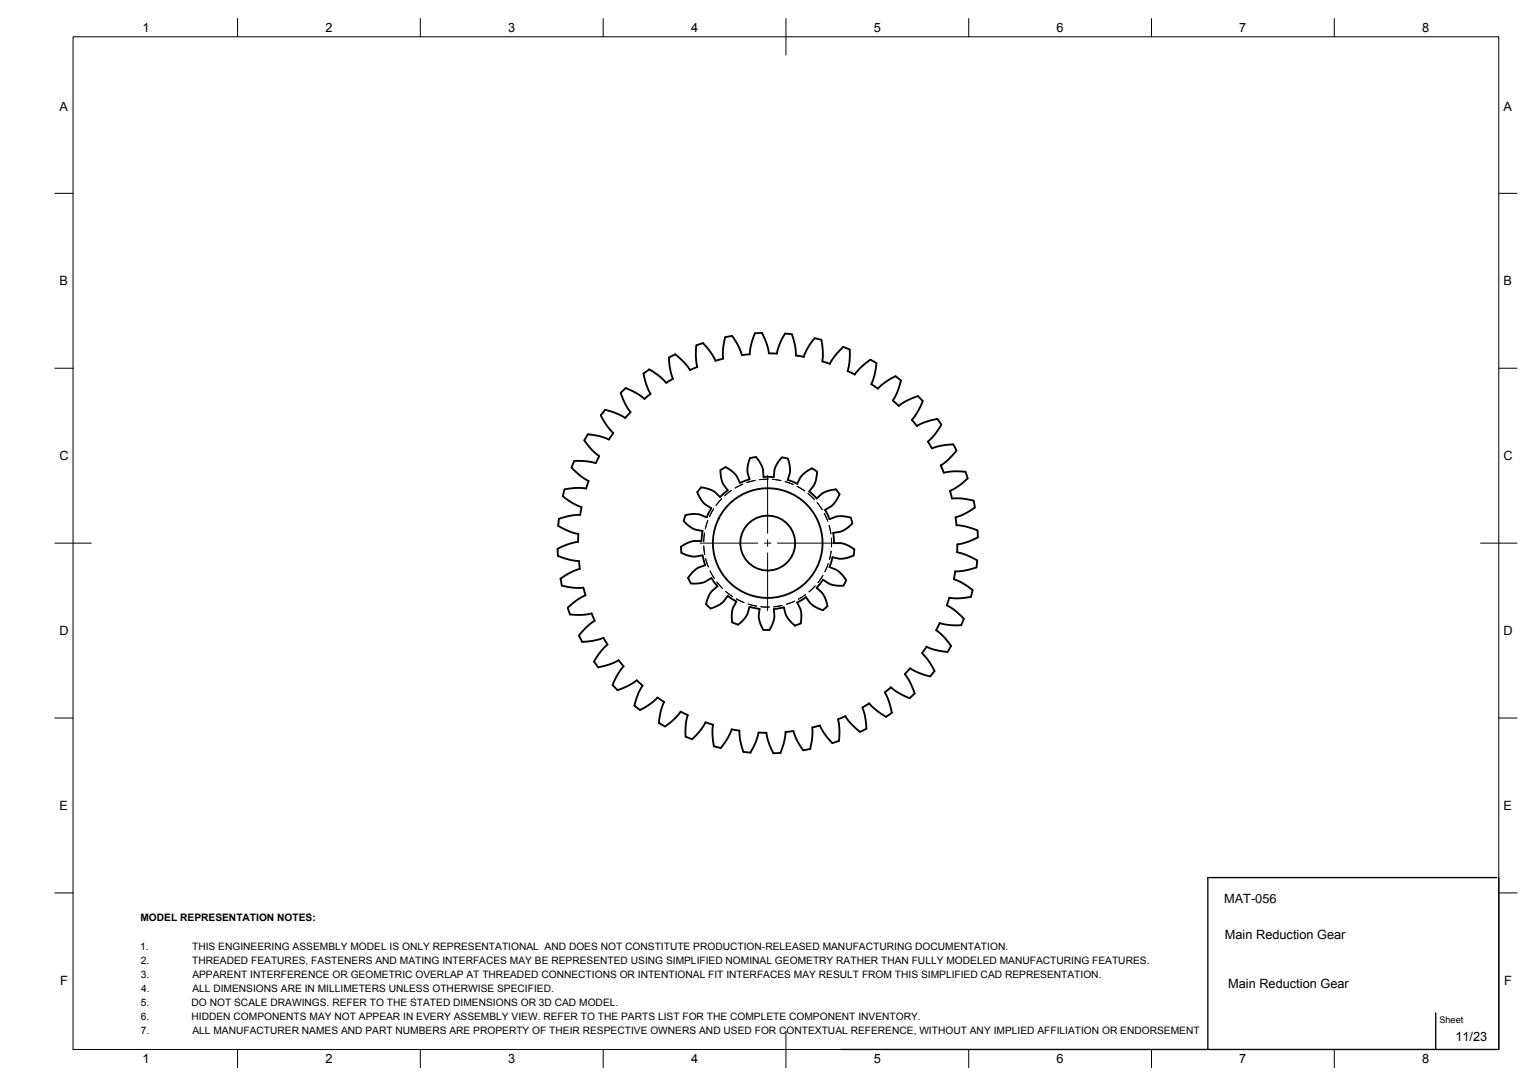
ISO-10303-21;
HEADER;
/* Generated by software containing ST-Developer
 * from STEP Tools, Inc. (www.steptools.com) 
 */

FILE_DESCRIPTION(
/* description */ (''),
/* implementation_level */ '2;1');

FILE_NAME(
/* name */ 'Main Reduction Gear.step',
/* time_stamp */ '2026-10-28T16:47:13+01:00',
/* author */ (''),
/* organization */ (''),
/* preprocessor_version */ 'ST-DEVELOPER v20.2',
/* originating_system */ 'Autodesk Translation Framework v15.17.0.0',
/* authorisation */ '');

FILE_SCHEMA (('AUTOMOTIVE_DESIGN { 1 0 10303 214 3 1 1 }'));
ENDSEC;

DATA;
#10=MECHANICAL_DESIGN_GEOMETRIC_PRESENTATION_REPRESENTATION('',(#4576,#4577),#459242);
#4412=SHAPE_REPRESENTATION_RELATIONSHIP('SRR','None',#459337,#4433);
#4433=ADVANCED_BREP_SHAPE_REPRESENTATION('',(#4456,#4457),#459226);
#4456=MANIFOLD_SOLID_BREP('Gear44',#94634);
#4457=MANIFOLD_SOLID_BREP('Gear17',#94635);
#4576=STYLED_ITEM('',(#459519),#4456);
#4577=STYLED_ITEM('',(#459519),#4457);
#5187=FACE_BOUND('',#13996,.T.);
#5188=FACE_BOUND('',#14004,.T.);
#5189=FACE_BOUND('',#14010,.T.);
#5190=FACE_BOUND('',#14013,.T.);
#5191=FACE_BOUND('',#14066,.T.);
#5192=FACE_BOUND('',#14120,.T.);
#5608=PLANE('',#98688);
#5609=PLANE('',#98701);
#5610=PLANE('',#98708);
#5611=PLANE('',#98709);
#5612=PLANE('',#98710);
#5613=PLANE('',#98749);
#5614=PLANE('',#98752);
#5615=PLANE('',#98755);
#5616=PLANE('',#98758);
#5617=PLANE('',#98761);
#5618=PLANE('',#98764);
#5619=PLANE('',#98767);
#5620=PLANE('',#98770);
#5621=PLANE('',#98773);
#5622=PLANE('',#98776);
#5623=PLANE('',#98779);
#5624=PLANE('',#98782);
#5625=PLANE('',#98785);
#5626=PLANE('',#98788);
#5627=PLANE('',#98791);
#5628=PLANE('',#98794);
#5629=PLANE('',#98797);
#5630=PLANE('',#98800);
#5631=PLANE('',#98801);
#5632=PLANE('',#98819);
#5633=PLANE('',#98821);
#5634=PLANE('',#98823);
#5635=PLANE('',#98825);
#5636=PLANE('',#98826);
#5637=PLANE('',#98828);
#5638=PLANE('',#98829);
#5639=PLANE('',#98832);
#5640=PLANE('',#98834);
#5641=PLANE('',#98837);
#5642=PLANE('',#98838);
#5643=PLANE('',#98840);
#5644=PLANE('',#98841);
#5645=PLANE('',#98844);
#5646=PLANE('',#98846);
#5647=PLANE('',#98849);
#5648=PLANE('',#98850);
#5649=PLANE('',#98855);
#6215=B_SPLINE_SURFACE_WITH_KNOTS('',5,1,((#153547,#153548),(#153549,#153550),
(#153551,#153552),(#153553,#153554),(#153555,#153556),(#153557,#153558),
(#153559,#153560),(#153561,#153562),(#153563,#153564),(#153565,#153566),
(#153567,#153568),(#153569,#153570),(#153571,#153572),(#153573,#153574),
(#153575,#153576),(#153577,#153578),(#153579,#153580),(#153581,#153582),
(#153583,#153584),(#153585,#153586),(#153587,#153588),(#153589,#153590),
(#153591,#153592),(#153593,#153594),(#153595,#153596),(#153597,#153598),
(#153599,#153600),(#153601,#153602),(#153603,#153604),(#153605,#153606),
(#153607,#153608),(#153609,#153610),(#153611,#153612),(#153613,#153614),
(#153615,#153616),(#153617,#153618),(#153619,#153620),(#153621,#153622),
(#153623,#153624),(#153625,#153626),(#153627,#153628),(#153629,#153630),
(#153631,#153632),(#153633,#153634),(#153635,#153636),(#153637,#153638),
(#153639,#153640),(#153641,#153642),(#153643,#153644),(#153645,#153646),
(#153647,#153648),(#153649,#153650),(#153651,#153652),(#153653,#153654),
(#153655,#153656),(#153657,#153658),(#153659,#153660),(#153661,#153662),
(#153663,#153664),(#153665,#153666),(#153667,#153668),(#153669,#153670),
(#153671,#153672),(#153673,#153674),(#153675,#153676),(#153677,#153678),
(#153679,#153680),(#153681,#153682),(#153683,#153684),(#153685,#153686),
(#153687,#153688),(#153689,#153690),(#153691,#153692),(#153693,#153694),
(#153695,#153696),(#153697,#153698),(#153699,#153700),(#153701,#153702),
(#153703,#153704),(#153705,#153706),(#153707,#153708),(#153709,#153710),
(#153711,#153712),(#153713,#153714),(#153715,#153716),(#153717,#153718),
(#153719,#153720),(#153721,#153722),(#153723,#153724),(#153725,#153726),
(#153727,#153728),(#153729,#153730),(#153731,#153732),(#153733,#153734),
(#153735,#153736),(#153737,#153738),(#153739,#153740),(#153741,#153742),
(#153743,#153744),(#153745,#153746),(#153747,#153748),(#153749,#153750),
(#153751,#153752),(#153753,#153754),(#153755,#153756),(#153757,#153758),
(#153759,#153760),(#153761,#153762),(#153763,#153764),(#153765,#153766),
(#153767,#153768),(#153769,#153770),(#153771,#153772),(#153773,#153774),
(#153775,#153776),(#153777,#153778),(#153779,#153780),(#153781,#153782),
(#153783,#153784),(#153785,#153786),(#153787,#153788),(#153789,#153790),
(#153791,#153792),(#153793,#153794),(#153795,#153796),(#153797,#153798),
(#153799,#153800),(#153801,#153802),(#153803,#153804),(#153805,#153806),
(#153807,#153808),(#153809,#153810),(#153811,#153812),(#153813,#153814),
(#153815,#153816),(#153817,#153818),(#153819,#153820),(#153821,#153822),
(#153823,#153824),(#153825,#153826),(#153827,#153828),(#153829,#153830),
(#153831,#153832),(#153833,#153834),(#153835,#153836),(#153837,#153838),
(#153839,#153840),(#153841,#153842),(#153843,#153844),(#153845,#153846),
(#153847,#153848),(#153849,#153850),(#153851,#153852),(#153853,#153854),
(#153855,#153856),(#153857,#153858),(#153859,#153860),(#153861,#153862),
(#153863,#153864),(#153865,#153866),(#153867,#153868),(#153869,#153870),
(#153871,#153872),(#153873,#153874),(#153875,#153876),(#153877,#153878),
(#153879,#153880),(#153881,#153882),(#153883,#153884),(#153885,#153886),
(#153887,#153888),(#153889,#153890),(#153891,#153892),(#153893,#153894),
(#153895,#153896),(#153897,#153898),(#153899,#153900),(#153901,#153902),
(#153903,#153904),(#153905,#153906),(#153907,#153908),(#153909,#153910),
(#153911,#153912),(#153913,#153914),(#153915,#153916),(#153917,#153918),
(#153919,#153920),(#153921,#153922),(#153923,#153924),(#153925,#153926),
(#153927,#153928),(#153929,#153930),(#153931,#153932),(#153933,#153934),
(#153935,#153936),(#153937,#153938),(#153939,#153940),(#153941,#153942),
(#153943,#153944),(#153945,#153946),(#153947,#153948),(#153949,#153950),
(#153951,#153952),(#153953,#153954),(#153955,#153956),(#153957,#153958),
(#153959,#153960),(#153961,#153962),(#153963,#153964),(#153965,#153966),
(#153967,#153968),(#153969,#153970),(#153971,#153972),(#153973,#153974),
(#153975,#153976),(#153977,#153978),(#153979,#153980),(#153981,#153982),
(#153983,#153984),(#153985,#153986),(#153987,#153988),(#153989,#153990),
(#153991,#153992),(#153993,#153994),(#153995,#153996),(#153997,#153998),
(#153999,#154000),(#154001,#154002),(#154003,#154004),(#154005,#154006),
(#154007,#154008),(#154009,#154010),(#154011,#154012),(#154013,#154014),
(#154015,#154016),(#154017,#154018),(#154019,#154020),(#154021,#154022),
(#154023,#154024),(#154025,#154026),(#154027,#154028),(#154029,#154030),
(#154031,#154032),(#154033,#154034),(#154035,#154036),(#154037,#154038),
(#154039,#154040),(#154041,#154042),(#154043,#154044),(#154045,#154046),
(#154047,#154048),(#154049,#154050),(#154051,#154052),(#154053,#154054),
(#154055,#154056),(#154057,#154058),(#154059,#154060),(#154061,#154062),
(#154063,#154064),(#154065,#154066),(#154067,#154068),(#154069,#154070),
(#154071,#154072),(#154073,#154074),(#154075,#154076),(#154077,#154078),
(#154079,#154080),(#154081,#154082),(#154083,#154084),(#154085,#154086),
(#154087,#154088),(#154089,#154090),(#154091,#154092),(#154093,#154094),
(#154095,#154096),(#154097,#154098),(#154099,#154100),(#154101,#154102),
(#154103,#154104),(#154105,#154106),(#154107,#154108),(#154109,#154110),
(#154111,#154112),(#154113,#154114),(#154115,#154116),(#154117,#154118),
(#154119,#154120),(#154121,#154122),(#154123,#154124),(#154125,#154126),
(#154127,#154128),(#154129,#154130),(#154131,#154132),(#154133,#154134),
(#154135,#154136),(#154137,#154138),(#154139,#154140),(#154141,#154142),
(#154143,#154144),(#154145,#154146),(#154147,#154148),(#154149,#154150),
(#154151,#154152),(#154153,#154154),(#154155,#154156),(#154157,#154158),
(#154159,#154160),(#154161,#154162),(#154163,#154164),(#154165,#154166),
(#154167,#154168),(#154169,#154170),(#154171,#154172),(#154173,#154174),
(#154175,#154176),(#154177,#154178),(#154179,#154180),(#154181,#154182),
(#154183,#154184),(#154185,#154186),(#154187,#154188),(#154189,#154190),
(#154191,#154192),(#154193,#154194),(#154195,#154196),(#154197,#154198),
(#154199,#154200),(#154201,#154202),(#154203,#154204),(#154205,#154206),
(#154207,#154208),(#154209,#154210),(#154211,#154212),(#154213,#154214),
(#154215,#154216),(#154217,#154218),(#154219,#154220),(#154221,#154222),
(#154223,#154224),(#154225,#154226),(#154227,#154228),(#154229,#154230),
(#154231,#154232),(#154233,#154234),(#154235,#154236),(#154237,#154238),
(#154239,#154240),(#154241,#154242),(#154243,#154244),(#154245,#154246),
(#154247,#154248),(#154249,#154250),(#154251,#154252),(#154253,#154254),
(#154255,#154256),(#154257,#154258),(#154259,#154260),(#154261,#154262),
(#154263,#154264),(#154265,#154266),(#154267,#154268),(#154269,#154270),
(#154271,#154272),(#154273,#154274),(#154275,#154276),(#154277,#154278),
(#154279,#154280),(#154281,#154282),(#154283,#154284),(#154285,#154286),
(#154287,#154288),(#154289,#154290),(#154291,#154292),(#154293,#154294),
(#154295,#154296),(#154297,#154298),(#154299,#154300),(#154301,#154302),
(#154303,#154304),(#154305,#154306),(#154307,#154308),(#154309,#154310),
(#154311,#154312),(#154313,#154314),(#154315,#154316),(#154317,#154318),
(#154319,#154320),(#154321,#154322),(#154323,#154324),(#154325,#154326),
(#154327,#154328),(#154329,#154330),(#154331,#154332),(#154333,#154334),
(#154335,#154336),(#154337,#154338),(#154339,#154340),(#154341,#154342),
(#154343,#154344),(#154345,#154346),(#154347,#154348),(#154349,#154350),
(#154351,#154352),(#154353,#154354),(#154355,#154356),(#154357,#154358),
(#154359,#154360),(#154361,#154362),(#154363,#154364),(#154365,#154366),
(#154367,#154368),(#154369,#154370),(#154371,#154372),(#154373,#154374),
(#154375,#154376),(#154377,#154378),(#154379,#154380),(#154381,#154382),
(#154383,#154384),(#154385,#154386),(#154387,#154388),(#154389,#154390),
(#154391,#154392),(#154393,#154394),(#154395,#154396),(#154397,#154398),
(#154399,#154400),(#154401,#154402),(#154403,#154404),(#154405,#154406),
(#154407,#154408),(#154409,#154410),(#154411,#154412),(#154413,#154414),
(#154415,#154416),(#154417,#154418),(#154419,#154420),(#154421,#154422),
(#154423,#154424),(#154425,#154426),(#154427,#154428),(#154429,#154430),
(#154431,#154432),(#154433,#154434),(#154435,#154436),(#154437,#154438),
(#154439,#154440),(#154441,#154442),(#154443,#154444),(#154445,#154446),
(#154447,#154448),(#154449,#154450),(#154451,#154452),(#154453,#154454),
(#154455,#154456),(#154457,#154458),(#154459,#154460),(#154461,#154462),
(#154463,#154464),(#154465,#154466),(#154467,#154468),(#154469,#154470),
(#154471,#154472),(#154473,#154474),(#154475,#154476),(#154477,#154478),
(#154479,#154480),(#154481,#154482),(#154483,#154484),(#154485,#154486),
(#154487,#154488),(#154489,#154490)),.UNSPECIFIED.,.F.,.F.,.F.,(6,1,1,1,
1,1,1,1,1,1,1,1,1,1,1,1,1,1,1,1,1,1,1,1,1,1,1,1,1,1,1,1,1,1,1,1,1,1,1,1,
1,1,1,1,1,1,1,1,1,1,1,1,1,1,1,1,1,1,1,1,1,1,1,1,1,1,1,1,1,1,1,1,1,1,1,1,
1,1,1,1,1,1,1,1,1,1,1,1,1,1,1,1,1,1,1,1,1,1,1,1,1,1,1,1,1,1,1,1,1,1,1,1,
1,1,1,1,1,1,1,1,1,1,1,1,1,1,1,1,1,1,1,1,1,1,1,1,1,1,1,1,1,1,1,1,1,1,1,1,
1,1,1,1,1,1,1,1,1,1,1,1,1,1,1,1,1,1,1,1,1,1,1,1,1,1,1,1,1,1,1,1,1,1,1,1,
1,1,1,1,1,1,1,1,1,1,1,1,1,1,1,1,1,1,1,1,1,1,1,1,1,1,1,1,1,1,1,1,1,1,1,1,
1,1,1,1,1,1,1,1,1,1,1,1,1,1,1,1,1,1,1,1,1,1,1,1,1,1,1,1,1,1,1,1,1,1,1,1,
1,1,1,1,1,1,1,1,1,1,1,1,1,1,1,1,1,1,1,1,1,1,1,1,1,1,1,1,1,1,1,1,1,1,1,1,
1,1,1,1,1,1,1,1,1,1,1,1,1,1,1,1,1,1,1,1,1,1,1,1,1,1,1,1,1,1,1,1,1,1,1,1,
1,1,1,1,1,1,1,1,1,1,1,1,1,1,1,1,1,1,1,1,1,1,1,1,1,1,1,1,1,1,1,1,1,1,1,1,
1,1,1,1,1,1,1,1,1,1,1,1,1,1,1,1,1,1,1,1,1,1,1,1,1,1,1,1,1,1,1,1,1,1,1,1,
1,1,1,1,1,1,1,1,1,1,1,1,1,1,1,1,1,1,1,1,1,1,1,1,1,1,1,1,1,1,1,1,1,1,1,1,
1,1,1,1,1,1,1,1,1,1,1,1,1,1,1,1,1,1,1,1,1,1,1,1,1,1,1,1,1,1,1,6),(2,2),
(0.143172103,0.144954128,0.146788991,0.148623853,0.150458716,0.152293578,
0.15412844,0.155963303,0.157798165,0.159633028,0.16146789,0.163302752,0.165137615,
0.166972477,0.168807339,0.170642202,0.172477064,0.174311927,0.176146789,
0.177981651,0.179816514,0.181651376,0.183486239,0.185321101,0.187155963,
0.188990826,0.190825688,0.19266055,0.194495413,0.196330275,0.198165138,
0.2,0.201834862,0.203669725,0.205504587,0.20733945,0.209174312,0.211009174,
0.212844037,0.214678899,0.216513761,0.218348624,0.220183486,0.222018349,
0.223853211,0.225688073,0.227522936,0.229357798,0.231192661,0.233027523,
0.234862385,0.236697248,0.23853211,0.240366972,0.242201835,0.244036697,
0.24587156,0.247706422,0.249541284,0.251376147,0.253211009,0.255045872,
0.256880734,0.258715596,0.260550459,0.262385321,0.264220183,0.266055046,
0.267889908,0.269724771,0.271559633,0.273394495,0.275229358,0.27706422,
0.278899083,0.280733945,0.282568807,0.28440367,0.286238532,0.288073394,
0.289908257,0.291743119,0.293577982,0.295412844,0.297247706,0.299082569,
0.300917431,0.302752294,0.304587156,0.306422018,0.308256881,0.310091743,
0.311926606,0.313761468,0.31559633,0.317431193,0.319266055,0.321100917,
0.32293578,0.324770642,0.326605505,0.328440367,0.330275229,0.332110092,
0.333944954,0.335779817,0.337614679,0.339449541,0.341284404,0.343119266,
0.344954128,0.346788991,0.348623853,0.350458716,0.352293578,0.35412844,
0.355963303,0.357798165,0.359633028,0.36146789,0.363302752,0.365137615,
0.366972477,0.368807339,0.370642202,0.372477064,0.374311927,0.376146789,
0.377981651,0.379816514,0.381651376,0.383486239,0.385321101,0.387155963,
0.388990826,0.390825688,0.39266055,0.394495413,0.396330275,0.398165138,
0.4,0.401834862,0.403669725,0.405504587,0.40733945,0.409174312,0.411009174,
0.412844037,0.414678899,0.416513761,0.418348624,0.420183486,0.422018349,
0.423853211,0.425688073,0.427522936,0.429357798,0.431192661,0.433027523,
0.434862385,0.436697248,0.43853211,0.440366972,0.442201835,0.444036697,
0.44587156,0.447706422,0.449541284,0.451376147,0.453211009,0.455045872,
0.456880734,0.458715596,0.460550459,0.462385321,0.464220183,0.466055046,
0.467889908,0.469724771,0.471559633,0.473394495,0.475229358,0.47706422,
0.478899083,0.480733945,0.482568807,0.48440367,0.486238532,0.488073394,
0.489908257,0.491743119,0.493577982,0.495412844,0.497247706,0.499082569,
0.500917431,0.502752294,0.504587156,0.506422018,0.508256881,0.510091743,
0.511926606,0.513761468,0.51559633,0.517431193,0.519266055,0.521100917,
0.52293578,0.524770642,0.526605505,0.528440367,0.530275229,0.532110092,
0.533944954,0.535779817,0.537614679,0.539449541,0.541284404,0.543119266,
0.544954128,0.546788991,0.548623853,0.550458716,0.552293578,0.55412844,
0.555963303,0.557798165,0.559633028,0.56146789,0.563302752,0.565137615,
0.566972477,0.568807339,0.570642202,0.572477064,0.574311927,0.576146789,
0.577981651,0.579816514,0.581651376,0.583486239,0.585321101,0.587155963,
0.588990826,0.590825688,0.59266055,0.594495413,0.596330275,0.598165138,
0.6,0.601834862,0.603669725,0.605504587,0.60733945,0.609174312,0.611009174,
0.612844037,0.614678899,0.616513761,0.618348624,0.620183486,0.622018349,
0.623853211,0.625688073,0.627522936,0.629357798,0.631192661,0.633027523,
0.634862385,0.636697248,0.63853211,0.640366972,0.642201835,0.644036697,
0.64587156,0.647706422,0.649541284,0.651376147,0.653211009,0.655045872,
0.656880734,0.658715596,0.660550459,0.662385321,0.664220183,0.666055046,
0.667889908,0.669724771,0.671559633,0.673394495,0.675229358,0.67706422,
0.678899083,0.680733945,0.682568807,0.68440367,0.686238532,0.688073394,
0.689908257,0.691743119,0.693577982,0.695412844,0.697247706,0.699082569,
0.700917431,0.702752294,0.704587156,0.706422018,0.708256881,0.710091743,
0.711926606,0.713761468,0.71559633,0.717431193,0.719266055,0.721100917,
0.72293578,0.724770642,0.726605505,0.728440367,0.730275229,0.732110092,
0.733944954,0.735779817,0.737614679,0.739449541,0.741284404,0.743119266,
0.744954128,0.746788991,0.748623853,0.750458716,0.752293578,0.75412844,
0.755963303,0.757798165,0.759633028,0.76146789,0.763302752,0.765137615,
0.766972477,0.768807339,0.770642202,0.772477064,0.774311927,0.776146789,
0.777981651,0.779816514,0.781651376,0.783486239,0.785321101,0.787155963,
0.788990826,0.790825688,0.79266055,0.794495413,0.796330275,0.798165138,
0.8,0.801834862,0.803669725,0.805504587,0.80733945,0.809174312,0.811009174,
0.812844037,0.814678899,0.816513761,0.818348624,0.820183486,0.822018349,
0.823853211,0.825688073,0.827522936,0.829357798,0.831192661,0.833027523,
0.834862385,0.836697248,0.83853211,0.840366972,0.842201835,0.844036697,
0.84587156,0.847706422,0.849541284,0.851376147,0.853211009,0.855045872,
0.856880734,0.858715596,0.860550459,0.862385321,0.864220183,0.866055046,
0.867889908,0.869724771,0.871559633,0.873394495,0.875229358,0.87706422,
0.878899083,0.880733945,0.882568807,0.88440367,0.886238532,0.888073394,
0.889908257,0.891743119,0.893577982,0.895412844,0.897247706,0.899082569,
0.900917431,0.902752294,0.904587156,0.906422018,0.908256881,0.910091743,
0.911926606,0.913761468,0.91559633,0.917431193,0.919266055,0.921100917,
0.92293578,0.924770642,0.926605505,0.928440367,0.930275229,0.932110092,
0.933944954,0.935779817,0.937614679,0.939449541,0.941284404,0.943119266,
0.944954128,0.946788991,0.948623853,0.950458716,0.952293578,0.95412844,
0.955963303,0.957798165,0.959633028,0.96146789,0.963302752,0.965137615,
0.966972477,0.968807339,0.970642202,0.972477064,0.974311927,0.976146789,
0.977981651,0.979816514,0.981651376,0.983486239,0.985321101,0.987155963,
0.988990826,0.990825688,0.99266055,0.994495413,0.996330275,0.998165138,
1.),(0.,0.36),.UNSPECIFIED.);
#6216=B_SPLINE_SURFACE_WITH_KNOTS('',5,1,((#155436,#155437),(#155438,#155439),
(#155440,#155441),(#155442,#155443),(#155444,#155445),(#155446,#155447),
(#155448,#155449),(#155450,#155451),(#155452,#155453),(#155454,#155455),
(#155456,#155457),(#155458,#155459),(#155460,#155461),(#155462,#155463),
(#155464,#155465),(#155466,#155467),(#155468,#155469),(#155470,#155471),
(#155472,#155473),(#155474,#155475),(#155476,#155477),(#155478,#155479),
(#155480,#155481),(#155482,#155483),(#155484,#155485),(#155486,#155487),
(#155488,#155489),(#155490,#155491),(#155492,#155493),(#155494,#155495),
(#155496,#155497),(#155498,#155499),(#155500,#155501),(#155502,#155503),
(#155504,#155505),(#155506,#155507),(#155508,#155509),(#155510,#155511),
(#155512,#155513),(#155514,#155515),(#155516,#155517),(#155518,#155519),
(#155520,#155521),(#155522,#155523),(#155524,#155525),(#155526,#155527),
(#155528,#155529),(#155530,#155531),(#155532,#155533),(#155534,#155535),
(#155536,#155537),(#155538,#155539),(#155540,#155541),(#155542,#155543),
(#155544,#155545),(#155546,#155547),(#155548,#155549),(#155550,#155551),
(#155552,#155553),(#155554,#155555),(#155556,#155557),(#155558,#155559),
(#155560,#155561),(#155562,#155563),(#155564,#155565),(#155566,#155567),
(#155568,#155569),(#155570,#155571),(#155572,#155573),(#155574,#155575),
(#155576,#155577),(#155578,#155579),(#155580,#155581),(#155582,#155583),
(#155584,#155585),(#155586,#155587),(#155588,#155589),(#155590,#155591),
(#155592,#155593),(#155594,#155595),(#155596,#155597),(#155598,#155599),
(#155600,#155601),(#155602,#155603),(#155604,#155605),(#155606,#155607),
(#155608,#155609),(#155610,#155611),(#155612,#155613),(#155614,#155615),
(#155616,#155617),(#155618,#155619),(#155620,#155621),(#155622,#155623),
(#155624,#155625),(#155626,#155627),(#155628,#155629),(#155630,#155631),
(#155632,#155633),(#155634,#155635),(#155636,#155637),(#155638,#155639),
(#155640,#155641),(#155642,#155643),(#155644,#155645),(#155646,#155647),
(#155648,#155649),(#155650,#155651),(#155652,#155653),(#155654,#155655),
(#155656,#155657),(#155658,#155659),(#155660,#155661),(#155662,#155663),
(#155664,#155665),(#155666,#155667),(#155668,#155669),(#155670,#155671),
(#155672,#155673),(#155674,#155675),(#155676,#155677),(#155678,#155679),
(#155680,#155681),(#155682,#155683),(#155684,#155685),(#155686,#155687),
(#155688,#155689),(#155690,#155691),(#155692,#155693),(#155694,#155695),
(#155696,#155697),(#155698,#155699),(#155700,#155701),(#155702,#155703),
(#155704,#155705),(#155706,#155707),(#155708,#155709),(#155710,#155711),
(#155712,#155713),(#155714,#155715),(#155716,#155717),(#155718,#155719),
(#155720,#155721),(#155722,#155723),(#155724,#155725),(#155726,#155727),
(#155728,#155729),(#155730,#155731),(#155732,#155733),(#155734,#155735),
(#155736,#155737),(#155738,#155739),(#155740,#155741),(#155742,#155743),
(#155744,#155745),(#155746,#155747),(#155748,#155749),(#155750,#155751),
(#155752,#155753),(#155754,#155755),(#155756,#155757),(#155758,#155759),
(#155760,#155761),(#155762,#155763),(#155764,#155765),(#155766,#155767),
(#155768,#155769),(#155770,#155771),(#155772,#155773),(#155774,#155775),
(#155776,#155777),(#155778,#155779),(#155780,#155781),(#155782,#155783),
(#155784,#155785),(#155786,#155787),(#155788,#155789),(#155790,#155791),
(#155792,#155793),(#155794,#155795),(#155796,#155797),(#155798,#155799),
(#155800,#155801),(#155802,#155803),(#155804,#155805),(#155806,#155807),
(#155808,#155809),(#155810,#155811),(#155812,#155813),(#155814,#155815),
(#155816,#155817),(#155818,#155819),(#155820,#155821),(#155822,#155823),
(#155824,#155825),(#155826,#155827),(#155828,#155829),(#155830,#155831),
(#155832,#155833),(#155834,#155835),(#155836,#155837),(#155838,#155839),
(#155840,#155841),(#155842,#155843),(#155844,#155845),(#155846,#155847),
(#155848,#155849),(#155850,#155851),(#155852,#155853),(#155854,#155855),
(#155856,#155857),(#155858,#155859),(#155860,#155861),(#155862,#155863),
(#155864,#155865),(#155866,#155867),(#155868,#155869),(#155870,#155871),
(#155872,#155873),(#155874,#155875),(#155876,#155877),(#155878,#155879),
(#155880,#155881),(#155882,#155883),(#155884,#155885),(#155886,#155887),
(#155888,#155889),(#155890,#155891),(#155892,#155893),(#155894,#155895),
(#155896,#155897),(#155898,#155899),(#155900,#155901),(#155902,#155903),
(#155904,#155905),(#155906,#155907),(#155908,#155909),(#155910,#155911),
(#155912,#155913),(#155914,#155915),(#155916,#155917),(#155918,#155919),
(#155920,#155921),(#155922,#155923),(#155924,#155925),(#155926,#155927),
(#155928,#155929),(#155930,#155931),(#155932,#155933),(#155934,#155935),
(#155936,#155937),(#155938,#155939),(#155940,#155941),(#155942,#155943),
(#155944,#155945),(#155946,#155947),(#155948,#155949),(#155950,#155951),
(#155952,#155953),(#155954,#155955),(#155956,#155957),(#155958,#155959),
(#155960,#155961),(#155962,#155963),(#155964,#155965),(#155966,#155967),
(#155968,#155969),(#155970,#155971),(#155972,#155973),(#155974,#155975),
(#155976,#155977),(#155978,#155979),(#155980,#155981),(#155982,#155983),
(#155984,#155985),(#155986,#155987),(#155988,#155989),(#155990,#155991),
(#155992,#155993),(#155994,#155995),(#155996,#155997),(#155998,#155999),
(#156000,#156001),(#156002,#156003),(#156004,#156005),(#156006,#156007),
(#156008,#156009),(#156010,#156011),(#156012,#156013),(#156014,#156015),
(#156016,#156017),(#156018,#156019),(#156020,#156021),(#156022,#156023),
(#156024,#156025),(#156026,#156027),(#156028,#156029),(#156030,#156031),
(#156032,#156033),(#156034,#156035),(#156036,#156037),(#156038,#156039),
(#156040,#156041),(#156042,#156043),(#156044,#156045),(#156046,#156047),
(#156048,#156049),(#156050,#156051),(#156052,#156053),(#156054,#156055),
(#156056,#156057),(#156058,#156059),(#156060,#156061),(#156062,#156063),
(#156064,#156065),(#156066,#156067),(#156068,#156069),(#156070,#156071),
(#156072,#156073),(#156074,#156075),(#156076,#156077),(#156078,#156079),
(#156080,#156081),(#156082,#156083),(#156084,#156085),(#156086,#156087),
(#156088,#156089),(#156090,#156091),(#156092,#156093),(#156094,#156095),
(#156096,#156097),(#156098,#156099),(#156100,#156101),(#156102,#156103),
(#156104,#156105),(#156106,#156107),(#156108,#156109),(#156110,#156111),
(#156112,#156113),(#156114,#156115),(#156116,#156117),(#156118,#156119),
(#156120,#156121),(#156122,#156123),(#156124,#156125),(#156126,#156127),
(#156128,#156129),(#156130,#156131),(#156132,#156133),(#156134,#156135),
(#156136,#156137),(#156138,#156139),(#156140,#156141),(#156142,#156143),
(#156144,#156145),(#156146,#156147),(#156148,#156149),(#156150,#156151),
(#156152,#156153),(#156154,#156155),(#156156,#156157),(#156158,#156159),
(#156160,#156161),(#156162,#156163),(#156164,#156165),(#156166,#156167),
(#156168,#156169),(#156170,#156171),(#156172,#156173),(#156174,#156175),
(#156176,#156177),(#156178,#156179),(#156180,#156181),(#156182,#156183),
(#156184,#156185),(#156186,#156187),(#156188,#156189),(#156190,#156191),
(#156192,#156193),(#156194,#156195),(#156196,#156197),(#156198,#156199),
(#156200,#156201),(#156202,#156203),(#156204,#156205),(#156206,#156207),
(#156208,#156209),(#156210,#156211),(#156212,#156213),(#156214,#156215),
(#156216,#156217),(#156218,#156219),(#156220,#156221),(#156222,#156223),
(#156224,#156225),(#156226,#156227),(#156228,#156229),(#156230,#156231),
(#156232,#156233),(#156234,#156235),(#156236,#156237),(#156238,#156239),
(#156240,#156241),(#156242,#156243),(#156244,#156245),(#156246,#156247),
(#156248,#156249),(#156250,#156251),(#156252,#156253),(#156254,#156255),
(#156256,#156257),(#156258,#156259),(#156260,#156261),(#156262,#156263),
(#156264,#156265),(#156266,#156267),(#156268,#156269),(#156270,#156271),
(#156272,#156273),(#156274,#156275),(#156276,#156277),(#156278,#156279),
(#156280,#156281),(#156282,#156283),(#156284,#156285),(#156286,#156287),
(#156288,#156289),(#156290,#156291),(#156292,#156293),(#156294,#156295),
(#156296,#156297),(#156298,#156299),(#156300,#156301),(#156302,#156303),
(#156304,#156305),(#156306,#156307),(#156308,#156309),(#156310,#156311),
(#156312,#156313),(#156314,#156315),(#156316,#156317),(#156318,#156319),
(#156320,#156321),(#156322,#156323),(#156324,#156325),(#156326,#156327),
(#156328,#156329),(#156330,#156331),(#156332,#156333),(#156334,#156335),
(#156336,#156337),(#156338,#156339),(#156340,#156341),(#156342,#156343),
(#156344,#156345),(#156346,#156347),(#156348,#156349),(#156350,#156351),
(#156352,#156353),(#156354,#156355),(#156356,#156357),(#156358,#156359),
(#156360,#156361),(#156362,#156363),(#156364,#156365),(#156366,#156367),
(#156368,#156369),(#156370,#156371),(#156372,#156373),(#156374,#156375),
(#156376,#156377),(#156378,#156379)),.UNSPECIFIED.,.F.,.F.,.F.,(6,1,1,1,
1,1,1,1,1,1,1,1,1,1,1,1,1,1,1,1,1,1,1,1,1,1,1,1,1,1,1,1,1,1,1,1,1,1,1,1,
1,1,1,1,1,1,1,1,1,1,1,1,1,1,1,1,1,1,1,1,1,1,1,1,1,1,1,1,1,1,1,1,1,1,1,1,
1,1,1,1,1,1,1,1,1,1,1,1,1,1,1,1,1,1,1,1,1,1,1,1,1,1,1,1,1,1,1,1,1,1,1,1,
1,1,1,1,1,1,1,1,1,1,1,1,1,1,1,1,1,1,1,1,1,1,1,1,1,1,1,1,1,1,1,1,1,1,1,1,
1,1,1,1,1,1,1,1,1,1,1,1,1,1,1,1,1,1,1,1,1,1,1,1,1,1,1,1,1,1,1,1,1,1,1,1,
1,1,1,1,1,1,1,1,1,1,1,1,1,1,1,1,1,1,1,1,1,1,1,1,1,1,1,1,1,1,1,1,1,1,1,1,
1,1,1,1,1,1,1,1,1,1,1,1,1,1,1,1,1,1,1,1,1,1,1,1,1,1,1,1,1,1,1,1,1,1,1,1,
1,1,1,1,1,1,1,1,1,1,1,1,1,1,1,1,1,1,1,1,1,1,1,1,1,1,1,1,1,1,1,1,1,1,1,1,
1,1,1,1,1,1,1,1,1,1,1,1,1,1,1,1,1,1,1,1,1,1,1,1,1,1,1,1,1,1,1,1,1,1,1,1,
1,1,1,1,1,1,1,1,1,1,1,1,1,1,1,1,1,1,1,1,1,1,1,1,1,1,1,1,1,1,1,1,1,1,1,1,
1,1,1,1,1,1,1,1,1,1,1,1,1,1,1,1,1,1,1,1,1,1,1,1,1,1,1,1,1,1,1,1,1,1,1,1,
1,1,1,1,1,1,1,1,1,1,1,1,1,1,1,1,1,1,1,1,1,1,1,1,1,1,1,1,1,1,1,1,1,1,1,1,
1,1,1,1,1,1,1,1,1,1,1,1,1,1,1,1,1,1,1,1,1,1,1,1,1,1,1,1,1,1,1,6),(2,2),
(-1.,-0.998165138,-0.996330275,-0.994495413,-0.99266055,-0.990825688,-0.988990826,
-0.987155963,-0.985321101,-0.983486239,-0.981651376,-0.979816514,-0.977981651,
-0.976146789,-0.974311927,-0.972477064,-0.970642202,-0.968807339,-0.966972477,
-0.965137615,-0.963302752,-0.96146789,-0.959633028,-0.957798165,-0.955963303,
-0.95412844,-0.952293578,-0.950458716,-0.948623853,-0.946788991,-0.944954128,
-0.943119266,-0.941284404,-0.939449541,-0.937614679,-0.935779817,-0.933944954,
-0.932110092,-0.930275229,-0.928440367,-0.926605505,-0.924770642,-0.92293578,
-0.921100917,-0.919266055,-0.917431193,-0.91559633,-0.913761468,-0.911926606,
-0.910091743,-0.908256881,-0.906422018,-0.904587156,-0.902752294,-0.900917431,
-0.899082569,-0.897247706,-0.895412844,-0.893577982,-0.891743119,-0.889908257,
-0.888073394,-0.886238532,-0.88440367,-0.882568807,-0.880733945,-0.878899083,
-0.87706422,-0.875229358,-0.873394495,-0.871559633,-0.869724771,-0.867889908,
-0.866055046,-0.864220183,-0.862385321,-0.860550459,-0.858715596,-0.856880734,
-0.855045872,-0.853211009,-0.851376147,-0.849541284,-0.847706422,-0.84587156,
-0.844036697,-0.842201835,-0.840366972,-0.83853211,-0.836697248,-0.834862385,
-0.833027523,-0.831192661,-0.829357798,-0.827522936,-0.825688073,-0.823853211,
-0.822018349,-0.820183486,-0.818348624,-0.816513761,-0.814678899,-0.812844037,
-0.811009174,-0.809174312,-0.80733945,-0.805504587,-0.803669725,-0.801834862,
-0.8,-0.798165138,-0.796330275,-0.794495413,-0.79266055,-0.790825688,-0.788990826,
-0.787155963,-0.785321101,-0.783486239,-0.781651376,-0.779816514,-0.777981651,
-0.776146789,-0.774311927,-0.772477064,-0.770642202,-0.768807339,-0.766972477,
-0.765137615,-0.763302752,-0.76146789,-0.759633028,-0.757798165,-0.755963303,
-0.75412844,-0.752293578,-0.750458716,-0.748623853,-0.746788991,-0.744954128,
-0.743119266,-0.741284404,-0.739449541,-0.737614679,-0.735779817,-0.733944954,
-0.732110092,-0.730275229,-0.728440367,-0.726605505,-0.724770642,-0.72293578,
-0.721100917,-0.719266055,-0.717431193,-0.71559633,-0.713761468,-0.711926606,
-0.710091743,-0.708256881,-0.706422018,-0.704587156,-0.702752294,-0.700917431,
-0.699082569,-0.697247706,-0.695412844,-0.693577982,-0.691743119,-0.689908257,
-0.688073394,-0.686238532,-0.68440367,-0.682568807,-0.680733945,-0.678899083,
-0.67706422,-0.675229358,-0.673394495,-0.671559633,-0.669724771,-0.667889908,
-0.666055046,-0.664220183,-0.662385321,-0.660550459,-0.658715596,-0.656880734,
-0.655045872,-0.653211009,-0.651376147,-0.649541284,-0.647706422,-0.64587156,
-0.644036697,-0.642201835,-0.640366972,-0.63853211,-0.636697248,-0.634862385,
-0.633027523,-0.631192661,-0.629357798,-0.627522936,-0.625688073,-0.623853211,
-0.622018349,-0.620183486,-0.618348624,-0.616513761,-0.614678899,-0.612844037,
-0.611009174,-0.609174312,-0.60733945,-0.605504587,-0.603669725,-0.601834862,
-0.6,-0.598165138,-0.596330275,-0.594495413,-0.59266055,-0.590825688,-0.588990826,
-0.587155963,-0.585321101,-0.583486239,-0.581651376,-0.579816514,-0.577981651,
-0.576146789,-0.574311927,-0.572477064,-0.570642202,-0.568807339,-0.566972477,
-0.565137615,-0.563302752,-0.56146789,-0.559633028,-0.557798165,-0.555963303,
-0.55412844,-0.552293578,-0.550458716,-0.548623853,-0.546788991,-0.544954128,
-0.543119266,-0.541284404,-0.539449541,-0.537614679,-0.535779817,-0.533944954,
-0.532110092,-0.530275229,-0.528440367,-0.526605505,-0.524770642,-0.52293578,
-0.521100917,-0.519266055,-0.517431193,-0.51559633,-0.513761468,-0.511926606,
-0.510091743,-0.508256881,-0.506422018,-0.504587156,-0.502752294,-0.500917431,
-0.499082569,-0.497247706,-0.495412844,-0.493577982,-0.491743119,-0.489908257,
-0.488073394,-0.486238532,-0.48440367,-0.482568807,-0.480733945,-0.478899083,
-0.47706422,-0.475229358,-0.473394495,-0.471559633,-0.469724771,-0.467889908,
-0.466055046,-0.464220183,-0.462385321,-0.460550459,-0.458715596,-0.456880734,
-0.455045872,-0.453211009,-0.451376147,-0.449541284,-0.447706422,-0.44587156,
-0.444036697,-0.442201835,-0.440366972,-0.43853211,-0.436697248,-0.434862385,
-0.433027523,-0.431192661,-0.429357798,-0.427522936,-0.425688073,-0.423853211,
-0.422018349,-0.420183486,-0.418348624,-0.416513761,-0.414678899,-0.412844037,
-0.411009174,-0.409174312,-0.40733945,-0.405504587,-0.403669725,-0.401834862,
-0.4,-0.398165138,-0.396330275,-0.394495413,-0.39266055,-0.390825688,-0.388990826,
-0.387155963,-0.385321101,-0.383486239,-0.381651376,-0.379816514,-0.377981651,
-0.376146789,-0.374311927,-0.372477064,-0.370642202,-0.368807339,-0.366972477,
-0.365137615,-0.363302752,-0.36146789,-0.359633028,-0.357798165,-0.355963303,
-0.35412844,-0.352293578,-0.350458716,-0.348623853,-0.346788991,-0.344954128,
-0.343119266,-0.341284404,-0.339449541,-0.337614679,-0.335779817,-0.333944954,
-0.332110092,-0.330275229,-0.328440367,-0.326605505,-0.324770642,-0.32293578,
-0.321100917,-0.319266055,-0.317431193,-0.31559633,-0.313761468,-0.311926606,
-0.310091743,-0.308256881,-0.306422018,-0.304587156,-0.302752294,-0.300917431,
-0.299082569,-0.297247706,-0.295412844,-0.293577982,-0.291743119,-0.289908257,
-0.288073394,-0.286238532,-0.28440367,-0.282568807,-0.280733945,-0.278899083,
-0.27706422,-0.275229358,-0.273394495,-0.271559633,-0.269724771,-0.267889908,
-0.266055046,-0.264220183,-0.262385321,-0.260550459,-0.258715596,-0.256880734,
-0.255045872,-0.253211009,-0.251376147,-0.249541284,-0.247706422,-0.24587156,
-0.244036697,-0.242201835,-0.240366972,-0.23853211,-0.236697248,-0.234862385,
-0.233027523,-0.231192661,-0.229357798,-0.227522936,-0.225688073,-0.223853211,
-0.222018349,-0.220183486,-0.218348624,-0.216513761,-0.214678899,-0.212844037,
-0.211009174,-0.209174312,-0.20733945,-0.205504587,-0.203669725,-0.201834862,
-0.2,-0.198165138,-0.196330275,-0.194495413,-0.19266055,-0.190825688,-0.188990826,
-0.187155963,-0.185321101,-0.183486239,-0.181651376,-0.179816514,-0.177981651,
-0.176146789,-0.174311927,-0.172477064,-0.170642202,-0.168807339,-0.166972477,
-0.165137615,-0.163302752,-0.16146789,-0.159633028,-0.157798165,-0.155963303,
-0.15412844,-0.152293578,-0.150458716,-0.148623853,-0.146788991,-0.144954128,
-0.143172103),(0.,0.36),.UNSPECIFIED.);
#6217=B_SPLINE_SURFACE_WITH_KNOTS('',5,1,((#157342,#157343),(#157344,#157345),
(#157346,#157347),(#157348,#157349),(#157350,#157351),(#157352,#157353),
(#157354,#157355),(#157356,#157357),(#157358,#157359),(#157360,#157361),
(#157362,#157363),(#157364,#157365),(#157366,#157367),(#157368,#157369),
(#157370,#157371),(#157372,#157373),(#157374,#157375),(#157376,#157377),
(#157378,#157379),(#157380,#157381),(#157382,#157383),(#157384,#157385),
(#157386,#157387),(#157388,#157389),(#157390,#157391),(#157392,#157393),
(#157394,#157395),(#157396,#157397),(#157398,#157399),(#157400,#157401),
(#157402,#157403),(#157404,#157405),(#157406,#157407),(#157408,#157409),
(#157410,#157411),(#157412,#157413),(#157414,#157415),(#157416,#157417),
(#157418,#157419),(#157420,#157421),(#157422,#157423),(#157424,#157425),
(#157426,#157427),(#157428,#157429),(#157430,#157431),(#157432,#157433),
(#157434,#157435),(#157436,#157437),(#157438,#157439),(#157440,#157441),
(#157442,#157443),(#157444,#157445),(#157446,#157447),(#157448,#157449),
(#157450,#157451),(#157452,#157453),(#157454,#157455),(#157456,#157457),
(#157458,#157459),(#157460,#157461),(#157462,#157463),(#157464,#157465),
(#157466,#157467),(#157468,#157469),(#157470,#157471),(#157472,#157473),
(#157474,#157475),(#157476,#157477),(#157478,#157479),(#157480,#157481),
(#157482,#157483),(#157484,#157485),(#157486,#157487),(#157488,#157489),
(#157490,#157491),(#157492,#157493),(#157494,#157495),(#157496,#157497),
(#157498,#157499),(#157500,#157501),(#157502,#157503),(#157504,#157505),
(#157506,#157507),(#157508,#157509),(#157510,#157511),(#157512,#157513),
(#157514,#157515),(#157516,#157517),(#157518,#157519),(#157520,#157521),
(#157522,#157523),(#157524,#157525),(#157526,#157527),(#157528,#157529),
(#157530,#157531),(#157532,#157533),(#157534,#157535),(#157536,#157537),
(#157538,#157539),(#157540,#157541),(#157542,#157543),(#157544,#157545),
(#157546,#157547),(#157548,#157549),(#157550,#157551),(#157552,#157553),
(#157554,#157555),(#157556,#157557),(#157558,#157559),(#157560,#157561),
(#157562,#157563),(#157564,#157565),(#157566,#157567),(#157568,#157569),
(#157570,#157571),(#157572,#157573),(#157574,#157575),(#157576,#157577),
(#157578,#157579),(#157580,#157581),(#157582,#157583),(#157584,#157585),
(#157586,#157587),(#157588,#157589),(#157590,#157591),(#157592,#157593),
(#157594,#157595),(#157596,#157597),(#157598,#157599),(#157600,#157601),
(#157602,#157603),(#157604,#157605),(#157606,#157607),(#157608,#157609),
(#157610,#157611),(#157612,#157613),(#157614,#157615),(#157616,#157617),
(#157618,#157619),(#157620,#157621),(#157622,#157623),(#157624,#157625),
(#157626,#157627),(#157628,#157629),(#157630,#157631),(#157632,#157633),
(#157634,#157635),(#157636,#157637),(#157638,#157639),(#157640,#157641),
(#157642,#157643),(#157644,#157645),(#157646,#157647),(#157648,#157649),
(#157650,#157651),(#157652,#157653),(#157654,#157655),(#157656,#157657),
(#157658,#157659),(#157660,#157661),(#157662,#157663),(#157664,#157665),
(#157666,#157667),(#157668,#157669),(#157670,#157671),(#157672,#157673),
(#157674,#157675),(#157676,#157677),(#157678,#157679),(#157680,#157681),
(#157682,#157683),(#157684,#157685),(#157686,#157687),(#157688,#157689),
(#157690,#157691),(#157692,#157693),(#157694,#157695),(#157696,#157697),
(#157698,#157699),(#157700,#157701),(#157702,#157703),(#157704,#157705),
(#157706,#157707),(#157708,#157709),(#157710,#157711),(#157712,#157713),
(#157714,#157715),(#157716,#157717),(#157718,#157719),(#157720,#157721),
(#157722,#157723),(#157724,#157725),(#157726,#157727),(#157728,#157729),
(#157730,#157731),(#157732,#157733),(#157734,#157735),(#157736,#157737),
(#157738,#157739),(#157740,#157741),(#157742,#157743),(#157744,#157745),
(#157746,#157747),(#157748,#157749),(#157750,#157751),(#157752,#157753),
(#157754,#157755),(#157756,#157757),(#157758,#157759),(#157760,#157761),
(#157762,#157763),(#157764,#157765),(#157766,#157767),(#157768,#157769),
(#157770,#157771),(#157772,#157773),(#157774,#157775),(#157776,#157777),
(#157778,#157779),(#157780,#157781),(#157782,#157783),(#157784,#157785),
(#157786,#157787),(#157788,#157789),(#157790,#157791),(#157792,#157793),
(#157794,#157795),(#157796,#157797),(#157798,#157799),(#157800,#157801),
(#157802,#157803),(#157804,#157805),(#157806,#157807),(#157808,#157809),
(#157810,#157811),(#157812,#157813),(#157814,#157815),(#157816,#157817),
(#157818,#157819),(#157820,#157821),(#157822,#157823),(#157824,#157825),
(#157826,#157827),(#157828,#157829),(#157830,#157831),(#157832,#157833),
(#157834,#157835),(#157836,#157837),(#157838,#157839),(#157840,#157841),
(#157842,#157843),(#157844,#157845),(#157846,#157847),(#157848,#157849),
(#157850,#157851),(#157852,#157853),(#157854,#157855),(#157856,#157857),
(#157858,#157859),(#157860,#157861),(#157862,#157863),(#157864,#157865),
(#157866,#157867),(#157868,#157869),(#157870,#157871),(#157872,#157873),
(#157874,#157875),(#157876,#157877),(#157878,#157879),(#157880,#157881),
(#157882,#157883),(#157884,#157885),(#157886,#157887),(#157888,#157889),
(#157890,#157891),(#157892,#157893),(#157894,#157895),(#157896,#157897),
(#157898,#157899),(#157900,#157901),(#157902,#157903),(#157904,#157905),
(#157906,#157907),(#157908,#157909),(#157910,#157911),(#157912,#157913),
(#157914,#157915),(#157916,#157917),(#157918,#157919),(#157920,#157921),
(#157922,#157923),(#157924,#157925),(#157926,#157927),(#157928,#157929),
(#157930,#157931),(#157932,#157933),(#157934,#157935),(#157936,#157937),
(#157938,#157939),(#157940,#157941),(#157942,#157943),(#157944,#157945),
(#157946,#157947),(#157948,#157949),(#157950,#157951),(#157952,#157953),
(#157954,#157955),(#157956,#157957),(#157958,#157959),(#157960,#157961),
(#157962,#157963),(#157964,#157965),(#157966,#157967),(#157968,#157969),
(#157970,#157971),(#157972,#157973),(#157974,#157975),(#157976,#157977),
(#157978,#157979),(#157980,#157981),(#157982,#157983),(#157984,#157985),
(#157986,#157987),(#157988,#157989),(#157990,#157991),(#157992,#157993),
(#157994,#157995),(#157996,#157997),(#157998,#157999),(#158000,#158001),
(#158002,#158003),(#158004,#158005),(#158006,#158007),(#158008,#158009),
(#158010,#158011),(#158012,#158013),(#158014,#158015),(#158016,#158017),
(#158018,#158019),(#158020,#158021),(#158022,#158023),(#158024,#158025),
(#158026,#158027),(#158028,#158029),(#158030,#158031),(#158032,#158033),
(#158034,#158035),(#158036,#158037),(#158038,#158039),(#158040,#158041),
(#158042,#158043),(#158044,#158045),(#158046,#158047),(#158048,#158049),
(#158050,#158051),(#158052,#158053),(#158054,#158055),(#158056,#158057),
(#158058,#158059),(#158060,#158061),(#158062,#158063),(#158064,#158065),
(#158066,#158067),(#158068,#158069),(#158070,#158071),(#158072,#158073),
(#158074,#158075),(#158076,#158077),(#158078,#158079),(#158080,#158081),
(#158082,#158083),(#158084,#158085),(#158086,#158087),(#158088,#158089),
(#158090,#158091),(#158092,#158093),(#158094,#158095),(#158096,#158097),
(#158098,#158099),(#158100,#158101),(#158102,#158103),(#158104,#158105),
(#158106,#158107),(#158108,#158109),(#158110,#158111),(#158112,#158113),
(#158114,#158115),(#158116,#158117),(#158118,#158119),(#158120,#158121),
(#158122,#158123),(#158124,#158125),(#158126,#158127),(#158128,#158129),
(#158130,#158131),(#158132,#158133),(#158134,#158135),(#158136,#158137),
(#158138,#158139),(#158140,#158141),(#158142,#158143),(#158144,#158145),
(#158146,#158147),(#158148,#158149),(#158150,#158151),(#158152,#158153),
(#158154,#158155),(#158156,#158157),(#158158,#158159),(#158160,#158161),
(#158162,#158163),(#158164,#158165),(#158166,#158167),(#158168,#158169),
(#158170,#158171),(#158172,#158173),(#158174,#158175),(#158176,#158177),
(#158178,#158179),(#158180,#158181),(#158182,#158183),(#158184,#158185),
(#158186,#158187),(#158188,#158189),(#158190,#158191),(#158192,#158193),
(#158194,#158195),(#158196,#158197),(#158198,#158199),(#158200,#158201),
(#158202,#158203),(#158204,#158205),(#158206,#158207),(#158208,#158209),
(#158210,#158211),(#158212,#158213),(#158214,#158215),(#158216,#158217),
(#158218,#158219),(#158220,#158221),(#158222,#158223),(#158224,#158225),
(#158226,#158227),(#158228,#158229),(#158230,#158231),(#158232,#158233),
(#158234,#158235),(#158236,#158237),(#158238,#158239),(#158240,#158241),
(#158242,#158243),(#158244,#158245),(#158246,#158247),(#158248,#158249),
(#158250,#158251),(#158252,#158253),(#158254,#158255),(#158256,#158257),
(#158258,#158259),(#158260,#158261),(#158262,#158263),(#158264,#158265),
(#158266,#158267),(#158268,#158269),(#158270,#158271),(#158272,#158273),
(#158274,#158275),(#158276,#158277),(#158278,#158279),(#158280,#158281),
(#158282,#158283),(#158284,#158285)),.UNSPECIFIED.,.F.,.F.,.F.,(6,1,1,1,
1,1,1,1,1,1,1,1,1,1,1,1,1,1,1,1,1,1,1,1,1,1,1,1,1,1,1,1,1,1,1,1,1,1,1,1,
1,1,1,1,1,1,1,1,1,1,1,1,1,1,1,1,1,1,1,1,1,1,1,1,1,1,1,1,1,1,1,1,1,1,1,1,
1,1,1,1,1,1,1,1,1,1,1,1,1,1,1,1,1,1,1,1,1,1,1,1,1,1,1,1,1,1,1,1,1,1,1,1,
1,1,1,1,1,1,1,1,1,1,1,1,1,1,1,1,1,1,1,1,1,1,1,1,1,1,1,1,1,1,1,1,1,1,1,1,
1,1,1,1,1,1,1,1,1,1,1,1,1,1,1,1,1,1,1,1,1,1,1,1,1,1,1,1,1,1,1,1,1,1,1,1,
1,1,1,1,1,1,1,1,1,1,1,1,1,1,1,1,1,1,1,1,1,1,1,1,1,1,1,1,1,1,1,1,1,1,1,1,
1,1,1,1,1,1,1,1,1,1,1,1,1,1,1,1,1,1,1,1,1,1,1,1,1,1,1,1,1,1,1,1,1,1,1,1,
1,1,1,1,1,1,1,1,1,1,1,1,1,1,1,1,1,1,1,1,1,1,1,1,1,1,1,1,1,1,1,1,1,1,1,1,
1,1,1,1,1,1,1,1,1,1,1,1,1,1,1,1,1,1,1,1,1,1,1,1,1,1,1,1,1,1,1,1,1,1,1,1,
1,1,1,1,1,1,1,1,1,1,1,1,1,1,1,1,1,1,1,1,1,1,1,1,1,1,1,1,1,1,1,1,1,1,1,1,
1,1,1,1,1,1,1,1,1,1,1,1,1,1,1,1,1,1,1,1,1,1,1,1,1,1,1,1,1,1,1,1,1,1,1,1,
1,1,1,1,1,1,1,1,1,1,1,1,1,1,1,1,1,1,1,1,1,1,1,1,1,1,1,1,1,1,1,1,1,1,1,1,
1,1,1,1,1,1,1,1,1,1,1,1,1,1,1,1,1,1,1,1,1,1,1,1,1,1,1,1,1,1,1,6),(2,2),
(-1.,-0.998165138,-0.996330275,-0.994495413,-0.99266055,-0.990825688,-0.988990826,
-0.987155963,-0.985321101,-0.983486239,-0.981651376,-0.979816514,-0.977981651,
-0.976146789,-0.974311927,-0.972477064,-0.970642202,-0.968807339,-0.966972477,
-0.965137615,-0.963302752,-0.96146789,-0.959633028,-0.957798165,-0.955963303,
-0.95412844,-0.952293578,-0.950458716,-0.948623853,-0.946788991,-0.944954128,
-0.943119266,-0.941284404,-0.939449541,-0.937614679,-0.935779817,-0.933944954,
-0.932110092,-0.930275229,-0.928440367,-0.926605505,-0.924770642,-0.92293578,
-0.921100917,-0.919266055,-0.917431193,-0.91559633,-0.913761468,-0.911926606,
-0.910091743,-0.908256881,-0.906422018,-0.904587156,-0.902752294,-0.900917431,
-0.899082569,-0.897247706,-0.895412844,-0.893577982,-0.891743119,-0.889908257,
-0.888073394,-0.886238532,-0.88440367,-0.882568807,-0.880733945,-0.878899083,
-0.87706422,-0.875229358,-0.873394495,-0.871559633,-0.869724771,-0.867889908,
-0.866055046,-0.864220183,-0.862385321,-0.860550459,-0.858715596,-0.856880734,
-0.855045872,-0.853211009,-0.851376147,-0.849541284,-0.847706422,-0.84587156,
-0.844036697,-0.842201835,-0.840366972,-0.83853211,-0.836697248,-0.834862385,
-0.833027523,-0.831192661,-0.829357798,-0.827522936,-0.825688073,-0.823853211,
-0.822018349,-0.820183486,-0.818348624,-0.816513761,-0.814678899,-0.812844037,
-0.811009174,-0.809174312,-0.80733945,-0.805504587,-0.803669725,-0.801834862,
-0.8,-0.798165138,-0.796330275,-0.794495413,-0.79266055,-0.790825688,-0.788990826,
-0.787155963,-0.785321101,-0.783486239,-0.781651376,-0.779816514,-0.777981651,
-0.776146789,-0.774311927,-0.772477064,-0.770642202,-0.768807339,-0.766972477,
-0.765137615,-0.763302752,-0.76146789,-0.759633028,-0.757798165,-0.755963303,
-0.75412844,-0.752293578,-0.750458716,-0.748623853,-0.746788991,-0.744954128,
-0.743119266,-0.741284404,-0.739449541,-0.737614679,-0.735779817,-0.733944954,
-0.732110092,-0.730275229,-0.728440367,-0.726605505,-0.724770642,-0.72293578,
-0.721100917,-0.719266055,-0.717431193,-0.71559633,-0.713761468,-0.711926606,
-0.710091743,-0.708256881,-0.706422018,-0.704587156,-0.702752294,-0.700917431,
-0.699082569,-0.697247706,-0.695412844,-0.693577982,-0.691743119,-0.689908257,
-0.688073394,-0.686238532,-0.68440367,-0.682568807,-0.680733945,-0.678899083,
-0.67706422,-0.675229358,-0.673394495,-0.671559633,-0.669724771,-0.667889908,
-0.666055046,-0.664220183,-0.662385321,-0.660550459,-0.658715596,-0.656880734,
-0.655045872,-0.653211009,-0.651376147,-0.649541284,-0.647706422,-0.64587156,
-0.644036697,-0.642201835,-0.640366972,-0.63853211,-0.636697248,-0.634862385,
-0.633027523,-0.631192661,-0.629357798,-0.627522936,-0.625688073,-0.623853211,
-0.622018349,-0.620183486,-0.618348624,-0.616513761,-0.614678899,-0.612844037,
-0.611009174,-0.609174312,-0.60733945,-0.605504587,-0.603669725,-0.601834862,
-0.6,-0.598165138,-0.596330275,-0.594495413,-0.59266055,-0.590825688,-0.588990826,
-0.587155963,-0.585321101,-0.583486239,-0.581651376,-0.579816514,-0.577981651,
-0.576146789,-0.574311927,-0.572477064,-0.570642202,-0.568807339,-0.566972477,
-0.565137615,-0.563302752,-0.56146789,-0.559633028,-0.557798165,-0.555963303,
-0.55412844,-0.552293578,-0.550458716,-0.548623853,-0.546788991,-0.544954128,
-0.543119266,-0.541284404,-0.539449541,-0.537614679,-0.535779817,-0.533944954,
-0.532110092,-0.530275229,-0.528440367,-0.526605505,-0.524770642,-0.52293578,
-0.521100917,-0.519266055,-0.517431193,-0.51559633,-0.513761468,-0.511926606,
-0.510091743,-0.508256881,-0.506422018,-0.504587156,-0.502752294,-0.500917431,
-0.499082569,-0.497247706,-0.495412844,-0.493577982,-0.491743119,-0.489908257,
-0.488073394,-0.486238532,-0.48440367,-0.482568807,-0.480733945,-0.478899083,
-0.47706422,-0.475229358,-0.473394495,-0.471559633,-0.469724771,-0.467889908,
-0.466055046,-0.464220183,-0.462385321,-0.460550459,-0.458715596,-0.456880734,
-0.455045872,-0.453211009,-0.451376147,-0.449541284,-0.447706422,-0.44587156,
-0.444036697,-0.442201835,-0.440366972,-0.43853211,-0.436697248,-0.434862385,
-0.433027523,-0.431192661,-0.429357798,-0.427522936,-0.425688073,-0.423853211,
-0.422018349,-0.420183486,-0.418348624,-0.416513761,-0.414678899,-0.412844037,
-0.411009174,-0.409174312,-0.40733945,-0.405504587,-0.403669725,-0.401834862,
-0.4,-0.398165138,-0.396330275,-0.394495413,-0.39266055,-0.390825688,-0.388990826,
-0.387155963,-0.385321101,-0.383486239,-0.381651376,-0.379816514,-0.377981651,
-0.376146789,-0.374311927,-0.372477064,-0.370642202,-0.368807339,-0.366972477,
-0.365137615,-0.363302752,-0.36146789,-0.359633028,-0.357798165,-0.355963303,
-0.35412844,-0.352293578,-0.350458716,-0.348623853,-0.346788991,-0.344954128,
-0.343119266,-0.341284404,-0.339449541,-0.337614679,-0.335779817,-0.333944954,
-0.332110092,-0.330275229,-0.328440367,-0.326605505,-0.324770642,-0.32293578,
-0.321100917,-0.319266055,-0.317431193,-0.31559633,-0.313761468,-0.311926606,
-0.310091743,-0.308256881,-0.306422018,-0.304587156,-0.302752294,-0.300917431,
-0.299082569,-0.297247706,-0.295412844,-0.293577982,-0.291743119,-0.289908257,
-0.288073394,-0.286238532,-0.28440367,-0.282568807,-0.280733945,-0.278899083,
-0.27706422,-0.275229358,-0.273394495,-0.271559633,-0.269724771,-0.267889908,
-0.266055046,-0.264220183,-0.262385321,-0.260550459,-0.258715596,-0.256880734,
-0.255045872,-0.253211009,-0.251376147,-0.249541284,-0.247706422,-0.24587156,
-0.244036697,-0.242201835,-0.240366972,-0.23853211,-0.236697248,-0.234862385,
-0.233027523,-0.231192661,-0.229357798,-0.227522936,-0.225688073,-0.223853211,
-0.222018349,-0.220183486,-0.218348624,-0.216513761,-0.214678899,-0.212844037,
-0.211009174,-0.209174312,-0.20733945,-0.205504587,-0.203669725,-0.201834862,
-0.2,-0.198165138,-0.196330275,-0.194495413,-0.19266055,-0.190825688,-0.188990826,
-0.187155963,-0.185321101,-0.183486239,-0.181651376,-0.179816514,-0.177981651,
-0.176146789,-0.174311927,-0.172477064,-0.170642202,-0.168807339,-0.166972477,
-0.165137615,-0.163302752,-0.16146789,-0.159633028,-0.157798165,-0.155963303,
-0.15412844,-0.152293578,-0.150458716,-0.148623853,-0.146788991,-0.144954128,
-0.143172103),(0.,0.36),.UNSPECIFIED.);
#6218=B_SPLINE_SURFACE_WITH_KNOTS('',5,1,((#158927,#158928),(#158929,#158930),
(#158931,#158932),(#158933,#158934),(#158935,#158936),(#158937,#158938),
(#158939,#158940),(#158941,#158942),(#158943,#158944),(#158945,#158946),
(#158947,#158948),(#158949,#158950),(#158951,#158952),(#158953,#158954),
(#158955,#158956),(#158957,#158958),(#158959,#158960),(#158961,#158962),
(#158963,#158964),(#158965,#158966),(#158967,#158968),(#158969,#158970),
(#158971,#158972),(#158973,#158974),(#158975,#158976),(#158977,#158978),
(#158979,#158980),(#158981,#158982),(#158983,#158984),(#158985,#158986),
(#158987,#158988),(#158989,#158990),(#158991,#158992),(#158993,#158994),
(#158995,#158996),(#158997,#158998),(#158999,#159000),(#159001,#159002),
(#159003,#159004),(#159005,#159006),(#159007,#159008),(#159009,#159010),
(#159011,#159012),(#159013,#159014),(#159015,#159016),(#159017,#159018),
(#159019,#159020),(#159021,#159022),(#159023,#159024),(#159025,#159026),
(#159027,#159028),(#159029,#159030),(#159031,#159032),(#159033,#159034),
(#159035,#159036),(#159037,#159038),(#159039,#159040),(#159041,#159042),
(#159043,#159044),(#159045,#159046),(#159047,#159048),(#159049,#159050),
(#159051,#159052),(#159053,#159054),(#159055,#159056),(#159057,#159058),
(#159059,#159060),(#159061,#159062),(#159063,#159064),(#159065,#159066),
(#159067,#159068),(#159069,#159070),(#159071,#159072),(#159073,#159074),
(#159075,#159076),(#159077,#159078),(#159079,#159080),(#159081,#159082),
(#159083,#159084),(#159085,#159086),(#159087,#159088),(#159089,#159090),
(#159091,#159092),(#159093,#159094),(#159095,#159096),(#159097,#159098),
(#159099,#159100),(#159101,#159102),(#159103,#159104),(#159105,#159106),
(#159107,#159108),(#159109,#159110),(#159111,#159112),(#159113,#159114),
(#159115,#159116),(#159117,#159118),(#159119,#159120),(#159121,#159122),
(#159123,#159124),(#159125,#159126),(#159127,#159128),(#159129,#159130),
(#159131,#159132),(#159133,#159134),(#159135,#159136),(#159137,#159138),
(#159139,#159140),(#159141,#159142),(#159143,#159144),(#159145,#159146),
(#159147,#159148),(#159149,#159150),(#159151,#159152),(#159153,#159154),
(#159155,#159156),(#159157,#159158),(#159159,#159160),(#159161,#159162),
(#159163,#159164),(#159165,#159166),(#159167,#159168),(#159169,#159170),
(#159171,#159172),(#159173,#159174),(#159175,#159176),(#159177,#159178),
(#159179,#159180),(#159181,#159182),(#159183,#159184),(#159185,#159186),
(#159187,#159188),(#159189,#159190),(#159191,#159192),(#159193,#159194),
(#159195,#159196),(#159197,#159198),(#159199,#159200),(#159201,#159202),
(#159203,#159204),(#159205,#159206),(#159207,#159208),(#159209,#159210),
(#159211,#159212),(#159213,#159214),(#159215,#159216),(#159217,#159218),
(#159219,#159220),(#159221,#159222),(#159223,#159224),(#159225,#159226),
(#159227,#159228),(#159229,#159230),(#159231,#159232),(#159233,#159234),
(#159235,#159236),(#159237,#159238),(#159239,#159240),(#159241,#159242),
(#159243,#159244),(#159245,#159246),(#159247,#159248),(#159249,#159250),
(#159251,#159252),(#159253,#159254),(#159255,#159256),(#159257,#159258),
(#159259,#159260),(#159261,#159262),(#159263,#159264),(#159265,#159266),
(#159267,#159268),(#159269,#159270),(#159271,#159272),(#159273,#159274),
(#159275,#159276),(#159277,#159278),(#159279,#159280),(#159281,#159282),
(#159283,#159284),(#159285,#159286),(#159287,#159288),(#159289,#159290),
(#159291,#159292),(#159293,#159294),(#159295,#159296),(#159297,#159298),
(#159299,#159300),(#159301,#159302),(#159303,#159304),(#159305,#159306),
(#159307,#159308),(#159309,#159310),(#159311,#159312),(#159313,#159314),
(#159315,#159316),(#159317,#159318),(#159319,#159320),(#159321,#159322),
(#159323,#159324),(#159325,#159326),(#159327,#159328),(#159329,#159330),
(#159331,#159332),(#159333,#159334),(#159335,#159336),(#159337,#159338),
(#159339,#159340),(#159341,#159342),(#159343,#159344),(#159345,#159346),
(#159347,#159348),(#159349,#159350),(#159351,#159352),(#159353,#159354),
(#159355,#159356),(#159357,#159358),(#159359,#159360),(#159361,#159362),
(#159363,#159364),(#159365,#159366),(#159367,#159368),(#159369,#159370),
(#159371,#159372),(#159373,#159374),(#159375,#159376),(#159377,#159378),
(#159379,#159380),(#159381,#159382),(#159383,#159384),(#159385,#159386),
(#159387,#159388),(#159389,#159390),(#159391,#159392),(#159393,#159394),
(#159395,#159396),(#159397,#159398),(#159399,#159400),(#159401,#159402),
(#159403,#159404),(#159405,#159406),(#159407,#159408),(#159409,#159410),
(#159411,#159412),(#159413,#159414),(#159415,#159416),(#159417,#159418),
(#159419,#159420),(#159421,#159422),(#159423,#159424),(#159425,#159426),
(#159427,#159428),(#159429,#159430),(#159431,#159432),(#159433,#159434),
(#159435,#159436),(#159437,#159438),(#159439,#159440),(#159441,#159442),
(#159443,#159444),(#159445,#159446),(#159447,#159448),(#159449,#159450),
(#159451,#159452),(#159453,#159454),(#159455,#159456),(#159457,#159458),
(#159459,#159460),(#159461,#159462),(#159463,#159464),(#159465,#159466),
(#159467,#159468),(#159469,#159470),(#159471,#159472),(#159473,#159474),
(#159475,#159476),(#159477,#159478),(#159479,#159480),(#159481,#159482),
(#159483,#159484),(#159485,#159486),(#159487,#159488),(#159489,#159490),
(#159491,#159492),(#159493,#159494),(#159495,#159496),(#159497,#159498),
(#159499,#159500),(#159501,#159502),(#159503,#159504),(#159505,#159506),
(#159507,#159508),(#159509,#159510),(#159511,#159512),(#159513,#159514),
(#159515,#159516),(#159517,#159518),(#159519,#159520),(#159521,#159522),
(#159523,#159524),(#159525,#159526),(#159527,#159528),(#159529,#159530),
(#159531,#159532),(#159533,#159534),(#159535,#159536),(#159537,#159538),
(#159539,#159540),(#159541,#159542),(#159543,#159544),(#159545,#159546),
(#159547,#159548),(#159549,#159550),(#159551,#159552),(#159553,#159554),
(#159555,#159556),(#159557,#159558),(#159559,#159560),(#159561,#159562),
(#159563,#159564),(#159565,#159566),(#159567,#159568),(#159569,#159570),
(#159571,#159572),(#159573,#159574),(#159575,#159576),(#159577,#159578),
(#159579,#159580),(#159581,#159582),(#159583,#159584),(#159585,#159586),
(#159587,#159588),(#159589,#159590),(#159591,#159592),(#159593,#159594),
(#159595,#159596),(#159597,#159598),(#159599,#159600),(#159601,#159602),
(#159603,#159604),(#159605,#159606),(#159607,#159608),(#159609,#159610),
(#159611,#159612),(#159613,#159614),(#159615,#159616),(#159617,#159618),
(#159619,#159620),(#159621,#159622),(#159623,#159624),(#159625,#159626),
(#159627,#159628),(#159629,#159630),(#159631,#159632),(#159633,#159634),
(#159635,#159636),(#159637,#159638),(#159639,#159640),(#159641,#159642),
(#159643,#159644),(#159645,#159646),(#159647,#159648),(#159649,#159650),
(#159651,#159652),(#159653,#159654),(#159655,#159656),(#159657,#159658),
(#159659,#159660),(#159661,#159662),(#159663,#159664),(#159665,#159666),
(#159667,#159668),(#159669,#159670),(#159671,#159672),(#159673,#159674),
(#159675,#159676),(#159677,#159678),(#159679,#159680),(#159681,#159682),
(#159683,#159684),(#159685,#159686),(#159687,#159688),(#159689,#159690),
(#159691,#159692),(#159693,#159694),(#159695,#159696),(#159697,#159698),
(#159699,#159700),(#159701,#159702),(#159703,#159704),(#159705,#159706),
(#159707,#159708),(#159709,#159710),(#159711,#159712),(#159713,#159714),
(#159715,#159716),(#159717,#159718),(#159719,#159720),(#159721,#159722),
(#159723,#159724),(#159725,#159726),(#159727,#159728),(#159729,#159730),
(#159731,#159732),(#159733,#159734),(#159735,#159736),(#159737,#159738),
(#159739,#159740),(#159741,#159742),(#159743,#159744),(#159745,#159746),
(#159747,#159748),(#159749,#159750),(#159751,#159752),(#159753,#159754),
(#159755,#159756),(#159757,#159758),(#159759,#159760),(#159761,#159762),
(#159763,#159764),(#159765,#159766),(#159767,#159768),(#159769,#159770),
(#159771,#159772),(#159773,#159774),(#159775,#159776),(#159777,#159778),
(#159779,#159780),(#159781,#159782),(#159783,#159784),(#159785,#159786),
(#159787,#159788),(#159789,#159790),(#159791,#159792),(#159793,#159794),
(#159795,#159796),(#159797,#159798),(#159799,#159800),(#159801,#159802),
(#159803,#159804),(#159805,#159806),(#159807,#159808),(#159809,#159810),
(#159811,#159812),(#159813,#159814),(#159815,#159816),(#159817,#159818),
(#159819,#159820),(#159821,#159822),(#159823,#159824),(#159825,#159826),
(#159827,#159828),(#159829,#159830),(#159831,#159832),(#159833,#159834),
(#159835,#159836),(#159837,#159838),(#159839,#159840),(#159841,#159842),
(#159843,#159844),(#159845,#159846),(#159847,#159848),(#159849,#159850),
(#159851,#159852),(#159853,#159854),(#159855,#159856),(#159857,#159858),
(#159859,#159860),(#159861,#159862),(#159863,#159864),(#159865,#159866),
(#159867,#159868),(#159869,#159870)),.UNSPECIFIED.,.F.,.F.,.F.,(6,1,1,1,
1,1,1,1,1,1,1,1,1,1,1,1,1,1,1,1,1,1,1,1,1,1,1,1,1,1,1,1,1,1,1,1,1,1,1,1,
1,1,1,1,1,1,1,1,1,1,1,1,1,1,1,1,1,1,1,1,1,1,1,1,1,1,1,1,1,1,1,1,1,1,1,1,
1,1,1,1,1,1,1,1,1,1,1,1,1,1,1,1,1,1,1,1,1,1,1,1,1,1,1,1,1,1,1,1,1,1,1,1,
1,1,1,1,1,1,1,1,1,1,1,1,1,1,1,1,1,1,1,1,1,1,1,1,1,1,1,1,1,1,1,1,1,1,1,1,
1,1,1,1,1,1,1,1,1,1,1,1,1,1,1,1,1,1,1,1,1,1,1,1,1,1,1,1,1,1,1,1,1,1,1,1,
1,1,1,1,1,1,1,1,1,1,1,1,1,1,1,1,1,1,1,1,1,1,1,1,1,1,1,1,1,1,1,1,1,1,1,1,
1,1,1,1,1,1,1,1,1,1,1,1,1,1,1,1,1,1,1,1,1,1,1,1,1,1,1,1,1,1,1,1,1,1,1,1,
1,1,1,1,1,1,1,1,1,1,1,1,1,1,1,1,1,1,1,1,1,1,1,1,1,1,1,1,1,1,1,1,1,1,1,1,
1,1,1,1,1,1,1,1,1,1,1,1,1,1,1,1,1,1,1,1,1,1,1,1,1,1,1,1,1,1,1,1,1,1,1,1,
1,1,1,1,1,1,1,1,1,1,1,1,1,1,1,1,1,1,1,1,1,1,1,1,1,1,1,1,1,1,1,1,1,1,1,1,
1,1,1,1,1,1,1,1,1,1,1,1,1,1,1,1,1,1,1,1,1,1,1,1,1,1,1,1,1,1,1,1,1,1,1,1,
1,1,1,1,1,1,1,1,1,1,1,1,1,1,1,1,1,1,1,1,1,1,1,1,1,1,1,1,1,1,1,1,1,1,1,1,
1,1,1,1,1,1,1,1,1,1,1,1,1,1,1,1,1,1,1,1,1,1,1,1,1,1,1,1,1,1,1,6),(2,2),
(0.143172103,0.144954128,0.146788991,0.148623853,0.150458716,0.152293578,
0.15412844,0.155963303,0.157798165,0.159633028,0.16146789,0.163302752,0.165137615,
0.166972477,0.168807339,0.170642202,0.172477064,0.174311927,0.176146789,
0.177981651,0.179816514,0.181651376,0.183486239,0.185321101,0.187155963,
0.188990826,0.190825688,0.19266055,0.194495413,0.196330275,0.198165138,
0.2,0.201834862,0.203669725,0.205504587,0.20733945,0.209174312,0.211009174,
0.212844037,0.214678899,0.216513761,0.218348624,0.220183486,0.222018349,
0.223853211,0.225688073,0.227522936,0.229357798,0.231192661,0.233027523,
0.234862385,0.236697248,0.23853211,0.240366972,0.242201835,0.244036697,
0.24587156,0.247706422,0.249541284,0.251376147,0.253211009,0.255045872,
0.256880734,0.258715596,0.260550459,0.262385321,0.264220183,0.266055046,
0.267889908,0.269724771,0.271559633,0.273394495,0.275229358,0.27706422,
0.278899083,0.280733945,0.282568807,0.28440367,0.286238532,0.288073394,
0.289908257,0.291743119,0.293577982,0.295412844,0.297247706,0.299082569,
0.300917431,0.302752294,0.304587156,0.306422018,0.308256881,0.310091743,
0.311926606,0.313761468,0.31559633,0.317431193,0.319266055,0.321100917,
0.32293578,0.324770642,0.326605505,0.328440367,0.330275229,0.332110092,
0.333944954,0.335779817,0.337614679,0.339449541,0.341284404,0.343119266,
0.344954128,0.346788991,0.348623853,0.350458716,0.352293578,0.35412844,
0.355963303,0.357798165,0.359633028,0.36146789,0.363302752,0.365137615,
0.366972477,0.368807339,0.370642202,0.372477064,0.374311927,0.376146789,
0.377981651,0.379816514,0.381651376,0.383486239,0.385321101,0.387155963,
0.388990826,0.390825688,0.39266055,0.394495413,0.396330275,0.398165138,
0.4,0.401834862,0.403669725,0.405504587,0.40733945,0.409174312,0.411009174,
0.412844037,0.414678899,0.416513761,0.418348624,0.420183486,0.422018349,
0.423853211,0.425688073,0.427522936,0.429357798,0.431192661,0.433027523,
0.434862385,0.436697248,0.43853211,0.440366972,0.442201835,0.444036697,
0.44587156,0.447706422,0.449541284,0.451376147,0.453211009,0.455045872,
0.456880734,0.458715596,0.460550459,0.462385321,0.464220183,0.466055046,
0.467889908,0.469724771,0.471559633,0.473394495,0.475229358,0.47706422,
0.478899083,0.480733945,0.482568807,0.48440367,0.486238532,0.488073394,
0.489908257,0.491743119,0.493577982,0.495412844,0.497247706,0.499082569,
0.500917431,0.502752294,0.504587156,0.506422018,0.508256881,0.510091743,
0.511926606,0.513761468,0.51559633,0.517431193,0.519266055,0.521100917,
0.52293578,0.524770642,0.526605505,0.528440367,0.530275229,0.532110092,
0.533944954,0.535779817,0.537614679,0.539449541,0.541284404,0.543119266,
0.544954128,0.546788991,0.548623853,0.550458716,0.552293578,0.55412844,
0.555963303,0.557798165,0.559633028,0.56146789,0.563302752,0.565137615,
0.566972477,0.568807339,0.570642202,0.572477064,0.574311927,0.576146789,
0.577981651,0.579816514,0.581651376,0.583486239,0.585321101,0.587155963,
0.588990826,0.590825688,0.59266055,0.594495413,0.596330275,0.598165138,
0.6,0.601834862,0.603669725,0.605504587,0.60733945,0.609174312,0.611009174,
0.612844037,0.614678899,0.616513761,0.618348624,0.620183486,0.622018349,
0.623853211,0.625688073,0.627522936,0.629357798,0.631192661,0.633027523,
0.634862385,0.636697248,0.63853211,0.640366972,0.642201835,0.644036697,
0.64587156,0.647706422,0.649541284,0.651376147,0.653211009,0.655045872,
0.656880734,0.658715596,0.660550459,0.662385321,0.664220183,0.666055046,
0.667889908,0.669724771,0.671559633,0.673394495,0.675229358,0.67706422,
0.678899083,0.680733945,0.682568807,0.68440367,0.686238532,0.688073394,
0.689908257,0.691743119,0.693577982,0.695412844,0.697247706,0.699082569,
0.700917431,0.702752294,0.704587156,0.706422018,0.708256881,0.710091743,
0.711926606,0.713761468,0.71559633,0.717431193,0.719266055,0.721100917,
0.72293578,0.724770642,0.726605505,0.728440367,0.730275229,0.732110092,
0.733944954,0.735779817,0.737614679,0.739449541,0.741284404,0.743119266,
0.744954128,0.746788991,0.748623853,0.750458716,0.752293578,0.75412844,
0.755963303,0.757798165,0.759633028,0.76146789,0.763302752,0.765137615,
0.766972477,0.768807339,0.770642202,0.772477064,0.774311927,0.776146789,
0.777981651,0.779816514,0.781651376,0.783486239,0.785321101,0.787155963,
0.788990826,0.790825688,0.79266055,0.794495413,0.796330275,0.798165138,
0.8,0.801834862,0.803669725,0.805504587,0.80733945,0.809174312,0.811009174,
0.812844037,0.814678899,0.816513761,0.818348624,0.820183486,0.822018349,
0.823853211,0.825688073,0.827522936,0.829357798,0.831192661,0.833027523,
0.834862385,0.836697248,0.83853211,0.840366972,0.842201835,0.844036697,
0.84587156,0.847706422,0.849541284,0.851376147,0.853211009,0.855045872,
0.856880734,0.858715596,0.860550459,0.862385321,0.864220183,0.866055046,
0.867889908,0.869724771,0.871559633,0.873394495,0.875229358,0.87706422,
0.878899083,0.880733945,0.882568807,0.88440367,0.886238532,0.888073394,
0.889908257,0.891743119,0.893577982,0.895412844,0.897247706,0.899082569,
0.900917431,0.902752294,0.904587156,0.906422018,0.908256881,0.910091743,
0.911926606,0.913761468,0.91559633,0.917431193,0.919266055,0.921100917,
0.92293578,0.924770642,0.926605505,0.928440367,0.930275229,0.932110092,
0.933944954,0.935779817,0.937614679,0.939449541,0.941284404,0.943119266,
0.944954128,0.946788991,0.948623853,0.950458716,0.952293578,0.95412844,
0.955963303,0.957798165,0.959633028,0.96146789,0.963302752,0.965137615,
0.966972477,0.968807339,0.970642202,0.972477064,0.974311927,0.976146789,
0.977981651,0.979816514,0.981651376,0.983486239,0.985321101,0.987155963,
0.988990826,0.990825688,0.99266055,0.994495413,0.996330275,0.998165138,
1.),(0.,0.36),.UNSPECIFIED.);
#6219=B_SPLINE_SURFACE_WITH_KNOTS('',5,1,((#160830,#160831),(#160832,#160833),
(#160834,#160835),(#160836,#160837),(#160838,#160839),(#160840,#160841),
(#160842,#160843),(#160844,#160845),(#160846,#160847),(#160848,#160849),
(#160850,#160851),(#160852,#160853),(#160854,#160855),(#160856,#160857),
(#160858,#160859),(#160860,#160861),(#160862,#160863),(#160864,#160865),
(#160866,#160867),(#160868,#160869),(#160870,#160871),(#160872,#160873),
(#160874,#160875),(#160876,#160877),(#160878,#160879),(#160880,#160881),
(#160882,#160883),(#160884,#160885),(#160886,#160887),(#160888,#160889),
(#160890,#160891),(#160892,#160893),(#160894,#160895),(#160896,#160897),
(#160898,#160899),(#160900,#160901),(#160902,#160903),(#160904,#160905),
(#160906,#160907),(#160908,#160909),(#160910,#160911),(#160912,#160913),
(#160914,#160915),(#160916,#160917),(#160918,#160919),(#160920,#160921),
(#160922,#160923),(#160924,#160925),(#160926,#160927),(#160928,#160929),
(#160930,#160931),(#160932,#160933),(#160934,#160935),(#160936,#160937),
(#160938,#160939),(#160940,#160941),(#160942,#160943),(#160944,#160945),
(#160946,#160947),(#160948,#160949),(#160950,#160951),(#160952,#160953),
(#160954,#160955),(#160956,#160957),(#160958,#160959),(#160960,#160961),
(#160962,#160963),(#160964,#160965),(#160966,#160967),(#160968,#160969),
(#160970,#160971),(#160972,#160973),(#160974,#160975),(#160976,#160977),
(#160978,#160979),(#160980,#160981),(#160982,#160983),(#160984,#160985),
(#160986,#160987),(#160988,#160989),(#160990,#160991),(#160992,#160993),
(#160994,#160995),(#160996,#160997),(#160998,#160999),(#161000,#161001),
(#161002,#161003),(#161004,#161005),(#161006,#161007),(#161008,#161009),
(#161010,#161011),(#161012,#161013),(#161014,#161015),(#161016,#161017),
(#161018,#161019),(#161020,#161021),(#161022,#161023),(#161024,#161025),
(#161026,#161027),(#161028,#161029),(#161030,#161031),(#161032,#161033),
(#161034,#161035),(#161036,#161037),(#161038,#161039),(#161040,#161041),
(#161042,#161043),(#161044,#161045),(#161046,#161047),(#161048,#161049),
(#161050,#161051),(#161052,#161053),(#161054,#161055),(#161056,#161057),
(#161058,#161059),(#161060,#161061),(#161062,#161063),(#161064,#161065),
(#161066,#161067),(#161068,#161069),(#161070,#161071),(#161072,#161073),
(#161074,#161075),(#161076,#161077),(#161078,#161079),(#161080,#161081),
(#161082,#161083),(#161084,#161085),(#161086,#161087),(#161088,#161089),
(#161090,#161091),(#161092,#161093),(#161094,#161095),(#161096,#161097),
(#161098,#161099),(#161100,#161101),(#161102,#161103),(#161104,#161105),
(#161106,#161107),(#161108,#161109),(#161110,#161111),(#161112,#161113),
(#161114,#161115),(#161116,#161117),(#161118,#161119),(#161120,#161121),
(#161122,#161123),(#161124,#161125),(#161126,#161127),(#161128,#161129),
(#161130,#161131),(#161132,#161133),(#161134,#161135),(#161136,#161137),
(#161138,#161139),(#161140,#161141),(#161142,#161143),(#161144,#161145),
(#161146,#161147),(#161148,#161149),(#161150,#161151),(#161152,#161153),
(#161154,#161155),(#161156,#161157),(#161158,#161159),(#161160,#161161),
(#161162,#161163),(#161164,#161165),(#161166,#161167),(#161168,#161169),
(#161170,#161171),(#161172,#161173),(#161174,#161175),(#161176,#161177),
(#161178,#161179),(#161180,#161181),(#161182,#161183),(#161184,#161185),
(#161186,#161187),(#161188,#161189),(#161190,#161191),(#161192,#161193),
(#161194,#161195),(#161196,#161197),(#161198,#161199),(#161200,#161201),
(#161202,#161203),(#161204,#161205),(#161206,#161207),(#161208,#161209),
(#161210,#161211),(#161212,#161213),(#161214,#161215),(#161216,#161217),
(#161218,#161219),(#161220,#161221),(#161222,#161223),(#161224,#161225),
(#161226,#161227),(#161228,#161229),(#161230,#161231),(#161232,#161233),
(#161234,#161235),(#161236,#161237),(#161238,#161239),(#161240,#161241),
(#161242,#161243),(#161244,#161245),(#161246,#161247),(#161248,#161249),
(#161250,#161251),(#161252,#161253),(#161254,#161255),(#161256,#161257),
(#161258,#161259),(#161260,#161261),(#161262,#161263),(#161264,#161265),
(#161266,#161267),(#161268,#161269),(#161270,#161271),(#161272,#161273),
(#161274,#161275),(#161276,#161277),(#161278,#161279),(#161280,#161281),
(#161282,#161283),(#161284,#161285),(#161286,#161287),(#161288,#161289),
(#161290,#161291),(#161292,#161293),(#161294,#161295),(#161296,#161297),
(#161298,#161299),(#161300,#161301),(#161302,#161303),(#161304,#161305),
(#161306,#161307),(#161308,#161309),(#161310,#161311),(#161312,#161313),
(#161314,#161315),(#161316,#161317),(#161318,#161319),(#161320,#161321),
(#161322,#161323),(#161324,#161325),(#161326,#161327),(#161328,#161329),
(#161330,#161331),(#161332,#161333),(#161334,#161335),(#161336,#161337),
(#161338,#161339),(#161340,#161341),(#161342,#161343),(#161344,#161345),
(#161346,#161347),(#161348,#161349),(#161350,#161351),(#161352,#161353),
(#161354,#161355),(#161356,#161357),(#161358,#161359),(#161360,#161361),
(#161362,#161363),(#161364,#161365),(#161366,#161367),(#161368,#161369),
(#161370,#161371),(#161372,#161373),(#161374,#161375),(#161376,#161377),
(#161378,#161379),(#161380,#161381),(#161382,#161383),(#161384,#161385),
(#161386,#161387),(#161388,#161389),(#161390,#161391),(#161392,#161393),
(#161394,#161395),(#161396,#161397),(#161398,#161399),(#161400,#161401),
(#161402,#161403),(#161404,#161405),(#161406,#161407),(#161408,#161409),
(#161410,#161411),(#161412,#161413),(#161414,#161415),(#161416,#161417),
(#161418,#161419),(#161420,#161421),(#161422,#161423),(#161424,#161425),
(#161426,#161427),(#161428,#161429),(#161430,#161431),(#161432,#161433),
(#161434,#161435),(#161436,#161437),(#161438,#161439),(#161440,#161441),
(#161442,#161443),(#161444,#161445),(#161446,#161447),(#161448,#161449),
(#161450,#161451),(#161452,#161453),(#161454,#161455),(#161456,#161457),
(#161458,#161459),(#161460,#161461),(#161462,#161463),(#161464,#161465),
(#161466,#161467),(#161468,#161469),(#161470,#161471),(#161472,#161473),
(#161474,#161475),(#161476,#161477),(#161478,#161479),(#161480,#161481),
(#161482,#161483),(#161484,#161485),(#161486,#161487),(#161488,#161489),
(#161490,#161491),(#161492,#161493),(#161494,#161495),(#161496,#161497),
(#161498,#161499),(#161500,#161501),(#161502,#161503),(#161504,#161505),
(#161506,#161507),(#161508,#161509),(#161510,#161511),(#161512,#161513),
(#161514,#161515),(#161516,#161517),(#161518,#161519),(#161520,#161521),
(#161522,#161523),(#161524,#161525),(#161526,#161527),(#161528,#161529),
(#161530,#161531),(#161532,#161533),(#161534,#161535),(#161536,#161537),
(#161538,#161539),(#161540,#161541),(#161542,#161543),(#161544,#161545),
(#161546,#161547),(#161548,#161549),(#161550,#161551),(#161552,#161553),
(#161554,#161555),(#161556,#161557),(#161558,#161559),(#161560,#161561),
(#161562,#161563),(#161564,#161565),(#161566,#161567),(#161568,#161569),
(#161570,#161571),(#161572,#161573),(#161574,#161575),(#161576,#161577),
(#161578,#161579),(#161580,#161581),(#161582,#161583),(#161584,#161585),
(#161586,#161587),(#161588,#161589),(#161590,#161591),(#161592,#161593),
(#161594,#161595),(#161596,#161597),(#161598,#161599),(#161600,#161601),
(#161602,#161603),(#161604,#161605),(#161606,#161607),(#161608,#161609),
(#161610,#161611),(#161612,#161613),(#161614,#161615),(#161616,#161617),
(#161618,#161619),(#161620,#161621),(#161622,#161623),(#161624,#161625),
(#161626,#161627),(#161628,#161629),(#161630,#161631),(#161632,#161633),
(#161634,#161635),(#161636,#161637),(#161638,#161639),(#161640,#161641),
(#161642,#161643),(#161644,#161645),(#161646,#161647),(#161648,#161649),
(#161650,#161651),(#161652,#161653),(#161654,#161655),(#161656,#161657),
(#161658,#161659),(#161660,#161661),(#161662,#161663),(#161664,#161665),
(#161666,#161667),(#161668,#161669),(#161670,#161671),(#161672,#161673),
(#161674,#161675),(#161676,#161677),(#161678,#161679),(#161680,#161681),
(#161682,#161683),(#161684,#161685),(#161686,#161687),(#161688,#161689),
(#161690,#161691),(#161692,#161693),(#161694,#161695),(#161696,#161697),
(#161698,#161699),(#161700,#161701),(#161702,#161703),(#161704,#161705),
(#161706,#161707),(#161708,#161709),(#161710,#161711),(#161712,#161713),
(#161714,#161715),(#161716,#161717),(#161718,#161719),(#161720,#161721),
(#161722,#161723),(#161724,#161725),(#161726,#161727),(#161728,#161729),
(#161730,#161731),(#161732,#161733),(#161734,#161735),(#161736,#161737),
(#161738,#161739),(#161740,#161741),(#161742,#161743),(#161744,#161745),
(#161746,#161747),(#161748,#161749),(#161750,#161751),(#161752,#161753),
(#161754,#161755),(#161756,#161757),(#161758,#161759),(#161760,#161761),
(#161762,#161763),(#161764,#161765),(#161766,#161767),(#161768,#161769),
(#161770,#161771),(#161772,#161773)),.UNSPECIFIED.,.F.,.F.,.F.,(6,1,1,1,
1,1,1,1,1,1,1,1,1,1,1,1,1,1,1,1,1,1,1,1,1,1,1,1,1,1,1,1,1,1,1,1,1,1,1,1,
1,1,1,1,1,1,1,1,1,1,1,1,1,1,1,1,1,1,1,1,1,1,1,1,1,1,1,1,1,1,1,1,1,1,1,1,
1,1,1,1,1,1,1,1,1,1,1,1,1,1,1,1,1,1,1,1,1,1,1,1,1,1,1,1,1,1,1,1,1,1,1,1,
1,1,1,1,1,1,1,1,1,1,1,1,1,1,1,1,1,1,1,1,1,1,1,1,1,1,1,1,1,1,1,1,1,1,1,1,
1,1,1,1,1,1,1,1,1,1,1,1,1,1,1,1,1,1,1,1,1,1,1,1,1,1,1,1,1,1,1,1,1,1,1,1,
1,1,1,1,1,1,1,1,1,1,1,1,1,1,1,1,1,1,1,1,1,1,1,1,1,1,1,1,1,1,1,1,1,1,1,1,
1,1,1,1,1,1,1,1,1,1,1,1,1,1,1,1,1,1,1,1,1,1,1,1,1,1,1,1,1,1,1,1,1,1,1,1,
1,1,1,1,1,1,1,1,1,1,1,1,1,1,1,1,1,1,1,1,1,1,1,1,1,1,1,1,1,1,1,1,1,1,1,1,
1,1,1,1,1,1,1,1,1,1,1,1,1,1,1,1,1,1,1,1,1,1,1,1,1,1,1,1,1,1,1,1,1,1,1,1,
1,1,1,1,1,1,1,1,1,1,1,1,1,1,1,1,1,1,1,1,1,1,1,1,1,1,1,1,1,1,1,1,1,1,1,1,
1,1,1,1,1,1,1,1,1,1,1,1,1,1,1,1,1,1,1,1,1,1,1,1,1,1,1,1,1,1,1,1,1,1,1,1,
1,1,1,1,1,1,1,1,1,1,1,1,1,1,1,1,1,1,1,1,1,1,1,1,1,1,1,1,1,1,1,1,1,1,1,1,
1,1,1,1,1,1,1,1,1,1,1,1,1,1,1,1,1,1,1,1,1,1,1,1,1,1,1,1,1,1,1,6),(2,2),
(0.143172103,0.144954128,0.146788991,0.148623853,0.150458716,0.152293578,
0.15412844,0.155963303,0.157798165,0.159633028,0.16146789,0.163302752,0.165137615,
0.166972477,0.168807339,0.170642202,0.172477064,0.174311927,0.176146789,
0.177981651,0.179816514,0.181651376,0.183486239,0.185321101,0.187155963,
0.188990826,0.190825688,0.19266055,0.194495413,0.196330275,0.198165138,
0.2,0.201834862,0.203669725,0.205504587,0.20733945,0.209174312,0.211009174,
0.212844037,0.214678899,0.216513761,0.218348624,0.220183486,0.222018349,
0.223853211,0.225688073,0.227522936,0.229357798,0.231192661,0.233027523,
0.234862385,0.236697248,0.23853211,0.240366972,0.242201835,0.244036697,
0.24587156,0.247706422,0.249541284,0.251376147,0.253211009,0.255045872,
0.256880734,0.258715596,0.260550459,0.262385321,0.264220183,0.266055046,
0.267889908,0.269724771,0.271559633,0.273394495,0.275229358,0.27706422,
0.278899083,0.280733945,0.282568807,0.28440367,0.286238532,0.288073394,
0.289908257,0.291743119,0.293577982,0.295412844,0.297247706,0.299082569,
0.300917431,0.302752294,0.304587156,0.306422018,0.308256881,0.310091743,
0.311926606,0.313761468,0.31559633,0.317431193,0.319266055,0.321100917,
0.32293578,0.324770642,0.326605505,0.328440367,0.330275229,0.332110092,
0.333944954,0.335779817,0.337614679,0.339449541,0.341284404,0.343119266,
0.344954128,0.346788991,0.348623853,0.350458716,0.352293578,0.35412844,
0.355963303,0.357798165,0.359633028,0.36146789,0.363302752,0.365137615,
0.366972477,0.368807339,0.370642202,0.372477064,0.374311927,0.376146789,
0.377981651,0.379816514,0.381651376,0.383486239,0.385321101,0.387155963,
0.388990826,0.390825688,0.39266055,0.394495413,0.396330275,0.398165138,
0.4,0.401834862,0.403669725,0.405504587,0.40733945,0.409174312,0.411009174,
0.412844037,0.414678899,0.416513761,0.418348624,0.420183486,0.422018349,
0.423853211,0.425688073,0.427522936,0.429357798,0.431192661,0.433027523,
0.434862385,0.436697248,0.43853211,0.440366972,0.442201835,0.444036697,
0.44587156,0.447706422,0.449541284,0.451376147,0.453211009,0.455045872,
0.456880734,0.458715596,0.460550459,0.462385321,0.464220183,0.466055046,
0.467889908,0.469724771,0.471559633,0.473394495,0.475229358,0.47706422,
0.478899083,0.480733945,0.482568807,0.48440367,0.486238532,0.488073394,
0.489908257,0.491743119,0.493577982,0.495412844,0.497247706,0.499082569,
0.500917431,0.502752294,0.504587156,0.506422018,0.508256881,0.510091743,
0.511926606,0.513761468,0.51559633,0.517431193,0.519266055,0.521100917,
0.52293578,0.524770642,0.526605505,0.528440367,0.530275229,0.532110092,
0.533944954,0.535779817,0.537614679,0.539449541,0.541284404,0.543119266,
0.544954128,0.546788991,0.548623853,0.550458716,0.552293578,0.55412844,
0.555963303,0.557798165,0.559633028,0.56146789,0.563302752,0.565137615,
0.566972477,0.568807339,0.570642202,0.572477064,0.574311927,0.576146789,
0.577981651,0.579816514,0.581651376,0.583486239,0.585321101,0.587155963,
0.588990826,0.590825688,0.59266055,0.594495413,0.596330275,0.598165138,
0.6,0.601834862,0.603669725,0.605504587,0.60733945,0.609174312,0.611009174,
0.612844037,0.614678899,0.616513761,0.618348624,0.620183486,0.622018349,
0.623853211,0.625688073,0.627522936,0.629357798,0.631192661,0.633027523,
0.634862385,0.636697248,0.63853211,0.640366972,0.642201835,0.644036697,
0.64587156,0.647706422,0.649541284,0.651376147,0.653211009,0.655045872,
0.656880734,0.658715596,0.660550459,0.662385321,0.664220183,0.666055046,
0.667889908,0.669724771,0.671559633,0.673394495,0.675229358,0.67706422,
0.678899083,0.680733945,0.682568807,0.68440367,0.686238532,0.688073394,
0.689908257,0.691743119,0.693577982,0.695412844,0.697247706,0.699082569,
0.700917431,0.702752294,0.704587156,0.706422018,0.708256881,0.710091743,
0.711926606,0.713761468,0.71559633,0.717431193,0.719266055,0.721100917,
0.72293578,0.724770642,0.726605505,0.728440367,0.730275229,0.732110092,
0.733944954,0.735779817,0.737614679,0.739449541,0.741284404,0.743119266,
0.744954128,0.746788991,0.748623853,0.750458716,0.752293578,0.75412844,
0.755963303,0.757798165,0.759633028,0.76146789,0.763302752,0.765137615,
0.766972477,0.768807339,0.770642202,0.772477064,0.774311927,0.776146789,
0.777981651,0.779816514,0.781651376,0.783486239,0.785321101,0.787155963,
0.788990826,0.790825688,0.79266055,0.794495413,0.796330275,0.798165138,
0.8,0.801834862,0.803669725,0.805504587,0.80733945,0.809174312,0.811009174,
0.812844037,0.814678899,0.816513761,0.818348624,0.820183486,0.822018349,
0.823853211,0.825688073,0.827522936,0.829357798,0.831192661,0.833027523,
0.834862385,0.836697248,0.83853211,0.840366972,0.842201835,0.844036697,
0.84587156,0.847706422,0.849541284,0.851376147,0.853211009,0.855045872,
0.856880734,0.858715596,0.860550459,0.862385321,0.864220183,0.866055046,
0.867889908,0.869724771,0.871559633,0.873394495,0.875229358,0.87706422,
0.878899083,0.880733945,0.882568807,0.88440367,0.886238532,0.888073394,
0.889908257,0.891743119,0.893577982,0.895412844,0.897247706,0.899082569,
0.900917431,0.902752294,0.904587156,0.906422018,0.908256881,0.910091743,
0.911926606,0.913761468,0.91559633,0.917431193,0.919266055,0.921100917,
0.92293578,0.924770642,0.926605505,0.928440367,0.930275229,0.932110092,
0.933944954,0.935779817,0.937614679,0.939449541,0.941284404,0.943119266,
0.944954128,0.946788991,0.948623853,0.950458716,0.952293578,0.95412844,
0.955963303,0.957798165,0.959633028,0.96146789,0.963302752,0.965137615,
0.966972477,0.968807339,0.970642202,0.972477064,0.974311927,0.976146789,
0.977981651,0.979816514,0.981651376,0.983486239,0.985321101,0.987155963,
0.988990826,0.990825688,0.99266055,0.994495413,0.996330275,0.998165138,
1.),(0.,0.36),.UNSPECIFIED.);
#6220=B_SPLINE_SURFACE_WITH_KNOTS('',5,1,((#162430,#162431),(#162432,#162433),
(#162434,#162435),(#162436,#162437),(#162438,#162439),(#162440,#162441),
(#162442,#162443),(#162444,#162445),(#162446,#162447),(#162448,#162449),
(#162450,#162451),(#162452,#162453),(#162454,#162455),(#162456,#162457),
(#162458,#162459),(#162460,#162461),(#162462,#162463),(#162464,#162465),
(#162466,#162467),(#162468,#162469),(#162470,#162471),(#162472,#162473),
(#162474,#162475),(#162476,#162477),(#162478,#162479),(#162480,#162481),
(#162482,#162483),(#162484,#162485),(#162486,#162487),(#162488,#162489),
(#162490,#162491),(#162492,#162493),(#162494,#162495),(#162496,#162497),
(#162498,#162499),(#162500,#162501),(#162502,#162503),(#162504,#162505),
(#162506,#162507),(#162508,#162509),(#162510,#162511),(#162512,#162513),
(#162514,#162515),(#162516,#162517),(#162518,#162519),(#162520,#162521),
(#162522,#162523),(#162524,#162525),(#162526,#162527),(#162528,#162529),
(#162530,#162531),(#162532,#162533),(#162534,#162535),(#162536,#162537),
(#162538,#162539),(#162540,#162541),(#162542,#162543),(#162544,#162545),
(#162546,#162547),(#162548,#162549),(#162550,#162551),(#162552,#162553),
(#162554,#162555),(#162556,#162557),(#162558,#162559),(#162560,#162561),
(#162562,#162563),(#162564,#162565),(#162566,#162567),(#162568,#162569),
(#162570,#162571),(#162572,#162573),(#162574,#162575),(#162576,#162577),
(#162578,#162579),(#162580,#162581),(#162582,#162583),(#162584,#162585),
(#162586,#162587),(#162588,#162589),(#162590,#162591),(#162592,#162593),
(#162594,#162595),(#162596,#162597),(#162598,#162599),(#162600,#162601),
(#162602,#162603),(#162604,#162605),(#162606,#162607),(#162608,#162609),
(#162610,#162611),(#162612,#162613),(#162614,#162615),(#162616,#162617),
(#162618,#162619),(#162620,#162621),(#162622,#162623),(#162624,#162625),
(#162626,#162627),(#162628,#162629),(#162630,#162631),(#162632,#162633),
(#162634,#162635),(#162636,#162637),(#162638,#162639),(#162640,#162641),
(#162642,#162643),(#162644,#162645),(#162646,#162647),(#162648,#162649),
(#162650,#162651),(#162652,#162653),(#162654,#162655),(#162656,#162657),
(#162658,#162659),(#162660,#162661),(#162662,#162663),(#162664,#162665),
(#162666,#162667),(#162668,#162669),(#162670,#162671),(#162672,#162673),
(#162674,#162675),(#162676,#162677),(#162678,#162679),(#162680,#162681),
(#162682,#162683),(#162684,#162685),(#162686,#162687),(#162688,#162689),
(#162690,#162691),(#162692,#162693),(#162694,#162695),(#162696,#162697),
(#162698,#162699),(#162700,#162701),(#162702,#162703),(#162704,#162705),
(#162706,#162707),(#162708,#162709),(#162710,#162711),(#162712,#162713),
(#162714,#162715),(#162716,#162717),(#162718,#162719),(#162720,#162721),
(#162722,#162723),(#162724,#162725),(#162726,#162727),(#162728,#162729),
(#162730,#162731),(#162732,#162733),(#162734,#162735),(#162736,#162737),
(#162738,#162739),(#162740,#162741),(#162742,#162743),(#162744,#162745),
(#162746,#162747),(#162748,#162749),(#162750,#162751),(#162752,#162753),
(#162754,#162755),(#162756,#162757),(#162758,#162759),(#162760,#162761),
(#162762,#162763),(#162764,#162765),(#162766,#162767),(#162768,#162769),
(#162770,#162771),(#162772,#162773),(#162774,#162775),(#162776,#162777),
(#162778,#162779),(#162780,#162781),(#162782,#162783),(#162784,#162785),
(#162786,#162787),(#162788,#162789),(#162790,#162791),(#162792,#162793),
(#162794,#162795),(#162796,#162797),(#162798,#162799),(#162800,#162801),
(#162802,#162803),(#162804,#162805),(#162806,#162807),(#162808,#162809),
(#162810,#162811),(#162812,#162813),(#162814,#162815),(#162816,#162817),
(#162818,#162819),(#162820,#162821),(#162822,#162823),(#162824,#162825),
(#162826,#162827),(#162828,#162829),(#162830,#162831),(#162832,#162833),
(#162834,#162835),(#162836,#162837),(#162838,#162839),(#162840,#162841),
(#162842,#162843),(#162844,#162845),(#162846,#162847),(#162848,#162849),
(#162850,#162851),(#162852,#162853),(#162854,#162855),(#162856,#162857),
(#162858,#162859),(#162860,#162861),(#162862,#162863),(#162864,#162865),
(#162866,#162867),(#162868,#162869),(#162870,#162871),(#162872,#162873),
(#162874,#162875),(#162876,#162877),(#162878,#162879),(#162880,#162881),
(#162882,#162883),(#162884,#162885),(#162886,#162887),(#162888,#162889),
(#162890,#162891),(#162892,#162893),(#162894,#162895),(#162896,#162897),
(#162898,#162899),(#162900,#162901),(#162902,#162903),(#162904,#162905),
(#162906,#162907),(#162908,#162909),(#162910,#162911),(#162912,#162913),
(#162914,#162915),(#162916,#162917),(#162918,#162919),(#162920,#162921),
(#162922,#162923),(#162924,#162925),(#162926,#162927),(#162928,#162929),
(#162930,#162931),(#162932,#162933),(#162934,#162935),(#162936,#162937),
(#162938,#162939),(#162940,#162941),(#162942,#162943),(#162944,#162945),
(#162946,#162947),(#162948,#162949),(#162950,#162951),(#162952,#162953),
(#162954,#162955),(#162956,#162957),(#162958,#162959),(#162960,#162961),
(#162962,#162963),(#162964,#162965),(#162966,#162967),(#162968,#162969),
(#162970,#162971),(#162972,#162973),(#162974,#162975),(#162976,#162977),
(#162978,#162979),(#162980,#162981),(#162982,#162983),(#162984,#162985),
(#162986,#162987),(#162988,#162989),(#162990,#162991),(#162992,#162993),
(#162994,#162995),(#162996,#162997),(#162998,#162999),(#163000,#163001),
(#163002,#163003),(#163004,#163005),(#163006,#163007),(#163008,#163009),
(#163010,#163011),(#163012,#163013),(#163014,#163015),(#163016,#163017),
(#163018,#163019),(#163020,#163021),(#163022,#163023),(#163024,#163025),
(#163026,#163027),(#163028,#163029),(#163030,#163031),(#163032,#163033),
(#163034,#163035),(#163036,#163037),(#163038,#163039),(#163040,#163041),
(#163042,#163043),(#163044,#163045),(#163046,#163047),(#163048,#163049),
(#163050,#163051),(#163052,#163053),(#163054,#163055),(#163056,#163057),
(#163058,#163059),(#163060,#163061),(#163062,#163063),(#163064,#163065),
(#163066,#163067),(#163068,#163069),(#163070,#163071),(#163072,#163073),
(#163074,#163075),(#163076,#163077),(#163078,#163079),(#163080,#163081),
(#163082,#163083),(#163084,#163085),(#163086,#163087),(#163088,#163089),
(#163090,#163091),(#163092,#163093),(#163094,#163095),(#163096,#163097),
(#163098,#163099),(#163100,#163101),(#163102,#163103),(#163104,#163105),
(#163106,#163107),(#163108,#163109),(#163110,#163111),(#163112,#163113),
(#163114,#163115),(#163116,#163117),(#163118,#163119),(#163120,#163121),
(#163122,#163123),(#163124,#163125),(#163126,#163127),(#163128,#163129),
(#163130,#163131),(#163132,#163133),(#163134,#163135),(#163136,#163137),
(#163138,#163139),(#163140,#163141),(#163142,#163143),(#163144,#163145),
(#163146,#163147),(#163148,#163149),(#163150,#163151),(#163152,#163153),
(#163154,#163155),(#163156,#163157),(#163158,#163159),(#163160,#163161),
(#163162,#163163),(#163164,#163165),(#163166,#163167),(#163168,#163169),
(#163170,#163171),(#163172,#163173),(#163174,#163175),(#163176,#163177),
(#163178,#163179),(#163180,#163181),(#163182,#163183),(#163184,#163185),
(#163186,#163187),(#163188,#163189),(#163190,#163191),(#163192,#163193),
(#163194,#163195),(#163196,#163197),(#163198,#163199),(#163200,#163201),
(#163202,#163203),(#163204,#163205),(#163206,#163207),(#163208,#163209),
(#163210,#163211),(#163212,#163213),(#163214,#163215),(#163216,#163217),
(#163218,#163219),(#163220,#163221),(#163222,#163223),(#163224,#163225),
(#163226,#163227),(#163228,#163229),(#163230,#163231),(#163232,#163233),
(#163234,#163235),(#163236,#163237),(#163238,#163239),(#163240,#163241),
(#163242,#163243),(#163244,#163245),(#163246,#163247),(#163248,#163249),
(#163250,#163251),(#163252,#163253),(#163254,#163255),(#163256,#163257),
(#163258,#163259),(#163260,#163261),(#163262,#163263),(#163264,#163265),
(#163266,#163267),(#163268,#163269),(#163270,#163271),(#163272,#163273),
(#163274,#163275),(#163276,#163277),(#163278,#163279),(#163280,#163281),
(#163282,#163283),(#163284,#163285),(#163286,#163287),(#163288,#163289),
(#163290,#163291),(#163292,#163293),(#163294,#163295),(#163296,#163297),
(#163298,#163299),(#163300,#163301),(#163302,#163303),(#163304,#163305),
(#163306,#163307),(#163308,#163309),(#163310,#163311),(#163312,#163313),
(#163314,#163315),(#163316,#163317),(#163318,#163319),(#163320,#163321),
(#163322,#163323),(#163324,#163325),(#163326,#163327),(#163328,#163329),
(#163330,#163331),(#163332,#163333),(#163334,#163335),(#163336,#163337),
(#163338,#163339),(#163340,#163341),(#163342,#163343),(#163344,#163345),
(#163346,#163347),(#163348,#163349),(#163350,#163351),(#163352,#163353),
(#163354,#163355),(#163356,#163357),(#163358,#163359),(#163360,#163361),
(#163362,#163363),(#163364,#163365),(#163366,#163367),(#163368,#163369),
(#163370,#163371),(#163372,#163373)),.UNSPECIFIED.,.F.,.F.,.F.,(6,1,1,1,
1,1,1,1,1,1,1,1,1,1,1,1,1,1,1,1,1,1,1,1,1,1,1,1,1,1,1,1,1,1,1,1,1,1,1,1,
1,1,1,1,1,1,1,1,1,1,1,1,1,1,1,1,1,1,1,1,1,1,1,1,1,1,1,1,1,1,1,1,1,1,1,1,
1,1,1,1,1,1,1,1,1,1,1,1,1,1,1,1,1,1,1,1,1,1,1,1,1,1,1,1,1,1,1,1,1,1,1,1,
1,1,1,1,1,1,1,1,1,1,1,1,1,1,1,1,1,1,1,1,1,1,1,1,1,1,1,1,1,1,1,1,1,1,1,1,
1,1,1,1,1,1,1,1,1,1,1,1,1,1,1,1,1,1,1,1,1,1,1,1,1,1,1,1,1,1,1,1,1,1,1,1,
1,1,1,1,1,1,1,1,1,1,1,1,1,1,1,1,1,1,1,1,1,1,1,1,1,1,1,1,1,1,1,1,1,1,1,1,
1,1,1,1,1,1,1,1,1,1,1,1,1,1,1,1,1,1,1,1,1,1,1,1,1,1,1,1,1,1,1,1,1,1,1,1,
1,1,1,1,1,1,1,1,1,1,1,1,1,1,1,1,1,1,1,1,1,1,1,1,1,1,1,1,1,1,1,1,1,1,1,1,
1,1,1,1,1,1,1,1,1,1,1,1,1,1,1,1,1,1,1,1,1,1,1,1,1,1,1,1,1,1,1,1,1,1,1,1,
1,1,1,1,1,1,1,1,1,1,1,1,1,1,1,1,1,1,1,1,1,1,1,1,1,1,1,1,1,1,1,1,1,1,1,1,
1,1,1,1,1,1,1,1,1,1,1,1,1,1,1,1,1,1,1,1,1,1,1,1,1,1,1,1,1,1,1,1,1,1,1,1,
1,1,1,1,1,1,1,1,1,1,1,1,1,1,1,1,1,1,1,1,1,1,1,1,1,1,1,1,1,1,1,1,1,1,1,1,
1,1,1,1,1,1,1,1,1,1,1,1,1,1,1,1,1,1,1,1,1,1,1,1,1,1,1,1,1,1,1,6),(2,2),
(-1.,-0.998165138,-0.996330275,-0.994495413,-0.99266055,-0.990825688,-0.988990826,
-0.987155963,-0.985321101,-0.983486239,-0.981651376,-0.979816514,-0.977981651,
-0.976146789,-0.974311927,-0.972477064,-0.970642202,-0.968807339,-0.966972477,
-0.965137615,-0.963302752,-0.96146789,-0.959633028,-0.957798165,-0.955963303,
-0.95412844,-0.952293578,-0.950458716,-0.948623853,-0.946788991,-0.944954128,
-0.943119266,-0.941284404,-0.939449541,-0.937614679,-0.935779817,-0.933944954,
-0.932110092,-0.930275229,-0.928440367,-0.926605505,-0.924770642,-0.92293578,
-0.921100917,-0.919266055,-0.917431193,-0.91559633,-0.913761468,-0.911926606,
-0.910091743,-0.908256881,-0.906422018,-0.904587156,-0.902752294,-0.900917431,
-0.899082569,-0.897247706,-0.895412844,-0.893577982,-0.891743119,-0.889908257,
-0.888073394,-0.886238532,-0.88440367,-0.882568807,-0.880733945,-0.878899083,
-0.87706422,-0.875229358,-0.873394495,-0.871559633,-0.869724771,-0.867889908,
-0.866055046,-0.864220183,-0.862385321,-0.860550459,-0.858715596,-0.856880734,
-0.855045872,-0.853211009,-0.851376147,-0.849541284,-0.847706422,-0.84587156,
-0.844036697,-0.842201835,-0.840366972,-0.83853211,-0.836697248,-0.834862385,
-0.833027523,-0.831192661,-0.829357798,-0.827522936,-0.825688073,-0.823853211,
-0.822018349,-0.820183486,-0.818348624,-0.816513761,-0.814678899,-0.812844037,
-0.811009174,-0.809174312,-0.80733945,-0.805504587,-0.803669725,-0.801834862,
-0.8,-0.798165138,-0.796330275,-0.794495413,-0.79266055,-0.790825688,-0.788990826,
-0.787155963,-0.785321101,-0.783486239,-0.781651376,-0.779816514,-0.777981651,
-0.776146789,-0.774311927,-0.772477064,-0.770642202,-0.768807339,-0.766972477,
-0.765137615,-0.763302752,-0.76146789,-0.759633028,-0.757798165,-0.755963303,
-0.75412844,-0.752293578,-0.750458716,-0.748623853,-0.746788991,-0.744954128,
-0.743119266,-0.741284404,-0.739449541,-0.737614679,-0.735779817,-0.733944954,
-0.732110092,-0.730275229,-0.728440367,-0.726605505,-0.724770642,-0.72293578,
-0.721100917,-0.719266055,-0.717431193,-0.71559633,-0.713761468,-0.711926606,
-0.710091743,-0.708256881,-0.706422018,-0.704587156,-0.702752294,-0.700917431,
-0.699082569,-0.697247706,-0.695412844,-0.693577982,-0.691743119,-0.689908257,
-0.688073394,-0.686238532,-0.68440367,-0.682568807,-0.680733945,-0.678899083,
-0.67706422,-0.675229358,-0.673394495,-0.671559633,-0.669724771,-0.667889908,
-0.666055046,-0.664220183,-0.662385321,-0.660550459,-0.658715596,-0.656880734,
-0.655045872,-0.653211009,-0.651376147,-0.649541284,-0.647706422,-0.64587156,
-0.644036697,-0.642201835,-0.640366972,-0.63853211,-0.636697248,-0.634862385,
-0.633027523,-0.631192661,-0.629357798,-0.627522936,-0.625688073,-0.623853211,
-0.622018349,-0.620183486,-0.618348624,-0.616513761,-0.614678899,-0.612844037,
-0.611009174,-0.609174312,-0.60733945,-0.605504587,-0.603669725,-0.601834862,
-0.6,-0.598165138,-0.596330275,-0.594495413,-0.59266055,-0.590825688,-0.588990826,
-0.587155963,-0.585321101,-0.583486239,-0.581651376,-0.579816514,-0.577981651,
-0.576146789,-0.574311927,-0.572477064,-0.570642202,-0.568807339,-0.566972477,
-0.565137615,-0.563302752,-0.56146789,-0.559633028,-0.557798165,-0.555963303,
-0.55412844,-0.552293578,-0.550458716,-0.548623853,-0.546788991,-0.544954128,
-0.543119266,-0.541284404,-0.539449541,-0.537614679,-0.535779817,-0.533944954,
-0.532110092,-0.530275229,-0.528440367,-0.526605505,-0.524770642,-0.52293578,
-0.521100917,-0.519266055,-0.517431193,-0.51559633,-0.513761468,-0.511926606,
-0.510091743,-0.508256881,-0.506422018,-0.504587156,-0.502752294,-0.500917431,
-0.499082569,-0.497247706,-0.495412844,-0.493577982,-0.491743119,-0.489908257,
-0.488073394,-0.486238532,-0.48440367,-0.482568807,-0.480733945,-0.478899083,
-0.47706422,-0.475229358,-0.473394495,-0.471559633,-0.469724771,-0.467889908,
-0.466055046,-0.464220183,-0.462385321,-0.460550459,-0.458715596,-0.456880734,
-0.455045872,-0.453211009,-0.451376147,-0.449541284,-0.447706422,-0.44587156,
-0.444036697,-0.442201835,-0.440366972,-0.43853211,-0.436697248,-0.434862385,
-0.433027523,-0.431192661,-0.429357798,-0.427522936,-0.425688073,-0.423853211,
-0.422018349,-0.420183486,-0.418348624,-0.416513761,-0.414678899,-0.412844037,
-0.411009174,-0.409174312,-0.40733945,-0.405504587,-0.403669725,-0.401834862,
-0.4,-0.398165138,-0.396330275,-0.394495413,-0.39266055,-0.390825688,-0.388990826,
-0.387155963,-0.385321101,-0.383486239,-0.381651376,-0.379816514,-0.377981651,
-0.376146789,-0.374311927,-0.372477064,-0.370642202,-0.368807339,-0.366972477,
-0.365137615,-0.363302752,-0.36146789,-0.359633028,-0.357798165,-0.355963303,
-0.35412844,-0.352293578,-0.350458716,-0.348623853,-0.346788991,-0.344954128,
-0.343119266,-0.341284404,-0.339449541,-0.337614679,-0.335779817,-0.333944954,
-0.332110092,-0.330275229,-0.328440367,-0.326605505,-0.324770642,-0.32293578,
-0.321100917,-0.319266055,-0.317431193,-0.31559633,-0.313761468,-0.311926606,
-0.310091743,-0.308256881,-0.306422018,-0.304587156,-0.302752294,-0.300917431,
-0.299082569,-0.297247706,-0.295412844,-0.293577982,-0.291743119,-0.289908257,
-0.288073394,-0.286238532,-0.28440367,-0.282568807,-0.280733945,-0.278899083,
-0.27706422,-0.275229358,-0.273394495,-0.271559633,-0.269724771,-0.267889908,
-0.266055046,-0.264220183,-0.262385321,-0.260550459,-0.258715596,-0.256880734,
-0.255045872,-0.253211009,-0.251376147,-0.249541284,-0.247706422,-0.24587156,
-0.244036697,-0.242201835,-0.240366972,-0.23853211,-0.236697248,-0.234862385,
-0.233027523,-0.231192661,-0.229357798,-0.227522936,-0.225688073,-0.223853211,
-0.222018349,-0.220183486,-0.218348624,-0.216513761,-0.214678899,-0.212844037,
-0.211009174,-0.209174312,-0.20733945,-0.205504587,-0.203669725,-0.201834862,
-0.2,-0.198165138,-0.196330275,-0.194495413,-0.19266055,-0.190825688,-0.188990826,
-0.187155963,-0.185321101,-0.183486239,-0.181651376,-0.179816514,-0.177981651,
-0.176146789,-0.174311927,-0.172477064,-0.170642202,-0.168807339,-0.166972477,
-0.165137615,-0.163302752,-0.16146789,-0.159633028,-0.157798165,-0.155963303,
-0.15412844,-0.152293578,-0.150458716,-0.148623853,-0.146788991,-0.144954128,
-0.143172103),(0.,0.36),.UNSPECIFIED.);
#6221=B_SPLINE_SURFACE_WITH_KNOTS('',5,1,((#164030,#164031),(#164032,#164033),
(#164034,#164035),(#164036,#164037),(#164038,#164039),(#164040,#164041),
(#164042,#164043),(#164044,#164045),(#164046,#164047),(#164048,#164049),
(#164050,#164051),(#164052,#164053),(#164054,#164055),(#164056,#164057),
(#164058,#164059),(#164060,#164061),(#164062,#164063),(#164064,#164065),
(#164066,#164067),(#164068,#164069),(#164070,#164071),(#164072,#164073),
(#164074,#164075),(#164076,#164077),(#164078,#164079),(#164080,#164081),
(#164082,#164083),(#164084,#164085),(#164086,#164087),(#164088,#164089),
(#164090,#164091),(#164092,#164093),(#164094,#164095),(#164096,#164097),
(#164098,#164099),(#164100,#164101),(#164102,#164103),(#164104,#164105),
(#164106,#164107),(#164108,#164109),(#164110,#164111),(#164112,#164113),
(#164114,#164115),(#164116,#164117),(#164118,#164119),(#164120,#164121),
(#164122,#164123),(#164124,#164125),(#164126,#164127),(#164128,#164129),
(#164130,#164131),(#164132,#164133),(#164134,#164135),(#164136,#164137),
(#164138,#164139),(#164140,#164141),(#164142,#164143),(#164144,#164145),
(#164146,#164147),(#164148,#164149),(#164150,#164151),(#164152,#164153),
(#164154,#164155),(#164156,#164157),(#164158,#164159),(#164160,#164161),
(#164162,#164163),(#164164,#164165),(#164166,#164167),(#164168,#164169),
(#164170,#164171),(#164172,#164173),(#164174,#164175),(#164176,#164177),
(#164178,#164179),(#164180,#164181),(#164182,#164183),(#164184,#164185),
(#164186,#164187),(#164188,#164189),(#164190,#164191),(#164192,#164193),
(#164194,#164195),(#164196,#164197),(#164198,#164199),(#164200,#164201),
(#164202,#164203),(#164204,#164205),(#164206,#164207),(#164208,#164209),
(#164210,#164211),(#164212,#164213),(#164214,#164215),(#164216,#164217),
(#164218,#164219),(#164220,#164221),(#164222,#164223),(#164224,#164225),
(#164226,#164227),(#164228,#164229),(#164230,#164231),(#164232,#164233),
(#164234,#164235),(#164236,#164237),(#164238,#164239),(#164240,#164241),
(#164242,#164243),(#164244,#164245),(#164246,#164247),(#164248,#164249),
(#164250,#164251),(#164252,#164253),(#164254,#164255),(#164256,#164257),
(#164258,#164259),(#164260,#164261),(#164262,#164263),(#164264,#164265),
(#164266,#164267),(#164268,#164269),(#164270,#164271),(#164272,#164273),
(#164274,#164275),(#164276,#164277),(#164278,#164279),(#164280,#164281),
(#164282,#164283),(#164284,#164285),(#164286,#164287),(#164288,#164289),
(#164290,#164291),(#164292,#164293),(#164294,#164295),(#164296,#164297),
(#164298,#164299),(#164300,#164301),(#164302,#164303),(#164304,#164305),
(#164306,#164307),(#164308,#164309),(#164310,#164311),(#164312,#164313),
(#164314,#164315),(#164316,#164317),(#164318,#164319),(#164320,#164321),
(#164322,#164323),(#164324,#164325),(#164326,#164327),(#164328,#164329),
(#164330,#164331),(#164332,#164333),(#164334,#164335),(#164336,#164337),
(#164338,#164339),(#164340,#164341),(#164342,#164343),(#164344,#164345),
(#164346,#164347),(#164348,#164349),(#164350,#164351),(#164352,#164353),
(#164354,#164355),(#164356,#164357),(#164358,#164359),(#164360,#164361),
(#164362,#164363),(#164364,#164365),(#164366,#164367),(#164368,#164369),
(#164370,#164371),(#164372,#164373),(#164374,#164375),(#164376,#164377),
(#164378,#164379),(#164380,#164381),(#164382,#164383),(#164384,#164385),
(#164386,#164387),(#164388,#164389),(#164390,#164391),(#164392,#164393),
(#164394,#164395),(#164396,#164397),(#164398,#164399),(#164400,#164401),
(#164402,#164403),(#164404,#164405),(#164406,#164407),(#164408,#164409),
(#164410,#164411),(#164412,#164413),(#164414,#164415),(#164416,#164417),
(#164418,#164419),(#164420,#164421),(#164422,#164423),(#164424,#164425),
(#164426,#164427),(#164428,#164429),(#164430,#164431),(#164432,#164433),
(#164434,#164435),(#164436,#164437),(#164438,#164439),(#164440,#164441),
(#164442,#164443),(#164444,#164445),(#164446,#164447),(#164448,#164449),
(#164450,#164451),(#164452,#164453),(#164454,#164455),(#164456,#164457),
(#164458,#164459),(#164460,#164461),(#164462,#164463),(#164464,#164465),
(#164466,#164467),(#164468,#164469),(#164470,#164471),(#164472,#164473),
(#164474,#164475),(#164476,#164477),(#164478,#164479),(#164480,#164481),
(#164482,#164483),(#164484,#164485),(#164486,#164487),(#164488,#164489),
(#164490,#164491),(#164492,#164493),(#164494,#164495),(#164496,#164497),
(#164498,#164499),(#164500,#164501),(#164502,#164503),(#164504,#164505),
(#164506,#164507),(#164508,#164509),(#164510,#164511),(#164512,#164513),
(#164514,#164515),(#164516,#164517),(#164518,#164519),(#164520,#164521),
(#164522,#164523),(#164524,#164525),(#164526,#164527),(#164528,#164529),
(#164530,#164531),(#164532,#164533),(#164534,#164535),(#164536,#164537),
(#164538,#164539),(#164540,#164541),(#164542,#164543),(#164544,#164545),
(#164546,#164547),(#164548,#164549),(#164550,#164551),(#164552,#164553),
(#164554,#164555),(#164556,#164557),(#164558,#164559),(#164560,#164561),
(#164562,#164563),(#164564,#164565),(#164566,#164567),(#164568,#164569),
(#164570,#164571),(#164572,#164573),(#164574,#164575),(#164576,#164577),
(#164578,#164579),(#164580,#164581),(#164582,#164583),(#164584,#164585),
(#164586,#164587),(#164588,#164589),(#164590,#164591),(#164592,#164593),
(#164594,#164595),(#164596,#164597),(#164598,#164599),(#164600,#164601),
(#164602,#164603),(#164604,#164605),(#164606,#164607),(#164608,#164609),
(#164610,#164611),(#164612,#164613),(#164614,#164615),(#164616,#164617),
(#164618,#164619),(#164620,#164621),(#164622,#164623),(#164624,#164625),
(#164626,#164627),(#164628,#164629),(#164630,#164631),(#164632,#164633),
(#164634,#164635),(#164636,#164637),(#164638,#164639),(#164640,#164641),
(#164642,#164643),(#164644,#164645),(#164646,#164647),(#164648,#164649),
(#164650,#164651),(#164652,#164653),(#164654,#164655),(#164656,#164657),
(#164658,#164659),(#164660,#164661),(#164662,#164663),(#164664,#164665),
(#164666,#164667),(#164668,#164669),(#164670,#164671),(#164672,#164673),
(#164674,#164675),(#164676,#164677),(#164678,#164679),(#164680,#164681),
(#164682,#164683),(#164684,#164685),(#164686,#164687),(#164688,#164689),
(#164690,#164691),(#164692,#164693),(#164694,#164695),(#164696,#164697),
(#164698,#164699),(#164700,#164701),(#164702,#164703),(#164704,#164705),
(#164706,#164707),(#164708,#164709),(#164710,#164711),(#164712,#164713),
(#164714,#164715),(#164716,#164717),(#164718,#164719),(#164720,#164721),
(#164722,#164723),(#164724,#164725),(#164726,#164727),(#164728,#164729),
(#164730,#164731),(#164732,#164733),(#164734,#164735),(#164736,#164737),
(#164738,#164739),(#164740,#164741),(#164742,#164743),(#164744,#164745),
(#164746,#164747),(#164748,#164749),(#164750,#164751),(#164752,#164753),
(#164754,#164755),(#164756,#164757),(#164758,#164759),(#164760,#164761),
(#164762,#164763),(#164764,#164765),(#164766,#164767),(#164768,#164769),
(#164770,#164771),(#164772,#164773),(#164774,#164775),(#164776,#164777),
(#164778,#164779),(#164780,#164781),(#164782,#164783),(#164784,#164785),
(#164786,#164787),(#164788,#164789),(#164790,#164791),(#164792,#164793),
(#164794,#164795),(#164796,#164797),(#164798,#164799),(#164800,#164801),
(#164802,#164803),(#164804,#164805),(#164806,#164807),(#164808,#164809),
(#164810,#164811),(#164812,#164813),(#164814,#164815),(#164816,#164817),
(#164818,#164819),(#164820,#164821),(#164822,#164823),(#164824,#164825),
(#164826,#164827),(#164828,#164829),(#164830,#164831),(#164832,#164833),
(#164834,#164835),(#164836,#164837),(#164838,#164839),(#164840,#164841),
(#164842,#164843),(#164844,#164845),(#164846,#164847),(#164848,#164849),
(#164850,#164851),(#164852,#164853),(#164854,#164855),(#164856,#164857),
(#164858,#164859),(#164860,#164861),(#164862,#164863),(#164864,#164865),
(#164866,#164867),(#164868,#164869),(#164870,#164871),(#164872,#164873),
(#164874,#164875),(#164876,#164877),(#164878,#164879),(#164880,#164881),
(#164882,#164883),(#164884,#164885),(#164886,#164887),(#164888,#164889),
(#164890,#164891),(#164892,#164893),(#164894,#164895),(#164896,#164897),
(#164898,#164899),(#164900,#164901),(#164902,#164903),(#164904,#164905),
(#164906,#164907),(#164908,#164909),(#164910,#164911),(#164912,#164913),
(#164914,#164915),(#164916,#164917),(#164918,#164919),(#164920,#164921),
(#164922,#164923),(#164924,#164925),(#164926,#164927),(#164928,#164929),
(#164930,#164931),(#164932,#164933),(#164934,#164935),(#164936,#164937),
(#164938,#164939),(#164940,#164941),(#164942,#164943),(#164944,#164945),
(#164946,#164947),(#164948,#164949),(#164950,#164951),(#164952,#164953),
(#164954,#164955),(#164956,#164957),(#164958,#164959),(#164960,#164961),
(#164962,#164963),(#164964,#164965),(#164966,#164967),(#164968,#164969),
(#164970,#164971),(#164972,#164973)),.UNSPECIFIED.,.F.,.F.,.F.,(6,1,1,1,
1,1,1,1,1,1,1,1,1,1,1,1,1,1,1,1,1,1,1,1,1,1,1,1,1,1,1,1,1,1,1,1,1,1,1,1,
1,1,1,1,1,1,1,1,1,1,1,1,1,1,1,1,1,1,1,1,1,1,1,1,1,1,1,1,1,1,1,1,1,1,1,1,
1,1,1,1,1,1,1,1,1,1,1,1,1,1,1,1,1,1,1,1,1,1,1,1,1,1,1,1,1,1,1,1,1,1,1,1,
1,1,1,1,1,1,1,1,1,1,1,1,1,1,1,1,1,1,1,1,1,1,1,1,1,1,1,1,1,1,1,1,1,1,1,1,
1,1,1,1,1,1,1,1,1,1,1,1,1,1,1,1,1,1,1,1,1,1,1,1,1,1,1,1,1,1,1,1,1,1,1,1,
1,1,1,1,1,1,1,1,1,1,1,1,1,1,1,1,1,1,1,1,1,1,1,1,1,1,1,1,1,1,1,1,1,1,1,1,
1,1,1,1,1,1,1,1,1,1,1,1,1,1,1,1,1,1,1,1,1,1,1,1,1,1,1,1,1,1,1,1,1,1,1,1,
1,1,1,1,1,1,1,1,1,1,1,1,1,1,1,1,1,1,1,1,1,1,1,1,1,1,1,1,1,1,1,1,1,1,1,1,
1,1,1,1,1,1,1,1,1,1,1,1,1,1,1,1,1,1,1,1,1,1,1,1,1,1,1,1,1,1,1,1,1,1,1,1,
1,1,1,1,1,1,1,1,1,1,1,1,1,1,1,1,1,1,1,1,1,1,1,1,1,1,1,1,1,1,1,1,1,1,1,1,
1,1,1,1,1,1,1,1,1,1,1,1,1,1,1,1,1,1,1,1,1,1,1,1,1,1,1,1,1,1,1,1,1,1,1,1,
1,1,1,1,1,1,1,1,1,1,1,1,1,1,1,1,1,1,1,1,1,1,1,1,1,1,1,1,1,1,1,1,1,1,1,1,
1,1,1,1,1,1,1,1,1,1,1,1,1,1,1,1,1,1,1,1,1,1,1,1,1,1,1,1,1,1,1,6),(2,2),
(-1.,-0.998165138,-0.996330275,-0.994495413,-0.99266055,-0.990825688,-0.988990826,
-0.987155963,-0.985321101,-0.983486239,-0.981651376,-0.979816514,-0.977981651,
-0.976146789,-0.974311927,-0.972477064,-0.970642202,-0.968807339,-0.966972477,
-0.965137615,-0.963302752,-0.96146789,-0.959633028,-0.957798165,-0.955963303,
-0.95412844,-0.952293578,-0.950458716,-0.948623853,-0.946788991,-0.944954128,
-0.943119266,-0.941284404,-0.939449541,-0.937614679,-0.935779817,-0.933944954,
-0.932110092,-0.930275229,-0.928440367,-0.926605505,-0.924770642,-0.92293578,
-0.921100917,-0.919266055,-0.917431193,-0.91559633,-0.913761468,-0.911926606,
-0.910091743,-0.908256881,-0.906422018,-0.904587156,-0.902752294,-0.900917431,
-0.899082569,-0.897247706,-0.895412844,-0.893577982,-0.891743119,-0.889908257,
-0.888073394,-0.886238532,-0.88440367,-0.882568807,-0.880733945,-0.878899083,
-0.87706422,-0.875229358,-0.873394495,-0.871559633,-0.869724771,-0.867889908,
-0.866055046,-0.864220183,-0.862385321,-0.860550459,-0.858715596,-0.856880734,
-0.855045872,-0.853211009,-0.851376147,-0.849541284,-0.847706422,-0.84587156,
-0.844036697,-0.842201835,-0.840366972,-0.83853211,-0.836697248,-0.834862385,
-0.833027523,-0.831192661,-0.829357798,-0.827522936,-0.825688073,-0.823853211,
-0.822018349,-0.820183486,-0.818348624,-0.816513761,-0.814678899,-0.812844037,
-0.811009174,-0.809174312,-0.80733945,-0.805504587,-0.803669725,-0.801834862,
-0.8,-0.798165138,-0.796330275,-0.794495413,-0.79266055,-0.790825688,-0.788990826,
-0.787155963,-0.785321101,-0.783486239,-0.781651376,-0.779816514,-0.777981651,
-0.776146789,-0.774311927,-0.772477064,-0.770642202,-0.768807339,-0.766972477,
-0.765137615,-0.763302752,-0.76146789,-0.759633028,-0.757798165,-0.755963303,
-0.75412844,-0.752293578,-0.750458716,-0.748623853,-0.746788991,-0.744954128,
-0.743119266,-0.741284404,-0.739449541,-0.737614679,-0.735779817,-0.733944954,
-0.732110092,-0.730275229,-0.728440367,-0.726605505,-0.724770642,-0.72293578,
-0.721100917,-0.719266055,-0.717431193,-0.71559633,-0.713761468,-0.711926606,
-0.710091743,-0.708256881,-0.706422018,-0.704587156,-0.702752294,-0.700917431,
-0.699082569,-0.697247706,-0.695412844,-0.693577982,-0.691743119,-0.689908257,
-0.688073394,-0.686238532,-0.68440367,-0.682568807,-0.680733945,-0.678899083,
-0.67706422,-0.675229358,-0.673394495,-0.671559633,-0.669724771,-0.667889908,
-0.666055046,-0.664220183,-0.662385321,-0.660550459,-0.658715596,-0.656880734,
-0.655045872,-0.653211009,-0.651376147,-0.649541284,-0.647706422,-0.64587156,
-0.644036697,-0.642201835,-0.640366972,-0.63853211,-0.636697248,-0.634862385,
-0.633027523,-0.631192661,-0.629357798,-0.627522936,-0.625688073,-0.623853211,
-0.622018349,-0.620183486,-0.618348624,-0.616513761,-0.614678899,-0.612844037,
-0.611009174,-0.609174312,-0.60733945,-0.605504587,-0.603669725,-0.601834862,
-0.6,-0.598165138,-0.596330275,-0.594495413,-0.59266055,-0.590825688,-0.588990826,
-0.587155963,-0.585321101,-0.583486239,-0.581651376,-0.579816514,-0.577981651,
-0.576146789,-0.574311927,-0.572477064,-0.570642202,-0.568807339,-0.566972477,
-0.565137615,-0.563302752,-0.56146789,-0.559633028,-0.557798165,-0.555963303,
-0.55412844,-0.552293578,-0.550458716,-0.548623853,-0.546788991,-0.544954128,
-0.543119266,-0.541284404,-0.539449541,-0.537614679,-0.535779817,-0.533944954,
-0.532110092,-0.530275229,-0.528440367,-0.526605505,-0.524770642,-0.52293578,
-0.521100917,-0.519266055,-0.517431193,-0.51559633,-0.513761468,-0.511926606,
-0.510091743,-0.508256881,-0.506422018,-0.504587156,-0.502752294,-0.500917431,
-0.499082569,-0.497247706,-0.495412844,-0.493577982,-0.491743119,-0.489908257,
-0.488073394,-0.486238532,-0.48440367,-0.482568807,-0.480733945,-0.478899083,
-0.47706422,-0.475229358,-0.473394495,-0.471559633,-0.469724771,-0.467889908,
-0.466055046,-0.464220183,-0.462385321,-0.460550459,-0.458715596,-0.456880734,
-0.455045872,-0.453211009,-0.451376147,-0.449541284,-0.447706422,-0.44587156,
-0.444036697,-0.442201835,-0.440366972,-0.43853211,-0.436697248,-0.434862385,
-0.433027523,-0.431192661,-0.429357798,-0.427522936,-0.425688073,-0.423853211,
-0.422018349,-0.420183486,-0.418348624,-0.416513761,-0.414678899,-0.412844037,
-0.411009174,-0.409174312,-0.40733945,-0.405504587,-0.403669725,-0.401834862,
-0.4,-0.398165138,-0.396330275,-0.394495413,-0.39266055,-0.390825688,-0.388990826,
-0.387155963,-0.385321101,-0.383486239,-0.381651376,-0.379816514,-0.377981651,
-0.376146789,-0.374311927,-0.372477064,-0.370642202,-0.368807339,-0.366972477,
-0.365137615,-0.363302752,-0.36146789,-0.359633028,-0.357798165,-0.355963303,
-0.35412844,-0.352293578,-0.350458716,-0.348623853,-0.346788991,-0.344954128,
-0.343119266,-0.341284404,-0.339449541,-0.337614679,-0.335779817,-0.333944954,
-0.332110092,-0.330275229,-0.328440367,-0.326605505,-0.324770642,-0.32293578,
-0.321100917,-0.319266055,-0.317431193,-0.31559633,-0.313761468,-0.311926606,
-0.310091743,-0.308256881,-0.306422018,-0.304587156,-0.302752294,-0.300917431,
-0.299082569,-0.297247706,-0.295412844,-0.293577982,-0.291743119,-0.289908257,
-0.288073394,-0.286238532,-0.28440367,-0.282568807,-0.280733945,-0.278899083,
-0.27706422,-0.275229358,-0.273394495,-0.271559633,-0.269724771,-0.267889908,
-0.266055046,-0.264220183,-0.262385321,-0.260550459,-0.258715596,-0.256880734,
-0.255045872,-0.253211009,-0.251376147,-0.249541284,-0.247706422,-0.24587156,
-0.244036697,-0.242201835,-0.240366972,-0.23853211,-0.236697248,-0.234862385,
-0.233027523,-0.231192661,-0.229357798,-0.227522936,-0.225688073,-0.223853211,
-0.222018349,-0.220183486,-0.218348624,-0.216513761,-0.214678899,-0.212844037,
-0.211009174,-0.209174312,-0.20733945,-0.205504587,-0.203669725,-0.201834862,
-0.2,-0.198165138,-0.196330275,-0.194495413,-0.19266055,-0.190825688,-0.188990826,
-0.187155963,-0.185321101,-0.183486239,-0.181651376,-0.179816514,-0.177981651,
-0.176146789,-0.174311927,-0.172477064,-0.170642202,-0.168807339,-0.166972477,
-0.165137615,-0.163302752,-0.16146789,-0.159633028,-0.157798165,-0.155963303,
-0.15412844,-0.152293578,-0.150458716,-0.148623853,-0.146788991,-0.144954128,
-0.143172103),(0.,0.36),.UNSPECIFIED.);
#6222=B_SPLINE_SURFACE_WITH_KNOTS('',5,1,((#165627,#165628),(#165629,#165630),
(#165631,#165632),(#165633,#165634),(#165635,#165636),(#165637,#165638),
(#165639,#165640),(#165641,#165642),(#165643,#165644),(#165645,#165646),
(#165647,#165648),(#165649,#165650),(#165651,#165652),(#165653,#165654),
(#165655,#165656),(#165657,#165658),(#165659,#165660),(#165661,#165662),
(#165663,#165664),(#165665,#165666),(#165667,#165668),(#165669,#165670),
(#165671,#165672),(#165673,#165674),(#165675,#165676),(#165677,#165678),
(#165679,#165680),(#165681,#165682),(#165683,#165684),(#165685,#165686),
(#165687,#165688),(#165689,#165690),(#165691,#165692),(#165693,#165694),
(#165695,#165696),(#165697,#165698),(#165699,#165700),(#165701,#165702),
(#165703,#165704),(#165705,#165706),(#165707,#165708),(#165709,#165710),
(#165711,#165712),(#165713,#165714),(#165715,#165716),(#165717,#165718),
(#165719,#165720),(#165721,#165722),(#165723,#165724),(#165725,#165726),
(#165727,#165728),(#165729,#165730),(#165731,#165732),(#165733,#165734),
(#165735,#165736),(#165737,#165738),(#165739,#165740),(#165741,#165742),
(#165743,#165744),(#165745,#165746),(#165747,#165748),(#165749,#165750),
(#165751,#165752),(#165753,#165754),(#165755,#165756),(#165757,#165758),
(#165759,#165760),(#165761,#165762),(#165763,#165764),(#165765,#165766),
(#165767,#165768),(#165769,#165770),(#165771,#165772),(#165773,#165774),
(#165775,#165776),(#165777,#165778),(#165779,#165780),(#165781,#165782),
(#165783,#165784),(#165785,#165786),(#165787,#165788),(#165789,#165790),
(#165791,#165792),(#165793,#165794),(#165795,#165796),(#165797,#165798),
(#165799,#165800),(#165801,#165802),(#165803,#165804),(#165805,#165806),
(#165807,#165808),(#165809,#165810),(#165811,#165812),(#165813,#165814),
(#165815,#165816),(#165817,#165818),(#165819,#165820),(#165821,#165822),
(#165823,#165824),(#165825,#165826),(#165827,#165828),(#165829,#165830),
(#165831,#165832),(#165833,#165834),(#165835,#165836),(#165837,#165838),
(#165839,#165840),(#165841,#165842),(#165843,#165844),(#165845,#165846),
(#165847,#165848),(#165849,#165850),(#165851,#165852),(#165853,#165854),
(#165855,#165856),(#165857,#165858),(#165859,#165860),(#165861,#165862),
(#165863,#165864),(#165865,#165866),(#165867,#165868),(#165869,#165870),
(#165871,#165872),(#165873,#165874),(#165875,#165876),(#165877,#165878),
(#165879,#165880),(#165881,#165882),(#165883,#165884),(#165885,#165886),
(#165887,#165888),(#165889,#165890),(#165891,#165892),(#165893,#165894),
(#165895,#165896),(#165897,#165898),(#165899,#165900),(#165901,#165902),
(#165903,#165904),(#165905,#165906),(#165907,#165908),(#165909,#165910),
(#165911,#165912),(#165913,#165914),(#165915,#165916),(#165917,#165918),
(#165919,#165920),(#165921,#165922),(#165923,#165924),(#165925,#165926),
(#165927,#165928),(#165929,#165930),(#165931,#165932),(#165933,#165934),
(#165935,#165936),(#165937,#165938),(#165939,#165940),(#165941,#165942),
(#165943,#165944),(#165945,#165946),(#165947,#165948),(#165949,#165950),
(#165951,#165952),(#165953,#165954),(#165955,#165956),(#165957,#165958),
(#165959,#165960),(#165961,#165962),(#165963,#165964),(#165965,#165966),
(#165967,#165968),(#165969,#165970),(#165971,#165972),(#165973,#165974),
(#165975,#165976),(#165977,#165978),(#165979,#165980),(#165981,#165982),
(#165983,#165984),(#165985,#165986),(#165987,#165988),(#165989,#165990),
(#165991,#165992),(#165993,#165994),(#165995,#165996),(#165997,#165998),
(#165999,#166000),(#166001,#166002),(#166003,#166004),(#166005,#166006),
(#166007,#166008),(#166009,#166010),(#166011,#166012),(#166013,#166014),
(#166015,#166016),(#166017,#166018),(#166019,#166020),(#166021,#166022),
(#166023,#166024),(#166025,#166026),(#166027,#166028),(#166029,#166030),
(#166031,#166032),(#166033,#166034),(#166035,#166036),(#166037,#166038),
(#166039,#166040),(#166041,#166042),(#166043,#166044),(#166045,#166046),
(#166047,#166048),(#166049,#166050),(#166051,#166052),(#166053,#166054),
(#166055,#166056),(#166057,#166058),(#166059,#166060),(#166061,#166062),
(#166063,#166064),(#166065,#166066),(#166067,#166068),(#166069,#166070),
(#166071,#166072),(#166073,#166074),(#166075,#166076),(#166077,#166078),
(#166079,#166080),(#166081,#166082),(#166083,#166084),(#166085,#166086),
(#166087,#166088),(#166089,#166090),(#166091,#166092),(#166093,#166094),
(#166095,#166096),(#166097,#166098),(#166099,#166100),(#166101,#166102),
(#166103,#166104),(#166105,#166106),(#166107,#166108),(#166109,#166110),
(#166111,#166112),(#166113,#166114),(#166115,#166116),(#166117,#166118),
(#166119,#166120),(#166121,#166122),(#166123,#166124),(#166125,#166126),
(#166127,#166128),(#166129,#166130),(#166131,#166132),(#166133,#166134),
(#166135,#166136),(#166137,#166138),(#166139,#166140),(#166141,#166142),
(#166143,#166144),(#166145,#166146),(#166147,#166148),(#166149,#166150),
(#166151,#166152),(#166153,#166154),(#166155,#166156),(#166157,#166158),
(#166159,#166160),(#166161,#166162),(#166163,#166164),(#166165,#166166),
(#166167,#166168),(#166169,#166170),(#166171,#166172),(#166173,#166174),
(#166175,#166176),(#166177,#166178),(#166179,#166180),(#166181,#166182),
(#166183,#166184),(#166185,#166186),(#166187,#166188),(#166189,#166190),
(#166191,#166192),(#166193,#166194),(#166195,#166196),(#166197,#166198),
(#166199,#166200),(#166201,#166202),(#166203,#166204),(#166205,#166206),
(#166207,#166208),(#166209,#166210),(#166211,#166212),(#166213,#166214),
(#166215,#166216),(#166217,#166218),(#166219,#166220),(#166221,#166222),
(#166223,#166224),(#166225,#166226),(#166227,#166228),(#166229,#166230),
(#166231,#166232),(#166233,#166234),(#166235,#166236),(#166237,#166238),
(#166239,#166240),(#166241,#166242),(#166243,#166244),(#166245,#166246),
(#166247,#166248),(#166249,#166250),(#166251,#166252),(#166253,#166254),
(#166255,#166256),(#166257,#166258),(#166259,#166260),(#166261,#166262),
(#166263,#166264),(#166265,#166266),(#166267,#166268),(#166269,#166270),
(#166271,#166272),(#166273,#166274),(#166275,#166276),(#166277,#166278),
(#166279,#166280),(#166281,#166282),(#166283,#166284),(#166285,#166286),
(#166287,#166288),(#166289,#166290),(#166291,#166292),(#166293,#166294),
(#166295,#166296),(#166297,#166298),(#166299,#166300),(#166301,#166302),
(#166303,#166304),(#166305,#166306),(#166307,#166308),(#166309,#166310),
(#166311,#166312),(#166313,#166314),(#166315,#166316),(#166317,#166318),
(#166319,#166320),(#166321,#166322),(#166323,#166324),(#166325,#166326),
(#166327,#166328),(#166329,#166330),(#166331,#166332),(#166333,#166334),
(#166335,#166336),(#166337,#166338),(#166339,#166340),(#166341,#166342),
(#166343,#166344),(#166345,#166346),(#166347,#166348),(#166349,#166350),
(#166351,#166352),(#166353,#166354),(#166355,#166356),(#166357,#166358),
(#166359,#166360),(#166361,#166362),(#166363,#166364),(#166365,#166366),
(#166367,#166368),(#166369,#166370),(#166371,#166372),(#166373,#166374),
(#166375,#166376),(#166377,#166378),(#166379,#166380),(#166381,#166382),
(#166383,#166384),(#166385,#166386),(#166387,#166388),(#166389,#166390),
(#166391,#166392),(#166393,#166394),(#166395,#166396),(#166397,#166398),
(#166399,#166400),(#166401,#166402),(#166403,#166404),(#166405,#166406),
(#166407,#166408),(#166409,#166410),(#166411,#166412),(#166413,#166414),
(#166415,#166416),(#166417,#166418),(#166419,#166420),(#166421,#166422),
(#166423,#166424),(#166425,#166426),(#166427,#166428),(#166429,#166430),
(#166431,#166432),(#166433,#166434),(#166435,#166436),(#166437,#166438),
(#166439,#166440),(#166441,#166442),(#166443,#166444),(#166445,#166446),
(#166447,#166448),(#166449,#166450),(#166451,#166452),(#166453,#166454),
(#166455,#166456),(#166457,#166458),(#166459,#166460),(#166461,#166462),
(#166463,#166464),(#166465,#166466),(#166467,#166468),(#166469,#166470),
(#166471,#166472),(#166473,#166474),(#166475,#166476),(#166477,#166478),
(#166479,#166480),(#166481,#166482),(#166483,#166484),(#166485,#166486),
(#166487,#166488),(#166489,#166490),(#166491,#166492),(#166493,#166494),
(#166495,#166496),(#166497,#166498),(#166499,#166500),(#166501,#166502),
(#166503,#166504),(#166505,#166506),(#166507,#166508),(#166509,#166510),
(#166511,#166512),(#166513,#166514),(#166515,#166516),(#166517,#166518),
(#166519,#166520),(#166521,#166522),(#166523,#166524),(#166525,#166526),
(#166527,#166528),(#166529,#166530),(#166531,#166532),(#166533,#166534),
(#166535,#166536),(#166537,#166538),(#166539,#166540),(#166541,#166542),
(#166543,#166544),(#166545,#166546),(#166547,#166548),(#166549,#166550),
(#166551,#166552),(#166553,#166554),(#166555,#166556),(#166557,#166558),
(#166559,#166560),(#166561,#166562),(#166563,#166564),(#166565,#166566),
(#166567,#166568),(#166569,#166570)),.UNSPECIFIED.,.F.,.F.,.F.,(6,1,1,1,
1,1,1,1,1,1,1,1,1,1,1,1,1,1,1,1,1,1,1,1,1,1,1,1,1,1,1,1,1,1,1,1,1,1,1,1,
1,1,1,1,1,1,1,1,1,1,1,1,1,1,1,1,1,1,1,1,1,1,1,1,1,1,1,1,1,1,1,1,1,1,1,1,
1,1,1,1,1,1,1,1,1,1,1,1,1,1,1,1,1,1,1,1,1,1,1,1,1,1,1,1,1,1,1,1,1,1,1,1,
1,1,1,1,1,1,1,1,1,1,1,1,1,1,1,1,1,1,1,1,1,1,1,1,1,1,1,1,1,1,1,1,1,1,1,1,
1,1,1,1,1,1,1,1,1,1,1,1,1,1,1,1,1,1,1,1,1,1,1,1,1,1,1,1,1,1,1,1,1,1,1,1,
1,1,1,1,1,1,1,1,1,1,1,1,1,1,1,1,1,1,1,1,1,1,1,1,1,1,1,1,1,1,1,1,1,1,1,1,
1,1,1,1,1,1,1,1,1,1,1,1,1,1,1,1,1,1,1,1,1,1,1,1,1,1,1,1,1,1,1,1,1,1,1,1,
1,1,1,1,1,1,1,1,1,1,1,1,1,1,1,1,1,1,1,1,1,1,1,1,1,1,1,1,1,1,1,1,1,1,1,1,
1,1,1,1,1,1,1,1,1,1,1,1,1,1,1,1,1,1,1,1,1,1,1,1,1,1,1,1,1,1,1,1,1,1,1,1,
1,1,1,1,1,1,1,1,1,1,1,1,1,1,1,1,1,1,1,1,1,1,1,1,1,1,1,1,1,1,1,1,1,1,1,1,
1,1,1,1,1,1,1,1,1,1,1,1,1,1,1,1,1,1,1,1,1,1,1,1,1,1,1,1,1,1,1,1,1,1,1,1,
1,1,1,1,1,1,1,1,1,1,1,1,1,1,1,1,1,1,1,1,1,1,1,1,1,1,1,1,1,1,1,1,1,1,1,1,
1,1,1,1,1,1,1,1,1,1,1,1,1,1,1,1,1,1,1,1,1,1,1,1,1,1,1,1,1,1,1,6),(2,2),
(0.143172103,0.144954128,0.146788991,0.148623853,0.150458716,0.152293578,
0.15412844,0.155963303,0.157798165,0.159633028,0.16146789,0.163302752,0.165137615,
0.166972477,0.168807339,0.170642202,0.172477064,0.174311927,0.176146789,
0.177981651,0.179816514,0.181651376,0.183486239,0.185321101,0.187155963,
0.188990826,0.190825688,0.19266055,0.194495413,0.196330275,0.198165138,
0.2,0.201834862,0.203669725,0.205504587,0.20733945,0.209174312,0.211009174,
0.212844037,0.214678899,0.216513761,0.218348624,0.220183486,0.222018349,
0.223853211,0.225688073,0.227522936,0.229357798,0.231192661,0.233027523,
0.234862385,0.236697248,0.23853211,0.240366972,0.242201835,0.244036697,
0.24587156,0.247706422,0.249541284,0.251376147,0.253211009,0.255045872,
0.256880734,0.258715596,0.260550459,0.262385321,0.264220183,0.266055046,
0.267889908,0.269724771,0.271559633,0.273394495,0.275229358,0.27706422,
0.278899083,0.280733945,0.282568807,0.28440367,0.286238532,0.288073394,
0.289908257,0.291743119,0.293577982,0.295412844,0.297247706,0.299082569,
0.300917431,0.302752294,0.304587156,0.306422018,0.308256881,0.310091743,
0.311926606,0.313761468,0.31559633,0.317431193,0.319266055,0.321100917,
0.32293578,0.324770642,0.326605505,0.328440367,0.330275229,0.332110092,
0.333944954,0.335779817,0.337614679,0.339449541,0.341284404,0.343119266,
0.344954128,0.346788991,0.348623853,0.350458716,0.352293578,0.35412844,
0.355963303,0.357798165,0.359633028,0.36146789,0.363302752,0.365137615,
0.366972477,0.368807339,0.370642202,0.372477064,0.374311927,0.376146789,
0.377981651,0.379816514,0.381651376,0.383486239,0.385321101,0.387155963,
0.388990826,0.390825688,0.39266055,0.394495413,0.396330275,0.398165138,
0.4,0.401834862,0.403669725,0.405504587,0.40733945,0.409174312,0.411009174,
0.412844037,0.414678899,0.416513761,0.418348624,0.420183486,0.422018349,
0.423853211,0.425688073,0.427522936,0.429357798,0.431192661,0.433027523,
0.434862385,0.436697248,0.43853211,0.440366972,0.442201835,0.444036697,
0.44587156,0.447706422,0.449541284,0.451376147,0.453211009,0.455045872,
0.456880734,0.458715596,0.460550459,0.462385321,0.464220183,0.466055046,
0.467889908,0.469724771,0.471559633,0.473394495,0.475229358,0.47706422,
0.478899083,0.480733945,0.482568807,0.48440367,0.486238532,0.488073394,
0.489908257,0.491743119,0.493577982,0.495412844,0.497247706,0.499082569,
0.500917431,0.502752294,0.504587156,0.506422018,0.508256881,0.510091743,
0.511926606,0.513761468,0.51559633,0.517431193,0.519266055,0.521100917,
0.52293578,0.524770642,0.526605505,0.528440367,0.530275229,0.532110092,
0.533944954,0.535779817,0.537614679,0.539449541,0.541284404,0.543119266,
0.544954128,0.546788991,0.548623853,0.550458716,0.552293578,0.55412844,
0.555963303,0.557798165,0.559633028,0.56146789,0.563302752,0.565137615,
0.566972477,0.568807339,0.570642202,0.572477064,0.574311927,0.576146789,
0.577981651,0.579816514,0.581651376,0.583486239,0.585321101,0.587155963,
0.588990826,0.590825688,0.59266055,0.594495413,0.596330275,0.598165138,
0.6,0.601834862,0.603669725,0.605504587,0.60733945,0.609174312,0.611009174,
0.612844037,0.614678899,0.616513761,0.618348624,0.620183486,0.622018349,
0.623853211,0.625688073,0.627522936,0.629357798,0.631192661,0.633027523,
0.634862385,0.636697248,0.63853211,0.640366972,0.642201835,0.644036697,
0.64587156,0.647706422,0.649541284,0.651376147,0.653211009,0.655045872,
0.656880734,0.658715596,0.660550459,0.662385321,0.664220183,0.666055046,
0.667889908,0.669724771,0.671559633,0.673394495,0.675229358,0.67706422,
0.678899083,0.680733945,0.682568807,0.68440367,0.686238532,0.688073394,
0.689908257,0.691743119,0.693577982,0.695412844,0.697247706,0.699082569,
0.700917431,0.702752294,0.704587156,0.706422018,0.708256881,0.710091743,
0.711926606,0.713761468,0.71559633,0.717431193,0.719266055,0.721100917,
0.72293578,0.724770642,0.726605505,0.728440367,0.730275229,0.732110092,
0.733944954,0.735779817,0.737614679,0.739449541,0.741284404,0.743119266,
0.744954128,0.746788991,0.748623853,0.750458716,0.752293578,0.75412844,
0.755963303,0.757798165,0.759633028,0.76146789,0.763302752,0.765137615,
0.766972477,0.768807339,0.770642202,0.772477064,0.774311927,0.776146789,
0.777981651,0.779816514,0.781651376,0.783486239,0.785321101,0.787155963,
0.788990826,0.790825688,0.79266055,0.794495413,0.796330275,0.798165138,
0.8,0.801834862,0.803669725,0.805504587,0.80733945,0.809174312,0.811009174,
0.812844037,0.814678899,0.816513761,0.818348624,0.820183486,0.822018349,
0.823853211,0.825688073,0.827522936,0.829357798,0.831192661,0.833027523,
0.834862385,0.836697248,0.83853211,0.840366972,0.842201835,0.844036697,
0.84587156,0.847706422,0.849541284,0.851376147,0.853211009,0.855045872,
0.856880734,0.858715596,0.860550459,0.862385321,0.864220183,0.866055046,
0.867889908,0.869724771,0.871559633,0.873394495,0.875229358,0.87706422,
0.878899083,0.880733945,0.882568807,0.88440367,0.886238532,0.888073394,
0.889908257,0.891743119,0.893577982,0.895412844,0.897247706,0.899082569,
0.900917431,0.902752294,0.904587156,0.906422018,0.908256881,0.910091743,
0.911926606,0.913761468,0.91559633,0.917431193,0.919266055,0.921100917,
0.92293578,0.924770642,0.926605505,0.928440367,0.930275229,0.932110092,
0.933944954,0.935779817,0.937614679,0.939449541,0.941284404,0.943119266,
0.944954128,0.946788991,0.948623853,0.950458716,0.952293578,0.95412844,
0.955963303,0.957798165,0.959633028,0.96146789,0.963302752,0.965137615,
0.966972477,0.968807339,0.970642202,0.972477064,0.974311927,0.976146789,
0.977981651,0.979816514,0.981651376,0.983486239,0.985321101,0.987155963,
0.988990826,0.990825688,0.99266055,0.994495413,0.996330275,0.998165138,
1.),(0.,0.36),.UNSPECIFIED.);
#6223=B_SPLINE_SURFACE_WITH_KNOTS('',5,1,((#167230,#167231),(#167232,#167233),
(#167234,#167235),(#167236,#167237),(#167238,#167239),(#167240,#167241),
(#167242,#167243),(#167244,#167245),(#167246,#167247),(#167248,#167249),
(#167250,#167251),(#167252,#167253),(#167254,#167255),(#167256,#167257),
(#167258,#167259),(#167260,#167261),(#167262,#167263),(#167264,#167265),
(#167266,#167267),(#167268,#167269),(#167270,#167271),(#167272,#167273),
(#167274,#167275),(#167276,#167277),(#167278,#167279),(#167280,#167281),
(#167282,#167283),(#167284,#167285),(#167286,#167287),(#167288,#167289),
(#167290,#167291),(#167292,#167293),(#167294,#167295),(#167296,#167297),
(#167298,#167299),(#167300,#167301),(#167302,#167303),(#167304,#167305),
(#167306,#167307),(#167308,#167309),(#167310,#167311),(#167312,#167313),
(#167314,#167315),(#167316,#167317),(#167318,#167319),(#167320,#167321),
(#167322,#167323),(#167324,#167325),(#167326,#167327),(#167328,#167329),
(#167330,#167331),(#167332,#167333),(#167334,#167335),(#167336,#167337),
(#167338,#167339),(#167340,#167341),(#167342,#167343),(#167344,#167345),
(#167346,#167347),(#167348,#167349),(#167350,#167351),(#167352,#167353),
(#167354,#167355),(#167356,#167357),(#167358,#167359),(#167360,#167361),
(#167362,#167363),(#167364,#167365),(#167366,#167367),(#167368,#167369),
(#167370,#167371),(#167372,#167373),(#167374,#167375),(#167376,#167377),
(#167378,#167379),(#167380,#167381),(#167382,#167383),(#167384,#167385),
(#167386,#167387),(#167388,#167389),(#167390,#167391),(#167392,#167393),
(#167394,#167395),(#167396,#167397),(#167398,#167399),(#167400,#167401),
(#167402,#167403),(#167404,#167405),(#167406,#167407),(#167408,#167409),
(#167410,#167411),(#167412,#167413),(#167414,#167415),(#167416,#167417),
(#167418,#167419),(#167420,#167421),(#167422,#167423),(#167424,#167425),
(#167426,#167427),(#167428,#167429),(#167430,#167431),(#167432,#167433),
(#167434,#167435),(#167436,#167437),(#167438,#167439),(#167440,#167441),
(#167442,#167443),(#167444,#167445),(#167446,#167447),(#167448,#167449),
(#167450,#167451),(#167452,#167453),(#167454,#167455),(#167456,#167457),
(#167458,#167459),(#167460,#167461),(#167462,#167463),(#167464,#167465),
(#167466,#167467),(#167468,#167469),(#167470,#167471),(#167472,#167473),
(#167474,#167475),(#167476,#167477),(#167478,#167479),(#167480,#167481),
(#167482,#167483),(#167484,#167485),(#167486,#167487),(#167488,#167489),
(#167490,#167491),(#167492,#167493),(#167494,#167495),(#167496,#167497),
(#167498,#167499),(#167500,#167501),(#167502,#167503),(#167504,#167505),
(#167506,#167507),(#167508,#167509),(#167510,#167511),(#167512,#167513),
(#167514,#167515),(#167516,#167517),(#167518,#167519),(#167520,#167521),
(#167522,#167523),(#167524,#167525),(#167526,#167527),(#167528,#167529),
(#167530,#167531),(#167532,#167533),(#167534,#167535),(#167536,#167537),
(#167538,#167539),(#167540,#167541),(#167542,#167543),(#167544,#167545),
(#167546,#167547),(#167548,#167549),(#167550,#167551),(#167552,#167553),
(#167554,#167555),(#167556,#167557),(#167558,#167559),(#167560,#167561),
(#167562,#167563),(#167564,#167565),(#167566,#167567),(#167568,#167569),
(#167570,#167571),(#167572,#167573),(#167574,#167575),(#167576,#167577),
(#167578,#167579),(#167580,#167581),(#167582,#167583),(#167584,#167585),
(#167586,#167587),(#167588,#167589),(#167590,#167591),(#167592,#167593),
(#167594,#167595),(#167596,#167597),(#167598,#167599),(#167600,#167601),
(#167602,#167603),(#167604,#167605),(#167606,#167607),(#167608,#167609),
(#167610,#167611),(#167612,#167613),(#167614,#167615),(#167616,#167617),
(#167618,#167619),(#167620,#167621),(#167622,#167623),(#167624,#167625),
(#167626,#167627),(#167628,#167629),(#167630,#167631),(#167632,#167633),
(#167634,#167635),(#167636,#167637),(#167638,#167639),(#167640,#167641),
(#167642,#167643),(#167644,#167645),(#167646,#167647),(#167648,#167649),
(#167650,#167651),(#167652,#167653),(#167654,#167655),(#167656,#167657),
(#167658,#167659),(#167660,#167661),(#167662,#167663),(#167664,#167665),
(#167666,#167667),(#167668,#167669),(#167670,#167671),(#167672,#167673),
(#167674,#167675),(#167676,#167677),(#167678,#167679),(#167680,#167681),
(#167682,#167683),(#167684,#167685),(#167686,#167687),(#167688,#167689),
(#167690,#167691),(#167692,#167693),(#167694,#167695),(#167696,#167697),
(#167698,#167699),(#167700,#167701),(#167702,#167703),(#167704,#167705),
(#167706,#167707),(#167708,#167709),(#167710,#167711),(#167712,#167713),
(#167714,#167715),(#167716,#167717),(#167718,#167719),(#167720,#167721),
(#167722,#167723),(#167724,#167725),(#167726,#167727),(#167728,#167729),
(#167730,#167731),(#167732,#167733),(#167734,#167735),(#167736,#167737),
(#167738,#167739),(#167740,#167741),(#167742,#167743),(#167744,#167745),
(#167746,#167747),(#167748,#167749),(#167750,#167751),(#167752,#167753),
(#167754,#167755),(#167756,#167757),(#167758,#167759),(#167760,#167761),
(#167762,#167763),(#167764,#167765),(#167766,#167767),(#167768,#167769),
(#167770,#167771),(#167772,#167773),(#167774,#167775),(#167776,#167777),
(#167778,#167779),(#167780,#167781),(#167782,#167783),(#167784,#167785),
(#167786,#167787),(#167788,#167789),(#167790,#167791),(#167792,#167793),
(#167794,#167795),(#167796,#167797),(#167798,#167799),(#167800,#167801),
(#167802,#167803),(#167804,#167805),(#167806,#167807),(#167808,#167809),
(#167810,#167811),(#167812,#167813),(#167814,#167815),(#167816,#167817),
(#167818,#167819),(#167820,#167821),(#167822,#167823),(#167824,#167825),
(#167826,#167827),(#167828,#167829),(#167830,#167831),(#167832,#167833),
(#167834,#167835),(#167836,#167837),(#167838,#167839),(#167840,#167841),
(#167842,#167843),(#167844,#167845),(#167846,#167847),(#167848,#167849),
(#167850,#167851),(#167852,#167853),(#167854,#167855),(#167856,#167857),
(#167858,#167859),(#167860,#167861),(#167862,#167863),(#167864,#167865),
(#167866,#167867),(#167868,#167869),(#167870,#167871),(#167872,#167873),
(#167874,#167875),(#167876,#167877),(#167878,#167879),(#167880,#167881),
(#167882,#167883),(#167884,#167885),(#167886,#167887),(#167888,#167889),
(#167890,#167891),(#167892,#167893),(#167894,#167895),(#167896,#167897),
(#167898,#167899),(#167900,#167901),(#167902,#167903),(#167904,#167905),
(#167906,#167907),(#167908,#167909),(#167910,#167911),(#167912,#167913),
(#167914,#167915),(#167916,#167917),(#167918,#167919),(#167920,#167921),
(#167922,#167923),(#167924,#167925),(#167926,#167927),(#167928,#167929),
(#167930,#167931),(#167932,#167933),(#167934,#167935),(#167936,#167937),
(#167938,#167939),(#167940,#167941),(#167942,#167943),(#167944,#167945),
(#167946,#167947),(#167948,#167949),(#167950,#167951),(#167952,#167953),
(#167954,#167955),(#167956,#167957),(#167958,#167959),(#167960,#167961),
(#167962,#167963),(#167964,#167965),(#167966,#167967),(#167968,#167969),
(#167970,#167971),(#167972,#167973),(#167974,#167975),(#167976,#167977),
(#167978,#167979),(#167980,#167981),(#167982,#167983),(#167984,#167985),
(#167986,#167987),(#167988,#167989),(#167990,#167991),(#167992,#167993),
(#167994,#167995),(#167996,#167997),(#167998,#167999),(#168000,#168001),
(#168002,#168003),(#168004,#168005),(#168006,#168007),(#168008,#168009),
(#168010,#168011),(#168012,#168013),(#168014,#168015),(#168016,#168017),
(#168018,#168019),(#168020,#168021),(#168022,#168023),(#168024,#168025),
(#168026,#168027),(#168028,#168029),(#168030,#168031),(#168032,#168033),
(#168034,#168035),(#168036,#168037),(#168038,#168039),(#168040,#168041),
(#168042,#168043),(#168044,#168045),(#168046,#168047),(#168048,#168049),
(#168050,#168051),(#168052,#168053),(#168054,#168055),(#168056,#168057),
(#168058,#168059),(#168060,#168061),(#168062,#168063),(#168064,#168065),
(#168066,#168067),(#168068,#168069),(#168070,#168071),(#168072,#168073),
(#168074,#168075),(#168076,#168077),(#168078,#168079),(#168080,#168081),
(#168082,#168083),(#168084,#168085),(#168086,#168087),(#168088,#168089),
(#168090,#168091),(#168092,#168093),(#168094,#168095),(#168096,#168097),
(#168098,#168099),(#168100,#168101),(#168102,#168103),(#168104,#168105),
(#168106,#168107),(#168108,#168109),(#168110,#168111),(#168112,#168113),
(#168114,#168115),(#168116,#168117),(#168118,#168119),(#168120,#168121),
(#168122,#168123),(#168124,#168125),(#168126,#168127),(#168128,#168129),
(#168130,#168131),(#168132,#168133),(#168134,#168135),(#168136,#168137),
(#168138,#168139),(#168140,#168141),(#168142,#168143),(#168144,#168145),
(#168146,#168147),(#168148,#168149),(#168150,#168151),(#168152,#168153),
(#168154,#168155),(#168156,#168157),(#168158,#168159),(#168160,#168161),
(#168162,#168163),(#168164,#168165),(#168166,#168167),(#168168,#168169),
(#168170,#168171),(#168172,#168173)),.UNSPECIFIED.,.F.,.F.,.F.,(6,1,1,1,
1,1,1,1,1,1,1,1,1,1,1,1,1,1,1,1,1,1,1,1,1,1,1,1,1,1,1,1,1,1,1,1,1,1,1,1,
1,1,1,1,1,1,1,1,1,1,1,1,1,1,1,1,1,1,1,1,1,1,1,1,1,1,1,1,1,1,1,1,1,1,1,1,
1,1,1,1,1,1,1,1,1,1,1,1,1,1,1,1,1,1,1,1,1,1,1,1,1,1,1,1,1,1,1,1,1,1,1,1,
1,1,1,1,1,1,1,1,1,1,1,1,1,1,1,1,1,1,1,1,1,1,1,1,1,1,1,1,1,1,1,1,1,1,1,1,
1,1,1,1,1,1,1,1,1,1,1,1,1,1,1,1,1,1,1,1,1,1,1,1,1,1,1,1,1,1,1,1,1,1,1,1,
1,1,1,1,1,1,1,1,1,1,1,1,1,1,1,1,1,1,1,1,1,1,1,1,1,1,1,1,1,1,1,1,1,1,1,1,
1,1,1,1,1,1,1,1,1,1,1,1,1,1,1,1,1,1,1,1,1,1,1,1,1,1,1,1,1,1,1,1,1,1,1,1,
1,1,1,1,1,1,1,1,1,1,1,1,1,1,1,1,1,1,1,1,1,1,1,1,1,1,1,1,1,1,1,1,1,1,1,1,
1,1,1,1,1,1,1,1,1,1,1,1,1,1,1,1,1,1,1,1,1,1,1,1,1,1,1,1,1,1,1,1,1,1,1,1,
1,1,1,1,1,1,1,1,1,1,1,1,1,1,1,1,1,1,1,1,1,1,1,1,1,1,1,1,1,1,1,1,1,1,1,1,
1,1,1,1,1,1,1,1,1,1,1,1,1,1,1,1,1,1,1,1,1,1,1,1,1,1,1,1,1,1,1,1,1,1,1,1,
1,1,1,1,1,1,1,1,1,1,1,1,1,1,1,1,1,1,1,1,1,1,1,1,1,1,1,1,1,1,1,1,1,1,1,1,
1,1,1,1,1,1,1,1,1,1,1,1,1,1,1,1,1,1,1,1,1,1,1,1,1,1,1,1,1,1,1,6),(2,2),
(0.143172103,0.144954128,0.146788991,0.148623853,0.150458716,0.152293578,
0.15412844,0.155963303,0.157798165,0.159633028,0.16146789,0.163302752,0.165137615,
0.166972477,0.168807339,0.170642202,0.172477064,0.174311927,0.176146789,
0.177981651,0.179816514,0.181651376,0.183486239,0.185321101,0.187155963,
0.188990826,0.190825688,0.19266055,0.194495413,0.196330275,0.198165138,
0.2,0.201834862,0.203669725,0.205504587,0.20733945,0.209174312,0.211009174,
0.212844037,0.214678899,0.216513761,0.218348624,0.220183486,0.222018349,
0.223853211,0.225688073,0.227522936,0.229357798,0.231192661,0.233027523,
0.234862385,0.236697248,0.23853211,0.240366972,0.242201835,0.244036697,
0.24587156,0.247706422,0.249541284,0.251376147,0.253211009,0.255045872,
0.256880734,0.258715596,0.260550459,0.262385321,0.264220183,0.266055046,
0.267889908,0.269724771,0.271559633,0.273394495,0.275229358,0.27706422,
0.278899083,0.280733945,0.282568807,0.28440367,0.286238532,0.288073394,
0.289908257,0.291743119,0.293577982,0.295412844,0.297247706,0.299082569,
0.300917431,0.302752294,0.304587156,0.306422018,0.308256881,0.310091743,
0.311926606,0.313761468,0.31559633,0.317431193,0.319266055,0.321100917,
0.32293578,0.324770642,0.326605505,0.328440367,0.330275229,0.332110092,
0.333944954,0.335779817,0.337614679,0.339449541,0.341284404,0.343119266,
0.344954128,0.346788991,0.348623853,0.350458716,0.352293578,0.35412844,
0.355963303,0.357798165,0.359633028,0.36146789,0.363302752,0.365137615,
0.366972477,0.368807339,0.370642202,0.372477064,0.374311927,0.376146789,
0.377981651,0.379816514,0.381651376,0.383486239,0.385321101,0.387155963,
0.388990826,0.390825688,0.39266055,0.394495413,0.396330275,0.398165138,
0.4,0.401834862,0.403669725,0.405504587,0.40733945,0.409174312,0.411009174,
0.412844037,0.414678899,0.416513761,0.418348624,0.420183486,0.422018349,
0.423853211,0.425688073,0.427522936,0.429357798,0.431192661,0.433027523,
0.434862385,0.436697248,0.43853211,0.440366972,0.442201835,0.444036697,
0.44587156,0.447706422,0.449541284,0.451376147,0.453211009,0.455045872,
0.456880734,0.458715596,0.460550459,0.462385321,0.464220183,0.466055046,
0.467889908,0.469724771,0.471559633,0.473394495,0.475229358,0.47706422,
0.478899083,0.480733945,0.482568807,0.48440367,0.486238532,0.488073394,
0.489908257,0.491743119,0.493577982,0.495412844,0.497247706,0.499082569,
0.500917431,0.502752294,0.504587156,0.506422018,0.508256881,0.510091743,
0.511926606,0.513761468,0.51559633,0.517431193,0.519266055,0.521100917,
0.52293578,0.524770642,0.526605505,0.528440367,0.530275229,0.532110092,
0.533944954,0.535779817,0.537614679,0.539449541,0.541284404,0.543119266,
0.544954128,0.546788991,0.548623853,0.550458716,0.552293578,0.55412844,
0.555963303,0.557798165,0.559633028,0.56146789,0.563302752,0.565137615,
0.566972477,0.568807339,0.570642202,0.572477064,0.574311927,0.576146789,
0.577981651,0.579816514,0.581651376,0.583486239,0.585321101,0.587155963,
0.588990826,0.590825688,0.59266055,0.594495413,0.596330275,0.598165138,
0.6,0.601834862,0.603669725,0.605504587,0.60733945,0.609174312,0.611009174,
0.612844037,0.614678899,0.616513761,0.618348624,0.620183486,0.622018349,
0.623853211,0.625688073,0.627522936,0.629357798,0.631192661,0.633027523,
0.634862385,0.636697248,0.63853211,0.640366972,0.642201835,0.644036697,
0.64587156,0.647706422,0.649541284,0.651376147,0.653211009,0.655045872,
0.656880734,0.658715596,0.660550459,0.662385321,0.664220183,0.666055046,
0.667889908,0.669724771,0.671559633,0.673394495,0.675229358,0.67706422,
0.678899083,0.680733945,0.682568807,0.68440367,0.686238532,0.688073394,
0.689908257,0.691743119,0.693577982,0.695412844,0.697247706,0.699082569,
0.700917431,0.702752294,0.704587156,0.706422018,0.708256881,0.710091743,
0.711926606,0.713761468,0.71559633,0.717431193,0.719266055,0.721100917,
0.72293578,0.724770642,0.726605505,0.728440367,0.730275229,0.732110092,
0.733944954,0.735779817,0.737614679,0.739449541,0.741284404,0.743119266,
0.744954128,0.746788991,0.748623853,0.750458716,0.752293578,0.75412844,
0.755963303,0.757798165,0.759633028,0.76146789,0.763302752,0.765137615,
0.766972477,0.768807339,0.770642202,0.772477064,0.774311927,0.776146789,
0.777981651,0.779816514,0.781651376,0.783486239,0.785321101,0.787155963,
0.788990826,0.790825688,0.79266055,0.794495413,0.796330275,0.798165138,
0.8,0.801834862,0.803669725,0.805504587,0.80733945,0.809174312,0.811009174,
0.812844037,0.814678899,0.816513761,0.818348624,0.820183486,0.822018349,
0.823853211,0.825688073,0.827522936,0.829357798,0.831192661,0.833027523,
0.834862385,0.836697248,0.83853211,0.840366972,0.842201835,0.844036697,
0.84587156,0.847706422,0.849541284,0.851376147,0.853211009,0.855045872,
0.856880734,0.858715596,0.860550459,0.862385321,0.864220183,0.866055046,
0.867889908,0.869724771,0.871559633,0.873394495,0.875229358,0.87706422,
0.878899083,0.880733945,0.882568807,0.88440367,0.886238532,0.888073394,
0.889908257,0.891743119,0.893577982,0.895412844,0.897247706,0.899082569,
0.900917431,0.902752294,0.904587156,0.906422018,0.908256881,0.910091743,
0.911926606,0.913761468,0.91559633,0.917431193,0.919266055,0.921100917,
0.92293578,0.924770642,0.926605505,0.928440367,0.930275229,0.932110092,
0.933944954,0.935779817,0.937614679,0.939449541,0.941284404,0.943119266,
0.944954128,0.946788991,0.948623853,0.950458716,0.952293578,0.95412844,
0.955963303,0.957798165,0.959633028,0.96146789,0.963302752,0.965137615,
0.966972477,0.968807339,0.970642202,0.972477064,0.974311927,0.976146789,
0.977981651,0.979816514,0.981651376,0.983486239,0.985321101,0.987155963,
0.988990826,0.990825688,0.99266055,0.994495413,0.996330275,0.998165138,
1.),(0.,0.36),.UNSPECIFIED.);
#6224=B_SPLINE_SURFACE_WITH_KNOTS('',5,1,((#169118,#169119),(#169120,#169121),
(#169122,#169123),(#169124,#169125),(#169126,#169127),(#169128,#169129),
(#169130,#169131),(#169132,#169133),(#169134,#169135),(#169136,#169137),
(#169138,#169139),(#169140,#169141),(#169142,#169143),(#169144,#169145),
(#169146,#169147),(#169148,#169149),(#169150,#169151),(#169152,#169153),
(#169154,#169155),(#169156,#169157),(#169158,#169159),(#169160,#169161),
(#169162,#169163),(#169164,#169165),(#169166,#169167),(#169168,#169169),
(#169170,#169171),(#169172,#169173),(#169174,#169175),(#169176,#169177),
(#169178,#169179),(#169180,#169181),(#169182,#169183),(#169184,#169185),
(#169186,#169187),(#169188,#169189),(#169190,#169191),(#169192,#169193),
(#169194,#169195),(#169196,#169197),(#169198,#169199),(#169200,#169201),
(#169202,#169203),(#169204,#169205),(#169206,#169207),(#169208,#169209),
(#169210,#169211),(#169212,#169213),(#169214,#169215),(#169216,#169217),
(#169218,#169219),(#169220,#169221),(#169222,#169223),(#169224,#169225),
(#169226,#169227),(#169228,#169229),(#169230,#169231),(#169232,#169233),
(#169234,#169235),(#169236,#169237),(#169238,#169239),(#169240,#169241),
(#169242,#169243),(#169244,#169245),(#169246,#169247),(#169248,#169249),
(#169250,#169251),(#169252,#169253),(#169254,#169255),(#169256,#169257),
(#169258,#169259),(#169260,#169261),(#169262,#169263),(#169264,#169265),
(#169266,#169267),(#169268,#169269),(#169270,#169271),(#169272,#169273),
(#169274,#169275),(#169276,#169277),(#169278,#169279),(#169280,#169281),
(#169282,#169283),(#169284,#169285),(#169286,#169287),(#169288,#169289),
(#169290,#169291),(#169292,#169293),(#169294,#169295),(#169296,#169297),
(#169298,#169299),(#169300,#169301),(#169302,#169303),(#169304,#169305),
(#169306,#169307),(#169308,#169309),(#169310,#169311),(#169312,#169313),
(#169314,#169315),(#169316,#169317),(#169318,#169319),(#169320,#169321),
(#169322,#169323),(#169324,#169325),(#169326,#169327),(#169328,#169329),
(#169330,#169331),(#169332,#169333),(#169334,#169335),(#169336,#169337),
(#169338,#169339),(#169340,#169341),(#169342,#169343),(#169344,#169345),
(#169346,#169347),(#169348,#169349),(#169350,#169351),(#169352,#169353),
(#169354,#169355),(#169356,#169357),(#169358,#169359),(#169360,#169361),
(#169362,#169363),(#169364,#169365),(#169366,#169367),(#169368,#169369),
(#169370,#169371),(#169372,#169373),(#169374,#169375),(#169376,#169377),
(#169378,#169379),(#169380,#169381),(#169382,#169383),(#169384,#169385),
(#169386,#169387),(#169388,#169389),(#169390,#169391),(#169392,#169393),
(#169394,#169395),(#169396,#169397),(#169398,#169399),(#169400,#169401),
(#169402,#169403),(#169404,#169405),(#169406,#169407),(#169408,#169409),
(#169410,#169411),(#169412,#169413),(#169414,#169415),(#169416,#169417),
(#169418,#169419),(#169420,#169421),(#169422,#169423),(#169424,#169425),
(#169426,#169427),(#169428,#169429),(#169430,#169431),(#169432,#169433),
(#169434,#169435),(#169436,#169437),(#169438,#169439),(#169440,#169441),
(#169442,#169443),(#169444,#169445),(#169446,#169447),(#169448,#169449),
(#169450,#169451),(#169452,#169453),(#169454,#169455),(#169456,#169457),
(#169458,#169459),(#169460,#169461),(#169462,#169463),(#169464,#169465),
(#169466,#169467),(#169468,#169469),(#169470,#169471),(#169472,#169473),
(#169474,#169475),(#169476,#169477),(#169478,#169479),(#169480,#169481),
(#169482,#169483),(#169484,#169485),(#169486,#169487),(#169488,#169489),
(#169490,#169491),(#169492,#169493),(#169494,#169495),(#169496,#169497),
(#169498,#169499),(#169500,#169501),(#169502,#169503),(#169504,#169505),
(#169506,#169507),(#169508,#169509),(#169510,#169511),(#169512,#169513),
(#169514,#169515),(#169516,#169517),(#169518,#169519),(#169520,#169521),
(#169522,#169523),(#169524,#169525),(#169526,#169527),(#169528,#169529),
(#169530,#169531),(#169532,#169533),(#169534,#169535),(#169536,#169537),
(#169538,#169539),(#169540,#169541),(#169542,#169543),(#169544,#169545),
(#169546,#169547),(#169548,#169549),(#169550,#169551),(#169552,#169553),
(#169554,#169555),(#169556,#169557),(#169558,#169559),(#169560,#169561),
(#169562,#169563),(#169564,#169565),(#169566,#169567),(#169568,#169569),
(#169570,#169571),(#169572,#169573),(#169574,#169575),(#169576,#169577),
(#169578,#169579),(#169580,#169581),(#169582,#169583),(#169584,#169585),
(#169586,#169587),(#169588,#169589),(#169590,#169591),(#169592,#169593),
(#169594,#169595),(#169596,#169597),(#169598,#169599),(#169600,#169601),
(#169602,#169603),(#169604,#169605),(#169606,#169607),(#169608,#169609),
(#169610,#169611),(#169612,#169613),(#169614,#169615),(#169616,#169617),
(#169618,#169619),(#169620,#169621),(#169622,#169623),(#169624,#169625),
(#169626,#169627),(#169628,#169629),(#169630,#169631),(#169632,#169633),
(#169634,#169635),(#169636,#169637),(#169638,#169639),(#169640,#169641),
(#169642,#169643),(#169644,#169645),(#169646,#169647),(#169648,#169649),
(#169650,#169651),(#169652,#169653),(#169654,#169655),(#169656,#169657),
(#169658,#169659),(#169660,#169661),(#169662,#169663),(#169664,#169665),
(#169666,#169667),(#169668,#169669),(#169670,#169671),(#169672,#169673),
(#169674,#169675),(#169676,#169677),(#169678,#169679),(#169680,#169681),
(#169682,#169683),(#169684,#169685),(#169686,#169687),(#169688,#169689),
(#169690,#169691),(#169692,#169693),(#169694,#169695),(#169696,#169697),
(#169698,#169699),(#169700,#169701),(#169702,#169703),(#169704,#169705),
(#169706,#169707),(#169708,#169709),(#169710,#169711),(#169712,#169713),
(#169714,#169715),(#169716,#169717),(#169718,#169719),(#169720,#169721),
(#169722,#169723),(#169724,#169725),(#169726,#169727),(#169728,#169729),
(#169730,#169731),(#169732,#169733),(#169734,#169735),(#169736,#169737),
(#169738,#169739),(#169740,#169741),(#169742,#169743),(#169744,#169745),
(#169746,#169747),(#169748,#169749),(#169750,#169751),(#169752,#169753),
(#169754,#169755),(#169756,#169757),(#169758,#169759),(#169760,#169761),
(#169762,#169763),(#169764,#169765),(#169766,#169767),(#169768,#169769),
(#169770,#169771),(#169772,#169773),(#169774,#169775),(#169776,#169777),
(#169778,#169779),(#169780,#169781),(#169782,#169783),(#169784,#169785),
(#169786,#169787),(#169788,#169789),(#169790,#169791),(#169792,#169793),
(#169794,#169795),(#169796,#169797),(#169798,#169799),(#169800,#169801),
(#169802,#169803),(#169804,#169805),(#169806,#169807),(#169808,#169809),
(#169810,#169811),(#169812,#169813),(#169814,#169815),(#169816,#169817),
(#169818,#169819),(#169820,#169821),(#169822,#169823),(#169824,#169825),
(#169826,#169827),(#169828,#169829),(#169830,#169831),(#169832,#169833),
(#169834,#169835),(#169836,#169837),(#169838,#169839),(#169840,#169841),
(#169842,#169843),(#169844,#169845),(#169846,#169847),(#169848,#169849),
(#169850,#169851),(#169852,#169853),(#169854,#169855),(#169856,#169857),
(#169858,#169859),(#169860,#169861),(#169862,#169863),(#169864,#169865),
(#169866,#169867),(#169868,#169869),(#169870,#169871),(#169872,#169873),
(#169874,#169875),(#169876,#169877),(#169878,#169879),(#169880,#169881),
(#169882,#169883),(#169884,#169885),(#169886,#169887),(#169888,#169889),
(#169890,#169891),(#169892,#169893),(#169894,#169895),(#169896,#169897),
(#169898,#169899),(#169900,#169901),(#169902,#169903),(#169904,#169905),
(#169906,#169907),(#169908,#169909),(#169910,#169911),(#169912,#169913),
(#169914,#169915),(#169916,#169917),(#169918,#169919),(#169920,#169921),
(#169922,#169923),(#169924,#169925),(#169926,#169927),(#169928,#169929),
(#169930,#169931),(#169932,#169933),(#169934,#169935),(#169936,#169937),
(#169938,#169939),(#169940,#169941),(#169942,#169943),(#169944,#169945),
(#169946,#169947),(#169948,#169949),(#169950,#169951),(#169952,#169953),
(#169954,#169955),(#169956,#169957),(#169958,#169959),(#169960,#169961),
(#169962,#169963),(#169964,#169965),(#169966,#169967),(#169968,#169969),
(#169970,#169971),(#169972,#169973),(#169974,#169975),(#169976,#169977),
(#169978,#169979),(#169980,#169981),(#169982,#169983),(#169984,#169985),
(#169986,#169987),(#169988,#169989),(#169990,#169991),(#169992,#169993),
(#169994,#169995),(#169996,#169997),(#169998,#169999),(#170000,#170001),
(#170002,#170003),(#170004,#170005),(#170006,#170007),(#170008,#170009),
(#170010,#170011),(#170012,#170013),(#170014,#170015),(#170016,#170017),
(#170018,#170019),(#170020,#170021),(#170022,#170023),(#170024,#170025),
(#170026,#170027),(#170028,#170029),(#170030,#170031),(#170032,#170033),
(#170034,#170035),(#170036,#170037),(#170038,#170039),(#170040,#170041),
(#170042,#170043),(#170044,#170045),(#170046,#170047),(#170048,#170049),
(#170050,#170051),(#170052,#170053),(#170054,#170055),(#170056,#170057),
(#170058,#170059),(#170060,#170061)),.UNSPECIFIED.,.F.,.F.,.F.,(6,1,1,1,
1,1,1,1,1,1,1,1,1,1,1,1,1,1,1,1,1,1,1,1,1,1,1,1,1,1,1,1,1,1,1,1,1,1,1,1,
1,1,1,1,1,1,1,1,1,1,1,1,1,1,1,1,1,1,1,1,1,1,1,1,1,1,1,1,1,1,1,1,1,1,1,1,
1,1,1,1,1,1,1,1,1,1,1,1,1,1,1,1,1,1,1,1,1,1,1,1,1,1,1,1,1,1,1,1,1,1,1,1,
1,1,1,1,1,1,1,1,1,1,1,1,1,1,1,1,1,1,1,1,1,1,1,1,1,1,1,1,1,1,1,1,1,1,1,1,
1,1,1,1,1,1,1,1,1,1,1,1,1,1,1,1,1,1,1,1,1,1,1,1,1,1,1,1,1,1,1,1,1,1,1,1,
1,1,1,1,1,1,1,1,1,1,1,1,1,1,1,1,1,1,1,1,1,1,1,1,1,1,1,1,1,1,1,1,1,1,1,1,
1,1,1,1,1,1,1,1,1,1,1,1,1,1,1,1,1,1,1,1,1,1,1,1,1,1,1,1,1,1,1,1,1,1,1,1,
1,1,1,1,1,1,1,1,1,1,1,1,1,1,1,1,1,1,1,1,1,1,1,1,1,1,1,1,1,1,1,1,1,1,1,1,
1,1,1,1,1,1,1,1,1,1,1,1,1,1,1,1,1,1,1,1,1,1,1,1,1,1,1,1,1,1,1,1,1,1,1,1,
1,1,1,1,1,1,1,1,1,1,1,1,1,1,1,1,1,1,1,1,1,1,1,1,1,1,1,1,1,1,1,1,1,1,1,1,
1,1,1,1,1,1,1,1,1,1,1,1,1,1,1,1,1,1,1,1,1,1,1,1,1,1,1,1,1,1,1,1,1,1,1,1,
1,1,1,1,1,1,1,1,1,1,1,1,1,1,1,1,1,1,1,1,1,1,1,1,1,1,1,1,1,1,1,1,1,1,1,1,
1,1,1,1,1,1,1,1,1,1,1,1,1,1,1,1,1,1,1,1,1,1,1,1,1,1,1,1,1,1,1,6),(2,2),
(-1.,-0.998165138,-0.996330275,-0.994495413,-0.99266055,-0.990825688,-0.988990826,
-0.987155963,-0.985321101,-0.983486239,-0.981651376,-0.979816514,-0.977981651,
-0.976146789,-0.974311927,-0.972477064,-0.970642202,-0.968807339,-0.966972477,
-0.965137615,-0.963302752,-0.96146789,-0.959633028,-0.957798165,-0.955963303,
-0.95412844,-0.952293578,-0.950458716,-0.948623853,-0.946788991,-0.944954128,
-0.943119266,-0.941284404,-0.939449541,-0.937614679,-0.935779817,-0.933944954,
-0.932110092,-0.930275229,-0.928440367,-0.926605505,-0.924770642,-0.92293578,
-0.921100917,-0.919266055,-0.917431193,-0.91559633,-0.913761468,-0.911926606,
-0.910091743,-0.908256881,-0.906422018,-0.904587156,-0.902752294,-0.900917431,
-0.899082569,-0.897247706,-0.895412844,-0.893577982,-0.891743119,-0.889908257,
-0.888073394,-0.886238532,-0.88440367,-0.882568807,-0.880733945,-0.878899083,
-0.87706422,-0.875229358,-0.873394495,-0.871559633,-0.869724771,-0.867889908,
-0.866055046,-0.864220183,-0.862385321,-0.860550459,-0.858715596,-0.856880734,
-0.855045872,-0.853211009,-0.851376147,-0.849541284,-0.847706422,-0.84587156,
-0.844036697,-0.842201835,-0.840366972,-0.83853211,-0.836697248,-0.834862385,
-0.833027523,-0.831192661,-0.829357798,-0.827522936,-0.825688073,-0.823853211,
-0.822018349,-0.820183486,-0.818348624,-0.816513761,-0.814678899,-0.812844037,
-0.811009174,-0.809174312,-0.80733945,-0.805504587,-0.803669725,-0.801834862,
-0.8,-0.798165138,-0.796330275,-0.794495413,-0.79266055,-0.790825688,-0.788990826,
-0.787155963,-0.785321101,-0.783486239,-0.781651376,-0.779816514,-0.777981651,
-0.776146789,-0.774311927,-0.772477064,-0.770642202,-0.768807339,-0.766972477,
-0.765137615,-0.763302752,-0.76146789,-0.759633028,-0.757798165,-0.755963303,
-0.75412844,-0.752293578,-0.750458716,-0.748623853,-0.746788991,-0.744954128,
-0.743119266,-0.741284404,-0.739449541,-0.737614679,-0.735779817,-0.733944954,
-0.732110092,-0.730275229,-0.728440367,-0.726605505,-0.724770642,-0.72293578,
-0.721100917,-0.719266055,-0.717431193,-0.71559633,-0.713761468,-0.711926606,
-0.710091743,-0.708256881,-0.706422018,-0.704587156,-0.702752294,-0.700917431,
-0.699082569,-0.697247706,-0.695412844,-0.693577982,-0.691743119,-0.689908257,
-0.688073394,-0.686238532,-0.68440367,-0.682568807,-0.680733945,-0.678899083,
-0.67706422,-0.675229358,-0.673394495,-0.671559633,-0.669724771,-0.667889908,
-0.666055046,-0.664220183,-0.662385321,-0.660550459,-0.658715596,-0.656880734,
-0.655045872,-0.653211009,-0.651376147,-0.649541284,-0.647706422,-0.64587156,
-0.644036697,-0.642201835,-0.640366972,-0.63853211,-0.636697248,-0.634862385,
-0.633027523,-0.631192661,-0.629357798,-0.627522936,-0.625688073,-0.623853211,
-0.622018349,-0.620183486,-0.618348624,-0.616513761,-0.614678899,-0.612844037,
-0.611009174,-0.609174312,-0.60733945,-0.605504587,-0.603669725,-0.601834862,
-0.6,-0.598165138,-0.596330275,-0.594495413,-0.59266055,-0.590825688,-0.588990826,
-0.587155963,-0.585321101,-0.583486239,-0.581651376,-0.579816514,-0.577981651,
-0.576146789,-0.574311927,-0.572477064,-0.570642202,-0.568807339,-0.566972477,
-0.565137615,-0.563302752,-0.56146789,-0.559633028,-0.557798165,-0.555963303,
-0.55412844,-0.552293578,-0.550458716,-0.548623853,-0.546788991,-0.544954128,
-0.543119266,-0.541284404,-0.539449541,-0.537614679,-0.535779817,-0.533944954,
-0.532110092,-0.530275229,-0.528440367,-0.526605505,-0.524770642,-0.52293578,
-0.521100917,-0.519266055,-0.517431193,-0.51559633,-0.513761468,-0.511926606,
-0.510091743,-0.508256881,-0.506422018,-0.504587156,-0.502752294,-0.500917431,
-0.499082569,-0.497247706,-0.495412844,-0.493577982,-0.491743119,-0.489908257,
-0.488073394,-0.486238532,-0.48440367,-0.482568807,-0.480733945,-0.478899083,
-0.47706422,-0.475229358,-0.473394495,-0.471559633,-0.469724771,-0.467889908,
-0.466055046,-0.464220183,-0.462385321,-0.460550459,-0.458715596,-0.456880734,
-0.455045872,-0.453211009,-0.451376147,-0.449541284,-0.447706422,-0.44587156,
-0.444036697,-0.442201835,-0.440366972,-0.43853211,-0.436697248,-0.434862385,
-0.433027523,-0.431192661,-0.429357798,-0.427522936,-0.425688073,-0.423853211,
-0.422018349,-0.420183486,-0.418348624,-0.416513761,-0.414678899,-0.412844037,
-0.411009174,-0.409174312,-0.40733945,-0.405504587,-0.403669725,-0.401834862,
-0.4,-0.398165138,-0.396330275,-0.394495413,-0.39266055,-0.390825688,-0.388990826,
-0.387155963,-0.385321101,-0.383486239,-0.381651376,-0.379816514,-0.377981651,
-0.376146789,-0.374311927,-0.372477064,-0.370642202,-0.368807339,-0.366972477,
-0.365137615,-0.363302752,-0.36146789,-0.359633028,-0.357798165,-0.355963303,
-0.35412844,-0.352293578,-0.350458716,-0.348623853,-0.346788991,-0.344954128,
-0.343119266,-0.341284404,-0.339449541,-0.337614679,-0.335779817,-0.333944954,
-0.332110092,-0.330275229,-0.328440367,-0.326605505,-0.324770642,-0.32293578,
-0.321100917,-0.319266055,-0.317431193,-0.31559633,-0.313761468,-0.311926606,
-0.310091743,-0.308256881,-0.306422018,-0.304587156,-0.302752294,-0.300917431,
-0.299082569,-0.297247706,-0.295412844,-0.293577982,-0.291743119,-0.289908257,
-0.288073394,-0.286238532,-0.28440367,-0.282568807,-0.280733945,-0.278899083,
-0.27706422,-0.275229358,-0.273394495,-0.271559633,-0.269724771,-0.267889908,
-0.266055046,-0.264220183,-0.262385321,-0.260550459,-0.258715596,-0.256880734,
-0.255045872,-0.253211009,-0.251376147,-0.249541284,-0.247706422,-0.24587156,
-0.244036697,-0.242201835,-0.240366972,-0.23853211,-0.236697248,-0.234862385,
-0.233027523,-0.231192661,-0.229357798,-0.227522936,-0.225688073,-0.223853211,
-0.222018349,-0.220183486,-0.218348624,-0.216513761,-0.214678899,-0.212844037,
-0.211009174,-0.209174312,-0.20733945,-0.205504587,-0.203669725,-0.201834862,
-0.2,-0.198165138,-0.196330275,-0.194495413,-0.19266055,-0.190825688,-0.188990826,
-0.187155963,-0.185321101,-0.183486239,-0.181651376,-0.179816514,-0.177981651,
-0.176146789,-0.174311927,-0.172477064,-0.170642202,-0.168807339,-0.166972477,
-0.165137615,-0.163302752,-0.16146789,-0.159633028,-0.157798165,-0.155963303,
-0.15412844,-0.152293578,-0.150458716,-0.148623853,-0.146788991,-0.144954128,
-0.143172103),(0.,0.36),.UNSPECIFIED.);
#6225=B_SPLINE_SURFACE_WITH_KNOTS('',5,1,((#171024,#171025),(#171026,#171027),
(#171028,#171029),(#171030,#171031),(#171032,#171033),(#171034,#171035),
(#171036,#171037),(#171038,#171039),(#171040,#171041),(#171042,#171043),
(#171044,#171045),(#171046,#171047),(#171048,#171049),(#171050,#171051),
(#171052,#171053),(#171054,#171055),(#171056,#171057),(#171058,#171059),
(#171060,#171061),(#171062,#171063),(#171064,#171065),(#171066,#171067),
(#171068,#171069),(#171070,#171071),(#171072,#171073),(#171074,#171075),
(#171076,#171077),(#171078,#171079),(#171080,#171081),(#171082,#171083),
(#171084,#171085),(#171086,#171087),(#171088,#171089),(#171090,#171091),
(#171092,#171093),(#171094,#171095),(#171096,#171097),(#171098,#171099),
(#171100,#171101),(#171102,#171103),(#171104,#171105),(#171106,#171107),
(#171108,#171109),(#171110,#171111),(#171112,#171113),(#171114,#171115),
(#171116,#171117),(#171118,#171119),(#171120,#171121),(#171122,#171123),
(#171124,#171125),(#171126,#171127),(#171128,#171129),(#171130,#171131),
(#171132,#171133),(#171134,#171135),(#171136,#171137),(#171138,#171139),
(#171140,#171141),(#171142,#171143),(#171144,#171145),(#171146,#171147),
(#171148,#171149),(#171150,#171151),(#171152,#171153),(#171154,#171155),
(#171156,#171157),(#171158,#171159),(#171160,#171161),(#171162,#171163),
(#171164,#171165),(#171166,#171167),(#171168,#171169),(#171170,#171171),
(#171172,#171173),(#171174,#171175),(#171176,#171177),(#171178,#171179),
(#171180,#171181),(#171182,#171183),(#171184,#171185),(#171186,#171187),
(#171188,#171189),(#171190,#171191),(#171192,#171193),(#171194,#171195),
(#171196,#171197),(#171198,#171199),(#171200,#171201),(#171202,#171203),
(#171204,#171205),(#171206,#171207),(#171208,#171209),(#171210,#171211),
(#171212,#171213),(#171214,#171215),(#171216,#171217),(#171218,#171219),
(#171220,#171221),(#171222,#171223),(#171224,#171225),(#171226,#171227),
(#171228,#171229),(#171230,#171231),(#171232,#171233),(#171234,#171235),
(#171236,#171237),(#171238,#171239),(#171240,#171241),(#171242,#171243),
(#171244,#171245),(#171246,#171247),(#171248,#171249),(#171250,#171251),
(#171252,#171253),(#171254,#171255),(#171256,#171257),(#171258,#171259),
(#171260,#171261),(#171262,#171263),(#171264,#171265),(#171266,#171267),
(#171268,#171269),(#171270,#171271),(#171272,#171273),(#171274,#171275),
(#171276,#171277),(#171278,#171279),(#171280,#171281),(#171282,#171283),
(#171284,#171285),(#171286,#171287),(#171288,#171289),(#171290,#171291),
(#171292,#171293),(#171294,#171295),(#171296,#171297),(#171298,#171299),
(#171300,#171301),(#171302,#171303),(#171304,#171305),(#171306,#171307),
(#171308,#171309),(#171310,#171311),(#171312,#171313),(#171314,#171315),
(#171316,#171317),(#171318,#171319),(#171320,#171321),(#171322,#171323),
(#171324,#171325),(#171326,#171327),(#171328,#171329),(#171330,#171331),
(#171332,#171333),(#171334,#171335),(#171336,#171337),(#171338,#171339),
(#171340,#171341),(#171342,#171343),(#171344,#171345),(#171346,#171347),
(#171348,#171349),(#171350,#171351),(#171352,#171353),(#171354,#171355),
(#171356,#171357),(#171358,#171359),(#171360,#171361),(#171362,#171363),
(#171364,#171365),(#171366,#171367),(#171368,#171369),(#171370,#171371),
(#171372,#171373),(#171374,#171375),(#171376,#171377),(#171378,#171379),
(#171380,#171381),(#171382,#171383),(#171384,#171385),(#171386,#171387),
(#171388,#171389),(#171390,#171391),(#171392,#171393),(#171394,#171395),
(#171396,#171397),(#171398,#171399),(#171400,#171401),(#171402,#171403),
(#171404,#171405),(#171406,#171407),(#171408,#171409),(#171410,#171411),
(#171412,#171413),(#171414,#171415),(#171416,#171417),(#171418,#171419),
(#171420,#171421),(#171422,#171423),(#171424,#171425),(#171426,#171427),
(#171428,#171429),(#171430,#171431),(#171432,#171433),(#171434,#171435),
(#171436,#171437),(#171438,#171439),(#171440,#171441),(#171442,#171443),
(#171444,#171445),(#171446,#171447),(#171448,#171449),(#171450,#171451),
(#171452,#171453),(#171454,#171455),(#171456,#171457),(#171458,#171459),
(#171460,#171461),(#171462,#171463),(#171464,#171465),(#171466,#171467),
(#171468,#171469),(#171470,#171471),(#171472,#171473),(#171474,#171475),
(#171476,#171477),(#171478,#171479),(#171480,#171481),(#171482,#171483),
(#171484,#171485),(#171486,#171487),(#171488,#171489),(#171490,#171491),
(#171492,#171493),(#171494,#171495),(#171496,#171497),(#171498,#171499),
(#171500,#171501),(#171502,#171503),(#171504,#171505),(#171506,#171507),
(#171508,#171509),(#171510,#171511),(#171512,#171513),(#171514,#171515),
(#171516,#171517),(#171518,#171519),(#171520,#171521),(#171522,#171523),
(#171524,#171525),(#171526,#171527),(#171528,#171529),(#171530,#171531),
(#171532,#171533),(#171534,#171535),(#171536,#171537),(#171538,#171539),
(#171540,#171541),(#171542,#171543),(#171544,#171545),(#171546,#171547),
(#171548,#171549),(#171550,#171551),(#171552,#171553),(#171554,#171555),
(#171556,#171557),(#171558,#171559),(#171560,#171561),(#171562,#171563),
(#171564,#171565),(#171566,#171567),(#171568,#171569),(#171570,#171571),
(#171572,#171573),(#171574,#171575),(#171576,#171577),(#171578,#171579),
(#171580,#171581),(#171582,#171583),(#171584,#171585),(#171586,#171587),
(#171588,#171589),(#171590,#171591),(#171592,#171593),(#171594,#171595),
(#171596,#171597),(#171598,#171599),(#171600,#171601),(#171602,#171603),
(#171604,#171605),(#171606,#171607),(#171608,#171609),(#171610,#171611),
(#171612,#171613),(#171614,#171615),(#171616,#171617),(#171618,#171619),
(#171620,#171621),(#171622,#171623),(#171624,#171625),(#171626,#171627),
(#171628,#171629),(#171630,#171631),(#171632,#171633),(#171634,#171635),
(#171636,#171637),(#171638,#171639),(#171640,#171641),(#171642,#171643),
(#171644,#171645),(#171646,#171647),(#171648,#171649),(#171650,#171651),
(#171652,#171653),(#171654,#171655),(#171656,#171657),(#171658,#171659),
(#171660,#171661),(#171662,#171663),(#171664,#171665),(#171666,#171667),
(#171668,#171669),(#171670,#171671),(#171672,#171673),(#171674,#171675),
(#171676,#171677),(#171678,#171679),(#171680,#171681),(#171682,#171683),
(#171684,#171685),(#171686,#171687),(#171688,#171689),(#171690,#171691),
(#171692,#171693),(#171694,#171695),(#171696,#171697),(#171698,#171699),
(#171700,#171701),(#171702,#171703),(#171704,#171705),(#171706,#171707),
(#171708,#171709),(#171710,#171711),(#171712,#171713),(#171714,#171715),
(#171716,#171717),(#171718,#171719),(#171720,#171721),(#171722,#171723),
(#171724,#171725),(#171726,#171727),(#171728,#171729),(#171730,#171731),
(#171732,#171733),(#171734,#171735),(#171736,#171737),(#171738,#171739),
(#171740,#171741),(#171742,#171743),(#171744,#171745),(#171746,#171747),
(#171748,#171749),(#171750,#171751),(#171752,#171753),(#171754,#171755),
(#171756,#171757),(#171758,#171759),(#171760,#171761),(#171762,#171763),
(#171764,#171765),(#171766,#171767),(#171768,#171769),(#171770,#171771),
(#171772,#171773),(#171774,#171775),(#171776,#171777),(#171778,#171779),
(#171780,#171781),(#171782,#171783),(#171784,#171785),(#171786,#171787),
(#171788,#171789),(#171790,#171791),(#171792,#171793),(#171794,#171795),
(#171796,#171797),(#171798,#171799),(#171800,#171801),(#171802,#171803),
(#171804,#171805),(#171806,#171807),(#171808,#171809),(#171810,#171811),
(#171812,#171813),(#171814,#171815),(#171816,#171817),(#171818,#171819),
(#171820,#171821),(#171822,#171823),(#171824,#171825),(#171826,#171827),
(#171828,#171829),(#171830,#171831),(#171832,#171833),(#171834,#171835),
(#171836,#171837),(#171838,#171839),(#171840,#171841),(#171842,#171843),
(#171844,#171845),(#171846,#171847),(#171848,#171849),(#171850,#171851),
(#171852,#171853),(#171854,#171855),(#171856,#171857),(#171858,#171859),
(#171860,#171861),(#171862,#171863),(#171864,#171865),(#171866,#171867),
(#171868,#171869),(#171870,#171871),(#171872,#171873),(#171874,#171875),
(#171876,#171877),(#171878,#171879),(#171880,#171881),(#171882,#171883),
(#171884,#171885),(#171886,#171887),(#171888,#171889),(#171890,#171891),
(#171892,#171893),(#171894,#171895),(#171896,#171897),(#171898,#171899),
(#171900,#171901),(#171902,#171903),(#171904,#171905),(#171906,#171907),
(#171908,#171909),(#171910,#171911),(#171912,#171913),(#171914,#171915),
(#171916,#171917),(#171918,#171919),(#171920,#171921),(#171922,#171923),
(#171924,#171925),(#171926,#171927),(#171928,#171929),(#171930,#171931),
(#171932,#171933),(#171934,#171935),(#171936,#171937),(#171938,#171939),
(#171940,#171941),(#171942,#171943),(#171944,#171945),(#171946,#171947),
(#171948,#171949),(#171950,#171951),(#171952,#171953),(#171954,#171955),
(#171956,#171957),(#171958,#171959),(#171960,#171961),(#171962,#171963),
(#171964,#171965),(#171966,#171967)),.UNSPECIFIED.,.F.,.F.,.F.,(6,1,1,1,
1,1,1,1,1,1,1,1,1,1,1,1,1,1,1,1,1,1,1,1,1,1,1,1,1,1,1,1,1,1,1,1,1,1,1,1,
1,1,1,1,1,1,1,1,1,1,1,1,1,1,1,1,1,1,1,1,1,1,1,1,1,1,1,1,1,1,1,1,1,1,1,1,
1,1,1,1,1,1,1,1,1,1,1,1,1,1,1,1,1,1,1,1,1,1,1,1,1,1,1,1,1,1,1,1,1,1,1,1,
1,1,1,1,1,1,1,1,1,1,1,1,1,1,1,1,1,1,1,1,1,1,1,1,1,1,1,1,1,1,1,1,1,1,1,1,
1,1,1,1,1,1,1,1,1,1,1,1,1,1,1,1,1,1,1,1,1,1,1,1,1,1,1,1,1,1,1,1,1,1,1,1,
1,1,1,1,1,1,1,1,1,1,1,1,1,1,1,1,1,1,1,1,1,1,1,1,1,1,1,1,1,1,1,1,1,1,1,1,
1,1,1,1,1,1,1,1,1,1,1,1,1,1,1,1,1,1,1,1,1,1,1,1,1,1,1,1,1,1,1,1,1,1,1,1,
1,1,1,1,1,1,1,1,1,1,1,1,1,1,1,1,1,1,1,1,1,1,1,1,1,1,1,1,1,1,1,1,1,1,1,1,
1,1,1,1,1,1,1,1,1,1,1,1,1,1,1,1,1,1,1,1,1,1,1,1,1,1,1,1,1,1,1,1,1,1,1,1,
1,1,1,1,1,1,1,1,1,1,1,1,1,1,1,1,1,1,1,1,1,1,1,1,1,1,1,1,1,1,1,1,1,1,1,1,
1,1,1,1,1,1,1,1,1,1,1,1,1,1,1,1,1,1,1,1,1,1,1,1,1,1,1,1,1,1,1,1,1,1,1,1,
1,1,1,1,1,1,1,1,1,1,1,1,1,1,1,1,1,1,1,1,1,1,1,1,1,1,1,1,1,1,1,1,1,1,1,1,
1,1,1,1,1,1,1,1,1,1,1,1,1,1,1,1,1,1,1,1,1,1,1,1,1,1,1,1,1,1,1,6),(2,2),
(-1.,-0.998165138,-0.996330275,-0.994495413,-0.99266055,-0.990825688,-0.988990826,
-0.987155963,-0.985321101,-0.983486239,-0.981651376,-0.979816514,-0.977981651,
-0.976146789,-0.974311927,-0.972477064,-0.970642202,-0.968807339,-0.966972477,
-0.965137615,-0.963302752,-0.96146789,-0.959633028,-0.957798165,-0.955963303,
-0.95412844,-0.952293578,-0.950458716,-0.948623853,-0.946788991,-0.944954128,
-0.943119266,-0.941284404,-0.939449541,-0.937614679,-0.935779817,-0.933944954,
-0.932110092,-0.930275229,-0.928440367,-0.926605505,-0.924770642,-0.92293578,
-0.921100917,-0.919266055,-0.917431193,-0.91559633,-0.913761468,-0.911926606,
-0.910091743,-0.908256881,-0.906422018,-0.904587156,-0.902752294,-0.900917431,
-0.899082569,-0.897247706,-0.895412844,-0.893577982,-0.891743119,-0.889908257,
-0.888073394,-0.886238532,-0.88440367,-0.882568807,-0.880733945,-0.878899083,
-0.87706422,-0.875229358,-0.873394495,-0.871559633,-0.869724771,-0.867889908,
-0.866055046,-0.864220183,-0.862385321,-0.860550459,-0.858715596,-0.856880734,
-0.855045872,-0.853211009,-0.851376147,-0.849541284,-0.847706422,-0.84587156,
-0.844036697,-0.842201835,-0.840366972,-0.83853211,-0.836697248,-0.834862385,
-0.833027523,-0.831192661,-0.829357798,-0.827522936,-0.825688073,-0.823853211,
-0.822018349,-0.820183486,-0.818348624,-0.816513761,-0.814678899,-0.812844037,
-0.811009174,-0.809174312,-0.80733945,-0.805504587,-0.803669725,-0.801834862,
-0.8,-0.798165138,-0.796330275,-0.794495413,-0.79266055,-0.790825688,-0.788990826,
-0.787155963,-0.785321101,-0.783486239,-0.781651376,-0.779816514,-0.777981651,
-0.776146789,-0.774311927,-0.772477064,-0.770642202,-0.768807339,-0.766972477,
-0.765137615,-0.763302752,-0.76146789,-0.759633028,-0.757798165,-0.755963303,
-0.75412844,-0.752293578,-0.750458716,-0.748623853,-0.746788991,-0.744954128,
-0.743119266,-0.741284404,-0.739449541,-0.737614679,-0.735779817,-0.733944954,
-0.732110092,-0.730275229,-0.728440367,-0.726605505,-0.724770642,-0.72293578,
-0.721100917,-0.719266055,-0.717431193,-0.71559633,-0.713761468,-0.711926606,
-0.710091743,-0.708256881,-0.706422018,-0.704587156,-0.702752294,-0.700917431,
-0.699082569,-0.697247706,-0.695412844,-0.693577982,-0.691743119,-0.689908257,
-0.688073394,-0.686238532,-0.68440367,-0.682568807,-0.680733945,-0.678899083,
-0.67706422,-0.675229358,-0.673394495,-0.671559633,-0.669724771,-0.667889908,
-0.666055046,-0.664220183,-0.662385321,-0.660550459,-0.658715596,-0.656880734,
-0.655045872,-0.653211009,-0.651376147,-0.649541284,-0.647706422,-0.64587156,
-0.644036697,-0.642201835,-0.640366972,-0.63853211,-0.636697248,-0.634862385,
-0.633027523,-0.631192661,-0.629357798,-0.627522936,-0.625688073,-0.623853211,
-0.622018349,-0.620183486,-0.618348624,-0.616513761,-0.614678899,-0.612844037,
-0.611009174,-0.609174312,-0.60733945,-0.605504587,-0.603669725,-0.601834862,
-0.6,-0.598165138,-0.596330275,-0.594495413,-0.59266055,-0.590825688,-0.588990826,
-0.587155963,-0.585321101,-0.583486239,-0.581651376,-0.579816514,-0.577981651,
-0.576146789,-0.574311927,-0.572477064,-0.570642202,-0.568807339,-0.566972477,
-0.565137615,-0.563302752,-0.56146789,-0.559633028,-0.557798165,-0.555963303,
-0.55412844,-0.552293578,-0.550458716,-0.548623853,-0.546788991,-0.544954128,
-0.543119266,-0.541284404,-0.539449541,-0.537614679,-0.535779817,-0.533944954,
-0.532110092,-0.530275229,-0.528440367,-0.526605505,-0.524770642,-0.52293578,
-0.521100917,-0.519266055,-0.517431193,-0.51559633,-0.513761468,-0.511926606,
-0.510091743,-0.508256881,-0.506422018,-0.504587156,-0.502752294,-0.500917431,
-0.499082569,-0.497247706,-0.495412844,-0.493577982,-0.491743119,-0.489908257,
-0.488073394,-0.486238532,-0.48440367,-0.482568807,-0.480733945,-0.478899083,
-0.47706422,-0.475229358,-0.473394495,-0.471559633,-0.469724771,-0.467889908,
-0.466055046,-0.464220183,-0.462385321,-0.460550459,-0.458715596,-0.456880734,
-0.455045872,-0.453211009,-0.451376147,-0.449541284,-0.447706422,-0.44587156,
-0.444036697,-0.442201835,-0.440366972,-0.43853211,-0.436697248,-0.434862385,
-0.433027523,-0.431192661,-0.429357798,-0.427522936,-0.425688073,-0.423853211,
-0.422018349,-0.420183486,-0.418348624,-0.416513761,-0.414678899,-0.412844037,
-0.411009174,-0.409174312,-0.40733945,-0.405504587,-0.403669725,-0.401834862,
-0.4,-0.398165138,-0.396330275,-0.394495413,-0.39266055,-0.390825688,-0.388990826,
-0.387155963,-0.385321101,-0.383486239,-0.381651376,-0.379816514,-0.377981651,
-0.376146789,-0.374311927,-0.372477064,-0.370642202,-0.368807339,-0.366972477,
-0.365137615,-0.363302752,-0.36146789,-0.359633028,-0.357798165,-0.355963303,
-0.35412844,-0.352293578,-0.350458716,-0.348623853,-0.346788991,-0.344954128,
-0.343119266,-0.341284404,-0.339449541,-0.337614679,-0.335779817,-0.333944954,
-0.332110092,-0.330275229,-0.328440367,-0.326605505,-0.324770642,-0.32293578,
-0.321100917,-0.319266055,-0.317431193,-0.31559633,-0.313761468,-0.311926606,
-0.310091743,-0.308256881,-0.306422018,-0.304587156,-0.302752294,-0.300917431,
-0.299082569,-0.297247706,-0.295412844,-0.293577982,-0.291743119,-0.289908257,
-0.288073394,-0.286238532,-0.28440367,-0.282568807,-0.280733945,-0.278899083,
-0.27706422,-0.275229358,-0.273394495,-0.271559633,-0.269724771,-0.267889908,
-0.266055046,-0.264220183,-0.262385321,-0.260550459,-0.258715596,-0.256880734,
-0.255045872,-0.253211009,-0.251376147,-0.249541284,-0.247706422,-0.24587156,
-0.244036697,-0.242201835,-0.240366972,-0.23853211,-0.236697248,-0.234862385,
-0.233027523,-0.231192661,-0.229357798,-0.227522936,-0.225688073,-0.223853211,
-0.222018349,-0.220183486,-0.218348624,-0.216513761,-0.214678899,-0.212844037,
-0.211009174,-0.209174312,-0.20733945,-0.205504587,-0.203669725,-0.201834862,
-0.2,-0.198165138,-0.196330275,-0.194495413,-0.19266055,-0.190825688,-0.188990826,
-0.187155963,-0.185321101,-0.183486239,-0.181651376,-0.179816514,-0.177981651,
-0.176146789,-0.174311927,-0.172477064,-0.170642202,-0.168807339,-0.166972477,
-0.165137615,-0.163302752,-0.16146789,-0.159633028,-0.157798165,-0.155963303,
-0.15412844,-0.152293578,-0.150458716,-0.148623853,-0.146788991,-0.144954128,
-0.143172103),(0.,0.36),.UNSPECIFIED.);
#6226=B_SPLINE_SURFACE_WITH_KNOTS('',5,1,((#172909,#172910),(#172911,#172912),
(#172913,#172914),(#172915,#172916),(#172917,#172918),(#172919,#172920),
(#172921,#172922),(#172923,#172924),(#172925,#172926),(#172927,#172928),
(#172929,#172930),(#172931,#172932),(#172933,#172934),(#172935,#172936),
(#172937,#172938),(#172939,#172940),(#172941,#172942),(#172943,#172944),
(#172945,#172946),(#172947,#172948),(#172949,#172950),(#172951,#172952),
(#172953,#172954),(#172955,#172956),(#172957,#172958),(#172959,#172960),
(#172961,#172962),(#172963,#172964),(#172965,#172966),(#172967,#172968),
(#172969,#172970),(#172971,#172972),(#172973,#172974),(#172975,#172976),
(#172977,#172978),(#172979,#172980),(#172981,#172982),(#172983,#172984),
(#172985,#172986),(#172987,#172988),(#172989,#172990),(#172991,#172992),
(#172993,#172994),(#172995,#172996),(#172997,#172998),(#172999,#173000),
(#173001,#173002),(#173003,#173004),(#173005,#173006),(#173007,#173008),
(#173009,#173010),(#173011,#173012),(#173013,#173014),(#173015,#173016),
(#173017,#173018),(#173019,#173020),(#173021,#173022),(#173023,#173024),
(#173025,#173026),(#173027,#173028),(#173029,#173030),(#173031,#173032),
(#173033,#173034),(#173035,#173036),(#173037,#173038),(#173039,#173040),
(#173041,#173042),(#173043,#173044),(#173045,#173046),(#173047,#173048),
(#173049,#173050),(#173051,#173052),(#173053,#173054),(#173055,#173056),
(#173057,#173058),(#173059,#173060),(#173061,#173062),(#173063,#173064),
(#173065,#173066),(#173067,#173068),(#173069,#173070),(#173071,#173072),
(#173073,#173074),(#173075,#173076),(#173077,#173078),(#173079,#173080),
(#173081,#173082),(#173083,#173084),(#173085,#173086),(#173087,#173088),
(#173089,#173090),(#173091,#173092),(#173093,#173094),(#173095,#173096),
(#173097,#173098),(#173099,#173100),(#173101,#173102),(#173103,#173104),
(#173105,#173106),(#173107,#173108),(#173109,#173110),(#173111,#173112),
(#173113,#173114),(#173115,#173116),(#173117,#173118),(#173119,#173120),
(#173121,#173122),(#173123,#173124),(#173125,#173126),(#173127,#173128),
(#173129,#173130),(#173131,#173132),(#173133,#173134),(#173135,#173136),
(#173137,#173138),(#173139,#173140),(#173141,#173142),(#173143,#173144),
(#173145,#173146),(#173147,#173148),(#173149,#173150),(#173151,#173152),
(#173153,#173154),(#173155,#173156),(#173157,#173158),(#173159,#173160),
(#173161,#173162),(#173163,#173164),(#173165,#173166),(#173167,#173168),
(#173169,#173170),(#173171,#173172),(#173173,#173174),(#173175,#173176),
(#173177,#173178),(#173179,#173180),(#173181,#173182),(#173183,#173184),
(#173185,#173186),(#173187,#173188),(#173189,#173190),(#173191,#173192),
(#173193,#173194),(#173195,#173196),(#173197,#173198),(#173199,#173200),
(#173201,#173202),(#173203,#173204),(#173205,#173206),(#173207,#173208),
(#173209,#173210),(#173211,#173212),(#173213,#173214),(#173215,#173216),
(#173217,#173218),(#173219,#173220),(#173221,#173222),(#173223,#173224),
(#173225,#173226),(#173227,#173228),(#173229,#173230),(#173231,#173232),
(#173233,#173234),(#173235,#173236),(#173237,#173238),(#173239,#173240),
(#173241,#173242),(#173243,#173244),(#173245,#173246),(#173247,#173248),
(#173249,#173250),(#173251,#173252),(#173253,#173254),(#173255,#173256),
(#173257,#173258),(#173259,#173260),(#173261,#173262),(#173263,#173264),
(#173265,#173266),(#173267,#173268),(#173269,#173270),(#173271,#173272),
(#173273,#173274),(#173275,#173276),(#173277,#173278),(#173279,#173280),
(#173281,#173282),(#173283,#173284),(#173285,#173286),(#173287,#173288),
(#173289,#173290),(#173291,#173292),(#173293,#173294),(#173295,#173296),
(#173297,#173298),(#173299,#173300),(#173301,#173302),(#173303,#173304),
(#173305,#173306),(#173307,#173308),(#173309,#173310),(#173311,#173312),
(#173313,#173314),(#173315,#173316),(#173317,#173318),(#173319,#173320),
(#173321,#173322),(#173323,#173324),(#173325,#173326),(#173327,#173328),
(#173329,#173330),(#173331,#173332),(#173333,#173334),(#173335,#173336),
(#173337,#173338),(#173339,#173340),(#173341,#173342),(#173343,#173344),
(#173345,#173346),(#173347,#173348),(#173349,#173350),(#173351,#173352),
(#173353,#173354),(#173355,#173356),(#173357,#173358),(#173359,#173360),
(#173361,#173362),(#173363,#173364),(#173365,#173366),(#173367,#173368),
(#173369,#173370),(#173371,#173372),(#173373,#173374),(#173375,#173376),
(#173377,#173378),(#173379,#173380),(#173381,#173382),(#173383,#173384),
(#173385,#173386),(#173387,#173388),(#173389,#173390),(#173391,#173392),
(#173393,#173394),(#173395,#173396),(#173397,#173398),(#173399,#173400),
(#173401,#173402),(#173403,#173404),(#173405,#173406),(#173407,#173408),
(#173409,#173410),(#173411,#173412),(#173413,#173414),(#173415,#173416),
(#173417,#173418),(#173419,#173420),(#173421,#173422),(#173423,#173424),
(#173425,#173426),(#173427,#173428),(#173429,#173430),(#173431,#173432),
(#173433,#173434),(#173435,#173436),(#173437,#173438),(#173439,#173440),
(#173441,#173442),(#173443,#173444),(#173445,#173446),(#173447,#173448),
(#173449,#173450),(#173451,#173452),(#173453,#173454),(#173455,#173456),
(#173457,#173458),(#173459,#173460),(#173461,#173462),(#173463,#173464),
(#173465,#173466),(#173467,#173468),(#173469,#173470),(#173471,#173472),
(#173473,#173474),(#173475,#173476),(#173477,#173478),(#173479,#173480),
(#173481,#173482),(#173483,#173484),(#173485,#173486),(#173487,#173488),
(#173489,#173490),(#173491,#173492),(#173493,#173494),(#173495,#173496),
(#173497,#173498),(#173499,#173500),(#173501,#173502),(#173503,#173504),
(#173505,#173506),(#173507,#173508),(#173509,#173510),(#173511,#173512),
(#173513,#173514),(#173515,#173516),(#173517,#173518),(#173519,#173520),
(#173521,#173522),(#173523,#173524),(#173525,#173526),(#173527,#173528),
(#173529,#173530),(#173531,#173532),(#173533,#173534),(#173535,#173536),
(#173537,#173538),(#173539,#173540),(#173541,#173542),(#173543,#173544),
(#173545,#173546),(#173547,#173548),(#173549,#173550),(#173551,#173552),
(#173553,#173554),(#173555,#173556),(#173557,#173558),(#173559,#173560),
(#173561,#173562),(#173563,#173564),(#173565,#173566),(#173567,#173568),
(#173569,#173570),(#173571,#173572),(#173573,#173574),(#173575,#173576),
(#173577,#173578),(#173579,#173580),(#173581,#173582),(#173583,#173584),
(#173585,#173586),(#173587,#173588),(#173589,#173590),(#173591,#173592),
(#173593,#173594),(#173595,#173596),(#173597,#173598),(#173599,#173600),
(#173601,#173602),(#173603,#173604),(#173605,#173606),(#173607,#173608),
(#173609,#173610),(#173611,#173612),(#173613,#173614),(#173615,#173616),
(#173617,#173618),(#173619,#173620),(#173621,#173622),(#173623,#173624),
(#173625,#173626),(#173627,#173628),(#173629,#173630),(#173631,#173632),
(#173633,#173634),(#173635,#173636),(#173637,#173638),(#173639,#173640),
(#173641,#173642),(#173643,#173644),(#173645,#173646),(#173647,#173648),
(#173649,#173650),(#173651,#173652),(#173653,#173654),(#173655,#173656),
(#173657,#173658),(#173659,#173660),(#173661,#173662),(#173663,#173664),
(#173665,#173666),(#173667,#173668),(#173669,#173670),(#173671,#173672),
(#173673,#173674),(#173675,#173676),(#173677,#173678),(#173679,#173680),
(#173681,#173682),(#173683,#173684),(#173685,#173686),(#173687,#173688),
(#173689,#173690),(#173691,#173692),(#173693,#173694),(#173695,#173696),
(#173697,#173698),(#173699,#173700),(#173701,#173702),(#173703,#173704),
(#173705,#173706),(#173707,#173708),(#173709,#173710),(#173711,#173712),
(#173713,#173714),(#173715,#173716),(#173717,#173718),(#173719,#173720),
(#173721,#173722),(#173723,#173724),(#173725,#173726),(#173727,#173728),
(#173729,#173730),(#173731,#173732),(#173733,#173734),(#173735,#173736),
(#173737,#173738),(#173739,#173740),(#173741,#173742),(#173743,#173744),
(#173745,#173746),(#173747,#173748),(#173749,#173750),(#173751,#173752),
(#173753,#173754),(#173755,#173756),(#173757,#173758),(#173759,#173760),
(#173761,#173762),(#173763,#173764),(#173765,#173766),(#173767,#173768),
(#173769,#173770),(#173771,#173772),(#173773,#173774),(#173775,#173776),
(#173777,#173778),(#173779,#173780),(#173781,#173782),(#173783,#173784),
(#173785,#173786),(#173787,#173788),(#173789,#173790),(#173791,#173792),
(#173793,#173794),(#173795,#173796),(#173797,#173798),(#173799,#173800),
(#173801,#173802),(#173803,#173804),(#173805,#173806),(#173807,#173808),
(#173809,#173810),(#173811,#173812),(#173813,#173814),(#173815,#173816),
(#173817,#173818),(#173819,#173820),(#173821,#173822),(#173823,#173824),
(#173825,#173826),(#173827,#173828),(#173829,#173830),(#173831,#173832),
(#173833,#173834),(#173835,#173836),(#173837,#173838),(#173839,#173840),
(#173841,#173842),(#173843,#173844),(#173845,#173846),(#173847,#173848),
(#173849,#173850),(#173851,#173852)),.UNSPECIFIED.,.F.,.F.,.F.,(6,1,1,1,
1,1,1,1,1,1,1,1,1,1,1,1,1,1,1,1,1,1,1,1,1,1,1,1,1,1,1,1,1,1,1,1,1,1,1,1,
1,1,1,1,1,1,1,1,1,1,1,1,1,1,1,1,1,1,1,1,1,1,1,1,1,1,1,1,1,1,1,1,1,1,1,1,
1,1,1,1,1,1,1,1,1,1,1,1,1,1,1,1,1,1,1,1,1,1,1,1,1,1,1,1,1,1,1,1,1,1,1,1,
1,1,1,1,1,1,1,1,1,1,1,1,1,1,1,1,1,1,1,1,1,1,1,1,1,1,1,1,1,1,1,1,1,1,1,1,
1,1,1,1,1,1,1,1,1,1,1,1,1,1,1,1,1,1,1,1,1,1,1,1,1,1,1,1,1,1,1,1,1,1,1,1,
1,1,1,1,1,1,1,1,1,1,1,1,1,1,1,1,1,1,1,1,1,1,1,1,1,1,1,1,1,1,1,1,1,1,1,1,
1,1,1,1,1,1,1,1,1,1,1,1,1,1,1,1,1,1,1,1,1,1,1,1,1,1,1,1,1,1,1,1,1,1,1,1,
1,1,1,1,1,1,1,1,1,1,1,1,1,1,1,1,1,1,1,1,1,1,1,1,1,1,1,1,1,1,1,1,1,1,1,1,
1,1,1,1,1,1,1,1,1,1,1,1,1,1,1,1,1,1,1,1,1,1,1,1,1,1,1,1,1,1,1,1,1,1,1,1,
1,1,1,1,1,1,1,1,1,1,1,1,1,1,1,1,1,1,1,1,1,1,1,1,1,1,1,1,1,1,1,1,1,1,1,1,
1,1,1,1,1,1,1,1,1,1,1,1,1,1,1,1,1,1,1,1,1,1,1,1,1,1,1,1,1,1,1,1,1,1,1,1,
1,1,1,1,1,1,1,1,1,1,1,1,1,1,1,1,1,1,1,1,1,1,1,1,1,1,1,1,1,1,1,1,1,1,1,1,
1,1,1,1,1,1,1,1,1,1,1,1,1,1,1,1,1,1,1,1,1,1,1,1,1,1,1,1,1,1,1,6),(2,2),
(0.143172103,0.144954128,0.146788991,0.148623853,0.150458716,0.152293578,
0.15412844,0.155963303,0.157798165,0.159633028,0.16146789,0.163302752,0.165137615,
0.166972477,0.168807339,0.170642202,0.172477064,0.174311927,0.176146789,
0.177981651,0.179816514,0.181651376,0.183486239,0.185321101,0.187155963,
0.188990826,0.190825688,0.19266055,0.194495413,0.196330275,0.198165138,
0.2,0.201834862,0.203669725,0.205504587,0.20733945,0.209174312,0.211009174,
0.212844037,0.214678899,0.216513761,0.218348624,0.220183486,0.222018349,
0.223853211,0.225688073,0.227522936,0.229357798,0.231192661,0.233027523,
0.234862385,0.236697248,0.23853211,0.240366972,0.242201835,0.244036697,
0.24587156,0.247706422,0.249541284,0.251376147,0.253211009,0.255045872,
0.256880734,0.258715596,0.260550459,0.262385321,0.264220183,0.266055046,
0.267889908,0.269724771,0.271559633,0.273394495,0.275229358,0.27706422,
0.278899083,0.280733945,0.282568807,0.28440367,0.286238532,0.288073394,
0.289908257,0.291743119,0.293577982,0.295412844,0.297247706,0.299082569,
0.300917431,0.302752294,0.304587156,0.306422018,0.308256881,0.310091743,
0.311926606,0.313761468,0.31559633,0.317431193,0.319266055,0.321100917,
0.32293578,0.324770642,0.326605505,0.328440367,0.330275229,0.332110092,
0.333944954,0.335779817,0.337614679,0.339449541,0.341284404,0.343119266,
0.344954128,0.346788991,0.348623853,0.350458716,0.352293578,0.35412844,
0.355963303,0.357798165,0.359633028,0.36146789,0.363302752,0.365137615,
0.366972477,0.368807339,0.370642202,0.372477064,0.374311927,0.376146789,
0.377981651,0.379816514,0.381651376,0.383486239,0.385321101,0.387155963,
0.388990826,0.390825688,0.39266055,0.394495413,0.396330275,0.398165138,
0.4,0.401834862,0.403669725,0.405504587,0.40733945,0.409174312,0.411009174,
0.412844037,0.414678899,0.416513761,0.418348624,0.420183486,0.422018349,
0.423853211,0.425688073,0.427522936,0.429357798,0.431192661,0.433027523,
0.434862385,0.436697248,0.43853211,0.440366972,0.442201835,0.444036697,
0.44587156,0.447706422,0.449541284,0.451376147,0.453211009,0.455045872,
0.456880734,0.458715596,0.460550459,0.462385321,0.464220183,0.466055046,
0.467889908,0.469724771,0.471559633,0.473394495,0.475229358,0.47706422,
0.478899083,0.480733945,0.482568807,0.48440367,0.486238532,0.488073394,
0.489908257,0.491743119,0.493577982,0.495412844,0.497247706,0.499082569,
0.500917431,0.502752294,0.504587156,0.506422018,0.508256881,0.510091743,
0.511926606,0.513761468,0.51559633,0.517431193,0.519266055,0.521100917,
0.52293578,0.524770642,0.526605505,0.528440367,0.530275229,0.532110092,
0.533944954,0.535779817,0.537614679,0.539449541,0.541284404,0.543119266,
0.544954128,0.546788991,0.548623853,0.550458716,0.552293578,0.55412844,
0.555963303,0.557798165,0.559633028,0.56146789,0.563302752,0.565137615,
0.566972477,0.568807339,0.570642202,0.572477064,0.574311927,0.576146789,
0.577981651,0.579816514,0.581651376,0.583486239,0.585321101,0.587155963,
0.588990826,0.590825688,0.59266055,0.594495413,0.596330275,0.598165138,
0.6,0.601834862,0.603669725,0.605504587,0.60733945,0.609174312,0.611009174,
0.612844037,0.614678899,0.616513761,0.618348624,0.620183486,0.622018349,
0.623853211,0.625688073,0.627522936,0.629357798,0.631192661,0.633027523,
0.634862385,0.636697248,0.63853211,0.640366972,0.642201835,0.644036697,
0.64587156,0.647706422,0.649541284,0.651376147,0.653211009,0.655045872,
0.656880734,0.658715596,0.660550459,0.662385321,0.664220183,0.666055046,
0.667889908,0.669724771,0.671559633,0.673394495,0.675229358,0.67706422,
0.678899083,0.680733945,0.682568807,0.68440367,0.686238532,0.688073394,
0.689908257,0.691743119,0.693577982,0.695412844,0.697247706,0.699082569,
0.700917431,0.702752294,0.704587156,0.706422018,0.708256881,0.710091743,
0.711926606,0.713761468,0.71559633,0.717431193,0.719266055,0.721100917,
0.72293578,0.724770642,0.726605505,0.728440367,0.730275229,0.732110092,
0.733944954,0.735779817,0.737614679,0.739449541,0.741284404,0.743119266,
0.744954128,0.746788991,0.748623853,0.750458716,0.752293578,0.75412844,
0.755963303,0.757798165,0.759633028,0.76146789,0.763302752,0.765137615,
0.766972477,0.768807339,0.770642202,0.772477064,0.774311927,0.776146789,
0.777981651,0.779816514,0.781651376,0.783486239,0.785321101,0.787155963,
0.788990826,0.790825688,0.79266055,0.794495413,0.796330275,0.798165138,
0.8,0.801834862,0.803669725,0.805504587,0.80733945,0.809174312,0.811009174,
0.812844037,0.814678899,0.816513761,0.818348624,0.820183486,0.822018349,
0.823853211,0.825688073,0.827522936,0.829357798,0.831192661,0.833027523,
0.834862385,0.836697248,0.83853211,0.840366972,0.842201835,0.844036697,
0.84587156,0.847706422,0.849541284,0.851376147,0.853211009,0.855045872,
0.856880734,0.858715596,0.860550459,0.862385321,0.864220183,0.866055046,
0.867889908,0.869724771,0.871559633,0.873394495,0.875229358,0.87706422,
0.878899083,0.880733945,0.882568807,0.88440367,0.886238532,0.888073394,
0.889908257,0.891743119,0.893577982,0.895412844,0.897247706,0.899082569,
0.900917431,0.902752294,0.904587156,0.906422018,0.908256881,0.910091743,
0.911926606,0.913761468,0.91559633,0.917431193,0.919266055,0.921100917,
0.92293578,0.924770642,0.926605505,0.928440367,0.930275229,0.932110092,
0.933944954,0.935779817,0.937614679,0.939449541,0.941284404,0.943119266,
0.944954128,0.946788991,0.948623853,0.950458716,0.952293578,0.95412844,
0.955963303,0.957798165,0.959633028,0.96146789,0.963302752,0.965137615,
0.966972477,0.968807339,0.970642202,0.972477064,0.974311927,0.976146789,
0.977981651,0.979816514,0.981651376,0.983486239,0.985321101,0.987155963,
0.988990826,0.990825688,0.99266055,0.994495413,0.996330275,0.998165138,
1.),(0.,0.36),.UNSPECIFIED.);
#6227=B_SPLINE_SURFACE_WITH_KNOTS('',5,1,((#174512,#174513),(#174514,#174515),
(#174516,#174517),(#174518,#174519),(#174520,#174521),(#174522,#174523),
(#174524,#174525),(#174526,#174527),(#174528,#174529),(#174530,#174531),
(#174532,#174533),(#174534,#174535),(#174536,#174537),(#174538,#174539),
(#174540,#174541),(#174542,#174543),(#174544,#174545),(#174546,#174547),
(#174548,#174549),(#174550,#174551),(#174552,#174553),(#174554,#174555),
(#174556,#174557),(#174558,#174559),(#174560,#174561),(#174562,#174563),
(#174564,#174565),(#174566,#174567),(#174568,#174569),(#174570,#174571),
(#174572,#174573),(#174574,#174575),(#174576,#174577),(#174578,#174579),
(#174580,#174581),(#174582,#174583),(#174584,#174585),(#174586,#174587),
(#174588,#174589),(#174590,#174591),(#174592,#174593),(#174594,#174595),
(#174596,#174597),(#174598,#174599),(#174600,#174601),(#174602,#174603),
(#174604,#174605),(#174606,#174607),(#174608,#174609),(#174610,#174611),
(#174612,#174613),(#174614,#174615),(#174616,#174617),(#174618,#174619),
(#174620,#174621),(#174622,#174623),(#174624,#174625),(#174626,#174627),
(#174628,#174629),(#174630,#174631),(#174632,#174633),(#174634,#174635),
(#174636,#174637),(#174638,#174639),(#174640,#174641),(#174642,#174643),
(#174644,#174645),(#174646,#174647),(#174648,#174649),(#174650,#174651),
(#174652,#174653),(#174654,#174655),(#174656,#174657),(#174658,#174659),
(#174660,#174661),(#174662,#174663),(#174664,#174665),(#174666,#174667),
(#174668,#174669),(#174670,#174671),(#174672,#174673),(#174674,#174675),
(#174676,#174677),(#174678,#174679),(#174680,#174681),(#174682,#174683),
(#174684,#174685),(#174686,#174687),(#174688,#174689),(#174690,#174691),
(#174692,#174693),(#174694,#174695),(#174696,#174697),(#174698,#174699),
(#174700,#174701),(#174702,#174703),(#174704,#174705),(#174706,#174707),
(#174708,#174709),(#174710,#174711),(#174712,#174713),(#174714,#174715),
(#174716,#174717),(#174718,#174719),(#174720,#174721),(#174722,#174723),
(#174724,#174725),(#174726,#174727),(#174728,#174729),(#174730,#174731),
(#174732,#174733),(#174734,#174735),(#174736,#174737),(#174738,#174739),
(#174740,#174741),(#174742,#174743),(#174744,#174745),(#174746,#174747),
(#174748,#174749),(#174750,#174751),(#174752,#174753),(#174754,#174755),
(#174756,#174757),(#174758,#174759),(#174760,#174761),(#174762,#174763),
(#174764,#174765),(#174766,#174767),(#174768,#174769),(#174770,#174771),
(#174772,#174773),(#174774,#174775),(#174776,#174777),(#174778,#174779),
(#174780,#174781),(#174782,#174783),(#174784,#174785),(#174786,#174787),
(#174788,#174789),(#174790,#174791),(#174792,#174793),(#174794,#174795),
(#174796,#174797),(#174798,#174799),(#174800,#174801),(#174802,#174803),
(#174804,#174805),(#174806,#174807),(#174808,#174809),(#174810,#174811),
(#174812,#174813),(#174814,#174815),(#174816,#174817),(#174818,#174819),
(#174820,#174821),(#174822,#174823),(#174824,#174825),(#174826,#174827),
(#174828,#174829),(#174830,#174831),(#174832,#174833),(#174834,#174835),
(#174836,#174837),(#174838,#174839),(#174840,#174841),(#174842,#174843),
(#174844,#174845),(#174846,#174847),(#174848,#174849),(#174850,#174851),
(#174852,#174853),(#174854,#174855),(#174856,#174857),(#174858,#174859),
(#174860,#174861),(#174862,#174863),(#174864,#174865),(#174866,#174867),
(#174868,#174869),(#174870,#174871),(#174872,#174873),(#174874,#174875),
(#174876,#174877),(#174878,#174879),(#174880,#174881),(#174882,#174883),
(#174884,#174885),(#174886,#174887),(#174888,#174889),(#174890,#174891),
(#174892,#174893),(#174894,#174895),(#174896,#174897),(#174898,#174899),
(#174900,#174901),(#174902,#174903),(#174904,#174905),(#174906,#174907),
(#174908,#174909),(#174910,#174911),(#174912,#174913),(#174914,#174915),
(#174916,#174917),(#174918,#174919),(#174920,#174921),(#174922,#174923),
(#174924,#174925),(#174926,#174927),(#174928,#174929),(#174930,#174931),
(#174932,#174933),(#174934,#174935),(#174936,#174937),(#174938,#174939),
(#174940,#174941),(#174942,#174943),(#174944,#174945),(#174946,#174947),
(#174948,#174949),(#174950,#174951),(#174952,#174953),(#174954,#174955),
(#174956,#174957),(#174958,#174959),(#174960,#174961),(#174962,#174963),
(#174964,#174965),(#174966,#174967),(#174968,#174969),(#174970,#174971),
(#174972,#174973),(#174974,#174975),(#174976,#174977),(#174978,#174979),
(#174980,#174981),(#174982,#174983),(#174984,#174985),(#174986,#174987),
(#174988,#174989),(#174990,#174991),(#174992,#174993),(#174994,#174995),
(#174996,#174997),(#174998,#174999),(#175000,#175001),(#175002,#175003),
(#175004,#175005),(#175006,#175007),(#175008,#175009),(#175010,#175011),
(#175012,#175013),(#175014,#175015),(#175016,#175017),(#175018,#175019),
(#175020,#175021),(#175022,#175023),(#175024,#175025),(#175026,#175027),
(#175028,#175029),(#175030,#175031),(#175032,#175033),(#175034,#175035),
(#175036,#175037),(#175038,#175039),(#175040,#175041),(#175042,#175043),
(#175044,#175045),(#175046,#175047),(#175048,#175049),(#175050,#175051),
(#175052,#175053),(#175054,#175055),(#175056,#175057),(#175058,#175059),
(#175060,#175061),(#175062,#175063),(#175064,#175065),(#175066,#175067),
(#175068,#175069),(#175070,#175071),(#175072,#175073),(#175074,#175075),
(#175076,#175077),(#175078,#175079),(#175080,#175081),(#175082,#175083),
(#175084,#175085),(#175086,#175087),(#175088,#175089),(#175090,#175091),
(#175092,#175093),(#175094,#175095),(#175096,#175097),(#175098,#175099),
(#175100,#175101),(#175102,#175103),(#175104,#175105),(#175106,#175107),
(#175108,#175109),(#175110,#175111),(#175112,#175113),(#175114,#175115),
(#175116,#175117),(#175118,#175119),(#175120,#175121),(#175122,#175123),
(#175124,#175125),(#175126,#175127),(#175128,#175129),(#175130,#175131),
(#175132,#175133),(#175134,#175135),(#175136,#175137),(#175138,#175139),
(#175140,#175141),(#175142,#175143),(#175144,#175145),(#175146,#175147),
(#175148,#175149),(#175150,#175151),(#175152,#175153),(#175154,#175155),
(#175156,#175157),(#175158,#175159),(#175160,#175161),(#175162,#175163),
(#175164,#175165),(#175166,#175167),(#175168,#175169),(#175170,#175171),
(#175172,#175173),(#175174,#175175),(#175176,#175177),(#175178,#175179),
(#175180,#175181),(#175182,#175183),(#175184,#175185),(#175186,#175187),
(#175188,#175189),(#175190,#175191),(#175192,#175193),(#175194,#175195),
(#175196,#175197),(#175198,#175199),(#175200,#175201),(#175202,#175203),
(#175204,#175205),(#175206,#175207),(#175208,#175209),(#175210,#175211),
(#175212,#175213),(#175214,#175215),(#175216,#175217),(#175218,#175219),
(#175220,#175221),(#175222,#175223),(#175224,#175225),(#175226,#175227),
(#175228,#175229),(#175230,#175231),(#175232,#175233),(#175234,#175235),
(#175236,#175237),(#175238,#175239),(#175240,#175241),(#175242,#175243),
(#175244,#175245),(#175246,#175247),(#175248,#175249),(#175250,#175251),
(#175252,#175253),(#175254,#175255),(#175256,#175257),(#175258,#175259),
(#175260,#175261),(#175262,#175263),(#175264,#175265),(#175266,#175267),
(#175268,#175269),(#175270,#175271),(#175272,#175273),(#175274,#175275),
(#175276,#175277),(#175278,#175279),(#175280,#175281),(#175282,#175283),
(#175284,#175285),(#175286,#175287),(#175288,#175289),(#175290,#175291),
(#175292,#175293),(#175294,#175295),(#175296,#175297),(#175298,#175299),
(#175300,#175301),(#175302,#175303),(#175304,#175305),(#175306,#175307),
(#175308,#175309),(#175310,#175311),(#175312,#175313),(#175314,#175315),
(#175316,#175317),(#175318,#175319),(#175320,#175321),(#175322,#175323),
(#175324,#175325),(#175326,#175327),(#175328,#175329),(#175330,#175331),
(#175332,#175333),(#175334,#175335),(#175336,#175337),(#175338,#175339),
(#175340,#175341),(#175342,#175343),(#175344,#175345),(#175346,#175347),
(#175348,#175349),(#175350,#175351),(#175352,#175353),(#175354,#175355),
(#175356,#175357),(#175358,#175359),(#175360,#175361),(#175362,#175363),
(#175364,#175365),(#175366,#175367),(#175368,#175369),(#175370,#175371),
(#175372,#175373),(#175374,#175375),(#175376,#175377),(#175378,#175379),
(#175380,#175381),(#175382,#175383),(#175384,#175385),(#175386,#175387),
(#175388,#175389),(#175390,#175391),(#175392,#175393),(#175394,#175395),
(#175396,#175397),(#175398,#175399),(#175400,#175401),(#175402,#175403),
(#175404,#175405),(#175406,#175407),(#175408,#175409),(#175410,#175411),
(#175412,#175413),(#175414,#175415),(#175416,#175417),(#175418,#175419),
(#175420,#175421),(#175422,#175423),(#175424,#175425),(#175426,#175427),
(#175428,#175429),(#175430,#175431),(#175432,#175433),(#175434,#175435),
(#175436,#175437),(#175438,#175439),(#175440,#175441),(#175442,#175443),
(#175444,#175445),(#175446,#175447),(#175448,#175449),(#175450,#175451),
(#175452,#175453),(#175454,#175455)),.UNSPECIFIED.,.F.,.F.,.F.,(6,1,1,1,
1,1,1,1,1,1,1,1,1,1,1,1,1,1,1,1,1,1,1,1,1,1,1,1,1,1,1,1,1,1,1,1,1,1,1,1,
1,1,1,1,1,1,1,1,1,1,1,1,1,1,1,1,1,1,1,1,1,1,1,1,1,1,1,1,1,1,1,1,1,1,1,1,
1,1,1,1,1,1,1,1,1,1,1,1,1,1,1,1,1,1,1,1,1,1,1,1,1,1,1,1,1,1,1,1,1,1,1,1,
1,1,1,1,1,1,1,1,1,1,1,1,1,1,1,1,1,1,1,1,1,1,1,1,1,1,1,1,1,1,1,1,1,1,1,1,
1,1,1,1,1,1,1,1,1,1,1,1,1,1,1,1,1,1,1,1,1,1,1,1,1,1,1,1,1,1,1,1,1,1,1,1,
1,1,1,1,1,1,1,1,1,1,1,1,1,1,1,1,1,1,1,1,1,1,1,1,1,1,1,1,1,1,1,1,1,1,1,1,
1,1,1,1,1,1,1,1,1,1,1,1,1,1,1,1,1,1,1,1,1,1,1,1,1,1,1,1,1,1,1,1,1,1,1,1,
1,1,1,1,1,1,1,1,1,1,1,1,1,1,1,1,1,1,1,1,1,1,1,1,1,1,1,1,1,1,1,1,1,1,1,1,
1,1,1,1,1,1,1,1,1,1,1,1,1,1,1,1,1,1,1,1,1,1,1,1,1,1,1,1,1,1,1,1,1,1,1,1,
1,1,1,1,1,1,1,1,1,1,1,1,1,1,1,1,1,1,1,1,1,1,1,1,1,1,1,1,1,1,1,1,1,1,1,1,
1,1,1,1,1,1,1,1,1,1,1,1,1,1,1,1,1,1,1,1,1,1,1,1,1,1,1,1,1,1,1,1,1,1,1,1,
1,1,1,1,1,1,1,1,1,1,1,1,1,1,1,1,1,1,1,1,1,1,1,1,1,1,1,1,1,1,1,1,1,1,1,1,
1,1,1,1,1,1,1,1,1,1,1,1,1,1,1,1,1,1,1,1,1,1,1,1,1,1,1,1,1,1,1,6),(2,2),
(0.143172103,0.144954128,0.146788991,0.148623853,0.150458716,0.152293578,
0.15412844,0.155963303,0.157798165,0.159633028,0.16146789,0.163302752,0.165137615,
0.166972477,0.168807339,0.170642202,0.172477064,0.174311927,0.176146789,
0.177981651,0.179816514,0.181651376,0.183486239,0.185321101,0.187155963,
0.188990826,0.190825688,0.19266055,0.194495413,0.196330275,0.198165138,
0.2,0.201834862,0.203669725,0.205504587,0.20733945,0.209174312,0.211009174,
0.212844037,0.214678899,0.216513761,0.218348624,0.220183486,0.222018349,
0.223853211,0.225688073,0.227522936,0.229357798,0.231192661,0.233027523,
0.234862385,0.236697248,0.23853211,0.240366972,0.242201835,0.244036697,
0.24587156,0.247706422,0.249541284,0.251376147,0.253211009,0.255045872,
0.256880734,0.258715596,0.260550459,0.262385321,0.264220183,0.266055046,
0.267889908,0.269724771,0.271559633,0.273394495,0.275229358,0.27706422,
0.278899083,0.280733945,0.282568807,0.28440367,0.286238532,0.288073394,
0.289908257,0.291743119,0.293577982,0.295412844,0.297247706,0.299082569,
0.300917431,0.302752294,0.304587156,0.306422018,0.308256881,0.310091743,
0.311926606,0.313761468,0.31559633,0.317431193,0.319266055,0.321100917,
0.32293578,0.324770642,0.326605505,0.328440367,0.330275229,0.332110092,
0.333944954,0.335779817,0.337614679,0.339449541,0.341284404,0.343119266,
0.344954128,0.346788991,0.348623853,0.350458716,0.352293578,0.35412844,
0.355963303,0.357798165,0.359633028,0.36146789,0.363302752,0.365137615,
0.366972477,0.368807339,0.370642202,0.372477064,0.374311927,0.376146789,
0.377981651,0.379816514,0.381651376,0.383486239,0.385321101,0.387155963,
0.388990826,0.390825688,0.39266055,0.394495413,0.396330275,0.398165138,
0.4,0.401834862,0.403669725,0.405504587,0.40733945,0.409174312,0.411009174,
0.412844037,0.414678899,0.416513761,0.418348624,0.420183486,0.422018349,
0.423853211,0.425688073,0.427522936,0.429357798,0.431192661,0.433027523,
0.434862385,0.436697248,0.43853211,0.440366972,0.442201835,0.444036697,
0.44587156,0.447706422,0.449541284,0.451376147,0.453211009,0.455045872,
0.456880734,0.458715596,0.460550459,0.462385321,0.464220183,0.466055046,
0.467889908,0.469724771,0.471559633,0.473394495,0.475229358,0.47706422,
0.478899083,0.480733945,0.482568807,0.48440367,0.486238532,0.488073394,
0.489908257,0.491743119,0.493577982,0.495412844,0.497247706,0.499082569,
0.500917431,0.502752294,0.504587156,0.506422018,0.508256881,0.510091743,
0.511926606,0.513761468,0.51559633,0.517431193,0.519266055,0.521100917,
0.52293578,0.524770642,0.526605505,0.528440367,0.530275229,0.532110092,
0.533944954,0.535779817,0.537614679,0.539449541,0.541284404,0.543119266,
0.544954128,0.546788991,0.548623853,0.550458716,0.552293578,0.55412844,
0.555963303,0.557798165,0.559633028,0.56146789,0.563302752,0.565137615,
0.566972477,0.568807339,0.570642202,0.572477064,0.574311927,0.576146789,
0.577981651,0.579816514,0.581651376,0.583486239,0.585321101,0.587155963,
0.588990826,0.590825688,0.59266055,0.594495413,0.596330275,0.598165138,
0.6,0.601834862,0.603669725,0.605504587,0.60733945,0.609174312,0.611009174,
0.612844037,0.614678899,0.616513761,0.618348624,0.620183486,0.622018349,
0.623853211,0.625688073,0.627522936,0.629357798,0.631192661,0.633027523,
0.634862385,0.636697248,0.63853211,0.640366972,0.642201835,0.644036697,
0.64587156,0.647706422,0.649541284,0.651376147,0.653211009,0.655045872,
0.656880734,0.658715596,0.660550459,0.662385321,0.664220183,0.666055046,
0.667889908,0.669724771,0.671559633,0.673394495,0.675229358,0.67706422,
0.678899083,0.680733945,0.682568807,0.68440367,0.686238532,0.688073394,
0.689908257,0.691743119,0.693577982,0.695412844,0.697247706,0.699082569,
0.700917431,0.702752294,0.704587156,0.706422018,0.708256881,0.710091743,
0.711926606,0.713761468,0.71559633,0.717431193,0.719266055,0.721100917,
0.72293578,0.724770642,0.726605505,0.728440367,0.730275229,0.732110092,
0.733944954,0.735779817,0.737614679,0.739449541,0.741284404,0.743119266,
0.744954128,0.746788991,0.748623853,0.750458716,0.752293578,0.75412844,
0.755963303,0.757798165,0.759633028,0.76146789,0.763302752,0.765137615,
0.766972477,0.768807339,0.770642202,0.772477064,0.774311927,0.776146789,
0.777981651,0.779816514,0.781651376,0.783486239,0.785321101,0.787155963,
0.788990826,0.790825688,0.79266055,0.794495413,0.796330275,0.798165138,
0.8,0.801834862,0.803669725,0.805504587,0.80733945,0.809174312,0.811009174,
0.812844037,0.814678899,0.816513761,0.818348624,0.820183486,0.822018349,
0.823853211,0.825688073,0.827522936,0.829357798,0.831192661,0.833027523,
0.834862385,0.836697248,0.83853211,0.840366972,0.842201835,0.844036697,
0.84587156,0.847706422,0.849541284,0.851376147,0.853211009,0.855045872,
0.856880734,0.858715596,0.860550459,0.862385321,0.864220183,0.866055046,
0.867889908,0.869724771,0.871559633,0.873394495,0.875229358,0.87706422,
0.878899083,0.880733945,0.882568807,0.88440367,0.886238532,0.888073394,
0.889908257,0.891743119,0.893577982,0.895412844,0.897247706,0.899082569,
0.900917431,0.902752294,0.904587156,0.906422018,0.908256881,0.910091743,
0.911926606,0.913761468,0.91559633,0.917431193,0.919266055,0.921100917,
0.92293578,0.924770642,0.926605505,0.928440367,0.930275229,0.932110092,
0.933944954,0.935779817,0.937614679,0.939449541,0.941284404,0.943119266,
0.944954128,0.946788991,0.948623853,0.950458716,0.952293578,0.95412844,
0.955963303,0.957798165,0.959633028,0.96146789,0.963302752,0.965137615,
0.966972477,0.968807339,0.970642202,0.972477064,0.974311927,0.976146789,
0.977981651,0.979816514,0.981651376,0.983486239,0.985321101,0.987155963,
0.988990826,0.990825688,0.99266055,0.994495413,0.996330275,0.998165138,
1.),(0.,0.36),.UNSPECIFIED.);
#6228=B_SPLINE_SURFACE_WITH_KNOTS('',5,1,((#176109,#176110),(#176111,#176112),
(#176113,#176114),(#176115,#176116),(#176117,#176118),(#176119,#176120),
(#176121,#176122),(#176123,#176124),(#176125,#176126),(#176127,#176128),
(#176129,#176130),(#176131,#176132),(#176133,#176134),(#176135,#176136),
(#176137,#176138),(#176139,#176140),(#176141,#176142),(#176143,#176144),
(#176145,#176146),(#176147,#176148),(#176149,#176150),(#176151,#176152),
(#176153,#176154),(#176155,#176156),(#176157,#176158),(#176159,#176160),
(#176161,#176162),(#176163,#176164),(#176165,#176166),(#176167,#176168),
(#176169,#176170),(#176171,#176172),(#176173,#176174),(#176175,#176176),
(#176177,#176178),(#176179,#176180),(#176181,#176182),(#176183,#176184),
(#176185,#176186),(#176187,#176188),(#176189,#176190),(#176191,#176192),
(#176193,#176194),(#176195,#176196),(#176197,#176198),(#176199,#176200),
(#176201,#176202),(#176203,#176204),(#176205,#176206),(#176207,#176208),
(#176209,#176210),(#176211,#176212),(#176213,#176214),(#176215,#176216),
(#176217,#176218),(#176219,#176220),(#176221,#176222),(#176223,#176224),
(#176225,#176226),(#176227,#176228),(#176229,#176230),(#176231,#176232),
(#176233,#176234),(#176235,#176236),(#176237,#176238),(#176239,#176240),
(#176241,#176242),(#176243,#176244),(#176245,#176246),(#176247,#176248),
(#176249,#176250),(#176251,#176252),(#176253,#176254),(#176255,#176256),
(#176257,#176258),(#176259,#176260),(#176261,#176262),(#176263,#176264),
(#176265,#176266),(#176267,#176268),(#176269,#176270),(#176271,#176272),
(#176273,#176274),(#176275,#176276),(#176277,#176278),(#176279,#176280),
(#176281,#176282),(#176283,#176284),(#176285,#176286),(#176287,#176288),
(#176289,#176290),(#176291,#176292),(#176293,#176294),(#176295,#176296),
(#176297,#176298),(#176299,#176300),(#176301,#176302),(#176303,#176304),
(#176305,#176306),(#176307,#176308),(#176309,#176310),(#176311,#176312),
(#176313,#176314),(#176315,#176316),(#176317,#176318),(#176319,#176320),
(#176321,#176322),(#176323,#176324),(#176325,#176326),(#176327,#176328),
(#176329,#176330),(#176331,#176332),(#176333,#176334),(#176335,#176336),
(#176337,#176338),(#176339,#176340),(#176341,#176342),(#176343,#176344),
(#176345,#176346),(#176347,#176348),(#176349,#176350),(#176351,#176352),
(#176353,#176354),(#176355,#176356),(#176357,#176358),(#176359,#176360),
(#176361,#176362),(#176363,#176364),(#176365,#176366),(#176367,#176368),
(#176369,#176370),(#176371,#176372),(#176373,#176374),(#176375,#176376),
(#176377,#176378),(#176379,#176380),(#176381,#176382),(#176383,#176384),
(#176385,#176386),(#176387,#176388),(#176389,#176390),(#176391,#176392),
(#176393,#176394),(#176395,#176396),(#176397,#176398),(#176399,#176400),
(#176401,#176402),(#176403,#176404),(#176405,#176406),(#176407,#176408),
(#176409,#176410),(#176411,#176412),(#176413,#176414),(#176415,#176416),
(#176417,#176418),(#176419,#176420),(#176421,#176422),(#176423,#176424),
(#176425,#176426),(#176427,#176428),(#176429,#176430),(#176431,#176432),
(#176433,#176434),(#176435,#176436),(#176437,#176438),(#176439,#176440),
(#176441,#176442),(#176443,#176444),(#176445,#176446),(#176447,#176448),
(#176449,#176450),(#176451,#176452),(#176453,#176454),(#176455,#176456),
(#176457,#176458),(#176459,#176460),(#176461,#176462),(#176463,#176464),
(#176465,#176466),(#176467,#176468),(#176469,#176470),(#176471,#176472),
(#176473,#176474),(#176475,#176476),(#176477,#176478),(#176479,#176480),
(#176481,#176482),(#176483,#176484),(#176485,#176486),(#176487,#176488),
(#176489,#176490),(#176491,#176492),(#176493,#176494),(#176495,#176496),
(#176497,#176498),(#176499,#176500),(#176501,#176502),(#176503,#176504),
(#176505,#176506),(#176507,#176508),(#176509,#176510),(#176511,#176512),
(#176513,#176514),(#176515,#176516),(#176517,#176518),(#176519,#176520),
(#176521,#176522),(#176523,#176524),(#176525,#176526),(#176527,#176528),
(#176529,#176530),(#176531,#176532),(#176533,#176534),(#176535,#176536),
(#176537,#176538),(#176539,#176540),(#176541,#176542),(#176543,#176544),
(#176545,#176546),(#176547,#176548),(#176549,#176550),(#176551,#176552),
(#176553,#176554),(#176555,#176556),(#176557,#176558),(#176559,#176560),
(#176561,#176562),(#176563,#176564),(#176565,#176566),(#176567,#176568),
(#176569,#176570),(#176571,#176572),(#176573,#176574),(#176575,#176576),
(#176577,#176578),(#176579,#176580),(#176581,#176582),(#176583,#176584),
(#176585,#176586),(#176587,#176588),(#176589,#176590),(#176591,#176592),
(#176593,#176594),(#176595,#176596),(#176597,#176598),(#176599,#176600),
(#176601,#176602),(#176603,#176604),(#176605,#176606),(#176607,#176608),
(#176609,#176610),(#176611,#176612),(#176613,#176614),(#176615,#176616),
(#176617,#176618),(#176619,#176620),(#176621,#176622),(#176623,#176624),
(#176625,#176626),(#176627,#176628),(#176629,#176630),(#176631,#176632),
(#176633,#176634),(#176635,#176636),(#176637,#176638),(#176639,#176640),
(#176641,#176642),(#176643,#176644),(#176645,#176646),(#176647,#176648),
(#176649,#176650),(#176651,#176652),(#176653,#176654),(#176655,#176656),
(#176657,#176658),(#176659,#176660),(#176661,#176662),(#176663,#176664),
(#176665,#176666),(#176667,#176668),(#176669,#176670),(#176671,#176672),
(#176673,#176674),(#176675,#176676),(#176677,#176678),(#176679,#176680),
(#176681,#176682),(#176683,#176684),(#176685,#176686),(#176687,#176688),
(#176689,#176690),(#176691,#176692),(#176693,#176694),(#176695,#176696),
(#176697,#176698),(#176699,#176700),(#176701,#176702),(#176703,#176704),
(#176705,#176706),(#176707,#176708),(#176709,#176710),(#176711,#176712),
(#176713,#176714),(#176715,#176716),(#176717,#176718),(#176719,#176720),
(#176721,#176722),(#176723,#176724),(#176725,#176726),(#176727,#176728),
(#176729,#176730),(#176731,#176732),(#176733,#176734),(#176735,#176736),
(#176737,#176738),(#176739,#176740),(#176741,#176742),(#176743,#176744),
(#176745,#176746),(#176747,#176748),(#176749,#176750),(#176751,#176752),
(#176753,#176754),(#176755,#176756),(#176757,#176758),(#176759,#176760),
(#176761,#176762),(#176763,#176764),(#176765,#176766),(#176767,#176768),
(#176769,#176770),(#176771,#176772),(#176773,#176774),(#176775,#176776),
(#176777,#176778),(#176779,#176780),(#176781,#176782),(#176783,#176784),
(#176785,#176786),(#176787,#176788),(#176789,#176790),(#176791,#176792),
(#176793,#176794),(#176795,#176796),(#176797,#176798),(#176799,#176800),
(#176801,#176802),(#176803,#176804),(#176805,#176806),(#176807,#176808),
(#176809,#176810),(#176811,#176812),(#176813,#176814),(#176815,#176816),
(#176817,#176818),(#176819,#176820),(#176821,#176822),(#176823,#176824),
(#176825,#176826),(#176827,#176828),(#176829,#176830),(#176831,#176832),
(#176833,#176834),(#176835,#176836),(#176837,#176838),(#176839,#176840),
(#176841,#176842),(#176843,#176844),(#176845,#176846),(#176847,#176848),
(#176849,#176850),(#176851,#176852),(#176853,#176854),(#176855,#176856),
(#176857,#176858),(#176859,#176860),(#176861,#176862),(#176863,#176864),
(#176865,#176866),(#176867,#176868),(#176869,#176870),(#176871,#176872),
(#176873,#176874),(#176875,#176876),(#176877,#176878),(#176879,#176880),
(#176881,#176882),(#176883,#176884),(#176885,#176886),(#176887,#176888),
(#176889,#176890),(#176891,#176892),(#176893,#176894),(#176895,#176896),
(#176897,#176898),(#176899,#176900),(#176901,#176902),(#176903,#176904),
(#176905,#176906),(#176907,#176908),(#176909,#176910),(#176911,#176912),
(#176913,#176914),(#176915,#176916),(#176917,#176918),(#176919,#176920),
(#176921,#176922),(#176923,#176924),(#176925,#176926),(#176927,#176928),
(#176929,#176930),(#176931,#176932),(#176933,#176934),(#176935,#176936),
(#176937,#176938),(#176939,#176940),(#176941,#176942),(#176943,#176944),
(#176945,#176946),(#176947,#176948),(#176949,#176950),(#176951,#176952),
(#176953,#176954),(#176955,#176956),(#176957,#176958),(#176959,#176960),
(#176961,#176962),(#176963,#176964),(#176965,#176966),(#176967,#176968),
(#176969,#176970),(#176971,#176972),(#176973,#176974),(#176975,#176976),
(#176977,#176978),(#176979,#176980),(#176981,#176982),(#176983,#176984),
(#176985,#176986),(#176987,#176988),(#176989,#176990),(#176991,#176992),
(#176993,#176994),(#176995,#176996),(#176997,#176998),(#176999,#177000),
(#177001,#177002),(#177003,#177004),(#177005,#177006),(#177007,#177008),
(#177009,#177010),(#177011,#177012),(#177013,#177014),(#177015,#177016),
(#177017,#177018),(#177019,#177020),(#177021,#177022),(#177023,#177024),
(#177025,#177026),(#177027,#177028),(#177029,#177030),(#177031,#177032),
(#177033,#177034),(#177035,#177036),(#177037,#177038),(#177039,#177040),
(#177041,#177042),(#177043,#177044),(#177045,#177046),(#177047,#177048),
(#177049,#177050),(#177051,#177052)),.UNSPECIFIED.,.F.,.F.,.F.,(6,1,1,1,
1,1,1,1,1,1,1,1,1,1,1,1,1,1,1,1,1,1,1,1,1,1,1,1,1,1,1,1,1,1,1,1,1,1,1,1,
1,1,1,1,1,1,1,1,1,1,1,1,1,1,1,1,1,1,1,1,1,1,1,1,1,1,1,1,1,1,1,1,1,1,1,1,
1,1,1,1,1,1,1,1,1,1,1,1,1,1,1,1,1,1,1,1,1,1,1,1,1,1,1,1,1,1,1,1,1,1,1,1,
1,1,1,1,1,1,1,1,1,1,1,1,1,1,1,1,1,1,1,1,1,1,1,1,1,1,1,1,1,1,1,1,1,1,1,1,
1,1,1,1,1,1,1,1,1,1,1,1,1,1,1,1,1,1,1,1,1,1,1,1,1,1,1,1,1,1,1,1,1,1,1,1,
1,1,1,1,1,1,1,1,1,1,1,1,1,1,1,1,1,1,1,1,1,1,1,1,1,1,1,1,1,1,1,1,1,1,1,1,
1,1,1,1,1,1,1,1,1,1,1,1,1,1,1,1,1,1,1,1,1,1,1,1,1,1,1,1,1,1,1,1,1,1,1,1,
1,1,1,1,1,1,1,1,1,1,1,1,1,1,1,1,1,1,1,1,1,1,1,1,1,1,1,1,1,1,1,1,1,1,1,1,
1,1,1,1,1,1,1,1,1,1,1,1,1,1,1,1,1,1,1,1,1,1,1,1,1,1,1,1,1,1,1,1,1,1,1,1,
1,1,1,1,1,1,1,1,1,1,1,1,1,1,1,1,1,1,1,1,1,1,1,1,1,1,1,1,1,1,1,1,1,1,1,1,
1,1,1,1,1,1,1,1,1,1,1,1,1,1,1,1,1,1,1,1,1,1,1,1,1,1,1,1,1,1,1,1,1,1,1,1,
1,1,1,1,1,1,1,1,1,1,1,1,1,1,1,1,1,1,1,1,1,1,1,1,1,1,1,1,1,1,1,1,1,1,1,1,
1,1,1,1,1,1,1,1,1,1,1,1,1,1,1,1,1,1,1,1,1,1,1,1,1,1,1,1,1,1,1,6),(2,2),
(-1.,-0.998165138,-0.996330275,-0.994495413,-0.99266055,-0.990825688,-0.988990826,
-0.987155963,-0.985321101,-0.983486239,-0.981651376,-0.979816514,-0.977981651,
-0.976146789,-0.974311927,-0.972477064,-0.970642202,-0.968807339,-0.966972477,
-0.965137615,-0.963302752,-0.96146789,-0.959633028,-0.957798165,-0.955963303,
-0.95412844,-0.952293578,-0.950458716,-0.948623853,-0.946788991,-0.944954128,
-0.943119266,-0.941284404,-0.939449541,-0.937614679,-0.935779817,-0.933944954,
-0.932110092,-0.930275229,-0.928440367,-0.926605505,-0.924770642,-0.92293578,
-0.921100917,-0.919266055,-0.917431193,-0.91559633,-0.913761468,-0.911926606,
-0.910091743,-0.908256881,-0.906422018,-0.904587156,-0.902752294,-0.900917431,
-0.899082569,-0.897247706,-0.895412844,-0.893577982,-0.891743119,-0.889908257,
-0.888073394,-0.886238532,-0.88440367,-0.882568807,-0.880733945,-0.878899083,
-0.87706422,-0.875229358,-0.873394495,-0.871559633,-0.869724771,-0.867889908,
-0.866055046,-0.864220183,-0.862385321,-0.860550459,-0.858715596,-0.856880734,
-0.855045872,-0.853211009,-0.851376147,-0.849541284,-0.847706422,-0.84587156,
-0.844036697,-0.842201835,-0.840366972,-0.83853211,-0.836697248,-0.834862385,
-0.833027523,-0.831192661,-0.829357798,-0.827522936,-0.825688073,-0.823853211,
-0.822018349,-0.820183486,-0.818348624,-0.816513761,-0.814678899,-0.812844037,
-0.811009174,-0.809174312,-0.80733945,-0.805504587,-0.803669725,-0.801834862,
-0.8,-0.798165138,-0.796330275,-0.794495413,-0.79266055,-0.790825688,-0.788990826,
-0.787155963,-0.785321101,-0.783486239,-0.781651376,-0.779816514,-0.777981651,
-0.776146789,-0.774311927,-0.772477064,-0.770642202,-0.768807339,-0.766972477,
-0.765137615,-0.763302752,-0.76146789,-0.759633028,-0.757798165,-0.755963303,
-0.75412844,-0.752293578,-0.750458716,-0.748623853,-0.746788991,-0.744954128,
-0.743119266,-0.741284404,-0.739449541,-0.737614679,-0.735779817,-0.733944954,
-0.732110092,-0.730275229,-0.728440367,-0.726605505,-0.724770642,-0.72293578,
-0.721100917,-0.719266055,-0.717431193,-0.71559633,-0.713761468,-0.711926606,
-0.710091743,-0.708256881,-0.706422018,-0.704587156,-0.702752294,-0.700917431,
-0.699082569,-0.697247706,-0.695412844,-0.693577982,-0.691743119,-0.689908257,
-0.688073394,-0.686238532,-0.68440367,-0.682568807,-0.680733945,-0.678899083,
-0.67706422,-0.675229358,-0.673394495,-0.671559633,-0.669724771,-0.667889908,
-0.666055046,-0.664220183,-0.662385321,-0.660550459,-0.658715596,-0.656880734,
-0.655045872,-0.653211009,-0.651376147,-0.649541284,-0.647706422,-0.64587156,
-0.644036697,-0.642201835,-0.640366972,-0.63853211,-0.636697248,-0.634862385,
-0.633027523,-0.631192661,-0.629357798,-0.627522936,-0.625688073,-0.623853211,
-0.622018349,-0.620183486,-0.618348624,-0.616513761,-0.614678899,-0.612844037,
-0.611009174,-0.609174312,-0.60733945,-0.605504587,-0.603669725,-0.601834862,
-0.6,-0.598165138,-0.596330275,-0.594495413,-0.59266055,-0.590825688,-0.588990826,
-0.587155963,-0.585321101,-0.583486239,-0.581651376,-0.579816514,-0.577981651,
-0.576146789,-0.574311927,-0.572477064,-0.570642202,-0.568807339,-0.566972477,
-0.565137615,-0.563302752,-0.56146789,-0.559633028,-0.557798165,-0.555963303,
-0.55412844,-0.552293578,-0.550458716,-0.548623853,-0.546788991,-0.544954128,
-0.543119266,-0.541284404,-0.539449541,-0.537614679,-0.535779817,-0.533944954,
-0.532110092,-0.530275229,-0.528440367,-0.526605505,-0.524770642,-0.52293578,
-0.521100917,-0.519266055,-0.517431193,-0.51559633,-0.513761468,-0.511926606,
-0.510091743,-0.508256881,-0.506422018,-0.504587156,-0.502752294,-0.500917431,
-0.499082569,-0.497247706,-0.495412844,-0.493577982,-0.491743119,-0.489908257,
-0.488073394,-0.486238532,-0.48440367,-0.482568807,-0.480733945,-0.478899083,
-0.47706422,-0.475229358,-0.473394495,-0.471559633,-0.469724771,-0.467889908,
-0.466055046,-0.464220183,-0.462385321,-0.460550459,-0.458715596,-0.456880734,
-0.455045872,-0.453211009,-0.451376147,-0.449541284,-0.447706422,-0.44587156,
-0.444036697,-0.442201835,-0.440366972,-0.43853211,-0.436697248,-0.434862385,
-0.433027523,-0.431192661,-0.429357798,-0.427522936,-0.425688073,-0.423853211,
-0.422018349,-0.420183486,-0.418348624,-0.416513761,-0.414678899,-0.412844037,
-0.411009174,-0.409174312,-0.40733945,-0.405504587,-0.403669725,-0.401834862,
-0.4,-0.398165138,-0.396330275,-0.394495413,-0.39266055,-0.390825688,-0.388990826,
-0.387155963,-0.385321101,-0.383486239,-0.381651376,-0.379816514,-0.377981651,
-0.376146789,-0.374311927,-0.372477064,-0.370642202,-0.368807339,-0.366972477,
-0.365137615,-0.363302752,-0.36146789,-0.359633028,-0.357798165,-0.355963303,
-0.35412844,-0.352293578,-0.350458716,-0.348623853,-0.346788991,-0.344954128,
-0.343119266,-0.341284404,-0.339449541,-0.337614679,-0.335779817,-0.333944954,
-0.332110092,-0.330275229,-0.328440367,-0.326605505,-0.324770642,-0.32293578,
-0.321100917,-0.319266055,-0.317431193,-0.31559633,-0.313761468,-0.311926606,
-0.310091743,-0.308256881,-0.306422018,-0.304587156,-0.302752294,-0.300917431,
-0.299082569,-0.297247706,-0.295412844,-0.293577982,-0.291743119,-0.289908257,
-0.288073394,-0.286238532,-0.28440367,-0.282568807,-0.280733945,-0.278899083,
-0.27706422,-0.275229358,-0.273394495,-0.271559633,-0.269724771,-0.267889908,
-0.266055046,-0.264220183,-0.262385321,-0.260550459,-0.258715596,-0.256880734,
-0.255045872,-0.253211009,-0.251376147,-0.249541284,-0.247706422,-0.24587156,
-0.244036697,-0.242201835,-0.240366972,-0.23853211,-0.236697248,-0.234862385,
-0.233027523,-0.231192661,-0.229357798,-0.227522936,-0.225688073,-0.223853211,
-0.222018349,-0.220183486,-0.218348624,-0.216513761,-0.214678899,-0.212844037,
-0.211009174,-0.209174312,-0.20733945,-0.205504587,-0.203669725,-0.201834862,
-0.2,-0.198165138,-0.196330275,-0.194495413,-0.19266055,-0.190825688,-0.188990826,
-0.187155963,-0.185321101,-0.183486239,-0.181651376,-0.179816514,-0.177981651,
-0.176146789,-0.174311927,-0.172477064,-0.170642202,-0.168807339,-0.166972477,
-0.165137615,-0.163302752,-0.16146789,-0.159633028,-0.157798165,-0.155963303,
-0.15412844,-0.152293578,-0.150458716,-0.148623853,-0.146788991,-0.144954128,
-0.143172103),(0.,0.36),.UNSPECIFIED.);
#6229=B_SPLINE_SURFACE_WITH_KNOTS('',5,1,((#177721,#177722),(#177723,#177724),
(#177725,#177726),(#177727,#177728),(#177729,#177730),(#177731,#177732),
(#177733,#177734),(#177735,#177736),(#177737,#177738),(#177739,#177740),
(#177741,#177742),(#177743,#177744),(#177745,#177746),(#177747,#177748),
(#177749,#177750),(#177751,#177752),(#177753,#177754),(#177755,#177756),
(#177757,#177758),(#177759,#177760),(#177761,#177762),(#177763,#177764),
(#177765,#177766),(#177767,#177768),(#177769,#177770),(#177771,#177772),
(#177773,#177774),(#177775,#177776),(#177777,#177778),(#177779,#177780),
(#177781,#177782),(#177783,#177784),(#177785,#177786),(#177787,#177788),
(#177789,#177790),(#177791,#177792),(#177793,#177794),(#177795,#177796),
(#177797,#177798),(#177799,#177800),(#177801,#177802),(#177803,#177804),
(#177805,#177806),(#177807,#177808),(#177809,#177810),(#177811,#177812),
(#177813,#177814),(#177815,#177816),(#177817,#177818),(#177819,#177820),
(#177821,#177822),(#177823,#177824),(#177825,#177826),(#177827,#177828),
(#177829,#177830),(#177831,#177832),(#177833,#177834),(#177835,#177836),
(#177837,#177838),(#177839,#177840),(#177841,#177842),(#177843,#177844),
(#177845,#177846),(#177847,#177848),(#177849,#177850),(#177851,#177852),
(#177853,#177854),(#177855,#177856),(#177857,#177858),(#177859,#177860),
(#177861,#177862),(#177863,#177864),(#177865,#177866),(#177867,#177868),
(#177869,#177870),(#177871,#177872),(#177873,#177874),(#177875,#177876),
(#177877,#177878),(#177879,#177880),(#177881,#177882),(#177883,#177884),
(#177885,#177886),(#177887,#177888),(#177889,#177890),(#177891,#177892),
(#177893,#177894),(#177895,#177896),(#177897,#177898),(#177899,#177900),
(#177901,#177902),(#177903,#177904),(#177905,#177906),(#177907,#177908),
(#177909,#177910),(#177911,#177912),(#177913,#177914),(#177915,#177916),
(#177917,#177918),(#177919,#177920),(#177921,#177922),(#177923,#177924),
(#177925,#177926),(#177927,#177928),(#177929,#177930),(#177931,#177932),
(#177933,#177934),(#177935,#177936),(#177937,#177938),(#177939,#177940),
(#177941,#177942),(#177943,#177944),(#177945,#177946),(#177947,#177948),
(#177949,#177950),(#177951,#177952),(#177953,#177954),(#177955,#177956),
(#177957,#177958),(#177959,#177960),(#177961,#177962),(#177963,#177964),
(#177965,#177966),(#177967,#177968),(#177969,#177970),(#177971,#177972),
(#177973,#177974),(#177975,#177976),(#177977,#177978),(#177979,#177980),
(#177981,#177982),(#177983,#177984),(#177985,#177986),(#177987,#177988),
(#177989,#177990),(#177991,#177992),(#177993,#177994),(#177995,#177996),
(#177997,#177998),(#177999,#178000),(#178001,#178002),(#178003,#178004),
(#178005,#178006),(#178007,#178008),(#178009,#178010),(#178011,#178012),
(#178013,#178014),(#178015,#178016),(#178017,#178018),(#178019,#178020),
(#178021,#178022),(#178023,#178024),(#178025,#178026),(#178027,#178028),
(#178029,#178030),(#178031,#178032),(#178033,#178034),(#178035,#178036),
(#178037,#178038),(#178039,#178040),(#178041,#178042),(#178043,#178044),
(#178045,#178046),(#178047,#178048),(#178049,#178050),(#178051,#178052),
(#178053,#178054),(#178055,#178056),(#178057,#178058),(#178059,#178060),
(#178061,#178062),(#178063,#178064),(#178065,#178066),(#178067,#178068),
(#178069,#178070),(#178071,#178072),(#178073,#178074),(#178075,#178076),
(#178077,#178078),(#178079,#178080),(#178081,#178082),(#178083,#178084),
(#178085,#178086),(#178087,#178088),(#178089,#178090),(#178091,#178092),
(#178093,#178094),(#178095,#178096),(#178097,#178098),(#178099,#178100),
(#178101,#178102),(#178103,#178104),(#178105,#178106),(#178107,#178108),
(#178109,#178110),(#178111,#178112),(#178113,#178114),(#178115,#178116),
(#178117,#178118),(#178119,#178120),(#178121,#178122),(#178123,#178124),
(#178125,#178126),(#178127,#178128),(#178129,#178130),(#178131,#178132),
(#178133,#178134),(#178135,#178136),(#178137,#178138),(#178139,#178140),
(#178141,#178142),(#178143,#178144),(#178145,#178146),(#178147,#178148),
(#178149,#178150),(#178151,#178152),(#178153,#178154),(#178155,#178156),
(#178157,#178158),(#178159,#178160),(#178161,#178162),(#178163,#178164),
(#178165,#178166),(#178167,#178168),(#178169,#178170),(#178171,#178172),
(#178173,#178174),(#178175,#178176),(#178177,#178178),(#178179,#178180),
(#178181,#178182),(#178183,#178184),(#178185,#178186),(#178187,#178188),
(#178189,#178190),(#178191,#178192),(#178193,#178194),(#178195,#178196),
(#178197,#178198),(#178199,#178200),(#178201,#178202),(#178203,#178204),
(#178205,#178206),(#178207,#178208),(#178209,#178210),(#178211,#178212),
(#178213,#178214),(#178215,#178216),(#178217,#178218),(#178219,#178220),
(#178221,#178222),(#178223,#178224),(#178225,#178226),(#178227,#178228),
(#178229,#178230),(#178231,#178232),(#178233,#178234),(#178235,#178236),
(#178237,#178238),(#178239,#178240),(#178241,#178242),(#178243,#178244),
(#178245,#178246),(#178247,#178248),(#178249,#178250),(#178251,#178252),
(#178253,#178254),(#178255,#178256),(#178257,#178258),(#178259,#178260),
(#178261,#178262),(#178263,#178264),(#178265,#178266),(#178267,#178268),
(#178269,#178270),(#178271,#178272),(#178273,#178274),(#178275,#178276),
(#178277,#178278),(#178279,#178280),(#178281,#178282),(#178283,#178284),
(#178285,#178286),(#178287,#178288),(#178289,#178290),(#178291,#178292),
(#178293,#178294),(#178295,#178296),(#178297,#178298),(#178299,#178300),
(#178301,#178302),(#178303,#178304),(#178305,#178306),(#178307,#178308),
(#178309,#178310),(#178311,#178312),(#178313,#178314),(#178315,#178316),
(#178317,#178318),(#178319,#178320),(#178321,#178322),(#178323,#178324),
(#178325,#178326),(#178327,#178328),(#178329,#178330),(#178331,#178332),
(#178333,#178334),(#178335,#178336),(#178337,#178338),(#178339,#178340),
(#178341,#178342),(#178343,#178344),(#178345,#178346),(#178347,#178348),
(#178349,#178350),(#178351,#178352),(#178353,#178354),(#178355,#178356),
(#178357,#178358),(#178359,#178360),(#178361,#178362),(#178363,#178364),
(#178365,#178366),(#178367,#178368),(#178369,#178370),(#178371,#178372),
(#178373,#178374),(#178375,#178376),(#178377,#178378),(#178379,#178380),
(#178381,#178382),(#178383,#178384),(#178385,#178386),(#178387,#178388),
(#178389,#178390),(#178391,#178392),(#178393,#178394),(#178395,#178396),
(#178397,#178398),(#178399,#178400),(#178401,#178402),(#178403,#178404),
(#178405,#178406),(#178407,#178408),(#178409,#178410),(#178411,#178412),
(#178413,#178414),(#178415,#178416),(#178417,#178418),(#178419,#178420),
(#178421,#178422),(#178423,#178424),(#178425,#178426),(#178427,#178428),
(#178429,#178430),(#178431,#178432),(#178433,#178434),(#178435,#178436),
(#178437,#178438),(#178439,#178440),(#178441,#178442),(#178443,#178444),
(#178445,#178446),(#178447,#178448),(#178449,#178450),(#178451,#178452),
(#178453,#178454),(#178455,#178456),(#178457,#178458),(#178459,#178460),
(#178461,#178462),(#178463,#178464),(#178465,#178466),(#178467,#178468),
(#178469,#178470),(#178471,#178472),(#178473,#178474),(#178475,#178476),
(#178477,#178478),(#178479,#178480),(#178481,#178482),(#178483,#178484),
(#178485,#178486),(#178487,#178488),(#178489,#178490),(#178491,#178492),
(#178493,#178494),(#178495,#178496),(#178497,#178498),(#178499,#178500),
(#178501,#178502),(#178503,#178504),(#178505,#178506),(#178507,#178508),
(#178509,#178510),(#178511,#178512),(#178513,#178514),(#178515,#178516),
(#178517,#178518),(#178519,#178520),(#178521,#178522),(#178523,#178524),
(#178525,#178526),(#178527,#178528),(#178529,#178530),(#178531,#178532),
(#178533,#178534),(#178535,#178536),(#178537,#178538),(#178539,#178540),
(#178541,#178542),(#178543,#178544),(#178545,#178546),(#178547,#178548),
(#178549,#178550),(#178551,#178552),(#178553,#178554),(#178555,#178556),
(#178557,#178558),(#178559,#178560),(#178561,#178562),(#178563,#178564),
(#178565,#178566),(#178567,#178568),(#178569,#178570),(#178571,#178572),
(#178573,#178574),(#178575,#178576),(#178577,#178578),(#178579,#178580),
(#178581,#178582),(#178583,#178584),(#178585,#178586),(#178587,#178588),
(#178589,#178590),(#178591,#178592),(#178593,#178594),(#178595,#178596),
(#178597,#178598),(#178599,#178600),(#178601,#178602),(#178603,#178604),
(#178605,#178606),(#178607,#178608),(#178609,#178610),(#178611,#178612),
(#178613,#178614),(#178615,#178616),(#178617,#178618),(#178619,#178620),
(#178621,#178622),(#178623,#178624),(#178625,#178626),(#178627,#178628),
(#178629,#178630),(#178631,#178632),(#178633,#178634),(#178635,#178636),
(#178637,#178638),(#178639,#178640),(#178641,#178642),(#178643,#178644),
(#178645,#178646),(#178647,#178648),(#178649,#178650),(#178651,#178652),
(#178653,#178654),(#178655,#178656),(#178657,#178658),(#178659,#178660),
(#178661,#178662),(#178663,#178664)),.UNSPECIFIED.,.F.,.F.,.F.,(6,1,1,1,
1,1,1,1,1,1,1,1,1,1,1,1,1,1,1,1,1,1,1,1,1,1,1,1,1,1,1,1,1,1,1,1,1,1,1,1,
1,1,1,1,1,1,1,1,1,1,1,1,1,1,1,1,1,1,1,1,1,1,1,1,1,1,1,1,1,1,1,1,1,1,1,1,
1,1,1,1,1,1,1,1,1,1,1,1,1,1,1,1,1,1,1,1,1,1,1,1,1,1,1,1,1,1,1,1,1,1,1,1,
1,1,1,1,1,1,1,1,1,1,1,1,1,1,1,1,1,1,1,1,1,1,1,1,1,1,1,1,1,1,1,1,1,1,1,1,
1,1,1,1,1,1,1,1,1,1,1,1,1,1,1,1,1,1,1,1,1,1,1,1,1,1,1,1,1,1,1,1,1,1,1,1,
1,1,1,1,1,1,1,1,1,1,1,1,1,1,1,1,1,1,1,1,1,1,1,1,1,1,1,1,1,1,1,1,1,1,1,1,
1,1,1,1,1,1,1,1,1,1,1,1,1,1,1,1,1,1,1,1,1,1,1,1,1,1,1,1,1,1,1,1,1,1,1,1,
1,1,1,1,1,1,1,1,1,1,1,1,1,1,1,1,1,1,1,1,1,1,1,1,1,1,1,1,1,1,1,1,1,1,1,1,
1,1,1,1,1,1,1,1,1,1,1,1,1,1,1,1,1,1,1,1,1,1,1,1,1,1,1,1,1,1,1,1,1,1,1,1,
1,1,1,1,1,1,1,1,1,1,1,1,1,1,1,1,1,1,1,1,1,1,1,1,1,1,1,1,1,1,1,1,1,1,1,1,
1,1,1,1,1,1,1,1,1,1,1,1,1,1,1,1,1,1,1,1,1,1,1,1,1,1,1,1,1,1,1,1,1,1,1,1,
1,1,1,1,1,1,1,1,1,1,1,1,1,1,1,1,1,1,1,1,1,1,1,1,1,1,1,1,1,1,1,1,1,1,1,1,
1,1,1,1,1,1,1,1,1,1,1,1,1,1,1,1,1,1,1,1,1,1,1,1,1,1,1,1,1,1,1,6),(2,2),
(-1.,-0.998165138,-0.996330275,-0.994495413,-0.99266055,-0.990825688,-0.988990826,
-0.987155963,-0.985321101,-0.983486239,-0.981651376,-0.979816514,-0.977981651,
-0.976146789,-0.974311927,-0.972477064,-0.970642202,-0.968807339,-0.966972477,
-0.965137615,-0.963302752,-0.96146789,-0.959633028,-0.957798165,-0.955963303,
-0.95412844,-0.952293578,-0.950458716,-0.948623853,-0.946788991,-0.944954128,
-0.943119266,-0.941284404,-0.939449541,-0.937614679,-0.935779817,-0.933944954,
-0.932110092,-0.930275229,-0.928440367,-0.926605505,-0.924770642,-0.92293578,
-0.921100917,-0.919266055,-0.917431193,-0.91559633,-0.913761468,-0.911926606,
-0.910091743,-0.908256881,-0.906422018,-0.904587156,-0.902752294,-0.900917431,
-0.899082569,-0.897247706,-0.895412844,-0.893577982,-0.891743119,-0.889908257,
-0.888073394,-0.886238532,-0.88440367,-0.882568807,-0.880733945,-0.878899083,
-0.87706422,-0.875229358,-0.873394495,-0.871559633,-0.869724771,-0.867889908,
-0.866055046,-0.864220183,-0.862385321,-0.860550459,-0.858715596,-0.856880734,
-0.855045872,-0.853211009,-0.851376147,-0.849541284,-0.847706422,-0.84587156,
-0.844036697,-0.842201835,-0.840366972,-0.83853211,-0.836697248,-0.834862385,
-0.833027523,-0.831192661,-0.829357798,-0.827522936,-0.825688073,-0.823853211,
-0.822018349,-0.820183486,-0.818348624,-0.816513761,-0.814678899,-0.812844037,
-0.811009174,-0.809174312,-0.80733945,-0.805504587,-0.803669725,-0.801834862,
-0.8,-0.798165138,-0.796330275,-0.794495413,-0.79266055,-0.790825688,-0.788990826,
-0.787155963,-0.785321101,-0.783486239,-0.781651376,-0.779816514,-0.777981651,
-0.776146789,-0.774311927,-0.772477064,-0.770642202,-0.768807339,-0.766972477,
-0.765137615,-0.763302752,-0.76146789,-0.759633028,-0.757798165,-0.755963303,
-0.75412844,-0.752293578,-0.750458716,-0.748623853,-0.746788991,-0.744954128,
-0.743119266,-0.741284404,-0.739449541,-0.737614679,-0.735779817,-0.733944954,
-0.732110092,-0.730275229,-0.728440367,-0.726605505,-0.724770642,-0.72293578,
-0.721100917,-0.719266055,-0.717431193,-0.71559633,-0.713761468,-0.711926606,
-0.710091743,-0.708256881,-0.706422018,-0.704587156,-0.702752294,-0.700917431,
-0.699082569,-0.697247706,-0.695412844,-0.693577982,-0.691743119,-0.689908257,
-0.688073394,-0.686238532,-0.68440367,-0.682568807,-0.680733945,-0.678899083,
-0.67706422,-0.675229358,-0.673394495,-0.671559633,-0.669724771,-0.667889908,
-0.666055046,-0.664220183,-0.662385321,-0.660550459,-0.658715596,-0.656880734,
-0.655045872,-0.653211009,-0.651376147,-0.649541284,-0.647706422,-0.64587156,
-0.644036697,-0.642201835,-0.640366972,-0.63853211,-0.636697248,-0.634862385,
-0.633027523,-0.631192661,-0.629357798,-0.627522936,-0.625688073,-0.623853211,
-0.622018349,-0.620183486,-0.618348624,-0.616513761,-0.614678899,-0.612844037,
-0.611009174,-0.609174312,-0.60733945,-0.605504587,-0.603669725,-0.601834862,
-0.6,-0.598165138,-0.596330275,-0.594495413,-0.59266055,-0.590825688,-0.588990826,
-0.587155963,-0.585321101,-0.583486239,-0.581651376,-0.579816514,-0.577981651,
-0.576146789,-0.574311927,-0.572477064,-0.570642202,-0.568807339,-0.566972477,
-0.565137615,-0.563302752,-0.56146789,-0.559633028,-0.557798165,-0.555963303,
-0.55412844,-0.552293578,-0.550458716,-0.548623853,-0.546788991,-0.544954128,
-0.543119266,-0.541284404,-0.539449541,-0.537614679,-0.535779817,-0.533944954,
-0.532110092,-0.530275229,-0.528440367,-0.526605505,-0.524770642,-0.52293578,
-0.521100917,-0.519266055,-0.517431193,-0.51559633,-0.513761468,-0.511926606,
-0.510091743,-0.508256881,-0.506422018,-0.504587156,-0.502752294,-0.500917431,
-0.499082569,-0.497247706,-0.495412844,-0.493577982,-0.491743119,-0.489908257,
-0.488073394,-0.486238532,-0.48440367,-0.482568807,-0.480733945,-0.478899083,
-0.47706422,-0.475229358,-0.473394495,-0.471559633,-0.469724771,-0.467889908,
-0.466055046,-0.464220183,-0.462385321,-0.460550459,-0.458715596,-0.456880734,
-0.455045872,-0.453211009,-0.451376147,-0.449541284,-0.447706422,-0.44587156,
-0.444036697,-0.442201835,-0.440366972,-0.43853211,-0.436697248,-0.434862385,
-0.433027523,-0.431192661,-0.429357798,-0.427522936,-0.425688073,-0.423853211,
-0.422018349,-0.420183486,-0.418348624,-0.416513761,-0.414678899,-0.412844037,
-0.411009174,-0.409174312,-0.40733945,-0.405504587,-0.403669725,-0.401834862,
-0.4,-0.398165138,-0.396330275,-0.394495413,-0.39266055,-0.390825688,-0.388990826,
-0.387155963,-0.385321101,-0.383486239,-0.381651376,-0.379816514,-0.377981651,
-0.376146789,-0.374311927,-0.372477064,-0.370642202,-0.368807339,-0.366972477,
-0.365137615,-0.363302752,-0.36146789,-0.359633028,-0.357798165,-0.355963303,
-0.35412844,-0.352293578,-0.350458716,-0.348623853,-0.346788991,-0.344954128,
-0.343119266,-0.341284404,-0.339449541,-0.337614679,-0.335779817,-0.333944954,
-0.332110092,-0.330275229,-0.328440367,-0.326605505,-0.324770642,-0.32293578,
-0.321100917,-0.319266055,-0.317431193,-0.31559633,-0.313761468,-0.311926606,
-0.310091743,-0.308256881,-0.306422018,-0.304587156,-0.302752294,-0.300917431,
-0.299082569,-0.297247706,-0.295412844,-0.293577982,-0.291743119,-0.289908257,
-0.288073394,-0.286238532,-0.28440367,-0.282568807,-0.280733945,-0.278899083,
-0.27706422,-0.275229358,-0.273394495,-0.271559633,-0.269724771,-0.267889908,
-0.266055046,-0.264220183,-0.262385321,-0.260550459,-0.258715596,-0.256880734,
-0.255045872,-0.253211009,-0.251376147,-0.249541284,-0.247706422,-0.24587156,
-0.244036697,-0.242201835,-0.240366972,-0.23853211,-0.236697248,-0.234862385,
-0.233027523,-0.231192661,-0.229357798,-0.227522936,-0.225688073,-0.223853211,
-0.222018349,-0.220183486,-0.218348624,-0.216513761,-0.214678899,-0.212844037,
-0.211009174,-0.209174312,-0.20733945,-0.205504587,-0.203669725,-0.201834862,
-0.2,-0.198165138,-0.196330275,-0.194495413,-0.19266055,-0.190825688,-0.188990826,
-0.187155963,-0.185321101,-0.183486239,-0.181651376,-0.179816514,-0.177981651,
-0.176146789,-0.174311927,-0.172477064,-0.170642202,-0.168807339,-0.166972477,
-0.165137615,-0.163302752,-0.16146789,-0.159633028,-0.157798165,-0.155963303,
-0.15412844,-0.152293578,-0.150458716,-0.148623853,-0.146788991,-0.144954128,
-0.143172104),(0.,0.36),.UNSPECIFIED.);
#6230=B_SPLINE_SURFACE_WITH_KNOTS('',5,1,((#179612,#179613),(#179614,#179615),
(#179616,#179617),(#179618,#179619),(#179620,#179621),(#179622,#179623),
(#179624,#179625),(#179626,#179627),(#179628,#179629),(#179630,#179631),
(#179632,#179633),(#179634,#179635),(#179636,#179637),(#179638,#179639),
(#179640,#179641),(#179642,#179643),(#179644,#179645),(#179646,#179647),
(#179648,#179649),(#179650,#179651),(#179652,#179653),(#179654,#179655),
(#179656,#179657),(#179658,#179659),(#179660,#179661),(#179662,#179663),
(#179664,#179665),(#179666,#179667),(#179668,#179669),(#179670,#179671),
(#179672,#179673),(#179674,#179675),(#179676,#179677),(#179678,#179679),
(#179680,#179681),(#179682,#179683),(#179684,#179685),(#179686,#179687),
(#179688,#179689),(#179690,#179691),(#179692,#179693),(#179694,#179695),
(#179696,#179697),(#179698,#179699),(#179700,#179701),(#179702,#179703),
(#179704,#179705),(#179706,#179707),(#179708,#179709),(#179710,#179711),
(#179712,#179713),(#179714,#179715),(#179716,#179717),(#179718,#179719),
(#179720,#179721),(#179722,#179723),(#179724,#179725),(#179726,#179727),
(#179728,#179729),(#179730,#179731),(#179732,#179733),(#179734,#179735),
(#179736,#179737),(#179738,#179739),(#179740,#179741),(#179742,#179743),
(#179744,#179745),(#179746,#179747),(#179748,#179749),(#179750,#179751),
(#179752,#179753),(#179754,#179755),(#179756,#179757),(#179758,#179759),
(#179760,#179761),(#179762,#179763),(#179764,#179765),(#179766,#179767),
(#179768,#179769),(#179770,#179771),(#179772,#179773),(#179774,#179775),
(#179776,#179777),(#179778,#179779),(#179780,#179781),(#179782,#179783),
(#179784,#179785),(#179786,#179787),(#179788,#179789),(#179790,#179791),
(#179792,#179793),(#179794,#179795),(#179796,#179797),(#179798,#179799),
(#179800,#179801),(#179802,#179803),(#179804,#179805),(#179806,#179807),
(#179808,#179809),(#179810,#179811),(#179812,#179813),(#179814,#179815),
(#179816,#179817),(#179818,#179819),(#179820,#179821),(#179822,#179823),
(#179824,#179825),(#179826,#179827),(#179828,#179829),(#179830,#179831),
(#179832,#179833),(#179834,#179835),(#179836,#179837),(#179838,#179839),
(#179840,#179841),(#179842,#179843),(#179844,#179845),(#179846,#179847),
(#179848,#179849),(#179850,#179851),(#179852,#179853),(#179854,#179855),
(#179856,#179857),(#179858,#179859),(#179860,#179861),(#179862,#179863),
(#179864,#179865),(#179866,#179867),(#179868,#179869),(#179870,#179871),
(#179872,#179873),(#179874,#179875),(#179876,#179877),(#179878,#179879),
(#179880,#179881),(#179882,#179883),(#179884,#179885),(#179886,#179887),
(#179888,#179889),(#179890,#179891),(#179892,#179893),(#179894,#179895),
(#179896,#179897),(#179898,#179899),(#179900,#179901),(#179902,#179903),
(#179904,#179905),(#179906,#179907),(#179908,#179909),(#179910,#179911),
(#179912,#179913),(#179914,#179915),(#179916,#179917),(#179918,#179919),
(#179920,#179921),(#179922,#179923),(#179924,#179925),(#179926,#179927),
(#179928,#179929),(#179930,#179931),(#179932,#179933),(#179934,#179935),
(#179936,#179937),(#179938,#179939),(#179940,#179941),(#179942,#179943),
(#179944,#179945),(#179946,#179947),(#179948,#179949),(#179950,#179951),
(#179952,#179953),(#179954,#179955),(#179956,#179957),(#179958,#179959),
(#179960,#179961),(#179962,#179963),(#179964,#179965),(#179966,#179967),
(#179968,#179969),(#179970,#179971),(#179972,#179973),(#179974,#179975),
(#179976,#179977),(#179978,#179979),(#179980,#179981),(#179982,#179983),
(#179984,#179985),(#179986,#179987),(#179988,#179989),(#179990,#179991),
(#179992,#179993),(#179994,#179995),(#179996,#179997),(#179998,#179999),
(#180000,#180001),(#180002,#180003),(#180004,#180005),(#180006,#180007),
(#180008,#180009),(#180010,#180011),(#180012,#180013),(#180014,#180015),
(#180016,#180017),(#180018,#180019),(#180020,#180021),(#180022,#180023),
(#180024,#180025),(#180026,#180027),(#180028,#180029),(#180030,#180031),
(#180032,#180033),(#180034,#180035),(#180036,#180037),(#180038,#180039),
(#180040,#180041),(#180042,#180043),(#180044,#180045),(#180046,#180047),
(#180048,#180049),(#180050,#180051),(#180052,#180053),(#180054,#180055),
(#180056,#180057),(#180058,#180059),(#180060,#180061),(#180062,#180063),
(#180064,#180065),(#180066,#180067),(#180068,#180069),(#180070,#180071),
(#180072,#180073),(#180074,#180075),(#180076,#180077),(#180078,#180079),
(#180080,#180081),(#180082,#180083),(#180084,#180085),(#180086,#180087),
(#180088,#180089),(#180090,#180091),(#180092,#180093),(#180094,#180095),
(#180096,#180097),(#180098,#180099),(#180100,#180101),(#180102,#180103),
(#180104,#180105),(#180106,#180107),(#180108,#180109),(#180110,#180111),
(#180112,#180113),(#180114,#180115),(#180116,#180117),(#180118,#180119),
(#180120,#180121),(#180122,#180123),(#180124,#180125),(#180126,#180127),
(#180128,#180129),(#180130,#180131),(#180132,#180133),(#180134,#180135),
(#180136,#180137),(#180138,#180139),(#180140,#180141),(#180142,#180143),
(#180144,#180145),(#180146,#180147),(#180148,#180149),(#180150,#180151),
(#180152,#180153),(#180154,#180155),(#180156,#180157),(#180158,#180159),
(#180160,#180161),(#180162,#180163),(#180164,#180165),(#180166,#180167),
(#180168,#180169),(#180170,#180171),(#180172,#180173),(#180174,#180175),
(#180176,#180177),(#180178,#180179),(#180180,#180181),(#180182,#180183),
(#180184,#180185),(#180186,#180187),(#180188,#180189),(#180190,#180191),
(#180192,#180193),(#180194,#180195),(#180196,#180197),(#180198,#180199),
(#180200,#180201),(#180202,#180203),(#180204,#180205),(#180206,#180207),
(#180208,#180209),(#180210,#180211),(#180212,#180213),(#180214,#180215),
(#180216,#180217),(#180218,#180219),(#180220,#180221),(#180222,#180223),
(#180224,#180225),(#180226,#180227),(#180228,#180229),(#180230,#180231),
(#180232,#180233),(#180234,#180235),(#180236,#180237),(#180238,#180239),
(#180240,#180241),(#180242,#180243),(#180244,#180245),(#180246,#180247),
(#180248,#180249),(#180250,#180251),(#180252,#180253),(#180254,#180255),
(#180256,#180257),(#180258,#180259),(#180260,#180261),(#180262,#180263),
(#180264,#180265),(#180266,#180267),(#180268,#180269),(#180270,#180271),
(#180272,#180273),(#180274,#180275),(#180276,#180277),(#180278,#180279),
(#180280,#180281),(#180282,#180283),(#180284,#180285),(#180286,#180287),
(#180288,#180289),(#180290,#180291),(#180292,#180293),(#180294,#180295),
(#180296,#180297),(#180298,#180299),(#180300,#180301),(#180302,#180303),
(#180304,#180305),(#180306,#180307),(#180308,#180309),(#180310,#180311),
(#180312,#180313),(#180314,#180315),(#180316,#180317),(#180318,#180319),
(#180320,#180321),(#180322,#180323),(#180324,#180325),(#180326,#180327),
(#180328,#180329),(#180330,#180331),(#180332,#180333),(#180334,#180335),
(#180336,#180337),(#180338,#180339),(#180340,#180341),(#180342,#180343),
(#180344,#180345),(#180346,#180347),(#180348,#180349),(#180350,#180351),
(#180352,#180353),(#180354,#180355),(#180356,#180357),(#180358,#180359),
(#180360,#180361),(#180362,#180363),(#180364,#180365),(#180366,#180367),
(#180368,#180369),(#180370,#180371),(#180372,#180373),(#180374,#180375),
(#180376,#180377),(#180378,#180379),(#180380,#180381),(#180382,#180383),
(#180384,#180385),(#180386,#180387),(#180388,#180389),(#180390,#180391),
(#180392,#180393),(#180394,#180395),(#180396,#180397),(#180398,#180399),
(#180400,#180401),(#180402,#180403),(#180404,#180405),(#180406,#180407),
(#180408,#180409),(#180410,#180411),(#180412,#180413),(#180414,#180415),
(#180416,#180417),(#180418,#180419),(#180420,#180421),(#180422,#180423),
(#180424,#180425),(#180426,#180427),(#180428,#180429),(#180430,#180431),
(#180432,#180433),(#180434,#180435),(#180436,#180437),(#180438,#180439),
(#180440,#180441),(#180442,#180443),(#180444,#180445),(#180446,#180447),
(#180448,#180449),(#180450,#180451),(#180452,#180453),(#180454,#180455),
(#180456,#180457),(#180458,#180459),(#180460,#180461),(#180462,#180463),
(#180464,#180465),(#180466,#180467),(#180468,#180469),(#180470,#180471),
(#180472,#180473),(#180474,#180475),(#180476,#180477),(#180478,#180479),
(#180480,#180481),(#180482,#180483),(#180484,#180485),(#180486,#180487),
(#180488,#180489),(#180490,#180491),(#180492,#180493),(#180494,#180495),
(#180496,#180497),(#180498,#180499),(#180500,#180501),(#180502,#180503),
(#180504,#180505),(#180506,#180507),(#180508,#180509),(#180510,#180511),
(#180512,#180513),(#180514,#180515),(#180516,#180517),(#180518,#180519),
(#180520,#180521),(#180522,#180523),(#180524,#180525),(#180526,#180527),
(#180528,#180529),(#180530,#180531),(#180532,#180533),(#180534,#180535),
(#180536,#180537),(#180538,#180539),(#180540,#180541),(#180542,#180543),
(#180544,#180545),(#180546,#180547),(#180548,#180549),(#180550,#180551),
(#180552,#180553),(#180554,#180555)),.UNSPECIFIED.,.F.,.F.,.F.,(6,1,1,1,
1,1,1,1,1,1,1,1,1,1,1,1,1,1,1,1,1,1,1,1,1,1,1,1,1,1,1,1,1,1,1,1,1,1,1,1,
1,1,1,1,1,1,1,1,1,1,1,1,1,1,1,1,1,1,1,1,1,1,1,1,1,1,1,1,1,1,1,1,1,1,1,1,
1,1,1,1,1,1,1,1,1,1,1,1,1,1,1,1,1,1,1,1,1,1,1,1,1,1,1,1,1,1,1,1,1,1,1,1,
1,1,1,1,1,1,1,1,1,1,1,1,1,1,1,1,1,1,1,1,1,1,1,1,1,1,1,1,1,1,1,1,1,1,1,1,
1,1,1,1,1,1,1,1,1,1,1,1,1,1,1,1,1,1,1,1,1,1,1,1,1,1,1,1,1,1,1,1,1,1,1,1,
1,1,1,1,1,1,1,1,1,1,1,1,1,1,1,1,1,1,1,1,1,1,1,1,1,1,1,1,1,1,1,1,1,1,1,1,
1,1,1,1,1,1,1,1,1,1,1,1,1,1,1,1,1,1,1,1,1,1,1,1,1,1,1,1,1,1,1,1,1,1,1,1,
1,1,1,1,1,1,1,1,1,1,1,1,1,1,1,1,1,1,1,1,1,1,1,1,1,1,1,1,1,1,1,1,1,1,1,1,
1,1,1,1,1,1,1,1,1,1,1,1,1,1,1,1,1,1,1,1,1,1,1,1,1,1,1,1,1,1,1,1,1,1,1,1,
1,1,1,1,1,1,1,1,1,1,1,1,1,1,1,1,1,1,1,1,1,1,1,1,1,1,1,1,1,1,1,1,1,1,1,1,
1,1,1,1,1,1,1,1,1,1,1,1,1,1,1,1,1,1,1,1,1,1,1,1,1,1,1,1,1,1,1,1,1,1,1,1,
1,1,1,1,1,1,1,1,1,1,1,1,1,1,1,1,1,1,1,1,1,1,1,1,1,1,1,1,1,1,1,1,1,1,1,1,
1,1,1,1,1,1,1,1,1,1,1,1,1,1,1,1,1,1,1,1,1,1,1,1,1,1,1,1,1,1,1,6),(2,2),
(0.143172103,0.144954128,0.146788991,0.148623853,0.150458716,0.152293578,
0.15412844,0.155963303,0.157798165,0.159633028,0.16146789,0.163302752,0.165137615,
0.166972477,0.168807339,0.170642202,0.172477064,0.174311927,0.176146789,
0.177981651,0.179816514,0.181651376,0.183486239,0.185321101,0.187155963,
0.188990826,0.190825688,0.19266055,0.194495413,0.196330275,0.198165138,
0.2,0.201834862,0.203669725,0.205504587,0.20733945,0.209174312,0.211009174,
0.212844037,0.214678899,0.216513761,0.218348624,0.220183486,0.222018349,
0.223853211,0.225688073,0.227522936,0.229357798,0.231192661,0.233027523,
0.234862385,0.236697248,0.23853211,0.240366972,0.242201835,0.244036697,
0.24587156,0.247706422,0.249541284,0.251376147,0.253211009,0.255045872,
0.256880734,0.258715596,0.260550459,0.262385321,0.264220183,0.266055046,
0.267889908,0.269724771,0.271559633,0.273394495,0.275229358,0.27706422,
0.278899083,0.280733945,0.282568807,0.28440367,0.286238532,0.288073394,
0.289908257,0.291743119,0.293577982,0.295412844,0.297247706,0.299082569,
0.300917431,0.302752294,0.304587156,0.306422018,0.308256881,0.310091743,
0.311926606,0.313761468,0.31559633,0.317431193,0.319266055,0.321100917,
0.32293578,0.324770642,0.326605505,0.328440367,0.330275229,0.332110092,
0.333944954,0.335779817,0.337614679,0.339449541,0.341284404,0.343119266,
0.344954128,0.346788991,0.348623853,0.350458716,0.352293578,0.35412844,
0.355963303,0.357798165,0.359633028,0.36146789,0.363302752,0.365137615,
0.366972477,0.368807339,0.370642202,0.372477064,0.374311927,0.376146789,
0.377981651,0.379816514,0.381651376,0.383486239,0.385321101,0.387155963,
0.388990826,0.390825688,0.39266055,0.394495413,0.396330275,0.398165138,
0.4,0.401834862,0.403669725,0.405504587,0.40733945,0.409174312,0.411009174,
0.412844037,0.414678899,0.416513761,0.418348624,0.420183486,0.422018349,
0.423853211,0.425688073,0.427522936,0.429357798,0.431192661,0.433027523,
0.434862385,0.436697248,0.43853211,0.440366972,0.442201835,0.444036697,
0.44587156,0.447706422,0.449541284,0.451376147,0.453211009,0.455045872,
0.456880734,0.458715596,0.460550459,0.462385321,0.464220183,0.466055046,
0.467889908,0.469724771,0.471559633,0.473394495,0.475229358,0.47706422,
0.478899083,0.480733945,0.482568807,0.48440367,0.486238532,0.488073394,
0.489908257,0.491743119,0.493577982,0.495412844,0.497247706,0.499082569,
0.500917431,0.502752294,0.504587156,0.506422018,0.508256881,0.510091743,
0.511926606,0.513761468,0.51559633,0.517431193,0.519266055,0.521100917,
0.52293578,0.524770642,0.526605505,0.528440367,0.530275229,0.532110092,
0.533944954,0.535779817,0.537614679,0.539449541,0.541284404,0.543119266,
0.544954128,0.546788991,0.548623853,0.550458716,0.552293578,0.55412844,
0.555963303,0.557798165,0.559633028,0.56146789,0.563302752,0.565137615,
0.566972477,0.568807339,0.570642202,0.572477064,0.574311927,0.576146789,
0.577981651,0.579816514,0.581651376,0.583486239,0.585321101,0.587155963,
0.588990826,0.590825688,0.59266055,0.594495413,0.596330275,0.598165138,
0.6,0.601834862,0.603669725,0.605504587,0.60733945,0.609174312,0.611009174,
0.612844037,0.614678899,0.616513761,0.618348624,0.620183486,0.622018349,
0.623853211,0.625688073,0.627522936,0.629357798,0.631192661,0.633027523,
0.634862385,0.636697248,0.63853211,0.640366972,0.642201835,0.644036697,
0.64587156,0.647706422,0.649541284,0.651376147,0.653211009,0.655045872,
0.656880734,0.658715596,0.660550459,0.662385321,0.664220183,0.666055046,
0.667889908,0.669724771,0.671559633,0.673394495,0.675229358,0.67706422,
0.678899083,0.680733945,0.682568807,0.68440367,0.686238532,0.688073394,
0.689908257,0.691743119,0.693577982,0.695412844,0.697247706,0.699082569,
0.700917431,0.702752294,0.704587156,0.706422018,0.708256881,0.710091743,
0.711926606,0.713761468,0.71559633,0.717431193,0.719266055,0.721100917,
0.72293578,0.724770642,0.726605505,0.728440367,0.730275229,0.732110092,
0.733944954,0.735779817,0.737614679,0.739449541,0.741284404,0.743119266,
0.744954128,0.746788991,0.748623853,0.750458716,0.752293578,0.75412844,
0.755963303,0.757798165,0.759633028,0.76146789,0.763302752,0.765137615,
0.766972477,0.768807339,0.770642202,0.772477064,0.774311927,0.776146789,
0.777981651,0.779816514,0.781651376,0.783486239,0.785321101,0.787155963,
0.788990826,0.790825688,0.79266055,0.794495413,0.796330275,0.798165138,
0.8,0.801834862,0.803669725,0.805504587,0.80733945,0.809174312,0.811009174,
0.812844037,0.814678899,0.816513761,0.818348624,0.820183486,0.822018349,
0.823853211,0.825688073,0.827522936,0.829357798,0.831192661,0.833027523,
0.834862385,0.836697248,0.83853211,0.840366972,0.842201835,0.844036697,
0.84587156,0.847706422,0.849541284,0.851376147,0.853211009,0.855045872,
0.856880734,0.858715596,0.860550459,0.862385321,0.864220183,0.866055046,
0.867889908,0.869724771,0.871559633,0.873394495,0.875229358,0.87706422,
0.878899083,0.880733945,0.882568807,0.88440367,0.886238532,0.888073394,
0.889908257,0.891743119,0.893577982,0.895412844,0.897247706,0.899082569,
0.900917431,0.902752294,0.904587156,0.906422018,0.908256881,0.910091743,
0.911926606,0.913761468,0.91559633,0.917431193,0.919266055,0.921100917,
0.92293578,0.924770642,0.926605505,0.928440367,0.930275229,0.932110092,
0.933944954,0.935779817,0.937614679,0.939449541,0.941284404,0.943119266,
0.944954128,0.946788991,0.948623853,0.950458716,0.952293578,0.95412844,
0.955963303,0.957798165,0.959633028,0.96146789,0.963302752,0.965137615,
0.966972477,0.968807339,0.970642202,0.972477064,0.974311927,0.976146789,
0.977981651,0.979816514,0.981651376,0.983486239,0.985321101,0.987155963,
0.988990826,0.990825688,0.99266055,0.994495413,0.996330275,0.998165138,
1.),(0.,0.36),.UNSPECIFIED.);
#6231=B_SPLINE_SURFACE_WITH_KNOTS('',5,1,((#181212,#181213),(#181214,#181215),
(#181216,#181217),(#181218,#181219),(#181220,#181221),(#181222,#181223),
(#181224,#181225),(#181226,#181227),(#181228,#181229),(#181230,#181231),
(#181232,#181233),(#181234,#181235),(#181236,#181237),(#181238,#181239),
(#181240,#181241),(#181242,#181243),(#181244,#181245),(#181246,#181247),
(#181248,#181249),(#181250,#181251),(#181252,#181253),(#181254,#181255),
(#181256,#181257),(#181258,#181259),(#181260,#181261),(#181262,#181263),
(#181264,#181265),(#181266,#181267),(#181268,#181269),(#181270,#181271),
(#181272,#181273),(#181274,#181275),(#181276,#181277),(#181278,#181279),
(#181280,#181281),(#181282,#181283),(#181284,#181285),(#181286,#181287),
(#181288,#181289),(#181290,#181291),(#181292,#181293),(#181294,#181295),
(#181296,#181297),(#181298,#181299),(#181300,#181301),(#181302,#181303),
(#181304,#181305),(#181306,#181307),(#181308,#181309),(#181310,#181311),
(#181312,#181313),(#181314,#181315),(#181316,#181317),(#181318,#181319),
(#181320,#181321),(#181322,#181323),(#181324,#181325),(#181326,#181327),
(#181328,#181329),(#181330,#181331),(#181332,#181333),(#181334,#181335),
(#181336,#181337),(#181338,#181339),(#181340,#181341),(#181342,#181343),
(#181344,#181345),(#181346,#181347),(#181348,#181349),(#181350,#181351),
(#181352,#181353),(#181354,#181355),(#181356,#181357),(#181358,#181359),
(#181360,#181361),(#181362,#181363),(#181364,#181365),(#181366,#181367),
(#181368,#181369),(#181370,#181371),(#181372,#181373),(#181374,#181375),
(#181376,#181377),(#181378,#181379),(#181380,#181381),(#181382,#181383),
(#181384,#181385),(#181386,#181387),(#181388,#181389),(#181390,#181391),
(#181392,#181393),(#181394,#181395),(#181396,#181397),(#181398,#181399),
(#181400,#181401),(#181402,#181403),(#181404,#181405),(#181406,#181407),
(#181408,#181409),(#181410,#181411),(#181412,#181413),(#181414,#181415),
(#181416,#181417),(#181418,#181419),(#181420,#181421),(#181422,#181423),
(#181424,#181425),(#181426,#181427),(#181428,#181429),(#181430,#181431),
(#181432,#181433),(#181434,#181435),(#181436,#181437),(#181438,#181439),
(#181440,#181441),(#181442,#181443),(#181444,#181445),(#181446,#181447),
(#181448,#181449),(#181450,#181451),(#181452,#181453),(#181454,#181455),
(#181456,#181457),(#181458,#181459),(#181460,#181461),(#181462,#181463),
(#181464,#181465),(#181466,#181467),(#181468,#181469),(#181470,#181471),
(#181472,#181473),(#181474,#181475),(#181476,#181477),(#181478,#181479),
(#181480,#181481),(#181482,#181483),(#181484,#181485),(#181486,#181487),
(#181488,#181489),(#181490,#181491),(#181492,#181493),(#181494,#181495),
(#181496,#181497),(#181498,#181499),(#181500,#181501),(#181502,#181503),
(#181504,#181505),(#181506,#181507),(#181508,#181509),(#181510,#181511),
(#181512,#181513),(#181514,#181515),(#181516,#181517),(#181518,#181519),
(#181520,#181521),(#181522,#181523),(#181524,#181525),(#181526,#181527),
(#181528,#181529),(#181530,#181531),(#181532,#181533),(#181534,#181535),
(#181536,#181537),(#181538,#181539),(#181540,#181541),(#181542,#181543),
(#181544,#181545),(#181546,#181547),(#181548,#181549),(#181550,#181551),
(#181552,#181553),(#181554,#181555),(#181556,#181557),(#181558,#181559),
(#181560,#181561),(#181562,#181563),(#181564,#181565),(#181566,#181567),
(#181568,#181569),(#181570,#181571),(#181572,#181573),(#181574,#181575),
(#181576,#181577),(#181578,#181579),(#181580,#181581),(#181582,#181583),
(#181584,#181585),(#181586,#181587),(#181588,#181589),(#181590,#181591),
(#181592,#181593),(#181594,#181595),(#181596,#181597),(#181598,#181599),
(#181600,#181601),(#181602,#181603),(#181604,#181605),(#181606,#181607),
(#181608,#181609),(#181610,#181611),(#181612,#181613),(#181614,#181615),
(#181616,#181617),(#181618,#181619),(#181620,#181621),(#181622,#181623),
(#181624,#181625),(#181626,#181627),(#181628,#181629),(#181630,#181631),
(#181632,#181633),(#181634,#181635),(#181636,#181637),(#181638,#181639),
(#181640,#181641),(#181642,#181643),(#181644,#181645),(#181646,#181647),
(#181648,#181649),(#181650,#181651),(#181652,#181653),(#181654,#181655),
(#181656,#181657),(#181658,#181659),(#181660,#181661),(#181662,#181663),
(#181664,#181665),(#181666,#181667),(#181668,#181669),(#181670,#181671),
(#181672,#181673),(#181674,#181675),(#181676,#181677),(#181678,#181679),
(#181680,#181681),(#181682,#181683),(#181684,#181685),(#181686,#181687),
(#181688,#181689),(#181690,#181691),(#181692,#181693),(#181694,#181695),
(#181696,#181697),(#181698,#181699),(#181700,#181701),(#181702,#181703),
(#181704,#181705),(#181706,#181707),(#181708,#181709),(#181710,#181711),
(#181712,#181713),(#181714,#181715),(#181716,#181717),(#181718,#181719),
(#181720,#181721),(#181722,#181723),(#181724,#181725),(#181726,#181727),
(#181728,#181729),(#181730,#181731),(#181732,#181733),(#181734,#181735),
(#181736,#181737),(#181738,#181739),(#181740,#181741),(#181742,#181743),
(#181744,#181745),(#181746,#181747),(#181748,#181749),(#181750,#181751),
(#181752,#181753),(#181754,#181755),(#181756,#181757),(#181758,#181759),
(#181760,#181761),(#181762,#181763),(#181764,#181765),(#181766,#181767),
(#181768,#181769),(#181770,#181771),(#181772,#181773),(#181774,#181775),
(#181776,#181777),(#181778,#181779),(#181780,#181781),(#181782,#181783),
(#181784,#181785),(#181786,#181787),(#181788,#181789),(#181790,#181791),
(#181792,#181793),(#181794,#181795),(#181796,#181797),(#181798,#181799),
(#181800,#181801),(#181802,#181803),(#181804,#181805),(#181806,#181807),
(#181808,#181809),(#181810,#181811),(#181812,#181813),(#181814,#181815),
(#181816,#181817),(#181818,#181819),(#181820,#181821),(#181822,#181823),
(#181824,#181825),(#181826,#181827),(#181828,#181829),(#181830,#181831),
(#181832,#181833),(#181834,#181835),(#181836,#181837),(#181838,#181839),
(#181840,#181841),(#181842,#181843),(#181844,#181845),(#181846,#181847),
(#181848,#181849),(#181850,#181851),(#181852,#181853),(#181854,#181855),
(#181856,#181857),(#181858,#181859),(#181860,#181861),(#181862,#181863),
(#181864,#181865),(#181866,#181867),(#181868,#181869),(#181870,#181871),
(#181872,#181873),(#181874,#181875),(#181876,#181877),(#181878,#181879),
(#181880,#181881),(#181882,#181883),(#181884,#181885),(#181886,#181887),
(#181888,#181889),(#181890,#181891),(#181892,#181893),(#181894,#181895),
(#181896,#181897),(#181898,#181899),(#181900,#181901),(#181902,#181903),
(#181904,#181905),(#181906,#181907),(#181908,#181909),(#181910,#181911),
(#181912,#181913),(#181914,#181915),(#181916,#181917),(#181918,#181919),
(#181920,#181921),(#181922,#181923),(#181924,#181925),(#181926,#181927),
(#181928,#181929),(#181930,#181931),(#181932,#181933),(#181934,#181935),
(#181936,#181937),(#181938,#181939),(#181940,#181941),(#181942,#181943),
(#181944,#181945),(#181946,#181947),(#181948,#181949),(#181950,#181951),
(#181952,#181953),(#181954,#181955),(#181956,#181957),(#181958,#181959),
(#181960,#181961),(#181962,#181963),(#181964,#181965),(#181966,#181967),
(#181968,#181969),(#181970,#181971),(#181972,#181973),(#181974,#181975),
(#181976,#181977),(#181978,#181979),(#181980,#181981),(#181982,#181983),
(#181984,#181985),(#181986,#181987),(#181988,#181989),(#181990,#181991),
(#181992,#181993),(#181994,#181995),(#181996,#181997),(#181998,#181999),
(#182000,#182001),(#182002,#182003),(#182004,#182005),(#182006,#182007),
(#182008,#182009),(#182010,#182011),(#182012,#182013),(#182014,#182015),
(#182016,#182017),(#182018,#182019),(#182020,#182021),(#182022,#182023),
(#182024,#182025),(#182026,#182027),(#182028,#182029),(#182030,#182031),
(#182032,#182033),(#182034,#182035),(#182036,#182037),(#182038,#182039),
(#182040,#182041),(#182042,#182043),(#182044,#182045),(#182046,#182047),
(#182048,#182049),(#182050,#182051),(#182052,#182053),(#182054,#182055),
(#182056,#182057),(#182058,#182059),(#182060,#182061),(#182062,#182063),
(#182064,#182065),(#182066,#182067),(#182068,#182069),(#182070,#182071),
(#182072,#182073),(#182074,#182075),(#182076,#182077),(#182078,#182079),
(#182080,#182081),(#182082,#182083),(#182084,#182085),(#182086,#182087),
(#182088,#182089),(#182090,#182091),(#182092,#182093),(#182094,#182095),
(#182096,#182097),(#182098,#182099),(#182100,#182101),(#182102,#182103),
(#182104,#182105),(#182106,#182107),(#182108,#182109),(#182110,#182111),
(#182112,#182113),(#182114,#182115),(#182116,#182117),(#182118,#182119),
(#182120,#182121),(#182122,#182123),(#182124,#182125),(#182126,#182127),
(#182128,#182129),(#182130,#182131),(#182132,#182133),(#182134,#182135),
(#182136,#182137),(#182138,#182139),(#182140,#182141),(#182142,#182143),
(#182144,#182145),(#182146,#182147),(#182148,#182149),(#182150,#182151),
(#182152,#182153),(#182154,#182155)),.UNSPECIFIED.,.F.,.F.,.F.,(6,1,1,1,
1,1,1,1,1,1,1,1,1,1,1,1,1,1,1,1,1,1,1,1,1,1,1,1,1,1,1,1,1,1,1,1,1,1,1,1,
1,1,1,1,1,1,1,1,1,1,1,1,1,1,1,1,1,1,1,1,1,1,1,1,1,1,1,1,1,1,1,1,1,1,1,1,
1,1,1,1,1,1,1,1,1,1,1,1,1,1,1,1,1,1,1,1,1,1,1,1,1,1,1,1,1,1,1,1,1,1,1,1,
1,1,1,1,1,1,1,1,1,1,1,1,1,1,1,1,1,1,1,1,1,1,1,1,1,1,1,1,1,1,1,1,1,1,1,1,
1,1,1,1,1,1,1,1,1,1,1,1,1,1,1,1,1,1,1,1,1,1,1,1,1,1,1,1,1,1,1,1,1,1,1,1,
1,1,1,1,1,1,1,1,1,1,1,1,1,1,1,1,1,1,1,1,1,1,1,1,1,1,1,1,1,1,1,1,1,1,1,1,
1,1,1,1,1,1,1,1,1,1,1,1,1,1,1,1,1,1,1,1,1,1,1,1,1,1,1,1,1,1,1,1,1,1,1,1,
1,1,1,1,1,1,1,1,1,1,1,1,1,1,1,1,1,1,1,1,1,1,1,1,1,1,1,1,1,1,1,1,1,1,1,1,
1,1,1,1,1,1,1,1,1,1,1,1,1,1,1,1,1,1,1,1,1,1,1,1,1,1,1,1,1,1,1,1,1,1,1,1,
1,1,1,1,1,1,1,1,1,1,1,1,1,1,1,1,1,1,1,1,1,1,1,1,1,1,1,1,1,1,1,1,1,1,1,1,
1,1,1,1,1,1,1,1,1,1,1,1,1,1,1,1,1,1,1,1,1,1,1,1,1,1,1,1,1,1,1,1,1,1,1,1,
1,1,1,1,1,1,1,1,1,1,1,1,1,1,1,1,1,1,1,1,1,1,1,1,1,1,1,1,1,1,1,1,1,1,1,1,
1,1,1,1,1,1,1,1,1,1,1,1,1,1,1,1,1,1,1,1,1,1,1,1,1,1,1,1,1,1,1,6),(2,2),
(0.143172103,0.144954128,0.146788991,0.148623853,0.150458716,0.152293578,
0.15412844,0.155963303,0.157798165,0.159633028,0.16146789,0.163302752,0.165137615,
0.166972477,0.168807339,0.170642202,0.172477064,0.174311927,0.176146789,
0.177981651,0.179816514,0.181651376,0.183486239,0.185321101,0.187155963,
0.188990826,0.190825688,0.19266055,0.194495413,0.196330275,0.198165138,
0.2,0.201834862,0.203669725,0.205504587,0.20733945,0.209174312,0.211009174,
0.212844037,0.214678899,0.216513761,0.218348624,0.220183486,0.222018349,
0.223853211,0.225688073,0.227522936,0.229357798,0.231192661,0.233027523,
0.234862385,0.236697248,0.23853211,0.240366972,0.242201835,0.244036697,
0.24587156,0.247706422,0.249541284,0.251376147,0.253211009,0.255045872,
0.256880734,0.258715596,0.260550459,0.262385321,0.264220183,0.266055046,
0.267889908,0.269724771,0.271559633,0.273394495,0.275229358,0.27706422,
0.278899083,0.280733945,0.282568807,0.28440367,0.286238532,0.288073394,
0.289908257,0.291743119,0.293577982,0.295412844,0.297247706,0.299082569,
0.300917431,0.302752294,0.304587156,0.306422018,0.308256881,0.310091743,
0.311926606,0.313761468,0.31559633,0.317431193,0.319266055,0.321100917,
0.32293578,0.324770642,0.326605505,0.328440367,0.330275229,0.332110092,
0.333944954,0.335779817,0.337614679,0.339449541,0.341284404,0.343119266,
0.344954128,0.346788991,0.348623853,0.350458716,0.352293578,0.35412844,
0.355963303,0.357798165,0.359633028,0.36146789,0.363302752,0.365137615,
0.366972477,0.368807339,0.370642202,0.372477064,0.374311927,0.376146789,
0.377981651,0.379816514,0.381651376,0.383486239,0.385321101,0.387155963,
0.388990826,0.390825688,0.39266055,0.394495413,0.396330275,0.398165138,
0.4,0.401834862,0.403669725,0.405504587,0.40733945,0.409174312,0.411009174,
0.412844037,0.414678899,0.416513761,0.418348624,0.420183486,0.422018349,
0.423853211,0.425688073,0.427522936,0.429357798,0.431192661,0.433027523,
0.434862385,0.436697248,0.43853211,0.440366972,0.442201835,0.444036697,
0.44587156,0.447706422,0.449541284,0.451376147,0.453211009,0.455045872,
0.456880734,0.458715596,0.460550459,0.462385321,0.464220183,0.466055046,
0.467889908,0.469724771,0.471559633,0.473394495,0.475229358,0.47706422,
0.478899083,0.480733945,0.482568807,0.48440367,0.486238532,0.488073394,
0.489908257,0.491743119,0.493577982,0.495412844,0.497247706,0.499082569,
0.500917431,0.502752294,0.504587156,0.506422018,0.508256881,0.510091743,
0.511926606,0.513761468,0.51559633,0.517431193,0.519266055,0.521100917,
0.52293578,0.524770642,0.526605505,0.528440367,0.530275229,0.532110092,
0.533944954,0.535779817,0.537614679,0.539449541,0.541284404,0.543119266,
0.544954128,0.546788991,0.548623853,0.550458716,0.552293578,0.55412844,
0.555963303,0.557798165,0.559633028,0.56146789,0.563302752,0.565137615,
0.566972477,0.568807339,0.570642202,0.572477064,0.574311927,0.576146789,
0.577981651,0.579816514,0.581651376,0.583486239,0.585321101,0.587155963,
0.588990826,0.590825688,0.59266055,0.594495413,0.596330275,0.598165138,
0.6,0.601834862,0.603669725,0.605504587,0.60733945,0.609174312,0.611009174,
0.612844037,0.614678899,0.616513761,0.618348624,0.620183486,0.622018349,
0.623853211,0.625688073,0.627522936,0.629357798,0.631192661,0.633027523,
0.634862385,0.636697248,0.63853211,0.640366972,0.642201835,0.644036697,
0.64587156,0.647706422,0.649541284,0.651376147,0.653211009,0.655045872,
0.656880734,0.658715596,0.660550459,0.662385321,0.664220183,0.666055046,
0.667889908,0.669724771,0.671559633,0.673394495,0.675229358,0.67706422,
0.678899083,0.680733945,0.682568807,0.68440367,0.686238532,0.688073394,
0.689908257,0.691743119,0.693577982,0.695412844,0.697247706,0.699082569,
0.700917431,0.702752294,0.704587156,0.706422018,0.708256881,0.710091743,
0.711926606,0.713761468,0.71559633,0.717431193,0.719266055,0.721100917,
0.72293578,0.724770642,0.726605505,0.728440367,0.730275229,0.732110092,
0.733944954,0.735779817,0.737614679,0.739449541,0.741284404,0.743119266,
0.744954128,0.746788991,0.748623853,0.750458716,0.752293578,0.75412844,
0.755963303,0.757798165,0.759633028,0.76146789,0.763302752,0.765137615,
0.766972477,0.768807339,0.770642202,0.772477064,0.774311927,0.776146789,
0.777981651,0.779816514,0.781651376,0.783486239,0.785321101,0.787155963,
0.788990826,0.790825688,0.79266055,0.794495413,0.796330275,0.798165138,
0.8,0.801834862,0.803669725,0.805504587,0.80733945,0.809174312,0.811009174,
0.812844037,0.814678899,0.816513761,0.818348624,0.820183486,0.822018349,
0.823853211,0.825688073,0.827522936,0.829357798,0.831192661,0.833027523,
0.834862385,0.836697248,0.83853211,0.840366972,0.842201835,0.844036697,
0.84587156,0.847706422,0.849541284,0.851376147,0.853211009,0.855045872,
0.856880734,0.858715596,0.860550459,0.862385321,0.864220183,0.866055046,
0.867889908,0.869724771,0.871559633,0.873394495,0.875229358,0.87706422,
0.878899083,0.880733945,0.882568807,0.88440367,0.886238532,0.888073394,
0.889908257,0.891743119,0.893577982,0.895412844,0.897247706,0.899082569,
0.900917431,0.902752294,0.904587156,0.906422018,0.908256881,0.910091743,
0.911926606,0.913761468,0.91559633,0.917431193,0.919266055,0.921100917,
0.92293578,0.924770642,0.926605505,0.928440367,0.930275229,0.932110092,
0.933944954,0.935779817,0.937614679,0.939449541,0.941284404,0.943119266,
0.944954128,0.946788991,0.948623853,0.950458716,0.952293578,0.95412844,
0.955963303,0.957798165,0.959633028,0.96146789,0.963302752,0.965137615,
0.966972477,0.968807339,0.970642202,0.972477064,0.974311927,0.976146789,
0.977981651,0.979816514,0.981651376,0.983486239,0.985321101,0.987155963,
0.988990826,0.990825688,0.99266055,0.994495413,0.996330275,0.998165138,
1.),(0.,0.36),.UNSPECIFIED.);
#6232=B_SPLINE_SURFACE_WITH_KNOTS('',5,1,((#182788,#182789),(#182790,#182791),
(#182792,#182793),(#182794,#182795),(#182796,#182797),(#182798,#182799),
(#182800,#182801),(#182802,#182803),(#182804,#182805),(#182806,#182807),
(#182808,#182809),(#182810,#182811),(#182812,#182813),(#182814,#182815),
(#182816,#182817),(#182818,#182819),(#182820,#182821),(#182822,#182823),
(#182824,#182825),(#182826,#182827),(#182828,#182829),(#182830,#182831),
(#182832,#182833),(#182834,#182835),(#182836,#182837),(#182838,#182839),
(#182840,#182841),(#182842,#182843),(#182844,#182845),(#182846,#182847),
(#182848,#182849),(#182850,#182851),(#182852,#182853),(#182854,#182855),
(#182856,#182857),(#182858,#182859),(#182860,#182861),(#182862,#182863),
(#182864,#182865),(#182866,#182867),(#182868,#182869),(#182870,#182871),
(#182872,#182873),(#182874,#182875),(#182876,#182877),(#182878,#182879),
(#182880,#182881),(#182882,#182883),(#182884,#182885),(#182886,#182887),
(#182888,#182889),(#182890,#182891),(#182892,#182893),(#182894,#182895),
(#182896,#182897),(#182898,#182899),(#182900,#182901),(#182902,#182903),
(#182904,#182905),(#182906,#182907),(#182908,#182909),(#182910,#182911),
(#182912,#182913),(#182914,#182915),(#182916,#182917),(#182918,#182919),
(#182920,#182921),(#182922,#182923),(#182924,#182925),(#182926,#182927),
(#182928,#182929),(#182930,#182931),(#182932,#182933),(#182934,#182935),
(#182936,#182937),(#182938,#182939),(#182940,#182941),(#182942,#182943),
(#182944,#182945),(#182946,#182947),(#182948,#182949),(#182950,#182951),
(#182952,#182953),(#182954,#182955),(#182956,#182957),(#182958,#182959),
(#182960,#182961),(#182962,#182963),(#182964,#182965),(#182966,#182967),
(#182968,#182969),(#182970,#182971),(#182972,#182973),(#182974,#182975),
(#182976,#182977),(#182978,#182979),(#182980,#182981),(#182982,#182983),
(#182984,#182985),(#182986,#182987),(#182988,#182989),(#182990,#182991),
(#182992,#182993),(#182994,#182995),(#182996,#182997),(#182998,#182999),
(#183000,#183001),(#183002,#183003),(#183004,#183005),(#183006,#183007),
(#183008,#183009),(#183010,#183011),(#183012,#183013),(#183014,#183015),
(#183016,#183017),(#183018,#183019),(#183020,#183021),(#183022,#183023),
(#183024,#183025),(#183026,#183027),(#183028,#183029),(#183030,#183031),
(#183032,#183033),(#183034,#183035),(#183036,#183037),(#183038,#183039),
(#183040,#183041),(#183042,#183043),(#183044,#183045),(#183046,#183047),
(#183048,#183049),(#183050,#183051),(#183052,#183053),(#183054,#183055),
(#183056,#183057),(#183058,#183059),(#183060,#183061),(#183062,#183063),
(#183064,#183065),(#183066,#183067),(#183068,#183069),(#183070,#183071),
(#183072,#183073),(#183074,#183075),(#183076,#183077),(#183078,#183079),
(#183080,#183081),(#183082,#183083),(#183084,#183085),(#183086,#183087),
(#183088,#183089),(#183090,#183091),(#183092,#183093),(#183094,#183095),
(#183096,#183097),(#183098,#183099),(#183100,#183101),(#183102,#183103),
(#183104,#183105),(#183106,#183107),(#183108,#183109),(#183110,#183111),
(#183112,#183113),(#183114,#183115),(#183116,#183117),(#183118,#183119),
(#183120,#183121),(#183122,#183123),(#183124,#183125),(#183126,#183127),
(#183128,#183129),(#183130,#183131),(#183132,#183133),(#183134,#183135),
(#183136,#183137),(#183138,#183139),(#183140,#183141),(#183142,#183143),
(#183144,#183145),(#183146,#183147),(#183148,#183149),(#183150,#183151),
(#183152,#183153),(#183154,#183155),(#183156,#183157),(#183158,#183159),
(#183160,#183161),(#183162,#183163),(#183164,#183165),(#183166,#183167),
(#183168,#183169),(#183170,#183171),(#183172,#183173),(#183174,#183175),
(#183176,#183177),(#183178,#183179),(#183180,#183181),(#183182,#183183),
(#183184,#183185),(#183186,#183187),(#183188,#183189),(#183190,#183191),
(#183192,#183193),(#183194,#183195),(#183196,#183197),(#183198,#183199),
(#183200,#183201),(#183202,#183203),(#183204,#183205),(#183206,#183207),
(#183208,#183209),(#183210,#183211),(#183212,#183213),(#183214,#183215),
(#183216,#183217),(#183218,#183219),(#183220,#183221),(#183222,#183223),
(#183224,#183225),(#183226,#183227),(#183228,#183229),(#183230,#183231),
(#183232,#183233),(#183234,#183235),(#183236,#183237),(#183238,#183239),
(#183240,#183241),(#183242,#183243),(#183244,#183245),(#183246,#183247),
(#183248,#183249),(#183250,#183251),(#183252,#183253),(#183254,#183255),
(#183256,#183257),(#183258,#183259),(#183260,#183261),(#183262,#183263),
(#183264,#183265),(#183266,#183267),(#183268,#183269),(#183270,#183271),
(#183272,#183273),(#183274,#183275),(#183276,#183277),(#183278,#183279),
(#183280,#183281),(#183282,#183283),(#183284,#183285),(#183286,#183287),
(#183288,#183289),(#183290,#183291),(#183292,#183293),(#183294,#183295),
(#183296,#183297),(#183298,#183299),(#183300,#183301),(#183302,#183303),
(#183304,#183305),(#183306,#183307),(#183308,#183309),(#183310,#183311),
(#183312,#183313),(#183314,#183315),(#183316,#183317),(#183318,#183319),
(#183320,#183321),(#183322,#183323),(#183324,#183325),(#183326,#183327),
(#183328,#183329),(#183330,#183331),(#183332,#183333),(#183334,#183335),
(#183336,#183337),(#183338,#183339),(#183340,#183341),(#183342,#183343),
(#183344,#183345),(#183346,#183347),(#183348,#183349),(#183350,#183351),
(#183352,#183353),(#183354,#183355),(#183356,#183357),(#183358,#183359),
(#183360,#183361),(#183362,#183363),(#183364,#183365),(#183366,#183367),
(#183368,#183369),(#183370,#183371),(#183372,#183373),(#183374,#183375),
(#183376,#183377),(#183378,#183379),(#183380,#183381),(#183382,#183383),
(#183384,#183385),(#183386,#183387),(#183388,#183389),(#183390,#183391),
(#183392,#183393),(#183394,#183395),(#183396,#183397),(#183398,#183399),
(#183400,#183401),(#183402,#183403),(#183404,#183405),(#183406,#183407),
(#183408,#183409),(#183410,#183411),(#183412,#183413),(#183414,#183415),
(#183416,#183417),(#183418,#183419),(#183420,#183421),(#183422,#183423),
(#183424,#183425),(#183426,#183427),(#183428,#183429),(#183430,#183431),
(#183432,#183433),(#183434,#183435),(#183436,#183437),(#183438,#183439),
(#183440,#183441),(#183442,#183443),(#183444,#183445),(#183446,#183447),
(#183448,#183449),(#183450,#183451),(#183452,#183453),(#183454,#183455),
(#183456,#183457),(#183458,#183459),(#183460,#183461),(#183462,#183463),
(#183464,#183465),(#183466,#183467),(#183468,#183469),(#183470,#183471),
(#183472,#183473),(#183474,#183475),(#183476,#183477),(#183478,#183479),
(#183480,#183481),(#183482,#183483),(#183484,#183485),(#183486,#183487),
(#183488,#183489),(#183490,#183491),(#183492,#183493),(#183494,#183495),
(#183496,#183497),(#183498,#183499),(#183500,#183501),(#183502,#183503),
(#183504,#183505),(#183506,#183507),(#183508,#183509),(#183510,#183511),
(#183512,#183513),(#183514,#183515),(#183516,#183517),(#183518,#183519),
(#183520,#183521),(#183522,#183523),(#183524,#183525),(#183526,#183527),
(#183528,#183529),(#183530,#183531),(#183532,#183533),(#183534,#183535),
(#183536,#183537),(#183538,#183539),(#183540,#183541),(#183542,#183543),
(#183544,#183545),(#183546,#183547),(#183548,#183549),(#183550,#183551),
(#183552,#183553),(#183554,#183555),(#183556,#183557),(#183558,#183559),
(#183560,#183561),(#183562,#183563),(#183564,#183565),(#183566,#183567),
(#183568,#183569),(#183570,#183571),(#183572,#183573),(#183574,#183575),
(#183576,#183577),(#183578,#183579),(#183580,#183581),(#183582,#183583),
(#183584,#183585),(#183586,#183587),(#183588,#183589),(#183590,#183591),
(#183592,#183593),(#183594,#183595),(#183596,#183597),(#183598,#183599),
(#183600,#183601),(#183602,#183603),(#183604,#183605),(#183606,#183607),
(#183608,#183609),(#183610,#183611),(#183612,#183613),(#183614,#183615),
(#183616,#183617),(#183618,#183619),(#183620,#183621),(#183622,#183623),
(#183624,#183625),(#183626,#183627),(#183628,#183629),(#183630,#183631),
(#183632,#183633),(#183634,#183635),(#183636,#183637),(#183638,#183639),
(#183640,#183641),(#183642,#183643),(#183644,#183645),(#183646,#183647),
(#183648,#183649),(#183650,#183651),(#183652,#183653),(#183654,#183655),
(#183656,#183657),(#183658,#183659),(#183660,#183661),(#183662,#183663),
(#183664,#183665),(#183666,#183667),(#183668,#183669),(#183670,#183671),
(#183672,#183673),(#183674,#183675),(#183676,#183677),(#183678,#183679),
(#183680,#183681),(#183682,#183683),(#183684,#183685),(#183686,#183687),
(#183688,#183689),(#183690,#183691),(#183692,#183693),(#183694,#183695),
(#183696,#183697),(#183698,#183699),(#183700,#183701),(#183702,#183703),
(#183704,#183705),(#183706,#183707),(#183708,#183709),(#183710,#183711),
(#183712,#183713),(#183714,#183715),(#183716,#183717),(#183718,#183719),
(#183720,#183721),(#183722,#183723),(#183724,#183725),(#183726,#183727),
(#183728,#183729),(#183730,#183731)),.UNSPECIFIED.,.F.,.F.,.F.,(6,1,1,1,
1,1,1,1,1,1,1,1,1,1,1,1,1,1,1,1,1,1,1,1,1,1,1,1,1,1,1,1,1,1,1,1,1,1,1,1,
1,1,1,1,1,1,1,1,1,1,1,1,1,1,1,1,1,1,1,1,1,1,1,1,1,1,1,1,1,1,1,1,1,1,1,1,
1,1,1,1,1,1,1,1,1,1,1,1,1,1,1,1,1,1,1,1,1,1,1,1,1,1,1,1,1,1,1,1,1,1,1,1,
1,1,1,1,1,1,1,1,1,1,1,1,1,1,1,1,1,1,1,1,1,1,1,1,1,1,1,1,1,1,1,1,1,1,1,1,
1,1,1,1,1,1,1,1,1,1,1,1,1,1,1,1,1,1,1,1,1,1,1,1,1,1,1,1,1,1,1,1,1,1,1,1,
1,1,1,1,1,1,1,1,1,1,1,1,1,1,1,1,1,1,1,1,1,1,1,1,1,1,1,1,1,1,1,1,1,1,1,1,
1,1,1,1,1,1,1,1,1,1,1,1,1,1,1,1,1,1,1,1,1,1,1,1,1,1,1,1,1,1,1,1,1,1,1,1,
1,1,1,1,1,1,1,1,1,1,1,1,1,1,1,1,1,1,1,1,1,1,1,1,1,1,1,1,1,1,1,1,1,1,1,1,
1,1,1,1,1,1,1,1,1,1,1,1,1,1,1,1,1,1,1,1,1,1,1,1,1,1,1,1,1,1,1,1,1,1,1,1,
1,1,1,1,1,1,1,1,1,1,1,1,1,1,1,1,1,1,1,1,1,1,1,1,1,1,1,1,1,1,1,1,1,1,1,1,
1,1,1,1,1,1,1,1,1,1,1,1,1,1,1,1,1,1,1,1,1,1,1,1,1,1,1,1,1,1,1,1,1,1,1,1,
1,1,1,1,1,1,1,1,1,1,1,1,1,1,1,1,1,1,1,1,1,1,1,1,1,1,1,1,1,1,1,1,1,1,1,1,
1,1,1,1,1,1,1,1,1,1,1,1,1,1,1,1,1,1,1,1,1,1,1,1,1,1,1,1,1,1,1,6),(2,2),
(-1.,-0.998165138,-0.996330275,-0.994495413,-0.99266055,-0.990825688,-0.988990826,
-0.987155963,-0.985321101,-0.983486239,-0.981651376,-0.979816514,-0.977981651,
-0.976146789,-0.974311927,-0.972477064,-0.970642202,-0.968807339,-0.966972477,
-0.965137615,-0.963302752,-0.96146789,-0.959633028,-0.957798165,-0.955963303,
-0.95412844,-0.952293578,-0.950458716,-0.948623853,-0.946788991,-0.944954128,
-0.943119266,-0.941284404,-0.939449541,-0.937614679,-0.935779817,-0.933944954,
-0.932110092,-0.930275229,-0.928440367,-0.926605505,-0.924770642,-0.92293578,
-0.921100917,-0.919266055,-0.917431193,-0.91559633,-0.913761468,-0.911926606,
-0.910091743,-0.908256881,-0.906422018,-0.904587156,-0.902752294,-0.900917431,
-0.899082569,-0.897247706,-0.895412844,-0.893577982,-0.891743119,-0.889908257,
-0.888073394,-0.886238532,-0.88440367,-0.882568807,-0.880733945,-0.878899083,
-0.87706422,-0.875229358,-0.873394495,-0.871559633,-0.869724771,-0.867889908,
-0.866055046,-0.864220183,-0.862385321,-0.860550459,-0.858715596,-0.856880734,
-0.855045872,-0.853211009,-0.851376147,-0.849541284,-0.847706422,-0.84587156,
-0.844036697,-0.842201835,-0.840366972,-0.83853211,-0.836697248,-0.834862385,
-0.833027523,-0.831192661,-0.829357798,-0.827522936,-0.825688073,-0.823853211,
-0.822018349,-0.820183486,-0.818348624,-0.816513761,-0.814678899,-0.812844037,
-0.811009174,-0.809174312,-0.80733945,-0.805504587,-0.803669725,-0.801834862,
-0.8,-0.798165138,-0.796330275,-0.794495413,-0.79266055,-0.790825688,-0.788990826,
-0.787155963,-0.785321101,-0.783486239,-0.781651376,-0.779816514,-0.777981651,
-0.776146789,-0.774311927,-0.772477064,-0.770642202,-0.768807339,-0.766972477,
-0.765137615,-0.763302752,-0.76146789,-0.759633028,-0.757798165,-0.755963303,
-0.75412844,-0.752293578,-0.750458716,-0.748623853,-0.746788991,-0.744954128,
-0.743119266,-0.741284404,-0.739449541,-0.737614679,-0.735779817,-0.733944954,
-0.732110092,-0.730275229,-0.728440367,-0.726605505,-0.724770642,-0.72293578,
-0.721100917,-0.719266055,-0.717431193,-0.71559633,-0.713761468,-0.711926606,
-0.710091743,-0.708256881,-0.706422018,-0.704587156,-0.702752294,-0.700917431,
-0.699082569,-0.697247706,-0.695412844,-0.693577982,-0.691743119,-0.689908257,
-0.688073394,-0.686238532,-0.68440367,-0.682568807,-0.680733945,-0.678899083,
-0.67706422,-0.675229358,-0.673394495,-0.671559633,-0.669724771,-0.667889908,
-0.666055046,-0.664220183,-0.662385321,-0.660550459,-0.658715596,-0.656880734,
-0.655045872,-0.653211009,-0.651376147,-0.649541284,-0.647706422,-0.64587156,
-0.644036697,-0.642201835,-0.640366972,-0.63853211,-0.636697248,-0.634862385,
-0.633027523,-0.631192661,-0.629357798,-0.627522936,-0.625688073,-0.623853211,
-0.622018349,-0.620183486,-0.618348624,-0.616513761,-0.614678899,-0.612844037,
-0.611009174,-0.609174312,-0.60733945,-0.605504587,-0.603669725,-0.601834862,
-0.6,-0.598165138,-0.596330275,-0.594495413,-0.59266055,-0.590825688,-0.588990826,
-0.587155963,-0.585321101,-0.583486239,-0.581651376,-0.579816514,-0.577981651,
-0.576146789,-0.574311927,-0.572477064,-0.570642202,-0.568807339,-0.566972477,
-0.565137615,-0.563302752,-0.56146789,-0.559633028,-0.557798165,-0.555963303,
-0.55412844,-0.552293578,-0.550458716,-0.548623853,-0.546788991,-0.544954128,
-0.543119266,-0.541284404,-0.539449541,-0.537614679,-0.535779817,-0.533944954,
-0.532110092,-0.530275229,-0.528440367,-0.526605505,-0.524770642,-0.52293578,
-0.521100917,-0.519266055,-0.517431193,-0.51559633,-0.513761468,-0.511926606,
-0.510091743,-0.508256881,-0.506422018,-0.504587156,-0.502752294,-0.500917431,
-0.499082569,-0.497247706,-0.495412844,-0.493577982,-0.491743119,-0.489908257,
-0.488073394,-0.486238532,-0.48440367,-0.482568807,-0.480733945,-0.478899083,
-0.47706422,-0.475229358,-0.473394495,-0.471559633,-0.469724771,-0.467889908,
-0.466055046,-0.464220183,-0.462385321,-0.460550459,-0.458715596,-0.456880734,
-0.455045872,-0.453211009,-0.451376147,-0.449541284,-0.447706422,-0.44587156,
-0.444036697,-0.442201835,-0.440366972,-0.43853211,-0.436697248,-0.434862385,
-0.433027523,-0.431192661,-0.429357798,-0.427522936,-0.425688073,-0.423853211,
-0.422018349,-0.420183486,-0.418348624,-0.416513761,-0.414678899,-0.412844037,
-0.411009174,-0.409174312,-0.40733945,-0.405504587,-0.403669725,-0.401834862,
-0.4,-0.398165138,-0.396330275,-0.394495413,-0.39266055,-0.390825688,-0.388990826,
-0.387155963,-0.385321101,-0.383486239,-0.381651376,-0.379816514,-0.377981651,
-0.376146789,-0.374311927,-0.372477064,-0.370642202,-0.368807339,-0.366972477,
-0.365137615,-0.363302752,-0.36146789,-0.359633028,-0.357798165,-0.355963303,
-0.35412844,-0.352293578,-0.350458716,-0.348623853,-0.346788991,-0.344954128,
-0.343119266,-0.341284404,-0.339449541,-0.337614679,-0.335779817,-0.333944954,
-0.332110092,-0.330275229,-0.328440367,-0.326605505,-0.324770642,-0.32293578,
-0.321100917,-0.319266055,-0.317431193,-0.31559633,-0.313761468,-0.311926606,
-0.310091743,-0.308256881,-0.306422018,-0.304587156,-0.302752294,-0.300917431,
-0.299082569,-0.297247706,-0.295412844,-0.293577982,-0.291743119,-0.289908257,
-0.288073394,-0.286238532,-0.28440367,-0.282568807,-0.280733945,-0.278899083,
-0.27706422,-0.275229358,-0.273394495,-0.271559633,-0.269724771,-0.267889908,
-0.266055046,-0.264220183,-0.262385321,-0.260550459,-0.258715596,-0.256880734,
-0.255045872,-0.253211009,-0.251376147,-0.249541284,-0.247706422,-0.24587156,
-0.244036697,-0.242201835,-0.240366972,-0.23853211,-0.236697248,-0.234862385,
-0.233027523,-0.231192661,-0.229357798,-0.227522936,-0.225688073,-0.223853211,
-0.222018349,-0.220183486,-0.218348624,-0.216513761,-0.214678899,-0.212844037,
-0.211009174,-0.209174312,-0.20733945,-0.205504587,-0.203669725,-0.201834862,
-0.2,-0.198165138,-0.196330275,-0.194495413,-0.19266055,-0.190825688,-0.188990826,
-0.187155963,-0.185321101,-0.183486239,-0.181651376,-0.179816514,-0.177981651,
-0.176146789,-0.174311927,-0.172477064,-0.170642202,-0.168807339,-0.166972477,
-0.165137615,-0.163302752,-0.16146789,-0.159633028,-0.157798165,-0.155963303,
-0.15412844,-0.152293578,-0.150458716,-0.148623853,-0.146788991,-0.144954128,
-0.143172103),(0.,0.36),.UNSPECIFIED.);
#6233=B_SPLINE_SURFACE_WITH_KNOTS('',5,1,((#184694,#184695),(#184696,#184697),
(#184698,#184699),(#184700,#184701),(#184702,#184703),(#184704,#184705),
(#184706,#184707),(#184708,#184709),(#184710,#184711),(#184712,#184713),
(#184714,#184715),(#184716,#184717),(#184718,#184719),(#184720,#184721),
(#184722,#184723),(#184724,#184725),(#184726,#184727),(#184728,#184729),
(#184730,#184731),(#184732,#184733),(#184734,#184735),(#184736,#184737),
(#184738,#184739),(#184740,#184741),(#184742,#184743),(#184744,#184745),
(#184746,#184747),(#184748,#184749),(#184750,#184751),(#184752,#184753),
(#184754,#184755),(#184756,#184757),(#184758,#184759),(#184760,#184761),
(#184762,#184763),(#184764,#184765),(#184766,#184767),(#184768,#184769),
(#184770,#184771),(#184772,#184773),(#184774,#184775),(#184776,#184777),
(#184778,#184779),(#184780,#184781),(#184782,#184783),(#184784,#184785),
(#184786,#184787),(#184788,#184789),(#184790,#184791),(#184792,#184793),
(#184794,#184795),(#184796,#184797),(#184798,#184799),(#184800,#184801),
(#184802,#184803),(#184804,#184805),(#184806,#184807),(#184808,#184809),
(#184810,#184811),(#184812,#184813),(#184814,#184815),(#184816,#184817),
(#184818,#184819),(#184820,#184821),(#184822,#184823),(#184824,#184825),
(#184826,#184827),(#184828,#184829),(#184830,#184831),(#184832,#184833),
(#184834,#184835),(#184836,#184837),(#184838,#184839),(#184840,#184841),
(#184842,#184843),(#184844,#184845),(#184846,#184847),(#184848,#184849),
(#184850,#184851),(#184852,#184853),(#184854,#184855),(#184856,#184857),
(#184858,#184859),(#184860,#184861),(#184862,#184863),(#184864,#184865),
(#184866,#184867),(#184868,#184869),(#184870,#184871),(#184872,#184873),
(#184874,#184875),(#184876,#184877),(#184878,#184879),(#184880,#184881),
(#184882,#184883),(#184884,#184885),(#184886,#184887),(#184888,#184889),
(#184890,#184891),(#184892,#184893),(#184894,#184895),(#184896,#184897),
(#184898,#184899),(#184900,#184901),(#184902,#184903),(#184904,#184905),
(#184906,#184907),(#184908,#184909),(#184910,#184911),(#184912,#184913),
(#184914,#184915),(#184916,#184917),(#184918,#184919),(#184920,#184921),
(#184922,#184923),(#184924,#184925),(#184926,#184927),(#184928,#184929),
(#184930,#184931),(#184932,#184933),(#184934,#184935),(#184936,#184937),
(#184938,#184939),(#184940,#184941),(#184942,#184943),(#184944,#184945),
(#184946,#184947),(#184948,#184949),(#184950,#184951),(#184952,#184953),
(#184954,#184955),(#184956,#184957),(#184958,#184959),(#184960,#184961),
(#184962,#184963),(#184964,#184965),(#184966,#184967),(#184968,#184969),
(#184970,#184971),(#184972,#184973),(#184974,#184975),(#184976,#184977),
(#184978,#184979),(#184980,#184981),(#184982,#184983),(#184984,#184985),
(#184986,#184987),(#184988,#184989),(#184990,#184991),(#184992,#184993),
(#184994,#184995),(#184996,#184997),(#184998,#184999),(#185000,#185001),
(#185002,#185003),(#185004,#185005),(#185006,#185007),(#185008,#185009),
(#185010,#185011),(#185012,#185013),(#185014,#185015),(#185016,#185017),
(#185018,#185019),(#185020,#185021),(#185022,#185023),(#185024,#185025),
(#185026,#185027),(#185028,#185029),(#185030,#185031),(#185032,#185033),
(#185034,#185035),(#185036,#185037),(#185038,#185039),(#185040,#185041),
(#185042,#185043),(#185044,#185045),(#185046,#185047),(#185048,#185049),
(#185050,#185051),(#185052,#185053),(#185054,#185055),(#185056,#185057),
(#185058,#185059),(#185060,#185061),(#185062,#185063),(#185064,#185065),
(#185066,#185067),(#185068,#185069),(#185070,#185071),(#185072,#185073),
(#185074,#185075),(#185076,#185077),(#185078,#185079),(#185080,#185081),
(#185082,#185083),(#185084,#185085),(#185086,#185087),(#185088,#185089),
(#185090,#185091),(#185092,#185093),(#185094,#185095),(#185096,#185097),
(#185098,#185099),(#185100,#185101),(#185102,#185103),(#185104,#185105),
(#185106,#185107),(#185108,#185109),(#185110,#185111),(#185112,#185113),
(#185114,#185115),(#185116,#185117),(#185118,#185119),(#185120,#185121),
(#185122,#185123),(#185124,#185125),(#185126,#185127),(#185128,#185129),
(#185130,#185131),(#185132,#185133),(#185134,#185135),(#185136,#185137),
(#185138,#185139),(#185140,#185141),(#185142,#185143),(#185144,#185145),
(#185146,#185147),(#185148,#185149),(#185150,#185151),(#185152,#185153),
(#185154,#185155),(#185156,#185157),(#185158,#185159),(#185160,#185161),
(#185162,#185163),(#185164,#185165),(#185166,#185167),(#185168,#185169),
(#185170,#185171),(#185172,#185173),(#185174,#185175),(#185176,#185177),
(#185178,#185179),(#185180,#185181),(#185182,#185183),(#185184,#185185),
(#185186,#185187),(#185188,#185189),(#185190,#185191),(#185192,#185193),
(#185194,#185195),(#185196,#185197),(#185198,#185199),(#185200,#185201),
(#185202,#185203),(#185204,#185205),(#185206,#185207),(#185208,#185209),
(#185210,#185211),(#185212,#185213),(#185214,#185215),(#185216,#185217),
(#185218,#185219),(#185220,#185221),(#185222,#185223),(#185224,#185225),
(#185226,#185227),(#185228,#185229),(#185230,#185231),(#185232,#185233),
(#185234,#185235),(#185236,#185237),(#185238,#185239),(#185240,#185241),
(#185242,#185243),(#185244,#185245),(#185246,#185247),(#185248,#185249),
(#185250,#185251),(#185252,#185253),(#185254,#185255),(#185256,#185257),
(#185258,#185259),(#185260,#185261),(#185262,#185263),(#185264,#185265),
(#185266,#185267),(#185268,#185269),(#185270,#185271),(#185272,#185273),
(#185274,#185275),(#185276,#185277),(#185278,#185279),(#185280,#185281),
(#185282,#185283),(#185284,#185285),(#185286,#185287),(#185288,#185289),
(#185290,#185291),(#185292,#185293),(#185294,#185295),(#185296,#185297),
(#185298,#185299),(#185300,#185301),(#185302,#185303),(#185304,#185305),
(#185306,#185307),(#185308,#185309),(#185310,#185311),(#185312,#185313),
(#185314,#185315),(#185316,#185317),(#185318,#185319),(#185320,#185321),
(#185322,#185323),(#185324,#185325),(#185326,#185327),(#185328,#185329),
(#185330,#185331),(#185332,#185333),(#185334,#185335),(#185336,#185337),
(#185338,#185339),(#185340,#185341),(#185342,#185343),(#185344,#185345),
(#185346,#185347),(#185348,#185349),(#185350,#185351),(#185352,#185353),
(#185354,#185355),(#185356,#185357),(#185358,#185359),(#185360,#185361),
(#185362,#185363),(#185364,#185365),(#185366,#185367),(#185368,#185369),
(#185370,#185371),(#185372,#185373),(#185374,#185375),(#185376,#185377),
(#185378,#185379),(#185380,#185381),(#185382,#185383),(#185384,#185385),
(#185386,#185387),(#185388,#185389),(#185390,#185391),(#185392,#185393),
(#185394,#185395),(#185396,#185397),(#185398,#185399),(#185400,#185401),
(#185402,#185403),(#185404,#185405),(#185406,#185407),(#185408,#185409),
(#185410,#185411),(#185412,#185413),(#185414,#185415),(#185416,#185417),
(#185418,#185419),(#185420,#185421),(#185422,#185423),(#185424,#185425),
(#185426,#185427),(#185428,#185429),(#185430,#185431),(#185432,#185433),
(#185434,#185435),(#185436,#185437),(#185438,#185439),(#185440,#185441),
(#185442,#185443),(#185444,#185445),(#185446,#185447),(#185448,#185449),
(#185450,#185451),(#185452,#185453),(#185454,#185455),(#185456,#185457),
(#185458,#185459),(#185460,#185461),(#185462,#185463),(#185464,#185465),
(#185466,#185467),(#185468,#185469),(#185470,#185471),(#185472,#185473),
(#185474,#185475),(#185476,#185477),(#185478,#185479),(#185480,#185481),
(#185482,#185483),(#185484,#185485),(#185486,#185487),(#185488,#185489),
(#185490,#185491),(#185492,#185493),(#185494,#185495),(#185496,#185497),
(#185498,#185499),(#185500,#185501),(#185502,#185503),(#185504,#185505),
(#185506,#185507),(#185508,#185509),(#185510,#185511),(#185512,#185513),
(#185514,#185515),(#185516,#185517),(#185518,#185519),(#185520,#185521),
(#185522,#185523),(#185524,#185525),(#185526,#185527),(#185528,#185529),
(#185530,#185531),(#185532,#185533),(#185534,#185535),(#185536,#185537),
(#185538,#185539),(#185540,#185541),(#185542,#185543),(#185544,#185545),
(#185546,#185547),(#185548,#185549),(#185550,#185551),(#185552,#185553),
(#185554,#185555),(#185556,#185557),(#185558,#185559),(#185560,#185561),
(#185562,#185563),(#185564,#185565),(#185566,#185567),(#185568,#185569),
(#185570,#185571),(#185572,#185573),(#185574,#185575),(#185576,#185577),
(#185578,#185579),(#185580,#185581),(#185582,#185583),(#185584,#185585),
(#185586,#185587),(#185588,#185589),(#185590,#185591),(#185592,#185593),
(#185594,#185595),(#185596,#185597),(#185598,#185599),(#185600,#185601),
(#185602,#185603),(#185604,#185605),(#185606,#185607),(#185608,#185609),
(#185610,#185611),(#185612,#185613),(#185614,#185615),(#185616,#185617),
(#185618,#185619),(#185620,#185621),(#185622,#185623),(#185624,#185625),
(#185626,#185627),(#185628,#185629),(#185630,#185631),(#185632,#185633),
(#185634,#185635),(#185636,#185637)),.UNSPECIFIED.,.F.,.F.,.F.,(6,1,1,1,
1,1,1,1,1,1,1,1,1,1,1,1,1,1,1,1,1,1,1,1,1,1,1,1,1,1,1,1,1,1,1,1,1,1,1,1,
1,1,1,1,1,1,1,1,1,1,1,1,1,1,1,1,1,1,1,1,1,1,1,1,1,1,1,1,1,1,1,1,1,1,1,1,
1,1,1,1,1,1,1,1,1,1,1,1,1,1,1,1,1,1,1,1,1,1,1,1,1,1,1,1,1,1,1,1,1,1,1,1,
1,1,1,1,1,1,1,1,1,1,1,1,1,1,1,1,1,1,1,1,1,1,1,1,1,1,1,1,1,1,1,1,1,1,1,1,
1,1,1,1,1,1,1,1,1,1,1,1,1,1,1,1,1,1,1,1,1,1,1,1,1,1,1,1,1,1,1,1,1,1,1,1,
1,1,1,1,1,1,1,1,1,1,1,1,1,1,1,1,1,1,1,1,1,1,1,1,1,1,1,1,1,1,1,1,1,1,1,1,
1,1,1,1,1,1,1,1,1,1,1,1,1,1,1,1,1,1,1,1,1,1,1,1,1,1,1,1,1,1,1,1,1,1,1,1,
1,1,1,1,1,1,1,1,1,1,1,1,1,1,1,1,1,1,1,1,1,1,1,1,1,1,1,1,1,1,1,1,1,1,1,1,
1,1,1,1,1,1,1,1,1,1,1,1,1,1,1,1,1,1,1,1,1,1,1,1,1,1,1,1,1,1,1,1,1,1,1,1,
1,1,1,1,1,1,1,1,1,1,1,1,1,1,1,1,1,1,1,1,1,1,1,1,1,1,1,1,1,1,1,1,1,1,1,1,
1,1,1,1,1,1,1,1,1,1,1,1,1,1,1,1,1,1,1,1,1,1,1,1,1,1,1,1,1,1,1,1,1,1,1,1,
1,1,1,1,1,1,1,1,1,1,1,1,1,1,1,1,1,1,1,1,1,1,1,1,1,1,1,1,1,1,1,1,1,1,1,1,
1,1,1,1,1,1,1,1,1,1,1,1,1,1,1,1,1,1,1,1,1,1,1,1,1,1,1,1,1,1,1,6),(2,2),
(-1.,-0.998165138,-0.996330275,-0.994495413,-0.99266055,-0.990825688,-0.988990826,
-0.987155963,-0.985321101,-0.983486239,-0.981651376,-0.979816514,-0.977981651,
-0.976146789,-0.974311927,-0.972477064,-0.970642202,-0.968807339,-0.966972477,
-0.965137615,-0.963302752,-0.96146789,-0.959633028,-0.957798165,-0.955963303,
-0.95412844,-0.952293578,-0.950458716,-0.948623853,-0.946788991,-0.944954128,
-0.943119266,-0.941284404,-0.939449541,-0.937614679,-0.935779817,-0.933944954,
-0.932110092,-0.930275229,-0.928440367,-0.926605505,-0.924770642,-0.92293578,
-0.921100917,-0.919266055,-0.917431193,-0.91559633,-0.913761468,-0.911926606,
-0.910091743,-0.908256881,-0.906422018,-0.904587156,-0.902752294,-0.900917431,
-0.899082569,-0.897247706,-0.895412844,-0.893577982,-0.891743119,-0.889908257,
-0.888073394,-0.886238532,-0.88440367,-0.882568807,-0.880733945,-0.878899083,
-0.87706422,-0.875229358,-0.873394495,-0.871559633,-0.869724771,-0.867889908,
-0.866055046,-0.864220183,-0.862385321,-0.860550459,-0.858715596,-0.856880734,
-0.855045872,-0.853211009,-0.851376147,-0.849541284,-0.847706422,-0.84587156,
-0.844036697,-0.842201835,-0.840366972,-0.83853211,-0.836697248,-0.834862385,
-0.833027523,-0.831192661,-0.829357798,-0.827522936,-0.825688073,-0.823853211,
-0.822018349,-0.820183486,-0.818348624,-0.816513761,-0.814678899,-0.812844037,
-0.811009174,-0.809174312,-0.80733945,-0.805504587,-0.803669725,-0.801834862,
-0.8,-0.798165138,-0.796330275,-0.794495413,-0.79266055,-0.790825688,-0.788990826,
-0.787155963,-0.785321101,-0.783486239,-0.781651376,-0.779816514,-0.777981651,
-0.776146789,-0.774311927,-0.772477064,-0.770642202,-0.768807339,-0.766972477,
-0.765137615,-0.763302752,-0.76146789,-0.759633028,-0.757798165,-0.755963303,
-0.75412844,-0.752293578,-0.750458716,-0.748623853,-0.746788991,-0.744954128,
-0.743119266,-0.741284404,-0.739449541,-0.737614679,-0.735779817,-0.733944954,
-0.732110092,-0.730275229,-0.728440367,-0.726605505,-0.724770642,-0.72293578,
-0.721100917,-0.719266055,-0.717431193,-0.71559633,-0.713761468,-0.711926606,
-0.710091743,-0.708256881,-0.706422018,-0.704587156,-0.702752294,-0.700917431,
-0.699082569,-0.697247706,-0.695412844,-0.693577982,-0.691743119,-0.689908257,
-0.688073394,-0.686238532,-0.68440367,-0.682568807,-0.680733945,-0.678899083,
-0.67706422,-0.675229358,-0.673394495,-0.671559633,-0.669724771,-0.667889908,
-0.666055046,-0.664220183,-0.662385321,-0.660550459,-0.658715596,-0.656880734,
-0.655045872,-0.653211009,-0.651376147,-0.649541284,-0.647706422,-0.64587156,
-0.644036697,-0.642201835,-0.640366972,-0.63853211,-0.636697248,-0.634862385,
-0.633027523,-0.631192661,-0.629357798,-0.627522936,-0.625688073,-0.623853211,
-0.622018349,-0.620183486,-0.618348624,-0.616513761,-0.614678899,-0.612844037,
-0.611009174,-0.609174312,-0.60733945,-0.605504587,-0.603669725,-0.601834862,
-0.6,-0.598165138,-0.596330275,-0.594495413,-0.59266055,-0.590825688,-0.588990826,
-0.587155963,-0.585321101,-0.583486239,-0.581651376,-0.579816514,-0.577981651,
-0.576146789,-0.574311927,-0.572477064,-0.570642202,-0.568807339,-0.566972477,
-0.565137615,-0.563302752,-0.56146789,-0.559633028,-0.557798165,-0.555963303,
-0.55412844,-0.552293578,-0.550458716,-0.548623853,-0.546788991,-0.544954128,
-0.543119266,-0.541284404,-0.539449541,-0.537614679,-0.535779817,-0.533944954,
-0.532110092,-0.530275229,-0.528440367,-0.526605505,-0.524770642,-0.52293578,
-0.521100917,-0.519266055,-0.517431193,-0.51559633,-0.513761468,-0.511926606,
-0.510091743,-0.508256881,-0.506422018,-0.504587156,-0.502752294,-0.500917431,
-0.499082569,-0.497247706,-0.495412844,-0.493577982,-0.491743119,-0.489908257,
-0.488073394,-0.486238532,-0.48440367,-0.482568807,-0.480733945,-0.478899083,
-0.47706422,-0.475229358,-0.473394495,-0.471559633,-0.469724771,-0.467889908,
-0.466055046,-0.464220183,-0.462385321,-0.460550459,-0.458715596,-0.456880734,
-0.455045872,-0.453211009,-0.451376147,-0.449541284,-0.447706422,-0.44587156,
-0.444036697,-0.442201835,-0.440366972,-0.43853211,-0.436697248,-0.434862385,
-0.433027523,-0.431192661,-0.429357798,-0.427522936,-0.425688073,-0.423853211,
-0.422018349,-0.420183486,-0.418348624,-0.416513761,-0.414678899,-0.412844037,
-0.411009174,-0.409174312,-0.40733945,-0.405504587,-0.403669725,-0.401834862,
-0.4,-0.398165138,-0.396330275,-0.394495413,-0.39266055,-0.390825688,-0.388990826,
-0.387155963,-0.385321101,-0.383486239,-0.381651376,-0.379816514,-0.377981651,
-0.376146789,-0.374311927,-0.372477064,-0.370642202,-0.368807339,-0.366972477,
-0.365137615,-0.363302752,-0.36146789,-0.359633028,-0.357798165,-0.355963303,
-0.35412844,-0.352293578,-0.350458716,-0.348623853,-0.346788991,-0.344954128,
-0.343119266,-0.341284404,-0.339449541,-0.337614679,-0.335779817,-0.333944954,
-0.332110092,-0.330275229,-0.328440367,-0.326605505,-0.324770642,-0.32293578,
-0.321100917,-0.319266055,-0.317431193,-0.31559633,-0.313761468,-0.311926606,
-0.310091743,-0.308256881,-0.306422018,-0.304587156,-0.302752294,-0.300917431,
-0.299082569,-0.297247706,-0.295412844,-0.293577982,-0.291743119,-0.289908257,
-0.288073394,-0.286238532,-0.28440367,-0.282568807,-0.280733945,-0.278899083,
-0.27706422,-0.275229358,-0.273394495,-0.271559633,-0.269724771,-0.267889908,
-0.266055046,-0.264220183,-0.262385321,-0.260550459,-0.258715596,-0.256880734,
-0.255045872,-0.253211009,-0.251376147,-0.249541284,-0.247706422,-0.24587156,
-0.244036697,-0.242201835,-0.240366972,-0.23853211,-0.236697248,-0.234862385,
-0.233027523,-0.231192661,-0.229357798,-0.227522936,-0.225688073,-0.223853211,
-0.222018349,-0.220183486,-0.218348624,-0.216513761,-0.214678899,-0.212844037,
-0.211009174,-0.209174312,-0.20733945,-0.205504587,-0.203669725,-0.201834862,
-0.2,-0.198165138,-0.196330275,-0.194495413,-0.19266055,-0.190825688,-0.188990826,
-0.187155963,-0.185321101,-0.183486239,-0.181651376,-0.179816514,-0.177981651,
-0.176146789,-0.174311927,-0.172477064,-0.170642202,-0.168807339,-0.166972477,
-0.165137615,-0.163302752,-0.16146789,-0.159633028,-0.157798165,-0.155963303,
-0.15412844,-0.152293578,-0.150458716,-0.148623853,-0.146788991,-0.144954128,
-0.143172103),(0.,0.36),.UNSPECIFIED.);
#6234=B_SPLINE_SURFACE_WITH_KNOTS('',5,1,((#186279,#186280),(#186281,#186282),
(#186283,#186284),(#186285,#186286),(#186287,#186288),(#186289,#186290),
(#186291,#186292),(#186293,#186294),(#186295,#186296),(#186297,#186298),
(#186299,#186300),(#186301,#186302),(#186303,#186304),(#186305,#186306),
(#186307,#186308),(#186309,#186310),(#186311,#186312),(#186313,#186314),
(#186315,#186316),(#186317,#186318),(#186319,#186320),(#186321,#186322),
(#186323,#186324),(#186325,#186326),(#186327,#186328),(#186329,#186330),
(#186331,#186332),(#186333,#186334),(#186335,#186336),(#186337,#186338),
(#186339,#186340),(#186341,#186342),(#186343,#186344),(#186345,#186346),
(#186347,#186348),(#186349,#186350),(#186351,#186352),(#186353,#186354),
(#186355,#186356),(#186357,#186358),(#186359,#186360),(#186361,#186362),
(#186363,#186364),(#186365,#186366),(#186367,#186368),(#186369,#186370),
(#186371,#186372),(#186373,#186374),(#186375,#186376),(#186377,#186378),
(#186379,#186380),(#186381,#186382),(#186383,#186384),(#186385,#186386),
(#186387,#186388),(#186389,#186390),(#186391,#186392),(#186393,#186394),
(#186395,#186396),(#186397,#186398),(#186399,#186400),(#186401,#186402),
(#186403,#186404),(#186405,#186406),(#186407,#186408),(#186409,#186410),
(#186411,#186412),(#186413,#186414),(#186415,#186416),(#186417,#186418),
(#186419,#186420),(#186421,#186422),(#186423,#186424),(#186425,#186426),
(#186427,#186428),(#186429,#186430),(#186431,#186432),(#186433,#186434),
(#186435,#186436),(#186437,#186438),(#186439,#186440),(#186441,#186442),
(#186443,#186444),(#186445,#186446),(#186447,#186448),(#186449,#186450),
(#186451,#186452),(#186453,#186454),(#186455,#186456),(#186457,#186458),
(#186459,#186460),(#186461,#186462),(#186463,#186464),(#186465,#186466),
(#186467,#186468),(#186469,#186470),(#186471,#186472),(#186473,#186474),
(#186475,#186476),(#186477,#186478),(#186479,#186480),(#186481,#186482),
(#186483,#186484),(#186485,#186486),(#186487,#186488),(#186489,#186490),
(#186491,#186492),(#186493,#186494),(#186495,#186496),(#186497,#186498),
(#186499,#186500),(#186501,#186502),(#186503,#186504),(#186505,#186506),
(#186507,#186508),(#186509,#186510),(#186511,#186512),(#186513,#186514),
(#186515,#186516),(#186517,#186518),(#186519,#186520),(#186521,#186522),
(#186523,#186524),(#186525,#186526),(#186527,#186528),(#186529,#186530),
(#186531,#186532),(#186533,#186534),(#186535,#186536),(#186537,#186538),
(#186539,#186540),(#186541,#186542),(#186543,#186544),(#186545,#186546),
(#186547,#186548),(#186549,#186550),(#186551,#186552),(#186553,#186554),
(#186555,#186556),(#186557,#186558),(#186559,#186560),(#186561,#186562),
(#186563,#186564),(#186565,#186566),(#186567,#186568),(#186569,#186570),
(#186571,#186572),(#186573,#186574),(#186575,#186576),(#186577,#186578),
(#186579,#186580),(#186581,#186582),(#186583,#186584),(#186585,#186586),
(#186587,#186588),(#186589,#186590),(#186591,#186592),(#186593,#186594),
(#186595,#186596),(#186597,#186598),(#186599,#186600),(#186601,#186602),
(#186603,#186604),(#186605,#186606),(#186607,#186608),(#186609,#186610),
(#186611,#186612),(#186613,#186614),(#186615,#186616),(#186617,#186618),
(#186619,#186620),(#186621,#186622),(#186623,#186624),(#186625,#186626),
(#186627,#186628),(#186629,#186630),(#186631,#186632),(#186633,#186634),
(#186635,#186636),(#186637,#186638),(#186639,#186640),(#186641,#186642),
(#186643,#186644),(#186645,#186646),(#186647,#186648),(#186649,#186650),
(#186651,#186652),(#186653,#186654),(#186655,#186656),(#186657,#186658),
(#186659,#186660),(#186661,#186662),(#186663,#186664),(#186665,#186666),
(#186667,#186668),(#186669,#186670),(#186671,#186672),(#186673,#186674),
(#186675,#186676),(#186677,#186678),(#186679,#186680),(#186681,#186682),
(#186683,#186684),(#186685,#186686),(#186687,#186688),(#186689,#186690),
(#186691,#186692),(#186693,#186694),(#186695,#186696),(#186697,#186698),
(#186699,#186700),(#186701,#186702),(#186703,#186704),(#186705,#186706),
(#186707,#186708),(#186709,#186710),(#186711,#186712),(#186713,#186714),
(#186715,#186716),(#186717,#186718),(#186719,#186720),(#186721,#186722),
(#186723,#186724),(#186725,#186726),(#186727,#186728),(#186729,#186730),
(#186731,#186732),(#186733,#186734),(#186735,#186736),(#186737,#186738),
(#186739,#186740),(#186741,#186742),(#186743,#186744),(#186745,#186746),
(#186747,#186748),(#186749,#186750),(#186751,#186752),(#186753,#186754),
(#186755,#186756),(#186757,#186758),(#186759,#186760),(#186761,#186762),
(#186763,#186764),(#186765,#186766),(#186767,#186768),(#186769,#186770),
(#186771,#186772),(#186773,#186774),(#186775,#186776),(#186777,#186778),
(#186779,#186780),(#186781,#186782),(#186783,#186784),(#186785,#186786),
(#186787,#186788),(#186789,#186790),(#186791,#186792),(#186793,#186794),
(#186795,#186796),(#186797,#186798),(#186799,#186800),(#186801,#186802),
(#186803,#186804),(#186805,#186806),(#186807,#186808),(#186809,#186810),
(#186811,#186812),(#186813,#186814),(#186815,#186816),(#186817,#186818),
(#186819,#186820),(#186821,#186822),(#186823,#186824),(#186825,#186826),
(#186827,#186828),(#186829,#186830),(#186831,#186832),(#186833,#186834),
(#186835,#186836),(#186837,#186838),(#186839,#186840),(#186841,#186842),
(#186843,#186844),(#186845,#186846),(#186847,#186848),(#186849,#186850),
(#186851,#186852),(#186853,#186854),(#186855,#186856),(#186857,#186858),
(#186859,#186860),(#186861,#186862),(#186863,#186864),(#186865,#186866),
(#186867,#186868),(#186869,#186870),(#186871,#186872),(#186873,#186874),
(#186875,#186876),(#186877,#186878),(#186879,#186880),(#186881,#186882),
(#186883,#186884),(#186885,#186886),(#186887,#186888),(#186889,#186890),
(#186891,#186892),(#186893,#186894),(#186895,#186896),(#186897,#186898),
(#186899,#186900),(#186901,#186902),(#186903,#186904),(#186905,#186906),
(#186907,#186908),(#186909,#186910),(#186911,#186912),(#186913,#186914),
(#186915,#186916),(#186917,#186918),(#186919,#186920),(#186921,#186922),
(#186923,#186924),(#186925,#186926),(#186927,#186928),(#186929,#186930),
(#186931,#186932),(#186933,#186934),(#186935,#186936),(#186937,#186938),
(#186939,#186940),(#186941,#186942),(#186943,#186944),(#186945,#186946),
(#186947,#186948),(#186949,#186950),(#186951,#186952),(#186953,#186954),
(#186955,#186956),(#186957,#186958),(#186959,#186960),(#186961,#186962),
(#186963,#186964),(#186965,#186966),(#186967,#186968),(#186969,#186970),
(#186971,#186972),(#186973,#186974),(#186975,#186976),(#186977,#186978),
(#186979,#186980),(#186981,#186982),(#186983,#186984),(#186985,#186986),
(#186987,#186988),(#186989,#186990),(#186991,#186992),(#186993,#186994),
(#186995,#186996),(#186997,#186998),(#186999,#187000),(#187001,#187002),
(#187003,#187004),(#187005,#187006),(#187007,#187008),(#187009,#187010),
(#187011,#187012),(#187013,#187014),(#187015,#187016),(#187017,#187018),
(#187019,#187020),(#187021,#187022),(#187023,#187024),(#187025,#187026),
(#187027,#187028),(#187029,#187030),(#187031,#187032),(#187033,#187034),
(#187035,#187036),(#187037,#187038),(#187039,#187040),(#187041,#187042),
(#187043,#187044),(#187045,#187046),(#187047,#187048),(#187049,#187050),
(#187051,#187052),(#187053,#187054),(#187055,#187056),(#187057,#187058),
(#187059,#187060),(#187061,#187062),(#187063,#187064),(#187065,#187066),
(#187067,#187068),(#187069,#187070),(#187071,#187072),(#187073,#187074),
(#187075,#187076),(#187077,#187078),(#187079,#187080),(#187081,#187082),
(#187083,#187084),(#187085,#187086),(#187087,#187088),(#187089,#187090),
(#187091,#187092),(#187093,#187094),(#187095,#187096),(#187097,#187098),
(#187099,#187100),(#187101,#187102),(#187103,#187104),(#187105,#187106),
(#187107,#187108),(#187109,#187110),(#187111,#187112),(#187113,#187114),
(#187115,#187116),(#187117,#187118),(#187119,#187120),(#187121,#187122),
(#187123,#187124),(#187125,#187126),(#187127,#187128),(#187129,#187130),
(#187131,#187132),(#187133,#187134),(#187135,#187136),(#187137,#187138),
(#187139,#187140),(#187141,#187142),(#187143,#187144),(#187145,#187146),
(#187147,#187148),(#187149,#187150),(#187151,#187152),(#187153,#187154),
(#187155,#187156),(#187157,#187158),(#187159,#187160),(#187161,#187162),
(#187163,#187164),(#187165,#187166),(#187167,#187168),(#187169,#187170),
(#187171,#187172),(#187173,#187174),(#187175,#187176),(#187177,#187178),
(#187179,#187180),(#187181,#187182),(#187183,#187184),(#187185,#187186),
(#187187,#187188),(#187189,#187190),(#187191,#187192),(#187193,#187194),
(#187195,#187196),(#187197,#187198),(#187199,#187200),(#187201,#187202),
(#187203,#187204),(#187205,#187206),(#187207,#187208),(#187209,#187210),
(#187211,#187212),(#187213,#187214),(#187215,#187216),(#187217,#187218),
(#187219,#187220),(#187221,#187222)),.UNSPECIFIED.,.F.,.F.,.F.,(6,1,1,1,
1,1,1,1,1,1,1,1,1,1,1,1,1,1,1,1,1,1,1,1,1,1,1,1,1,1,1,1,1,1,1,1,1,1,1,1,
1,1,1,1,1,1,1,1,1,1,1,1,1,1,1,1,1,1,1,1,1,1,1,1,1,1,1,1,1,1,1,1,1,1,1,1,
1,1,1,1,1,1,1,1,1,1,1,1,1,1,1,1,1,1,1,1,1,1,1,1,1,1,1,1,1,1,1,1,1,1,1,1,
1,1,1,1,1,1,1,1,1,1,1,1,1,1,1,1,1,1,1,1,1,1,1,1,1,1,1,1,1,1,1,1,1,1,1,1,
1,1,1,1,1,1,1,1,1,1,1,1,1,1,1,1,1,1,1,1,1,1,1,1,1,1,1,1,1,1,1,1,1,1,1,1,
1,1,1,1,1,1,1,1,1,1,1,1,1,1,1,1,1,1,1,1,1,1,1,1,1,1,1,1,1,1,1,1,1,1,1,1,
1,1,1,1,1,1,1,1,1,1,1,1,1,1,1,1,1,1,1,1,1,1,1,1,1,1,1,1,1,1,1,1,1,1,1,1,
1,1,1,1,1,1,1,1,1,1,1,1,1,1,1,1,1,1,1,1,1,1,1,1,1,1,1,1,1,1,1,1,1,1,1,1,
1,1,1,1,1,1,1,1,1,1,1,1,1,1,1,1,1,1,1,1,1,1,1,1,1,1,1,1,1,1,1,1,1,1,1,1,
1,1,1,1,1,1,1,1,1,1,1,1,1,1,1,1,1,1,1,1,1,1,1,1,1,1,1,1,1,1,1,1,1,1,1,1,
1,1,1,1,1,1,1,1,1,1,1,1,1,1,1,1,1,1,1,1,1,1,1,1,1,1,1,1,1,1,1,1,1,1,1,1,
1,1,1,1,1,1,1,1,1,1,1,1,1,1,1,1,1,1,1,1,1,1,1,1,1,1,1,1,1,1,1,1,1,1,1,1,
1,1,1,1,1,1,1,1,1,1,1,1,1,1,1,1,1,1,1,1,1,1,1,1,1,1,1,1,1,1,1,6),(2,2),
(0.143172103,0.144954128,0.146788991,0.148623853,0.150458716,0.152293578,
0.15412844,0.155963303,0.157798165,0.159633028,0.16146789,0.163302752,0.165137615,
0.166972477,0.168807339,0.170642202,0.172477064,0.174311927,0.176146789,
0.177981651,0.179816514,0.181651376,0.183486239,0.185321101,0.187155963,
0.188990826,0.190825688,0.19266055,0.194495413,0.196330275,0.198165138,
0.2,0.201834862,0.203669725,0.205504587,0.20733945,0.209174312,0.211009174,
0.212844037,0.214678899,0.216513761,0.218348624,0.220183486,0.222018349,
0.223853211,0.225688073,0.227522936,0.229357798,0.231192661,0.233027523,
0.234862385,0.236697248,0.23853211,0.240366972,0.242201835,0.244036697,
0.24587156,0.247706422,0.249541284,0.251376147,0.253211009,0.255045872,
0.256880734,0.258715596,0.260550459,0.262385321,0.264220183,0.266055046,
0.267889908,0.269724771,0.271559633,0.273394495,0.275229358,0.27706422,
0.278899083,0.280733945,0.282568807,0.28440367,0.286238532,0.288073394,
0.289908257,0.291743119,0.293577982,0.295412844,0.297247706,0.299082569,
0.300917431,0.302752294,0.304587156,0.306422018,0.308256881,0.310091743,
0.311926606,0.313761468,0.31559633,0.317431193,0.319266055,0.321100917,
0.32293578,0.324770642,0.326605505,0.328440367,0.330275229,0.332110092,
0.333944954,0.335779817,0.337614679,0.339449541,0.341284404,0.343119266,
0.344954128,0.346788991,0.348623853,0.350458716,0.352293578,0.35412844,
0.355963303,0.357798165,0.359633028,0.36146789,0.363302752,0.365137615,
0.366972477,0.368807339,0.370642202,0.372477064,0.374311927,0.376146789,
0.377981651,0.379816514,0.381651376,0.383486239,0.385321101,0.387155963,
0.388990826,0.390825688,0.39266055,0.394495413,0.396330275,0.398165138,
0.4,0.401834862,0.403669725,0.405504587,0.40733945,0.409174312,0.411009174,
0.412844037,0.414678899,0.416513761,0.418348624,0.420183486,0.422018349,
0.423853211,0.425688073,0.427522936,0.429357798,0.431192661,0.433027523,
0.434862385,0.436697248,0.43853211,0.440366972,0.442201835,0.444036697,
0.44587156,0.447706422,0.449541284,0.451376147,0.453211009,0.455045872,
0.456880734,0.458715596,0.460550459,0.462385321,0.464220183,0.466055046,
0.467889908,0.469724771,0.471559633,0.473394495,0.475229358,0.47706422,
0.478899083,0.480733945,0.482568807,0.48440367,0.486238532,0.488073394,
0.489908257,0.491743119,0.493577982,0.495412844,0.497247706,0.499082569,
0.500917431,0.502752294,0.504587156,0.506422018,0.508256881,0.510091743,
0.511926606,0.513761468,0.51559633,0.517431193,0.519266055,0.521100917,
0.52293578,0.524770642,0.526605505,0.528440367,0.530275229,0.532110092,
0.533944954,0.535779817,0.537614679,0.539449541,0.541284404,0.543119266,
0.544954128,0.546788991,0.548623853,0.550458716,0.552293578,0.55412844,
0.555963303,0.557798165,0.559633028,0.56146789,0.563302752,0.565137615,
0.566972477,0.568807339,0.570642202,0.572477064,0.574311927,0.576146789,
0.577981651,0.579816514,0.581651376,0.583486239,0.585321101,0.587155963,
0.588990826,0.590825688,0.59266055,0.594495413,0.596330275,0.598165138,
0.6,0.601834862,0.603669725,0.605504587,0.60733945,0.609174312,0.611009174,
0.612844037,0.614678899,0.616513761,0.618348624,0.620183486,0.622018349,
0.623853211,0.625688073,0.627522936,0.629357798,0.631192661,0.633027523,
0.634862385,0.636697248,0.63853211,0.640366972,0.642201835,0.644036697,
0.64587156,0.647706422,0.649541284,0.651376147,0.653211009,0.655045872,
0.656880734,0.658715596,0.660550459,0.662385321,0.664220183,0.666055046,
0.667889908,0.669724771,0.671559633,0.673394495,0.675229358,0.67706422,
0.678899083,0.680733945,0.682568807,0.68440367,0.686238532,0.688073394,
0.689908257,0.691743119,0.693577982,0.695412844,0.697247706,0.699082569,
0.700917431,0.702752294,0.704587156,0.706422018,0.708256881,0.710091743,
0.711926606,0.713761468,0.71559633,0.717431193,0.719266055,0.721100917,
0.72293578,0.724770642,0.726605505,0.728440367,0.730275229,0.732110092,
0.733944954,0.735779817,0.737614679,0.739449541,0.741284404,0.743119266,
0.744954128,0.746788991,0.748623853,0.750458716,0.752293578,0.75412844,
0.755963303,0.757798165,0.759633028,0.76146789,0.763302752,0.765137615,
0.766972477,0.768807339,0.770642202,0.772477064,0.774311927,0.776146789,
0.777981651,0.779816514,0.781651376,0.783486239,0.785321101,0.787155963,
0.788990826,0.790825688,0.79266055,0.794495413,0.796330275,0.798165138,
0.8,0.801834862,0.803669725,0.805504587,0.80733945,0.809174312,0.811009174,
0.812844037,0.814678899,0.816513761,0.818348624,0.820183486,0.822018349,
0.823853211,0.825688073,0.827522936,0.829357798,0.831192661,0.833027523,
0.834862385,0.836697248,0.83853211,0.840366972,0.842201835,0.844036697,
0.84587156,0.847706422,0.849541284,0.851376147,0.853211009,0.855045872,
0.856880734,0.858715596,0.860550459,0.862385321,0.864220183,0.866055046,
0.867889908,0.869724771,0.871559633,0.873394495,0.875229358,0.87706422,
0.878899083,0.880733945,0.882568807,0.88440367,0.886238532,0.888073394,
0.889908257,0.891743119,0.893577982,0.895412844,0.897247706,0.899082569,
0.900917431,0.902752294,0.904587156,0.906422018,0.908256881,0.910091743,
0.911926606,0.913761468,0.91559633,0.917431193,0.919266055,0.921100917,
0.92293578,0.924770642,0.926605505,0.928440367,0.930275229,0.932110092,
0.933944954,0.935779817,0.937614679,0.939449541,0.941284404,0.943119266,
0.944954128,0.946788991,0.948623853,0.950458716,0.952293578,0.95412844,
0.955963303,0.957798165,0.959633028,0.96146789,0.963302752,0.965137615,
0.966972477,0.968807339,0.970642202,0.972477064,0.974311927,0.976146789,
0.977981651,0.979816514,0.981651376,0.983486239,0.985321101,0.987155963,
0.988990826,0.990825688,0.99266055,0.994495413,0.996330275,0.998165138,
1.),(0.,0.36),.UNSPECIFIED.);
#6235=B_SPLINE_SURFACE_WITH_KNOTS('',5,1,((#187882,#187883),(#187884,#187885),
(#187886,#187887),(#187888,#187889),(#187890,#187891),(#187892,#187893),
(#187894,#187895),(#187896,#187897),(#187898,#187899),(#187900,#187901),
(#187902,#187903),(#187904,#187905),(#187906,#187907),(#187908,#187909),
(#187910,#187911),(#187912,#187913),(#187914,#187915),(#187916,#187917),
(#187918,#187919),(#187920,#187921),(#187922,#187923),(#187924,#187925),
(#187926,#187927),(#187928,#187929),(#187930,#187931),(#187932,#187933),
(#187934,#187935),(#187936,#187937),(#187938,#187939),(#187940,#187941),
(#187942,#187943),(#187944,#187945),(#187946,#187947),(#187948,#187949),
(#187950,#187951),(#187952,#187953),(#187954,#187955),(#187956,#187957),
(#187958,#187959),(#187960,#187961),(#187962,#187963),(#187964,#187965),
(#187966,#187967),(#187968,#187969),(#187970,#187971),(#187972,#187973),
(#187974,#187975),(#187976,#187977),(#187978,#187979),(#187980,#187981),
(#187982,#187983),(#187984,#187985),(#187986,#187987),(#187988,#187989),
(#187990,#187991),(#187992,#187993),(#187994,#187995),(#187996,#187997),
(#187998,#187999),(#188000,#188001),(#188002,#188003),(#188004,#188005),
(#188006,#188007),(#188008,#188009),(#188010,#188011),(#188012,#188013),
(#188014,#188015),(#188016,#188017),(#188018,#188019),(#188020,#188021),
(#188022,#188023),(#188024,#188025),(#188026,#188027),(#188028,#188029),
(#188030,#188031),(#188032,#188033),(#188034,#188035),(#188036,#188037),
(#188038,#188039),(#188040,#188041),(#188042,#188043),(#188044,#188045),
(#188046,#188047),(#188048,#188049),(#188050,#188051),(#188052,#188053),
(#188054,#188055),(#188056,#188057),(#188058,#188059),(#188060,#188061),
(#188062,#188063),(#188064,#188065),(#188066,#188067),(#188068,#188069),
(#188070,#188071),(#188072,#188073),(#188074,#188075),(#188076,#188077),
(#188078,#188079),(#188080,#188081),(#188082,#188083),(#188084,#188085),
(#188086,#188087),(#188088,#188089),(#188090,#188091),(#188092,#188093),
(#188094,#188095),(#188096,#188097),(#188098,#188099),(#188100,#188101),
(#188102,#188103),(#188104,#188105),(#188106,#188107),(#188108,#188109),
(#188110,#188111),(#188112,#188113),(#188114,#188115),(#188116,#188117),
(#188118,#188119),(#188120,#188121),(#188122,#188123),(#188124,#188125),
(#188126,#188127),(#188128,#188129),(#188130,#188131),(#188132,#188133),
(#188134,#188135),(#188136,#188137),(#188138,#188139),(#188140,#188141),
(#188142,#188143),(#188144,#188145),(#188146,#188147),(#188148,#188149),
(#188150,#188151),(#188152,#188153),(#188154,#188155),(#188156,#188157),
(#188158,#188159),(#188160,#188161),(#188162,#188163),(#188164,#188165),
(#188166,#188167),(#188168,#188169),(#188170,#188171),(#188172,#188173),
(#188174,#188175),(#188176,#188177),(#188178,#188179),(#188180,#188181),
(#188182,#188183),(#188184,#188185),(#188186,#188187),(#188188,#188189),
(#188190,#188191),(#188192,#188193),(#188194,#188195),(#188196,#188197),
(#188198,#188199),(#188200,#188201),(#188202,#188203),(#188204,#188205),
(#188206,#188207),(#188208,#188209),(#188210,#188211),(#188212,#188213),
(#188214,#188215),(#188216,#188217),(#188218,#188219),(#188220,#188221),
(#188222,#188223),(#188224,#188225),(#188226,#188227),(#188228,#188229),
(#188230,#188231),(#188232,#188233),(#188234,#188235),(#188236,#188237),
(#188238,#188239),(#188240,#188241),(#188242,#188243),(#188244,#188245),
(#188246,#188247),(#188248,#188249),(#188250,#188251),(#188252,#188253),
(#188254,#188255),(#188256,#188257),(#188258,#188259),(#188260,#188261),
(#188262,#188263),(#188264,#188265),(#188266,#188267),(#188268,#188269),
(#188270,#188271),(#188272,#188273),(#188274,#188275),(#188276,#188277),
(#188278,#188279),(#188280,#188281),(#188282,#188283),(#188284,#188285),
(#188286,#188287),(#188288,#188289),(#188290,#188291),(#188292,#188293),
(#188294,#188295),(#188296,#188297),(#188298,#188299),(#188300,#188301),
(#188302,#188303),(#188304,#188305),(#188306,#188307),(#188308,#188309),
(#188310,#188311),(#188312,#188313),(#188314,#188315),(#188316,#188317),
(#188318,#188319),(#188320,#188321),(#188322,#188323),(#188324,#188325),
(#188326,#188327),(#188328,#188329),(#188330,#188331),(#188332,#188333),
(#188334,#188335),(#188336,#188337),(#188338,#188339),(#188340,#188341),
(#188342,#188343),(#188344,#188345),(#188346,#188347),(#188348,#188349),
(#188350,#188351),(#188352,#188353),(#188354,#188355),(#188356,#188357),
(#188358,#188359),(#188360,#188361),(#188362,#188363),(#188364,#188365),
(#188366,#188367),(#188368,#188369),(#188370,#188371),(#188372,#188373),
(#188374,#188375),(#188376,#188377),(#188378,#188379),(#188380,#188381),
(#188382,#188383),(#188384,#188385),(#188386,#188387),(#188388,#188389),
(#188390,#188391),(#188392,#188393),(#188394,#188395),(#188396,#188397),
(#188398,#188399),(#188400,#188401),(#188402,#188403),(#188404,#188405),
(#188406,#188407),(#188408,#188409),(#188410,#188411),(#188412,#188413),
(#188414,#188415),(#188416,#188417),(#188418,#188419),(#188420,#188421),
(#188422,#188423),(#188424,#188425),(#188426,#188427),(#188428,#188429),
(#188430,#188431),(#188432,#188433),(#188434,#188435),(#188436,#188437),
(#188438,#188439),(#188440,#188441),(#188442,#188443),(#188444,#188445),
(#188446,#188447),(#188448,#188449),(#188450,#188451),(#188452,#188453),
(#188454,#188455),(#188456,#188457),(#188458,#188459),(#188460,#188461),
(#188462,#188463),(#188464,#188465),(#188466,#188467),(#188468,#188469),
(#188470,#188471),(#188472,#188473),(#188474,#188475),(#188476,#188477),
(#188478,#188479),(#188480,#188481),(#188482,#188483),(#188484,#188485),
(#188486,#188487),(#188488,#188489),(#188490,#188491),(#188492,#188493),
(#188494,#188495),(#188496,#188497),(#188498,#188499),(#188500,#188501),
(#188502,#188503),(#188504,#188505),(#188506,#188507),(#188508,#188509),
(#188510,#188511),(#188512,#188513),(#188514,#188515),(#188516,#188517),
(#188518,#188519),(#188520,#188521),(#188522,#188523),(#188524,#188525),
(#188526,#188527),(#188528,#188529),(#188530,#188531),(#188532,#188533),
(#188534,#188535),(#188536,#188537),(#188538,#188539),(#188540,#188541),
(#188542,#188543),(#188544,#188545),(#188546,#188547),(#188548,#188549),
(#188550,#188551),(#188552,#188553),(#188554,#188555),(#188556,#188557),
(#188558,#188559),(#188560,#188561),(#188562,#188563),(#188564,#188565),
(#188566,#188567),(#188568,#188569),(#188570,#188571),(#188572,#188573),
(#188574,#188575),(#188576,#188577),(#188578,#188579),(#188580,#188581),
(#188582,#188583),(#188584,#188585),(#188586,#188587),(#188588,#188589),
(#188590,#188591),(#188592,#188593),(#188594,#188595),(#188596,#188597),
(#188598,#188599),(#188600,#188601),(#188602,#188603),(#188604,#188605),
(#188606,#188607),(#188608,#188609),(#188610,#188611),(#188612,#188613),
(#188614,#188615),(#188616,#188617),(#188618,#188619),(#188620,#188621),
(#188622,#188623),(#188624,#188625),(#188626,#188627),(#188628,#188629),
(#188630,#188631),(#188632,#188633),(#188634,#188635),(#188636,#188637),
(#188638,#188639),(#188640,#188641),(#188642,#188643),(#188644,#188645),
(#188646,#188647),(#188648,#188649),(#188650,#188651),(#188652,#188653),
(#188654,#188655),(#188656,#188657),(#188658,#188659),(#188660,#188661),
(#188662,#188663),(#188664,#188665),(#188666,#188667),(#188668,#188669),
(#188670,#188671),(#188672,#188673),(#188674,#188675),(#188676,#188677),
(#188678,#188679),(#188680,#188681),(#188682,#188683),(#188684,#188685),
(#188686,#188687),(#188688,#188689),(#188690,#188691),(#188692,#188693),
(#188694,#188695),(#188696,#188697),(#188698,#188699),(#188700,#188701),
(#188702,#188703),(#188704,#188705),(#188706,#188707),(#188708,#188709),
(#188710,#188711),(#188712,#188713),(#188714,#188715),(#188716,#188717),
(#188718,#188719),(#188720,#188721),(#188722,#188723),(#188724,#188725),
(#188726,#188727),(#188728,#188729),(#188730,#188731),(#188732,#188733),
(#188734,#188735),(#188736,#188737),(#188738,#188739),(#188740,#188741),
(#188742,#188743),(#188744,#188745),(#188746,#188747),(#188748,#188749),
(#188750,#188751),(#188752,#188753),(#188754,#188755),(#188756,#188757),
(#188758,#188759),(#188760,#188761),(#188762,#188763),(#188764,#188765),
(#188766,#188767),(#188768,#188769),(#188770,#188771),(#188772,#188773),
(#188774,#188775),(#188776,#188777),(#188778,#188779),(#188780,#188781),
(#188782,#188783),(#188784,#188785),(#188786,#188787),(#188788,#188789),
(#188790,#188791),(#188792,#188793),(#188794,#188795),(#188796,#188797),
(#188798,#188799),(#188800,#188801),(#188802,#188803),(#188804,#188805),
(#188806,#188807),(#188808,#188809),(#188810,#188811),(#188812,#188813),
(#188814,#188815),(#188816,#188817),(#188818,#188819),(#188820,#188821),
(#188822,#188823),(#188824,#188825)),.UNSPECIFIED.,.F.,.F.,.F.,(6,1,1,1,
1,1,1,1,1,1,1,1,1,1,1,1,1,1,1,1,1,1,1,1,1,1,1,1,1,1,1,1,1,1,1,1,1,1,1,1,
1,1,1,1,1,1,1,1,1,1,1,1,1,1,1,1,1,1,1,1,1,1,1,1,1,1,1,1,1,1,1,1,1,1,1,1,
1,1,1,1,1,1,1,1,1,1,1,1,1,1,1,1,1,1,1,1,1,1,1,1,1,1,1,1,1,1,1,1,1,1,1,1,
1,1,1,1,1,1,1,1,1,1,1,1,1,1,1,1,1,1,1,1,1,1,1,1,1,1,1,1,1,1,1,1,1,1,1,1,
1,1,1,1,1,1,1,1,1,1,1,1,1,1,1,1,1,1,1,1,1,1,1,1,1,1,1,1,1,1,1,1,1,1,1,1,
1,1,1,1,1,1,1,1,1,1,1,1,1,1,1,1,1,1,1,1,1,1,1,1,1,1,1,1,1,1,1,1,1,1,1,1,
1,1,1,1,1,1,1,1,1,1,1,1,1,1,1,1,1,1,1,1,1,1,1,1,1,1,1,1,1,1,1,1,1,1,1,1,
1,1,1,1,1,1,1,1,1,1,1,1,1,1,1,1,1,1,1,1,1,1,1,1,1,1,1,1,1,1,1,1,1,1,1,1,
1,1,1,1,1,1,1,1,1,1,1,1,1,1,1,1,1,1,1,1,1,1,1,1,1,1,1,1,1,1,1,1,1,1,1,1,
1,1,1,1,1,1,1,1,1,1,1,1,1,1,1,1,1,1,1,1,1,1,1,1,1,1,1,1,1,1,1,1,1,1,1,1,
1,1,1,1,1,1,1,1,1,1,1,1,1,1,1,1,1,1,1,1,1,1,1,1,1,1,1,1,1,1,1,1,1,1,1,1,
1,1,1,1,1,1,1,1,1,1,1,1,1,1,1,1,1,1,1,1,1,1,1,1,1,1,1,1,1,1,1,1,1,1,1,1,
1,1,1,1,1,1,1,1,1,1,1,1,1,1,1,1,1,1,1,1,1,1,1,1,1,1,1,1,1,1,1,6),(2,2),
(0.143172103,0.144954128,0.146788991,0.148623853,0.150458716,0.152293578,
0.15412844,0.155963303,0.157798165,0.159633028,0.16146789,0.163302752,0.165137615,
0.166972477,0.168807339,0.170642202,0.172477064,0.174311927,0.176146789,
0.177981651,0.179816514,0.181651376,0.183486239,0.185321101,0.187155963,
0.188990826,0.190825688,0.19266055,0.194495413,0.196330275,0.198165138,
0.2,0.201834862,0.203669725,0.205504587,0.20733945,0.209174312,0.211009174,
0.212844037,0.214678899,0.216513761,0.218348624,0.220183486,0.222018349,
0.223853211,0.225688073,0.227522936,0.229357798,0.231192661,0.233027523,
0.234862385,0.236697248,0.23853211,0.240366972,0.242201835,0.244036697,
0.24587156,0.247706422,0.249541284,0.251376147,0.253211009,0.255045872,
0.256880734,0.258715596,0.260550459,0.262385321,0.264220183,0.266055046,
0.267889908,0.269724771,0.271559633,0.273394495,0.275229358,0.27706422,
0.278899083,0.280733945,0.282568807,0.28440367,0.286238532,0.288073394,
0.289908257,0.291743119,0.293577982,0.295412844,0.297247706,0.299082569,
0.300917431,0.302752294,0.304587156,0.306422018,0.308256881,0.310091743,
0.311926606,0.313761468,0.31559633,0.317431193,0.319266055,0.321100917,
0.32293578,0.324770642,0.326605505,0.328440367,0.330275229,0.332110092,
0.333944954,0.335779817,0.337614679,0.339449541,0.341284404,0.343119266,
0.344954128,0.346788991,0.348623853,0.350458716,0.352293578,0.35412844,
0.355963303,0.357798165,0.359633028,0.36146789,0.363302752,0.365137615,
0.366972477,0.368807339,0.370642202,0.372477064,0.374311927,0.376146789,
0.377981651,0.379816514,0.381651376,0.383486239,0.385321101,0.387155963,
0.388990826,0.390825688,0.39266055,0.394495413,0.396330275,0.398165138,
0.4,0.401834862,0.403669725,0.405504587,0.40733945,0.409174312,0.411009174,
0.412844037,0.414678899,0.416513761,0.418348624,0.420183486,0.422018349,
0.423853211,0.425688073,0.427522936,0.429357798,0.431192661,0.433027523,
0.434862385,0.436697248,0.43853211,0.440366972,0.442201835,0.444036697,
0.44587156,0.447706422,0.449541284,0.451376147,0.453211009,0.455045872,
0.456880734,0.458715596,0.460550459,0.462385321,0.464220183,0.466055046,
0.467889908,0.469724771,0.471559633,0.473394495,0.475229358,0.47706422,
0.478899083,0.480733945,0.482568807,0.48440367,0.486238532,0.488073394,
0.489908257,0.491743119,0.493577982,0.495412844,0.497247706,0.499082569,
0.500917431,0.502752294,0.504587156,0.506422018,0.508256881,0.510091743,
0.511926606,0.513761468,0.51559633,0.517431193,0.519266055,0.521100917,
0.52293578,0.524770642,0.526605505,0.528440367,0.530275229,0.532110092,
0.533944954,0.535779817,0.537614679,0.539449541,0.541284404,0.543119266,
0.544954128,0.546788991,0.548623853,0.550458716,0.552293578,0.55412844,
0.555963303,0.557798165,0.559633028,0.56146789,0.563302752,0.565137615,
0.566972477,0.568807339,0.570642202,0.572477064,0.574311927,0.576146789,
0.577981651,0.579816514,0.581651376,0.583486239,0.585321101,0.587155963,
0.588990826,0.590825688,0.59266055,0.594495413,0.596330275,0.598165138,
0.6,0.601834862,0.603669725,0.605504587,0.60733945,0.609174312,0.611009174,
0.612844037,0.614678899,0.616513761,0.618348624,0.620183486,0.622018349,
0.623853211,0.625688073,0.627522936,0.629357798,0.631192661,0.633027523,
0.634862385,0.636697248,0.63853211,0.640366972,0.642201835,0.644036697,
0.64587156,0.647706422,0.649541284,0.651376147,0.653211009,0.655045872,
0.656880734,0.658715596,0.660550459,0.662385321,0.664220183,0.666055046,
0.667889908,0.669724771,0.671559633,0.673394495,0.675229358,0.67706422,
0.678899083,0.680733945,0.682568807,0.68440367,0.686238532,0.688073394,
0.689908257,0.691743119,0.693577982,0.695412844,0.697247706,0.699082569,
0.700917431,0.702752294,0.704587156,0.706422018,0.708256881,0.710091743,
0.711926606,0.713761468,0.71559633,0.717431193,0.719266055,0.721100917,
0.72293578,0.724770642,0.726605505,0.728440367,0.730275229,0.732110092,
0.733944954,0.735779817,0.737614679,0.739449541,0.741284404,0.743119266,
0.744954128,0.746788991,0.748623853,0.750458716,0.752293578,0.75412844,
0.755963303,0.757798165,0.759633028,0.76146789,0.763302752,0.765137615,
0.766972477,0.768807339,0.770642202,0.772477064,0.774311927,0.776146789,
0.777981651,0.779816514,0.781651376,0.783486239,0.785321101,0.787155963,
0.788990826,0.790825688,0.79266055,0.794495413,0.796330275,0.798165138,
0.8,0.801834862,0.803669725,0.805504587,0.80733945,0.809174312,0.811009174,
0.812844037,0.814678899,0.816513761,0.818348624,0.820183486,0.822018349,
0.823853211,0.825688073,0.827522936,0.829357798,0.831192661,0.833027523,
0.834862385,0.836697248,0.83853211,0.840366972,0.842201835,0.844036697,
0.84587156,0.847706422,0.849541284,0.851376147,0.853211009,0.855045872,
0.856880734,0.858715596,0.860550459,0.862385321,0.864220183,0.866055046,
0.867889908,0.869724771,0.871559633,0.873394495,0.875229358,0.87706422,
0.878899083,0.880733945,0.882568807,0.88440367,0.886238532,0.888073394,
0.889908257,0.891743119,0.893577982,0.895412844,0.897247706,0.899082569,
0.900917431,0.902752294,0.904587156,0.906422018,0.908256881,0.910091743,
0.911926606,0.913761468,0.91559633,0.917431193,0.919266055,0.921100917,
0.92293578,0.924770642,0.926605505,0.928440367,0.930275229,0.932110092,
0.933944954,0.935779817,0.937614679,0.939449541,0.941284404,0.943119266,
0.944954128,0.946788991,0.948623853,0.950458716,0.952293578,0.95412844,
0.955963303,0.957798165,0.959633028,0.96146789,0.963302752,0.965137615,
0.966972477,0.968807339,0.970642202,0.972477064,0.974311927,0.976146789,
0.977981651,0.979816514,0.981651376,0.983486239,0.985321101,0.987155963,
0.988990826,0.990825688,0.99266055,0.994495413,0.996330275,0.998165138,
1.),(0.,0.36),.UNSPECIFIED.);
#6236=B_SPLINE_SURFACE_WITH_KNOTS('',5,1,((#189434,#189435),(#189436,#189437),
(#189438,#189439),(#189440,#189441),(#189442,#189443),(#189444,#189445),
(#189446,#189447),(#189448,#189449),(#189450,#189451),(#189452,#189453),
(#189454,#189455),(#189456,#189457),(#189458,#189459),(#189460,#189461),
(#189462,#189463),(#189464,#189465),(#189466,#189467),(#189468,#189469),
(#189470,#189471),(#189472,#189473),(#189474,#189475),(#189476,#189477),
(#189478,#189479),(#189480,#189481),(#189482,#189483),(#189484,#189485),
(#189486,#189487),(#189488,#189489),(#189490,#189491),(#189492,#189493),
(#189494,#189495),(#189496,#189497),(#189498,#189499),(#189500,#189501),
(#189502,#189503),(#189504,#189505),(#189506,#189507),(#189508,#189509),
(#189510,#189511),(#189512,#189513),(#189514,#189515),(#189516,#189517),
(#189518,#189519),(#189520,#189521),(#189522,#189523),(#189524,#189525),
(#189526,#189527),(#189528,#189529),(#189530,#189531),(#189532,#189533),
(#189534,#189535),(#189536,#189537),(#189538,#189539),(#189540,#189541),
(#189542,#189543),(#189544,#189545),(#189546,#189547),(#189548,#189549),
(#189550,#189551),(#189552,#189553),(#189554,#189555),(#189556,#189557),
(#189558,#189559),(#189560,#189561),(#189562,#189563),(#189564,#189565),
(#189566,#189567),(#189568,#189569),(#189570,#189571),(#189572,#189573),
(#189574,#189575),(#189576,#189577),(#189578,#189579),(#189580,#189581),
(#189582,#189583),(#189584,#189585),(#189586,#189587),(#189588,#189589),
(#189590,#189591),(#189592,#189593),(#189594,#189595),(#189596,#189597),
(#189598,#189599),(#189600,#189601),(#189602,#189603),(#189604,#189605),
(#189606,#189607),(#189608,#189609),(#189610,#189611),(#189612,#189613),
(#189614,#189615),(#189616,#189617),(#189618,#189619),(#189620,#189621),
(#189622,#189623),(#189624,#189625),(#189626,#189627),(#189628,#189629),
(#189630,#189631),(#189632,#189633),(#189634,#189635),(#189636,#189637),
(#189638,#189639),(#189640,#189641),(#189642,#189643),(#189644,#189645),
(#189646,#189647),(#189648,#189649),(#189650,#189651),(#189652,#189653),
(#189654,#189655),(#189656,#189657),(#189658,#189659),(#189660,#189661),
(#189662,#189663),(#189664,#189665),(#189666,#189667),(#189668,#189669),
(#189670,#189671),(#189672,#189673),(#189674,#189675),(#189676,#189677),
(#189678,#189679),(#189680,#189681),(#189682,#189683),(#189684,#189685),
(#189686,#189687),(#189688,#189689),(#189690,#189691),(#189692,#189693),
(#189694,#189695),(#189696,#189697),(#189698,#189699),(#189700,#189701),
(#189702,#189703),(#189704,#189705),(#189706,#189707),(#189708,#189709),
(#189710,#189711),(#189712,#189713),(#189714,#189715),(#189716,#189717),
(#189718,#189719),(#189720,#189721),(#189722,#189723),(#189724,#189725),
(#189726,#189727),(#189728,#189729),(#189730,#189731),(#189732,#189733),
(#189734,#189735),(#189736,#189737),(#189738,#189739),(#189740,#189741),
(#189742,#189743),(#189744,#189745),(#189746,#189747),(#189748,#189749),
(#189750,#189751),(#189752,#189753),(#189754,#189755),(#189756,#189757),
(#189758,#189759),(#189760,#189761),(#189762,#189763),(#189764,#189765),
(#189766,#189767),(#189768,#189769),(#189770,#189771),(#189772,#189773),
(#189774,#189775),(#189776,#189777),(#189778,#189779),(#189780,#189781),
(#189782,#189783),(#189784,#189785),(#189786,#189787),(#189788,#189789),
(#189790,#189791),(#189792,#189793),(#189794,#189795),(#189796,#189797),
(#189798,#189799),(#189800,#189801),(#189802,#189803),(#189804,#189805),
(#189806,#189807),(#189808,#189809),(#189810,#189811),(#189812,#189813),
(#189814,#189815),(#189816,#189817),(#189818,#189819),(#189820,#189821),
(#189822,#189823),(#189824,#189825),(#189826,#189827),(#189828,#189829),
(#189830,#189831),(#189832,#189833),(#189834,#189835),(#189836,#189837),
(#189838,#189839),(#189840,#189841),(#189842,#189843),(#189844,#189845),
(#189846,#189847),(#189848,#189849),(#189850,#189851),(#189852,#189853),
(#189854,#189855),(#189856,#189857),(#189858,#189859),(#189860,#189861),
(#189862,#189863),(#189864,#189865),(#189866,#189867),(#189868,#189869),
(#189870,#189871),(#189872,#189873),(#189874,#189875),(#189876,#189877),
(#189878,#189879),(#189880,#189881),(#189882,#189883),(#189884,#189885),
(#189886,#189887),(#189888,#189889),(#189890,#189891),(#189892,#189893),
(#189894,#189895),(#189896,#189897),(#189898,#189899),(#189900,#189901),
(#189902,#189903),(#189904,#189905),(#189906,#189907),(#189908,#189909),
(#189910,#189911),(#189912,#189913),(#189914,#189915),(#189916,#189917),
(#189918,#189919),(#189920,#189921),(#189922,#189923),(#189924,#189925),
(#189926,#189927),(#189928,#189929),(#189930,#189931),(#189932,#189933),
(#189934,#189935),(#189936,#189937),(#189938,#189939),(#189940,#189941),
(#189942,#189943),(#189944,#189945),(#189946,#189947),(#189948,#189949),
(#189950,#189951),(#189952,#189953),(#189954,#189955),(#189956,#189957),
(#189958,#189959),(#189960,#189961),(#189962,#189963),(#189964,#189965),
(#189966,#189967),(#189968,#189969),(#189970,#189971),(#189972,#189973),
(#189974,#189975),(#189976,#189977),(#189978,#189979),(#189980,#189981),
(#189982,#189983),(#189984,#189985),(#189986,#189987),(#189988,#189989),
(#189990,#189991),(#189992,#189993),(#189994,#189995),(#189996,#189997),
(#189998,#189999),(#190000,#190001),(#190002,#190003),(#190004,#190005),
(#190006,#190007),(#190008,#190009),(#190010,#190011),(#190012,#190013),
(#190014,#190015),(#190016,#190017),(#190018,#190019),(#190020,#190021),
(#190022,#190023),(#190024,#190025),(#190026,#190027),(#190028,#190029),
(#190030,#190031),(#190032,#190033),(#190034,#190035),(#190036,#190037),
(#190038,#190039),(#190040,#190041),(#190042,#190043),(#190044,#190045),
(#190046,#190047),(#190048,#190049),(#190050,#190051),(#190052,#190053),
(#190054,#190055),(#190056,#190057),(#190058,#190059),(#190060,#190061),
(#190062,#190063),(#190064,#190065),(#190066,#190067),(#190068,#190069),
(#190070,#190071),(#190072,#190073),(#190074,#190075),(#190076,#190077),
(#190078,#190079),(#190080,#190081),(#190082,#190083),(#190084,#190085),
(#190086,#190087),(#190088,#190089),(#190090,#190091),(#190092,#190093),
(#190094,#190095),(#190096,#190097),(#190098,#190099),(#190100,#190101),
(#190102,#190103),(#190104,#190105),(#190106,#190107),(#190108,#190109),
(#190110,#190111),(#190112,#190113),(#190114,#190115),(#190116,#190117),
(#190118,#190119),(#190120,#190121),(#190122,#190123),(#190124,#190125),
(#190126,#190127),(#190128,#190129),(#190130,#190131),(#190132,#190133),
(#190134,#190135),(#190136,#190137),(#190138,#190139),(#190140,#190141),
(#190142,#190143),(#190144,#190145),(#190146,#190147),(#190148,#190149),
(#190150,#190151),(#190152,#190153),(#190154,#190155),(#190156,#190157),
(#190158,#190159),(#190160,#190161),(#190162,#190163),(#190164,#190165),
(#190166,#190167),(#190168,#190169),(#190170,#190171),(#190172,#190173),
(#190174,#190175),(#190176,#190177),(#190178,#190179),(#190180,#190181),
(#190182,#190183),(#190184,#190185),(#190186,#190187),(#190188,#190189),
(#190190,#190191),(#190192,#190193),(#190194,#190195),(#190196,#190197),
(#190198,#190199),(#190200,#190201),(#190202,#190203),(#190204,#190205),
(#190206,#190207),(#190208,#190209),(#190210,#190211),(#190212,#190213),
(#190214,#190215),(#190216,#190217),(#190218,#190219),(#190220,#190221),
(#190222,#190223),(#190224,#190225),(#190226,#190227),(#190228,#190229),
(#190230,#190231),(#190232,#190233),(#190234,#190235),(#190236,#190237),
(#190238,#190239),(#190240,#190241),(#190242,#190243),(#190244,#190245),
(#190246,#190247),(#190248,#190249),(#190250,#190251),(#190252,#190253),
(#190254,#190255),(#190256,#190257),(#190258,#190259),(#190260,#190261),
(#190262,#190263),(#190264,#190265),(#190266,#190267),(#190268,#190269),
(#190270,#190271),(#190272,#190273),(#190274,#190275),(#190276,#190277),
(#190278,#190279),(#190280,#190281),(#190282,#190283),(#190284,#190285),
(#190286,#190287),(#190288,#190289),(#190290,#190291),(#190292,#190293),
(#190294,#190295),(#190296,#190297),(#190298,#190299),(#190300,#190301),
(#190302,#190303),(#190304,#190305),(#190306,#190307),(#190308,#190309),
(#190310,#190311),(#190312,#190313),(#190314,#190315),(#190316,#190317),
(#190318,#190319),(#190320,#190321),(#190322,#190323),(#190324,#190325),
(#190326,#190327),(#190328,#190329),(#190330,#190331),(#190332,#190333),
(#190334,#190335),(#190336,#190337),(#190338,#190339),(#190340,#190341),
(#190342,#190343),(#190344,#190345),(#190346,#190347),(#190348,#190349),
(#190350,#190351),(#190352,#190353),(#190354,#190355),(#190356,#190357),
(#190358,#190359),(#190360,#190361),(#190362,#190363),(#190364,#190365),
(#190366,#190367),(#190368,#190369),(#190370,#190371),(#190372,#190373),
(#190374,#190375),(#190376,#190377)),.UNSPECIFIED.,.F.,.F.,.F.,(6,1,1,1,
1,1,1,1,1,1,1,1,1,1,1,1,1,1,1,1,1,1,1,1,1,1,1,1,1,1,1,1,1,1,1,1,1,1,1,1,
1,1,1,1,1,1,1,1,1,1,1,1,1,1,1,1,1,1,1,1,1,1,1,1,1,1,1,1,1,1,1,1,1,1,1,1,
1,1,1,1,1,1,1,1,1,1,1,1,1,1,1,1,1,1,1,1,1,1,1,1,1,1,1,1,1,1,1,1,1,1,1,1,
1,1,1,1,1,1,1,1,1,1,1,1,1,1,1,1,1,1,1,1,1,1,1,1,1,1,1,1,1,1,1,1,1,1,1,1,
1,1,1,1,1,1,1,1,1,1,1,1,1,1,1,1,1,1,1,1,1,1,1,1,1,1,1,1,1,1,1,1,1,1,1,1,
1,1,1,1,1,1,1,1,1,1,1,1,1,1,1,1,1,1,1,1,1,1,1,1,1,1,1,1,1,1,1,1,1,1,1,1,
1,1,1,1,1,1,1,1,1,1,1,1,1,1,1,1,1,1,1,1,1,1,1,1,1,1,1,1,1,1,1,1,1,1,1,1,
1,1,1,1,1,1,1,1,1,1,1,1,1,1,1,1,1,1,1,1,1,1,1,1,1,1,1,1,1,1,1,1,1,1,1,1,
1,1,1,1,1,1,1,1,1,1,1,1,1,1,1,1,1,1,1,1,1,1,1,1,1,1,1,1,1,1,1,1,1,1,1,1,
1,1,1,1,1,1,1,1,1,1,1,1,1,1,1,1,1,1,1,1,1,1,1,1,1,1,1,1,1,1,1,1,1,1,1,1,
1,1,1,1,1,1,1,1,1,1,1,1,1,1,1,1,1,1,1,1,1,1,1,1,1,1,1,1,1,1,1,1,1,1,1,1,
1,1,1,1,1,1,1,1,1,1,1,1,1,1,1,1,1,1,1,1,1,1,1,1,1,1,1,1,1,1,1,1,1,1,1,1,
1,1,1,1,1,1,1,1,1,1,1,1,1,1,1,1,1,1,1,1,1,1,1,1,1,1,1,1,1,1,1,6),(2,2),
(-1.,-0.998165138,-0.996330275,-0.994495413,-0.99266055,-0.990825688,-0.988990826,
-0.987155963,-0.985321101,-0.983486239,-0.981651376,-0.979816514,-0.977981651,
-0.976146789,-0.974311927,-0.972477064,-0.970642202,-0.968807339,-0.966972477,
-0.965137615,-0.963302752,-0.96146789,-0.959633028,-0.957798165,-0.955963303,
-0.95412844,-0.952293578,-0.950458716,-0.948623853,-0.946788991,-0.944954128,
-0.943119266,-0.941284404,-0.939449541,-0.937614679,-0.935779817,-0.933944954,
-0.932110092,-0.930275229,-0.928440367,-0.926605505,-0.924770642,-0.92293578,
-0.921100917,-0.919266055,-0.917431193,-0.91559633,-0.913761468,-0.911926606,
-0.910091743,-0.908256881,-0.906422018,-0.904587156,-0.902752294,-0.900917431,
-0.899082569,-0.897247706,-0.895412844,-0.893577982,-0.891743119,-0.889908257,
-0.888073394,-0.886238532,-0.88440367,-0.882568807,-0.880733945,-0.878899083,
-0.87706422,-0.875229358,-0.873394495,-0.871559633,-0.869724771,-0.867889908,
-0.866055046,-0.864220183,-0.862385321,-0.860550459,-0.858715596,-0.856880734,
-0.855045872,-0.853211009,-0.851376147,-0.849541284,-0.847706422,-0.84587156,
-0.844036697,-0.842201835,-0.840366972,-0.83853211,-0.836697248,-0.834862385,
-0.833027523,-0.831192661,-0.829357798,-0.827522936,-0.825688073,-0.823853211,
-0.822018349,-0.820183486,-0.818348624,-0.816513761,-0.814678899,-0.812844037,
-0.811009174,-0.809174312,-0.80733945,-0.805504587,-0.803669725,-0.801834862,
-0.8,-0.798165138,-0.796330275,-0.794495413,-0.79266055,-0.790825688,-0.788990826,
-0.787155963,-0.785321101,-0.783486239,-0.781651376,-0.779816514,-0.777981651,
-0.776146789,-0.774311927,-0.772477064,-0.770642202,-0.768807339,-0.766972477,
-0.765137615,-0.763302752,-0.76146789,-0.759633028,-0.757798165,-0.755963303,
-0.75412844,-0.752293578,-0.750458716,-0.748623853,-0.746788991,-0.744954128,
-0.743119266,-0.741284404,-0.739449541,-0.737614679,-0.735779817,-0.733944954,
-0.732110092,-0.730275229,-0.728440367,-0.726605505,-0.724770642,-0.72293578,
-0.721100917,-0.719266055,-0.717431193,-0.71559633,-0.713761468,-0.711926606,
-0.710091743,-0.708256881,-0.706422018,-0.704587156,-0.702752294,-0.700917431,
-0.699082569,-0.697247706,-0.695412844,-0.693577982,-0.691743119,-0.689908257,
-0.688073394,-0.686238532,-0.68440367,-0.682568807,-0.680733945,-0.678899083,
-0.67706422,-0.675229358,-0.673394495,-0.671559633,-0.669724771,-0.667889908,
-0.666055046,-0.664220183,-0.662385321,-0.660550459,-0.658715596,-0.656880734,
-0.655045872,-0.653211009,-0.651376147,-0.649541284,-0.647706422,-0.64587156,
-0.644036697,-0.642201835,-0.640366972,-0.63853211,-0.636697248,-0.634862385,
-0.633027523,-0.631192661,-0.629357798,-0.627522936,-0.625688073,-0.623853211,
-0.622018349,-0.620183486,-0.618348624,-0.616513761,-0.614678899,-0.612844037,
-0.611009174,-0.609174312,-0.60733945,-0.605504587,-0.603669725,-0.601834862,
-0.6,-0.598165138,-0.596330275,-0.594495413,-0.59266055,-0.590825688,-0.588990826,
-0.587155963,-0.585321101,-0.583486239,-0.581651376,-0.579816514,-0.577981651,
-0.576146789,-0.574311927,-0.572477064,-0.570642202,-0.568807339,-0.566972477,
-0.565137615,-0.563302752,-0.56146789,-0.559633028,-0.557798165,-0.555963303,
-0.55412844,-0.552293578,-0.550458716,-0.548623853,-0.546788991,-0.544954128,
-0.543119266,-0.541284404,-0.539449541,-0.537614679,-0.535779817,-0.533944954,
-0.532110092,-0.530275229,-0.528440367,-0.526605505,-0.524770642,-0.52293578,
-0.521100917,-0.519266055,-0.517431193,-0.51559633,-0.513761468,-0.511926606,
-0.510091743,-0.508256881,-0.506422018,-0.504587156,-0.502752294,-0.500917431,
-0.499082569,-0.497247706,-0.495412844,-0.493577982,-0.491743119,-0.489908257,
-0.488073394,-0.486238532,-0.48440367,-0.482568807,-0.480733945,-0.478899083,
-0.47706422,-0.475229358,-0.473394495,-0.471559633,-0.469724771,-0.467889908,
-0.466055046,-0.464220183,-0.462385321,-0.460550459,-0.458715596,-0.456880734,
-0.455045872,-0.453211009,-0.451376147,-0.449541284,-0.447706422,-0.44587156,
-0.444036697,-0.442201835,-0.440366972,-0.43853211,-0.436697248,-0.434862385,
-0.433027523,-0.431192661,-0.429357798,-0.427522936,-0.425688073,-0.423853211,
-0.422018349,-0.420183486,-0.418348624,-0.416513761,-0.414678899,-0.412844037,
-0.411009174,-0.409174312,-0.40733945,-0.405504587,-0.403669725,-0.401834862,
-0.4,-0.398165138,-0.396330275,-0.394495413,-0.39266055,-0.390825688,-0.388990826,
-0.387155963,-0.385321101,-0.383486239,-0.381651376,-0.379816514,-0.377981651,
-0.376146789,-0.374311927,-0.372477064,-0.370642202,-0.368807339,-0.366972477,
-0.365137615,-0.363302752,-0.36146789,-0.359633028,-0.357798165,-0.355963303,
-0.35412844,-0.352293578,-0.350458716,-0.348623853,-0.346788991,-0.344954128,
-0.343119266,-0.341284404,-0.339449541,-0.337614679,-0.335779817,-0.333944954,
-0.332110092,-0.330275229,-0.328440367,-0.326605505,-0.324770642,-0.32293578,
-0.321100917,-0.319266055,-0.317431193,-0.31559633,-0.313761468,-0.311926606,
-0.310091743,-0.308256881,-0.306422018,-0.304587156,-0.302752294,-0.300917431,
-0.299082569,-0.297247706,-0.295412844,-0.293577982,-0.291743119,-0.289908257,
-0.288073394,-0.286238532,-0.28440367,-0.282568807,-0.280733945,-0.278899083,
-0.27706422,-0.275229358,-0.273394495,-0.271559633,-0.269724771,-0.267889908,
-0.266055046,-0.264220183,-0.262385321,-0.260550459,-0.258715596,-0.256880734,
-0.255045872,-0.253211009,-0.251376147,-0.249541284,-0.247706422,-0.24587156,
-0.244036697,-0.242201835,-0.240366972,-0.23853211,-0.236697248,-0.234862385,
-0.233027523,-0.231192661,-0.229357798,-0.227522936,-0.225688073,-0.223853211,
-0.222018349,-0.220183486,-0.218348624,-0.216513761,-0.214678899,-0.212844037,
-0.211009174,-0.209174312,-0.20733945,-0.205504587,-0.203669725,-0.201834862,
-0.2,-0.198165138,-0.196330275,-0.194495413,-0.19266055,-0.190825688,-0.188990826,
-0.187155963,-0.185321101,-0.183486239,-0.181651376,-0.179816514,-0.177981651,
-0.176146789,-0.174311927,-0.172477064,-0.170642202,-0.168807339,-0.166972477,
-0.165137615,-0.163302752,-0.16146789,-0.159633028,-0.157798165,-0.155963303,
-0.15412844,-0.152293578,-0.150458716,-0.148623853,-0.146788991,-0.144954128,
-0.143172103),(0.,0.36),.UNSPECIFIED.);
#6237=B_SPLINE_SURFACE_WITH_KNOTS('',5,1,((#191016,#191017),(#191018,#191019),
(#191020,#191021),(#191022,#191023),(#191024,#191025),(#191026,#191027),
(#191028,#191029),(#191030,#191031),(#191032,#191033),(#191034,#191035),
(#191036,#191037),(#191038,#191039),(#191040,#191041),(#191042,#191043),
(#191044,#191045),(#191046,#191047),(#191048,#191049),(#191050,#191051),
(#191052,#191053),(#191054,#191055),(#191056,#191057),(#191058,#191059),
(#191060,#191061),(#191062,#191063),(#191064,#191065),(#191066,#191067),
(#191068,#191069),(#191070,#191071),(#191072,#191073),(#191074,#191075),
(#191076,#191077),(#191078,#191079),(#191080,#191081),(#191082,#191083),
(#191084,#191085),(#191086,#191087),(#191088,#191089),(#191090,#191091),
(#191092,#191093),(#191094,#191095),(#191096,#191097),(#191098,#191099),
(#191100,#191101),(#191102,#191103),(#191104,#191105),(#191106,#191107),
(#191108,#191109),(#191110,#191111),(#191112,#191113),(#191114,#191115),
(#191116,#191117),(#191118,#191119),(#191120,#191121),(#191122,#191123),
(#191124,#191125),(#191126,#191127),(#191128,#191129),(#191130,#191131),
(#191132,#191133),(#191134,#191135),(#191136,#191137),(#191138,#191139),
(#191140,#191141),(#191142,#191143),(#191144,#191145),(#191146,#191147),
(#191148,#191149),(#191150,#191151),(#191152,#191153),(#191154,#191155),
(#191156,#191157),(#191158,#191159),(#191160,#191161),(#191162,#191163),
(#191164,#191165),(#191166,#191167),(#191168,#191169),(#191170,#191171),
(#191172,#191173),(#191174,#191175),(#191176,#191177),(#191178,#191179),
(#191180,#191181),(#191182,#191183),(#191184,#191185),(#191186,#191187),
(#191188,#191189),(#191190,#191191),(#191192,#191193),(#191194,#191195),
(#191196,#191197),(#191198,#191199),(#191200,#191201),(#191202,#191203),
(#191204,#191205),(#191206,#191207),(#191208,#191209),(#191210,#191211),
(#191212,#191213),(#191214,#191215),(#191216,#191217),(#191218,#191219),
(#191220,#191221),(#191222,#191223),(#191224,#191225),(#191226,#191227),
(#191228,#191229),(#191230,#191231),(#191232,#191233),(#191234,#191235),
(#191236,#191237),(#191238,#191239),(#191240,#191241),(#191242,#191243),
(#191244,#191245),(#191246,#191247),(#191248,#191249),(#191250,#191251),
(#191252,#191253),(#191254,#191255),(#191256,#191257),(#191258,#191259),
(#191260,#191261),(#191262,#191263),(#191264,#191265),(#191266,#191267),
(#191268,#191269),(#191270,#191271),(#191272,#191273),(#191274,#191275),
(#191276,#191277),(#191278,#191279),(#191280,#191281),(#191282,#191283),
(#191284,#191285),(#191286,#191287),(#191288,#191289),(#191290,#191291),
(#191292,#191293),(#191294,#191295),(#191296,#191297),(#191298,#191299),
(#191300,#191301),(#191302,#191303),(#191304,#191305),(#191306,#191307),
(#191308,#191309),(#191310,#191311),(#191312,#191313),(#191314,#191315),
(#191316,#191317),(#191318,#191319),(#191320,#191321),(#191322,#191323),
(#191324,#191325),(#191326,#191327),(#191328,#191329),(#191330,#191331),
(#191332,#191333),(#191334,#191335),(#191336,#191337),(#191338,#191339),
(#191340,#191341),(#191342,#191343),(#191344,#191345),(#191346,#191347),
(#191348,#191349),(#191350,#191351),(#191352,#191353),(#191354,#191355),
(#191356,#191357),(#191358,#191359),(#191360,#191361),(#191362,#191363),
(#191364,#191365),(#191366,#191367),(#191368,#191369),(#191370,#191371),
(#191372,#191373),(#191374,#191375),(#191376,#191377),(#191378,#191379),
(#191380,#191381),(#191382,#191383),(#191384,#191385),(#191386,#191387),
(#191388,#191389),(#191390,#191391),(#191392,#191393),(#191394,#191395),
(#191396,#191397),(#191398,#191399),(#191400,#191401),(#191402,#191403),
(#191404,#191405),(#191406,#191407),(#191408,#191409),(#191410,#191411),
(#191412,#191413),(#191414,#191415),(#191416,#191417),(#191418,#191419),
(#191420,#191421),(#191422,#191423),(#191424,#191425),(#191426,#191427),
(#191428,#191429),(#191430,#191431),(#191432,#191433),(#191434,#191435),
(#191436,#191437),(#191438,#191439),(#191440,#191441),(#191442,#191443),
(#191444,#191445),(#191446,#191447),(#191448,#191449),(#191450,#191451),
(#191452,#191453),(#191454,#191455),(#191456,#191457),(#191458,#191459),
(#191460,#191461),(#191462,#191463),(#191464,#191465),(#191466,#191467),
(#191468,#191469),(#191470,#191471),(#191472,#191473),(#191474,#191475),
(#191476,#191477),(#191478,#191479),(#191480,#191481),(#191482,#191483),
(#191484,#191485),(#191486,#191487),(#191488,#191489),(#191490,#191491),
(#191492,#191493),(#191494,#191495),(#191496,#191497),(#191498,#191499),
(#191500,#191501),(#191502,#191503),(#191504,#191505),(#191506,#191507),
(#191508,#191509),(#191510,#191511),(#191512,#191513),(#191514,#191515),
(#191516,#191517),(#191518,#191519),(#191520,#191521),(#191522,#191523),
(#191524,#191525),(#191526,#191527),(#191528,#191529),(#191530,#191531),
(#191532,#191533),(#191534,#191535),(#191536,#191537),(#191538,#191539),
(#191540,#191541),(#191542,#191543),(#191544,#191545),(#191546,#191547),
(#191548,#191549),(#191550,#191551),(#191552,#191553),(#191554,#191555),
(#191556,#191557),(#191558,#191559),(#191560,#191561),(#191562,#191563),
(#191564,#191565),(#191566,#191567),(#191568,#191569),(#191570,#191571),
(#191572,#191573),(#191574,#191575),(#191576,#191577),(#191578,#191579),
(#191580,#191581),(#191582,#191583),(#191584,#191585),(#191586,#191587),
(#191588,#191589),(#191590,#191591),(#191592,#191593),(#191594,#191595),
(#191596,#191597),(#191598,#191599),(#191600,#191601),(#191602,#191603),
(#191604,#191605),(#191606,#191607),(#191608,#191609),(#191610,#191611),
(#191612,#191613),(#191614,#191615),(#191616,#191617),(#191618,#191619),
(#191620,#191621),(#191622,#191623),(#191624,#191625),(#191626,#191627),
(#191628,#191629),(#191630,#191631),(#191632,#191633),(#191634,#191635),
(#191636,#191637),(#191638,#191639),(#191640,#191641),(#191642,#191643),
(#191644,#191645),(#191646,#191647),(#191648,#191649),(#191650,#191651),
(#191652,#191653),(#191654,#191655),(#191656,#191657),(#191658,#191659),
(#191660,#191661),(#191662,#191663),(#191664,#191665),(#191666,#191667),
(#191668,#191669),(#191670,#191671),(#191672,#191673),(#191674,#191675),
(#191676,#191677),(#191678,#191679),(#191680,#191681),(#191682,#191683),
(#191684,#191685),(#191686,#191687),(#191688,#191689),(#191690,#191691),
(#191692,#191693),(#191694,#191695),(#191696,#191697),(#191698,#191699),
(#191700,#191701),(#191702,#191703),(#191704,#191705),(#191706,#191707),
(#191708,#191709),(#191710,#191711),(#191712,#191713),(#191714,#191715),
(#191716,#191717),(#191718,#191719),(#191720,#191721),(#191722,#191723),
(#191724,#191725),(#191726,#191727),(#191728,#191729),(#191730,#191731),
(#191732,#191733),(#191734,#191735),(#191736,#191737),(#191738,#191739),
(#191740,#191741),(#191742,#191743),(#191744,#191745),(#191746,#191747),
(#191748,#191749),(#191750,#191751),(#191752,#191753),(#191754,#191755),
(#191756,#191757),(#191758,#191759),(#191760,#191761),(#191762,#191763),
(#191764,#191765),(#191766,#191767),(#191768,#191769),(#191770,#191771),
(#191772,#191773),(#191774,#191775),(#191776,#191777),(#191778,#191779),
(#191780,#191781),(#191782,#191783),(#191784,#191785),(#191786,#191787),
(#191788,#191789),(#191790,#191791),(#191792,#191793),(#191794,#191795),
(#191796,#191797),(#191798,#191799),(#191800,#191801),(#191802,#191803),
(#191804,#191805),(#191806,#191807),(#191808,#191809),(#191810,#191811),
(#191812,#191813),(#191814,#191815),(#191816,#191817),(#191818,#191819),
(#191820,#191821),(#191822,#191823),(#191824,#191825),(#191826,#191827),
(#191828,#191829),(#191830,#191831),(#191832,#191833),(#191834,#191835),
(#191836,#191837),(#191838,#191839),(#191840,#191841),(#191842,#191843),
(#191844,#191845),(#191846,#191847),(#191848,#191849),(#191850,#191851),
(#191852,#191853),(#191854,#191855),(#191856,#191857),(#191858,#191859),
(#191860,#191861),(#191862,#191863),(#191864,#191865),(#191866,#191867),
(#191868,#191869),(#191870,#191871),(#191872,#191873),(#191874,#191875),
(#191876,#191877),(#191878,#191879),(#191880,#191881),(#191882,#191883),
(#191884,#191885),(#191886,#191887),(#191888,#191889),(#191890,#191891),
(#191892,#191893),(#191894,#191895),(#191896,#191897),(#191898,#191899),
(#191900,#191901),(#191902,#191903),(#191904,#191905),(#191906,#191907),
(#191908,#191909),(#191910,#191911),(#191912,#191913),(#191914,#191915),
(#191916,#191917),(#191918,#191919),(#191920,#191921),(#191922,#191923),
(#191924,#191925),(#191926,#191927),(#191928,#191929),(#191930,#191931),
(#191932,#191933),(#191934,#191935),(#191936,#191937),(#191938,#191939),
(#191940,#191941),(#191942,#191943),(#191944,#191945),(#191946,#191947),
(#191948,#191949),(#191950,#191951),(#191952,#191953),(#191954,#191955),
(#191956,#191957),(#191958,#191959)),.UNSPECIFIED.,.F.,.F.,.F.,(6,1,1,1,
1,1,1,1,1,1,1,1,1,1,1,1,1,1,1,1,1,1,1,1,1,1,1,1,1,1,1,1,1,1,1,1,1,1,1,1,
1,1,1,1,1,1,1,1,1,1,1,1,1,1,1,1,1,1,1,1,1,1,1,1,1,1,1,1,1,1,1,1,1,1,1,1,
1,1,1,1,1,1,1,1,1,1,1,1,1,1,1,1,1,1,1,1,1,1,1,1,1,1,1,1,1,1,1,1,1,1,1,1,
1,1,1,1,1,1,1,1,1,1,1,1,1,1,1,1,1,1,1,1,1,1,1,1,1,1,1,1,1,1,1,1,1,1,1,1,
1,1,1,1,1,1,1,1,1,1,1,1,1,1,1,1,1,1,1,1,1,1,1,1,1,1,1,1,1,1,1,1,1,1,1,1,
1,1,1,1,1,1,1,1,1,1,1,1,1,1,1,1,1,1,1,1,1,1,1,1,1,1,1,1,1,1,1,1,1,1,1,1,
1,1,1,1,1,1,1,1,1,1,1,1,1,1,1,1,1,1,1,1,1,1,1,1,1,1,1,1,1,1,1,1,1,1,1,1,
1,1,1,1,1,1,1,1,1,1,1,1,1,1,1,1,1,1,1,1,1,1,1,1,1,1,1,1,1,1,1,1,1,1,1,1,
1,1,1,1,1,1,1,1,1,1,1,1,1,1,1,1,1,1,1,1,1,1,1,1,1,1,1,1,1,1,1,1,1,1,1,1,
1,1,1,1,1,1,1,1,1,1,1,1,1,1,1,1,1,1,1,1,1,1,1,1,1,1,1,1,1,1,1,1,1,1,1,1,
1,1,1,1,1,1,1,1,1,1,1,1,1,1,1,1,1,1,1,1,1,1,1,1,1,1,1,1,1,1,1,1,1,1,1,1,
1,1,1,1,1,1,1,1,1,1,1,1,1,1,1,1,1,1,1,1,1,1,1,1,1,1,1,1,1,1,1,1,1,1,1,1,
1,1,1,1,1,1,1,1,1,1,1,1,1,1,1,1,1,1,1,1,1,1,1,1,1,1,1,1,1,1,1,6),(2,2),
(-1.,-0.998165138,-0.996330275,-0.994495413,-0.99266055,-0.990825688,-0.988990826,
-0.987155963,-0.985321101,-0.983486239,-0.981651376,-0.979816514,-0.977981651,
-0.976146789,-0.974311927,-0.972477064,-0.970642202,-0.968807339,-0.966972477,
-0.965137615,-0.963302752,-0.96146789,-0.959633028,-0.957798165,-0.955963303,
-0.95412844,-0.952293578,-0.950458716,-0.948623853,-0.946788991,-0.944954128,
-0.943119266,-0.941284404,-0.939449541,-0.937614679,-0.935779817,-0.933944954,
-0.932110092,-0.930275229,-0.928440367,-0.926605505,-0.924770642,-0.92293578,
-0.921100917,-0.919266055,-0.917431193,-0.91559633,-0.913761468,-0.911926606,
-0.910091743,-0.908256881,-0.906422018,-0.904587156,-0.902752294,-0.900917431,
-0.899082569,-0.897247706,-0.895412844,-0.893577982,-0.891743119,-0.889908257,
-0.888073394,-0.886238532,-0.88440367,-0.882568807,-0.880733945,-0.878899083,
-0.87706422,-0.875229358,-0.873394495,-0.871559633,-0.869724771,-0.867889908,
-0.866055046,-0.864220183,-0.862385321,-0.860550459,-0.858715596,-0.856880734,
-0.855045872,-0.853211009,-0.851376147,-0.849541284,-0.847706422,-0.84587156,
-0.844036697,-0.842201835,-0.840366972,-0.83853211,-0.836697248,-0.834862385,
-0.833027523,-0.831192661,-0.829357798,-0.827522936,-0.825688073,-0.823853211,
-0.822018349,-0.820183486,-0.818348624,-0.816513761,-0.814678899,-0.812844037,
-0.811009174,-0.809174312,-0.80733945,-0.805504587,-0.803669725,-0.801834862,
-0.8,-0.798165138,-0.796330275,-0.794495413,-0.79266055,-0.790825688,-0.788990826,
-0.787155963,-0.785321101,-0.783486239,-0.781651376,-0.779816514,-0.777981651,
-0.776146789,-0.774311927,-0.772477064,-0.770642202,-0.768807339,-0.766972477,
-0.765137615,-0.763302752,-0.76146789,-0.759633028,-0.757798165,-0.755963303,
-0.75412844,-0.752293578,-0.750458716,-0.748623853,-0.746788991,-0.744954128,
-0.743119266,-0.741284404,-0.739449541,-0.737614679,-0.735779817,-0.733944954,
-0.732110092,-0.730275229,-0.728440367,-0.726605505,-0.724770642,-0.72293578,
-0.721100917,-0.719266055,-0.717431193,-0.71559633,-0.713761468,-0.711926606,
-0.710091743,-0.708256881,-0.706422018,-0.704587156,-0.702752294,-0.700917431,
-0.699082569,-0.697247706,-0.695412844,-0.693577982,-0.691743119,-0.689908257,
-0.688073394,-0.686238532,-0.68440367,-0.682568807,-0.680733945,-0.678899083,
-0.67706422,-0.675229358,-0.673394495,-0.671559633,-0.669724771,-0.667889908,
-0.666055046,-0.664220183,-0.662385321,-0.660550459,-0.658715596,-0.656880734,
-0.655045872,-0.653211009,-0.651376147,-0.649541284,-0.647706422,-0.64587156,
-0.644036697,-0.642201835,-0.640366972,-0.63853211,-0.636697248,-0.634862385,
-0.633027523,-0.631192661,-0.629357798,-0.627522936,-0.625688073,-0.623853211,
-0.622018349,-0.620183486,-0.618348624,-0.616513761,-0.614678899,-0.612844037,
-0.611009174,-0.609174312,-0.60733945,-0.605504587,-0.603669725,-0.601834862,
-0.6,-0.598165138,-0.596330275,-0.594495413,-0.59266055,-0.590825688,-0.588990826,
-0.587155963,-0.585321101,-0.583486239,-0.581651376,-0.579816514,-0.577981651,
-0.576146789,-0.574311927,-0.572477064,-0.570642202,-0.568807339,-0.566972477,
-0.565137615,-0.563302752,-0.56146789,-0.559633028,-0.557798165,-0.555963303,
-0.55412844,-0.552293578,-0.550458716,-0.548623853,-0.546788991,-0.544954128,
-0.543119266,-0.541284404,-0.539449541,-0.537614679,-0.535779817,-0.533944954,
-0.532110092,-0.530275229,-0.528440367,-0.526605505,-0.524770642,-0.52293578,
-0.521100917,-0.519266055,-0.517431193,-0.51559633,-0.513761468,-0.511926606,
-0.510091743,-0.508256881,-0.506422018,-0.504587156,-0.502752294,-0.500917431,
-0.499082569,-0.497247706,-0.495412844,-0.493577982,-0.491743119,-0.489908257,
-0.488073394,-0.486238532,-0.48440367,-0.482568807,-0.480733945,-0.478899083,
-0.47706422,-0.475229358,-0.473394495,-0.471559633,-0.469724771,-0.467889908,
-0.466055046,-0.464220183,-0.462385321,-0.460550459,-0.458715596,-0.456880734,
-0.455045872,-0.453211009,-0.451376147,-0.449541284,-0.447706422,-0.44587156,
-0.444036697,-0.442201835,-0.440366972,-0.43853211,-0.436697248,-0.434862385,
-0.433027523,-0.431192661,-0.429357798,-0.427522936,-0.425688073,-0.423853211,
-0.422018349,-0.420183486,-0.418348624,-0.416513761,-0.414678899,-0.412844037,
-0.411009174,-0.409174312,-0.40733945,-0.405504587,-0.403669725,-0.401834862,
-0.4,-0.398165138,-0.396330275,-0.394495413,-0.39266055,-0.390825688,-0.388990826,
-0.387155963,-0.385321101,-0.383486239,-0.381651376,-0.379816514,-0.377981651,
-0.376146789,-0.374311927,-0.372477064,-0.370642202,-0.368807339,-0.366972477,
-0.365137615,-0.363302752,-0.36146789,-0.359633028,-0.357798165,-0.355963303,
-0.35412844,-0.352293578,-0.350458716,-0.348623853,-0.346788991,-0.344954128,
-0.343119266,-0.341284404,-0.339449541,-0.337614679,-0.335779817,-0.333944954,
-0.332110092,-0.330275229,-0.328440367,-0.326605505,-0.324770642,-0.32293578,
-0.321100917,-0.319266055,-0.317431193,-0.31559633,-0.313761468,-0.311926606,
-0.310091743,-0.308256881,-0.306422018,-0.304587156,-0.302752294,-0.300917431,
-0.299082569,-0.297247706,-0.295412844,-0.293577982,-0.291743119,-0.289908257,
-0.288073394,-0.286238532,-0.28440367,-0.282568807,-0.280733945,-0.278899083,
-0.27706422,-0.275229358,-0.273394495,-0.271559633,-0.269724771,-0.267889908,
-0.266055046,-0.264220183,-0.262385321,-0.260550459,-0.258715596,-0.256880734,
-0.255045872,-0.253211009,-0.251376147,-0.249541284,-0.247706422,-0.24587156,
-0.244036697,-0.242201835,-0.240366972,-0.23853211,-0.236697248,-0.234862385,
-0.233027523,-0.231192661,-0.229357798,-0.227522936,-0.225688073,-0.223853211,
-0.222018349,-0.220183486,-0.218348624,-0.216513761,-0.214678899,-0.212844037,
-0.211009174,-0.209174312,-0.20733945,-0.205504587,-0.203669725,-0.201834862,
-0.2,-0.198165138,-0.196330275,-0.194495413,-0.19266055,-0.190825688,-0.188990826,
-0.187155963,-0.185321101,-0.183486239,-0.181651376,-0.179816514,-0.177981651,
-0.176146789,-0.174311927,-0.172477064,-0.170642202,-0.168807339,-0.166972477,
-0.165137615,-0.163302752,-0.16146789,-0.159633028,-0.157798165,-0.155963303,
-0.15412844,-0.152293578,-0.150458716,-0.148623853,-0.146788991,-0.144954128,
-0.143172103),(0.,0.36),.UNSPECIFIED.);
#6238=B_SPLINE_SURFACE_WITH_KNOTS('',5,1,((#192905,#192906),(#192907,#192908),
(#192909,#192910),(#192911,#192912),(#192913,#192914),(#192915,#192916),
(#192917,#192918),(#192919,#192920),(#192921,#192922),(#192923,#192924),
(#192925,#192926),(#192927,#192928),(#192929,#192930),(#192931,#192932),
(#192933,#192934),(#192935,#192936),(#192937,#192938),(#192939,#192940),
(#192941,#192942),(#192943,#192944),(#192945,#192946),(#192947,#192948),
(#192949,#192950),(#192951,#192952),(#192953,#192954),(#192955,#192956),
(#192957,#192958),(#192959,#192960),(#192961,#192962),(#192963,#192964),
(#192965,#192966),(#192967,#192968),(#192969,#192970),(#192971,#192972),
(#192973,#192974),(#192975,#192976),(#192977,#192978),(#192979,#192980),
(#192981,#192982),(#192983,#192984),(#192985,#192986),(#192987,#192988),
(#192989,#192990),(#192991,#192992),(#192993,#192994),(#192995,#192996),
(#192997,#192998),(#192999,#193000),(#193001,#193002),(#193003,#193004),
(#193005,#193006),(#193007,#193008),(#193009,#193010),(#193011,#193012),
(#193013,#193014),(#193015,#193016),(#193017,#193018),(#193019,#193020),
(#193021,#193022),(#193023,#193024),(#193025,#193026),(#193027,#193028),
(#193029,#193030),(#193031,#193032),(#193033,#193034),(#193035,#193036),
(#193037,#193038),(#193039,#193040),(#193041,#193042),(#193043,#193044),
(#193045,#193046),(#193047,#193048),(#193049,#193050),(#193051,#193052),
(#193053,#193054),(#193055,#193056),(#193057,#193058),(#193059,#193060),
(#193061,#193062),(#193063,#193064),(#193065,#193066),(#193067,#193068),
(#193069,#193070),(#193071,#193072),(#193073,#193074),(#193075,#193076),
(#193077,#193078),(#193079,#193080),(#193081,#193082),(#193083,#193084),
(#193085,#193086),(#193087,#193088),(#193089,#193090),(#193091,#193092),
(#193093,#193094),(#193095,#193096),(#193097,#193098),(#193099,#193100),
(#193101,#193102),(#193103,#193104),(#193105,#193106),(#193107,#193108),
(#193109,#193110),(#193111,#193112),(#193113,#193114),(#193115,#193116),
(#193117,#193118),(#193119,#193120),(#193121,#193122),(#193123,#193124),
(#193125,#193126),(#193127,#193128),(#193129,#193130),(#193131,#193132),
(#193133,#193134),(#193135,#193136),(#193137,#193138),(#193139,#193140),
(#193141,#193142),(#193143,#193144),(#193145,#193146),(#193147,#193148),
(#193149,#193150),(#193151,#193152),(#193153,#193154),(#193155,#193156),
(#193157,#193158),(#193159,#193160),(#193161,#193162),(#193163,#193164),
(#193165,#193166),(#193167,#193168),(#193169,#193170),(#193171,#193172),
(#193173,#193174),(#193175,#193176),(#193177,#193178),(#193179,#193180),
(#193181,#193182),(#193183,#193184),(#193185,#193186),(#193187,#193188),
(#193189,#193190),(#193191,#193192),(#193193,#193194),(#193195,#193196),
(#193197,#193198),(#193199,#193200),(#193201,#193202),(#193203,#193204),
(#193205,#193206),(#193207,#193208),(#193209,#193210),(#193211,#193212),
(#193213,#193214),(#193215,#193216),(#193217,#193218),(#193219,#193220),
(#193221,#193222),(#193223,#193224),(#193225,#193226),(#193227,#193228),
(#193229,#193230),(#193231,#193232),(#193233,#193234),(#193235,#193236),
(#193237,#193238),(#193239,#193240),(#193241,#193242),(#193243,#193244),
(#193245,#193246),(#193247,#193248),(#193249,#193250),(#193251,#193252),
(#193253,#193254),(#193255,#193256),(#193257,#193258),(#193259,#193260),
(#193261,#193262),(#193263,#193264),(#193265,#193266),(#193267,#193268),
(#193269,#193270),(#193271,#193272),(#193273,#193274),(#193275,#193276),
(#193277,#193278),(#193279,#193280),(#193281,#193282),(#193283,#193284),
(#193285,#193286),(#193287,#193288),(#193289,#193290),(#193291,#193292),
(#193293,#193294),(#193295,#193296),(#193297,#193298),(#193299,#193300),
(#193301,#193302),(#193303,#193304),(#193305,#193306),(#193307,#193308),
(#193309,#193310),(#193311,#193312),(#193313,#193314),(#193315,#193316),
(#193317,#193318),(#193319,#193320),(#193321,#193322),(#193323,#193324),
(#193325,#193326),(#193327,#193328),(#193329,#193330),(#193331,#193332),
(#193333,#193334),(#193335,#193336),(#193337,#193338),(#193339,#193340),
(#193341,#193342),(#193343,#193344),(#193345,#193346),(#193347,#193348),
(#193349,#193350),(#193351,#193352),(#193353,#193354),(#193355,#193356),
(#193357,#193358),(#193359,#193360),(#193361,#193362),(#193363,#193364),
(#193365,#193366),(#193367,#193368),(#193369,#193370),(#193371,#193372),
(#193373,#193374),(#193375,#193376),(#193377,#193378),(#193379,#193380),
(#193381,#193382),(#193383,#193384),(#193385,#193386),(#193387,#193388),
(#193389,#193390),(#193391,#193392),(#193393,#193394),(#193395,#193396),
(#193397,#193398),(#193399,#193400),(#193401,#193402),(#193403,#193404),
(#193405,#193406),(#193407,#193408),(#193409,#193410),(#193411,#193412),
(#193413,#193414),(#193415,#193416),(#193417,#193418),(#193419,#193420),
(#193421,#193422),(#193423,#193424),(#193425,#193426),(#193427,#193428),
(#193429,#193430),(#193431,#193432),(#193433,#193434),(#193435,#193436),
(#193437,#193438),(#193439,#193440),(#193441,#193442),(#193443,#193444),
(#193445,#193446),(#193447,#193448),(#193449,#193450),(#193451,#193452),
(#193453,#193454),(#193455,#193456),(#193457,#193458),(#193459,#193460),
(#193461,#193462),(#193463,#193464),(#193465,#193466),(#193467,#193468),
(#193469,#193470),(#193471,#193472),(#193473,#193474),(#193475,#193476),
(#193477,#193478),(#193479,#193480),(#193481,#193482),(#193483,#193484),
(#193485,#193486),(#193487,#193488),(#193489,#193490),(#193491,#193492),
(#193493,#193494),(#193495,#193496),(#193497,#193498),(#193499,#193500),
(#193501,#193502),(#193503,#193504),(#193505,#193506),(#193507,#193508),
(#193509,#193510),(#193511,#193512),(#193513,#193514),(#193515,#193516),
(#193517,#193518),(#193519,#193520),(#193521,#193522),(#193523,#193524),
(#193525,#193526),(#193527,#193528),(#193529,#193530),(#193531,#193532),
(#193533,#193534),(#193535,#193536),(#193537,#193538),(#193539,#193540),
(#193541,#193542),(#193543,#193544),(#193545,#193546),(#193547,#193548),
(#193549,#193550),(#193551,#193552),(#193553,#193554),(#193555,#193556),
(#193557,#193558),(#193559,#193560),(#193561,#193562),(#193563,#193564),
(#193565,#193566),(#193567,#193568),(#193569,#193570),(#193571,#193572),
(#193573,#193574),(#193575,#193576),(#193577,#193578),(#193579,#193580),
(#193581,#193582),(#193583,#193584),(#193585,#193586),(#193587,#193588),
(#193589,#193590),(#193591,#193592),(#193593,#193594),(#193595,#193596),
(#193597,#193598),(#193599,#193600),(#193601,#193602),(#193603,#193604),
(#193605,#193606),(#193607,#193608),(#193609,#193610),(#193611,#193612),
(#193613,#193614),(#193615,#193616),(#193617,#193618),(#193619,#193620),
(#193621,#193622),(#193623,#193624),(#193625,#193626),(#193627,#193628),
(#193629,#193630),(#193631,#193632),(#193633,#193634),(#193635,#193636),
(#193637,#193638),(#193639,#193640),(#193641,#193642),(#193643,#193644),
(#193645,#193646),(#193647,#193648),(#193649,#193650),(#193651,#193652),
(#193653,#193654),(#193655,#193656),(#193657,#193658),(#193659,#193660),
(#193661,#193662),(#193663,#193664),(#193665,#193666),(#193667,#193668),
(#193669,#193670),(#193671,#193672),(#193673,#193674),(#193675,#193676),
(#193677,#193678),(#193679,#193680),(#193681,#193682),(#193683,#193684),
(#193685,#193686),(#193687,#193688),(#193689,#193690),(#193691,#193692),
(#193693,#193694),(#193695,#193696),(#193697,#193698),(#193699,#193700),
(#193701,#193702),(#193703,#193704),(#193705,#193706),(#193707,#193708),
(#193709,#193710),(#193711,#193712),(#193713,#193714),(#193715,#193716),
(#193717,#193718),(#193719,#193720),(#193721,#193722),(#193723,#193724),
(#193725,#193726),(#193727,#193728),(#193729,#193730),(#193731,#193732),
(#193733,#193734),(#193735,#193736),(#193737,#193738),(#193739,#193740),
(#193741,#193742),(#193743,#193744),(#193745,#193746),(#193747,#193748),
(#193749,#193750),(#193751,#193752),(#193753,#193754),(#193755,#193756),
(#193757,#193758),(#193759,#193760),(#193761,#193762),(#193763,#193764),
(#193765,#193766),(#193767,#193768),(#193769,#193770),(#193771,#193772),
(#193773,#193774),(#193775,#193776),(#193777,#193778),(#193779,#193780),
(#193781,#193782),(#193783,#193784),(#193785,#193786),(#193787,#193788),
(#193789,#193790),(#193791,#193792),(#193793,#193794),(#193795,#193796),
(#193797,#193798),(#193799,#193800),(#193801,#193802),(#193803,#193804),
(#193805,#193806),(#193807,#193808),(#193809,#193810),(#193811,#193812),
(#193813,#193814),(#193815,#193816),(#193817,#193818),(#193819,#193820),
(#193821,#193822),(#193823,#193824),(#193825,#193826),(#193827,#193828),
(#193829,#193830),(#193831,#193832),(#193833,#193834),(#193835,#193836),
(#193837,#193838),(#193839,#193840),(#193841,#193842),(#193843,#193844),
(#193845,#193846),(#193847,#193848)),.UNSPECIFIED.,.F.,.F.,.F.,(6,1,1,1,
1,1,1,1,1,1,1,1,1,1,1,1,1,1,1,1,1,1,1,1,1,1,1,1,1,1,1,1,1,1,1,1,1,1,1,1,
1,1,1,1,1,1,1,1,1,1,1,1,1,1,1,1,1,1,1,1,1,1,1,1,1,1,1,1,1,1,1,1,1,1,1,1,
1,1,1,1,1,1,1,1,1,1,1,1,1,1,1,1,1,1,1,1,1,1,1,1,1,1,1,1,1,1,1,1,1,1,1,1,
1,1,1,1,1,1,1,1,1,1,1,1,1,1,1,1,1,1,1,1,1,1,1,1,1,1,1,1,1,1,1,1,1,1,1,1,
1,1,1,1,1,1,1,1,1,1,1,1,1,1,1,1,1,1,1,1,1,1,1,1,1,1,1,1,1,1,1,1,1,1,1,1,
1,1,1,1,1,1,1,1,1,1,1,1,1,1,1,1,1,1,1,1,1,1,1,1,1,1,1,1,1,1,1,1,1,1,1,1,
1,1,1,1,1,1,1,1,1,1,1,1,1,1,1,1,1,1,1,1,1,1,1,1,1,1,1,1,1,1,1,1,1,1,1,1,
1,1,1,1,1,1,1,1,1,1,1,1,1,1,1,1,1,1,1,1,1,1,1,1,1,1,1,1,1,1,1,1,1,1,1,1,
1,1,1,1,1,1,1,1,1,1,1,1,1,1,1,1,1,1,1,1,1,1,1,1,1,1,1,1,1,1,1,1,1,1,1,1,
1,1,1,1,1,1,1,1,1,1,1,1,1,1,1,1,1,1,1,1,1,1,1,1,1,1,1,1,1,1,1,1,1,1,1,1,
1,1,1,1,1,1,1,1,1,1,1,1,1,1,1,1,1,1,1,1,1,1,1,1,1,1,1,1,1,1,1,1,1,1,1,1,
1,1,1,1,1,1,1,1,1,1,1,1,1,1,1,1,1,1,1,1,1,1,1,1,1,1,1,1,1,1,1,1,1,1,1,1,
1,1,1,1,1,1,1,1,1,1,1,1,1,1,1,1,1,1,1,1,1,1,1,1,1,1,1,1,1,1,1,6),(2,2),
(0.143172103,0.144954128,0.146788991,0.148623853,0.150458716,0.152293578,
0.15412844,0.155963303,0.157798165,0.159633028,0.16146789,0.163302752,0.165137615,
0.166972477,0.168807339,0.170642202,0.172477064,0.174311927,0.176146789,
0.177981651,0.179816514,0.181651376,0.183486239,0.185321101,0.187155963,
0.188990826,0.190825688,0.19266055,0.194495413,0.196330275,0.198165138,
0.2,0.201834862,0.203669725,0.205504587,0.20733945,0.209174312,0.211009174,
0.212844037,0.214678899,0.216513761,0.218348624,0.220183486,0.222018349,
0.223853211,0.225688073,0.227522936,0.229357798,0.231192661,0.233027523,
0.234862385,0.236697248,0.23853211,0.240366972,0.242201835,0.244036697,
0.24587156,0.247706422,0.249541284,0.251376147,0.253211009,0.255045872,
0.256880734,0.258715596,0.260550459,0.262385321,0.264220183,0.266055046,
0.267889908,0.269724771,0.271559633,0.273394495,0.275229358,0.27706422,
0.278899083,0.280733945,0.282568807,0.28440367,0.286238532,0.288073394,
0.289908257,0.291743119,0.293577982,0.295412844,0.297247706,0.299082569,
0.300917431,0.302752294,0.304587156,0.306422018,0.308256881,0.310091743,
0.311926606,0.313761468,0.31559633,0.317431193,0.319266055,0.321100917,
0.32293578,0.324770642,0.326605505,0.328440367,0.330275229,0.332110092,
0.333944954,0.335779817,0.337614679,0.339449541,0.341284404,0.343119266,
0.344954128,0.346788991,0.348623853,0.350458716,0.352293578,0.35412844,
0.355963303,0.357798165,0.359633028,0.36146789,0.363302752,0.365137615,
0.366972477,0.368807339,0.370642202,0.372477064,0.374311927,0.376146789,
0.377981651,0.379816514,0.381651376,0.383486239,0.385321101,0.387155963,
0.388990826,0.390825688,0.39266055,0.394495413,0.396330275,0.398165138,
0.4,0.401834862,0.403669725,0.405504587,0.40733945,0.409174312,0.411009174,
0.412844037,0.414678899,0.416513761,0.418348624,0.420183486,0.422018349,
0.423853211,0.425688073,0.427522936,0.429357798,0.431192661,0.433027523,
0.434862385,0.436697248,0.43853211,0.440366972,0.442201835,0.444036697,
0.44587156,0.447706422,0.449541284,0.451376147,0.453211009,0.455045872,
0.456880734,0.458715596,0.460550459,0.462385321,0.464220183,0.466055046,
0.467889908,0.469724771,0.471559633,0.473394495,0.475229358,0.47706422,
0.478899083,0.480733945,0.482568807,0.48440367,0.486238532,0.488073394,
0.489908257,0.491743119,0.493577982,0.495412844,0.497247706,0.499082569,
0.500917431,0.502752294,0.504587156,0.506422018,0.508256881,0.510091743,
0.511926606,0.513761468,0.51559633,0.517431193,0.519266055,0.521100917,
0.52293578,0.524770642,0.526605505,0.528440367,0.530275229,0.532110092,
0.533944954,0.535779817,0.537614679,0.539449541,0.541284404,0.543119266,
0.544954128,0.546788991,0.548623853,0.550458716,0.552293578,0.55412844,
0.555963303,0.557798165,0.559633028,0.56146789,0.563302752,0.565137615,
0.566972477,0.568807339,0.570642202,0.572477064,0.574311927,0.576146789,
0.577981651,0.579816514,0.581651376,0.583486239,0.585321101,0.587155963,
0.588990826,0.590825688,0.59266055,0.594495413,0.596330275,0.598165138,
0.6,0.601834862,0.603669725,0.605504587,0.60733945,0.609174312,0.611009174,
0.612844037,0.614678899,0.616513761,0.618348624,0.620183486,0.622018349,
0.623853211,0.625688073,0.627522936,0.629357798,0.631192661,0.633027523,
0.634862385,0.636697248,0.63853211,0.640366972,0.642201835,0.644036697,
0.64587156,0.647706422,0.649541284,0.651376147,0.653211009,0.655045872,
0.656880734,0.658715596,0.660550459,0.662385321,0.664220183,0.666055046,
0.667889908,0.669724771,0.671559633,0.673394495,0.675229358,0.67706422,
0.678899083,0.680733945,0.682568807,0.68440367,0.686238532,0.688073394,
0.689908257,0.691743119,0.693577982,0.695412844,0.697247706,0.699082569,
0.700917431,0.702752294,0.704587156,0.706422018,0.708256881,0.710091743,
0.711926606,0.713761468,0.71559633,0.717431193,0.719266055,0.721100917,
0.72293578,0.724770642,0.726605505,0.728440367,0.730275229,0.732110092,
0.733944954,0.735779817,0.737614679,0.739449541,0.741284404,0.743119266,
0.744954128,0.746788991,0.748623853,0.750458716,0.752293578,0.75412844,
0.755963303,0.757798165,0.759633028,0.76146789,0.763302752,0.765137615,
0.766972477,0.768807339,0.770642202,0.772477064,0.774311927,0.776146789,
0.777981651,0.779816514,0.781651376,0.783486239,0.785321101,0.787155963,
0.788990826,0.790825688,0.79266055,0.794495413,0.796330275,0.798165138,
0.8,0.801834862,0.803669725,0.805504587,0.80733945,0.809174312,0.811009174,
0.812844037,0.814678899,0.816513761,0.818348624,0.820183486,0.822018349,
0.823853211,0.825688073,0.827522936,0.829357798,0.831192661,0.833027523,
0.834862385,0.836697248,0.83853211,0.840366972,0.842201835,0.844036697,
0.84587156,0.847706422,0.849541284,0.851376147,0.853211009,0.855045872,
0.856880734,0.858715596,0.860550459,0.862385321,0.864220183,0.866055046,
0.867889908,0.869724771,0.871559633,0.873394495,0.875229358,0.87706422,
0.878899083,0.880733945,0.882568807,0.88440367,0.886238532,0.888073394,
0.889908257,0.891743119,0.893577982,0.895412844,0.897247706,0.899082569,
0.900917431,0.902752294,0.904587156,0.906422018,0.908256881,0.910091743,
0.911926606,0.913761468,0.91559633,0.917431193,0.919266055,0.921100917,
0.92293578,0.924770642,0.926605505,0.928440367,0.930275229,0.932110092,
0.933944954,0.935779817,0.937614679,0.939449541,0.941284404,0.943119266,
0.944954128,0.946788991,0.948623853,0.950458716,0.952293578,0.95412844,
0.955963303,0.957798165,0.959633028,0.96146789,0.963302752,0.965137615,
0.966972477,0.968807339,0.970642202,0.972477064,0.974311927,0.976146789,
0.977981651,0.979816514,0.981651376,0.983486239,0.985321101,0.987155963,
0.988990826,0.990825688,0.99266055,0.994495413,0.996330275,0.998165138,
1.),(0.,0.36),.UNSPECIFIED.);
#6239=B_SPLINE_SURFACE_WITH_KNOTS('',5,1,((#194484,#194485),(#194486,#194487),
(#194488,#194489),(#194490,#194491),(#194492,#194493),(#194494,#194495),
(#194496,#194497),(#194498,#194499),(#194500,#194501),(#194502,#194503),
(#194504,#194505),(#194506,#194507),(#194508,#194509),(#194510,#194511),
(#194512,#194513),(#194514,#194515),(#194516,#194517),(#194518,#194519),
(#194520,#194521),(#194522,#194523),(#194524,#194525),(#194526,#194527),
(#194528,#194529),(#194530,#194531),(#194532,#194533),(#194534,#194535),
(#194536,#194537),(#194538,#194539),(#194540,#194541),(#194542,#194543),
(#194544,#194545),(#194546,#194547),(#194548,#194549),(#194550,#194551),
(#194552,#194553),(#194554,#194555),(#194556,#194557),(#194558,#194559),
(#194560,#194561),(#194562,#194563),(#194564,#194565),(#194566,#194567),
(#194568,#194569),(#194570,#194571),(#194572,#194573),(#194574,#194575),
(#194576,#194577),(#194578,#194579),(#194580,#194581),(#194582,#194583),
(#194584,#194585),(#194586,#194587),(#194588,#194589),(#194590,#194591),
(#194592,#194593),(#194594,#194595),(#194596,#194597),(#194598,#194599),
(#194600,#194601),(#194602,#194603),(#194604,#194605),(#194606,#194607),
(#194608,#194609),(#194610,#194611),(#194612,#194613),(#194614,#194615),
(#194616,#194617),(#194618,#194619),(#194620,#194621),(#194622,#194623),
(#194624,#194625),(#194626,#194627),(#194628,#194629),(#194630,#194631),
(#194632,#194633),(#194634,#194635),(#194636,#194637),(#194638,#194639),
(#194640,#194641),(#194642,#194643),(#194644,#194645),(#194646,#194647),
(#194648,#194649),(#194650,#194651),(#194652,#194653),(#194654,#194655),
(#194656,#194657),(#194658,#194659),(#194660,#194661),(#194662,#194663),
(#194664,#194665),(#194666,#194667),(#194668,#194669),(#194670,#194671),
(#194672,#194673),(#194674,#194675),(#194676,#194677),(#194678,#194679),
(#194680,#194681),(#194682,#194683),(#194684,#194685),(#194686,#194687),
(#194688,#194689),(#194690,#194691),(#194692,#194693),(#194694,#194695),
(#194696,#194697),(#194698,#194699),(#194700,#194701),(#194702,#194703),
(#194704,#194705),(#194706,#194707),(#194708,#194709),(#194710,#194711),
(#194712,#194713),(#194714,#194715),(#194716,#194717),(#194718,#194719),
(#194720,#194721),(#194722,#194723),(#194724,#194725),(#194726,#194727),
(#194728,#194729),(#194730,#194731),(#194732,#194733),(#194734,#194735),
(#194736,#194737),(#194738,#194739),(#194740,#194741),(#194742,#194743),
(#194744,#194745),(#194746,#194747),(#194748,#194749),(#194750,#194751),
(#194752,#194753),(#194754,#194755),(#194756,#194757),(#194758,#194759),
(#194760,#194761),(#194762,#194763),(#194764,#194765),(#194766,#194767),
(#194768,#194769),(#194770,#194771),(#194772,#194773),(#194774,#194775),
(#194776,#194777),(#194778,#194779),(#194780,#194781),(#194782,#194783),
(#194784,#194785),(#194786,#194787),(#194788,#194789),(#194790,#194791),
(#194792,#194793),(#194794,#194795),(#194796,#194797),(#194798,#194799),
(#194800,#194801),(#194802,#194803),(#194804,#194805),(#194806,#194807),
(#194808,#194809),(#194810,#194811),(#194812,#194813),(#194814,#194815),
(#194816,#194817),(#194818,#194819),(#194820,#194821),(#194822,#194823),
(#194824,#194825),(#194826,#194827),(#194828,#194829),(#194830,#194831),
(#194832,#194833),(#194834,#194835),(#194836,#194837),(#194838,#194839),
(#194840,#194841),(#194842,#194843),(#194844,#194845),(#194846,#194847),
(#194848,#194849),(#194850,#194851),(#194852,#194853),(#194854,#194855),
(#194856,#194857),(#194858,#194859),(#194860,#194861),(#194862,#194863),
(#194864,#194865),(#194866,#194867),(#194868,#194869),(#194870,#194871),
(#194872,#194873),(#194874,#194875),(#194876,#194877),(#194878,#194879),
(#194880,#194881),(#194882,#194883),(#194884,#194885),(#194886,#194887),
(#194888,#194889),(#194890,#194891),(#194892,#194893),(#194894,#194895),
(#194896,#194897),(#194898,#194899),(#194900,#194901),(#194902,#194903),
(#194904,#194905),(#194906,#194907),(#194908,#194909),(#194910,#194911),
(#194912,#194913),(#194914,#194915),(#194916,#194917),(#194918,#194919),
(#194920,#194921),(#194922,#194923),(#194924,#194925),(#194926,#194927),
(#194928,#194929),(#194930,#194931),(#194932,#194933),(#194934,#194935),
(#194936,#194937),(#194938,#194939),(#194940,#194941),(#194942,#194943),
(#194944,#194945),(#194946,#194947),(#194948,#194949),(#194950,#194951),
(#194952,#194953),(#194954,#194955),(#194956,#194957),(#194958,#194959),
(#194960,#194961),(#194962,#194963),(#194964,#194965),(#194966,#194967),
(#194968,#194969),(#194970,#194971),(#194972,#194973),(#194974,#194975),
(#194976,#194977),(#194978,#194979),(#194980,#194981),(#194982,#194983),
(#194984,#194985),(#194986,#194987),(#194988,#194989),(#194990,#194991),
(#194992,#194993),(#194994,#194995),(#194996,#194997),(#194998,#194999),
(#195000,#195001),(#195002,#195003),(#195004,#195005),(#195006,#195007),
(#195008,#195009),(#195010,#195011),(#195012,#195013),(#195014,#195015),
(#195016,#195017),(#195018,#195019),(#195020,#195021),(#195022,#195023),
(#195024,#195025),(#195026,#195027),(#195028,#195029),(#195030,#195031),
(#195032,#195033),(#195034,#195035),(#195036,#195037),(#195038,#195039),
(#195040,#195041),(#195042,#195043),(#195044,#195045),(#195046,#195047),
(#195048,#195049),(#195050,#195051),(#195052,#195053),(#195054,#195055),
(#195056,#195057),(#195058,#195059),(#195060,#195061),(#195062,#195063),
(#195064,#195065),(#195066,#195067),(#195068,#195069),(#195070,#195071),
(#195072,#195073),(#195074,#195075),(#195076,#195077),(#195078,#195079),
(#195080,#195081),(#195082,#195083),(#195084,#195085),(#195086,#195087),
(#195088,#195089),(#195090,#195091),(#195092,#195093),(#195094,#195095),
(#195096,#195097),(#195098,#195099),(#195100,#195101),(#195102,#195103),
(#195104,#195105),(#195106,#195107),(#195108,#195109),(#195110,#195111),
(#195112,#195113),(#195114,#195115),(#195116,#195117),(#195118,#195119),
(#195120,#195121),(#195122,#195123),(#195124,#195125),(#195126,#195127),
(#195128,#195129),(#195130,#195131),(#195132,#195133),(#195134,#195135),
(#195136,#195137),(#195138,#195139),(#195140,#195141),(#195142,#195143),
(#195144,#195145),(#195146,#195147),(#195148,#195149),(#195150,#195151),
(#195152,#195153),(#195154,#195155),(#195156,#195157),(#195158,#195159),
(#195160,#195161),(#195162,#195163),(#195164,#195165),(#195166,#195167),
(#195168,#195169),(#195170,#195171),(#195172,#195173),(#195174,#195175),
(#195176,#195177),(#195178,#195179),(#195180,#195181),(#195182,#195183),
(#195184,#195185),(#195186,#195187),(#195188,#195189),(#195190,#195191),
(#195192,#195193),(#195194,#195195),(#195196,#195197),(#195198,#195199),
(#195200,#195201),(#195202,#195203),(#195204,#195205),(#195206,#195207),
(#195208,#195209),(#195210,#195211),(#195212,#195213),(#195214,#195215),
(#195216,#195217),(#195218,#195219),(#195220,#195221),(#195222,#195223),
(#195224,#195225),(#195226,#195227),(#195228,#195229),(#195230,#195231),
(#195232,#195233),(#195234,#195235),(#195236,#195237),(#195238,#195239),
(#195240,#195241),(#195242,#195243),(#195244,#195245),(#195246,#195247),
(#195248,#195249),(#195250,#195251),(#195252,#195253),(#195254,#195255),
(#195256,#195257),(#195258,#195259),(#195260,#195261),(#195262,#195263),
(#195264,#195265),(#195266,#195267),(#195268,#195269),(#195270,#195271),
(#195272,#195273),(#195274,#195275),(#195276,#195277),(#195278,#195279),
(#195280,#195281),(#195282,#195283),(#195284,#195285),(#195286,#195287),
(#195288,#195289),(#195290,#195291),(#195292,#195293),(#195294,#195295),
(#195296,#195297),(#195298,#195299),(#195300,#195301),(#195302,#195303),
(#195304,#195305),(#195306,#195307),(#195308,#195309),(#195310,#195311),
(#195312,#195313),(#195314,#195315),(#195316,#195317),(#195318,#195319),
(#195320,#195321),(#195322,#195323),(#195324,#195325),(#195326,#195327),
(#195328,#195329),(#195330,#195331),(#195332,#195333),(#195334,#195335),
(#195336,#195337),(#195338,#195339),(#195340,#195341),(#195342,#195343),
(#195344,#195345),(#195346,#195347),(#195348,#195349),(#195350,#195351),
(#195352,#195353),(#195354,#195355),(#195356,#195357),(#195358,#195359),
(#195360,#195361),(#195362,#195363),(#195364,#195365),(#195366,#195367),
(#195368,#195369),(#195370,#195371),(#195372,#195373),(#195374,#195375),
(#195376,#195377),(#195378,#195379),(#195380,#195381),(#195382,#195383),
(#195384,#195385),(#195386,#195387),(#195388,#195389),(#195390,#195391),
(#195392,#195393),(#195394,#195395),(#195396,#195397),(#195398,#195399),
(#195400,#195401),(#195402,#195403),(#195404,#195405),(#195406,#195407),
(#195408,#195409),(#195410,#195411),(#195412,#195413),(#195414,#195415),
(#195416,#195417),(#195418,#195419),(#195420,#195421),(#195422,#195423),
(#195424,#195425),(#195426,#195427)),.UNSPECIFIED.,.F.,.F.,.F.,(6,1,1,1,
1,1,1,1,1,1,1,1,1,1,1,1,1,1,1,1,1,1,1,1,1,1,1,1,1,1,1,1,1,1,1,1,1,1,1,1,
1,1,1,1,1,1,1,1,1,1,1,1,1,1,1,1,1,1,1,1,1,1,1,1,1,1,1,1,1,1,1,1,1,1,1,1,
1,1,1,1,1,1,1,1,1,1,1,1,1,1,1,1,1,1,1,1,1,1,1,1,1,1,1,1,1,1,1,1,1,1,1,1,
1,1,1,1,1,1,1,1,1,1,1,1,1,1,1,1,1,1,1,1,1,1,1,1,1,1,1,1,1,1,1,1,1,1,1,1,
1,1,1,1,1,1,1,1,1,1,1,1,1,1,1,1,1,1,1,1,1,1,1,1,1,1,1,1,1,1,1,1,1,1,1,1,
1,1,1,1,1,1,1,1,1,1,1,1,1,1,1,1,1,1,1,1,1,1,1,1,1,1,1,1,1,1,1,1,1,1,1,1,
1,1,1,1,1,1,1,1,1,1,1,1,1,1,1,1,1,1,1,1,1,1,1,1,1,1,1,1,1,1,1,1,1,1,1,1,
1,1,1,1,1,1,1,1,1,1,1,1,1,1,1,1,1,1,1,1,1,1,1,1,1,1,1,1,1,1,1,1,1,1,1,1,
1,1,1,1,1,1,1,1,1,1,1,1,1,1,1,1,1,1,1,1,1,1,1,1,1,1,1,1,1,1,1,1,1,1,1,1,
1,1,1,1,1,1,1,1,1,1,1,1,1,1,1,1,1,1,1,1,1,1,1,1,1,1,1,1,1,1,1,1,1,1,1,1,
1,1,1,1,1,1,1,1,1,1,1,1,1,1,1,1,1,1,1,1,1,1,1,1,1,1,1,1,1,1,1,1,1,1,1,1,
1,1,1,1,1,1,1,1,1,1,1,1,1,1,1,1,1,1,1,1,1,1,1,1,1,1,1,1,1,1,1,1,1,1,1,1,
1,1,1,1,1,1,1,1,1,1,1,1,1,1,1,1,1,1,1,1,1,1,1,1,1,1,1,1,1,1,1,6),(2,2),
(0.143172103,0.144954128,0.146788991,0.148623853,0.150458716,0.152293578,
0.15412844,0.155963303,0.157798165,0.159633028,0.16146789,0.163302752,0.165137615,
0.166972477,0.168807339,0.170642202,0.172477064,0.174311927,0.176146789,
0.177981651,0.179816514,0.181651376,0.183486239,0.185321101,0.187155963,
0.188990826,0.190825688,0.19266055,0.194495413,0.196330275,0.198165138,
0.2,0.201834862,0.203669725,0.205504587,0.20733945,0.209174312,0.211009174,
0.212844037,0.214678899,0.216513761,0.218348624,0.220183486,0.222018349,
0.223853211,0.225688073,0.227522936,0.229357798,0.231192661,0.233027523,
0.234862385,0.236697248,0.23853211,0.240366972,0.242201835,0.244036697,
0.24587156,0.247706422,0.249541284,0.251376147,0.253211009,0.255045872,
0.256880734,0.258715596,0.260550459,0.262385321,0.264220183,0.266055046,
0.267889908,0.269724771,0.271559633,0.273394495,0.275229358,0.27706422,
0.278899083,0.280733945,0.282568807,0.28440367,0.286238532,0.288073394,
0.289908257,0.291743119,0.293577982,0.295412844,0.297247706,0.299082569,
0.300917431,0.302752294,0.304587156,0.306422018,0.308256881,0.310091743,
0.311926606,0.313761468,0.31559633,0.317431193,0.319266055,0.321100917,
0.32293578,0.324770642,0.326605505,0.328440367,0.330275229,0.332110092,
0.333944954,0.335779817,0.337614679,0.339449541,0.341284404,0.343119266,
0.344954128,0.346788991,0.348623853,0.350458716,0.352293578,0.35412844,
0.355963303,0.357798165,0.359633028,0.36146789,0.363302752,0.365137615,
0.366972477,0.368807339,0.370642202,0.372477064,0.374311927,0.376146789,
0.377981651,0.379816514,0.381651376,0.383486239,0.385321101,0.387155963,
0.388990826,0.390825688,0.39266055,0.394495413,0.396330275,0.398165138,
0.4,0.401834862,0.403669725,0.405504587,0.40733945,0.409174312,0.411009174,
0.412844037,0.414678899,0.416513761,0.418348624,0.420183486,0.422018349,
0.423853211,0.425688073,0.427522936,0.429357798,0.431192661,0.433027523,
0.434862385,0.436697248,0.43853211,0.440366972,0.442201835,0.444036697,
0.44587156,0.447706422,0.449541284,0.451376147,0.453211009,0.455045872,
0.456880734,0.458715596,0.460550459,0.462385321,0.464220183,0.466055046,
0.467889908,0.469724771,0.471559633,0.473394495,0.475229358,0.47706422,
0.478899083,0.480733945,0.482568807,0.48440367,0.486238532,0.488073394,
0.489908257,0.491743119,0.493577982,0.495412844,0.497247706,0.499082569,
0.500917431,0.502752294,0.504587156,0.506422018,0.508256881,0.510091743,
0.511926606,0.513761468,0.51559633,0.517431193,0.519266055,0.521100917,
0.52293578,0.524770642,0.526605505,0.528440367,0.530275229,0.532110092,
0.533944954,0.535779817,0.537614679,0.539449541,0.541284404,0.543119266,
0.544954128,0.546788991,0.548623853,0.550458716,0.552293578,0.55412844,
0.555963303,0.557798165,0.559633028,0.56146789,0.563302752,0.565137615,
0.566972477,0.568807339,0.570642202,0.572477064,0.574311927,0.576146789,
0.577981651,0.579816514,0.581651376,0.583486239,0.585321101,0.587155963,
0.588990826,0.590825688,0.59266055,0.594495413,0.596330275,0.598165138,
0.6,0.601834862,0.603669725,0.605504587,0.60733945,0.609174312,0.611009174,
0.612844037,0.614678899,0.616513761,0.618348624,0.620183486,0.622018349,
0.623853211,0.625688073,0.627522936,0.629357798,0.631192661,0.633027523,
0.634862385,0.636697248,0.63853211,0.640366972,0.642201835,0.644036697,
0.64587156,0.647706422,0.649541284,0.651376147,0.653211009,0.655045872,
0.656880734,0.658715596,0.660550459,0.662385321,0.664220183,0.666055046,
0.667889908,0.669724771,0.671559633,0.673394495,0.675229358,0.67706422,
0.678899083,0.680733945,0.682568807,0.68440367,0.686238532,0.688073394,
0.689908257,0.691743119,0.693577982,0.695412844,0.697247706,0.699082569,
0.700917431,0.702752294,0.704587156,0.706422018,0.708256881,0.710091743,
0.711926606,0.713761468,0.71559633,0.717431193,0.719266055,0.721100917,
0.72293578,0.724770642,0.726605505,0.728440367,0.730275229,0.732110092,
0.733944954,0.735779817,0.737614679,0.739449541,0.741284404,0.743119266,
0.744954128,0.746788991,0.748623853,0.750458716,0.752293578,0.75412844,
0.755963303,0.757798165,0.759633028,0.76146789,0.763302752,0.765137615,
0.766972477,0.768807339,0.770642202,0.772477064,0.774311927,0.776146789,
0.777981651,0.779816514,0.781651376,0.783486239,0.785321101,0.787155963,
0.788990826,0.790825688,0.79266055,0.794495413,0.796330275,0.798165138,
0.8,0.801834862,0.803669725,0.805504587,0.80733945,0.809174312,0.811009174,
0.812844037,0.814678899,0.816513761,0.818348624,0.820183486,0.822018349,
0.823853211,0.825688073,0.827522936,0.829357798,0.831192661,0.833027523,
0.834862385,0.836697248,0.83853211,0.840366972,0.842201835,0.844036697,
0.84587156,0.847706422,0.849541284,0.851376147,0.853211009,0.855045872,
0.856880734,0.858715596,0.860550459,0.862385321,0.864220183,0.866055046,
0.867889908,0.869724771,0.871559633,0.873394495,0.875229358,0.87706422,
0.878899083,0.880733945,0.882568807,0.88440367,0.886238532,0.888073394,
0.889908257,0.891743119,0.893577982,0.895412844,0.897247706,0.899082569,
0.900917431,0.902752294,0.904587156,0.906422018,0.908256881,0.910091743,
0.911926606,0.913761468,0.91559633,0.917431193,0.919266055,0.921100917,
0.92293578,0.924770642,0.926605505,0.928440367,0.930275229,0.932110092,
0.933944954,0.935779817,0.937614679,0.939449541,0.941284404,0.943119266,
0.944954128,0.946788991,0.948623853,0.950458716,0.952293578,0.95412844,
0.955963303,0.957798165,0.959633028,0.96146789,0.963302752,0.965137615,
0.966972477,0.968807339,0.970642202,0.972477064,0.974311927,0.976146789,
0.977981651,0.979816514,0.981651376,0.983486239,0.985321101,0.987155963,
0.988990826,0.990825688,0.99266055,0.994495413,0.996330275,0.998165138,
1.),(0.,0.36),.UNSPECIFIED.);
#6240=B_SPLINE_SURFACE_WITH_KNOTS('',5,1,((#196054,#196055),(#196056,#196057),
(#196058,#196059),(#196060,#196061),(#196062,#196063),(#196064,#196065),
(#196066,#196067),(#196068,#196069),(#196070,#196071),(#196072,#196073),
(#196074,#196075),(#196076,#196077),(#196078,#196079),(#196080,#196081),
(#196082,#196083),(#196084,#196085),(#196086,#196087),(#196088,#196089),
(#196090,#196091),(#196092,#196093),(#196094,#196095),(#196096,#196097),
(#196098,#196099),(#196100,#196101),(#196102,#196103),(#196104,#196105),
(#196106,#196107),(#196108,#196109),(#196110,#196111),(#196112,#196113),
(#196114,#196115),(#196116,#196117),(#196118,#196119),(#196120,#196121),
(#196122,#196123),(#196124,#196125),(#196126,#196127),(#196128,#196129),
(#196130,#196131),(#196132,#196133),(#196134,#196135),(#196136,#196137),
(#196138,#196139),(#196140,#196141),(#196142,#196143),(#196144,#196145),
(#196146,#196147),(#196148,#196149),(#196150,#196151),(#196152,#196153),
(#196154,#196155),(#196156,#196157),(#196158,#196159),(#196160,#196161),
(#196162,#196163),(#196164,#196165),(#196166,#196167),(#196168,#196169),
(#196170,#196171),(#196172,#196173),(#196174,#196175),(#196176,#196177),
(#196178,#196179),(#196180,#196181),(#196182,#196183),(#196184,#196185),
(#196186,#196187),(#196188,#196189),(#196190,#196191),(#196192,#196193),
(#196194,#196195),(#196196,#196197),(#196198,#196199),(#196200,#196201),
(#196202,#196203),(#196204,#196205),(#196206,#196207),(#196208,#196209),
(#196210,#196211),(#196212,#196213),(#196214,#196215),(#196216,#196217),
(#196218,#196219),(#196220,#196221),(#196222,#196223),(#196224,#196225),
(#196226,#196227),(#196228,#196229),(#196230,#196231),(#196232,#196233),
(#196234,#196235),(#196236,#196237),(#196238,#196239),(#196240,#196241),
(#196242,#196243),(#196244,#196245),(#196246,#196247),(#196248,#196249),
(#196250,#196251),(#196252,#196253),(#196254,#196255),(#196256,#196257),
(#196258,#196259),(#196260,#196261),(#196262,#196263),(#196264,#196265),
(#196266,#196267),(#196268,#196269),(#196270,#196271),(#196272,#196273),
(#196274,#196275),(#196276,#196277),(#196278,#196279),(#196280,#196281),
(#196282,#196283),(#196284,#196285),(#196286,#196287),(#196288,#196289),
(#196290,#196291),(#196292,#196293),(#196294,#196295),(#196296,#196297),
(#196298,#196299),(#196300,#196301),(#196302,#196303),(#196304,#196305),
(#196306,#196307),(#196308,#196309),(#196310,#196311),(#196312,#196313),
(#196314,#196315),(#196316,#196317),(#196318,#196319),(#196320,#196321),
(#196322,#196323),(#196324,#196325),(#196326,#196327),(#196328,#196329),
(#196330,#196331),(#196332,#196333),(#196334,#196335),(#196336,#196337),
(#196338,#196339),(#196340,#196341),(#196342,#196343),(#196344,#196345),
(#196346,#196347),(#196348,#196349),(#196350,#196351),(#196352,#196353),
(#196354,#196355),(#196356,#196357),(#196358,#196359),(#196360,#196361),
(#196362,#196363),(#196364,#196365),(#196366,#196367),(#196368,#196369),
(#196370,#196371),(#196372,#196373),(#196374,#196375),(#196376,#196377),
(#196378,#196379),(#196380,#196381),(#196382,#196383),(#196384,#196385),
(#196386,#196387),(#196388,#196389),(#196390,#196391),(#196392,#196393),
(#196394,#196395),(#196396,#196397),(#196398,#196399),(#196400,#196401),
(#196402,#196403),(#196404,#196405),(#196406,#196407),(#196408,#196409),
(#196410,#196411),(#196412,#196413),(#196414,#196415),(#196416,#196417),
(#196418,#196419),(#196420,#196421),(#196422,#196423),(#196424,#196425),
(#196426,#196427),(#196428,#196429),(#196430,#196431),(#196432,#196433),
(#196434,#196435),(#196436,#196437),(#196438,#196439),(#196440,#196441),
(#196442,#196443),(#196444,#196445),(#196446,#196447),(#196448,#196449),
(#196450,#196451),(#196452,#196453),(#196454,#196455),(#196456,#196457),
(#196458,#196459),(#196460,#196461),(#196462,#196463),(#196464,#196465),
(#196466,#196467),(#196468,#196469),(#196470,#196471),(#196472,#196473),
(#196474,#196475),(#196476,#196477),(#196478,#196479),(#196480,#196481),
(#196482,#196483),(#196484,#196485),(#196486,#196487),(#196488,#196489),
(#196490,#196491),(#196492,#196493),(#196494,#196495),(#196496,#196497),
(#196498,#196499),(#196500,#196501),(#196502,#196503),(#196504,#196505),
(#196506,#196507),(#196508,#196509),(#196510,#196511),(#196512,#196513),
(#196514,#196515),(#196516,#196517),(#196518,#196519),(#196520,#196521),
(#196522,#196523),(#196524,#196525),(#196526,#196527),(#196528,#196529),
(#196530,#196531),(#196532,#196533),(#196534,#196535),(#196536,#196537),
(#196538,#196539),(#196540,#196541),(#196542,#196543),(#196544,#196545),
(#196546,#196547),(#196548,#196549),(#196550,#196551),(#196552,#196553),
(#196554,#196555),(#196556,#196557),(#196558,#196559),(#196560,#196561),
(#196562,#196563),(#196564,#196565),(#196566,#196567),(#196568,#196569),
(#196570,#196571),(#196572,#196573),(#196574,#196575),(#196576,#196577),
(#196578,#196579),(#196580,#196581),(#196582,#196583),(#196584,#196585),
(#196586,#196587),(#196588,#196589),(#196590,#196591),(#196592,#196593),
(#196594,#196595),(#196596,#196597),(#196598,#196599),(#196600,#196601),
(#196602,#196603),(#196604,#196605),(#196606,#196607),(#196608,#196609),
(#196610,#196611),(#196612,#196613),(#196614,#196615),(#196616,#196617),
(#196618,#196619),(#196620,#196621),(#196622,#196623),(#196624,#196625),
(#196626,#196627),(#196628,#196629),(#196630,#196631),(#196632,#196633),
(#196634,#196635),(#196636,#196637),(#196638,#196639),(#196640,#196641),
(#196642,#196643),(#196644,#196645),(#196646,#196647),(#196648,#196649),
(#196650,#196651),(#196652,#196653),(#196654,#196655),(#196656,#196657),
(#196658,#196659),(#196660,#196661),(#196662,#196663),(#196664,#196665),
(#196666,#196667),(#196668,#196669),(#196670,#196671),(#196672,#196673),
(#196674,#196675),(#196676,#196677),(#196678,#196679),(#196680,#196681),
(#196682,#196683),(#196684,#196685),(#196686,#196687),(#196688,#196689),
(#196690,#196691),(#196692,#196693),(#196694,#196695),(#196696,#196697),
(#196698,#196699),(#196700,#196701),(#196702,#196703),(#196704,#196705),
(#196706,#196707),(#196708,#196709),(#196710,#196711),(#196712,#196713),
(#196714,#196715),(#196716,#196717),(#196718,#196719),(#196720,#196721),
(#196722,#196723),(#196724,#196725),(#196726,#196727),(#196728,#196729),
(#196730,#196731),(#196732,#196733),(#196734,#196735),(#196736,#196737),
(#196738,#196739),(#196740,#196741),(#196742,#196743),(#196744,#196745),
(#196746,#196747),(#196748,#196749),(#196750,#196751),(#196752,#196753),
(#196754,#196755),(#196756,#196757),(#196758,#196759),(#196760,#196761),
(#196762,#196763),(#196764,#196765),(#196766,#196767),(#196768,#196769),
(#196770,#196771),(#196772,#196773),(#196774,#196775),(#196776,#196777),
(#196778,#196779),(#196780,#196781),(#196782,#196783),(#196784,#196785),
(#196786,#196787),(#196788,#196789),(#196790,#196791),(#196792,#196793),
(#196794,#196795),(#196796,#196797),(#196798,#196799),(#196800,#196801),
(#196802,#196803),(#196804,#196805),(#196806,#196807),(#196808,#196809),
(#196810,#196811),(#196812,#196813),(#196814,#196815),(#196816,#196817),
(#196818,#196819),(#196820,#196821),(#196822,#196823),(#196824,#196825),
(#196826,#196827),(#196828,#196829),(#196830,#196831),(#196832,#196833),
(#196834,#196835),(#196836,#196837),(#196838,#196839),(#196840,#196841),
(#196842,#196843),(#196844,#196845),(#196846,#196847),(#196848,#196849),
(#196850,#196851),(#196852,#196853),(#196854,#196855),(#196856,#196857),
(#196858,#196859),(#196860,#196861),(#196862,#196863),(#196864,#196865),
(#196866,#196867),(#196868,#196869),(#196870,#196871),(#196872,#196873),
(#196874,#196875),(#196876,#196877),(#196878,#196879),(#196880,#196881),
(#196882,#196883),(#196884,#196885),(#196886,#196887),(#196888,#196889),
(#196890,#196891),(#196892,#196893),(#196894,#196895),(#196896,#196897),
(#196898,#196899),(#196900,#196901),(#196902,#196903),(#196904,#196905),
(#196906,#196907),(#196908,#196909),(#196910,#196911),(#196912,#196913),
(#196914,#196915),(#196916,#196917),(#196918,#196919),(#196920,#196921),
(#196922,#196923),(#196924,#196925),(#196926,#196927),(#196928,#196929),
(#196930,#196931),(#196932,#196933),(#196934,#196935),(#196936,#196937),
(#196938,#196939),(#196940,#196941),(#196942,#196943),(#196944,#196945),
(#196946,#196947),(#196948,#196949),(#196950,#196951),(#196952,#196953),
(#196954,#196955),(#196956,#196957),(#196958,#196959),(#196960,#196961),
(#196962,#196963),(#196964,#196965),(#196966,#196967),(#196968,#196969),
(#196970,#196971),(#196972,#196973),(#196974,#196975),(#196976,#196977),
(#196978,#196979),(#196980,#196981),(#196982,#196983),(#196984,#196985),
(#196986,#196987),(#196988,#196989),(#196990,#196991),(#196992,#196993),
(#196994,#196995),(#196996,#196997)),.UNSPECIFIED.,.F.,.F.,.F.,(6,1,1,1,
1,1,1,1,1,1,1,1,1,1,1,1,1,1,1,1,1,1,1,1,1,1,1,1,1,1,1,1,1,1,1,1,1,1,1,1,
1,1,1,1,1,1,1,1,1,1,1,1,1,1,1,1,1,1,1,1,1,1,1,1,1,1,1,1,1,1,1,1,1,1,1,1,
1,1,1,1,1,1,1,1,1,1,1,1,1,1,1,1,1,1,1,1,1,1,1,1,1,1,1,1,1,1,1,1,1,1,1,1,
1,1,1,1,1,1,1,1,1,1,1,1,1,1,1,1,1,1,1,1,1,1,1,1,1,1,1,1,1,1,1,1,1,1,1,1,
1,1,1,1,1,1,1,1,1,1,1,1,1,1,1,1,1,1,1,1,1,1,1,1,1,1,1,1,1,1,1,1,1,1,1,1,
1,1,1,1,1,1,1,1,1,1,1,1,1,1,1,1,1,1,1,1,1,1,1,1,1,1,1,1,1,1,1,1,1,1,1,1,
1,1,1,1,1,1,1,1,1,1,1,1,1,1,1,1,1,1,1,1,1,1,1,1,1,1,1,1,1,1,1,1,1,1,1,1,
1,1,1,1,1,1,1,1,1,1,1,1,1,1,1,1,1,1,1,1,1,1,1,1,1,1,1,1,1,1,1,1,1,1,1,1,
1,1,1,1,1,1,1,1,1,1,1,1,1,1,1,1,1,1,1,1,1,1,1,1,1,1,1,1,1,1,1,1,1,1,1,1,
1,1,1,1,1,1,1,1,1,1,1,1,1,1,1,1,1,1,1,1,1,1,1,1,1,1,1,1,1,1,1,1,1,1,1,1,
1,1,1,1,1,1,1,1,1,1,1,1,1,1,1,1,1,1,1,1,1,1,1,1,1,1,1,1,1,1,1,1,1,1,1,1,
1,1,1,1,1,1,1,1,1,1,1,1,1,1,1,1,1,1,1,1,1,1,1,1,1,1,1,1,1,1,1,1,1,1,1,1,
1,1,1,1,1,1,1,1,1,1,1,1,1,1,1,1,1,1,1,1,1,1,1,1,1,1,1,1,1,1,1,6),(2,2),
(-1.,-0.998165138,-0.996330275,-0.994495413,-0.99266055,-0.990825688,-0.988990826,
-0.987155963,-0.985321101,-0.983486239,-0.981651376,-0.979816514,-0.977981651,
-0.976146789,-0.974311927,-0.972477064,-0.970642202,-0.968807339,-0.966972477,
-0.965137615,-0.963302752,-0.96146789,-0.959633028,-0.957798165,-0.955963303,
-0.95412844,-0.952293578,-0.950458716,-0.948623853,-0.946788991,-0.944954128,
-0.943119266,-0.941284404,-0.939449541,-0.937614679,-0.935779817,-0.933944954,
-0.932110092,-0.930275229,-0.928440367,-0.926605505,-0.924770642,-0.92293578,
-0.921100917,-0.919266055,-0.917431193,-0.91559633,-0.913761468,-0.911926606,
-0.910091743,-0.908256881,-0.906422018,-0.904587156,-0.902752294,-0.900917431,
-0.899082569,-0.897247706,-0.895412844,-0.893577982,-0.891743119,-0.889908257,
-0.888073394,-0.886238532,-0.88440367,-0.882568807,-0.880733945,-0.878899083,
-0.87706422,-0.875229358,-0.873394495,-0.871559633,-0.869724771,-0.867889908,
-0.866055046,-0.864220183,-0.862385321,-0.860550459,-0.858715596,-0.856880734,
-0.855045872,-0.853211009,-0.851376147,-0.849541284,-0.847706422,-0.84587156,
-0.844036697,-0.842201835,-0.840366972,-0.83853211,-0.836697248,-0.834862385,
-0.833027523,-0.831192661,-0.829357798,-0.827522936,-0.825688073,-0.823853211,
-0.822018349,-0.820183486,-0.818348624,-0.816513761,-0.814678899,-0.812844037,
-0.811009174,-0.809174312,-0.80733945,-0.805504587,-0.803669725,-0.801834862,
-0.8,-0.798165138,-0.796330275,-0.794495413,-0.79266055,-0.790825688,-0.788990826,
-0.787155963,-0.785321101,-0.783486239,-0.781651376,-0.779816514,-0.777981651,
-0.776146789,-0.774311927,-0.772477064,-0.770642202,-0.768807339,-0.766972477,
-0.765137615,-0.763302752,-0.76146789,-0.759633028,-0.757798165,-0.755963303,
-0.75412844,-0.752293578,-0.750458716,-0.748623853,-0.746788991,-0.744954128,
-0.743119266,-0.741284404,-0.739449541,-0.737614679,-0.735779817,-0.733944954,
-0.732110092,-0.730275229,-0.728440367,-0.726605505,-0.724770642,-0.72293578,
-0.721100917,-0.719266055,-0.717431193,-0.71559633,-0.713761468,-0.711926606,
-0.710091743,-0.708256881,-0.706422018,-0.704587156,-0.702752294,-0.700917431,
-0.699082569,-0.697247706,-0.695412844,-0.693577982,-0.691743119,-0.689908257,
-0.688073394,-0.686238532,-0.68440367,-0.682568807,-0.680733945,-0.678899083,
-0.67706422,-0.675229358,-0.673394495,-0.671559633,-0.669724771,-0.667889908,
-0.666055046,-0.664220183,-0.662385321,-0.660550459,-0.658715596,-0.656880734,
-0.655045872,-0.653211009,-0.651376147,-0.649541284,-0.647706422,-0.64587156,
-0.644036697,-0.642201835,-0.640366972,-0.63853211,-0.636697248,-0.634862385,
-0.633027523,-0.631192661,-0.629357798,-0.627522936,-0.625688073,-0.623853211,
-0.622018349,-0.620183486,-0.618348624,-0.616513761,-0.614678899,-0.612844037,
-0.611009174,-0.609174312,-0.60733945,-0.605504587,-0.603669725,-0.601834862,
-0.6,-0.598165138,-0.596330275,-0.594495413,-0.59266055,-0.590825688,-0.588990826,
-0.587155963,-0.585321101,-0.583486239,-0.581651376,-0.579816514,-0.577981651,
-0.576146789,-0.574311927,-0.572477064,-0.570642202,-0.568807339,-0.566972477,
-0.565137615,-0.563302752,-0.56146789,-0.559633028,-0.557798165,-0.555963303,
-0.55412844,-0.552293578,-0.550458716,-0.548623853,-0.546788991,-0.544954128,
-0.543119266,-0.541284404,-0.539449541,-0.537614679,-0.535779817,-0.533944954,
-0.532110092,-0.530275229,-0.528440367,-0.526605505,-0.524770642,-0.52293578,
-0.521100917,-0.519266055,-0.517431193,-0.51559633,-0.513761468,-0.511926606,
-0.510091743,-0.508256881,-0.506422018,-0.504587156,-0.502752294,-0.500917431,
-0.499082569,-0.497247706,-0.495412844,-0.493577982,-0.491743119,-0.489908257,
-0.488073394,-0.486238532,-0.48440367,-0.482568807,-0.480733945,-0.478899083,
-0.47706422,-0.475229358,-0.473394495,-0.471559633,-0.469724771,-0.467889908,
-0.466055046,-0.464220183,-0.462385321,-0.460550459,-0.458715596,-0.456880734,
-0.455045872,-0.453211009,-0.451376147,-0.449541284,-0.447706422,-0.44587156,
-0.444036697,-0.442201835,-0.440366972,-0.43853211,-0.436697248,-0.434862385,
-0.433027523,-0.431192661,-0.429357798,-0.427522936,-0.425688073,-0.423853211,
-0.422018349,-0.420183486,-0.418348624,-0.416513761,-0.414678899,-0.412844037,
-0.411009174,-0.409174312,-0.40733945,-0.405504587,-0.403669725,-0.401834862,
-0.4,-0.398165138,-0.396330275,-0.394495413,-0.39266055,-0.390825688,-0.388990826,
-0.387155963,-0.385321101,-0.383486239,-0.381651376,-0.379816514,-0.377981651,
-0.376146789,-0.374311927,-0.372477064,-0.370642202,-0.368807339,-0.366972477,
-0.365137615,-0.363302752,-0.36146789,-0.359633028,-0.357798165,-0.355963303,
-0.35412844,-0.352293578,-0.350458716,-0.348623853,-0.346788991,-0.344954128,
-0.343119266,-0.341284404,-0.339449541,-0.337614679,-0.335779817,-0.333944954,
-0.332110092,-0.330275229,-0.328440367,-0.326605505,-0.324770642,-0.32293578,
-0.321100917,-0.319266055,-0.317431193,-0.31559633,-0.313761468,-0.311926606,
-0.310091743,-0.308256881,-0.306422018,-0.304587156,-0.302752294,-0.300917431,
-0.299082569,-0.297247706,-0.295412844,-0.293577982,-0.291743119,-0.289908257,
-0.288073394,-0.286238532,-0.28440367,-0.282568807,-0.280733945,-0.278899083,
-0.27706422,-0.275229358,-0.273394495,-0.271559633,-0.269724771,-0.267889908,
-0.266055046,-0.264220183,-0.262385321,-0.260550459,-0.258715596,-0.256880734,
-0.255045872,-0.253211009,-0.251376147,-0.249541284,-0.247706422,-0.24587156,
-0.244036697,-0.242201835,-0.240366972,-0.23853211,-0.236697248,-0.234862385,
-0.233027523,-0.231192661,-0.229357798,-0.227522936,-0.225688073,-0.223853211,
-0.222018349,-0.220183486,-0.218348624,-0.216513761,-0.214678899,-0.212844037,
-0.211009174,-0.209174312,-0.20733945,-0.205504587,-0.203669725,-0.201834862,
-0.2,-0.198165138,-0.196330275,-0.194495413,-0.19266055,-0.190825688,-0.188990826,
-0.187155963,-0.185321101,-0.183486239,-0.181651376,-0.179816514,-0.177981651,
-0.176146789,-0.174311927,-0.172477064,-0.170642202,-0.168807339,-0.166972477,
-0.165137615,-0.163302752,-0.16146789,-0.159633028,-0.157798165,-0.155963303,
-0.15412844,-0.152293578,-0.150458716,-0.148623853,-0.146788991,-0.144954128,
-0.143172103),(0.,0.36),.UNSPECIFIED.);
#6241=B_SPLINE_SURFACE_WITH_KNOTS('',5,1,((#197960,#197961),(#197962,#197963),
(#197964,#197965),(#197966,#197967),(#197968,#197969),(#197970,#197971),
(#197972,#197973),(#197974,#197975),(#197976,#197977),(#197978,#197979),
(#197980,#197981),(#197982,#197983),(#197984,#197985),(#197986,#197987),
(#197988,#197989),(#197990,#197991),(#197992,#197993),(#197994,#197995),
(#197996,#197997),(#197998,#197999),(#198000,#198001),(#198002,#198003),
(#198004,#198005),(#198006,#198007),(#198008,#198009),(#198010,#198011),
(#198012,#198013),(#198014,#198015),(#198016,#198017),(#198018,#198019),
(#198020,#198021),(#198022,#198023),(#198024,#198025),(#198026,#198027),
(#198028,#198029),(#198030,#198031),(#198032,#198033),(#198034,#198035),
(#198036,#198037),(#198038,#198039),(#198040,#198041),(#198042,#198043),
(#198044,#198045),(#198046,#198047),(#198048,#198049),(#198050,#198051),
(#198052,#198053),(#198054,#198055),(#198056,#198057),(#198058,#198059),
(#198060,#198061),(#198062,#198063),(#198064,#198065),(#198066,#198067),
(#198068,#198069),(#198070,#198071),(#198072,#198073),(#198074,#198075),
(#198076,#198077),(#198078,#198079),(#198080,#198081),(#198082,#198083),
(#198084,#198085),(#198086,#198087),(#198088,#198089),(#198090,#198091),
(#198092,#198093),(#198094,#198095),(#198096,#198097),(#198098,#198099),
(#198100,#198101),(#198102,#198103),(#198104,#198105),(#198106,#198107),
(#198108,#198109),(#198110,#198111),(#198112,#198113),(#198114,#198115),
(#198116,#198117),(#198118,#198119),(#198120,#198121),(#198122,#198123),
(#198124,#198125),(#198126,#198127),(#198128,#198129),(#198130,#198131),
(#198132,#198133),(#198134,#198135),(#198136,#198137),(#198138,#198139),
(#198140,#198141),(#198142,#198143),(#198144,#198145),(#198146,#198147),
(#198148,#198149),(#198150,#198151),(#198152,#198153),(#198154,#198155),
(#198156,#198157),(#198158,#198159),(#198160,#198161),(#198162,#198163),
(#198164,#198165),(#198166,#198167),(#198168,#198169),(#198170,#198171),
(#198172,#198173),(#198174,#198175),(#198176,#198177),(#198178,#198179),
(#198180,#198181),(#198182,#198183),(#198184,#198185),(#198186,#198187),
(#198188,#198189),(#198190,#198191),(#198192,#198193),(#198194,#198195),
(#198196,#198197),(#198198,#198199),(#198200,#198201),(#198202,#198203),
(#198204,#198205),(#198206,#198207),(#198208,#198209),(#198210,#198211),
(#198212,#198213),(#198214,#198215),(#198216,#198217),(#198218,#198219),
(#198220,#198221),(#198222,#198223),(#198224,#198225),(#198226,#198227),
(#198228,#198229),(#198230,#198231),(#198232,#198233),(#198234,#198235),
(#198236,#198237),(#198238,#198239),(#198240,#198241),(#198242,#198243),
(#198244,#198245),(#198246,#198247),(#198248,#198249),(#198250,#198251),
(#198252,#198253),(#198254,#198255),(#198256,#198257),(#198258,#198259),
(#198260,#198261),(#198262,#198263),(#198264,#198265),(#198266,#198267),
(#198268,#198269),(#198270,#198271),(#198272,#198273),(#198274,#198275),
(#198276,#198277),(#198278,#198279),(#198280,#198281),(#198282,#198283),
(#198284,#198285),(#198286,#198287),(#198288,#198289),(#198290,#198291),
(#198292,#198293),(#198294,#198295),(#198296,#198297),(#198298,#198299),
(#198300,#198301),(#198302,#198303),(#198304,#198305),(#198306,#198307),
(#198308,#198309),(#198310,#198311),(#198312,#198313),(#198314,#198315),
(#198316,#198317),(#198318,#198319),(#198320,#198321),(#198322,#198323),
(#198324,#198325),(#198326,#198327),(#198328,#198329),(#198330,#198331),
(#198332,#198333),(#198334,#198335),(#198336,#198337),(#198338,#198339),
(#198340,#198341),(#198342,#198343),(#198344,#198345),(#198346,#198347),
(#198348,#198349),(#198350,#198351),(#198352,#198353),(#198354,#198355),
(#198356,#198357),(#198358,#198359),(#198360,#198361),(#198362,#198363),
(#198364,#198365),(#198366,#198367),(#198368,#198369),(#198370,#198371),
(#198372,#198373),(#198374,#198375),(#198376,#198377),(#198378,#198379),
(#198380,#198381),(#198382,#198383),(#198384,#198385),(#198386,#198387),
(#198388,#198389),(#198390,#198391),(#198392,#198393),(#198394,#198395),
(#198396,#198397),(#198398,#198399),(#198400,#198401),(#198402,#198403),
(#198404,#198405),(#198406,#198407),(#198408,#198409),(#198410,#198411),
(#198412,#198413),(#198414,#198415),(#198416,#198417),(#198418,#198419),
(#198420,#198421),(#198422,#198423),(#198424,#198425),(#198426,#198427),
(#198428,#198429),(#198430,#198431),(#198432,#198433),(#198434,#198435),
(#198436,#198437),(#198438,#198439),(#198440,#198441),(#198442,#198443),
(#198444,#198445),(#198446,#198447),(#198448,#198449),(#198450,#198451),
(#198452,#198453),(#198454,#198455),(#198456,#198457),(#198458,#198459),
(#198460,#198461),(#198462,#198463),(#198464,#198465),(#198466,#198467),
(#198468,#198469),(#198470,#198471),(#198472,#198473),(#198474,#198475),
(#198476,#198477),(#198478,#198479),(#198480,#198481),(#198482,#198483),
(#198484,#198485),(#198486,#198487),(#198488,#198489),(#198490,#198491),
(#198492,#198493),(#198494,#198495),(#198496,#198497),(#198498,#198499),
(#198500,#198501),(#198502,#198503),(#198504,#198505),(#198506,#198507),
(#198508,#198509),(#198510,#198511),(#198512,#198513),(#198514,#198515),
(#198516,#198517),(#198518,#198519),(#198520,#198521),(#198522,#198523),
(#198524,#198525),(#198526,#198527),(#198528,#198529),(#198530,#198531),
(#198532,#198533),(#198534,#198535),(#198536,#198537),(#198538,#198539),
(#198540,#198541),(#198542,#198543),(#198544,#198545),(#198546,#198547),
(#198548,#198549),(#198550,#198551),(#198552,#198553),(#198554,#198555),
(#198556,#198557),(#198558,#198559),(#198560,#198561),(#198562,#198563),
(#198564,#198565),(#198566,#198567),(#198568,#198569),(#198570,#198571),
(#198572,#198573),(#198574,#198575),(#198576,#198577),(#198578,#198579),
(#198580,#198581),(#198582,#198583),(#198584,#198585),(#198586,#198587),
(#198588,#198589),(#198590,#198591),(#198592,#198593),(#198594,#198595),
(#198596,#198597),(#198598,#198599),(#198600,#198601),(#198602,#198603),
(#198604,#198605),(#198606,#198607),(#198608,#198609),(#198610,#198611),
(#198612,#198613),(#198614,#198615),(#198616,#198617),(#198618,#198619),
(#198620,#198621),(#198622,#198623),(#198624,#198625),(#198626,#198627),
(#198628,#198629),(#198630,#198631),(#198632,#198633),(#198634,#198635),
(#198636,#198637),(#198638,#198639),(#198640,#198641),(#198642,#198643),
(#198644,#198645),(#198646,#198647),(#198648,#198649),(#198650,#198651),
(#198652,#198653),(#198654,#198655),(#198656,#198657),(#198658,#198659),
(#198660,#198661),(#198662,#198663),(#198664,#198665),(#198666,#198667),
(#198668,#198669),(#198670,#198671),(#198672,#198673),(#198674,#198675),
(#198676,#198677),(#198678,#198679),(#198680,#198681),(#198682,#198683),
(#198684,#198685),(#198686,#198687),(#198688,#198689),(#198690,#198691),
(#198692,#198693),(#198694,#198695),(#198696,#198697),(#198698,#198699),
(#198700,#198701),(#198702,#198703),(#198704,#198705),(#198706,#198707),
(#198708,#198709),(#198710,#198711),(#198712,#198713),(#198714,#198715),
(#198716,#198717),(#198718,#198719),(#198720,#198721),(#198722,#198723),
(#198724,#198725),(#198726,#198727),(#198728,#198729),(#198730,#198731),
(#198732,#198733),(#198734,#198735),(#198736,#198737),(#198738,#198739),
(#198740,#198741),(#198742,#198743),(#198744,#198745),(#198746,#198747),
(#198748,#198749),(#198750,#198751),(#198752,#198753),(#198754,#198755),
(#198756,#198757),(#198758,#198759),(#198760,#198761),(#198762,#198763),
(#198764,#198765),(#198766,#198767),(#198768,#198769),(#198770,#198771),
(#198772,#198773),(#198774,#198775),(#198776,#198777),(#198778,#198779),
(#198780,#198781),(#198782,#198783),(#198784,#198785),(#198786,#198787),
(#198788,#198789),(#198790,#198791),(#198792,#198793),(#198794,#198795),
(#198796,#198797),(#198798,#198799),(#198800,#198801),(#198802,#198803),
(#198804,#198805),(#198806,#198807),(#198808,#198809),(#198810,#198811),
(#198812,#198813),(#198814,#198815),(#198816,#198817),(#198818,#198819),
(#198820,#198821),(#198822,#198823),(#198824,#198825),(#198826,#198827),
(#198828,#198829),(#198830,#198831),(#198832,#198833),(#198834,#198835),
(#198836,#198837),(#198838,#198839),(#198840,#198841),(#198842,#198843),
(#198844,#198845),(#198846,#198847),(#198848,#198849),(#198850,#198851),
(#198852,#198853),(#198854,#198855),(#198856,#198857),(#198858,#198859),
(#198860,#198861),(#198862,#198863),(#198864,#198865),(#198866,#198867),
(#198868,#198869),(#198870,#198871),(#198872,#198873),(#198874,#198875),
(#198876,#198877),(#198878,#198879),(#198880,#198881),(#198882,#198883),
(#198884,#198885),(#198886,#198887),(#198888,#198889),(#198890,#198891),
(#198892,#198893),(#198894,#198895),(#198896,#198897),(#198898,#198899),
(#198900,#198901),(#198902,#198903)),.UNSPECIFIED.,.F.,.F.,.F.,(6,1,1,1,
1,1,1,1,1,1,1,1,1,1,1,1,1,1,1,1,1,1,1,1,1,1,1,1,1,1,1,1,1,1,1,1,1,1,1,1,
1,1,1,1,1,1,1,1,1,1,1,1,1,1,1,1,1,1,1,1,1,1,1,1,1,1,1,1,1,1,1,1,1,1,1,1,
1,1,1,1,1,1,1,1,1,1,1,1,1,1,1,1,1,1,1,1,1,1,1,1,1,1,1,1,1,1,1,1,1,1,1,1,
1,1,1,1,1,1,1,1,1,1,1,1,1,1,1,1,1,1,1,1,1,1,1,1,1,1,1,1,1,1,1,1,1,1,1,1,
1,1,1,1,1,1,1,1,1,1,1,1,1,1,1,1,1,1,1,1,1,1,1,1,1,1,1,1,1,1,1,1,1,1,1,1,
1,1,1,1,1,1,1,1,1,1,1,1,1,1,1,1,1,1,1,1,1,1,1,1,1,1,1,1,1,1,1,1,1,1,1,1,
1,1,1,1,1,1,1,1,1,1,1,1,1,1,1,1,1,1,1,1,1,1,1,1,1,1,1,1,1,1,1,1,1,1,1,1,
1,1,1,1,1,1,1,1,1,1,1,1,1,1,1,1,1,1,1,1,1,1,1,1,1,1,1,1,1,1,1,1,1,1,1,1,
1,1,1,1,1,1,1,1,1,1,1,1,1,1,1,1,1,1,1,1,1,1,1,1,1,1,1,1,1,1,1,1,1,1,1,1,
1,1,1,1,1,1,1,1,1,1,1,1,1,1,1,1,1,1,1,1,1,1,1,1,1,1,1,1,1,1,1,1,1,1,1,1,
1,1,1,1,1,1,1,1,1,1,1,1,1,1,1,1,1,1,1,1,1,1,1,1,1,1,1,1,1,1,1,1,1,1,1,1,
1,1,1,1,1,1,1,1,1,1,1,1,1,1,1,1,1,1,1,1,1,1,1,1,1,1,1,1,1,1,1,1,1,1,1,1,
1,1,1,1,1,1,1,1,1,1,1,1,1,1,1,1,1,1,1,1,1,1,1,1,1,1,1,1,1,1,1,6),(2,2),
(-1.,-0.998165138,-0.996330275,-0.994495413,-0.99266055,-0.990825688,-0.988990826,
-0.987155963,-0.985321101,-0.983486239,-0.981651376,-0.979816514,-0.977981651,
-0.976146789,-0.974311927,-0.972477064,-0.970642202,-0.968807339,-0.966972477,
-0.965137615,-0.963302752,-0.96146789,-0.959633028,-0.957798165,-0.955963303,
-0.95412844,-0.952293578,-0.950458716,-0.948623853,-0.946788991,-0.944954128,
-0.943119266,-0.941284404,-0.939449541,-0.937614679,-0.935779817,-0.933944954,
-0.932110092,-0.930275229,-0.928440367,-0.926605505,-0.924770642,-0.92293578,
-0.921100917,-0.919266055,-0.917431193,-0.91559633,-0.913761468,-0.911926606,
-0.910091743,-0.908256881,-0.906422018,-0.904587156,-0.902752294,-0.900917431,
-0.899082569,-0.897247706,-0.895412844,-0.893577982,-0.891743119,-0.889908257,
-0.888073394,-0.886238532,-0.88440367,-0.882568807,-0.880733945,-0.878899083,
-0.87706422,-0.875229358,-0.873394495,-0.871559633,-0.869724771,-0.867889908,
-0.866055046,-0.864220183,-0.862385321,-0.860550459,-0.858715596,-0.856880734,
-0.855045872,-0.853211009,-0.851376147,-0.849541284,-0.847706422,-0.84587156,
-0.844036697,-0.842201835,-0.840366972,-0.83853211,-0.836697248,-0.834862385,
-0.833027523,-0.831192661,-0.829357798,-0.827522936,-0.825688073,-0.823853211,
-0.822018349,-0.820183486,-0.818348624,-0.816513761,-0.814678899,-0.812844037,
-0.811009174,-0.809174312,-0.80733945,-0.805504587,-0.803669725,-0.801834862,
-0.8,-0.798165138,-0.796330275,-0.794495413,-0.79266055,-0.790825688,-0.788990826,
-0.787155963,-0.785321101,-0.783486239,-0.781651376,-0.779816514,-0.777981651,
-0.776146789,-0.774311927,-0.772477064,-0.770642202,-0.768807339,-0.766972477,
-0.765137615,-0.763302752,-0.76146789,-0.759633028,-0.757798165,-0.755963303,
-0.75412844,-0.752293578,-0.750458716,-0.748623853,-0.746788991,-0.744954128,
-0.743119266,-0.741284404,-0.739449541,-0.737614679,-0.735779817,-0.733944954,
-0.732110092,-0.730275229,-0.728440367,-0.726605505,-0.724770642,-0.72293578,
-0.721100917,-0.719266055,-0.717431193,-0.71559633,-0.713761468,-0.711926606,
-0.710091743,-0.708256881,-0.706422018,-0.704587156,-0.702752294,-0.700917431,
-0.699082569,-0.697247706,-0.695412844,-0.693577982,-0.691743119,-0.689908257,
-0.688073394,-0.686238532,-0.68440367,-0.682568807,-0.680733945,-0.678899083,
-0.67706422,-0.675229358,-0.673394495,-0.671559633,-0.669724771,-0.667889908,
-0.666055046,-0.664220183,-0.662385321,-0.660550459,-0.658715596,-0.656880734,
-0.655045872,-0.653211009,-0.651376147,-0.649541284,-0.647706422,-0.64587156,
-0.644036697,-0.642201835,-0.640366972,-0.63853211,-0.636697248,-0.634862385,
-0.633027523,-0.631192661,-0.629357798,-0.627522936,-0.625688073,-0.623853211,
-0.622018349,-0.620183486,-0.618348624,-0.616513761,-0.614678899,-0.612844037,
-0.611009174,-0.609174312,-0.60733945,-0.605504587,-0.603669725,-0.601834862,
-0.6,-0.598165138,-0.596330275,-0.594495413,-0.59266055,-0.590825688,-0.588990826,
-0.587155963,-0.585321101,-0.583486239,-0.581651376,-0.579816514,-0.577981651,
-0.576146789,-0.574311927,-0.572477064,-0.570642202,-0.568807339,-0.566972477,
-0.565137615,-0.563302752,-0.56146789,-0.559633028,-0.557798165,-0.555963303,
-0.55412844,-0.552293578,-0.550458716,-0.548623853,-0.546788991,-0.544954128,
-0.543119266,-0.541284404,-0.539449541,-0.537614679,-0.535779817,-0.533944954,
-0.532110092,-0.530275229,-0.528440367,-0.526605505,-0.524770642,-0.52293578,
-0.521100917,-0.519266055,-0.517431193,-0.51559633,-0.513761468,-0.511926606,
-0.510091743,-0.508256881,-0.506422018,-0.504587156,-0.502752294,-0.500917431,
-0.499082569,-0.497247706,-0.495412844,-0.493577982,-0.491743119,-0.489908257,
-0.488073394,-0.486238532,-0.48440367,-0.482568807,-0.480733945,-0.478899083,
-0.47706422,-0.475229358,-0.473394495,-0.471559633,-0.469724771,-0.467889908,
-0.466055046,-0.464220183,-0.462385321,-0.460550459,-0.458715596,-0.456880734,
-0.455045872,-0.453211009,-0.451376147,-0.449541284,-0.447706422,-0.44587156,
-0.444036697,-0.442201835,-0.440366972,-0.43853211,-0.436697248,-0.434862385,
-0.433027523,-0.431192661,-0.429357798,-0.427522936,-0.425688073,-0.423853211,
-0.422018349,-0.420183486,-0.418348624,-0.416513761,-0.414678899,-0.412844037,
-0.411009174,-0.409174312,-0.40733945,-0.405504587,-0.403669725,-0.401834862,
-0.4,-0.398165138,-0.396330275,-0.394495413,-0.39266055,-0.390825688,-0.388990826,
-0.387155963,-0.385321101,-0.383486239,-0.381651376,-0.379816514,-0.377981651,
-0.376146789,-0.374311927,-0.372477064,-0.370642202,-0.368807339,-0.366972477,
-0.365137615,-0.363302752,-0.36146789,-0.359633028,-0.357798165,-0.355963303,
-0.35412844,-0.352293578,-0.350458716,-0.348623853,-0.346788991,-0.344954128,
-0.343119266,-0.341284404,-0.339449541,-0.337614679,-0.335779817,-0.333944954,
-0.332110092,-0.330275229,-0.328440367,-0.326605505,-0.324770642,-0.32293578,
-0.321100917,-0.319266055,-0.317431193,-0.31559633,-0.313761468,-0.311926606,
-0.310091743,-0.308256881,-0.306422018,-0.304587156,-0.302752294,-0.300917431,
-0.299082569,-0.297247706,-0.295412844,-0.293577982,-0.291743119,-0.289908257,
-0.288073394,-0.286238532,-0.28440367,-0.282568807,-0.280733945,-0.278899083,
-0.27706422,-0.275229358,-0.273394495,-0.271559633,-0.269724771,-0.267889908,
-0.266055046,-0.264220183,-0.262385321,-0.260550459,-0.258715596,-0.256880734,
-0.255045872,-0.253211009,-0.251376147,-0.249541284,-0.247706422,-0.24587156,
-0.244036697,-0.242201835,-0.240366972,-0.23853211,-0.236697248,-0.234862385,
-0.233027523,-0.231192661,-0.229357798,-0.227522936,-0.225688073,-0.223853211,
-0.222018349,-0.220183486,-0.218348624,-0.216513761,-0.214678899,-0.212844037,
-0.211009174,-0.209174312,-0.20733945,-0.205504587,-0.203669725,-0.201834862,
-0.2,-0.198165138,-0.196330275,-0.194495413,-0.19266055,-0.190825688,-0.188990826,
-0.187155963,-0.185321101,-0.183486239,-0.181651376,-0.179816514,-0.177981651,
-0.176146789,-0.174311927,-0.172477064,-0.170642202,-0.168807339,-0.166972477,
-0.165137615,-0.163302752,-0.16146789,-0.159633028,-0.157798165,-0.155963303,
-0.15412844,-0.152293578,-0.150458716,-0.148623853,-0.146788991,-0.144954128,
-0.143172104),(0.,0.36),.UNSPECIFIED.);
#6242=B_SPLINE_SURFACE_WITH_KNOTS('',5,1,((#199518,#199519),(#199520,#199521),
(#199522,#199523),(#199524,#199525),(#199526,#199527),(#199528,#199529),
(#199530,#199531),(#199532,#199533),(#199534,#199535),(#199536,#199537),
(#199538,#199539),(#199540,#199541),(#199542,#199543),(#199544,#199545),
(#199546,#199547),(#199548,#199549),(#199550,#199551),(#199552,#199553),
(#199554,#199555),(#199556,#199557),(#199558,#199559),(#199560,#199561),
(#199562,#199563),(#199564,#199565),(#199566,#199567),(#199568,#199569),
(#199570,#199571),(#199572,#199573),(#199574,#199575),(#199576,#199577),
(#199578,#199579),(#199580,#199581),(#199582,#199583),(#199584,#199585),
(#199586,#199587),(#199588,#199589),(#199590,#199591),(#199592,#199593),
(#199594,#199595),(#199596,#199597),(#199598,#199599),(#199600,#199601),
(#199602,#199603),(#199604,#199605),(#199606,#199607),(#199608,#199609),
(#199610,#199611),(#199612,#199613),(#199614,#199615),(#199616,#199617),
(#199618,#199619),(#199620,#199621),(#199622,#199623),(#199624,#199625),
(#199626,#199627),(#199628,#199629),(#199630,#199631),(#199632,#199633),
(#199634,#199635),(#199636,#199637),(#199638,#199639),(#199640,#199641),
(#199642,#199643),(#199644,#199645),(#199646,#199647),(#199648,#199649),
(#199650,#199651),(#199652,#199653),(#199654,#199655),(#199656,#199657),
(#199658,#199659),(#199660,#199661),(#199662,#199663),(#199664,#199665),
(#199666,#199667),(#199668,#199669),(#199670,#199671),(#199672,#199673),
(#199674,#199675),(#199676,#199677),(#199678,#199679),(#199680,#199681),
(#199682,#199683),(#199684,#199685),(#199686,#199687),(#199688,#199689),
(#199690,#199691),(#199692,#199693),(#199694,#199695),(#199696,#199697),
(#199698,#199699),(#199700,#199701),(#199702,#199703),(#199704,#199705),
(#199706,#199707),(#199708,#199709),(#199710,#199711),(#199712,#199713),
(#199714,#199715),(#199716,#199717),(#199718,#199719),(#199720,#199721),
(#199722,#199723),(#199724,#199725),(#199726,#199727),(#199728,#199729),
(#199730,#199731),(#199732,#199733),(#199734,#199735),(#199736,#199737),
(#199738,#199739),(#199740,#199741),(#199742,#199743),(#199744,#199745),
(#199746,#199747),(#199748,#199749),(#199750,#199751),(#199752,#199753),
(#199754,#199755),(#199756,#199757),(#199758,#199759),(#199760,#199761),
(#199762,#199763),(#199764,#199765),(#199766,#199767),(#199768,#199769),
(#199770,#199771),(#199772,#199773),(#199774,#199775),(#199776,#199777),
(#199778,#199779),(#199780,#199781),(#199782,#199783),(#199784,#199785),
(#199786,#199787),(#199788,#199789),(#199790,#199791),(#199792,#199793),
(#199794,#199795),(#199796,#199797),(#199798,#199799),(#199800,#199801),
(#199802,#199803),(#199804,#199805),(#199806,#199807),(#199808,#199809),
(#199810,#199811),(#199812,#199813),(#199814,#199815),(#199816,#199817),
(#199818,#199819),(#199820,#199821),(#199822,#199823),(#199824,#199825),
(#199826,#199827),(#199828,#199829),(#199830,#199831),(#199832,#199833),
(#199834,#199835),(#199836,#199837),(#199838,#199839),(#199840,#199841),
(#199842,#199843),(#199844,#199845),(#199846,#199847),(#199848,#199849),
(#199850,#199851),(#199852,#199853),(#199854,#199855),(#199856,#199857),
(#199858,#199859),(#199860,#199861),(#199862,#199863),(#199864,#199865),
(#199866,#199867),(#199868,#199869),(#199870,#199871),(#199872,#199873),
(#199874,#199875),(#199876,#199877),(#199878,#199879),(#199880,#199881),
(#199882,#199883),(#199884,#199885),(#199886,#199887),(#199888,#199889),
(#199890,#199891),(#199892,#199893),(#199894,#199895),(#199896,#199897),
(#199898,#199899),(#199900,#199901),(#199902,#199903),(#199904,#199905),
(#199906,#199907),(#199908,#199909),(#199910,#199911),(#199912,#199913),
(#199914,#199915),(#199916,#199917),(#199918,#199919),(#199920,#199921),
(#199922,#199923),(#199924,#199925),(#199926,#199927),(#199928,#199929),
(#199930,#199931),(#199932,#199933),(#199934,#199935),(#199936,#199937),
(#199938,#199939),(#199940,#199941),(#199942,#199943),(#199944,#199945),
(#199946,#199947),(#199948,#199949),(#199950,#199951),(#199952,#199953),
(#199954,#199955),(#199956,#199957),(#199958,#199959),(#199960,#199961),
(#199962,#199963),(#199964,#199965),(#199966,#199967),(#199968,#199969),
(#199970,#199971),(#199972,#199973),(#199974,#199975),(#199976,#199977),
(#199978,#199979),(#199980,#199981),(#199982,#199983),(#199984,#199985),
(#199986,#199987),(#199988,#199989),(#199990,#199991),(#199992,#199993),
(#199994,#199995),(#199996,#199997),(#199998,#199999),(#200000,#200001),
(#200002,#200003),(#200004,#200005),(#200006,#200007),(#200008,#200009),
(#200010,#200011),(#200012,#200013),(#200014,#200015),(#200016,#200017),
(#200018,#200019),(#200020,#200021),(#200022,#200023),(#200024,#200025),
(#200026,#200027),(#200028,#200029),(#200030,#200031),(#200032,#200033),
(#200034,#200035),(#200036,#200037),(#200038,#200039),(#200040,#200041),
(#200042,#200043),(#200044,#200045),(#200046,#200047),(#200048,#200049),
(#200050,#200051),(#200052,#200053),(#200054,#200055),(#200056,#200057),
(#200058,#200059),(#200060,#200061),(#200062,#200063),(#200064,#200065),
(#200066,#200067),(#200068,#200069),(#200070,#200071),(#200072,#200073),
(#200074,#200075),(#200076,#200077),(#200078,#200079),(#200080,#200081),
(#200082,#200083),(#200084,#200085),(#200086,#200087),(#200088,#200089),
(#200090,#200091),(#200092,#200093),(#200094,#200095),(#200096,#200097),
(#200098,#200099),(#200100,#200101),(#200102,#200103),(#200104,#200105),
(#200106,#200107),(#200108,#200109),(#200110,#200111),(#200112,#200113),
(#200114,#200115),(#200116,#200117),(#200118,#200119),(#200120,#200121),
(#200122,#200123),(#200124,#200125),(#200126,#200127),(#200128,#200129),
(#200130,#200131),(#200132,#200133),(#200134,#200135),(#200136,#200137),
(#200138,#200139),(#200140,#200141),(#200142,#200143),(#200144,#200145),
(#200146,#200147),(#200148,#200149),(#200150,#200151),(#200152,#200153),
(#200154,#200155),(#200156,#200157),(#200158,#200159),(#200160,#200161),
(#200162,#200163),(#200164,#200165),(#200166,#200167),(#200168,#200169),
(#200170,#200171),(#200172,#200173),(#200174,#200175),(#200176,#200177),
(#200178,#200179),(#200180,#200181),(#200182,#200183),(#200184,#200185),
(#200186,#200187),(#200188,#200189),(#200190,#200191),(#200192,#200193),
(#200194,#200195),(#200196,#200197),(#200198,#200199),(#200200,#200201),
(#200202,#200203),(#200204,#200205),(#200206,#200207),(#200208,#200209),
(#200210,#200211),(#200212,#200213),(#200214,#200215),(#200216,#200217),
(#200218,#200219),(#200220,#200221),(#200222,#200223),(#200224,#200225),
(#200226,#200227),(#200228,#200229),(#200230,#200231),(#200232,#200233),
(#200234,#200235),(#200236,#200237),(#200238,#200239),(#200240,#200241),
(#200242,#200243),(#200244,#200245),(#200246,#200247),(#200248,#200249),
(#200250,#200251),(#200252,#200253),(#200254,#200255),(#200256,#200257),
(#200258,#200259),(#200260,#200261),(#200262,#200263),(#200264,#200265),
(#200266,#200267),(#200268,#200269),(#200270,#200271),(#200272,#200273),
(#200274,#200275),(#200276,#200277),(#200278,#200279),(#200280,#200281),
(#200282,#200283),(#200284,#200285),(#200286,#200287),(#200288,#200289),
(#200290,#200291),(#200292,#200293),(#200294,#200295),(#200296,#200297),
(#200298,#200299),(#200300,#200301),(#200302,#200303),(#200304,#200305),
(#200306,#200307),(#200308,#200309),(#200310,#200311),(#200312,#200313),
(#200314,#200315),(#200316,#200317),(#200318,#200319),(#200320,#200321),
(#200322,#200323),(#200324,#200325),(#200326,#200327),(#200328,#200329),
(#200330,#200331),(#200332,#200333),(#200334,#200335),(#200336,#200337),
(#200338,#200339),(#200340,#200341),(#200342,#200343),(#200344,#200345),
(#200346,#200347),(#200348,#200349),(#200350,#200351),(#200352,#200353),
(#200354,#200355),(#200356,#200357),(#200358,#200359),(#200360,#200361),
(#200362,#200363),(#200364,#200365),(#200366,#200367),(#200368,#200369),
(#200370,#200371),(#200372,#200373),(#200374,#200375),(#200376,#200377),
(#200378,#200379),(#200380,#200381),(#200382,#200383),(#200384,#200385),
(#200386,#200387),(#200388,#200389),(#200390,#200391),(#200392,#200393),
(#200394,#200395),(#200396,#200397),(#200398,#200399),(#200400,#200401),
(#200402,#200403),(#200404,#200405),(#200406,#200407),(#200408,#200409),
(#200410,#200411),(#200412,#200413),(#200414,#200415),(#200416,#200417),
(#200418,#200419),(#200420,#200421),(#200422,#200423),(#200424,#200425),
(#200426,#200427),(#200428,#200429),(#200430,#200431),(#200432,#200433),
(#200434,#200435),(#200436,#200437),(#200438,#200439),(#200440,#200441),
(#200442,#200443),(#200444,#200445),(#200446,#200447),(#200448,#200449),
(#200450,#200451),(#200452,#200453),(#200454,#200455),(#200456,#200457),
(#200458,#200459),(#200460,#200461)),.UNSPECIFIED.,.F.,.F.,.F.,(6,1,1,1,
1,1,1,1,1,1,1,1,1,1,1,1,1,1,1,1,1,1,1,1,1,1,1,1,1,1,1,1,1,1,1,1,1,1,1,1,
1,1,1,1,1,1,1,1,1,1,1,1,1,1,1,1,1,1,1,1,1,1,1,1,1,1,1,1,1,1,1,1,1,1,1,1,
1,1,1,1,1,1,1,1,1,1,1,1,1,1,1,1,1,1,1,1,1,1,1,1,1,1,1,1,1,1,1,1,1,1,1,1,
1,1,1,1,1,1,1,1,1,1,1,1,1,1,1,1,1,1,1,1,1,1,1,1,1,1,1,1,1,1,1,1,1,1,1,1,
1,1,1,1,1,1,1,1,1,1,1,1,1,1,1,1,1,1,1,1,1,1,1,1,1,1,1,1,1,1,1,1,1,1,1,1,
1,1,1,1,1,1,1,1,1,1,1,1,1,1,1,1,1,1,1,1,1,1,1,1,1,1,1,1,1,1,1,1,1,1,1,1,
1,1,1,1,1,1,1,1,1,1,1,1,1,1,1,1,1,1,1,1,1,1,1,1,1,1,1,1,1,1,1,1,1,1,1,1,
1,1,1,1,1,1,1,1,1,1,1,1,1,1,1,1,1,1,1,1,1,1,1,1,1,1,1,1,1,1,1,1,1,1,1,1,
1,1,1,1,1,1,1,1,1,1,1,1,1,1,1,1,1,1,1,1,1,1,1,1,1,1,1,1,1,1,1,1,1,1,1,1,
1,1,1,1,1,1,1,1,1,1,1,1,1,1,1,1,1,1,1,1,1,1,1,1,1,1,1,1,1,1,1,1,1,1,1,1,
1,1,1,1,1,1,1,1,1,1,1,1,1,1,1,1,1,1,1,1,1,1,1,1,1,1,1,1,1,1,1,1,1,1,1,1,
1,1,1,1,1,1,1,1,1,1,1,1,1,1,1,1,1,1,1,1,1,1,1,1,1,1,1,1,1,1,1,1,1,1,1,1,
1,1,1,1,1,1,1,1,1,1,1,1,1,1,1,1,1,1,1,1,1,1,1,1,1,1,1,1,1,1,1,6),(2,2),
(0.143172104,0.144954128,0.146788991,0.148623853,0.150458716,0.152293578,
0.15412844,0.155963303,0.157798165,0.159633028,0.16146789,0.163302752,0.165137615,
0.166972477,0.168807339,0.170642202,0.172477064,0.174311927,0.176146789,
0.177981651,0.179816514,0.181651376,0.183486239,0.185321101,0.187155963,
0.188990826,0.190825688,0.19266055,0.194495413,0.196330275,0.198165138,
0.2,0.201834862,0.203669725,0.205504587,0.20733945,0.209174312,0.211009174,
0.212844037,0.214678899,0.216513761,0.218348624,0.220183486,0.222018349,
0.223853211,0.225688073,0.227522936,0.229357798,0.231192661,0.233027523,
0.234862385,0.236697248,0.23853211,0.240366972,0.242201835,0.244036697,
0.24587156,0.247706422,0.249541284,0.251376147,0.253211009,0.255045872,
0.256880734,0.258715596,0.260550459,0.262385321,0.264220183,0.266055046,
0.267889908,0.269724771,0.271559633,0.273394495,0.275229358,0.27706422,
0.278899083,0.280733945,0.282568807,0.28440367,0.286238532,0.288073394,
0.289908257,0.291743119,0.293577982,0.295412844,0.297247706,0.299082569,
0.300917431,0.302752294,0.304587156,0.306422018,0.308256881,0.310091743,
0.311926606,0.313761468,0.31559633,0.317431193,0.319266055,0.321100917,
0.32293578,0.324770642,0.326605505,0.328440367,0.330275229,0.332110092,
0.333944954,0.335779817,0.337614679,0.339449541,0.341284404,0.343119266,
0.344954128,0.346788991,0.348623853,0.350458716,0.352293578,0.35412844,
0.355963303,0.357798165,0.359633028,0.36146789,0.363302752,0.365137615,
0.366972477,0.368807339,0.370642202,0.372477064,0.374311927,0.376146789,
0.377981651,0.379816514,0.381651376,0.383486239,0.385321101,0.387155963,
0.388990826,0.390825688,0.39266055,0.394495413,0.396330275,0.398165138,
0.4,0.401834862,0.403669725,0.405504587,0.40733945,0.409174312,0.411009174,
0.412844037,0.414678899,0.416513761,0.418348624,0.420183486,0.422018349,
0.423853211,0.425688073,0.427522936,0.429357798,0.431192661,0.433027523,
0.434862385,0.436697248,0.43853211,0.440366972,0.442201835,0.444036697,
0.44587156,0.447706422,0.449541284,0.451376147,0.453211009,0.455045872,
0.456880734,0.458715596,0.460550459,0.462385321,0.464220183,0.466055046,
0.467889908,0.469724771,0.471559633,0.473394495,0.475229358,0.47706422,
0.478899083,0.480733945,0.482568807,0.48440367,0.486238532,0.488073394,
0.489908257,0.491743119,0.493577982,0.495412844,0.497247706,0.499082569,
0.500917431,0.502752294,0.504587156,0.506422018,0.508256881,0.510091743,
0.511926606,0.513761468,0.51559633,0.517431193,0.519266055,0.521100917,
0.52293578,0.524770642,0.526605505,0.528440367,0.530275229,0.532110092,
0.533944954,0.535779817,0.537614679,0.539449541,0.541284404,0.543119266,
0.544954128,0.546788991,0.548623853,0.550458716,0.552293578,0.55412844,
0.555963303,0.557798165,0.559633028,0.56146789,0.563302752,0.565137615,
0.566972477,0.568807339,0.570642202,0.572477064,0.574311927,0.576146789,
0.577981651,0.579816514,0.581651376,0.583486239,0.585321101,0.587155963,
0.588990826,0.590825688,0.59266055,0.594495413,0.596330275,0.598165138,
0.6,0.601834862,0.603669725,0.605504587,0.60733945,0.609174312,0.611009174,
0.612844037,0.614678899,0.616513761,0.618348624,0.620183486,0.622018349,
0.623853211,0.625688073,0.627522936,0.629357798,0.631192661,0.633027523,
0.634862385,0.636697248,0.63853211,0.640366972,0.642201835,0.644036697,
0.64587156,0.647706422,0.649541284,0.651376147,0.653211009,0.655045872,
0.656880734,0.658715596,0.660550459,0.662385321,0.664220183,0.666055046,
0.667889908,0.669724771,0.671559633,0.673394495,0.675229358,0.67706422,
0.678899083,0.680733945,0.682568807,0.68440367,0.686238532,0.688073394,
0.689908257,0.691743119,0.693577982,0.695412844,0.697247706,0.699082569,
0.700917431,0.702752294,0.704587156,0.706422018,0.708256881,0.710091743,
0.711926606,0.713761468,0.71559633,0.717431193,0.719266055,0.721100917,
0.72293578,0.724770642,0.726605505,0.728440367,0.730275229,0.732110092,
0.733944954,0.735779817,0.737614679,0.739449541,0.741284404,0.743119266,
0.744954128,0.746788991,0.748623853,0.750458716,0.752293578,0.75412844,
0.755963303,0.757798165,0.759633028,0.76146789,0.763302752,0.765137615,
0.766972477,0.768807339,0.770642202,0.772477064,0.774311927,0.776146789,
0.777981651,0.779816514,0.781651376,0.783486239,0.785321101,0.787155963,
0.788990826,0.790825688,0.79266055,0.794495413,0.796330275,0.798165138,
0.8,0.801834862,0.803669725,0.805504587,0.80733945,0.809174312,0.811009174,
0.812844037,0.814678899,0.816513761,0.818348624,0.820183486,0.822018349,
0.823853211,0.825688073,0.827522936,0.829357798,0.831192661,0.833027523,
0.834862385,0.836697248,0.83853211,0.840366972,0.842201835,0.844036697,
0.84587156,0.847706422,0.849541284,0.851376147,0.853211009,0.855045872,
0.856880734,0.858715596,0.860550459,0.862385321,0.864220183,0.866055046,
0.867889908,0.869724771,0.871559633,0.873394495,0.875229358,0.87706422,
0.878899083,0.880733945,0.882568807,0.88440367,0.886238532,0.888073394,
0.889908257,0.891743119,0.893577982,0.895412844,0.897247706,0.899082569,
0.900917431,0.902752294,0.904587156,0.906422018,0.908256881,0.910091743,
0.911926606,0.913761468,0.91559633,0.917431193,0.919266055,0.921100917,
0.92293578,0.924770642,0.926605505,0.928440367,0.930275229,0.932110092,
0.933944954,0.935779817,0.937614679,0.939449541,0.941284404,0.943119266,
0.944954128,0.946788991,0.948623853,0.950458716,0.952293578,0.95412844,
0.955963303,0.957798165,0.959633028,0.96146789,0.963302752,0.965137615,
0.966972477,0.968807339,0.970642202,0.972477064,0.974311927,0.976146789,
0.977981651,0.979816514,0.981651376,0.983486239,0.985321101,0.987155963,
0.988990826,0.990825688,0.99266055,0.994495413,0.996330275,0.998165138,
1.),(0.,0.36),.UNSPECIFIED.);
#6243=B_SPLINE_SURFACE_WITH_KNOTS('',5,1,((#201118,#201119),(#201120,#201121),
(#201122,#201123),(#201124,#201125),(#201126,#201127),(#201128,#201129),
(#201130,#201131),(#201132,#201133),(#201134,#201135),(#201136,#201137),
(#201138,#201139),(#201140,#201141),(#201142,#201143),(#201144,#201145),
(#201146,#201147),(#201148,#201149),(#201150,#201151),(#201152,#201153),
(#201154,#201155),(#201156,#201157),(#201158,#201159),(#201160,#201161),
(#201162,#201163),(#201164,#201165),(#201166,#201167),(#201168,#201169),
(#201170,#201171),(#201172,#201173),(#201174,#201175),(#201176,#201177),
(#201178,#201179),(#201180,#201181),(#201182,#201183),(#201184,#201185),
(#201186,#201187),(#201188,#201189),(#201190,#201191),(#201192,#201193),
(#201194,#201195),(#201196,#201197),(#201198,#201199),(#201200,#201201),
(#201202,#201203),(#201204,#201205),(#201206,#201207),(#201208,#201209),
(#201210,#201211),(#201212,#201213),(#201214,#201215),(#201216,#201217),
(#201218,#201219),(#201220,#201221),(#201222,#201223),(#201224,#201225),
(#201226,#201227),(#201228,#201229),(#201230,#201231),(#201232,#201233),
(#201234,#201235),(#201236,#201237),(#201238,#201239),(#201240,#201241),
(#201242,#201243),(#201244,#201245),(#201246,#201247),(#201248,#201249),
(#201250,#201251),(#201252,#201253),(#201254,#201255),(#201256,#201257),
(#201258,#201259),(#201260,#201261),(#201262,#201263),(#201264,#201265),
(#201266,#201267),(#201268,#201269),(#201270,#201271),(#201272,#201273),
(#201274,#201275),(#201276,#201277),(#201278,#201279),(#201280,#201281),
(#201282,#201283),(#201284,#201285),(#201286,#201287),(#201288,#201289),
(#201290,#201291),(#201292,#201293),(#201294,#201295),(#201296,#201297),
(#201298,#201299),(#201300,#201301),(#201302,#201303),(#201304,#201305),
(#201306,#201307),(#201308,#201309),(#201310,#201311),(#201312,#201313),
(#201314,#201315),(#201316,#201317),(#201318,#201319),(#201320,#201321),
(#201322,#201323),(#201324,#201325),(#201326,#201327),(#201328,#201329),
(#201330,#201331),(#201332,#201333),(#201334,#201335),(#201336,#201337),
(#201338,#201339),(#201340,#201341),(#201342,#201343),(#201344,#201345),
(#201346,#201347),(#201348,#201349),(#201350,#201351),(#201352,#201353),
(#201354,#201355),(#201356,#201357),(#201358,#201359),(#201360,#201361),
(#201362,#201363),(#201364,#201365),(#201366,#201367),(#201368,#201369),
(#201370,#201371),(#201372,#201373),(#201374,#201375),(#201376,#201377),
(#201378,#201379),(#201380,#201381),(#201382,#201383),(#201384,#201385),
(#201386,#201387),(#201388,#201389),(#201390,#201391),(#201392,#201393),
(#201394,#201395),(#201396,#201397),(#201398,#201399),(#201400,#201401),
(#201402,#201403),(#201404,#201405),(#201406,#201407),(#201408,#201409),
(#201410,#201411),(#201412,#201413),(#201414,#201415),(#201416,#201417),
(#201418,#201419),(#201420,#201421),(#201422,#201423),(#201424,#201425),
(#201426,#201427),(#201428,#201429),(#201430,#201431),(#201432,#201433),
(#201434,#201435),(#201436,#201437),(#201438,#201439),(#201440,#201441),
(#201442,#201443),(#201444,#201445),(#201446,#201447),(#201448,#201449),
(#201450,#201451),(#201452,#201453),(#201454,#201455),(#201456,#201457),
(#201458,#201459),(#201460,#201461),(#201462,#201463),(#201464,#201465),
(#201466,#201467),(#201468,#201469),(#201470,#201471),(#201472,#201473),
(#201474,#201475),(#201476,#201477),(#201478,#201479),(#201480,#201481),
(#201482,#201483),(#201484,#201485),(#201486,#201487),(#201488,#201489),
(#201490,#201491),(#201492,#201493),(#201494,#201495),(#201496,#201497),
(#201498,#201499),(#201500,#201501),(#201502,#201503),(#201504,#201505),
(#201506,#201507),(#201508,#201509),(#201510,#201511),(#201512,#201513),
(#201514,#201515),(#201516,#201517),(#201518,#201519),(#201520,#201521),
(#201522,#201523),(#201524,#201525),(#201526,#201527),(#201528,#201529),
(#201530,#201531),(#201532,#201533),(#201534,#201535),(#201536,#201537),
(#201538,#201539),(#201540,#201541),(#201542,#201543),(#201544,#201545),
(#201546,#201547),(#201548,#201549),(#201550,#201551),(#201552,#201553),
(#201554,#201555),(#201556,#201557),(#201558,#201559),(#201560,#201561),
(#201562,#201563),(#201564,#201565),(#201566,#201567),(#201568,#201569),
(#201570,#201571),(#201572,#201573),(#201574,#201575),(#201576,#201577),
(#201578,#201579),(#201580,#201581),(#201582,#201583),(#201584,#201585),
(#201586,#201587),(#201588,#201589),(#201590,#201591),(#201592,#201593),
(#201594,#201595),(#201596,#201597),(#201598,#201599),(#201600,#201601),
(#201602,#201603),(#201604,#201605),(#201606,#201607),(#201608,#201609),
(#201610,#201611),(#201612,#201613),(#201614,#201615),(#201616,#201617),
(#201618,#201619),(#201620,#201621),(#201622,#201623),(#201624,#201625),
(#201626,#201627),(#201628,#201629),(#201630,#201631),(#201632,#201633),
(#201634,#201635),(#201636,#201637),(#201638,#201639),(#201640,#201641),
(#201642,#201643),(#201644,#201645),(#201646,#201647),(#201648,#201649),
(#201650,#201651),(#201652,#201653),(#201654,#201655),(#201656,#201657),
(#201658,#201659),(#201660,#201661),(#201662,#201663),(#201664,#201665),
(#201666,#201667),(#201668,#201669),(#201670,#201671),(#201672,#201673),
(#201674,#201675),(#201676,#201677),(#201678,#201679),(#201680,#201681),
(#201682,#201683),(#201684,#201685),(#201686,#201687),(#201688,#201689),
(#201690,#201691),(#201692,#201693),(#201694,#201695),(#201696,#201697),
(#201698,#201699),(#201700,#201701),(#201702,#201703),(#201704,#201705),
(#201706,#201707),(#201708,#201709),(#201710,#201711),(#201712,#201713),
(#201714,#201715),(#201716,#201717),(#201718,#201719),(#201720,#201721),
(#201722,#201723),(#201724,#201725),(#201726,#201727),(#201728,#201729),
(#201730,#201731),(#201732,#201733),(#201734,#201735),(#201736,#201737),
(#201738,#201739),(#201740,#201741),(#201742,#201743),(#201744,#201745),
(#201746,#201747),(#201748,#201749),(#201750,#201751),(#201752,#201753),
(#201754,#201755),(#201756,#201757),(#201758,#201759),(#201760,#201761),
(#201762,#201763),(#201764,#201765),(#201766,#201767),(#201768,#201769),
(#201770,#201771),(#201772,#201773),(#201774,#201775),(#201776,#201777),
(#201778,#201779),(#201780,#201781),(#201782,#201783),(#201784,#201785),
(#201786,#201787),(#201788,#201789),(#201790,#201791),(#201792,#201793),
(#201794,#201795),(#201796,#201797),(#201798,#201799),(#201800,#201801),
(#201802,#201803),(#201804,#201805),(#201806,#201807),(#201808,#201809),
(#201810,#201811),(#201812,#201813),(#201814,#201815),(#201816,#201817),
(#201818,#201819),(#201820,#201821),(#201822,#201823),(#201824,#201825),
(#201826,#201827),(#201828,#201829),(#201830,#201831),(#201832,#201833),
(#201834,#201835),(#201836,#201837),(#201838,#201839),(#201840,#201841),
(#201842,#201843),(#201844,#201845),(#201846,#201847),(#201848,#201849),
(#201850,#201851),(#201852,#201853),(#201854,#201855),(#201856,#201857),
(#201858,#201859),(#201860,#201861),(#201862,#201863),(#201864,#201865),
(#201866,#201867),(#201868,#201869),(#201870,#201871),(#201872,#201873),
(#201874,#201875),(#201876,#201877),(#201878,#201879),(#201880,#201881),
(#201882,#201883),(#201884,#201885),(#201886,#201887),(#201888,#201889),
(#201890,#201891),(#201892,#201893),(#201894,#201895),(#201896,#201897),
(#201898,#201899),(#201900,#201901),(#201902,#201903),(#201904,#201905),
(#201906,#201907),(#201908,#201909),(#201910,#201911),(#201912,#201913),
(#201914,#201915),(#201916,#201917),(#201918,#201919),(#201920,#201921),
(#201922,#201923),(#201924,#201925),(#201926,#201927),(#201928,#201929),
(#201930,#201931),(#201932,#201933),(#201934,#201935),(#201936,#201937),
(#201938,#201939),(#201940,#201941),(#201942,#201943),(#201944,#201945),
(#201946,#201947),(#201948,#201949),(#201950,#201951),(#201952,#201953),
(#201954,#201955),(#201956,#201957),(#201958,#201959),(#201960,#201961),
(#201962,#201963),(#201964,#201965),(#201966,#201967),(#201968,#201969),
(#201970,#201971),(#201972,#201973),(#201974,#201975),(#201976,#201977),
(#201978,#201979),(#201980,#201981),(#201982,#201983),(#201984,#201985),
(#201986,#201987),(#201988,#201989),(#201990,#201991),(#201992,#201993),
(#201994,#201995),(#201996,#201997),(#201998,#201999),(#202000,#202001),
(#202002,#202003),(#202004,#202005),(#202006,#202007),(#202008,#202009),
(#202010,#202011),(#202012,#202013),(#202014,#202015),(#202016,#202017),
(#202018,#202019),(#202020,#202021),(#202022,#202023),(#202024,#202025),
(#202026,#202027),(#202028,#202029),(#202030,#202031),(#202032,#202033),
(#202034,#202035),(#202036,#202037),(#202038,#202039),(#202040,#202041),
(#202042,#202043),(#202044,#202045),(#202046,#202047),(#202048,#202049),
(#202050,#202051),(#202052,#202053),(#202054,#202055),(#202056,#202057),
(#202058,#202059),(#202060,#202061)),.UNSPECIFIED.,.F.,.F.,.F.,(6,1,1,1,
1,1,1,1,1,1,1,1,1,1,1,1,1,1,1,1,1,1,1,1,1,1,1,1,1,1,1,1,1,1,1,1,1,1,1,1,
1,1,1,1,1,1,1,1,1,1,1,1,1,1,1,1,1,1,1,1,1,1,1,1,1,1,1,1,1,1,1,1,1,1,1,1,
1,1,1,1,1,1,1,1,1,1,1,1,1,1,1,1,1,1,1,1,1,1,1,1,1,1,1,1,1,1,1,1,1,1,1,1,
1,1,1,1,1,1,1,1,1,1,1,1,1,1,1,1,1,1,1,1,1,1,1,1,1,1,1,1,1,1,1,1,1,1,1,1,
1,1,1,1,1,1,1,1,1,1,1,1,1,1,1,1,1,1,1,1,1,1,1,1,1,1,1,1,1,1,1,1,1,1,1,1,
1,1,1,1,1,1,1,1,1,1,1,1,1,1,1,1,1,1,1,1,1,1,1,1,1,1,1,1,1,1,1,1,1,1,1,1,
1,1,1,1,1,1,1,1,1,1,1,1,1,1,1,1,1,1,1,1,1,1,1,1,1,1,1,1,1,1,1,1,1,1,1,1,
1,1,1,1,1,1,1,1,1,1,1,1,1,1,1,1,1,1,1,1,1,1,1,1,1,1,1,1,1,1,1,1,1,1,1,1,
1,1,1,1,1,1,1,1,1,1,1,1,1,1,1,1,1,1,1,1,1,1,1,1,1,1,1,1,1,1,1,1,1,1,1,1,
1,1,1,1,1,1,1,1,1,1,1,1,1,1,1,1,1,1,1,1,1,1,1,1,1,1,1,1,1,1,1,1,1,1,1,1,
1,1,1,1,1,1,1,1,1,1,1,1,1,1,1,1,1,1,1,1,1,1,1,1,1,1,1,1,1,1,1,1,1,1,1,1,
1,1,1,1,1,1,1,1,1,1,1,1,1,1,1,1,1,1,1,1,1,1,1,1,1,1,1,1,1,1,1,1,1,1,1,1,
1,1,1,1,1,1,1,1,1,1,1,1,1,1,1,1,1,1,1,1,1,1,1,1,1,1,1,1,1,1,1,6),(2,2),
(0.143172103,0.144954128,0.146788991,0.148623853,0.150458716,0.152293578,
0.15412844,0.155963303,0.157798165,0.159633028,0.16146789,0.163302752,0.165137615,
0.166972477,0.168807339,0.170642202,0.172477064,0.174311927,0.176146789,
0.177981651,0.179816514,0.181651376,0.183486239,0.185321101,0.187155963,
0.188990826,0.190825688,0.19266055,0.194495413,0.196330275,0.198165138,
0.2,0.201834862,0.203669725,0.205504587,0.20733945,0.209174312,0.211009174,
0.212844037,0.214678899,0.216513761,0.218348624,0.220183486,0.222018349,
0.223853211,0.225688073,0.227522936,0.229357798,0.231192661,0.233027523,
0.234862385,0.236697248,0.23853211,0.240366972,0.242201835,0.244036697,
0.24587156,0.247706422,0.249541284,0.251376147,0.253211009,0.255045872,
0.256880734,0.258715596,0.260550459,0.262385321,0.264220183,0.266055046,
0.267889908,0.269724771,0.271559633,0.273394495,0.275229358,0.27706422,
0.278899083,0.280733945,0.282568807,0.28440367,0.286238532,0.288073394,
0.289908257,0.291743119,0.293577982,0.295412844,0.297247706,0.299082569,
0.300917431,0.302752294,0.304587156,0.306422018,0.308256881,0.310091743,
0.311926606,0.313761468,0.31559633,0.317431193,0.319266055,0.321100917,
0.32293578,0.324770642,0.326605505,0.328440367,0.330275229,0.332110092,
0.333944954,0.335779817,0.337614679,0.339449541,0.341284404,0.343119266,
0.344954128,0.346788991,0.348623853,0.350458716,0.352293578,0.35412844,
0.355963303,0.357798165,0.359633028,0.36146789,0.363302752,0.365137615,
0.366972477,0.368807339,0.370642202,0.372477064,0.374311927,0.376146789,
0.377981651,0.379816514,0.381651376,0.383486239,0.385321101,0.387155963,
0.388990826,0.390825688,0.39266055,0.394495413,0.396330275,0.398165138,
0.4,0.401834862,0.403669725,0.405504587,0.40733945,0.409174312,0.411009174,
0.412844037,0.414678899,0.416513761,0.418348624,0.420183486,0.422018349,
0.423853211,0.425688073,0.427522936,0.429357798,0.431192661,0.433027523,
0.434862385,0.436697248,0.43853211,0.440366972,0.442201835,0.444036697,
0.44587156,0.447706422,0.449541284,0.451376147,0.453211009,0.455045872,
0.456880734,0.458715596,0.460550459,0.462385321,0.464220183,0.466055046,
0.467889908,0.469724771,0.471559633,0.473394495,0.475229358,0.47706422,
0.478899083,0.480733945,0.482568807,0.48440367,0.486238532,0.488073394,
0.489908257,0.491743119,0.493577982,0.495412844,0.497247706,0.499082569,
0.500917431,0.502752294,0.504587156,0.506422018,0.508256881,0.510091743,
0.511926606,0.513761468,0.51559633,0.517431193,0.519266055,0.521100917,
0.52293578,0.524770642,0.526605505,0.528440367,0.530275229,0.532110092,
0.533944954,0.535779817,0.537614679,0.539449541,0.541284404,0.543119266,
0.544954128,0.546788991,0.548623853,0.550458716,0.552293578,0.55412844,
0.555963303,0.557798165,0.559633028,0.56146789,0.563302752,0.565137615,
0.566972477,0.568807339,0.570642202,0.572477064,0.574311927,0.576146789,
0.577981651,0.579816514,0.581651376,0.583486239,0.585321101,0.587155963,
0.588990826,0.590825688,0.59266055,0.594495413,0.596330275,0.598165138,
0.6,0.601834862,0.603669725,0.605504587,0.60733945,0.609174312,0.611009174,
0.612844037,0.614678899,0.616513761,0.618348624,0.620183486,0.622018349,
0.623853211,0.625688073,0.627522936,0.629357798,0.631192661,0.633027523,
0.634862385,0.636697248,0.63853211,0.640366972,0.642201835,0.644036697,
0.64587156,0.647706422,0.649541284,0.651376147,0.653211009,0.655045872,
0.656880734,0.658715596,0.660550459,0.662385321,0.664220183,0.666055046,
0.667889908,0.669724771,0.671559633,0.673394495,0.675229358,0.67706422,
0.678899083,0.680733945,0.682568807,0.68440367,0.686238532,0.688073394,
0.689908257,0.691743119,0.693577982,0.695412844,0.697247706,0.699082569,
0.700917431,0.702752294,0.704587156,0.706422018,0.708256881,0.710091743,
0.711926606,0.713761468,0.71559633,0.717431193,0.719266055,0.721100917,
0.72293578,0.724770642,0.726605505,0.728440367,0.730275229,0.732110092,
0.733944954,0.735779817,0.737614679,0.739449541,0.741284404,0.743119266,
0.744954128,0.746788991,0.748623853,0.750458716,0.752293578,0.75412844,
0.755963303,0.757798165,0.759633028,0.76146789,0.763302752,0.765137615,
0.766972477,0.768807339,0.770642202,0.772477064,0.774311927,0.776146789,
0.777981651,0.779816514,0.781651376,0.783486239,0.785321101,0.787155963,
0.788990826,0.790825688,0.79266055,0.794495413,0.796330275,0.798165138,
0.8,0.801834862,0.803669725,0.805504587,0.80733945,0.809174312,0.811009174,
0.812844037,0.814678899,0.816513761,0.818348624,0.820183486,0.822018349,
0.823853211,0.825688073,0.827522936,0.829357798,0.831192661,0.833027523,
0.834862385,0.836697248,0.83853211,0.840366972,0.842201835,0.844036697,
0.84587156,0.847706422,0.849541284,0.851376147,0.853211009,0.855045872,
0.856880734,0.858715596,0.860550459,0.862385321,0.864220183,0.866055046,
0.867889908,0.869724771,0.871559633,0.873394495,0.875229358,0.87706422,
0.878899083,0.880733945,0.882568807,0.88440367,0.886238532,0.888073394,
0.889908257,0.891743119,0.893577982,0.895412844,0.897247706,0.899082569,
0.900917431,0.902752294,0.904587156,0.906422018,0.908256881,0.910091743,
0.911926606,0.913761468,0.91559633,0.917431193,0.919266055,0.921100917,
0.92293578,0.924770642,0.926605505,0.928440367,0.930275229,0.932110092,
0.933944954,0.935779817,0.937614679,0.939449541,0.941284404,0.943119266,
0.944954128,0.946788991,0.948623853,0.950458716,0.952293578,0.95412844,
0.955963303,0.957798165,0.959633028,0.96146789,0.963302752,0.965137615,
0.966972477,0.968807339,0.970642202,0.972477064,0.974311927,0.976146789,
0.977981651,0.979816514,0.981651376,0.983486239,0.985321101,0.987155963,
0.988990826,0.990825688,0.99266055,0.994495413,0.996330275,0.998165138,
1.),(0.,0.36),.UNSPECIFIED.);
#6244=B_SPLINE_SURFACE_WITH_KNOTS('',5,1,((#202700,#202701),(#202702,#202703),
(#202704,#202705),(#202706,#202707),(#202708,#202709),(#202710,#202711),
(#202712,#202713),(#202714,#202715),(#202716,#202717),(#202718,#202719),
(#202720,#202721),(#202722,#202723),(#202724,#202725),(#202726,#202727),
(#202728,#202729),(#202730,#202731),(#202732,#202733),(#202734,#202735),
(#202736,#202737),(#202738,#202739),(#202740,#202741),(#202742,#202743),
(#202744,#202745),(#202746,#202747),(#202748,#202749),(#202750,#202751),
(#202752,#202753),(#202754,#202755),(#202756,#202757),(#202758,#202759),
(#202760,#202761),(#202762,#202763),(#202764,#202765),(#202766,#202767),
(#202768,#202769),(#202770,#202771),(#202772,#202773),(#202774,#202775),
(#202776,#202777),(#202778,#202779),(#202780,#202781),(#202782,#202783),
(#202784,#202785),(#202786,#202787),(#202788,#202789),(#202790,#202791),
(#202792,#202793),(#202794,#202795),(#202796,#202797),(#202798,#202799),
(#202800,#202801),(#202802,#202803),(#202804,#202805),(#202806,#202807),
(#202808,#202809),(#202810,#202811),(#202812,#202813),(#202814,#202815),
(#202816,#202817),(#202818,#202819),(#202820,#202821),(#202822,#202823),
(#202824,#202825),(#202826,#202827),(#202828,#202829),(#202830,#202831),
(#202832,#202833),(#202834,#202835),(#202836,#202837),(#202838,#202839),
(#202840,#202841),(#202842,#202843),(#202844,#202845),(#202846,#202847),
(#202848,#202849),(#202850,#202851),(#202852,#202853),(#202854,#202855),
(#202856,#202857),(#202858,#202859),(#202860,#202861),(#202862,#202863),
(#202864,#202865),(#202866,#202867),(#202868,#202869),(#202870,#202871),
(#202872,#202873),(#202874,#202875),(#202876,#202877),(#202878,#202879),
(#202880,#202881),(#202882,#202883),(#202884,#202885),(#202886,#202887),
(#202888,#202889),(#202890,#202891),(#202892,#202893),(#202894,#202895),
(#202896,#202897),(#202898,#202899),(#202900,#202901),(#202902,#202903),
(#202904,#202905),(#202906,#202907),(#202908,#202909),(#202910,#202911),
(#202912,#202913),(#202914,#202915),(#202916,#202917),(#202918,#202919),
(#202920,#202921),(#202922,#202923),(#202924,#202925),(#202926,#202927),
(#202928,#202929),(#202930,#202931),(#202932,#202933),(#202934,#202935),
(#202936,#202937),(#202938,#202939),(#202940,#202941),(#202942,#202943),
(#202944,#202945),(#202946,#202947),(#202948,#202949),(#202950,#202951),
(#202952,#202953),(#202954,#202955),(#202956,#202957),(#202958,#202959),
(#202960,#202961),(#202962,#202963),(#202964,#202965),(#202966,#202967),
(#202968,#202969),(#202970,#202971),(#202972,#202973),(#202974,#202975),
(#202976,#202977),(#202978,#202979),(#202980,#202981),(#202982,#202983),
(#202984,#202985),(#202986,#202987),(#202988,#202989),(#202990,#202991),
(#202992,#202993),(#202994,#202995),(#202996,#202997),(#202998,#202999),
(#203000,#203001),(#203002,#203003),(#203004,#203005),(#203006,#203007),
(#203008,#203009),(#203010,#203011),(#203012,#203013),(#203014,#203015),
(#203016,#203017),(#203018,#203019),(#203020,#203021),(#203022,#203023),
(#203024,#203025),(#203026,#203027),(#203028,#203029),(#203030,#203031),
(#203032,#203033),(#203034,#203035),(#203036,#203037),(#203038,#203039),
(#203040,#203041),(#203042,#203043),(#203044,#203045),(#203046,#203047),
(#203048,#203049),(#203050,#203051),(#203052,#203053),(#203054,#203055),
(#203056,#203057),(#203058,#203059),(#203060,#203061),(#203062,#203063),
(#203064,#203065),(#203066,#203067),(#203068,#203069),(#203070,#203071),
(#203072,#203073),(#203074,#203075),(#203076,#203077),(#203078,#203079),
(#203080,#203081),(#203082,#203083),(#203084,#203085),(#203086,#203087),
(#203088,#203089),(#203090,#203091),(#203092,#203093),(#203094,#203095),
(#203096,#203097),(#203098,#203099),(#203100,#203101),(#203102,#203103),
(#203104,#203105),(#203106,#203107),(#203108,#203109),(#203110,#203111),
(#203112,#203113),(#203114,#203115),(#203116,#203117),(#203118,#203119),
(#203120,#203121),(#203122,#203123),(#203124,#203125),(#203126,#203127),
(#203128,#203129),(#203130,#203131),(#203132,#203133),(#203134,#203135),
(#203136,#203137),(#203138,#203139),(#203140,#203141),(#203142,#203143),
(#203144,#203145),(#203146,#203147),(#203148,#203149),(#203150,#203151),
(#203152,#203153),(#203154,#203155),(#203156,#203157),(#203158,#203159),
(#203160,#203161),(#203162,#203163),(#203164,#203165),(#203166,#203167),
(#203168,#203169),(#203170,#203171),(#203172,#203173),(#203174,#203175),
(#203176,#203177),(#203178,#203179),(#203180,#203181),(#203182,#203183),
(#203184,#203185),(#203186,#203187),(#203188,#203189),(#203190,#203191),
(#203192,#203193),(#203194,#203195),(#203196,#203197),(#203198,#203199),
(#203200,#203201),(#203202,#203203),(#203204,#203205),(#203206,#203207),
(#203208,#203209),(#203210,#203211),(#203212,#203213),(#203214,#203215),
(#203216,#203217),(#203218,#203219),(#203220,#203221),(#203222,#203223),
(#203224,#203225),(#203226,#203227),(#203228,#203229),(#203230,#203231),
(#203232,#203233),(#203234,#203235),(#203236,#203237),(#203238,#203239),
(#203240,#203241),(#203242,#203243),(#203244,#203245),(#203246,#203247),
(#203248,#203249),(#203250,#203251),(#203252,#203253),(#203254,#203255),
(#203256,#203257),(#203258,#203259),(#203260,#203261),(#203262,#203263),
(#203264,#203265),(#203266,#203267),(#203268,#203269),(#203270,#203271),
(#203272,#203273),(#203274,#203275),(#203276,#203277),(#203278,#203279),
(#203280,#203281),(#203282,#203283),(#203284,#203285),(#203286,#203287),
(#203288,#203289),(#203290,#203291),(#203292,#203293),(#203294,#203295),
(#203296,#203297),(#203298,#203299),(#203300,#203301),(#203302,#203303),
(#203304,#203305),(#203306,#203307),(#203308,#203309),(#203310,#203311),
(#203312,#203313),(#203314,#203315),(#203316,#203317),(#203318,#203319),
(#203320,#203321),(#203322,#203323),(#203324,#203325),(#203326,#203327),
(#203328,#203329),(#203330,#203331),(#203332,#203333),(#203334,#203335),
(#203336,#203337),(#203338,#203339),(#203340,#203341),(#203342,#203343),
(#203344,#203345),(#203346,#203347),(#203348,#203349),(#203350,#203351),
(#203352,#203353),(#203354,#203355),(#203356,#203357),(#203358,#203359),
(#203360,#203361),(#203362,#203363),(#203364,#203365),(#203366,#203367),
(#203368,#203369),(#203370,#203371),(#203372,#203373),(#203374,#203375),
(#203376,#203377),(#203378,#203379),(#203380,#203381),(#203382,#203383),
(#203384,#203385),(#203386,#203387),(#203388,#203389),(#203390,#203391),
(#203392,#203393),(#203394,#203395),(#203396,#203397),(#203398,#203399),
(#203400,#203401),(#203402,#203403),(#203404,#203405),(#203406,#203407),
(#203408,#203409),(#203410,#203411),(#203412,#203413),(#203414,#203415),
(#203416,#203417),(#203418,#203419),(#203420,#203421),(#203422,#203423),
(#203424,#203425),(#203426,#203427),(#203428,#203429),(#203430,#203431),
(#203432,#203433),(#203434,#203435),(#203436,#203437),(#203438,#203439),
(#203440,#203441),(#203442,#203443),(#203444,#203445),(#203446,#203447),
(#203448,#203449),(#203450,#203451),(#203452,#203453),(#203454,#203455),
(#203456,#203457),(#203458,#203459),(#203460,#203461),(#203462,#203463),
(#203464,#203465),(#203466,#203467),(#203468,#203469),(#203470,#203471),
(#203472,#203473),(#203474,#203475),(#203476,#203477),(#203478,#203479),
(#203480,#203481),(#203482,#203483),(#203484,#203485),(#203486,#203487),
(#203488,#203489),(#203490,#203491),(#203492,#203493),(#203494,#203495),
(#203496,#203497),(#203498,#203499),(#203500,#203501),(#203502,#203503),
(#203504,#203505),(#203506,#203507),(#203508,#203509),(#203510,#203511),
(#203512,#203513),(#203514,#203515),(#203516,#203517),(#203518,#203519),
(#203520,#203521),(#203522,#203523),(#203524,#203525),(#203526,#203527),
(#203528,#203529),(#203530,#203531),(#203532,#203533),(#203534,#203535),
(#203536,#203537),(#203538,#203539),(#203540,#203541),(#203542,#203543),
(#203544,#203545),(#203546,#203547),(#203548,#203549),(#203550,#203551),
(#203552,#203553),(#203554,#203555),(#203556,#203557),(#203558,#203559),
(#203560,#203561),(#203562,#203563),(#203564,#203565),(#203566,#203567),
(#203568,#203569),(#203570,#203571),(#203572,#203573),(#203574,#203575),
(#203576,#203577),(#203578,#203579),(#203580,#203581),(#203582,#203583),
(#203584,#203585),(#203586,#203587),(#203588,#203589),(#203590,#203591),
(#203592,#203593),(#203594,#203595),(#203596,#203597),(#203598,#203599),
(#203600,#203601),(#203602,#203603),(#203604,#203605),(#203606,#203607),
(#203608,#203609),(#203610,#203611),(#203612,#203613),(#203614,#203615),
(#203616,#203617),(#203618,#203619),(#203620,#203621),(#203622,#203623),
(#203624,#203625),(#203626,#203627),(#203628,#203629),(#203630,#203631),
(#203632,#203633),(#203634,#203635),(#203636,#203637),(#203638,#203639),
(#203640,#203641),(#203642,#203643)),.UNSPECIFIED.,.F.,.F.,.F.,(6,1,1,1,
1,1,1,1,1,1,1,1,1,1,1,1,1,1,1,1,1,1,1,1,1,1,1,1,1,1,1,1,1,1,1,1,1,1,1,1,
1,1,1,1,1,1,1,1,1,1,1,1,1,1,1,1,1,1,1,1,1,1,1,1,1,1,1,1,1,1,1,1,1,1,1,1,
1,1,1,1,1,1,1,1,1,1,1,1,1,1,1,1,1,1,1,1,1,1,1,1,1,1,1,1,1,1,1,1,1,1,1,1,
1,1,1,1,1,1,1,1,1,1,1,1,1,1,1,1,1,1,1,1,1,1,1,1,1,1,1,1,1,1,1,1,1,1,1,1,
1,1,1,1,1,1,1,1,1,1,1,1,1,1,1,1,1,1,1,1,1,1,1,1,1,1,1,1,1,1,1,1,1,1,1,1,
1,1,1,1,1,1,1,1,1,1,1,1,1,1,1,1,1,1,1,1,1,1,1,1,1,1,1,1,1,1,1,1,1,1,1,1,
1,1,1,1,1,1,1,1,1,1,1,1,1,1,1,1,1,1,1,1,1,1,1,1,1,1,1,1,1,1,1,1,1,1,1,1,
1,1,1,1,1,1,1,1,1,1,1,1,1,1,1,1,1,1,1,1,1,1,1,1,1,1,1,1,1,1,1,1,1,1,1,1,
1,1,1,1,1,1,1,1,1,1,1,1,1,1,1,1,1,1,1,1,1,1,1,1,1,1,1,1,1,1,1,1,1,1,1,1,
1,1,1,1,1,1,1,1,1,1,1,1,1,1,1,1,1,1,1,1,1,1,1,1,1,1,1,1,1,1,1,1,1,1,1,1,
1,1,1,1,1,1,1,1,1,1,1,1,1,1,1,1,1,1,1,1,1,1,1,1,1,1,1,1,1,1,1,1,1,1,1,1,
1,1,1,1,1,1,1,1,1,1,1,1,1,1,1,1,1,1,1,1,1,1,1,1,1,1,1,1,1,1,1,1,1,1,1,1,
1,1,1,1,1,1,1,1,1,1,1,1,1,1,1,1,1,1,1,1,1,1,1,1,1,1,1,1,1,1,1,6),(2,2),
(-1.,-0.998165138,-0.996330275,-0.994495413,-0.99266055,-0.990825688,-0.988990826,
-0.987155963,-0.985321101,-0.983486239,-0.981651376,-0.979816514,-0.977981651,
-0.976146789,-0.974311927,-0.972477064,-0.970642202,-0.968807339,-0.966972477,
-0.965137615,-0.963302752,-0.96146789,-0.959633028,-0.957798165,-0.955963303,
-0.95412844,-0.952293578,-0.950458716,-0.948623853,-0.946788991,-0.944954128,
-0.943119266,-0.941284404,-0.939449541,-0.937614679,-0.935779817,-0.933944954,
-0.932110092,-0.930275229,-0.928440367,-0.926605505,-0.924770642,-0.92293578,
-0.921100917,-0.919266055,-0.917431193,-0.91559633,-0.913761468,-0.911926606,
-0.910091743,-0.908256881,-0.906422018,-0.904587156,-0.902752294,-0.900917431,
-0.899082569,-0.897247706,-0.895412844,-0.893577982,-0.891743119,-0.889908257,
-0.888073394,-0.886238532,-0.88440367,-0.882568807,-0.880733945,-0.878899083,
-0.87706422,-0.875229358,-0.873394495,-0.871559633,-0.869724771,-0.867889908,
-0.866055046,-0.864220183,-0.862385321,-0.860550459,-0.858715596,-0.856880734,
-0.855045872,-0.853211009,-0.851376147,-0.849541284,-0.847706422,-0.84587156,
-0.844036697,-0.842201835,-0.840366972,-0.83853211,-0.836697248,-0.834862385,
-0.833027523,-0.831192661,-0.829357798,-0.827522936,-0.825688073,-0.823853211,
-0.822018349,-0.820183486,-0.818348624,-0.816513761,-0.814678899,-0.812844037,
-0.811009174,-0.809174312,-0.80733945,-0.805504587,-0.803669725,-0.801834862,
-0.8,-0.798165138,-0.796330275,-0.794495413,-0.79266055,-0.790825688,-0.788990826,
-0.787155963,-0.785321101,-0.783486239,-0.781651376,-0.779816514,-0.777981651,
-0.776146789,-0.774311927,-0.772477064,-0.770642202,-0.768807339,-0.766972477,
-0.765137615,-0.763302752,-0.76146789,-0.759633028,-0.757798165,-0.755963303,
-0.75412844,-0.752293578,-0.750458716,-0.748623853,-0.746788991,-0.744954128,
-0.743119266,-0.741284404,-0.739449541,-0.737614679,-0.735779817,-0.733944954,
-0.732110092,-0.730275229,-0.728440367,-0.726605505,-0.724770642,-0.72293578,
-0.721100917,-0.719266055,-0.717431193,-0.71559633,-0.713761468,-0.711926606,
-0.710091743,-0.708256881,-0.706422018,-0.704587156,-0.702752294,-0.700917431,
-0.699082569,-0.697247706,-0.695412844,-0.693577982,-0.691743119,-0.689908257,
-0.688073394,-0.686238532,-0.68440367,-0.682568807,-0.680733945,-0.678899083,
-0.67706422,-0.675229358,-0.673394495,-0.671559633,-0.669724771,-0.667889908,
-0.666055046,-0.664220183,-0.662385321,-0.660550459,-0.658715596,-0.656880734,
-0.655045872,-0.653211009,-0.651376147,-0.649541284,-0.647706422,-0.64587156,
-0.644036697,-0.642201835,-0.640366972,-0.63853211,-0.636697248,-0.634862385,
-0.633027523,-0.631192661,-0.629357798,-0.627522936,-0.625688073,-0.623853211,
-0.622018349,-0.620183486,-0.618348624,-0.616513761,-0.614678899,-0.612844037,
-0.611009174,-0.609174312,-0.60733945,-0.605504587,-0.603669725,-0.601834862,
-0.6,-0.598165138,-0.596330275,-0.594495413,-0.59266055,-0.590825688,-0.588990826,
-0.587155963,-0.585321101,-0.583486239,-0.581651376,-0.579816514,-0.577981651,
-0.576146789,-0.574311927,-0.572477064,-0.570642202,-0.568807339,-0.566972477,
-0.565137615,-0.563302752,-0.56146789,-0.559633028,-0.557798165,-0.555963303,
-0.55412844,-0.552293578,-0.550458716,-0.548623853,-0.546788991,-0.544954128,
-0.543119266,-0.541284404,-0.539449541,-0.537614679,-0.535779817,-0.533944954,
-0.532110092,-0.530275229,-0.528440367,-0.526605505,-0.524770642,-0.52293578,
-0.521100917,-0.519266055,-0.517431193,-0.51559633,-0.513761468,-0.511926606,
-0.510091743,-0.508256881,-0.506422018,-0.504587156,-0.502752294,-0.500917431,
-0.499082569,-0.497247706,-0.495412844,-0.493577982,-0.491743119,-0.489908257,
-0.488073394,-0.486238532,-0.48440367,-0.482568807,-0.480733945,-0.478899083,
-0.47706422,-0.475229358,-0.473394495,-0.471559633,-0.469724771,-0.467889908,
-0.466055046,-0.464220183,-0.462385321,-0.460550459,-0.458715596,-0.456880734,
-0.455045872,-0.453211009,-0.451376147,-0.449541284,-0.447706422,-0.44587156,
-0.444036697,-0.442201835,-0.440366972,-0.43853211,-0.436697248,-0.434862385,
-0.433027523,-0.431192661,-0.429357798,-0.427522936,-0.425688073,-0.423853211,
-0.422018349,-0.420183486,-0.418348624,-0.416513761,-0.414678899,-0.412844037,
-0.411009174,-0.409174312,-0.40733945,-0.405504587,-0.403669725,-0.401834862,
-0.4,-0.398165138,-0.396330275,-0.394495413,-0.39266055,-0.390825688,-0.388990826,
-0.387155963,-0.385321101,-0.383486239,-0.381651376,-0.379816514,-0.377981651,
-0.376146789,-0.374311927,-0.372477064,-0.370642202,-0.368807339,-0.366972477,
-0.365137615,-0.363302752,-0.36146789,-0.359633028,-0.357798165,-0.355963303,
-0.35412844,-0.352293578,-0.350458716,-0.348623853,-0.346788991,-0.344954128,
-0.343119266,-0.341284404,-0.339449541,-0.337614679,-0.335779817,-0.333944954,
-0.332110092,-0.330275229,-0.328440367,-0.326605505,-0.324770642,-0.32293578,
-0.321100917,-0.319266055,-0.317431193,-0.31559633,-0.313761468,-0.311926606,
-0.310091743,-0.308256881,-0.306422018,-0.304587156,-0.302752294,-0.300917431,
-0.299082569,-0.297247706,-0.295412844,-0.293577982,-0.291743119,-0.289908257,
-0.288073394,-0.286238532,-0.28440367,-0.282568807,-0.280733945,-0.278899083,
-0.27706422,-0.275229358,-0.273394495,-0.271559633,-0.269724771,-0.267889908,
-0.266055046,-0.264220183,-0.262385321,-0.260550459,-0.258715596,-0.256880734,
-0.255045872,-0.253211009,-0.251376147,-0.249541284,-0.247706422,-0.24587156,
-0.244036697,-0.242201835,-0.240366972,-0.23853211,-0.236697248,-0.234862385,
-0.233027523,-0.231192661,-0.229357798,-0.227522936,-0.225688073,-0.223853211,
-0.222018349,-0.220183486,-0.218348624,-0.216513761,-0.214678899,-0.212844037,
-0.211009174,-0.209174312,-0.20733945,-0.205504587,-0.203669725,-0.201834862,
-0.2,-0.198165138,-0.196330275,-0.194495413,-0.19266055,-0.190825688,-0.188990826,
-0.187155963,-0.185321101,-0.183486239,-0.181651376,-0.179816514,-0.177981651,
-0.176146789,-0.174311927,-0.172477064,-0.170642202,-0.168807339,-0.166972477,
-0.165137615,-0.163302752,-0.16146789,-0.159633028,-0.157798165,-0.155963303,
-0.15412844,-0.152293578,-0.150458716,-0.148623853,-0.146788991,-0.144954128,
-0.143172103),(0.,0.36),.UNSPECIFIED.);
#6245=B_SPLINE_SURFACE_WITH_KNOTS('',5,1,((#204294,#204295),(#204296,#204297),
(#204298,#204299),(#204300,#204301),(#204302,#204303),(#204304,#204305),
(#204306,#204307),(#204308,#204309),(#204310,#204311),(#204312,#204313),
(#204314,#204315),(#204316,#204317),(#204318,#204319),(#204320,#204321),
(#204322,#204323),(#204324,#204325),(#204326,#204327),(#204328,#204329),
(#204330,#204331),(#204332,#204333),(#204334,#204335),(#204336,#204337),
(#204338,#204339),(#204340,#204341),(#204342,#204343),(#204344,#204345),
(#204346,#204347),(#204348,#204349),(#204350,#204351),(#204352,#204353),
(#204354,#204355),(#204356,#204357),(#204358,#204359),(#204360,#204361),
(#204362,#204363),(#204364,#204365),(#204366,#204367),(#204368,#204369),
(#204370,#204371),(#204372,#204373),(#204374,#204375),(#204376,#204377),
(#204378,#204379),(#204380,#204381),(#204382,#204383),(#204384,#204385),
(#204386,#204387),(#204388,#204389),(#204390,#204391),(#204392,#204393),
(#204394,#204395),(#204396,#204397),(#204398,#204399),(#204400,#204401),
(#204402,#204403),(#204404,#204405),(#204406,#204407),(#204408,#204409),
(#204410,#204411),(#204412,#204413),(#204414,#204415),(#204416,#204417),
(#204418,#204419),(#204420,#204421),(#204422,#204423),(#204424,#204425),
(#204426,#204427),(#204428,#204429),(#204430,#204431),(#204432,#204433),
(#204434,#204435),(#204436,#204437),(#204438,#204439),(#204440,#204441),
(#204442,#204443),(#204444,#204445),(#204446,#204447),(#204448,#204449),
(#204450,#204451),(#204452,#204453),(#204454,#204455),(#204456,#204457),
(#204458,#204459),(#204460,#204461),(#204462,#204463),(#204464,#204465),
(#204466,#204467),(#204468,#204469),(#204470,#204471),(#204472,#204473),
(#204474,#204475),(#204476,#204477),(#204478,#204479),(#204480,#204481),
(#204482,#204483),(#204484,#204485),(#204486,#204487),(#204488,#204489),
(#204490,#204491),(#204492,#204493),(#204494,#204495),(#204496,#204497),
(#204498,#204499),(#204500,#204501),(#204502,#204503),(#204504,#204505),
(#204506,#204507),(#204508,#204509),(#204510,#204511),(#204512,#204513),
(#204514,#204515),(#204516,#204517),(#204518,#204519),(#204520,#204521),
(#204522,#204523),(#204524,#204525),(#204526,#204527),(#204528,#204529),
(#204530,#204531),(#204532,#204533),(#204534,#204535),(#204536,#204537),
(#204538,#204539),(#204540,#204541),(#204542,#204543),(#204544,#204545),
(#204546,#204547),(#204548,#204549),(#204550,#204551),(#204552,#204553),
(#204554,#204555),(#204556,#204557),(#204558,#204559),(#204560,#204561),
(#204562,#204563),(#204564,#204565),(#204566,#204567),(#204568,#204569),
(#204570,#204571),(#204572,#204573),(#204574,#204575),(#204576,#204577),
(#204578,#204579),(#204580,#204581),(#204582,#204583),(#204584,#204585),
(#204586,#204587),(#204588,#204589),(#204590,#204591),(#204592,#204593),
(#204594,#204595),(#204596,#204597),(#204598,#204599),(#204600,#204601),
(#204602,#204603),(#204604,#204605),(#204606,#204607),(#204608,#204609),
(#204610,#204611),(#204612,#204613),(#204614,#204615),(#204616,#204617),
(#204618,#204619),(#204620,#204621),(#204622,#204623),(#204624,#204625),
(#204626,#204627),(#204628,#204629),(#204630,#204631),(#204632,#204633),
(#204634,#204635),(#204636,#204637),(#204638,#204639),(#204640,#204641),
(#204642,#204643),(#204644,#204645),(#204646,#204647),(#204648,#204649),
(#204650,#204651),(#204652,#204653),(#204654,#204655),(#204656,#204657),
(#204658,#204659),(#204660,#204661),(#204662,#204663),(#204664,#204665),
(#204666,#204667),(#204668,#204669),(#204670,#204671),(#204672,#204673),
(#204674,#204675),(#204676,#204677),(#204678,#204679),(#204680,#204681),
(#204682,#204683),(#204684,#204685),(#204686,#204687),(#204688,#204689),
(#204690,#204691),(#204692,#204693),(#204694,#204695),(#204696,#204697),
(#204698,#204699),(#204700,#204701),(#204702,#204703),(#204704,#204705),
(#204706,#204707),(#204708,#204709),(#204710,#204711),(#204712,#204713),
(#204714,#204715),(#204716,#204717),(#204718,#204719),(#204720,#204721),
(#204722,#204723),(#204724,#204725),(#204726,#204727),(#204728,#204729),
(#204730,#204731),(#204732,#204733),(#204734,#204735),(#204736,#204737),
(#204738,#204739),(#204740,#204741),(#204742,#204743),(#204744,#204745),
(#204746,#204747),(#204748,#204749),(#204750,#204751),(#204752,#204753),
(#204754,#204755),(#204756,#204757),(#204758,#204759),(#204760,#204761),
(#204762,#204763),(#204764,#204765),(#204766,#204767),(#204768,#204769),
(#204770,#204771),(#204772,#204773),(#204774,#204775),(#204776,#204777),
(#204778,#204779),(#204780,#204781),(#204782,#204783),(#204784,#204785),
(#204786,#204787),(#204788,#204789),(#204790,#204791),(#204792,#204793),
(#204794,#204795),(#204796,#204797),(#204798,#204799),(#204800,#204801),
(#204802,#204803),(#204804,#204805),(#204806,#204807),(#204808,#204809),
(#204810,#204811),(#204812,#204813),(#204814,#204815),(#204816,#204817),
(#204818,#204819),(#204820,#204821),(#204822,#204823),(#204824,#204825),
(#204826,#204827),(#204828,#204829),(#204830,#204831),(#204832,#204833),
(#204834,#204835),(#204836,#204837),(#204838,#204839),(#204840,#204841),
(#204842,#204843),(#204844,#204845),(#204846,#204847),(#204848,#204849),
(#204850,#204851),(#204852,#204853),(#204854,#204855),(#204856,#204857),
(#204858,#204859),(#204860,#204861),(#204862,#204863),(#204864,#204865),
(#204866,#204867),(#204868,#204869),(#204870,#204871),(#204872,#204873),
(#204874,#204875),(#204876,#204877),(#204878,#204879),(#204880,#204881),
(#204882,#204883),(#204884,#204885),(#204886,#204887),(#204888,#204889),
(#204890,#204891),(#204892,#204893),(#204894,#204895),(#204896,#204897),
(#204898,#204899),(#204900,#204901),(#204902,#204903),(#204904,#204905),
(#204906,#204907),(#204908,#204909),(#204910,#204911),(#204912,#204913),
(#204914,#204915),(#204916,#204917),(#204918,#204919),(#204920,#204921),
(#204922,#204923),(#204924,#204925),(#204926,#204927),(#204928,#204929),
(#204930,#204931),(#204932,#204933),(#204934,#204935),(#204936,#204937),
(#204938,#204939),(#204940,#204941),(#204942,#204943),(#204944,#204945),
(#204946,#204947),(#204948,#204949),(#204950,#204951),(#204952,#204953),
(#204954,#204955),(#204956,#204957),(#204958,#204959),(#204960,#204961),
(#204962,#204963),(#204964,#204965),(#204966,#204967),(#204968,#204969),
(#204970,#204971),(#204972,#204973),(#204974,#204975),(#204976,#204977),
(#204978,#204979),(#204980,#204981),(#204982,#204983),(#204984,#204985),
(#204986,#204987),(#204988,#204989),(#204990,#204991),(#204992,#204993),
(#204994,#204995),(#204996,#204997),(#204998,#204999),(#205000,#205001),
(#205002,#205003),(#205004,#205005),(#205006,#205007),(#205008,#205009),
(#205010,#205011),(#205012,#205013),(#205014,#205015),(#205016,#205017),
(#205018,#205019),(#205020,#205021),(#205022,#205023),(#205024,#205025),
(#205026,#205027),(#205028,#205029),(#205030,#205031),(#205032,#205033),
(#205034,#205035),(#205036,#205037),(#205038,#205039),(#205040,#205041),
(#205042,#205043),(#205044,#205045),(#205046,#205047),(#205048,#205049),
(#205050,#205051),(#205052,#205053),(#205054,#205055),(#205056,#205057),
(#205058,#205059),(#205060,#205061),(#205062,#205063),(#205064,#205065),
(#205066,#205067),(#205068,#205069),(#205070,#205071),(#205072,#205073),
(#205074,#205075),(#205076,#205077),(#205078,#205079),(#205080,#205081),
(#205082,#205083),(#205084,#205085),(#205086,#205087),(#205088,#205089),
(#205090,#205091),(#205092,#205093),(#205094,#205095),(#205096,#205097),
(#205098,#205099),(#205100,#205101),(#205102,#205103),(#205104,#205105),
(#205106,#205107),(#205108,#205109),(#205110,#205111),(#205112,#205113),
(#205114,#205115),(#205116,#205117),(#205118,#205119),(#205120,#205121),
(#205122,#205123),(#205124,#205125),(#205126,#205127),(#205128,#205129),
(#205130,#205131),(#205132,#205133),(#205134,#205135),(#205136,#205137),
(#205138,#205139),(#205140,#205141),(#205142,#205143),(#205144,#205145),
(#205146,#205147),(#205148,#205149),(#205150,#205151),(#205152,#205153),
(#205154,#205155),(#205156,#205157),(#205158,#205159),(#205160,#205161),
(#205162,#205163),(#205164,#205165),(#205166,#205167),(#205168,#205169),
(#205170,#205171),(#205172,#205173),(#205174,#205175),(#205176,#205177),
(#205178,#205179),(#205180,#205181),(#205182,#205183),(#205184,#205185),
(#205186,#205187),(#205188,#205189),(#205190,#205191),(#205192,#205193),
(#205194,#205195),(#205196,#205197),(#205198,#205199),(#205200,#205201),
(#205202,#205203),(#205204,#205205),(#205206,#205207),(#205208,#205209),
(#205210,#205211),(#205212,#205213),(#205214,#205215),(#205216,#205217),
(#205218,#205219),(#205220,#205221),(#205222,#205223),(#205224,#205225),
(#205226,#205227),(#205228,#205229),(#205230,#205231),(#205232,#205233),
(#205234,#205235),(#205236,#205237)),.UNSPECIFIED.,.F.,.F.,.F.,(6,1,1,1,
1,1,1,1,1,1,1,1,1,1,1,1,1,1,1,1,1,1,1,1,1,1,1,1,1,1,1,1,1,1,1,1,1,1,1,1,
1,1,1,1,1,1,1,1,1,1,1,1,1,1,1,1,1,1,1,1,1,1,1,1,1,1,1,1,1,1,1,1,1,1,1,1,
1,1,1,1,1,1,1,1,1,1,1,1,1,1,1,1,1,1,1,1,1,1,1,1,1,1,1,1,1,1,1,1,1,1,1,1,
1,1,1,1,1,1,1,1,1,1,1,1,1,1,1,1,1,1,1,1,1,1,1,1,1,1,1,1,1,1,1,1,1,1,1,1,
1,1,1,1,1,1,1,1,1,1,1,1,1,1,1,1,1,1,1,1,1,1,1,1,1,1,1,1,1,1,1,1,1,1,1,1,
1,1,1,1,1,1,1,1,1,1,1,1,1,1,1,1,1,1,1,1,1,1,1,1,1,1,1,1,1,1,1,1,1,1,1,1,
1,1,1,1,1,1,1,1,1,1,1,1,1,1,1,1,1,1,1,1,1,1,1,1,1,1,1,1,1,1,1,1,1,1,1,1,
1,1,1,1,1,1,1,1,1,1,1,1,1,1,1,1,1,1,1,1,1,1,1,1,1,1,1,1,1,1,1,1,1,1,1,1,
1,1,1,1,1,1,1,1,1,1,1,1,1,1,1,1,1,1,1,1,1,1,1,1,1,1,1,1,1,1,1,1,1,1,1,1,
1,1,1,1,1,1,1,1,1,1,1,1,1,1,1,1,1,1,1,1,1,1,1,1,1,1,1,1,1,1,1,1,1,1,1,1,
1,1,1,1,1,1,1,1,1,1,1,1,1,1,1,1,1,1,1,1,1,1,1,1,1,1,1,1,1,1,1,1,1,1,1,1,
1,1,1,1,1,1,1,1,1,1,1,1,1,1,1,1,1,1,1,1,1,1,1,1,1,1,1,1,1,1,1,1,1,1,1,1,
1,1,1,1,1,1,1,1,1,1,1,1,1,1,1,1,1,1,1,1,1,1,1,1,1,1,1,1,1,1,1,6),(2,2),
(-1.,-0.998165138,-0.996330275,-0.994495413,-0.99266055,-0.990825688,-0.988990826,
-0.987155963,-0.985321101,-0.983486239,-0.981651376,-0.979816514,-0.977981651,
-0.976146789,-0.974311927,-0.972477064,-0.970642202,-0.968807339,-0.966972477,
-0.965137615,-0.963302752,-0.96146789,-0.959633028,-0.957798165,-0.955963303,
-0.95412844,-0.952293578,-0.950458716,-0.948623853,-0.946788991,-0.944954128,
-0.943119266,-0.941284404,-0.939449541,-0.937614679,-0.935779817,-0.933944954,
-0.932110092,-0.930275229,-0.928440367,-0.926605505,-0.924770642,-0.92293578,
-0.921100917,-0.919266055,-0.917431193,-0.91559633,-0.913761468,-0.911926606,
-0.910091743,-0.908256881,-0.906422018,-0.904587156,-0.902752294,-0.900917431,
-0.899082569,-0.897247706,-0.895412844,-0.893577982,-0.891743119,-0.889908257,
-0.888073394,-0.886238532,-0.88440367,-0.882568807,-0.880733945,-0.878899083,
-0.87706422,-0.875229358,-0.873394495,-0.871559633,-0.869724771,-0.867889908,
-0.866055046,-0.864220183,-0.862385321,-0.860550459,-0.858715596,-0.856880734,
-0.855045872,-0.853211009,-0.851376147,-0.849541284,-0.847706422,-0.84587156,
-0.844036697,-0.842201835,-0.840366972,-0.83853211,-0.836697248,-0.834862385,
-0.833027523,-0.831192661,-0.829357798,-0.827522936,-0.825688073,-0.823853211,
-0.822018349,-0.820183486,-0.818348624,-0.816513761,-0.814678899,-0.812844037,
-0.811009174,-0.809174312,-0.80733945,-0.805504587,-0.803669725,-0.801834862,
-0.8,-0.798165138,-0.796330275,-0.794495413,-0.79266055,-0.790825688,-0.788990826,
-0.787155963,-0.785321101,-0.783486239,-0.781651376,-0.779816514,-0.777981651,
-0.776146789,-0.774311927,-0.772477064,-0.770642202,-0.768807339,-0.766972477,
-0.765137615,-0.763302752,-0.76146789,-0.759633028,-0.757798165,-0.755963303,
-0.75412844,-0.752293578,-0.750458716,-0.748623853,-0.746788991,-0.744954128,
-0.743119266,-0.741284404,-0.739449541,-0.737614679,-0.735779817,-0.733944954,
-0.732110092,-0.730275229,-0.728440367,-0.726605505,-0.724770642,-0.72293578,
-0.721100917,-0.719266055,-0.717431193,-0.71559633,-0.713761468,-0.711926606,
-0.710091743,-0.708256881,-0.706422018,-0.704587156,-0.702752294,-0.700917431,
-0.699082569,-0.697247706,-0.695412844,-0.693577982,-0.691743119,-0.689908257,
-0.688073394,-0.686238532,-0.68440367,-0.682568807,-0.680733945,-0.678899083,
-0.67706422,-0.675229358,-0.673394495,-0.671559633,-0.669724771,-0.667889908,
-0.666055046,-0.664220183,-0.662385321,-0.660550459,-0.658715596,-0.656880734,
-0.655045872,-0.653211009,-0.651376147,-0.649541284,-0.647706422,-0.64587156,
-0.644036697,-0.642201835,-0.640366972,-0.63853211,-0.636697248,-0.634862385,
-0.633027523,-0.631192661,-0.629357798,-0.627522936,-0.625688073,-0.623853211,
-0.622018349,-0.620183486,-0.618348624,-0.616513761,-0.614678899,-0.612844037,
-0.611009174,-0.609174312,-0.60733945,-0.605504587,-0.603669725,-0.601834862,
-0.6,-0.598165138,-0.596330275,-0.594495413,-0.59266055,-0.590825688,-0.588990826,
-0.587155963,-0.585321101,-0.583486239,-0.581651376,-0.579816514,-0.577981651,
-0.576146789,-0.574311927,-0.572477064,-0.570642202,-0.568807339,-0.566972477,
-0.565137615,-0.563302752,-0.56146789,-0.559633028,-0.557798165,-0.555963303,
-0.55412844,-0.552293578,-0.550458716,-0.548623853,-0.546788991,-0.544954128,
-0.543119266,-0.541284404,-0.539449541,-0.537614679,-0.535779817,-0.533944954,
-0.532110092,-0.530275229,-0.528440367,-0.526605505,-0.524770642,-0.52293578,
-0.521100917,-0.519266055,-0.517431193,-0.51559633,-0.513761468,-0.511926606,
-0.510091743,-0.508256881,-0.506422018,-0.504587156,-0.502752294,-0.500917431,
-0.499082569,-0.497247706,-0.495412844,-0.493577982,-0.491743119,-0.489908257,
-0.488073394,-0.486238532,-0.48440367,-0.482568807,-0.480733945,-0.478899083,
-0.47706422,-0.475229358,-0.473394495,-0.471559633,-0.469724771,-0.467889908,
-0.466055046,-0.464220183,-0.462385321,-0.460550459,-0.458715596,-0.456880734,
-0.455045872,-0.453211009,-0.451376147,-0.449541284,-0.447706422,-0.44587156,
-0.444036697,-0.442201835,-0.440366972,-0.43853211,-0.436697248,-0.434862385,
-0.433027523,-0.431192661,-0.429357798,-0.427522936,-0.425688073,-0.423853211,
-0.422018349,-0.420183486,-0.418348624,-0.416513761,-0.414678899,-0.412844037,
-0.411009174,-0.409174312,-0.40733945,-0.405504587,-0.403669725,-0.401834862,
-0.4,-0.398165138,-0.396330275,-0.394495413,-0.39266055,-0.390825688,-0.388990826,
-0.387155963,-0.385321101,-0.383486239,-0.381651376,-0.379816514,-0.377981651,
-0.376146789,-0.374311927,-0.372477064,-0.370642202,-0.368807339,-0.366972477,
-0.365137615,-0.363302752,-0.36146789,-0.359633028,-0.357798165,-0.355963303,
-0.35412844,-0.352293578,-0.350458716,-0.348623853,-0.346788991,-0.344954128,
-0.343119266,-0.341284404,-0.339449541,-0.337614679,-0.335779817,-0.333944954,
-0.332110092,-0.330275229,-0.328440367,-0.326605505,-0.324770642,-0.32293578,
-0.321100917,-0.319266055,-0.317431193,-0.31559633,-0.313761468,-0.311926606,
-0.310091743,-0.308256881,-0.306422018,-0.304587156,-0.302752294,-0.300917431,
-0.299082569,-0.297247706,-0.295412844,-0.293577982,-0.291743119,-0.289908257,
-0.288073394,-0.286238532,-0.28440367,-0.282568807,-0.280733945,-0.278899083,
-0.27706422,-0.275229358,-0.273394495,-0.271559633,-0.269724771,-0.267889908,
-0.266055046,-0.264220183,-0.262385321,-0.260550459,-0.258715596,-0.256880734,
-0.255045872,-0.253211009,-0.251376147,-0.249541284,-0.247706422,-0.24587156,
-0.244036697,-0.242201835,-0.240366972,-0.23853211,-0.236697248,-0.234862385,
-0.233027523,-0.231192661,-0.229357798,-0.227522936,-0.225688073,-0.223853211,
-0.222018349,-0.220183486,-0.218348624,-0.216513761,-0.214678899,-0.212844037,
-0.211009174,-0.209174312,-0.20733945,-0.205504587,-0.203669725,-0.201834862,
-0.2,-0.198165138,-0.196330275,-0.194495413,-0.19266055,-0.190825688,-0.188990826,
-0.187155963,-0.185321101,-0.183486239,-0.181651376,-0.179816514,-0.177981651,
-0.176146789,-0.174311927,-0.172477064,-0.170642202,-0.168807339,-0.166972477,
-0.165137615,-0.163302752,-0.16146789,-0.159633028,-0.157798165,-0.155963303,
-0.15412844,-0.152293578,-0.150458716,-0.148623853,-0.146788991,-0.144954128,
-0.143172103),(0.,0.36),.UNSPECIFIED.);
#6246=B_SPLINE_SURFACE_WITH_KNOTS('',5,1,((#205867,#205868),(#205869,#205870),
(#205871,#205872),(#205873,#205874),(#205875,#205876),(#205877,#205878),
(#205879,#205880),(#205881,#205882),(#205883,#205884),(#205885,#205886),
(#205887,#205888),(#205889,#205890),(#205891,#205892),(#205893,#205894),
(#205895,#205896),(#205897,#205898),(#205899,#205900),(#205901,#205902),
(#205903,#205904),(#205905,#205906),(#205907,#205908),(#205909,#205910),
(#205911,#205912),(#205913,#205914),(#205915,#205916),(#205917,#205918),
(#205919,#205920),(#205921,#205922),(#205923,#205924),(#205925,#205926),
(#205927,#205928),(#205929,#205930),(#205931,#205932),(#205933,#205934),
(#205935,#205936),(#205937,#205938),(#205939,#205940),(#205941,#205942),
(#205943,#205944),(#205945,#205946),(#205947,#205948),(#205949,#205950),
(#205951,#205952),(#205953,#205954),(#205955,#205956),(#205957,#205958),
(#205959,#205960),(#205961,#205962),(#205963,#205964),(#205965,#205966),
(#205967,#205968),(#205969,#205970),(#205971,#205972),(#205973,#205974),
(#205975,#205976),(#205977,#205978),(#205979,#205980),(#205981,#205982),
(#205983,#205984),(#205985,#205986),(#205987,#205988),(#205989,#205990),
(#205991,#205992),(#205993,#205994),(#205995,#205996),(#205997,#205998),
(#205999,#206000),(#206001,#206002),(#206003,#206004),(#206005,#206006),
(#206007,#206008),(#206009,#206010),(#206011,#206012),(#206013,#206014),
(#206015,#206016),(#206017,#206018),(#206019,#206020),(#206021,#206022),
(#206023,#206024),(#206025,#206026),(#206027,#206028),(#206029,#206030),
(#206031,#206032),(#206033,#206034),(#206035,#206036),(#206037,#206038),
(#206039,#206040),(#206041,#206042),(#206043,#206044),(#206045,#206046),
(#206047,#206048),(#206049,#206050),(#206051,#206052),(#206053,#206054),
(#206055,#206056),(#206057,#206058),(#206059,#206060),(#206061,#206062),
(#206063,#206064),(#206065,#206066),(#206067,#206068),(#206069,#206070),
(#206071,#206072),(#206073,#206074),(#206075,#206076),(#206077,#206078),
(#206079,#206080),(#206081,#206082),(#206083,#206084),(#206085,#206086),
(#206087,#206088),(#206089,#206090),(#206091,#206092),(#206093,#206094),
(#206095,#206096),(#206097,#206098),(#206099,#206100),(#206101,#206102),
(#206103,#206104),(#206105,#206106),(#206107,#206108),(#206109,#206110),
(#206111,#206112),(#206113,#206114),(#206115,#206116),(#206117,#206118),
(#206119,#206120),(#206121,#206122),(#206123,#206124),(#206125,#206126),
(#206127,#206128),(#206129,#206130),(#206131,#206132),(#206133,#206134),
(#206135,#206136),(#206137,#206138),(#206139,#206140),(#206141,#206142),
(#206143,#206144),(#206145,#206146),(#206147,#206148),(#206149,#206150),
(#206151,#206152),(#206153,#206154),(#206155,#206156),(#206157,#206158),
(#206159,#206160),(#206161,#206162),(#206163,#206164),(#206165,#206166),
(#206167,#206168),(#206169,#206170),(#206171,#206172),(#206173,#206174),
(#206175,#206176),(#206177,#206178),(#206179,#206180),(#206181,#206182),
(#206183,#206184),(#206185,#206186),(#206187,#206188),(#206189,#206190),
(#206191,#206192),(#206193,#206194),(#206195,#206196),(#206197,#206198),
(#206199,#206200),(#206201,#206202),(#206203,#206204),(#206205,#206206),
(#206207,#206208),(#206209,#206210),(#206211,#206212),(#206213,#206214),
(#206215,#206216),(#206217,#206218),(#206219,#206220),(#206221,#206222),
(#206223,#206224),(#206225,#206226),(#206227,#206228),(#206229,#206230),
(#206231,#206232),(#206233,#206234),(#206235,#206236),(#206237,#206238),
(#206239,#206240),(#206241,#206242),(#206243,#206244),(#206245,#206246),
(#206247,#206248),(#206249,#206250),(#206251,#206252),(#206253,#206254),
(#206255,#206256),(#206257,#206258),(#206259,#206260),(#206261,#206262),
(#206263,#206264),(#206265,#206266),(#206267,#206268),(#206269,#206270),
(#206271,#206272),(#206273,#206274),(#206275,#206276),(#206277,#206278),
(#206279,#206280),(#206281,#206282),(#206283,#206284),(#206285,#206286),
(#206287,#206288),(#206289,#206290),(#206291,#206292),(#206293,#206294),
(#206295,#206296),(#206297,#206298),(#206299,#206300),(#206301,#206302),
(#206303,#206304),(#206305,#206306),(#206307,#206308),(#206309,#206310),
(#206311,#206312),(#206313,#206314),(#206315,#206316),(#206317,#206318),
(#206319,#206320),(#206321,#206322),(#206323,#206324),(#206325,#206326),
(#206327,#206328),(#206329,#206330),(#206331,#206332),(#206333,#206334),
(#206335,#206336),(#206337,#206338),(#206339,#206340),(#206341,#206342),
(#206343,#206344),(#206345,#206346),(#206347,#206348),(#206349,#206350),
(#206351,#206352),(#206353,#206354),(#206355,#206356),(#206357,#206358),
(#206359,#206360),(#206361,#206362),(#206363,#206364),(#206365,#206366),
(#206367,#206368),(#206369,#206370),(#206371,#206372),(#206373,#206374),
(#206375,#206376),(#206377,#206378),(#206379,#206380),(#206381,#206382),
(#206383,#206384),(#206385,#206386),(#206387,#206388),(#206389,#206390),
(#206391,#206392),(#206393,#206394),(#206395,#206396),(#206397,#206398),
(#206399,#206400),(#206401,#206402),(#206403,#206404),(#206405,#206406),
(#206407,#206408),(#206409,#206410),(#206411,#206412),(#206413,#206414),
(#206415,#206416),(#206417,#206418),(#206419,#206420),(#206421,#206422),
(#206423,#206424),(#206425,#206426),(#206427,#206428),(#206429,#206430),
(#206431,#206432),(#206433,#206434),(#206435,#206436),(#206437,#206438),
(#206439,#206440),(#206441,#206442),(#206443,#206444),(#206445,#206446),
(#206447,#206448),(#206449,#206450),(#206451,#206452),(#206453,#206454),
(#206455,#206456),(#206457,#206458),(#206459,#206460),(#206461,#206462),
(#206463,#206464),(#206465,#206466),(#206467,#206468),(#206469,#206470),
(#206471,#206472),(#206473,#206474),(#206475,#206476),(#206477,#206478),
(#206479,#206480),(#206481,#206482),(#206483,#206484),(#206485,#206486),
(#206487,#206488),(#206489,#206490),(#206491,#206492),(#206493,#206494),
(#206495,#206496),(#206497,#206498),(#206499,#206500),(#206501,#206502),
(#206503,#206504),(#206505,#206506),(#206507,#206508),(#206509,#206510),
(#206511,#206512),(#206513,#206514),(#206515,#206516),(#206517,#206518),
(#206519,#206520),(#206521,#206522),(#206523,#206524),(#206525,#206526),
(#206527,#206528),(#206529,#206530),(#206531,#206532),(#206533,#206534),
(#206535,#206536),(#206537,#206538),(#206539,#206540),(#206541,#206542),
(#206543,#206544),(#206545,#206546),(#206547,#206548),(#206549,#206550),
(#206551,#206552),(#206553,#206554),(#206555,#206556),(#206557,#206558),
(#206559,#206560),(#206561,#206562),(#206563,#206564),(#206565,#206566),
(#206567,#206568),(#206569,#206570),(#206571,#206572),(#206573,#206574),
(#206575,#206576),(#206577,#206578),(#206579,#206580),(#206581,#206582),
(#206583,#206584),(#206585,#206586),(#206587,#206588),(#206589,#206590),
(#206591,#206592),(#206593,#206594),(#206595,#206596),(#206597,#206598),
(#206599,#206600),(#206601,#206602),(#206603,#206604),(#206605,#206606),
(#206607,#206608),(#206609,#206610),(#206611,#206612),(#206613,#206614),
(#206615,#206616),(#206617,#206618),(#206619,#206620),(#206621,#206622),
(#206623,#206624),(#206625,#206626),(#206627,#206628),(#206629,#206630),
(#206631,#206632),(#206633,#206634),(#206635,#206636),(#206637,#206638),
(#206639,#206640),(#206641,#206642),(#206643,#206644),(#206645,#206646),
(#206647,#206648),(#206649,#206650),(#206651,#206652),(#206653,#206654),
(#206655,#206656),(#206657,#206658),(#206659,#206660),(#206661,#206662),
(#206663,#206664),(#206665,#206666),(#206667,#206668),(#206669,#206670),
(#206671,#206672),(#206673,#206674),(#206675,#206676),(#206677,#206678),
(#206679,#206680),(#206681,#206682),(#206683,#206684),(#206685,#206686),
(#206687,#206688),(#206689,#206690),(#206691,#206692),(#206693,#206694),
(#206695,#206696),(#206697,#206698),(#206699,#206700),(#206701,#206702),
(#206703,#206704),(#206705,#206706),(#206707,#206708),(#206709,#206710),
(#206711,#206712),(#206713,#206714),(#206715,#206716),(#206717,#206718),
(#206719,#206720),(#206721,#206722),(#206723,#206724),(#206725,#206726),
(#206727,#206728),(#206729,#206730),(#206731,#206732),(#206733,#206734),
(#206735,#206736),(#206737,#206738),(#206739,#206740),(#206741,#206742),
(#206743,#206744),(#206745,#206746),(#206747,#206748),(#206749,#206750),
(#206751,#206752),(#206753,#206754),(#206755,#206756),(#206757,#206758),
(#206759,#206760),(#206761,#206762),(#206763,#206764),(#206765,#206766),
(#206767,#206768),(#206769,#206770),(#206771,#206772),(#206773,#206774),
(#206775,#206776),(#206777,#206778),(#206779,#206780),(#206781,#206782),
(#206783,#206784),(#206785,#206786),(#206787,#206788),(#206789,#206790),
(#206791,#206792),(#206793,#206794),(#206795,#206796),(#206797,#206798),
(#206799,#206800),(#206801,#206802),(#206803,#206804),(#206805,#206806),
(#206807,#206808),(#206809,#206810)),.UNSPECIFIED.,.F.,.F.,.F.,(6,1,1,1,
1,1,1,1,1,1,1,1,1,1,1,1,1,1,1,1,1,1,1,1,1,1,1,1,1,1,1,1,1,1,1,1,1,1,1,1,
1,1,1,1,1,1,1,1,1,1,1,1,1,1,1,1,1,1,1,1,1,1,1,1,1,1,1,1,1,1,1,1,1,1,1,1,
1,1,1,1,1,1,1,1,1,1,1,1,1,1,1,1,1,1,1,1,1,1,1,1,1,1,1,1,1,1,1,1,1,1,1,1,
1,1,1,1,1,1,1,1,1,1,1,1,1,1,1,1,1,1,1,1,1,1,1,1,1,1,1,1,1,1,1,1,1,1,1,1,
1,1,1,1,1,1,1,1,1,1,1,1,1,1,1,1,1,1,1,1,1,1,1,1,1,1,1,1,1,1,1,1,1,1,1,1,
1,1,1,1,1,1,1,1,1,1,1,1,1,1,1,1,1,1,1,1,1,1,1,1,1,1,1,1,1,1,1,1,1,1,1,1,
1,1,1,1,1,1,1,1,1,1,1,1,1,1,1,1,1,1,1,1,1,1,1,1,1,1,1,1,1,1,1,1,1,1,1,1,
1,1,1,1,1,1,1,1,1,1,1,1,1,1,1,1,1,1,1,1,1,1,1,1,1,1,1,1,1,1,1,1,1,1,1,1,
1,1,1,1,1,1,1,1,1,1,1,1,1,1,1,1,1,1,1,1,1,1,1,1,1,1,1,1,1,1,1,1,1,1,1,1,
1,1,1,1,1,1,1,1,1,1,1,1,1,1,1,1,1,1,1,1,1,1,1,1,1,1,1,1,1,1,1,1,1,1,1,1,
1,1,1,1,1,1,1,1,1,1,1,1,1,1,1,1,1,1,1,1,1,1,1,1,1,1,1,1,1,1,1,1,1,1,1,1,
1,1,1,1,1,1,1,1,1,1,1,1,1,1,1,1,1,1,1,1,1,1,1,1,1,1,1,1,1,1,1,1,1,1,1,1,
1,1,1,1,1,1,1,1,1,1,1,1,1,1,1,1,1,1,1,1,1,1,1,1,1,1,1,1,1,1,1,6),(2,2),
(0.143172103,0.144954128,0.146788991,0.148623853,0.150458716,0.152293578,
0.15412844,0.155963303,0.157798165,0.159633028,0.16146789,0.163302752,0.165137615,
0.166972477,0.168807339,0.170642202,0.172477064,0.174311927,0.176146789,
0.177981651,0.179816514,0.181651376,0.183486239,0.185321101,0.187155963,
0.188990826,0.190825688,0.19266055,0.194495413,0.196330275,0.198165138,
0.2,0.201834862,0.203669725,0.205504587,0.20733945,0.209174312,0.211009174,
0.212844037,0.214678899,0.216513761,0.218348624,0.220183486,0.222018349,
0.223853211,0.225688073,0.227522936,0.229357798,0.231192661,0.233027523,
0.234862385,0.236697248,0.23853211,0.240366972,0.242201835,0.244036697,
0.24587156,0.247706422,0.249541284,0.251376147,0.253211009,0.255045872,
0.256880734,0.258715596,0.260550459,0.262385321,0.264220183,0.266055046,
0.267889908,0.269724771,0.271559633,0.273394495,0.275229358,0.27706422,
0.278899083,0.280733945,0.282568807,0.28440367,0.286238532,0.288073394,
0.289908257,0.291743119,0.293577982,0.295412844,0.297247706,0.299082569,
0.300917431,0.302752294,0.304587156,0.306422018,0.308256881,0.310091743,
0.311926606,0.313761468,0.31559633,0.317431193,0.319266055,0.321100917,
0.32293578,0.324770642,0.326605505,0.328440367,0.330275229,0.332110092,
0.333944954,0.335779817,0.337614679,0.339449541,0.341284404,0.343119266,
0.344954128,0.346788991,0.348623853,0.350458716,0.352293578,0.35412844,
0.355963303,0.357798165,0.359633028,0.36146789,0.363302752,0.365137615,
0.366972477,0.368807339,0.370642202,0.372477064,0.374311927,0.376146789,
0.377981651,0.379816514,0.381651376,0.383486239,0.385321101,0.387155963,
0.388990826,0.390825688,0.39266055,0.394495413,0.396330275,0.398165138,
0.4,0.401834862,0.403669725,0.405504587,0.40733945,0.409174312,0.411009174,
0.412844037,0.414678899,0.416513761,0.418348624,0.420183486,0.422018349,
0.423853211,0.425688073,0.427522936,0.429357798,0.431192661,0.433027523,
0.434862385,0.436697248,0.43853211,0.440366972,0.442201835,0.444036697,
0.44587156,0.447706422,0.449541284,0.451376147,0.453211009,0.455045872,
0.456880734,0.458715596,0.460550459,0.462385321,0.464220183,0.466055046,
0.467889908,0.469724771,0.471559633,0.473394495,0.475229358,0.47706422,
0.478899083,0.480733945,0.482568807,0.48440367,0.486238532,0.488073394,
0.489908257,0.491743119,0.493577982,0.495412844,0.497247706,0.499082569,
0.500917431,0.502752294,0.504587156,0.506422018,0.508256881,0.510091743,
0.511926606,0.513761468,0.51559633,0.517431193,0.519266055,0.521100917,
0.52293578,0.524770642,0.526605505,0.528440367,0.530275229,0.532110092,
0.533944954,0.535779817,0.537614679,0.539449541,0.541284404,0.543119266,
0.544954128,0.546788991,0.548623853,0.550458716,0.552293578,0.55412844,
0.555963303,0.557798165,0.559633028,0.56146789,0.563302752,0.565137615,
0.566972477,0.568807339,0.570642202,0.572477064,0.574311927,0.576146789,
0.577981651,0.579816514,0.581651376,0.583486239,0.585321101,0.587155963,
0.588990826,0.590825688,0.59266055,0.594495413,0.596330275,0.598165138,
0.6,0.601834862,0.603669725,0.605504587,0.60733945,0.609174312,0.611009174,
0.612844037,0.614678899,0.616513761,0.618348624,0.620183486,0.622018349,
0.623853211,0.625688073,0.627522936,0.629357798,0.631192661,0.633027523,
0.634862385,0.636697248,0.63853211,0.640366972,0.642201835,0.644036697,
0.64587156,0.647706422,0.649541284,0.651376147,0.653211009,0.655045872,
0.656880734,0.658715596,0.660550459,0.662385321,0.664220183,0.666055046,
0.667889908,0.669724771,0.671559633,0.673394495,0.675229358,0.67706422,
0.678899083,0.680733945,0.682568807,0.68440367,0.686238532,0.688073394,
0.689908257,0.691743119,0.693577982,0.695412844,0.697247706,0.699082569,
0.700917431,0.702752294,0.704587156,0.706422018,0.708256881,0.710091743,
0.711926606,0.713761468,0.71559633,0.717431193,0.719266055,0.721100917,
0.72293578,0.724770642,0.726605505,0.728440367,0.730275229,0.732110092,
0.733944954,0.735779817,0.737614679,0.739449541,0.741284404,0.743119266,
0.744954128,0.746788991,0.748623853,0.750458716,0.752293578,0.75412844,
0.755963303,0.757798165,0.759633028,0.76146789,0.763302752,0.765137615,
0.766972477,0.768807339,0.770642202,0.772477064,0.774311927,0.776146789,
0.777981651,0.779816514,0.781651376,0.783486239,0.785321101,0.787155963,
0.788990826,0.790825688,0.79266055,0.794495413,0.796330275,0.798165138,
0.8,0.801834862,0.803669725,0.805504587,0.80733945,0.809174312,0.811009174,
0.812844037,0.814678899,0.816513761,0.818348624,0.820183486,0.822018349,
0.823853211,0.825688073,0.827522936,0.829357798,0.831192661,0.833027523,
0.834862385,0.836697248,0.83853211,0.840366972,0.842201835,0.844036697,
0.84587156,0.847706422,0.849541284,0.851376147,0.853211009,0.855045872,
0.856880734,0.858715596,0.860550459,0.862385321,0.864220183,0.866055046,
0.867889908,0.869724771,0.871559633,0.873394495,0.875229358,0.87706422,
0.878899083,0.880733945,0.882568807,0.88440367,0.886238532,0.888073394,
0.889908257,0.891743119,0.893577982,0.895412844,0.897247706,0.899082569,
0.900917431,0.902752294,0.904587156,0.906422018,0.908256881,0.910091743,
0.911926606,0.913761468,0.91559633,0.917431193,0.919266055,0.921100917,
0.92293578,0.924770642,0.926605505,0.928440367,0.930275229,0.932110092,
0.933944954,0.935779817,0.937614679,0.939449541,0.941284404,0.943119266,
0.944954128,0.946788991,0.948623853,0.950458716,0.952293578,0.95412844,
0.955963303,0.957798165,0.959633028,0.96146789,0.963302752,0.965137615,
0.966972477,0.968807339,0.970642202,0.972477064,0.974311927,0.976146789,
0.977981651,0.979816514,0.981651376,0.983486239,0.985321101,0.987155963,
0.988990826,0.990825688,0.99266055,0.994495413,0.996330275,0.998165138,
1.),(0.,0.36),.UNSPECIFIED.);
#6247=B_SPLINE_SURFACE_WITH_KNOTS('',5,1,((#207446,#207447),(#207448,#207449),
(#207450,#207451),(#207452,#207453),(#207454,#207455),(#207456,#207457),
(#207458,#207459),(#207460,#207461),(#207462,#207463),(#207464,#207465),
(#207466,#207467),(#207468,#207469),(#207470,#207471),(#207472,#207473),
(#207474,#207475),(#207476,#207477),(#207478,#207479),(#207480,#207481),
(#207482,#207483),(#207484,#207485),(#207486,#207487),(#207488,#207489),
(#207490,#207491),(#207492,#207493),(#207494,#207495),(#207496,#207497),
(#207498,#207499),(#207500,#207501),(#207502,#207503),(#207504,#207505),
(#207506,#207507),(#207508,#207509),(#207510,#207511),(#207512,#207513),
(#207514,#207515),(#207516,#207517),(#207518,#207519),(#207520,#207521),
(#207522,#207523),(#207524,#207525),(#207526,#207527),(#207528,#207529),
(#207530,#207531),(#207532,#207533),(#207534,#207535),(#207536,#207537),
(#207538,#207539),(#207540,#207541),(#207542,#207543),(#207544,#207545),
(#207546,#207547),(#207548,#207549),(#207550,#207551),(#207552,#207553),
(#207554,#207555),(#207556,#207557),(#207558,#207559),(#207560,#207561),
(#207562,#207563),(#207564,#207565),(#207566,#207567),(#207568,#207569),
(#207570,#207571),(#207572,#207573),(#207574,#207575),(#207576,#207577),
(#207578,#207579),(#207580,#207581),(#207582,#207583),(#207584,#207585),
(#207586,#207587),(#207588,#207589),(#207590,#207591),(#207592,#207593),
(#207594,#207595),(#207596,#207597),(#207598,#207599),(#207600,#207601),
(#207602,#207603),(#207604,#207605),(#207606,#207607),(#207608,#207609),
(#207610,#207611),(#207612,#207613),(#207614,#207615),(#207616,#207617),
(#207618,#207619),(#207620,#207621),(#207622,#207623),(#207624,#207625),
(#207626,#207627),(#207628,#207629),(#207630,#207631),(#207632,#207633),
(#207634,#207635),(#207636,#207637),(#207638,#207639),(#207640,#207641),
(#207642,#207643),(#207644,#207645),(#207646,#207647),(#207648,#207649),
(#207650,#207651),(#207652,#207653),(#207654,#207655),(#207656,#207657),
(#207658,#207659),(#207660,#207661),(#207662,#207663),(#207664,#207665),
(#207666,#207667),(#207668,#207669),(#207670,#207671),(#207672,#207673),
(#207674,#207675),(#207676,#207677),(#207678,#207679),(#207680,#207681),
(#207682,#207683),(#207684,#207685),(#207686,#207687),(#207688,#207689),
(#207690,#207691),(#207692,#207693),(#207694,#207695),(#207696,#207697),
(#207698,#207699),(#207700,#207701),(#207702,#207703),(#207704,#207705),
(#207706,#207707),(#207708,#207709),(#207710,#207711),(#207712,#207713),
(#207714,#207715),(#207716,#207717),(#207718,#207719),(#207720,#207721),
(#207722,#207723),(#207724,#207725),(#207726,#207727),(#207728,#207729),
(#207730,#207731),(#207732,#207733),(#207734,#207735),(#207736,#207737),
(#207738,#207739),(#207740,#207741),(#207742,#207743),(#207744,#207745),
(#207746,#207747),(#207748,#207749),(#207750,#207751),(#207752,#207753),
(#207754,#207755),(#207756,#207757),(#207758,#207759),(#207760,#207761),
(#207762,#207763),(#207764,#207765),(#207766,#207767),(#207768,#207769),
(#207770,#207771),(#207772,#207773),(#207774,#207775),(#207776,#207777),
(#207778,#207779),(#207780,#207781),(#207782,#207783),(#207784,#207785),
(#207786,#207787),(#207788,#207789),(#207790,#207791),(#207792,#207793),
(#207794,#207795),(#207796,#207797),(#207798,#207799),(#207800,#207801),
(#207802,#207803),(#207804,#207805),(#207806,#207807),(#207808,#207809),
(#207810,#207811),(#207812,#207813),(#207814,#207815),(#207816,#207817),
(#207818,#207819),(#207820,#207821),(#207822,#207823),(#207824,#207825),
(#207826,#207827),(#207828,#207829),(#207830,#207831),(#207832,#207833),
(#207834,#207835),(#207836,#207837),(#207838,#207839),(#207840,#207841),
(#207842,#207843),(#207844,#207845),(#207846,#207847),(#207848,#207849),
(#207850,#207851),(#207852,#207853),(#207854,#207855),(#207856,#207857),
(#207858,#207859),(#207860,#207861),(#207862,#207863),(#207864,#207865),
(#207866,#207867),(#207868,#207869),(#207870,#207871),(#207872,#207873),
(#207874,#207875),(#207876,#207877),(#207878,#207879),(#207880,#207881),
(#207882,#207883),(#207884,#207885),(#207886,#207887),(#207888,#207889),
(#207890,#207891),(#207892,#207893),(#207894,#207895),(#207896,#207897),
(#207898,#207899),(#207900,#207901),(#207902,#207903),(#207904,#207905),
(#207906,#207907),(#207908,#207909),(#207910,#207911),(#207912,#207913),
(#207914,#207915),(#207916,#207917),(#207918,#207919),(#207920,#207921),
(#207922,#207923),(#207924,#207925),(#207926,#207927),(#207928,#207929),
(#207930,#207931),(#207932,#207933),(#207934,#207935),(#207936,#207937),
(#207938,#207939),(#207940,#207941),(#207942,#207943),(#207944,#207945),
(#207946,#207947),(#207948,#207949),(#207950,#207951),(#207952,#207953),
(#207954,#207955),(#207956,#207957),(#207958,#207959),(#207960,#207961),
(#207962,#207963),(#207964,#207965),(#207966,#207967),(#207968,#207969),
(#207970,#207971),(#207972,#207973),(#207974,#207975),(#207976,#207977),
(#207978,#207979),(#207980,#207981),(#207982,#207983),(#207984,#207985),
(#207986,#207987),(#207988,#207989),(#207990,#207991),(#207992,#207993),
(#207994,#207995),(#207996,#207997),(#207998,#207999),(#208000,#208001),
(#208002,#208003),(#208004,#208005),(#208006,#208007),(#208008,#208009),
(#208010,#208011),(#208012,#208013),(#208014,#208015),(#208016,#208017),
(#208018,#208019),(#208020,#208021),(#208022,#208023),(#208024,#208025),
(#208026,#208027),(#208028,#208029),(#208030,#208031),(#208032,#208033),
(#208034,#208035),(#208036,#208037),(#208038,#208039),(#208040,#208041),
(#208042,#208043),(#208044,#208045),(#208046,#208047),(#208048,#208049),
(#208050,#208051),(#208052,#208053),(#208054,#208055),(#208056,#208057),
(#208058,#208059),(#208060,#208061),(#208062,#208063),(#208064,#208065),
(#208066,#208067),(#208068,#208069),(#208070,#208071),(#208072,#208073),
(#208074,#208075),(#208076,#208077),(#208078,#208079),(#208080,#208081),
(#208082,#208083),(#208084,#208085),(#208086,#208087),(#208088,#208089),
(#208090,#208091),(#208092,#208093),(#208094,#208095),(#208096,#208097),
(#208098,#208099),(#208100,#208101),(#208102,#208103),(#208104,#208105),
(#208106,#208107),(#208108,#208109),(#208110,#208111),(#208112,#208113),
(#208114,#208115),(#208116,#208117),(#208118,#208119),(#208120,#208121),
(#208122,#208123),(#208124,#208125),(#208126,#208127),(#208128,#208129),
(#208130,#208131),(#208132,#208133),(#208134,#208135),(#208136,#208137),
(#208138,#208139),(#208140,#208141),(#208142,#208143),(#208144,#208145),
(#208146,#208147),(#208148,#208149),(#208150,#208151),(#208152,#208153),
(#208154,#208155),(#208156,#208157),(#208158,#208159),(#208160,#208161),
(#208162,#208163),(#208164,#208165),(#208166,#208167),(#208168,#208169),
(#208170,#208171),(#208172,#208173),(#208174,#208175),(#208176,#208177),
(#208178,#208179),(#208180,#208181),(#208182,#208183),(#208184,#208185),
(#208186,#208187),(#208188,#208189),(#208190,#208191),(#208192,#208193),
(#208194,#208195),(#208196,#208197),(#208198,#208199),(#208200,#208201),
(#208202,#208203),(#208204,#208205),(#208206,#208207),(#208208,#208209),
(#208210,#208211),(#208212,#208213),(#208214,#208215),(#208216,#208217),
(#208218,#208219),(#208220,#208221),(#208222,#208223),(#208224,#208225),
(#208226,#208227),(#208228,#208229),(#208230,#208231),(#208232,#208233),
(#208234,#208235),(#208236,#208237),(#208238,#208239),(#208240,#208241),
(#208242,#208243),(#208244,#208245),(#208246,#208247),(#208248,#208249),
(#208250,#208251),(#208252,#208253),(#208254,#208255),(#208256,#208257),
(#208258,#208259),(#208260,#208261),(#208262,#208263),(#208264,#208265),
(#208266,#208267),(#208268,#208269),(#208270,#208271),(#208272,#208273),
(#208274,#208275),(#208276,#208277),(#208278,#208279),(#208280,#208281),
(#208282,#208283),(#208284,#208285),(#208286,#208287),(#208288,#208289),
(#208290,#208291),(#208292,#208293),(#208294,#208295),(#208296,#208297),
(#208298,#208299),(#208300,#208301),(#208302,#208303),(#208304,#208305),
(#208306,#208307),(#208308,#208309),(#208310,#208311),(#208312,#208313),
(#208314,#208315),(#208316,#208317),(#208318,#208319),(#208320,#208321),
(#208322,#208323),(#208324,#208325),(#208326,#208327),(#208328,#208329),
(#208330,#208331),(#208332,#208333),(#208334,#208335),(#208336,#208337),
(#208338,#208339),(#208340,#208341),(#208342,#208343),(#208344,#208345),
(#208346,#208347),(#208348,#208349),(#208350,#208351),(#208352,#208353),
(#208354,#208355),(#208356,#208357),(#208358,#208359),(#208360,#208361),
(#208362,#208363),(#208364,#208365),(#208366,#208367),(#208368,#208369),
(#208370,#208371),(#208372,#208373),(#208374,#208375),(#208376,#208377),
(#208378,#208379),(#208380,#208381),(#208382,#208383),(#208384,#208385),
(#208386,#208387),(#208388,#208389)),.UNSPECIFIED.,.F.,.F.,.F.,(6,1,1,1,
1,1,1,1,1,1,1,1,1,1,1,1,1,1,1,1,1,1,1,1,1,1,1,1,1,1,1,1,1,1,1,1,1,1,1,1,
1,1,1,1,1,1,1,1,1,1,1,1,1,1,1,1,1,1,1,1,1,1,1,1,1,1,1,1,1,1,1,1,1,1,1,1,
1,1,1,1,1,1,1,1,1,1,1,1,1,1,1,1,1,1,1,1,1,1,1,1,1,1,1,1,1,1,1,1,1,1,1,1,
1,1,1,1,1,1,1,1,1,1,1,1,1,1,1,1,1,1,1,1,1,1,1,1,1,1,1,1,1,1,1,1,1,1,1,1,
1,1,1,1,1,1,1,1,1,1,1,1,1,1,1,1,1,1,1,1,1,1,1,1,1,1,1,1,1,1,1,1,1,1,1,1,
1,1,1,1,1,1,1,1,1,1,1,1,1,1,1,1,1,1,1,1,1,1,1,1,1,1,1,1,1,1,1,1,1,1,1,1,
1,1,1,1,1,1,1,1,1,1,1,1,1,1,1,1,1,1,1,1,1,1,1,1,1,1,1,1,1,1,1,1,1,1,1,1,
1,1,1,1,1,1,1,1,1,1,1,1,1,1,1,1,1,1,1,1,1,1,1,1,1,1,1,1,1,1,1,1,1,1,1,1,
1,1,1,1,1,1,1,1,1,1,1,1,1,1,1,1,1,1,1,1,1,1,1,1,1,1,1,1,1,1,1,1,1,1,1,1,
1,1,1,1,1,1,1,1,1,1,1,1,1,1,1,1,1,1,1,1,1,1,1,1,1,1,1,1,1,1,1,1,1,1,1,1,
1,1,1,1,1,1,1,1,1,1,1,1,1,1,1,1,1,1,1,1,1,1,1,1,1,1,1,1,1,1,1,1,1,1,1,1,
1,1,1,1,1,1,1,1,1,1,1,1,1,1,1,1,1,1,1,1,1,1,1,1,1,1,1,1,1,1,1,1,1,1,1,1,
1,1,1,1,1,1,1,1,1,1,1,1,1,1,1,1,1,1,1,1,1,1,1,1,1,1,1,1,1,1,1,6),(2,2),
(0.143172104,0.144954128,0.146788991,0.148623853,0.150458716,0.152293578,
0.15412844,0.155963303,0.157798165,0.159633028,0.16146789,0.163302752,0.165137615,
0.166972477,0.168807339,0.170642202,0.172477064,0.174311927,0.176146789,
0.177981651,0.179816514,0.181651376,0.183486239,0.185321101,0.187155963,
0.188990826,0.190825688,0.19266055,0.194495413,0.196330275,0.198165138,
0.2,0.201834862,0.203669725,0.205504587,0.20733945,0.209174312,0.211009174,
0.212844037,0.214678899,0.216513761,0.218348624,0.220183486,0.222018349,
0.223853211,0.225688073,0.227522936,0.229357798,0.231192661,0.233027523,
0.234862385,0.236697248,0.23853211,0.240366972,0.242201835,0.244036697,
0.24587156,0.247706422,0.249541284,0.251376147,0.253211009,0.255045872,
0.256880734,0.258715596,0.260550459,0.262385321,0.264220183,0.266055046,
0.267889908,0.269724771,0.271559633,0.273394495,0.275229358,0.27706422,
0.278899083,0.280733945,0.282568807,0.28440367,0.286238532,0.288073394,
0.289908257,0.291743119,0.293577982,0.295412844,0.297247706,0.299082569,
0.300917431,0.302752294,0.304587156,0.306422018,0.308256881,0.310091743,
0.311926606,0.313761468,0.31559633,0.317431193,0.319266055,0.321100917,
0.32293578,0.324770642,0.326605505,0.328440367,0.330275229,0.332110092,
0.333944954,0.335779817,0.337614679,0.339449541,0.341284404,0.343119266,
0.344954128,0.346788991,0.348623853,0.350458716,0.352293578,0.35412844,
0.355963303,0.357798165,0.359633028,0.36146789,0.363302752,0.365137615,
0.366972477,0.368807339,0.370642202,0.372477064,0.374311927,0.376146789,
0.377981651,0.379816514,0.381651376,0.383486239,0.385321101,0.387155963,
0.388990826,0.390825688,0.39266055,0.394495413,0.396330275,0.398165138,
0.4,0.401834862,0.403669725,0.405504587,0.40733945,0.409174312,0.411009174,
0.412844037,0.414678899,0.416513761,0.418348624,0.420183486,0.422018349,
0.423853211,0.425688073,0.427522936,0.429357798,0.431192661,0.433027523,
0.434862385,0.436697248,0.43853211,0.440366972,0.442201835,0.444036697,
0.44587156,0.447706422,0.449541284,0.451376147,0.453211009,0.455045872,
0.456880734,0.458715596,0.460550459,0.462385321,0.464220183,0.466055046,
0.467889908,0.469724771,0.471559633,0.473394495,0.475229358,0.47706422,
0.478899083,0.480733945,0.482568807,0.48440367,0.486238532,0.488073394,
0.489908257,0.491743119,0.493577982,0.495412844,0.497247706,0.499082569,
0.500917431,0.502752294,0.504587156,0.506422018,0.508256881,0.510091743,
0.511926606,0.513761468,0.51559633,0.517431193,0.519266055,0.521100917,
0.52293578,0.524770642,0.526605505,0.528440367,0.530275229,0.532110092,
0.533944954,0.535779817,0.537614679,0.539449541,0.541284404,0.543119266,
0.544954128,0.546788991,0.548623853,0.550458716,0.552293578,0.55412844,
0.555963303,0.557798165,0.559633028,0.56146789,0.563302752,0.565137615,
0.566972477,0.568807339,0.570642202,0.572477064,0.574311927,0.576146789,
0.577981651,0.579816514,0.581651376,0.583486239,0.585321101,0.587155963,
0.588990826,0.590825688,0.59266055,0.594495413,0.596330275,0.598165138,
0.6,0.601834862,0.603669725,0.605504587,0.60733945,0.609174312,0.611009174,
0.612844037,0.614678899,0.616513761,0.618348624,0.620183486,0.622018349,
0.623853211,0.625688073,0.627522936,0.629357798,0.631192661,0.633027523,
0.634862385,0.636697248,0.63853211,0.640366972,0.642201835,0.644036697,
0.64587156,0.647706422,0.649541284,0.651376147,0.653211009,0.655045872,
0.656880734,0.658715596,0.660550459,0.662385321,0.664220183,0.666055046,
0.667889908,0.669724771,0.671559633,0.673394495,0.675229358,0.67706422,
0.678899083,0.680733945,0.682568807,0.68440367,0.686238532,0.688073394,
0.689908257,0.691743119,0.693577982,0.695412844,0.697247706,0.699082569,
0.700917431,0.702752294,0.704587156,0.706422018,0.708256881,0.710091743,
0.711926606,0.713761468,0.71559633,0.717431193,0.719266055,0.721100917,
0.72293578,0.724770642,0.726605505,0.728440367,0.730275229,0.732110092,
0.733944954,0.735779817,0.737614679,0.739449541,0.741284404,0.743119266,
0.744954128,0.746788991,0.748623853,0.750458716,0.752293578,0.75412844,
0.755963303,0.757798165,0.759633028,0.76146789,0.763302752,0.765137615,
0.766972477,0.768807339,0.770642202,0.772477064,0.774311927,0.776146789,
0.777981651,0.779816514,0.781651376,0.783486239,0.785321101,0.787155963,
0.788990826,0.790825688,0.79266055,0.794495413,0.796330275,0.798165138,
0.8,0.801834862,0.803669725,0.805504587,0.80733945,0.809174312,0.811009174,
0.812844037,0.814678899,0.816513761,0.818348624,0.820183486,0.822018349,
0.823853211,0.825688073,0.827522936,0.829357798,0.831192661,0.833027523,
0.834862385,0.836697248,0.83853211,0.840366972,0.842201835,0.844036697,
0.84587156,0.847706422,0.849541284,0.851376147,0.853211009,0.855045872,
0.856880734,0.858715596,0.860550459,0.862385321,0.864220183,0.866055046,
0.867889908,0.869724771,0.871559633,0.873394495,0.875229358,0.87706422,
0.878899083,0.880733945,0.882568807,0.88440367,0.886238532,0.888073394,
0.889908257,0.891743119,0.893577982,0.895412844,0.897247706,0.899082569,
0.900917431,0.902752294,0.904587156,0.906422018,0.908256881,0.910091743,
0.911926606,0.913761468,0.91559633,0.917431193,0.919266055,0.921100917,
0.92293578,0.924770642,0.926605505,0.928440367,0.930275229,0.932110092,
0.933944954,0.935779817,0.937614679,0.939449541,0.941284404,0.943119266,
0.944954128,0.946788991,0.948623853,0.950458716,0.952293578,0.95412844,
0.955963303,0.957798165,0.959633028,0.96146789,0.963302752,0.965137615,
0.966972477,0.968807339,0.970642202,0.972477064,0.974311927,0.976146789,
0.977981651,0.979816514,0.981651376,0.983486239,0.985321101,0.987155963,
0.988990826,0.990825688,0.99266055,0.994495413,0.996330275,0.998165138,
1.),(0.,0.36),.UNSPECIFIED.);
#6248=B_SPLINE_SURFACE_WITH_KNOTS('',5,1,((#209028,#209029),(#209030,#209031),
(#209032,#209033),(#209034,#209035),(#209036,#209037),(#209038,#209039),
(#209040,#209041),(#209042,#209043),(#209044,#209045),(#209046,#209047),
(#209048,#209049),(#209050,#209051),(#209052,#209053),(#209054,#209055),
(#209056,#209057),(#209058,#209059),(#209060,#209061),(#209062,#209063),
(#209064,#209065),(#209066,#209067),(#209068,#209069),(#209070,#209071),
(#209072,#209073),(#209074,#209075),(#209076,#209077),(#209078,#209079),
(#209080,#209081),(#209082,#209083),(#209084,#209085),(#209086,#209087),
(#209088,#209089),(#209090,#209091),(#209092,#209093),(#209094,#209095),
(#209096,#209097),(#209098,#209099),(#209100,#209101),(#209102,#209103),
(#209104,#209105),(#209106,#209107),(#209108,#209109),(#209110,#209111),
(#209112,#209113),(#209114,#209115),(#209116,#209117),(#209118,#209119),
(#209120,#209121),(#209122,#209123),(#209124,#209125),(#209126,#209127),
(#209128,#209129),(#209130,#209131),(#209132,#209133),(#209134,#209135),
(#209136,#209137),(#209138,#209139),(#209140,#209141),(#209142,#209143),
(#209144,#209145),(#209146,#209147),(#209148,#209149),(#209150,#209151),
(#209152,#209153),(#209154,#209155),(#209156,#209157),(#209158,#209159),
(#209160,#209161),(#209162,#209163),(#209164,#209165),(#209166,#209167),
(#209168,#209169),(#209170,#209171),(#209172,#209173),(#209174,#209175),
(#209176,#209177),(#209178,#209179),(#209180,#209181),(#209182,#209183),
(#209184,#209185),(#209186,#209187),(#209188,#209189),(#209190,#209191),
(#209192,#209193),(#209194,#209195),(#209196,#209197),(#209198,#209199),
(#209200,#209201),(#209202,#209203),(#209204,#209205),(#209206,#209207),
(#209208,#209209),(#209210,#209211),(#209212,#209213),(#209214,#209215),
(#209216,#209217),(#209218,#209219),(#209220,#209221),(#209222,#209223),
(#209224,#209225),(#209226,#209227),(#209228,#209229),(#209230,#209231),
(#209232,#209233),(#209234,#209235),(#209236,#209237),(#209238,#209239),
(#209240,#209241),(#209242,#209243),(#209244,#209245),(#209246,#209247),
(#209248,#209249),(#209250,#209251),(#209252,#209253),(#209254,#209255),
(#209256,#209257),(#209258,#209259),(#209260,#209261),(#209262,#209263),
(#209264,#209265),(#209266,#209267),(#209268,#209269),(#209270,#209271),
(#209272,#209273),(#209274,#209275),(#209276,#209277),(#209278,#209279),
(#209280,#209281),(#209282,#209283),(#209284,#209285),(#209286,#209287),
(#209288,#209289),(#209290,#209291),(#209292,#209293),(#209294,#209295),
(#209296,#209297),(#209298,#209299),(#209300,#209301),(#209302,#209303),
(#209304,#209305),(#209306,#209307),(#209308,#209309),(#209310,#209311),
(#209312,#209313),(#209314,#209315),(#209316,#209317),(#209318,#209319),
(#209320,#209321),(#209322,#209323),(#209324,#209325),(#209326,#209327),
(#209328,#209329),(#209330,#209331),(#209332,#209333),(#209334,#209335),
(#209336,#209337),(#209338,#209339),(#209340,#209341),(#209342,#209343),
(#209344,#209345),(#209346,#209347),(#209348,#209349),(#209350,#209351),
(#209352,#209353),(#209354,#209355),(#209356,#209357),(#209358,#209359),
(#209360,#209361),(#209362,#209363),(#209364,#209365),(#209366,#209367),
(#209368,#209369),(#209370,#209371),(#209372,#209373),(#209374,#209375),
(#209376,#209377),(#209378,#209379),(#209380,#209381),(#209382,#209383),
(#209384,#209385),(#209386,#209387),(#209388,#209389),(#209390,#209391),
(#209392,#209393),(#209394,#209395),(#209396,#209397),(#209398,#209399),
(#209400,#209401),(#209402,#209403),(#209404,#209405),(#209406,#209407),
(#209408,#209409),(#209410,#209411),(#209412,#209413),(#209414,#209415),
(#209416,#209417),(#209418,#209419),(#209420,#209421),(#209422,#209423),
(#209424,#209425),(#209426,#209427),(#209428,#209429),(#209430,#209431),
(#209432,#209433),(#209434,#209435),(#209436,#209437),(#209438,#209439),
(#209440,#209441),(#209442,#209443),(#209444,#209445),(#209446,#209447),
(#209448,#209449),(#209450,#209451),(#209452,#209453),(#209454,#209455),
(#209456,#209457),(#209458,#209459),(#209460,#209461),(#209462,#209463),
(#209464,#209465),(#209466,#209467),(#209468,#209469),(#209470,#209471),
(#209472,#209473),(#209474,#209475),(#209476,#209477),(#209478,#209479),
(#209480,#209481),(#209482,#209483),(#209484,#209485),(#209486,#209487),
(#209488,#209489),(#209490,#209491),(#209492,#209493),(#209494,#209495),
(#209496,#209497),(#209498,#209499),(#209500,#209501),(#209502,#209503),
(#209504,#209505),(#209506,#209507),(#209508,#209509),(#209510,#209511),
(#209512,#209513),(#209514,#209515),(#209516,#209517),(#209518,#209519),
(#209520,#209521),(#209522,#209523),(#209524,#209525),(#209526,#209527),
(#209528,#209529),(#209530,#209531),(#209532,#209533),(#209534,#209535),
(#209536,#209537),(#209538,#209539),(#209540,#209541),(#209542,#209543),
(#209544,#209545),(#209546,#209547),(#209548,#209549),(#209550,#209551),
(#209552,#209553),(#209554,#209555),(#209556,#209557),(#209558,#209559),
(#209560,#209561),(#209562,#209563),(#209564,#209565),(#209566,#209567),
(#209568,#209569),(#209570,#209571),(#209572,#209573),(#209574,#209575),
(#209576,#209577),(#209578,#209579),(#209580,#209581),(#209582,#209583),
(#209584,#209585),(#209586,#209587),(#209588,#209589),(#209590,#209591),
(#209592,#209593),(#209594,#209595),(#209596,#209597),(#209598,#209599),
(#209600,#209601),(#209602,#209603),(#209604,#209605),(#209606,#209607),
(#209608,#209609),(#209610,#209611),(#209612,#209613),(#209614,#209615),
(#209616,#209617),(#209618,#209619),(#209620,#209621),(#209622,#209623),
(#209624,#209625),(#209626,#209627),(#209628,#209629),(#209630,#209631),
(#209632,#209633),(#209634,#209635),(#209636,#209637),(#209638,#209639),
(#209640,#209641),(#209642,#209643),(#209644,#209645),(#209646,#209647),
(#209648,#209649),(#209650,#209651),(#209652,#209653),(#209654,#209655),
(#209656,#209657),(#209658,#209659),(#209660,#209661),(#209662,#209663),
(#209664,#209665),(#209666,#209667),(#209668,#209669),(#209670,#209671),
(#209672,#209673),(#209674,#209675),(#209676,#209677),(#209678,#209679),
(#209680,#209681),(#209682,#209683),(#209684,#209685),(#209686,#209687),
(#209688,#209689),(#209690,#209691),(#209692,#209693),(#209694,#209695),
(#209696,#209697),(#209698,#209699),(#209700,#209701),(#209702,#209703),
(#209704,#209705),(#209706,#209707),(#209708,#209709),(#209710,#209711),
(#209712,#209713),(#209714,#209715),(#209716,#209717),(#209718,#209719),
(#209720,#209721),(#209722,#209723),(#209724,#209725),(#209726,#209727),
(#209728,#209729),(#209730,#209731),(#209732,#209733),(#209734,#209735),
(#209736,#209737),(#209738,#209739),(#209740,#209741),(#209742,#209743),
(#209744,#209745),(#209746,#209747),(#209748,#209749),(#209750,#209751),
(#209752,#209753),(#209754,#209755),(#209756,#209757),(#209758,#209759),
(#209760,#209761),(#209762,#209763),(#209764,#209765),(#209766,#209767),
(#209768,#209769),(#209770,#209771),(#209772,#209773),(#209774,#209775),
(#209776,#209777),(#209778,#209779),(#209780,#209781),(#209782,#209783),
(#209784,#209785),(#209786,#209787),(#209788,#209789),(#209790,#209791),
(#209792,#209793),(#209794,#209795),(#209796,#209797),(#209798,#209799),
(#209800,#209801),(#209802,#209803),(#209804,#209805),(#209806,#209807),
(#209808,#209809),(#209810,#209811),(#209812,#209813),(#209814,#209815),
(#209816,#209817),(#209818,#209819),(#209820,#209821),(#209822,#209823),
(#209824,#209825),(#209826,#209827),(#209828,#209829),(#209830,#209831),
(#209832,#209833),(#209834,#209835),(#209836,#209837),(#209838,#209839),
(#209840,#209841),(#209842,#209843),(#209844,#209845),(#209846,#209847),
(#209848,#209849),(#209850,#209851),(#209852,#209853),(#209854,#209855),
(#209856,#209857),(#209858,#209859),(#209860,#209861),(#209862,#209863),
(#209864,#209865),(#209866,#209867),(#209868,#209869),(#209870,#209871),
(#209872,#209873),(#209874,#209875),(#209876,#209877),(#209878,#209879),
(#209880,#209881),(#209882,#209883),(#209884,#209885),(#209886,#209887),
(#209888,#209889),(#209890,#209891),(#209892,#209893),(#209894,#209895),
(#209896,#209897),(#209898,#209899),(#209900,#209901),(#209902,#209903),
(#209904,#209905),(#209906,#209907),(#209908,#209909),(#209910,#209911),
(#209912,#209913),(#209914,#209915),(#209916,#209917),(#209918,#209919),
(#209920,#209921),(#209922,#209923),(#209924,#209925),(#209926,#209927),
(#209928,#209929),(#209930,#209931),(#209932,#209933),(#209934,#209935),
(#209936,#209937),(#209938,#209939),(#209940,#209941),(#209942,#209943),
(#209944,#209945),(#209946,#209947),(#209948,#209949),(#209950,#209951),
(#209952,#209953),(#209954,#209955),(#209956,#209957),(#209958,#209959),
(#209960,#209961),(#209962,#209963),(#209964,#209965),(#209966,#209967),
(#209968,#209969),(#209970,#209971)),.UNSPECIFIED.,.F.,.F.,.F.,(6,1,1,1,
1,1,1,1,1,1,1,1,1,1,1,1,1,1,1,1,1,1,1,1,1,1,1,1,1,1,1,1,1,1,1,1,1,1,1,1,
1,1,1,1,1,1,1,1,1,1,1,1,1,1,1,1,1,1,1,1,1,1,1,1,1,1,1,1,1,1,1,1,1,1,1,1,
1,1,1,1,1,1,1,1,1,1,1,1,1,1,1,1,1,1,1,1,1,1,1,1,1,1,1,1,1,1,1,1,1,1,1,1,
1,1,1,1,1,1,1,1,1,1,1,1,1,1,1,1,1,1,1,1,1,1,1,1,1,1,1,1,1,1,1,1,1,1,1,1,
1,1,1,1,1,1,1,1,1,1,1,1,1,1,1,1,1,1,1,1,1,1,1,1,1,1,1,1,1,1,1,1,1,1,1,1,
1,1,1,1,1,1,1,1,1,1,1,1,1,1,1,1,1,1,1,1,1,1,1,1,1,1,1,1,1,1,1,1,1,1,1,1,
1,1,1,1,1,1,1,1,1,1,1,1,1,1,1,1,1,1,1,1,1,1,1,1,1,1,1,1,1,1,1,1,1,1,1,1,
1,1,1,1,1,1,1,1,1,1,1,1,1,1,1,1,1,1,1,1,1,1,1,1,1,1,1,1,1,1,1,1,1,1,1,1,
1,1,1,1,1,1,1,1,1,1,1,1,1,1,1,1,1,1,1,1,1,1,1,1,1,1,1,1,1,1,1,1,1,1,1,1,
1,1,1,1,1,1,1,1,1,1,1,1,1,1,1,1,1,1,1,1,1,1,1,1,1,1,1,1,1,1,1,1,1,1,1,1,
1,1,1,1,1,1,1,1,1,1,1,1,1,1,1,1,1,1,1,1,1,1,1,1,1,1,1,1,1,1,1,1,1,1,1,1,
1,1,1,1,1,1,1,1,1,1,1,1,1,1,1,1,1,1,1,1,1,1,1,1,1,1,1,1,1,1,1,1,1,1,1,1,
1,1,1,1,1,1,1,1,1,1,1,1,1,1,1,1,1,1,1,1,1,1,1,1,1,1,1,1,1,1,1,6),(2,2),
(-1.,-0.998165138,-0.996330275,-0.994495413,-0.99266055,-0.990825688,-0.988990826,
-0.987155963,-0.985321101,-0.983486239,-0.981651376,-0.979816514,-0.977981651,
-0.976146789,-0.974311927,-0.972477064,-0.970642202,-0.968807339,-0.966972477,
-0.965137615,-0.963302752,-0.96146789,-0.959633028,-0.957798165,-0.955963303,
-0.95412844,-0.952293578,-0.950458716,-0.948623853,-0.946788991,-0.944954128,
-0.943119266,-0.941284404,-0.939449541,-0.937614679,-0.935779817,-0.933944954,
-0.932110092,-0.930275229,-0.928440367,-0.926605505,-0.924770642,-0.92293578,
-0.921100917,-0.919266055,-0.917431193,-0.91559633,-0.913761468,-0.911926606,
-0.910091743,-0.908256881,-0.906422018,-0.904587156,-0.902752294,-0.900917431,
-0.899082569,-0.897247706,-0.895412844,-0.893577982,-0.891743119,-0.889908257,
-0.888073394,-0.886238532,-0.88440367,-0.882568807,-0.880733945,-0.878899083,
-0.87706422,-0.875229358,-0.873394495,-0.871559633,-0.869724771,-0.867889908,
-0.866055046,-0.864220183,-0.862385321,-0.860550459,-0.858715596,-0.856880734,
-0.855045872,-0.853211009,-0.851376147,-0.849541284,-0.847706422,-0.84587156,
-0.844036697,-0.842201835,-0.840366972,-0.83853211,-0.836697248,-0.834862385,
-0.833027523,-0.831192661,-0.829357798,-0.827522936,-0.825688073,-0.823853211,
-0.822018349,-0.820183486,-0.818348624,-0.816513761,-0.814678899,-0.812844037,
-0.811009174,-0.809174312,-0.80733945,-0.805504587,-0.803669725,-0.801834862,
-0.8,-0.798165138,-0.796330275,-0.794495413,-0.79266055,-0.790825688,-0.788990826,
-0.787155963,-0.785321101,-0.783486239,-0.781651376,-0.779816514,-0.777981651,
-0.776146789,-0.774311927,-0.772477064,-0.770642202,-0.768807339,-0.766972477,
-0.765137615,-0.763302752,-0.76146789,-0.759633028,-0.757798165,-0.755963303,
-0.75412844,-0.752293578,-0.750458716,-0.748623853,-0.746788991,-0.744954128,
-0.743119266,-0.741284404,-0.739449541,-0.737614679,-0.735779817,-0.733944954,
-0.732110092,-0.730275229,-0.728440367,-0.726605505,-0.724770642,-0.72293578,
-0.721100917,-0.719266055,-0.717431193,-0.71559633,-0.713761468,-0.711926606,
-0.710091743,-0.708256881,-0.706422018,-0.704587156,-0.702752294,-0.700917431,
-0.699082569,-0.697247706,-0.695412844,-0.693577982,-0.691743119,-0.689908257,
-0.688073394,-0.686238532,-0.68440367,-0.682568807,-0.680733945,-0.678899083,
-0.67706422,-0.675229358,-0.673394495,-0.671559633,-0.669724771,-0.667889908,
-0.666055046,-0.664220183,-0.662385321,-0.660550459,-0.658715596,-0.656880734,
-0.655045872,-0.653211009,-0.651376147,-0.649541284,-0.647706422,-0.64587156,
-0.644036697,-0.642201835,-0.640366972,-0.63853211,-0.636697248,-0.634862385,
-0.633027523,-0.631192661,-0.629357798,-0.627522936,-0.625688073,-0.623853211,
-0.622018349,-0.620183486,-0.618348624,-0.616513761,-0.614678899,-0.612844037,
-0.611009174,-0.609174312,-0.60733945,-0.605504587,-0.603669725,-0.601834862,
-0.6,-0.598165138,-0.596330275,-0.594495413,-0.59266055,-0.590825688,-0.588990826,
-0.587155963,-0.585321101,-0.583486239,-0.581651376,-0.579816514,-0.577981651,
-0.576146789,-0.574311927,-0.572477064,-0.570642202,-0.568807339,-0.566972477,
-0.565137615,-0.563302752,-0.56146789,-0.559633028,-0.557798165,-0.555963303,
-0.55412844,-0.552293578,-0.550458716,-0.548623853,-0.546788991,-0.544954128,
-0.543119266,-0.541284404,-0.539449541,-0.537614679,-0.535779817,-0.533944954,
-0.532110092,-0.530275229,-0.528440367,-0.526605505,-0.524770642,-0.52293578,
-0.521100917,-0.519266055,-0.517431193,-0.51559633,-0.513761468,-0.511926606,
-0.510091743,-0.508256881,-0.506422018,-0.504587156,-0.502752294,-0.500917431,
-0.499082569,-0.497247706,-0.495412844,-0.493577982,-0.491743119,-0.489908257,
-0.488073394,-0.486238532,-0.48440367,-0.482568807,-0.480733945,-0.478899083,
-0.47706422,-0.475229358,-0.473394495,-0.471559633,-0.469724771,-0.467889908,
-0.466055046,-0.464220183,-0.462385321,-0.460550459,-0.458715596,-0.456880734,
-0.455045872,-0.453211009,-0.451376147,-0.449541284,-0.447706422,-0.44587156,
-0.444036697,-0.442201835,-0.440366972,-0.43853211,-0.436697248,-0.434862385,
-0.433027523,-0.431192661,-0.429357798,-0.427522936,-0.425688073,-0.423853211,
-0.422018349,-0.420183486,-0.418348624,-0.416513761,-0.414678899,-0.412844037,
-0.411009174,-0.409174312,-0.40733945,-0.405504587,-0.403669725,-0.401834862,
-0.4,-0.398165138,-0.396330275,-0.394495413,-0.39266055,-0.390825688,-0.388990826,
-0.387155963,-0.385321101,-0.383486239,-0.381651376,-0.379816514,-0.377981651,
-0.376146789,-0.374311927,-0.372477064,-0.370642202,-0.368807339,-0.366972477,
-0.365137615,-0.363302752,-0.36146789,-0.359633028,-0.357798165,-0.355963303,
-0.35412844,-0.352293578,-0.350458716,-0.348623853,-0.346788991,-0.344954128,
-0.343119266,-0.341284404,-0.339449541,-0.337614679,-0.335779817,-0.333944954,
-0.332110092,-0.330275229,-0.328440367,-0.326605505,-0.324770642,-0.32293578,
-0.321100917,-0.319266055,-0.317431193,-0.31559633,-0.313761468,-0.311926606,
-0.310091743,-0.308256881,-0.306422018,-0.304587156,-0.302752294,-0.300917431,
-0.299082569,-0.297247706,-0.295412844,-0.293577982,-0.291743119,-0.289908257,
-0.288073394,-0.286238532,-0.28440367,-0.282568807,-0.280733945,-0.278899083,
-0.27706422,-0.275229358,-0.273394495,-0.271559633,-0.269724771,-0.267889908,
-0.266055046,-0.264220183,-0.262385321,-0.260550459,-0.258715596,-0.256880734,
-0.255045872,-0.253211009,-0.251376147,-0.249541284,-0.247706422,-0.24587156,
-0.244036697,-0.242201835,-0.240366972,-0.23853211,-0.236697248,-0.234862385,
-0.233027523,-0.231192661,-0.229357798,-0.227522936,-0.225688073,-0.223853211,
-0.222018349,-0.220183486,-0.218348624,-0.216513761,-0.214678899,-0.212844037,
-0.211009174,-0.209174312,-0.20733945,-0.205504587,-0.203669725,-0.201834862,
-0.2,-0.198165138,-0.196330275,-0.194495413,-0.19266055,-0.190825688,-0.188990826,
-0.187155963,-0.185321101,-0.183486239,-0.181651376,-0.179816514,-0.177981651,
-0.176146789,-0.174311927,-0.172477064,-0.170642202,-0.168807339,-0.166972477,
-0.165137615,-0.163302752,-0.16146789,-0.159633028,-0.157798165,-0.155963303,
-0.15412844,-0.152293578,-0.150458716,-0.148623853,-0.146788991,-0.144954128,
-0.143172103),(0.,0.36),.UNSPECIFIED.);
#6249=B_SPLINE_SURFACE_WITH_KNOTS('',5,1,((#210625,#210626),(#210627,#210628),
(#210629,#210630),(#210631,#210632),(#210633,#210634),(#210635,#210636),
(#210637,#210638),(#210639,#210640),(#210641,#210642),(#210643,#210644),
(#210645,#210646),(#210647,#210648),(#210649,#210650),(#210651,#210652),
(#210653,#210654),(#210655,#210656),(#210657,#210658),(#210659,#210660),
(#210661,#210662),(#210663,#210664),(#210665,#210666),(#210667,#210668),
(#210669,#210670),(#210671,#210672),(#210673,#210674),(#210675,#210676),
(#210677,#210678),(#210679,#210680),(#210681,#210682),(#210683,#210684),
(#210685,#210686),(#210687,#210688),(#210689,#210690),(#210691,#210692),
(#210693,#210694),(#210695,#210696),(#210697,#210698),(#210699,#210700),
(#210701,#210702),(#210703,#210704),(#210705,#210706),(#210707,#210708),
(#210709,#210710),(#210711,#210712),(#210713,#210714),(#210715,#210716),
(#210717,#210718),(#210719,#210720),(#210721,#210722),(#210723,#210724),
(#210725,#210726),(#210727,#210728),(#210729,#210730),(#210731,#210732),
(#210733,#210734),(#210735,#210736),(#210737,#210738),(#210739,#210740),
(#210741,#210742),(#210743,#210744),(#210745,#210746),(#210747,#210748),
(#210749,#210750),(#210751,#210752),(#210753,#210754),(#210755,#210756),
(#210757,#210758),(#210759,#210760),(#210761,#210762),(#210763,#210764),
(#210765,#210766),(#210767,#210768),(#210769,#210770),(#210771,#210772),
(#210773,#210774),(#210775,#210776),(#210777,#210778),(#210779,#210780),
(#210781,#210782),(#210783,#210784),(#210785,#210786),(#210787,#210788),
(#210789,#210790),(#210791,#210792),(#210793,#210794),(#210795,#210796),
(#210797,#210798),(#210799,#210800),(#210801,#210802),(#210803,#210804),
(#210805,#210806),(#210807,#210808),(#210809,#210810),(#210811,#210812),
(#210813,#210814),(#210815,#210816),(#210817,#210818),(#210819,#210820),
(#210821,#210822),(#210823,#210824),(#210825,#210826),(#210827,#210828),
(#210829,#210830),(#210831,#210832),(#210833,#210834),(#210835,#210836),
(#210837,#210838),(#210839,#210840),(#210841,#210842),(#210843,#210844),
(#210845,#210846),(#210847,#210848),(#210849,#210850),(#210851,#210852),
(#210853,#210854),(#210855,#210856),(#210857,#210858),(#210859,#210860),
(#210861,#210862),(#210863,#210864),(#210865,#210866),(#210867,#210868),
(#210869,#210870),(#210871,#210872),(#210873,#210874),(#210875,#210876),
(#210877,#210878),(#210879,#210880),(#210881,#210882),(#210883,#210884),
(#210885,#210886),(#210887,#210888),(#210889,#210890),(#210891,#210892),
(#210893,#210894),(#210895,#210896),(#210897,#210898),(#210899,#210900),
(#210901,#210902),(#210903,#210904),(#210905,#210906),(#210907,#210908),
(#210909,#210910),(#210911,#210912),(#210913,#210914),(#210915,#210916),
(#210917,#210918),(#210919,#210920),(#210921,#210922),(#210923,#210924),
(#210925,#210926),(#210927,#210928),(#210929,#210930),(#210931,#210932),
(#210933,#210934),(#210935,#210936),(#210937,#210938),(#210939,#210940),
(#210941,#210942),(#210943,#210944),(#210945,#210946),(#210947,#210948),
(#210949,#210950),(#210951,#210952),(#210953,#210954),(#210955,#210956),
(#210957,#210958),(#210959,#210960),(#210961,#210962),(#210963,#210964),
(#210965,#210966),(#210967,#210968),(#210969,#210970),(#210971,#210972),
(#210973,#210974),(#210975,#210976),(#210977,#210978),(#210979,#210980),
(#210981,#210982),(#210983,#210984),(#210985,#210986),(#210987,#210988),
(#210989,#210990),(#210991,#210992),(#210993,#210994),(#210995,#210996),
(#210997,#210998),(#210999,#211000),(#211001,#211002),(#211003,#211004),
(#211005,#211006),(#211007,#211008),(#211009,#211010),(#211011,#211012),
(#211013,#211014),(#211015,#211016),(#211017,#211018),(#211019,#211020),
(#211021,#211022),(#211023,#211024),(#211025,#211026),(#211027,#211028),
(#211029,#211030),(#211031,#211032),(#211033,#211034),(#211035,#211036),
(#211037,#211038),(#211039,#211040),(#211041,#211042),(#211043,#211044),
(#211045,#211046),(#211047,#211048),(#211049,#211050),(#211051,#211052),
(#211053,#211054),(#211055,#211056),(#211057,#211058),(#211059,#211060),
(#211061,#211062),(#211063,#211064),(#211065,#211066),(#211067,#211068),
(#211069,#211070),(#211071,#211072),(#211073,#211074),(#211075,#211076),
(#211077,#211078),(#211079,#211080),(#211081,#211082),(#211083,#211084),
(#211085,#211086),(#211087,#211088),(#211089,#211090),(#211091,#211092),
(#211093,#211094),(#211095,#211096),(#211097,#211098),(#211099,#211100),
(#211101,#211102),(#211103,#211104),(#211105,#211106),(#211107,#211108),
(#211109,#211110),(#211111,#211112),(#211113,#211114),(#211115,#211116),
(#211117,#211118),(#211119,#211120),(#211121,#211122),(#211123,#211124),
(#211125,#211126),(#211127,#211128),(#211129,#211130),(#211131,#211132),
(#211133,#211134),(#211135,#211136),(#211137,#211138),(#211139,#211140),
(#211141,#211142),(#211143,#211144),(#211145,#211146),(#211147,#211148),
(#211149,#211150),(#211151,#211152),(#211153,#211154),(#211155,#211156),
(#211157,#211158),(#211159,#211160),(#211161,#211162),(#211163,#211164),
(#211165,#211166),(#211167,#211168),(#211169,#211170),(#211171,#211172),
(#211173,#211174),(#211175,#211176),(#211177,#211178),(#211179,#211180),
(#211181,#211182),(#211183,#211184),(#211185,#211186),(#211187,#211188),
(#211189,#211190),(#211191,#211192),(#211193,#211194),(#211195,#211196),
(#211197,#211198),(#211199,#211200),(#211201,#211202),(#211203,#211204),
(#211205,#211206),(#211207,#211208),(#211209,#211210),(#211211,#211212),
(#211213,#211214),(#211215,#211216),(#211217,#211218),(#211219,#211220),
(#211221,#211222),(#211223,#211224),(#211225,#211226),(#211227,#211228),
(#211229,#211230),(#211231,#211232),(#211233,#211234),(#211235,#211236),
(#211237,#211238),(#211239,#211240),(#211241,#211242),(#211243,#211244),
(#211245,#211246),(#211247,#211248),(#211249,#211250),(#211251,#211252),
(#211253,#211254),(#211255,#211256),(#211257,#211258),(#211259,#211260),
(#211261,#211262),(#211263,#211264),(#211265,#211266),(#211267,#211268),
(#211269,#211270),(#211271,#211272),(#211273,#211274),(#211275,#211276),
(#211277,#211278),(#211279,#211280),(#211281,#211282),(#211283,#211284),
(#211285,#211286),(#211287,#211288),(#211289,#211290),(#211291,#211292),
(#211293,#211294),(#211295,#211296),(#211297,#211298),(#211299,#211300),
(#211301,#211302),(#211303,#211304),(#211305,#211306),(#211307,#211308),
(#211309,#211310),(#211311,#211312),(#211313,#211314),(#211315,#211316),
(#211317,#211318),(#211319,#211320),(#211321,#211322),(#211323,#211324),
(#211325,#211326),(#211327,#211328),(#211329,#211330),(#211331,#211332),
(#211333,#211334),(#211335,#211336),(#211337,#211338),(#211339,#211340),
(#211341,#211342),(#211343,#211344),(#211345,#211346),(#211347,#211348),
(#211349,#211350),(#211351,#211352),(#211353,#211354),(#211355,#211356),
(#211357,#211358),(#211359,#211360),(#211361,#211362),(#211363,#211364),
(#211365,#211366),(#211367,#211368),(#211369,#211370),(#211371,#211372),
(#211373,#211374),(#211375,#211376),(#211377,#211378),(#211379,#211380),
(#211381,#211382),(#211383,#211384),(#211385,#211386),(#211387,#211388),
(#211389,#211390),(#211391,#211392),(#211393,#211394),(#211395,#211396),
(#211397,#211398),(#211399,#211400),(#211401,#211402),(#211403,#211404),
(#211405,#211406),(#211407,#211408),(#211409,#211410),(#211411,#211412),
(#211413,#211414),(#211415,#211416),(#211417,#211418),(#211419,#211420),
(#211421,#211422),(#211423,#211424),(#211425,#211426),(#211427,#211428),
(#211429,#211430),(#211431,#211432),(#211433,#211434),(#211435,#211436),
(#211437,#211438),(#211439,#211440),(#211441,#211442),(#211443,#211444),
(#211445,#211446),(#211447,#211448),(#211449,#211450),(#211451,#211452),
(#211453,#211454),(#211455,#211456),(#211457,#211458),(#211459,#211460),
(#211461,#211462),(#211463,#211464),(#211465,#211466),(#211467,#211468),
(#211469,#211470),(#211471,#211472),(#211473,#211474),(#211475,#211476),
(#211477,#211478),(#211479,#211480),(#211481,#211482),(#211483,#211484),
(#211485,#211486),(#211487,#211488),(#211489,#211490),(#211491,#211492),
(#211493,#211494),(#211495,#211496),(#211497,#211498),(#211499,#211500),
(#211501,#211502),(#211503,#211504),(#211505,#211506),(#211507,#211508),
(#211509,#211510),(#211511,#211512),(#211513,#211514),(#211515,#211516),
(#211517,#211518),(#211519,#211520),(#211521,#211522),(#211523,#211524),
(#211525,#211526),(#211527,#211528),(#211529,#211530),(#211531,#211532),
(#211533,#211534),(#211535,#211536),(#211537,#211538),(#211539,#211540),
(#211541,#211542),(#211543,#211544),(#211545,#211546),(#211547,#211548),
(#211549,#211550),(#211551,#211552),(#211553,#211554),(#211555,#211556),
(#211557,#211558),(#211559,#211560),(#211561,#211562),(#211563,#211564),
(#211565,#211566),(#211567,#211568)),.UNSPECIFIED.,.F.,.F.,.F.,(6,1,1,1,
1,1,1,1,1,1,1,1,1,1,1,1,1,1,1,1,1,1,1,1,1,1,1,1,1,1,1,1,1,1,1,1,1,1,1,1,
1,1,1,1,1,1,1,1,1,1,1,1,1,1,1,1,1,1,1,1,1,1,1,1,1,1,1,1,1,1,1,1,1,1,1,1,
1,1,1,1,1,1,1,1,1,1,1,1,1,1,1,1,1,1,1,1,1,1,1,1,1,1,1,1,1,1,1,1,1,1,1,1,
1,1,1,1,1,1,1,1,1,1,1,1,1,1,1,1,1,1,1,1,1,1,1,1,1,1,1,1,1,1,1,1,1,1,1,1,
1,1,1,1,1,1,1,1,1,1,1,1,1,1,1,1,1,1,1,1,1,1,1,1,1,1,1,1,1,1,1,1,1,1,1,1,
1,1,1,1,1,1,1,1,1,1,1,1,1,1,1,1,1,1,1,1,1,1,1,1,1,1,1,1,1,1,1,1,1,1,1,1,
1,1,1,1,1,1,1,1,1,1,1,1,1,1,1,1,1,1,1,1,1,1,1,1,1,1,1,1,1,1,1,1,1,1,1,1,
1,1,1,1,1,1,1,1,1,1,1,1,1,1,1,1,1,1,1,1,1,1,1,1,1,1,1,1,1,1,1,1,1,1,1,1,
1,1,1,1,1,1,1,1,1,1,1,1,1,1,1,1,1,1,1,1,1,1,1,1,1,1,1,1,1,1,1,1,1,1,1,1,
1,1,1,1,1,1,1,1,1,1,1,1,1,1,1,1,1,1,1,1,1,1,1,1,1,1,1,1,1,1,1,1,1,1,1,1,
1,1,1,1,1,1,1,1,1,1,1,1,1,1,1,1,1,1,1,1,1,1,1,1,1,1,1,1,1,1,1,1,1,1,1,1,
1,1,1,1,1,1,1,1,1,1,1,1,1,1,1,1,1,1,1,1,1,1,1,1,1,1,1,1,1,1,1,1,1,1,1,1,
1,1,1,1,1,1,1,1,1,1,1,1,1,1,1,1,1,1,1,1,1,1,1,1,1,1,1,1,1,1,1,6),(2,2),
(-1.,-0.998165138,-0.996330275,-0.994495413,-0.99266055,-0.990825688,-0.988990826,
-0.987155963,-0.985321101,-0.983486239,-0.981651376,-0.979816514,-0.977981651,
-0.976146789,-0.974311927,-0.972477064,-0.970642202,-0.968807339,-0.966972477,
-0.965137615,-0.963302752,-0.96146789,-0.959633028,-0.957798165,-0.955963303,
-0.95412844,-0.952293578,-0.950458716,-0.948623853,-0.946788991,-0.944954128,
-0.943119266,-0.941284404,-0.939449541,-0.937614679,-0.935779817,-0.933944954,
-0.932110092,-0.930275229,-0.928440367,-0.926605505,-0.924770642,-0.92293578,
-0.921100917,-0.919266055,-0.917431193,-0.91559633,-0.913761468,-0.911926606,
-0.910091743,-0.908256881,-0.906422018,-0.904587156,-0.902752294,-0.900917431,
-0.899082569,-0.897247706,-0.895412844,-0.893577982,-0.891743119,-0.889908257,
-0.888073394,-0.886238532,-0.88440367,-0.882568807,-0.880733945,-0.878899083,
-0.87706422,-0.875229358,-0.873394495,-0.871559633,-0.869724771,-0.867889908,
-0.866055046,-0.864220183,-0.862385321,-0.860550459,-0.858715596,-0.856880734,
-0.855045872,-0.853211009,-0.851376147,-0.849541284,-0.847706422,-0.84587156,
-0.844036697,-0.842201835,-0.840366972,-0.83853211,-0.836697248,-0.834862385,
-0.833027523,-0.831192661,-0.829357798,-0.827522936,-0.825688073,-0.823853211,
-0.822018349,-0.820183486,-0.818348624,-0.816513761,-0.814678899,-0.812844037,
-0.811009174,-0.809174312,-0.80733945,-0.805504587,-0.803669725,-0.801834862,
-0.8,-0.798165138,-0.796330275,-0.794495413,-0.79266055,-0.790825688,-0.788990826,
-0.787155963,-0.785321101,-0.783486239,-0.781651376,-0.779816514,-0.777981651,
-0.776146789,-0.774311927,-0.772477064,-0.770642202,-0.768807339,-0.766972477,
-0.765137615,-0.763302752,-0.76146789,-0.759633028,-0.757798165,-0.755963303,
-0.75412844,-0.752293578,-0.750458716,-0.748623853,-0.746788991,-0.744954128,
-0.743119266,-0.741284404,-0.739449541,-0.737614679,-0.735779817,-0.733944954,
-0.732110092,-0.730275229,-0.728440367,-0.726605505,-0.724770642,-0.72293578,
-0.721100917,-0.719266055,-0.717431193,-0.71559633,-0.713761468,-0.711926606,
-0.710091743,-0.708256881,-0.706422018,-0.704587156,-0.702752294,-0.700917431,
-0.699082569,-0.697247706,-0.695412844,-0.693577982,-0.691743119,-0.689908257,
-0.688073394,-0.686238532,-0.68440367,-0.682568807,-0.680733945,-0.678899083,
-0.67706422,-0.675229358,-0.673394495,-0.671559633,-0.669724771,-0.667889908,
-0.666055046,-0.664220183,-0.662385321,-0.660550459,-0.658715596,-0.656880734,
-0.655045872,-0.653211009,-0.651376147,-0.649541284,-0.647706422,-0.64587156,
-0.644036697,-0.642201835,-0.640366972,-0.63853211,-0.636697248,-0.634862385,
-0.633027523,-0.631192661,-0.629357798,-0.627522936,-0.625688073,-0.623853211,
-0.622018349,-0.620183486,-0.618348624,-0.616513761,-0.614678899,-0.612844037,
-0.611009174,-0.609174312,-0.60733945,-0.605504587,-0.603669725,-0.601834862,
-0.6,-0.598165138,-0.596330275,-0.594495413,-0.59266055,-0.590825688,-0.588990826,
-0.587155963,-0.585321101,-0.583486239,-0.581651376,-0.579816514,-0.577981651,
-0.576146789,-0.574311927,-0.572477064,-0.570642202,-0.568807339,-0.566972477,
-0.565137615,-0.563302752,-0.56146789,-0.559633028,-0.557798165,-0.555963303,
-0.55412844,-0.552293578,-0.550458716,-0.548623853,-0.546788991,-0.544954128,
-0.543119266,-0.541284404,-0.539449541,-0.537614679,-0.535779817,-0.533944954,
-0.532110092,-0.530275229,-0.528440367,-0.526605505,-0.524770642,-0.52293578,
-0.521100917,-0.519266055,-0.517431193,-0.51559633,-0.513761468,-0.511926606,
-0.510091743,-0.508256881,-0.506422018,-0.504587156,-0.502752294,-0.500917431,
-0.499082569,-0.497247706,-0.495412844,-0.493577982,-0.491743119,-0.489908257,
-0.488073394,-0.486238532,-0.48440367,-0.482568807,-0.480733945,-0.478899083,
-0.47706422,-0.475229358,-0.473394495,-0.471559633,-0.469724771,-0.467889908,
-0.466055046,-0.464220183,-0.462385321,-0.460550459,-0.458715596,-0.456880734,
-0.455045872,-0.453211009,-0.451376147,-0.449541284,-0.447706422,-0.44587156,
-0.444036697,-0.442201835,-0.440366972,-0.43853211,-0.436697248,-0.434862385,
-0.433027523,-0.431192661,-0.429357798,-0.427522936,-0.425688073,-0.423853211,
-0.422018349,-0.420183486,-0.418348624,-0.416513761,-0.414678899,-0.412844037,
-0.411009174,-0.409174312,-0.40733945,-0.405504587,-0.403669725,-0.401834862,
-0.4,-0.398165138,-0.396330275,-0.394495413,-0.39266055,-0.390825688,-0.388990826,
-0.387155963,-0.385321101,-0.383486239,-0.381651376,-0.379816514,-0.377981651,
-0.376146789,-0.374311927,-0.372477064,-0.370642202,-0.368807339,-0.366972477,
-0.365137615,-0.363302752,-0.36146789,-0.359633028,-0.357798165,-0.355963303,
-0.35412844,-0.352293578,-0.350458716,-0.348623853,-0.346788991,-0.344954128,
-0.343119266,-0.341284404,-0.339449541,-0.337614679,-0.335779817,-0.333944954,
-0.332110092,-0.330275229,-0.328440367,-0.326605505,-0.324770642,-0.32293578,
-0.321100917,-0.319266055,-0.317431193,-0.31559633,-0.313761468,-0.311926606,
-0.310091743,-0.308256881,-0.306422018,-0.304587156,-0.302752294,-0.300917431,
-0.299082569,-0.297247706,-0.295412844,-0.293577982,-0.291743119,-0.289908257,
-0.288073394,-0.286238532,-0.28440367,-0.282568807,-0.280733945,-0.278899083,
-0.27706422,-0.275229358,-0.273394495,-0.271559633,-0.269724771,-0.267889908,
-0.266055046,-0.264220183,-0.262385321,-0.260550459,-0.258715596,-0.256880734,
-0.255045872,-0.253211009,-0.251376147,-0.249541284,-0.247706422,-0.24587156,
-0.244036697,-0.242201835,-0.240366972,-0.23853211,-0.236697248,-0.234862385,
-0.233027523,-0.231192661,-0.229357798,-0.227522936,-0.225688073,-0.223853211,
-0.222018349,-0.220183486,-0.218348624,-0.216513761,-0.214678899,-0.212844037,
-0.211009174,-0.209174312,-0.20733945,-0.205504587,-0.203669725,-0.201834862,
-0.2,-0.198165138,-0.196330275,-0.194495413,-0.19266055,-0.190825688,-0.188990826,
-0.187155963,-0.185321101,-0.183486239,-0.181651376,-0.179816514,-0.177981651,
-0.176146789,-0.174311927,-0.172477064,-0.170642202,-0.168807339,-0.166972477,
-0.165137615,-0.163302752,-0.16146789,-0.159633028,-0.157798165,-0.155963303,
-0.15412844,-0.152293578,-0.150458716,-0.148623853,-0.146788991,-0.144954128,
-0.143172103),(0.,0.36),.UNSPECIFIED.);
#6250=B_SPLINE_SURFACE_WITH_KNOTS('',5,1,((#212195,#212196),(#212197,#212198),
(#212199,#212200),(#212201,#212202),(#212203,#212204),(#212205,#212206),
(#212207,#212208),(#212209,#212210),(#212211,#212212),(#212213,#212214),
(#212215,#212216),(#212217,#212218),(#212219,#212220),(#212221,#212222),
(#212223,#212224),(#212225,#212226),(#212227,#212228),(#212229,#212230),
(#212231,#212232),(#212233,#212234),(#212235,#212236),(#212237,#212238),
(#212239,#212240),(#212241,#212242),(#212243,#212244),(#212245,#212246),
(#212247,#212248),(#212249,#212250),(#212251,#212252),(#212253,#212254),
(#212255,#212256),(#212257,#212258),(#212259,#212260),(#212261,#212262),
(#212263,#212264),(#212265,#212266),(#212267,#212268),(#212269,#212270),
(#212271,#212272),(#212273,#212274),(#212275,#212276),(#212277,#212278),
(#212279,#212280),(#212281,#212282),(#212283,#212284),(#212285,#212286),
(#212287,#212288),(#212289,#212290),(#212291,#212292),(#212293,#212294),
(#212295,#212296),(#212297,#212298),(#212299,#212300),(#212301,#212302),
(#212303,#212304),(#212305,#212306),(#212307,#212308),(#212309,#212310),
(#212311,#212312),(#212313,#212314),(#212315,#212316),(#212317,#212318),
(#212319,#212320),(#212321,#212322),(#212323,#212324),(#212325,#212326),
(#212327,#212328),(#212329,#212330),(#212331,#212332),(#212333,#212334),
(#212335,#212336),(#212337,#212338),(#212339,#212340),(#212341,#212342),
(#212343,#212344),(#212345,#212346),(#212347,#212348),(#212349,#212350),
(#212351,#212352),(#212353,#212354),(#212355,#212356),(#212357,#212358),
(#212359,#212360),(#212361,#212362),(#212363,#212364),(#212365,#212366),
(#212367,#212368),(#212369,#212370),(#212371,#212372),(#212373,#212374),
(#212375,#212376),(#212377,#212378),(#212379,#212380),(#212381,#212382),
(#212383,#212384),(#212385,#212386),(#212387,#212388),(#212389,#212390),
(#212391,#212392),(#212393,#212394),(#212395,#212396),(#212397,#212398),
(#212399,#212400),(#212401,#212402),(#212403,#212404),(#212405,#212406),
(#212407,#212408),(#212409,#212410),(#212411,#212412),(#212413,#212414),
(#212415,#212416),(#212417,#212418),(#212419,#212420),(#212421,#212422),
(#212423,#212424),(#212425,#212426),(#212427,#212428),(#212429,#212430),
(#212431,#212432),(#212433,#212434),(#212435,#212436),(#212437,#212438),
(#212439,#212440),(#212441,#212442),(#212443,#212444),(#212445,#212446),
(#212447,#212448),(#212449,#212450),(#212451,#212452),(#212453,#212454),
(#212455,#212456),(#212457,#212458),(#212459,#212460),(#212461,#212462),
(#212463,#212464),(#212465,#212466),(#212467,#212468),(#212469,#212470),
(#212471,#212472),(#212473,#212474),(#212475,#212476),(#212477,#212478),
(#212479,#212480),(#212481,#212482),(#212483,#212484),(#212485,#212486),
(#212487,#212488),(#212489,#212490),(#212491,#212492),(#212493,#212494),
(#212495,#212496),(#212497,#212498),(#212499,#212500),(#212501,#212502),
(#212503,#212504),(#212505,#212506),(#212507,#212508),(#212509,#212510),
(#212511,#212512),(#212513,#212514),(#212515,#212516),(#212517,#212518),
(#212519,#212520),(#212521,#212522),(#212523,#212524),(#212525,#212526),
(#212527,#212528),(#212529,#212530),(#212531,#212532),(#212533,#212534),
(#212535,#212536),(#212537,#212538),(#212539,#212540),(#212541,#212542),
(#212543,#212544),(#212545,#212546),(#212547,#212548),(#212549,#212550),
(#212551,#212552),(#212553,#212554),(#212555,#212556),(#212557,#212558),
(#212559,#212560),(#212561,#212562),(#212563,#212564),(#212565,#212566),
(#212567,#212568),(#212569,#212570),(#212571,#212572),(#212573,#212574),
(#212575,#212576),(#212577,#212578),(#212579,#212580),(#212581,#212582),
(#212583,#212584),(#212585,#212586),(#212587,#212588),(#212589,#212590),
(#212591,#212592),(#212593,#212594),(#212595,#212596),(#212597,#212598),
(#212599,#212600),(#212601,#212602),(#212603,#212604),(#212605,#212606),
(#212607,#212608),(#212609,#212610),(#212611,#212612),(#212613,#212614),
(#212615,#212616),(#212617,#212618),(#212619,#212620),(#212621,#212622),
(#212623,#212624),(#212625,#212626),(#212627,#212628),(#212629,#212630),
(#212631,#212632),(#212633,#212634),(#212635,#212636),(#212637,#212638),
(#212639,#212640),(#212641,#212642),(#212643,#212644),(#212645,#212646),
(#212647,#212648),(#212649,#212650),(#212651,#212652),(#212653,#212654),
(#212655,#212656),(#212657,#212658),(#212659,#212660),(#212661,#212662),
(#212663,#212664),(#212665,#212666),(#212667,#212668),(#212669,#212670),
(#212671,#212672),(#212673,#212674),(#212675,#212676),(#212677,#212678),
(#212679,#212680),(#212681,#212682),(#212683,#212684),(#212685,#212686),
(#212687,#212688),(#212689,#212690),(#212691,#212692),(#212693,#212694),
(#212695,#212696),(#212697,#212698),(#212699,#212700),(#212701,#212702),
(#212703,#212704),(#212705,#212706),(#212707,#212708),(#212709,#212710),
(#212711,#212712),(#212713,#212714),(#212715,#212716),(#212717,#212718),
(#212719,#212720),(#212721,#212722),(#212723,#212724),(#212725,#212726),
(#212727,#212728),(#212729,#212730),(#212731,#212732),(#212733,#212734),
(#212735,#212736),(#212737,#212738),(#212739,#212740),(#212741,#212742),
(#212743,#212744),(#212745,#212746),(#212747,#212748),(#212749,#212750),
(#212751,#212752),(#212753,#212754),(#212755,#212756),(#212757,#212758),
(#212759,#212760),(#212761,#212762),(#212763,#212764),(#212765,#212766),
(#212767,#212768),(#212769,#212770),(#212771,#212772),(#212773,#212774),
(#212775,#212776),(#212777,#212778),(#212779,#212780),(#212781,#212782),
(#212783,#212784),(#212785,#212786),(#212787,#212788),(#212789,#212790),
(#212791,#212792),(#212793,#212794),(#212795,#212796),(#212797,#212798),
(#212799,#212800),(#212801,#212802),(#212803,#212804),(#212805,#212806),
(#212807,#212808),(#212809,#212810),(#212811,#212812),(#212813,#212814),
(#212815,#212816),(#212817,#212818),(#212819,#212820),(#212821,#212822),
(#212823,#212824),(#212825,#212826),(#212827,#212828),(#212829,#212830),
(#212831,#212832),(#212833,#212834),(#212835,#212836),(#212837,#212838),
(#212839,#212840),(#212841,#212842),(#212843,#212844),(#212845,#212846),
(#212847,#212848),(#212849,#212850),(#212851,#212852),(#212853,#212854),
(#212855,#212856),(#212857,#212858),(#212859,#212860),(#212861,#212862),
(#212863,#212864),(#212865,#212866),(#212867,#212868),(#212869,#212870),
(#212871,#212872),(#212873,#212874),(#212875,#212876),(#212877,#212878),
(#212879,#212880),(#212881,#212882),(#212883,#212884),(#212885,#212886),
(#212887,#212888),(#212889,#212890),(#212891,#212892),(#212893,#212894),
(#212895,#212896),(#212897,#212898),(#212899,#212900),(#212901,#212902),
(#212903,#212904),(#212905,#212906),(#212907,#212908),(#212909,#212910),
(#212911,#212912),(#212913,#212914),(#212915,#212916),(#212917,#212918),
(#212919,#212920),(#212921,#212922),(#212923,#212924),(#212925,#212926),
(#212927,#212928),(#212929,#212930),(#212931,#212932),(#212933,#212934),
(#212935,#212936),(#212937,#212938),(#212939,#212940),(#212941,#212942),
(#212943,#212944),(#212945,#212946),(#212947,#212948),(#212949,#212950),
(#212951,#212952),(#212953,#212954),(#212955,#212956),(#212957,#212958),
(#212959,#212960),(#212961,#212962),(#212963,#212964),(#212965,#212966),
(#212967,#212968),(#212969,#212970),(#212971,#212972),(#212973,#212974),
(#212975,#212976),(#212977,#212978),(#212979,#212980),(#212981,#212982),
(#212983,#212984),(#212985,#212986),(#212987,#212988),(#212989,#212990),
(#212991,#212992),(#212993,#212994),(#212995,#212996),(#212997,#212998),
(#212999,#213000),(#213001,#213002),(#213003,#213004),(#213005,#213006),
(#213007,#213008),(#213009,#213010),(#213011,#213012),(#213013,#213014),
(#213015,#213016),(#213017,#213018),(#213019,#213020),(#213021,#213022),
(#213023,#213024),(#213025,#213026),(#213027,#213028),(#213029,#213030),
(#213031,#213032),(#213033,#213034),(#213035,#213036),(#213037,#213038),
(#213039,#213040),(#213041,#213042),(#213043,#213044),(#213045,#213046),
(#213047,#213048),(#213049,#213050),(#213051,#213052),(#213053,#213054),
(#213055,#213056),(#213057,#213058),(#213059,#213060),(#213061,#213062),
(#213063,#213064),(#213065,#213066),(#213067,#213068),(#213069,#213070),
(#213071,#213072),(#213073,#213074),(#213075,#213076),(#213077,#213078),
(#213079,#213080),(#213081,#213082),(#213083,#213084),(#213085,#213086),
(#213087,#213088),(#213089,#213090),(#213091,#213092),(#213093,#213094),
(#213095,#213096),(#213097,#213098),(#213099,#213100),(#213101,#213102),
(#213103,#213104),(#213105,#213106),(#213107,#213108),(#213109,#213110),
(#213111,#213112),(#213113,#213114),(#213115,#213116),(#213117,#213118),
(#213119,#213120),(#213121,#213122),(#213123,#213124),(#213125,#213126),
(#213127,#213128),(#213129,#213130),(#213131,#213132),(#213133,#213134),
(#213135,#213136),(#213137,#213138)),.UNSPECIFIED.,.F.,.F.,.F.,(6,1,1,1,
1,1,1,1,1,1,1,1,1,1,1,1,1,1,1,1,1,1,1,1,1,1,1,1,1,1,1,1,1,1,1,1,1,1,1,1,
1,1,1,1,1,1,1,1,1,1,1,1,1,1,1,1,1,1,1,1,1,1,1,1,1,1,1,1,1,1,1,1,1,1,1,1,
1,1,1,1,1,1,1,1,1,1,1,1,1,1,1,1,1,1,1,1,1,1,1,1,1,1,1,1,1,1,1,1,1,1,1,1,
1,1,1,1,1,1,1,1,1,1,1,1,1,1,1,1,1,1,1,1,1,1,1,1,1,1,1,1,1,1,1,1,1,1,1,1,
1,1,1,1,1,1,1,1,1,1,1,1,1,1,1,1,1,1,1,1,1,1,1,1,1,1,1,1,1,1,1,1,1,1,1,1,
1,1,1,1,1,1,1,1,1,1,1,1,1,1,1,1,1,1,1,1,1,1,1,1,1,1,1,1,1,1,1,1,1,1,1,1,
1,1,1,1,1,1,1,1,1,1,1,1,1,1,1,1,1,1,1,1,1,1,1,1,1,1,1,1,1,1,1,1,1,1,1,1,
1,1,1,1,1,1,1,1,1,1,1,1,1,1,1,1,1,1,1,1,1,1,1,1,1,1,1,1,1,1,1,1,1,1,1,1,
1,1,1,1,1,1,1,1,1,1,1,1,1,1,1,1,1,1,1,1,1,1,1,1,1,1,1,1,1,1,1,1,1,1,1,1,
1,1,1,1,1,1,1,1,1,1,1,1,1,1,1,1,1,1,1,1,1,1,1,1,1,1,1,1,1,1,1,1,1,1,1,1,
1,1,1,1,1,1,1,1,1,1,1,1,1,1,1,1,1,1,1,1,1,1,1,1,1,1,1,1,1,1,1,1,1,1,1,1,
1,1,1,1,1,1,1,1,1,1,1,1,1,1,1,1,1,1,1,1,1,1,1,1,1,1,1,1,1,1,1,1,1,1,1,1,
1,1,1,1,1,1,1,1,1,1,1,1,1,1,1,1,1,1,1,1,1,1,1,1,1,1,1,1,1,1,1,6),(2,2),
(0.143172103,0.144954128,0.146788991,0.148623853,0.150458716,0.152293578,
0.15412844,0.155963303,0.157798165,0.159633028,0.16146789,0.163302752,0.165137615,
0.166972477,0.168807339,0.170642202,0.172477064,0.174311927,0.176146789,
0.177981651,0.179816514,0.181651376,0.183486239,0.185321101,0.187155963,
0.188990826,0.190825688,0.19266055,0.194495413,0.196330275,0.198165138,
0.2,0.201834862,0.203669725,0.205504587,0.20733945,0.209174312,0.211009174,
0.212844037,0.214678899,0.216513761,0.218348624,0.220183486,0.222018349,
0.223853211,0.225688073,0.227522936,0.229357798,0.231192661,0.233027523,
0.234862385,0.236697248,0.23853211,0.240366972,0.242201835,0.244036697,
0.24587156,0.247706422,0.249541284,0.251376147,0.253211009,0.255045872,
0.256880734,0.258715596,0.260550459,0.262385321,0.264220183,0.266055046,
0.267889908,0.269724771,0.271559633,0.273394495,0.275229358,0.27706422,
0.278899083,0.280733945,0.282568807,0.28440367,0.286238532,0.288073394,
0.289908257,0.291743119,0.293577982,0.295412844,0.297247706,0.299082569,
0.300917431,0.302752294,0.304587156,0.306422018,0.308256881,0.310091743,
0.311926606,0.313761468,0.31559633,0.317431193,0.319266055,0.321100917,
0.32293578,0.324770642,0.326605505,0.328440367,0.330275229,0.332110092,
0.333944954,0.335779817,0.337614679,0.339449541,0.341284404,0.343119266,
0.344954128,0.346788991,0.348623853,0.350458716,0.352293578,0.35412844,
0.355963303,0.357798165,0.359633028,0.36146789,0.363302752,0.365137615,
0.366972477,0.368807339,0.370642202,0.372477064,0.374311927,0.376146789,
0.377981651,0.379816514,0.381651376,0.383486239,0.385321101,0.387155963,
0.388990826,0.390825688,0.39266055,0.394495413,0.396330275,0.398165138,
0.4,0.401834862,0.403669725,0.405504587,0.40733945,0.409174312,0.411009174,
0.412844037,0.414678899,0.416513761,0.418348624,0.420183486,0.422018349,
0.423853211,0.425688073,0.427522936,0.429357798,0.431192661,0.433027523,
0.434862385,0.436697248,0.43853211,0.440366972,0.442201835,0.444036697,
0.44587156,0.447706422,0.449541284,0.451376147,0.453211009,0.455045872,
0.456880734,0.458715596,0.460550459,0.462385321,0.464220183,0.466055046,
0.467889908,0.469724771,0.471559633,0.473394495,0.475229358,0.47706422,
0.478899083,0.480733945,0.482568807,0.48440367,0.486238532,0.488073394,
0.489908257,0.491743119,0.493577982,0.495412844,0.497247706,0.499082569,
0.500917431,0.502752294,0.504587156,0.506422018,0.508256881,0.510091743,
0.511926606,0.513761468,0.51559633,0.517431193,0.519266055,0.521100917,
0.52293578,0.524770642,0.526605505,0.528440367,0.530275229,0.532110092,
0.533944954,0.535779817,0.537614679,0.539449541,0.541284404,0.543119266,
0.544954128,0.546788991,0.548623853,0.550458716,0.552293578,0.55412844,
0.555963303,0.557798165,0.559633028,0.56146789,0.563302752,0.565137615,
0.566972477,0.568807339,0.570642202,0.572477064,0.574311927,0.576146789,
0.577981651,0.579816514,0.581651376,0.583486239,0.585321101,0.587155963,
0.588990826,0.590825688,0.59266055,0.594495413,0.596330275,0.598165138,
0.6,0.601834862,0.603669725,0.605504587,0.60733945,0.609174312,0.611009174,
0.612844037,0.614678899,0.616513761,0.618348624,0.620183486,0.622018349,
0.623853211,0.625688073,0.627522936,0.629357798,0.631192661,0.633027523,
0.634862385,0.636697248,0.63853211,0.640366972,0.642201835,0.644036697,
0.64587156,0.647706422,0.649541284,0.651376147,0.653211009,0.655045872,
0.656880734,0.658715596,0.660550459,0.662385321,0.664220183,0.666055046,
0.667889908,0.669724771,0.671559633,0.673394495,0.675229358,0.67706422,
0.678899083,0.680733945,0.682568807,0.68440367,0.686238532,0.688073394,
0.689908257,0.691743119,0.693577982,0.695412844,0.697247706,0.699082569,
0.700917431,0.702752294,0.704587156,0.706422018,0.708256881,0.710091743,
0.711926606,0.713761468,0.71559633,0.717431193,0.719266055,0.721100917,
0.72293578,0.724770642,0.726605505,0.728440367,0.730275229,0.732110092,
0.733944954,0.735779817,0.737614679,0.739449541,0.741284404,0.743119266,
0.744954128,0.746788991,0.748623853,0.750458716,0.752293578,0.75412844,
0.755963303,0.757798165,0.759633028,0.76146789,0.763302752,0.765137615,
0.766972477,0.768807339,0.770642202,0.772477064,0.774311927,0.776146789,
0.777981651,0.779816514,0.781651376,0.783486239,0.785321101,0.787155963,
0.788990826,0.790825688,0.79266055,0.794495413,0.796330275,0.798165138,
0.8,0.801834862,0.803669725,0.805504587,0.80733945,0.809174312,0.811009174,
0.812844037,0.814678899,0.816513761,0.818348624,0.820183486,0.822018349,
0.823853211,0.825688073,0.827522936,0.829357798,0.831192661,0.833027523,
0.834862385,0.836697248,0.83853211,0.840366972,0.842201835,0.844036697,
0.84587156,0.847706422,0.849541284,0.851376147,0.853211009,0.855045872,
0.856880734,0.858715596,0.860550459,0.862385321,0.864220183,0.866055046,
0.867889908,0.869724771,0.871559633,0.873394495,0.875229358,0.87706422,
0.878899083,0.880733945,0.882568807,0.88440367,0.886238532,0.888073394,
0.889908257,0.891743119,0.893577982,0.895412844,0.897247706,0.899082569,
0.900917431,0.902752294,0.904587156,0.906422018,0.908256881,0.910091743,
0.911926606,0.913761468,0.91559633,0.917431193,0.919266055,0.921100917,
0.92293578,0.924770642,0.926605505,0.928440367,0.930275229,0.932110092,
0.933944954,0.935779817,0.937614679,0.939449541,0.941284404,0.943119266,
0.944954128,0.946788991,0.948623853,0.950458716,0.952293578,0.95412844,
0.955963303,0.957798165,0.959633028,0.96146789,0.963302752,0.965137615,
0.966972477,0.968807339,0.970642202,0.972477064,0.974311927,0.976146789,
0.977981651,0.979816514,0.981651376,0.983486239,0.985321101,0.987155963,
0.988990826,0.990825688,0.99266055,0.994495413,0.996330275,0.998165138,
1.),(0.,0.36),.UNSPECIFIED.);
#6251=B_SPLINE_SURFACE_WITH_KNOTS('',5,1,((#213789,#213790),(#213791,#213792),
(#213793,#213794),(#213795,#213796),(#213797,#213798),(#213799,#213800),
(#213801,#213802),(#213803,#213804),(#213805,#213806),(#213807,#213808),
(#213809,#213810),(#213811,#213812),(#213813,#213814),(#213815,#213816),
(#213817,#213818),(#213819,#213820),(#213821,#213822),(#213823,#213824),
(#213825,#213826),(#213827,#213828),(#213829,#213830),(#213831,#213832),
(#213833,#213834),(#213835,#213836),(#213837,#213838),(#213839,#213840),
(#213841,#213842),(#213843,#213844),(#213845,#213846),(#213847,#213848),
(#213849,#213850),(#213851,#213852),(#213853,#213854),(#213855,#213856),
(#213857,#213858),(#213859,#213860),(#213861,#213862),(#213863,#213864),
(#213865,#213866),(#213867,#213868),(#213869,#213870),(#213871,#213872),
(#213873,#213874),(#213875,#213876),(#213877,#213878),(#213879,#213880),
(#213881,#213882),(#213883,#213884),(#213885,#213886),(#213887,#213888),
(#213889,#213890),(#213891,#213892),(#213893,#213894),(#213895,#213896),
(#213897,#213898),(#213899,#213900),(#213901,#213902),(#213903,#213904),
(#213905,#213906),(#213907,#213908),(#213909,#213910),(#213911,#213912),
(#213913,#213914),(#213915,#213916),(#213917,#213918),(#213919,#213920),
(#213921,#213922),(#213923,#213924),(#213925,#213926),(#213927,#213928),
(#213929,#213930),(#213931,#213932),(#213933,#213934),(#213935,#213936),
(#213937,#213938),(#213939,#213940),(#213941,#213942),(#213943,#213944),
(#213945,#213946),(#213947,#213948),(#213949,#213950),(#213951,#213952),
(#213953,#213954),(#213955,#213956),(#213957,#213958),(#213959,#213960),
(#213961,#213962),(#213963,#213964),(#213965,#213966),(#213967,#213968),
(#213969,#213970),(#213971,#213972),(#213973,#213974),(#213975,#213976),
(#213977,#213978),(#213979,#213980),(#213981,#213982),(#213983,#213984),
(#213985,#213986),(#213987,#213988),(#213989,#213990),(#213991,#213992),
(#213993,#213994),(#213995,#213996),(#213997,#213998),(#213999,#214000),
(#214001,#214002),(#214003,#214004),(#214005,#214006),(#214007,#214008),
(#214009,#214010),(#214011,#214012),(#214013,#214014),(#214015,#214016),
(#214017,#214018),(#214019,#214020),(#214021,#214022),(#214023,#214024),
(#214025,#214026),(#214027,#214028),(#214029,#214030),(#214031,#214032),
(#214033,#214034),(#214035,#214036),(#214037,#214038),(#214039,#214040),
(#214041,#214042),(#214043,#214044),(#214045,#214046),(#214047,#214048),
(#214049,#214050),(#214051,#214052),(#214053,#214054),(#214055,#214056),
(#214057,#214058),(#214059,#214060),(#214061,#214062),(#214063,#214064),
(#214065,#214066),(#214067,#214068),(#214069,#214070),(#214071,#214072),
(#214073,#214074),(#214075,#214076),(#214077,#214078),(#214079,#214080),
(#214081,#214082),(#214083,#214084),(#214085,#214086),(#214087,#214088),
(#214089,#214090),(#214091,#214092),(#214093,#214094),(#214095,#214096),
(#214097,#214098),(#214099,#214100),(#214101,#214102),(#214103,#214104),
(#214105,#214106),(#214107,#214108),(#214109,#214110),(#214111,#214112),
(#214113,#214114),(#214115,#214116),(#214117,#214118),(#214119,#214120),
(#214121,#214122),(#214123,#214124),(#214125,#214126),(#214127,#214128),
(#214129,#214130),(#214131,#214132),(#214133,#214134),(#214135,#214136),
(#214137,#214138),(#214139,#214140),(#214141,#214142),(#214143,#214144),
(#214145,#214146),(#214147,#214148),(#214149,#214150),(#214151,#214152),
(#214153,#214154),(#214155,#214156),(#214157,#214158),(#214159,#214160),
(#214161,#214162),(#214163,#214164),(#214165,#214166),(#214167,#214168),
(#214169,#214170),(#214171,#214172),(#214173,#214174),(#214175,#214176),
(#214177,#214178),(#214179,#214180),(#214181,#214182),(#214183,#214184),
(#214185,#214186),(#214187,#214188),(#214189,#214190),(#214191,#214192),
(#214193,#214194),(#214195,#214196),(#214197,#214198),(#214199,#214200),
(#214201,#214202),(#214203,#214204),(#214205,#214206),(#214207,#214208),
(#214209,#214210),(#214211,#214212),(#214213,#214214),(#214215,#214216),
(#214217,#214218),(#214219,#214220),(#214221,#214222),(#214223,#214224),
(#214225,#214226),(#214227,#214228),(#214229,#214230),(#214231,#214232),
(#214233,#214234),(#214235,#214236),(#214237,#214238),(#214239,#214240),
(#214241,#214242),(#214243,#214244),(#214245,#214246),(#214247,#214248),
(#214249,#214250),(#214251,#214252),(#214253,#214254),(#214255,#214256),
(#214257,#214258),(#214259,#214260),(#214261,#214262),(#214263,#214264),
(#214265,#214266),(#214267,#214268),(#214269,#214270),(#214271,#214272),
(#214273,#214274),(#214275,#214276),(#214277,#214278),(#214279,#214280),
(#214281,#214282),(#214283,#214284),(#214285,#214286),(#214287,#214288),
(#214289,#214290),(#214291,#214292),(#214293,#214294),(#214295,#214296),
(#214297,#214298),(#214299,#214300),(#214301,#214302),(#214303,#214304),
(#214305,#214306),(#214307,#214308),(#214309,#214310),(#214311,#214312),
(#214313,#214314),(#214315,#214316),(#214317,#214318),(#214319,#214320),
(#214321,#214322),(#214323,#214324),(#214325,#214326),(#214327,#214328),
(#214329,#214330),(#214331,#214332),(#214333,#214334),(#214335,#214336),
(#214337,#214338),(#214339,#214340),(#214341,#214342),(#214343,#214344),
(#214345,#214346),(#214347,#214348),(#214349,#214350),(#214351,#214352),
(#214353,#214354),(#214355,#214356),(#214357,#214358),(#214359,#214360),
(#214361,#214362),(#214363,#214364),(#214365,#214366),(#214367,#214368),
(#214369,#214370),(#214371,#214372),(#214373,#214374),(#214375,#214376),
(#214377,#214378),(#214379,#214380),(#214381,#214382),(#214383,#214384),
(#214385,#214386),(#214387,#214388),(#214389,#214390),(#214391,#214392),
(#214393,#214394),(#214395,#214396),(#214397,#214398),(#214399,#214400),
(#214401,#214402),(#214403,#214404),(#214405,#214406),(#214407,#214408),
(#214409,#214410),(#214411,#214412),(#214413,#214414),(#214415,#214416),
(#214417,#214418),(#214419,#214420),(#214421,#214422),(#214423,#214424),
(#214425,#214426),(#214427,#214428),(#214429,#214430),(#214431,#214432),
(#214433,#214434),(#214435,#214436),(#214437,#214438),(#214439,#214440),
(#214441,#214442),(#214443,#214444),(#214445,#214446),(#214447,#214448),
(#214449,#214450),(#214451,#214452),(#214453,#214454),(#214455,#214456),
(#214457,#214458),(#214459,#214460),(#214461,#214462),(#214463,#214464),
(#214465,#214466),(#214467,#214468),(#214469,#214470),(#214471,#214472),
(#214473,#214474),(#214475,#214476),(#214477,#214478),(#214479,#214480),
(#214481,#214482),(#214483,#214484),(#214485,#214486),(#214487,#214488),
(#214489,#214490),(#214491,#214492),(#214493,#214494),(#214495,#214496),
(#214497,#214498),(#214499,#214500),(#214501,#214502),(#214503,#214504),
(#214505,#214506),(#214507,#214508),(#214509,#214510),(#214511,#214512),
(#214513,#214514),(#214515,#214516),(#214517,#214518),(#214519,#214520),
(#214521,#214522),(#214523,#214524),(#214525,#214526),(#214527,#214528),
(#214529,#214530),(#214531,#214532),(#214533,#214534),(#214535,#214536),
(#214537,#214538),(#214539,#214540),(#214541,#214542),(#214543,#214544),
(#214545,#214546),(#214547,#214548),(#214549,#214550),(#214551,#214552),
(#214553,#214554),(#214555,#214556),(#214557,#214558),(#214559,#214560),
(#214561,#214562),(#214563,#214564),(#214565,#214566),(#214567,#214568),
(#214569,#214570),(#214571,#214572),(#214573,#214574),(#214575,#214576),
(#214577,#214578),(#214579,#214580),(#214581,#214582),(#214583,#214584),
(#214585,#214586),(#214587,#214588),(#214589,#214590),(#214591,#214592),
(#214593,#214594),(#214595,#214596),(#214597,#214598),(#214599,#214600),
(#214601,#214602),(#214603,#214604),(#214605,#214606),(#214607,#214608),
(#214609,#214610),(#214611,#214612),(#214613,#214614),(#214615,#214616),
(#214617,#214618),(#214619,#214620),(#214621,#214622),(#214623,#214624),
(#214625,#214626),(#214627,#214628),(#214629,#214630),(#214631,#214632),
(#214633,#214634),(#214635,#214636),(#214637,#214638),(#214639,#214640),
(#214641,#214642),(#214643,#214644),(#214645,#214646),(#214647,#214648),
(#214649,#214650),(#214651,#214652),(#214653,#214654),(#214655,#214656),
(#214657,#214658),(#214659,#214660),(#214661,#214662),(#214663,#214664),
(#214665,#214666),(#214667,#214668),(#214669,#214670),(#214671,#214672),
(#214673,#214674),(#214675,#214676),(#214677,#214678),(#214679,#214680),
(#214681,#214682),(#214683,#214684),(#214685,#214686),(#214687,#214688),
(#214689,#214690),(#214691,#214692),(#214693,#214694),(#214695,#214696),
(#214697,#214698),(#214699,#214700),(#214701,#214702),(#214703,#214704),
(#214705,#214706),(#214707,#214708),(#214709,#214710),(#214711,#214712),
(#214713,#214714),(#214715,#214716),(#214717,#214718),(#214719,#214720),
(#214721,#214722),(#214723,#214724),(#214725,#214726),(#214727,#214728),
(#214729,#214730),(#214731,#214732)),.UNSPECIFIED.,.F.,.F.,.F.,(6,1,1,1,
1,1,1,1,1,1,1,1,1,1,1,1,1,1,1,1,1,1,1,1,1,1,1,1,1,1,1,1,1,1,1,1,1,1,1,1,
1,1,1,1,1,1,1,1,1,1,1,1,1,1,1,1,1,1,1,1,1,1,1,1,1,1,1,1,1,1,1,1,1,1,1,1,
1,1,1,1,1,1,1,1,1,1,1,1,1,1,1,1,1,1,1,1,1,1,1,1,1,1,1,1,1,1,1,1,1,1,1,1,
1,1,1,1,1,1,1,1,1,1,1,1,1,1,1,1,1,1,1,1,1,1,1,1,1,1,1,1,1,1,1,1,1,1,1,1,
1,1,1,1,1,1,1,1,1,1,1,1,1,1,1,1,1,1,1,1,1,1,1,1,1,1,1,1,1,1,1,1,1,1,1,1,
1,1,1,1,1,1,1,1,1,1,1,1,1,1,1,1,1,1,1,1,1,1,1,1,1,1,1,1,1,1,1,1,1,1,1,1,
1,1,1,1,1,1,1,1,1,1,1,1,1,1,1,1,1,1,1,1,1,1,1,1,1,1,1,1,1,1,1,1,1,1,1,1,
1,1,1,1,1,1,1,1,1,1,1,1,1,1,1,1,1,1,1,1,1,1,1,1,1,1,1,1,1,1,1,1,1,1,1,1,
1,1,1,1,1,1,1,1,1,1,1,1,1,1,1,1,1,1,1,1,1,1,1,1,1,1,1,1,1,1,1,1,1,1,1,1,
1,1,1,1,1,1,1,1,1,1,1,1,1,1,1,1,1,1,1,1,1,1,1,1,1,1,1,1,1,1,1,1,1,1,1,1,
1,1,1,1,1,1,1,1,1,1,1,1,1,1,1,1,1,1,1,1,1,1,1,1,1,1,1,1,1,1,1,1,1,1,1,1,
1,1,1,1,1,1,1,1,1,1,1,1,1,1,1,1,1,1,1,1,1,1,1,1,1,1,1,1,1,1,1,1,1,1,1,1,
1,1,1,1,1,1,1,1,1,1,1,1,1,1,1,1,1,1,1,1,1,1,1,1,1,1,1,1,1,1,1,6),(2,2),
(0.143172104,0.144954128,0.146788991,0.148623853,0.150458716,0.152293578,
0.15412844,0.155963303,0.157798165,0.159633028,0.16146789,0.163302752,0.165137615,
0.166972477,0.168807339,0.170642202,0.172477064,0.174311927,0.176146789,
0.177981651,0.179816514,0.181651376,0.183486239,0.185321101,0.187155963,
0.188990826,0.190825688,0.19266055,0.194495413,0.196330275,0.198165138,
0.2,0.201834862,0.203669725,0.205504587,0.20733945,0.209174312,0.211009174,
0.212844037,0.214678899,0.216513761,0.218348624,0.220183486,0.222018349,
0.223853211,0.225688073,0.227522936,0.229357798,0.231192661,0.233027523,
0.234862385,0.236697248,0.23853211,0.240366972,0.242201835,0.244036697,
0.24587156,0.247706422,0.249541284,0.251376147,0.253211009,0.255045872,
0.256880734,0.258715596,0.260550459,0.262385321,0.264220183,0.266055046,
0.267889908,0.269724771,0.271559633,0.273394495,0.275229358,0.27706422,
0.278899083,0.280733945,0.282568807,0.28440367,0.286238532,0.288073394,
0.289908257,0.291743119,0.293577982,0.295412844,0.297247706,0.299082569,
0.300917431,0.302752294,0.304587156,0.306422018,0.308256881,0.310091743,
0.311926606,0.313761468,0.31559633,0.317431193,0.319266055,0.321100917,
0.32293578,0.324770642,0.326605505,0.328440367,0.330275229,0.332110092,
0.333944954,0.335779817,0.337614679,0.339449541,0.341284404,0.343119266,
0.344954128,0.346788991,0.348623853,0.350458716,0.352293578,0.35412844,
0.355963303,0.357798165,0.359633028,0.36146789,0.363302752,0.365137615,
0.366972477,0.368807339,0.370642202,0.372477064,0.374311927,0.376146789,
0.377981651,0.379816514,0.381651376,0.383486239,0.385321101,0.387155963,
0.388990826,0.390825688,0.39266055,0.394495413,0.396330275,0.398165138,
0.4,0.401834862,0.403669725,0.405504587,0.40733945,0.409174312,0.411009174,
0.412844037,0.414678899,0.416513761,0.418348624,0.420183486,0.422018349,
0.423853211,0.425688073,0.427522936,0.429357798,0.431192661,0.433027523,
0.434862385,0.436697248,0.43853211,0.440366972,0.442201835,0.444036697,
0.44587156,0.447706422,0.449541284,0.451376147,0.453211009,0.455045872,
0.456880734,0.458715596,0.460550459,0.462385321,0.464220183,0.466055046,
0.467889908,0.469724771,0.471559633,0.473394495,0.475229358,0.47706422,
0.478899083,0.480733945,0.482568807,0.48440367,0.486238532,0.488073394,
0.489908257,0.491743119,0.493577982,0.495412844,0.497247706,0.499082569,
0.500917431,0.502752294,0.504587156,0.506422018,0.508256881,0.510091743,
0.511926606,0.513761468,0.51559633,0.517431193,0.519266055,0.521100917,
0.52293578,0.524770642,0.526605505,0.528440367,0.530275229,0.532110092,
0.533944954,0.535779817,0.537614679,0.539449541,0.541284404,0.543119266,
0.544954128,0.546788991,0.548623853,0.550458716,0.552293578,0.55412844,
0.555963303,0.557798165,0.559633028,0.56146789,0.563302752,0.565137615,
0.566972477,0.568807339,0.570642202,0.572477064,0.574311927,0.576146789,
0.577981651,0.579816514,0.581651376,0.583486239,0.585321101,0.587155963,
0.588990826,0.590825688,0.59266055,0.594495413,0.596330275,0.598165138,
0.6,0.601834862,0.603669725,0.605504587,0.60733945,0.609174312,0.611009174,
0.612844037,0.614678899,0.616513761,0.618348624,0.620183486,0.622018349,
0.623853211,0.625688073,0.627522936,0.629357798,0.631192661,0.633027523,
0.634862385,0.636697248,0.63853211,0.640366972,0.642201835,0.644036697,
0.64587156,0.647706422,0.649541284,0.651376147,0.653211009,0.655045872,
0.656880734,0.658715596,0.660550459,0.662385321,0.664220183,0.666055046,
0.667889908,0.669724771,0.671559633,0.673394495,0.675229358,0.67706422,
0.678899083,0.680733945,0.682568807,0.68440367,0.686238532,0.688073394,
0.689908257,0.691743119,0.693577982,0.695412844,0.697247706,0.699082569,
0.700917431,0.702752294,0.704587156,0.706422018,0.708256881,0.710091743,
0.711926606,0.713761468,0.71559633,0.717431193,0.719266055,0.721100917,
0.72293578,0.724770642,0.726605505,0.728440367,0.730275229,0.732110092,
0.733944954,0.735779817,0.737614679,0.739449541,0.741284404,0.743119266,
0.744954128,0.746788991,0.748623853,0.750458716,0.752293578,0.75412844,
0.755963303,0.757798165,0.759633028,0.76146789,0.763302752,0.765137615,
0.766972477,0.768807339,0.770642202,0.772477064,0.774311927,0.776146789,
0.777981651,0.779816514,0.781651376,0.783486239,0.785321101,0.787155963,
0.788990826,0.790825688,0.79266055,0.794495413,0.796330275,0.798165138,
0.8,0.801834862,0.803669725,0.805504587,0.80733945,0.809174312,0.811009174,
0.812844037,0.814678899,0.816513761,0.818348624,0.820183486,0.822018349,
0.823853211,0.825688073,0.827522936,0.829357798,0.831192661,0.833027523,
0.834862385,0.836697248,0.83853211,0.840366972,0.842201835,0.844036697,
0.84587156,0.847706422,0.849541284,0.851376147,0.853211009,0.855045872,
0.856880734,0.858715596,0.860550459,0.862385321,0.864220183,0.866055046,
0.867889908,0.869724771,0.871559633,0.873394495,0.875229358,0.87706422,
0.878899083,0.880733945,0.882568807,0.88440367,0.886238532,0.888073394,
0.889908257,0.891743119,0.893577982,0.895412844,0.897247706,0.899082569,
0.900917431,0.902752294,0.904587156,0.906422018,0.908256881,0.910091743,
0.911926606,0.913761468,0.91559633,0.917431193,0.919266055,0.921100917,
0.92293578,0.924770642,0.926605505,0.928440367,0.930275229,0.932110092,
0.933944954,0.935779817,0.937614679,0.939449541,0.941284404,0.943119266,
0.944954128,0.946788991,0.948623853,0.950458716,0.952293578,0.95412844,
0.955963303,0.957798165,0.959633028,0.96146789,0.963302752,0.965137615,
0.966972477,0.968807339,0.970642202,0.972477064,0.974311927,0.976146789,
0.977981651,0.979816514,0.981651376,0.983486239,0.985321101,0.987155963,
0.988990826,0.990825688,0.99266055,0.994495413,0.996330275,0.998165138,
1.),(0.,0.36),.UNSPECIFIED.);
#6252=B_SPLINE_SURFACE_WITH_KNOTS('',5,1,((#215365,#215366),(#215367,#215368),
(#215369,#215370),(#215371,#215372),(#215373,#215374),(#215375,#215376),
(#215377,#215378),(#215379,#215380),(#215381,#215382),(#215383,#215384),
(#215385,#215386),(#215387,#215388),(#215389,#215390),(#215391,#215392),
(#215393,#215394),(#215395,#215396),(#215397,#215398),(#215399,#215400),
(#215401,#215402),(#215403,#215404),(#215405,#215406),(#215407,#215408),
(#215409,#215410),(#215411,#215412),(#215413,#215414),(#215415,#215416),
(#215417,#215418),(#215419,#215420),(#215421,#215422),(#215423,#215424),
(#215425,#215426),(#215427,#215428),(#215429,#215430),(#215431,#215432),
(#215433,#215434),(#215435,#215436),(#215437,#215438),(#215439,#215440),
(#215441,#215442),(#215443,#215444),(#215445,#215446),(#215447,#215448),
(#215449,#215450),(#215451,#215452),(#215453,#215454),(#215455,#215456),
(#215457,#215458),(#215459,#215460),(#215461,#215462),(#215463,#215464),
(#215465,#215466),(#215467,#215468),(#215469,#215470),(#215471,#215472),
(#215473,#215474),(#215475,#215476),(#215477,#215478),(#215479,#215480),
(#215481,#215482),(#215483,#215484),(#215485,#215486),(#215487,#215488),
(#215489,#215490),(#215491,#215492),(#215493,#215494),(#215495,#215496),
(#215497,#215498),(#215499,#215500),(#215501,#215502),(#215503,#215504),
(#215505,#215506),(#215507,#215508),(#215509,#215510),(#215511,#215512),
(#215513,#215514),(#215515,#215516),(#215517,#215518),(#215519,#215520),
(#215521,#215522),(#215523,#215524),(#215525,#215526),(#215527,#215528),
(#215529,#215530),(#215531,#215532),(#215533,#215534),(#215535,#215536),
(#215537,#215538),(#215539,#215540),(#215541,#215542),(#215543,#215544),
(#215545,#215546),(#215547,#215548),(#215549,#215550),(#215551,#215552),
(#215553,#215554),(#215555,#215556),(#215557,#215558),(#215559,#215560),
(#215561,#215562),(#215563,#215564),(#215565,#215566),(#215567,#215568),
(#215569,#215570),(#215571,#215572),(#215573,#215574),(#215575,#215576),
(#215577,#215578),(#215579,#215580),(#215581,#215582),(#215583,#215584),
(#215585,#215586),(#215587,#215588),(#215589,#215590),(#215591,#215592),
(#215593,#215594),(#215595,#215596),(#215597,#215598),(#215599,#215600),
(#215601,#215602),(#215603,#215604),(#215605,#215606),(#215607,#215608),
(#215609,#215610),(#215611,#215612),(#215613,#215614),(#215615,#215616),
(#215617,#215618),(#215619,#215620),(#215621,#215622),(#215623,#215624),
(#215625,#215626),(#215627,#215628),(#215629,#215630),(#215631,#215632),
(#215633,#215634),(#215635,#215636),(#215637,#215638),(#215639,#215640),
(#215641,#215642),(#215643,#215644),(#215645,#215646),(#215647,#215648),
(#215649,#215650),(#215651,#215652),(#215653,#215654),(#215655,#215656),
(#215657,#215658),(#215659,#215660),(#215661,#215662),(#215663,#215664),
(#215665,#215666),(#215667,#215668),(#215669,#215670),(#215671,#215672),
(#215673,#215674),(#215675,#215676),(#215677,#215678),(#215679,#215680),
(#215681,#215682),(#215683,#215684),(#215685,#215686),(#215687,#215688),
(#215689,#215690),(#215691,#215692),(#215693,#215694),(#215695,#215696),
(#215697,#215698),(#215699,#215700),(#215701,#215702),(#215703,#215704),
(#215705,#215706),(#215707,#215708),(#215709,#215710),(#215711,#215712),
(#215713,#215714),(#215715,#215716),(#215717,#215718),(#215719,#215720),
(#215721,#215722),(#215723,#215724),(#215725,#215726),(#215727,#215728),
(#215729,#215730),(#215731,#215732),(#215733,#215734),(#215735,#215736),
(#215737,#215738),(#215739,#215740),(#215741,#215742),(#215743,#215744),
(#215745,#215746),(#215747,#215748),(#215749,#215750),(#215751,#215752),
(#215753,#215754),(#215755,#215756),(#215757,#215758),(#215759,#215760),
(#215761,#215762),(#215763,#215764),(#215765,#215766),(#215767,#215768),
(#215769,#215770),(#215771,#215772),(#215773,#215774),(#215775,#215776),
(#215777,#215778),(#215779,#215780),(#215781,#215782),(#215783,#215784),
(#215785,#215786),(#215787,#215788),(#215789,#215790),(#215791,#215792),
(#215793,#215794),(#215795,#215796),(#215797,#215798),(#215799,#215800),
(#215801,#215802),(#215803,#215804),(#215805,#215806),(#215807,#215808),
(#215809,#215810),(#215811,#215812),(#215813,#215814),(#215815,#215816),
(#215817,#215818),(#215819,#215820),(#215821,#215822),(#215823,#215824),
(#215825,#215826),(#215827,#215828),(#215829,#215830),(#215831,#215832),
(#215833,#215834),(#215835,#215836),(#215837,#215838),(#215839,#215840),
(#215841,#215842),(#215843,#215844),(#215845,#215846),(#215847,#215848),
(#215849,#215850),(#215851,#215852),(#215853,#215854),(#215855,#215856),
(#215857,#215858),(#215859,#215860),(#215861,#215862),(#215863,#215864),
(#215865,#215866),(#215867,#215868),(#215869,#215870),(#215871,#215872),
(#215873,#215874),(#215875,#215876),(#215877,#215878),(#215879,#215880),
(#215881,#215882),(#215883,#215884),(#215885,#215886),(#215887,#215888),
(#215889,#215890),(#215891,#215892),(#215893,#215894),(#215895,#215896),
(#215897,#215898),(#215899,#215900),(#215901,#215902),(#215903,#215904),
(#215905,#215906),(#215907,#215908),(#215909,#215910),(#215911,#215912),
(#215913,#215914),(#215915,#215916),(#215917,#215918),(#215919,#215920),
(#215921,#215922),(#215923,#215924),(#215925,#215926),(#215927,#215928),
(#215929,#215930),(#215931,#215932),(#215933,#215934),(#215935,#215936),
(#215937,#215938),(#215939,#215940),(#215941,#215942),(#215943,#215944),
(#215945,#215946),(#215947,#215948),(#215949,#215950),(#215951,#215952),
(#215953,#215954),(#215955,#215956),(#215957,#215958),(#215959,#215960),
(#215961,#215962),(#215963,#215964),(#215965,#215966),(#215967,#215968),
(#215969,#215970),(#215971,#215972),(#215973,#215974),(#215975,#215976),
(#215977,#215978),(#215979,#215980),(#215981,#215982),(#215983,#215984),
(#215985,#215986),(#215987,#215988),(#215989,#215990),(#215991,#215992),
(#215993,#215994),(#215995,#215996),(#215997,#215998),(#215999,#216000),
(#216001,#216002),(#216003,#216004),(#216005,#216006),(#216007,#216008),
(#216009,#216010),(#216011,#216012),(#216013,#216014),(#216015,#216016),
(#216017,#216018),(#216019,#216020),(#216021,#216022),(#216023,#216024),
(#216025,#216026),(#216027,#216028),(#216029,#216030),(#216031,#216032),
(#216033,#216034),(#216035,#216036),(#216037,#216038),(#216039,#216040),
(#216041,#216042),(#216043,#216044),(#216045,#216046),(#216047,#216048),
(#216049,#216050),(#216051,#216052),(#216053,#216054),(#216055,#216056),
(#216057,#216058),(#216059,#216060),(#216061,#216062),(#216063,#216064),
(#216065,#216066),(#216067,#216068),(#216069,#216070),(#216071,#216072),
(#216073,#216074),(#216075,#216076),(#216077,#216078),(#216079,#216080),
(#216081,#216082),(#216083,#216084),(#216085,#216086),(#216087,#216088),
(#216089,#216090),(#216091,#216092),(#216093,#216094),(#216095,#216096),
(#216097,#216098),(#216099,#216100),(#216101,#216102),(#216103,#216104),
(#216105,#216106),(#216107,#216108),(#216109,#216110),(#216111,#216112),
(#216113,#216114),(#216115,#216116),(#216117,#216118),(#216119,#216120),
(#216121,#216122),(#216123,#216124),(#216125,#216126),(#216127,#216128),
(#216129,#216130),(#216131,#216132),(#216133,#216134),(#216135,#216136),
(#216137,#216138),(#216139,#216140),(#216141,#216142),(#216143,#216144),
(#216145,#216146),(#216147,#216148),(#216149,#216150),(#216151,#216152),
(#216153,#216154),(#216155,#216156),(#216157,#216158),(#216159,#216160),
(#216161,#216162),(#216163,#216164),(#216165,#216166),(#216167,#216168),
(#216169,#216170),(#216171,#216172),(#216173,#216174),(#216175,#216176),
(#216177,#216178),(#216179,#216180),(#216181,#216182),(#216183,#216184),
(#216185,#216186),(#216187,#216188),(#216189,#216190),(#216191,#216192),
(#216193,#216194),(#216195,#216196),(#216197,#216198),(#216199,#216200),
(#216201,#216202),(#216203,#216204),(#216205,#216206),(#216207,#216208),
(#216209,#216210),(#216211,#216212),(#216213,#216214),(#216215,#216216),
(#216217,#216218),(#216219,#216220),(#216221,#216222),(#216223,#216224),
(#216225,#216226),(#216227,#216228),(#216229,#216230),(#216231,#216232),
(#216233,#216234),(#216235,#216236),(#216237,#216238),(#216239,#216240),
(#216241,#216242),(#216243,#216244),(#216245,#216246),(#216247,#216248),
(#216249,#216250),(#216251,#216252),(#216253,#216254),(#216255,#216256),
(#216257,#216258),(#216259,#216260),(#216261,#216262),(#216263,#216264),
(#216265,#216266),(#216267,#216268),(#216269,#216270),(#216271,#216272),
(#216273,#216274),(#216275,#216276),(#216277,#216278),(#216279,#216280),
(#216281,#216282),(#216283,#216284),(#216285,#216286),(#216287,#216288),
(#216289,#216290),(#216291,#216292),(#216293,#216294),(#216295,#216296),
(#216297,#216298),(#216299,#216300),(#216301,#216302),(#216303,#216304),
(#216305,#216306),(#216307,#216308)),.UNSPECIFIED.,.F.,.F.,.F.,(6,1,1,1,
1,1,1,1,1,1,1,1,1,1,1,1,1,1,1,1,1,1,1,1,1,1,1,1,1,1,1,1,1,1,1,1,1,1,1,1,
1,1,1,1,1,1,1,1,1,1,1,1,1,1,1,1,1,1,1,1,1,1,1,1,1,1,1,1,1,1,1,1,1,1,1,1,
1,1,1,1,1,1,1,1,1,1,1,1,1,1,1,1,1,1,1,1,1,1,1,1,1,1,1,1,1,1,1,1,1,1,1,1,
1,1,1,1,1,1,1,1,1,1,1,1,1,1,1,1,1,1,1,1,1,1,1,1,1,1,1,1,1,1,1,1,1,1,1,1,
1,1,1,1,1,1,1,1,1,1,1,1,1,1,1,1,1,1,1,1,1,1,1,1,1,1,1,1,1,1,1,1,1,1,1,1,
1,1,1,1,1,1,1,1,1,1,1,1,1,1,1,1,1,1,1,1,1,1,1,1,1,1,1,1,1,1,1,1,1,1,1,1,
1,1,1,1,1,1,1,1,1,1,1,1,1,1,1,1,1,1,1,1,1,1,1,1,1,1,1,1,1,1,1,1,1,1,1,1,
1,1,1,1,1,1,1,1,1,1,1,1,1,1,1,1,1,1,1,1,1,1,1,1,1,1,1,1,1,1,1,1,1,1,1,1,
1,1,1,1,1,1,1,1,1,1,1,1,1,1,1,1,1,1,1,1,1,1,1,1,1,1,1,1,1,1,1,1,1,1,1,1,
1,1,1,1,1,1,1,1,1,1,1,1,1,1,1,1,1,1,1,1,1,1,1,1,1,1,1,1,1,1,1,1,1,1,1,1,
1,1,1,1,1,1,1,1,1,1,1,1,1,1,1,1,1,1,1,1,1,1,1,1,1,1,1,1,1,1,1,1,1,1,1,1,
1,1,1,1,1,1,1,1,1,1,1,1,1,1,1,1,1,1,1,1,1,1,1,1,1,1,1,1,1,1,1,1,1,1,1,1,
1,1,1,1,1,1,1,1,1,1,1,1,1,1,1,1,1,1,1,1,1,1,1,1,1,1,1,1,1,1,1,6),(2,2),
(-1.,-0.998165138,-0.996330275,-0.994495413,-0.99266055,-0.990825688,-0.988990826,
-0.987155963,-0.985321101,-0.983486239,-0.981651376,-0.979816514,-0.977981651,
-0.976146789,-0.974311927,-0.972477064,-0.970642202,-0.968807339,-0.966972477,
-0.965137615,-0.963302752,-0.96146789,-0.959633028,-0.957798165,-0.955963303,
-0.95412844,-0.952293578,-0.950458716,-0.948623853,-0.946788991,-0.944954128,
-0.943119266,-0.941284404,-0.939449541,-0.937614679,-0.935779817,-0.933944954,
-0.932110092,-0.930275229,-0.928440367,-0.926605505,-0.924770642,-0.92293578,
-0.921100917,-0.919266055,-0.917431193,-0.91559633,-0.913761468,-0.911926606,
-0.910091743,-0.908256881,-0.906422018,-0.904587156,-0.902752294,-0.900917431,
-0.899082569,-0.897247706,-0.895412844,-0.893577982,-0.891743119,-0.889908257,
-0.888073394,-0.886238532,-0.88440367,-0.882568807,-0.880733945,-0.878899083,
-0.87706422,-0.875229358,-0.873394495,-0.871559633,-0.869724771,-0.867889908,
-0.866055046,-0.864220183,-0.862385321,-0.860550459,-0.858715596,-0.856880734,
-0.855045872,-0.853211009,-0.851376147,-0.849541284,-0.847706422,-0.84587156,
-0.844036697,-0.842201835,-0.840366972,-0.83853211,-0.836697248,-0.834862385,
-0.833027523,-0.831192661,-0.829357798,-0.827522936,-0.825688073,-0.823853211,
-0.822018349,-0.820183486,-0.818348624,-0.816513761,-0.814678899,-0.812844037,
-0.811009174,-0.809174312,-0.80733945,-0.805504587,-0.803669725,-0.801834862,
-0.8,-0.798165138,-0.796330275,-0.794495413,-0.79266055,-0.790825688,-0.788990826,
-0.787155963,-0.785321101,-0.783486239,-0.781651376,-0.779816514,-0.777981651,
-0.776146789,-0.774311927,-0.772477064,-0.770642202,-0.768807339,-0.766972477,
-0.765137615,-0.763302752,-0.76146789,-0.759633028,-0.757798165,-0.755963303,
-0.75412844,-0.752293578,-0.750458716,-0.748623853,-0.746788991,-0.744954128,
-0.743119266,-0.741284404,-0.739449541,-0.737614679,-0.735779817,-0.733944954,
-0.732110092,-0.730275229,-0.728440367,-0.726605505,-0.724770642,-0.72293578,
-0.721100917,-0.719266055,-0.717431193,-0.71559633,-0.713761468,-0.711926606,
-0.710091743,-0.708256881,-0.706422018,-0.704587156,-0.702752294,-0.700917431,
-0.699082569,-0.697247706,-0.695412844,-0.693577982,-0.691743119,-0.689908257,
-0.688073394,-0.686238532,-0.68440367,-0.682568807,-0.680733945,-0.678899083,
-0.67706422,-0.675229358,-0.673394495,-0.671559633,-0.669724771,-0.667889908,
-0.666055046,-0.664220183,-0.662385321,-0.660550459,-0.658715596,-0.656880734,
-0.655045872,-0.653211009,-0.651376147,-0.649541284,-0.647706422,-0.64587156,
-0.644036697,-0.642201835,-0.640366972,-0.63853211,-0.636697248,-0.634862385,
-0.633027523,-0.631192661,-0.629357798,-0.627522936,-0.625688073,-0.623853211,
-0.622018349,-0.620183486,-0.618348624,-0.616513761,-0.614678899,-0.612844037,
-0.611009174,-0.609174312,-0.60733945,-0.605504587,-0.603669725,-0.601834862,
-0.6,-0.598165138,-0.596330275,-0.594495413,-0.59266055,-0.590825688,-0.588990826,
-0.587155963,-0.585321101,-0.583486239,-0.581651376,-0.579816514,-0.577981651,
-0.576146789,-0.574311927,-0.572477064,-0.570642202,-0.568807339,-0.566972477,
-0.565137615,-0.563302752,-0.56146789,-0.559633028,-0.557798165,-0.555963303,
-0.55412844,-0.552293578,-0.550458716,-0.548623853,-0.546788991,-0.544954128,
-0.543119266,-0.541284404,-0.539449541,-0.537614679,-0.535779817,-0.533944954,
-0.532110092,-0.530275229,-0.528440367,-0.526605505,-0.524770642,-0.52293578,
-0.521100917,-0.519266055,-0.517431193,-0.51559633,-0.513761468,-0.511926606,
-0.510091743,-0.508256881,-0.506422018,-0.504587156,-0.502752294,-0.500917431,
-0.499082569,-0.497247706,-0.495412844,-0.493577982,-0.491743119,-0.489908257,
-0.488073394,-0.486238532,-0.48440367,-0.482568807,-0.480733945,-0.478899083,
-0.47706422,-0.475229358,-0.473394495,-0.471559633,-0.469724771,-0.467889908,
-0.466055046,-0.464220183,-0.462385321,-0.460550459,-0.458715596,-0.456880734,
-0.455045872,-0.453211009,-0.451376147,-0.449541284,-0.447706422,-0.44587156,
-0.444036697,-0.442201835,-0.440366972,-0.43853211,-0.436697248,-0.434862385,
-0.433027523,-0.431192661,-0.429357798,-0.427522936,-0.425688073,-0.423853211,
-0.422018349,-0.420183486,-0.418348624,-0.416513761,-0.414678899,-0.412844037,
-0.411009174,-0.409174312,-0.40733945,-0.405504587,-0.403669725,-0.401834862,
-0.4,-0.398165138,-0.396330275,-0.394495413,-0.39266055,-0.390825688,-0.388990826,
-0.387155963,-0.385321101,-0.383486239,-0.381651376,-0.379816514,-0.377981651,
-0.376146789,-0.374311927,-0.372477064,-0.370642202,-0.368807339,-0.366972477,
-0.365137615,-0.363302752,-0.36146789,-0.359633028,-0.357798165,-0.355963303,
-0.35412844,-0.352293578,-0.350458716,-0.348623853,-0.346788991,-0.344954128,
-0.343119266,-0.341284404,-0.339449541,-0.337614679,-0.335779817,-0.333944954,
-0.332110092,-0.330275229,-0.328440367,-0.326605505,-0.324770642,-0.32293578,
-0.321100917,-0.319266055,-0.317431193,-0.31559633,-0.313761468,-0.311926606,
-0.310091743,-0.308256881,-0.306422018,-0.304587156,-0.302752294,-0.300917431,
-0.299082569,-0.297247706,-0.295412844,-0.293577982,-0.291743119,-0.289908257,
-0.288073394,-0.286238532,-0.28440367,-0.282568807,-0.280733945,-0.278899083,
-0.27706422,-0.275229358,-0.273394495,-0.271559633,-0.269724771,-0.267889908,
-0.266055046,-0.264220183,-0.262385321,-0.260550459,-0.258715596,-0.256880734,
-0.255045872,-0.253211009,-0.251376147,-0.249541284,-0.247706422,-0.24587156,
-0.244036697,-0.242201835,-0.240366972,-0.23853211,-0.236697248,-0.234862385,
-0.233027523,-0.231192661,-0.229357798,-0.227522936,-0.225688073,-0.223853211,
-0.222018349,-0.220183486,-0.218348624,-0.216513761,-0.214678899,-0.212844037,
-0.211009174,-0.209174312,-0.20733945,-0.205504587,-0.203669725,-0.201834862,
-0.2,-0.198165138,-0.196330275,-0.194495413,-0.19266055,-0.190825688,-0.188990826,
-0.187155963,-0.185321101,-0.183486239,-0.181651376,-0.179816514,-0.177981651,
-0.176146789,-0.174311927,-0.172477064,-0.170642202,-0.168807339,-0.166972477,
-0.165137615,-0.163302752,-0.16146789,-0.159633028,-0.157798165,-0.155963303,
-0.15412844,-0.152293578,-0.150458716,-0.148623853,-0.146788991,-0.144954128,
-0.143172104),(0.,0.36),.UNSPECIFIED.);
#6253=B_SPLINE_SURFACE_WITH_KNOTS('',5,1,((#216956,#216957),(#216958,#216959),
(#216960,#216961),(#216962,#216963),(#216964,#216965),(#216966,#216967),
(#216968,#216969),(#216970,#216971),(#216972,#216973),(#216974,#216975),
(#216976,#216977),(#216978,#216979),(#216980,#216981),(#216982,#216983),
(#216984,#216985),(#216986,#216987),(#216988,#216989),(#216990,#216991),
(#216992,#216993),(#216994,#216995),(#216996,#216997),(#216998,#216999),
(#217000,#217001),(#217002,#217003),(#217004,#217005),(#217006,#217007),
(#217008,#217009),(#217010,#217011),(#217012,#217013),(#217014,#217015),
(#217016,#217017),(#217018,#217019),(#217020,#217021),(#217022,#217023),
(#217024,#217025),(#217026,#217027),(#217028,#217029),(#217030,#217031),
(#217032,#217033),(#217034,#217035),(#217036,#217037),(#217038,#217039),
(#217040,#217041),(#217042,#217043),(#217044,#217045),(#217046,#217047),
(#217048,#217049),(#217050,#217051),(#217052,#217053),(#217054,#217055),
(#217056,#217057),(#217058,#217059),(#217060,#217061),(#217062,#217063),
(#217064,#217065),(#217066,#217067),(#217068,#217069),(#217070,#217071),
(#217072,#217073),(#217074,#217075),(#217076,#217077),(#217078,#217079),
(#217080,#217081),(#217082,#217083),(#217084,#217085),(#217086,#217087),
(#217088,#217089),(#217090,#217091),(#217092,#217093),(#217094,#217095),
(#217096,#217097),(#217098,#217099),(#217100,#217101),(#217102,#217103),
(#217104,#217105),(#217106,#217107),(#217108,#217109),(#217110,#217111),
(#217112,#217113),(#217114,#217115),(#217116,#217117),(#217118,#217119),
(#217120,#217121),(#217122,#217123),(#217124,#217125),(#217126,#217127),
(#217128,#217129),(#217130,#217131),(#217132,#217133),(#217134,#217135),
(#217136,#217137),(#217138,#217139),(#217140,#217141),(#217142,#217143),
(#217144,#217145),(#217146,#217147),(#217148,#217149),(#217150,#217151),
(#217152,#217153),(#217154,#217155),(#217156,#217157),(#217158,#217159),
(#217160,#217161),(#217162,#217163),(#217164,#217165),(#217166,#217167),
(#217168,#217169),(#217170,#217171),(#217172,#217173),(#217174,#217175),
(#217176,#217177),(#217178,#217179),(#217180,#217181),(#217182,#217183),
(#217184,#217185),(#217186,#217187),(#217188,#217189),(#217190,#217191),
(#217192,#217193),(#217194,#217195),(#217196,#217197),(#217198,#217199),
(#217200,#217201),(#217202,#217203),(#217204,#217205),(#217206,#217207),
(#217208,#217209),(#217210,#217211),(#217212,#217213),(#217214,#217215),
(#217216,#217217),(#217218,#217219),(#217220,#217221),(#217222,#217223),
(#217224,#217225),(#217226,#217227),(#217228,#217229),(#217230,#217231),
(#217232,#217233),(#217234,#217235),(#217236,#217237),(#217238,#217239),
(#217240,#217241),(#217242,#217243),(#217244,#217245),(#217246,#217247),
(#217248,#217249),(#217250,#217251),(#217252,#217253),(#217254,#217255),
(#217256,#217257),(#217258,#217259),(#217260,#217261),(#217262,#217263),
(#217264,#217265),(#217266,#217267),(#217268,#217269),(#217270,#217271),
(#217272,#217273),(#217274,#217275),(#217276,#217277),(#217278,#217279),
(#217280,#217281),(#217282,#217283),(#217284,#217285),(#217286,#217287),
(#217288,#217289),(#217290,#217291),(#217292,#217293),(#217294,#217295),
(#217296,#217297),(#217298,#217299),(#217300,#217301),(#217302,#217303),
(#217304,#217305),(#217306,#217307),(#217308,#217309),(#217310,#217311),
(#217312,#217313),(#217314,#217315),(#217316,#217317),(#217318,#217319),
(#217320,#217321),(#217322,#217323),(#217324,#217325),(#217326,#217327),
(#217328,#217329),(#217330,#217331),(#217332,#217333),(#217334,#217335),
(#217336,#217337),(#217338,#217339),(#217340,#217341),(#217342,#217343),
(#217344,#217345),(#217346,#217347),(#217348,#217349),(#217350,#217351),
(#217352,#217353),(#217354,#217355),(#217356,#217357),(#217358,#217359),
(#217360,#217361),(#217362,#217363),(#217364,#217365),(#217366,#217367),
(#217368,#217369),(#217370,#217371),(#217372,#217373),(#217374,#217375),
(#217376,#217377),(#217378,#217379),(#217380,#217381),(#217382,#217383),
(#217384,#217385),(#217386,#217387),(#217388,#217389),(#217390,#217391),
(#217392,#217393),(#217394,#217395),(#217396,#217397),(#217398,#217399),
(#217400,#217401),(#217402,#217403),(#217404,#217405),(#217406,#217407),
(#217408,#217409),(#217410,#217411),(#217412,#217413),(#217414,#217415),
(#217416,#217417),(#217418,#217419),(#217420,#217421),(#217422,#217423),
(#217424,#217425),(#217426,#217427),(#217428,#217429),(#217430,#217431),
(#217432,#217433),(#217434,#217435),(#217436,#217437),(#217438,#217439),
(#217440,#217441),(#217442,#217443),(#217444,#217445),(#217446,#217447),
(#217448,#217449),(#217450,#217451),(#217452,#217453),(#217454,#217455),
(#217456,#217457),(#217458,#217459),(#217460,#217461),(#217462,#217463),
(#217464,#217465),(#217466,#217467),(#217468,#217469),(#217470,#217471),
(#217472,#217473),(#217474,#217475),(#217476,#217477),(#217478,#217479),
(#217480,#217481),(#217482,#217483),(#217484,#217485),(#217486,#217487),
(#217488,#217489),(#217490,#217491),(#217492,#217493),(#217494,#217495),
(#217496,#217497),(#217498,#217499),(#217500,#217501),(#217502,#217503),
(#217504,#217505),(#217506,#217507),(#217508,#217509),(#217510,#217511),
(#217512,#217513),(#217514,#217515),(#217516,#217517),(#217518,#217519),
(#217520,#217521),(#217522,#217523),(#217524,#217525),(#217526,#217527),
(#217528,#217529),(#217530,#217531),(#217532,#217533),(#217534,#217535),
(#217536,#217537),(#217538,#217539),(#217540,#217541),(#217542,#217543),
(#217544,#217545),(#217546,#217547),(#217548,#217549),(#217550,#217551),
(#217552,#217553),(#217554,#217555),(#217556,#217557),(#217558,#217559),
(#217560,#217561),(#217562,#217563),(#217564,#217565),(#217566,#217567),
(#217568,#217569),(#217570,#217571),(#217572,#217573),(#217574,#217575),
(#217576,#217577),(#217578,#217579),(#217580,#217581),(#217582,#217583),
(#217584,#217585),(#217586,#217587),(#217588,#217589),(#217590,#217591),
(#217592,#217593),(#217594,#217595),(#217596,#217597),(#217598,#217599),
(#217600,#217601),(#217602,#217603),(#217604,#217605),(#217606,#217607),
(#217608,#217609),(#217610,#217611),(#217612,#217613),(#217614,#217615),
(#217616,#217617),(#217618,#217619),(#217620,#217621),(#217622,#217623),
(#217624,#217625),(#217626,#217627),(#217628,#217629),(#217630,#217631),
(#217632,#217633),(#217634,#217635),(#217636,#217637),(#217638,#217639),
(#217640,#217641),(#217642,#217643),(#217644,#217645),(#217646,#217647),
(#217648,#217649),(#217650,#217651),(#217652,#217653),(#217654,#217655),
(#217656,#217657),(#217658,#217659),(#217660,#217661),(#217662,#217663),
(#217664,#217665),(#217666,#217667),(#217668,#217669),(#217670,#217671),
(#217672,#217673),(#217674,#217675),(#217676,#217677),(#217678,#217679),
(#217680,#217681),(#217682,#217683),(#217684,#217685),(#217686,#217687),
(#217688,#217689),(#217690,#217691),(#217692,#217693),(#217694,#217695),
(#217696,#217697),(#217698,#217699),(#217700,#217701),(#217702,#217703),
(#217704,#217705),(#217706,#217707),(#217708,#217709),(#217710,#217711),
(#217712,#217713),(#217714,#217715),(#217716,#217717),(#217718,#217719),
(#217720,#217721),(#217722,#217723),(#217724,#217725),(#217726,#217727),
(#217728,#217729),(#217730,#217731),(#217732,#217733),(#217734,#217735),
(#217736,#217737),(#217738,#217739),(#217740,#217741),(#217742,#217743),
(#217744,#217745),(#217746,#217747),(#217748,#217749),(#217750,#217751),
(#217752,#217753),(#217754,#217755),(#217756,#217757),(#217758,#217759),
(#217760,#217761),(#217762,#217763),(#217764,#217765),(#217766,#217767),
(#217768,#217769),(#217770,#217771),(#217772,#217773),(#217774,#217775),
(#217776,#217777),(#217778,#217779),(#217780,#217781),(#217782,#217783),
(#217784,#217785),(#217786,#217787),(#217788,#217789),(#217790,#217791),
(#217792,#217793),(#217794,#217795),(#217796,#217797),(#217798,#217799),
(#217800,#217801),(#217802,#217803),(#217804,#217805),(#217806,#217807),
(#217808,#217809),(#217810,#217811),(#217812,#217813),(#217814,#217815),
(#217816,#217817),(#217818,#217819),(#217820,#217821),(#217822,#217823),
(#217824,#217825),(#217826,#217827),(#217828,#217829),(#217830,#217831),
(#217832,#217833),(#217834,#217835),(#217836,#217837),(#217838,#217839),
(#217840,#217841),(#217842,#217843),(#217844,#217845),(#217846,#217847),
(#217848,#217849),(#217850,#217851),(#217852,#217853),(#217854,#217855),
(#217856,#217857),(#217858,#217859),(#217860,#217861),(#217862,#217863),
(#217864,#217865),(#217866,#217867),(#217868,#217869),(#217870,#217871),
(#217872,#217873),(#217874,#217875),(#217876,#217877),(#217878,#217879),
(#217880,#217881),(#217882,#217883),(#217884,#217885),(#217886,#217887),
(#217888,#217889),(#217890,#217891),(#217892,#217893),(#217894,#217895),
(#217896,#217897),(#217898,#217899)),.UNSPECIFIED.,.F.,.F.,.F.,(6,1,1,1,
1,1,1,1,1,1,1,1,1,1,1,1,1,1,1,1,1,1,1,1,1,1,1,1,1,1,1,1,1,1,1,1,1,1,1,1,
1,1,1,1,1,1,1,1,1,1,1,1,1,1,1,1,1,1,1,1,1,1,1,1,1,1,1,1,1,1,1,1,1,1,1,1,
1,1,1,1,1,1,1,1,1,1,1,1,1,1,1,1,1,1,1,1,1,1,1,1,1,1,1,1,1,1,1,1,1,1,1,1,
1,1,1,1,1,1,1,1,1,1,1,1,1,1,1,1,1,1,1,1,1,1,1,1,1,1,1,1,1,1,1,1,1,1,1,1,
1,1,1,1,1,1,1,1,1,1,1,1,1,1,1,1,1,1,1,1,1,1,1,1,1,1,1,1,1,1,1,1,1,1,1,1,
1,1,1,1,1,1,1,1,1,1,1,1,1,1,1,1,1,1,1,1,1,1,1,1,1,1,1,1,1,1,1,1,1,1,1,1,
1,1,1,1,1,1,1,1,1,1,1,1,1,1,1,1,1,1,1,1,1,1,1,1,1,1,1,1,1,1,1,1,1,1,1,1,
1,1,1,1,1,1,1,1,1,1,1,1,1,1,1,1,1,1,1,1,1,1,1,1,1,1,1,1,1,1,1,1,1,1,1,1,
1,1,1,1,1,1,1,1,1,1,1,1,1,1,1,1,1,1,1,1,1,1,1,1,1,1,1,1,1,1,1,1,1,1,1,1,
1,1,1,1,1,1,1,1,1,1,1,1,1,1,1,1,1,1,1,1,1,1,1,1,1,1,1,1,1,1,1,1,1,1,1,1,
1,1,1,1,1,1,1,1,1,1,1,1,1,1,1,1,1,1,1,1,1,1,1,1,1,1,1,1,1,1,1,1,1,1,1,1,
1,1,1,1,1,1,1,1,1,1,1,1,1,1,1,1,1,1,1,1,1,1,1,1,1,1,1,1,1,1,1,1,1,1,1,1,
1,1,1,1,1,1,1,1,1,1,1,1,1,1,1,1,1,1,1,1,1,1,1,1,1,1,1,1,1,1,1,6),(2,2),
(-1.,-0.998165138,-0.996330275,-0.994495413,-0.99266055,-0.990825688,-0.988990826,
-0.987155963,-0.985321101,-0.983486239,-0.981651376,-0.979816514,-0.977981651,
-0.976146789,-0.974311927,-0.972477064,-0.970642202,-0.968807339,-0.966972477,
-0.965137615,-0.963302752,-0.96146789,-0.959633028,-0.957798165,-0.955963303,
-0.95412844,-0.952293578,-0.950458716,-0.948623853,-0.946788991,-0.944954128,
-0.943119266,-0.941284404,-0.939449541,-0.937614679,-0.935779817,-0.933944954,
-0.932110092,-0.930275229,-0.928440367,-0.926605505,-0.924770642,-0.92293578,
-0.921100917,-0.919266055,-0.917431193,-0.91559633,-0.913761468,-0.911926606,
-0.910091743,-0.908256881,-0.906422018,-0.904587156,-0.902752294,-0.900917431,
-0.899082569,-0.897247706,-0.895412844,-0.893577982,-0.891743119,-0.889908257,
-0.888073394,-0.886238532,-0.88440367,-0.882568807,-0.880733945,-0.878899083,
-0.87706422,-0.875229358,-0.873394495,-0.871559633,-0.869724771,-0.867889908,
-0.866055046,-0.864220183,-0.862385321,-0.860550459,-0.858715596,-0.856880734,
-0.855045872,-0.853211009,-0.851376147,-0.849541284,-0.847706422,-0.84587156,
-0.844036697,-0.842201835,-0.840366972,-0.83853211,-0.836697248,-0.834862385,
-0.833027523,-0.831192661,-0.829357798,-0.827522936,-0.825688073,-0.823853211,
-0.822018349,-0.820183486,-0.818348624,-0.816513761,-0.814678899,-0.812844037,
-0.811009174,-0.809174312,-0.80733945,-0.805504587,-0.803669725,-0.801834862,
-0.8,-0.798165138,-0.796330275,-0.794495413,-0.79266055,-0.790825688,-0.788990826,
-0.787155963,-0.785321101,-0.783486239,-0.781651376,-0.779816514,-0.777981651,
-0.776146789,-0.774311927,-0.772477064,-0.770642202,-0.768807339,-0.766972477,
-0.765137615,-0.763302752,-0.76146789,-0.759633028,-0.757798165,-0.755963303,
-0.75412844,-0.752293578,-0.750458716,-0.748623853,-0.746788991,-0.744954128,
-0.743119266,-0.741284404,-0.739449541,-0.737614679,-0.735779817,-0.733944954,
-0.732110092,-0.730275229,-0.728440367,-0.726605505,-0.724770642,-0.72293578,
-0.721100917,-0.719266055,-0.717431193,-0.71559633,-0.713761468,-0.711926606,
-0.710091743,-0.708256881,-0.706422018,-0.704587156,-0.702752294,-0.700917431,
-0.699082569,-0.697247706,-0.695412844,-0.693577982,-0.691743119,-0.689908257,
-0.688073394,-0.686238532,-0.68440367,-0.682568807,-0.680733945,-0.678899083,
-0.67706422,-0.675229358,-0.673394495,-0.671559633,-0.669724771,-0.667889908,
-0.666055046,-0.664220183,-0.662385321,-0.660550459,-0.658715596,-0.656880734,
-0.655045872,-0.653211009,-0.651376147,-0.649541284,-0.647706422,-0.64587156,
-0.644036697,-0.642201835,-0.640366972,-0.63853211,-0.636697248,-0.634862385,
-0.633027523,-0.631192661,-0.629357798,-0.627522936,-0.625688073,-0.623853211,
-0.622018349,-0.620183486,-0.618348624,-0.616513761,-0.614678899,-0.612844037,
-0.611009174,-0.609174312,-0.60733945,-0.605504587,-0.603669725,-0.601834862,
-0.6,-0.598165138,-0.596330275,-0.594495413,-0.59266055,-0.590825688,-0.588990826,
-0.587155963,-0.585321101,-0.583486239,-0.581651376,-0.579816514,-0.577981651,
-0.576146789,-0.574311927,-0.572477064,-0.570642202,-0.568807339,-0.566972477,
-0.565137615,-0.563302752,-0.56146789,-0.559633028,-0.557798165,-0.555963303,
-0.55412844,-0.552293578,-0.550458716,-0.548623853,-0.546788991,-0.544954128,
-0.543119266,-0.541284404,-0.539449541,-0.537614679,-0.535779817,-0.533944954,
-0.532110092,-0.530275229,-0.528440367,-0.526605505,-0.524770642,-0.52293578,
-0.521100917,-0.519266055,-0.517431193,-0.51559633,-0.513761468,-0.511926606,
-0.510091743,-0.508256881,-0.506422018,-0.504587156,-0.502752294,-0.500917431,
-0.499082569,-0.497247706,-0.495412844,-0.493577982,-0.491743119,-0.489908257,
-0.488073394,-0.486238532,-0.48440367,-0.482568807,-0.480733945,-0.478899083,
-0.47706422,-0.475229358,-0.473394495,-0.471559633,-0.469724771,-0.467889908,
-0.466055046,-0.464220183,-0.462385321,-0.460550459,-0.458715596,-0.456880734,
-0.455045872,-0.453211009,-0.451376147,-0.449541284,-0.447706422,-0.44587156,
-0.444036697,-0.442201835,-0.440366972,-0.43853211,-0.436697248,-0.434862385,
-0.433027523,-0.431192661,-0.429357798,-0.427522936,-0.425688073,-0.423853211,
-0.422018349,-0.420183486,-0.418348624,-0.416513761,-0.414678899,-0.412844037,
-0.411009174,-0.409174312,-0.40733945,-0.405504587,-0.403669725,-0.401834862,
-0.4,-0.398165138,-0.396330275,-0.394495413,-0.39266055,-0.390825688,-0.388990826,
-0.387155963,-0.385321101,-0.383486239,-0.381651376,-0.379816514,-0.377981651,
-0.376146789,-0.374311927,-0.372477064,-0.370642202,-0.368807339,-0.366972477,
-0.365137615,-0.363302752,-0.36146789,-0.359633028,-0.357798165,-0.355963303,
-0.35412844,-0.352293578,-0.350458716,-0.348623853,-0.346788991,-0.344954128,
-0.343119266,-0.341284404,-0.339449541,-0.337614679,-0.335779817,-0.333944954,
-0.332110092,-0.330275229,-0.328440367,-0.326605505,-0.324770642,-0.32293578,
-0.321100917,-0.319266055,-0.317431193,-0.31559633,-0.313761468,-0.311926606,
-0.310091743,-0.308256881,-0.306422018,-0.304587156,-0.302752294,-0.300917431,
-0.299082569,-0.297247706,-0.295412844,-0.293577982,-0.291743119,-0.289908257,
-0.288073394,-0.286238532,-0.28440367,-0.282568807,-0.280733945,-0.278899083,
-0.27706422,-0.275229358,-0.273394495,-0.271559633,-0.269724771,-0.267889908,
-0.266055046,-0.264220183,-0.262385321,-0.260550459,-0.258715596,-0.256880734,
-0.255045872,-0.253211009,-0.251376147,-0.249541284,-0.247706422,-0.24587156,
-0.244036697,-0.242201835,-0.240366972,-0.23853211,-0.236697248,-0.234862385,
-0.233027523,-0.231192661,-0.229357798,-0.227522936,-0.225688073,-0.223853211,
-0.222018349,-0.220183486,-0.218348624,-0.216513761,-0.214678899,-0.212844037,
-0.211009174,-0.209174312,-0.20733945,-0.205504587,-0.203669725,-0.201834862,
-0.2,-0.198165138,-0.196330275,-0.194495413,-0.19266055,-0.190825688,-0.188990826,
-0.187155963,-0.185321101,-0.183486239,-0.181651376,-0.179816514,-0.177981651,
-0.176146789,-0.174311927,-0.172477064,-0.170642202,-0.168807339,-0.166972477,
-0.165137615,-0.163302752,-0.16146789,-0.159633028,-0.157798165,-0.155963303,
-0.15412844,-0.152293578,-0.150458716,-0.148623853,-0.146788991,-0.144954128,
-0.143172103),(0.,0.36),.UNSPECIFIED.);
#6254=B_SPLINE_SURFACE_WITH_KNOTS('',5,1,((#218845,#218846),(#218847,#218848),
(#218849,#218850),(#218851,#218852),(#218853,#218854),(#218855,#218856),
(#218857,#218858),(#218859,#218860),(#218861,#218862),(#218863,#218864),
(#218865,#218866),(#218867,#218868),(#218869,#218870),(#218871,#218872),
(#218873,#218874),(#218875,#218876),(#218877,#218878),(#218879,#218880),
(#218881,#218882),(#218883,#218884),(#218885,#218886),(#218887,#218888),
(#218889,#218890),(#218891,#218892),(#218893,#218894),(#218895,#218896),
(#218897,#218898),(#218899,#218900),(#218901,#218902),(#218903,#218904),
(#218905,#218906),(#218907,#218908),(#218909,#218910),(#218911,#218912),
(#218913,#218914),(#218915,#218916),(#218917,#218918),(#218919,#218920),
(#218921,#218922),(#218923,#218924),(#218925,#218926),(#218927,#218928),
(#218929,#218930),(#218931,#218932),(#218933,#218934),(#218935,#218936),
(#218937,#218938),(#218939,#218940),(#218941,#218942),(#218943,#218944),
(#218945,#218946),(#218947,#218948),(#218949,#218950),(#218951,#218952),
(#218953,#218954),(#218955,#218956),(#218957,#218958),(#218959,#218960),
(#218961,#218962),(#218963,#218964),(#218965,#218966),(#218967,#218968),
(#218969,#218970),(#218971,#218972),(#218973,#218974),(#218975,#218976),
(#218977,#218978),(#218979,#218980),(#218981,#218982),(#218983,#218984),
(#218985,#218986),(#218987,#218988),(#218989,#218990),(#218991,#218992),
(#218993,#218994),(#218995,#218996),(#218997,#218998),(#218999,#219000),
(#219001,#219002),(#219003,#219004),(#219005,#219006),(#219007,#219008),
(#219009,#219010),(#219011,#219012),(#219013,#219014),(#219015,#219016),
(#219017,#219018),(#219019,#219020),(#219021,#219022),(#219023,#219024),
(#219025,#219026),(#219027,#219028),(#219029,#219030),(#219031,#219032),
(#219033,#219034),(#219035,#219036),(#219037,#219038),(#219039,#219040),
(#219041,#219042),(#219043,#219044),(#219045,#219046),(#219047,#219048),
(#219049,#219050),(#219051,#219052),(#219053,#219054),(#219055,#219056),
(#219057,#219058),(#219059,#219060),(#219061,#219062),(#219063,#219064),
(#219065,#219066),(#219067,#219068),(#219069,#219070),(#219071,#219072),
(#219073,#219074),(#219075,#219076),(#219077,#219078),(#219079,#219080),
(#219081,#219082),(#219083,#219084),(#219085,#219086),(#219087,#219088),
(#219089,#219090),(#219091,#219092),(#219093,#219094),(#219095,#219096),
(#219097,#219098),(#219099,#219100),(#219101,#219102),(#219103,#219104),
(#219105,#219106),(#219107,#219108),(#219109,#219110),(#219111,#219112),
(#219113,#219114),(#219115,#219116),(#219117,#219118),(#219119,#219120),
(#219121,#219122),(#219123,#219124),(#219125,#219126),(#219127,#219128),
(#219129,#219130),(#219131,#219132),(#219133,#219134),(#219135,#219136),
(#219137,#219138),(#219139,#219140),(#219141,#219142),(#219143,#219144),
(#219145,#219146),(#219147,#219148),(#219149,#219150),(#219151,#219152),
(#219153,#219154),(#219155,#219156),(#219157,#219158),(#219159,#219160),
(#219161,#219162),(#219163,#219164),(#219165,#219166),(#219167,#219168),
(#219169,#219170),(#219171,#219172),(#219173,#219174),(#219175,#219176),
(#219177,#219178),(#219179,#219180),(#219181,#219182),(#219183,#219184),
(#219185,#219186),(#219187,#219188),(#219189,#219190),(#219191,#219192),
(#219193,#219194),(#219195,#219196),(#219197,#219198),(#219199,#219200),
(#219201,#219202),(#219203,#219204),(#219205,#219206),(#219207,#219208),
(#219209,#219210),(#219211,#219212),(#219213,#219214),(#219215,#219216),
(#219217,#219218),(#219219,#219220),(#219221,#219222),(#219223,#219224),
(#219225,#219226),(#219227,#219228),(#219229,#219230),(#219231,#219232),
(#219233,#219234),(#219235,#219236),(#219237,#219238),(#219239,#219240),
(#219241,#219242),(#219243,#219244),(#219245,#219246),(#219247,#219248),
(#219249,#219250),(#219251,#219252),(#219253,#219254),(#219255,#219256),
(#219257,#219258),(#219259,#219260),(#219261,#219262),(#219263,#219264),
(#219265,#219266),(#219267,#219268),(#219269,#219270),(#219271,#219272),
(#219273,#219274),(#219275,#219276),(#219277,#219278),(#219279,#219280),
(#219281,#219282),(#219283,#219284),(#219285,#219286),(#219287,#219288),
(#219289,#219290),(#219291,#219292),(#219293,#219294),(#219295,#219296),
(#219297,#219298),(#219299,#219300),(#219301,#219302),(#219303,#219304),
(#219305,#219306),(#219307,#219308),(#219309,#219310),(#219311,#219312),
(#219313,#219314),(#219315,#219316),(#219317,#219318),(#219319,#219320),
(#219321,#219322),(#219323,#219324),(#219325,#219326),(#219327,#219328),
(#219329,#219330),(#219331,#219332),(#219333,#219334),(#219335,#219336),
(#219337,#219338),(#219339,#219340),(#219341,#219342),(#219343,#219344),
(#219345,#219346),(#219347,#219348),(#219349,#219350),(#219351,#219352),
(#219353,#219354),(#219355,#219356),(#219357,#219358),(#219359,#219360),
(#219361,#219362),(#219363,#219364),(#219365,#219366),(#219367,#219368),
(#219369,#219370),(#219371,#219372),(#219373,#219374),(#219375,#219376),
(#219377,#219378),(#219379,#219380),(#219381,#219382),(#219383,#219384),
(#219385,#219386),(#219387,#219388),(#219389,#219390),(#219391,#219392),
(#219393,#219394),(#219395,#219396),(#219397,#219398),(#219399,#219400),
(#219401,#219402),(#219403,#219404),(#219405,#219406),(#219407,#219408),
(#219409,#219410),(#219411,#219412),(#219413,#219414),(#219415,#219416),
(#219417,#219418),(#219419,#219420),(#219421,#219422),(#219423,#219424),
(#219425,#219426),(#219427,#219428),(#219429,#219430),(#219431,#219432),
(#219433,#219434),(#219435,#219436),(#219437,#219438),(#219439,#219440),
(#219441,#219442),(#219443,#219444),(#219445,#219446),(#219447,#219448),
(#219449,#219450),(#219451,#219452),(#219453,#219454),(#219455,#219456),
(#219457,#219458),(#219459,#219460),(#219461,#219462),(#219463,#219464),
(#219465,#219466),(#219467,#219468),(#219469,#219470),(#219471,#219472),
(#219473,#219474),(#219475,#219476),(#219477,#219478),(#219479,#219480),
(#219481,#219482),(#219483,#219484),(#219485,#219486),(#219487,#219488),
(#219489,#219490),(#219491,#219492),(#219493,#219494),(#219495,#219496),
(#219497,#219498),(#219499,#219500),(#219501,#219502),(#219503,#219504),
(#219505,#219506),(#219507,#219508),(#219509,#219510),(#219511,#219512),
(#219513,#219514),(#219515,#219516),(#219517,#219518),(#219519,#219520),
(#219521,#219522),(#219523,#219524),(#219525,#219526),(#219527,#219528),
(#219529,#219530),(#219531,#219532),(#219533,#219534),(#219535,#219536),
(#219537,#219538),(#219539,#219540),(#219541,#219542),(#219543,#219544),
(#219545,#219546),(#219547,#219548),(#219549,#219550),(#219551,#219552),
(#219553,#219554),(#219555,#219556),(#219557,#219558),(#219559,#219560),
(#219561,#219562),(#219563,#219564),(#219565,#219566),(#219567,#219568),
(#219569,#219570),(#219571,#219572),(#219573,#219574),(#219575,#219576),
(#219577,#219578),(#219579,#219580),(#219581,#219582),(#219583,#219584),
(#219585,#219586),(#219587,#219588),(#219589,#219590),(#219591,#219592),
(#219593,#219594),(#219595,#219596),(#219597,#219598),(#219599,#219600),
(#219601,#219602),(#219603,#219604),(#219605,#219606),(#219607,#219608),
(#219609,#219610),(#219611,#219612),(#219613,#219614),(#219615,#219616),
(#219617,#219618),(#219619,#219620),(#219621,#219622),(#219623,#219624),
(#219625,#219626),(#219627,#219628),(#219629,#219630),(#219631,#219632),
(#219633,#219634),(#219635,#219636),(#219637,#219638),(#219639,#219640),
(#219641,#219642),(#219643,#219644),(#219645,#219646),(#219647,#219648),
(#219649,#219650),(#219651,#219652),(#219653,#219654),(#219655,#219656),
(#219657,#219658),(#219659,#219660),(#219661,#219662),(#219663,#219664),
(#219665,#219666),(#219667,#219668),(#219669,#219670),(#219671,#219672),
(#219673,#219674),(#219675,#219676),(#219677,#219678),(#219679,#219680),
(#219681,#219682),(#219683,#219684),(#219685,#219686),(#219687,#219688),
(#219689,#219690),(#219691,#219692),(#219693,#219694),(#219695,#219696),
(#219697,#219698),(#219699,#219700),(#219701,#219702),(#219703,#219704),
(#219705,#219706),(#219707,#219708),(#219709,#219710),(#219711,#219712),
(#219713,#219714),(#219715,#219716),(#219717,#219718),(#219719,#219720),
(#219721,#219722),(#219723,#219724),(#219725,#219726),(#219727,#219728),
(#219729,#219730),(#219731,#219732),(#219733,#219734),(#219735,#219736),
(#219737,#219738),(#219739,#219740),(#219741,#219742),(#219743,#219744),
(#219745,#219746),(#219747,#219748),(#219749,#219750),(#219751,#219752),
(#219753,#219754),(#219755,#219756),(#219757,#219758),(#219759,#219760),
(#219761,#219762),(#219763,#219764),(#219765,#219766),(#219767,#219768),
(#219769,#219770),(#219771,#219772),(#219773,#219774),(#219775,#219776),
(#219777,#219778),(#219779,#219780),(#219781,#219782),(#219783,#219784),
(#219785,#219786),(#219787,#219788)),.UNSPECIFIED.,.F.,.F.,.F.,(6,1,1,1,
1,1,1,1,1,1,1,1,1,1,1,1,1,1,1,1,1,1,1,1,1,1,1,1,1,1,1,1,1,1,1,1,1,1,1,1,
1,1,1,1,1,1,1,1,1,1,1,1,1,1,1,1,1,1,1,1,1,1,1,1,1,1,1,1,1,1,1,1,1,1,1,1,
1,1,1,1,1,1,1,1,1,1,1,1,1,1,1,1,1,1,1,1,1,1,1,1,1,1,1,1,1,1,1,1,1,1,1,1,
1,1,1,1,1,1,1,1,1,1,1,1,1,1,1,1,1,1,1,1,1,1,1,1,1,1,1,1,1,1,1,1,1,1,1,1,
1,1,1,1,1,1,1,1,1,1,1,1,1,1,1,1,1,1,1,1,1,1,1,1,1,1,1,1,1,1,1,1,1,1,1,1,
1,1,1,1,1,1,1,1,1,1,1,1,1,1,1,1,1,1,1,1,1,1,1,1,1,1,1,1,1,1,1,1,1,1,1,1,
1,1,1,1,1,1,1,1,1,1,1,1,1,1,1,1,1,1,1,1,1,1,1,1,1,1,1,1,1,1,1,1,1,1,1,1,
1,1,1,1,1,1,1,1,1,1,1,1,1,1,1,1,1,1,1,1,1,1,1,1,1,1,1,1,1,1,1,1,1,1,1,1,
1,1,1,1,1,1,1,1,1,1,1,1,1,1,1,1,1,1,1,1,1,1,1,1,1,1,1,1,1,1,1,1,1,1,1,1,
1,1,1,1,1,1,1,1,1,1,1,1,1,1,1,1,1,1,1,1,1,1,1,1,1,1,1,1,1,1,1,1,1,1,1,1,
1,1,1,1,1,1,1,1,1,1,1,1,1,1,1,1,1,1,1,1,1,1,1,1,1,1,1,1,1,1,1,1,1,1,1,1,
1,1,1,1,1,1,1,1,1,1,1,1,1,1,1,1,1,1,1,1,1,1,1,1,1,1,1,1,1,1,1,1,1,1,1,1,
1,1,1,1,1,1,1,1,1,1,1,1,1,1,1,1,1,1,1,1,1,1,1,1,1,1,1,1,1,1,1,6),(2,2),
(0.143172104,0.144954128,0.146788991,0.148623853,0.150458716,0.152293578,
0.15412844,0.155963303,0.157798165,0.159633028,0.16146789,0.163302752,0.165137615,
0.166972477,0.168807339,0.170642202,0.172477064,0.174311927,0.176146789,
0.177981651,0.179816514,0.181651376,0.183486239,0.185321101,0.187155963,
0.188990826,0.190825688,0.19266055,0.194495413,0.196330275,0.198165138,
0.2,0.201834862,0.203669725,0.205504587,0.20733945,0.209174312,0.211009174,
0.212844037,0.214678899,0.216513761,0.218348624,0.220183486,0.222018349,
0.223853211,0.225688073,0.227522936,0.229357798,0.231192661,0.233027523,
0.234862385,0.236697248,0.23853211,0.240366972,0.242201835,0.244036697,
0.24587156,0.247706422,0.249541284,0.251376147,0.253211009,0.255045872,
0.256880734,0.258715596,0.260550459,0.262385321,0.264220183,0.266055046,
0.267889908,0.269724771,0.271559633,0.273394495,0.275229358,0.27706422,
0.278899083,0.280733945,0.282568807,0.28440367,0.286238532,0.288073394,
0.289908257,0.291743119,0.293577982,0.295412844,0.297247706,0.299082569,
0.300917431,0.302752294,0.304587156,0.306422018,0.308256881,0.310091743,
0.311926606,0.313761468,0.31559633,0.317431193,0.319266055,0.321100917,
0.32293578,0.324770642,0.326605505,0.328440367,0.330275229,0.332110092,
0.333944954,0.335779817,0.337614679,0.339449541,0.341284404,0.343119266,
0.344954128,0.346788991,0.348623853,0.350458716,0.352293578,0.35412844,
0.355963303,0.357798165,0.359633028,0.36146789,0.363302752,0.365137615,
0.366972477,0.368807339,0.370642202,0.372477064,0.374311927,0.376146789,
0.377981651,0.379816514,0.381651376,0.383486239,0.385321101,0.387155963,
0.388990826,0.390825688,0.39266055,0.394495413,0.396330275,0.398165138,
0.4,0.401834862,0.403669725,0.405504587,0.40733945,0.409174312,0.411009174,
0.412844037,0.414678899,0.416513761,0.418348624,0.420183486,0.422018349,
0.423853211,0.425688073,0.427522936,0.429357798,0.431192661,0.433027523,
0.434862385,0.436697248,0.43853211,0.440366972,0.442201835,0.444036697,
0.44587156,0.447706422,0.449541284,0.451376147,0.453211009,0.455045872,
0.456880734,0.458715596,0.460550459,0.462385321,0.464220183,0.466055046,
0.467889908,0.469724771,0.471559633,0.473394495,0.475229358,0.47706422,
0.478899083,0.480733945,0.482568807,0.48440367,0.486238532,0.488073394,
0.489908257,0.491743119,0.493577982,0.495412844,0.497247706,0.499082569,
0.500917431,0.502752294,0.504587156,0.506422018,0.508256881,0.510091743,
0.511926606,0.513761468,0.51559633,0.517431193,0.519266055,0.521100917,
0.52293578,0.524770642,0.526605505,0.528440367,0.530275229,0.532110092,
0.533944954,0.535779817,0.537614679,0.539449541,0.541284404,0.543119266,
0.544954128,0.546788991,0.548623853,0.550458716,0.552293578,0.55412844,
0.555963303,0.557798165,0.559633028,0.56146789,0.563302752,0.565137615,
0.566972477,0.568807339,0.570642202,0.572477064,0.574311927,0.576146789,
0.577981651,0.579816514,0.581651376,0.583486239,0.585321101,0.587155963,
0.588990826,0.590825688,0.59266055,0.594495413,0.596330275,0.598165138,
0.6,0.601834862,0.603669725,0.605504587,0.60733945,0.609174312,0.611009174,
0.612844037,0.614678899,0.616513761,0.618348624,0.620183486,0.622018349,
0.623853211,0.625688073,0.627522936,0.629357798,0.631192661,0.633027523,
0.634862385,0.636697248,0.63853211,0.640366972,0.642201835,0.644036697,
0.64587156,0.647706422,0.649541284,0.651376147,0.653211009,0.655045872,
0.656880734,0.658715596,0.660550459,0.662385321,0.664220183,0.666055046,
0.667889908,0.669724771,0.671559633,0.673394495,0.675229358,0.67706422,
0.678899083,0.680733945,0.682568807,0.68440367,0.686238532,0.688073394,
0.689908257,0.691743119,0.693577982,0.695412844,0.697247706,0.699082569,
0.700917431,0.702752294,0.704587156,0.706422018,0.708256881,0.710091743,
0.711926606,0.713761468,0.71559633,0.717431193,0.719266055,0.721100917,
0.72293578,0.724770642,0.726605505,0.728440367,0.730275229,0.732110092,
0.733944954,0.735779817,0.737614679,0.739449541,0.741284404,0.743119266,
0.744954128,0.746788991,0.748623853,0.750458716,0.752293578,0.75412844,
0.755963303,0.757798165,0.759633028,0.76146789,0.763302752,0.765137615,
0.766972477,0.768807339,0.770642202,0.772477064,0.774311927,0.776146789,
0.777981651,0.779816514,0.781651376,0.783486239,0.785321101,0.787155963,
0.788990826,0.790825688,0.79266055,0.794495413,0.796330275,0.798165138,
0.8,0.801834862,0.803669725,0.805504587,0.80733945,0.809174312,0.811009174,
0.812844037,0.814678899,0.816513761,0.818348624,0.820183486,0.822018349,
0.823853211,0.825688073,0.827522936,0.829357798,0.831192661,0.833027523,
0.834862385,0.836697248,0.83853211,0.840366972,0.842201835,0.844036697,
0.84587156,0.847706422,0.849541284,0.851376147,0.853211009,0.855045872,
0.856880734,0.858715596,0.860550459,0.862385321,0.864220183,0.866055046,
0.867889908,0.869724771,0.871559633,0.873394495,0.875229358,0.87706422,
0.878899083,0.880733945,0.882568807,0.88440367,0.886238532,0.888073394,
0.889908257,0.891743119,0.893577982,0.895412844,0.897247706,0.899082569,
0.900917431,0.902752294,0.904587156,0.906422018,0.908256881,0.910091743,
0.911926606,0.913761468,0.91559633,0.917431193,0.919266055,0.921100917,
0.92293578,0.924770642,0.926605505,0.928440367,0.930275229,0.932110092,
0.933944954,0.935779817,0.937614679,0.939449541,0.941284404,0.943119266,
0.944954128,0.946788991,0.948623853,0.950458716,0.952293578,0.95412844,
0.955963303,0.957798165,0.959633028,0.96146789,0.963302752,0.965137615,
0.966972477,0.968807339,0.970642202,0.972477064,0.974311927,0.976146789,
0.977981651,0.979816514,0.981651376,0.983486239,0.985321101,0.987155963,
0.988990826,0.990825688,0.99266055,0.994495413,0.996330275,0.998165138,
1.),(0.,0.36),.UNSPECIFIED.);
#6255=B_SPLINE_SURFACE_WITH_KNOTS('',5,1,((#220421,#220422),(#220423,#220424),
(#220425,#220426),(#220427,#220428),(#220429,#220430),(#220431,#220432),
(#220433,#220434),(#220435,#220436),(#220437,#220438),(#220439,#220440),
(#220441,#220442),(#220443,#220444),(#220445,#220446),(#220447,#220448),
(#220449,#220450),(#220451,#220452),(#220453,#220454),(#220455,#220456),
(#220457,#220458),(#220459,#220460),(#220461,#220462),(#220463,#220464),
(#220465,#220466),(#220467,#220468),(#220469,#220470),(#220471,#220472),
(#220473,#220474),(#220475,#220476),(#220477,#220478),(#220479,#220480),
(#220481,#220482),(#220483,#220484),(#220485,#220486),(#220487,#220488),
(#220489,#220490),(#220491,#220492),(#220493,#220494),(#220495,#220496),
(#220497,#220498),(#220499,#220500),(#220501,#220502),(#220503,#220504),
(#220505,#220506),(#220507,#220508),(#220509,#220510),(#220511,#220512),
(#220513,#220514),(#220515,#220516),(#220517,#220518),(#220519,#220520),
(#220521,#220522),(#220523,#220524),(#220525,#220526),(#220527,#220528),
(#220529,#220530),(#220531,#220532),(#220533,#220534),(#220535,#220536),
(#220537,#220538),(#220539,#220540),(#220541,#220542),(#220543,#220544),
(#220545,#220546),(#220547,#220548),(#220549,#220550),(#220551,#220552),
(#220553,#220554),(#220555,#220556),(#220557,#220558),(#220559,#220560),
(#220561,#220562),(#220563,#220564),(#220565,#220566),(#220567,#220568),
(#220569,#220570),(#220571,#220572),(#220573,#220574),(#220575,#220576),
(#220577,#220578),(#220579,#220580),(#220581,#220582),(#220583,#220584),
(#220585,#220586),(#220587,#220588),(#220589,#220590),(#220591,#220592),
(#220593,#220594),(#220595,#220596),(#220597,#220598),(#220599,#220600),
(#220601,#220602),(#220603,#220604),(#220605,#220606),(#220607,#220608),
(#220609,#220610),(#220611,#220612),(#220613,#220614),(#220615,#220616),
(#220617,#220618),(#220619,#220620),(#220621,#220622),(#220623,#220624),
(#220625,#220626),(#220627,#220628),(#220629,#220630),(#220631,#220632),
(#220633,#220634),(#220635,#220636),(#220637,#220638),(#220639,#220640),
(#220641,#220642),(#220643,#220644),(#220645,#220646),(#220647,#220648),
(#220649,#220650),(#220651,#220652),(#220653,#220654),(#220655,#220656),
(#220657,#220658),(#220659,#220660),(#220661,#220662),(#220663,#220664),
(#220665,#220666),(#220667,#220668),(#220669,#220670),(#220671,#220672),
(#220673,#220674),(#220675,#220676),(#220677,#220678),(#220679,#220680),
(#220681,#220682),(#220683,#220684),(#220685,#220686),(#220687,#220688),
(#220689,#220690),(#220691,#220692),(#220693,#220694),(#220695,#220696),
(#220697,#220698),(#220699,#220700),(#220701,#220702),(#220703,#220704),
(#220705,#220706),(#220707,#220708),(#220709,#220710),(#220711,#220712),
(#220713,#220714),(#220715,#220716),(#220717,#220718),(#220719,#220720),
(#220721,#220722),(#220723,#220724),(#220725,#220726),(#220727,#220728),
(#220729,#220730),(#220731,#220732),(#220733,#220734),(#220735,#220736),
(#220737,#220738),(#220739,#220740),(#220741,#220742),(#220743,#220744),
(#220745,#220746),(#220747,#220748),(#220749,#220750),(#220751,#220752),
(#220753,#220754),(#220755,#220756),(#220757,#220758),(#220759,#220760),
(#220761,#220762),(#220763,#220764),(#220765,#220766),(#220767,#220768),
(#220769,#220770),(#220771,#220772),(#220773,#220774),(#220775,#220776),
(#220777,#220778),(#220779,#220780),(#220781,#220782),(#220783,#220784),
(#220785,#220786),(#220787,#220788),(#220789,#220790),(#220791,#220792),
(#220793,#220794),(#220795,#220796),(#220797,#220798),(#220799,#220800),
(#220801,#220802),(#220803,#220804),(#220805,#220806),(#220807,#220808),
(#220809,#220810),(#220811,#220812),(#220813,#220814),(#220815,#220816),
(#220817,#220818),(#220819,#220820),(#220821,#220822),(#220823,#220824),
(#220825,#220826),(#220827,#220828),(#220829,#220830),(#220831,#220832),
(#220833,#220834),(#220835,#220836),(#220837,#220838),(#220839,#220840),
(#220841,#220842),(#220843,#220844),(#220845,#220846),(#220847,#220848),
(#220849,#220850),(#220851,#220852),(#220853,#220854),(#220855,#220856),
(#220857,#220858),(#220859,#220860),(#220861,#220862),(#220863,#220864),
(#220865,#220866),(#220867,#220868),(#220869,#220870),(#220871,#220872),
(#220873,#220874),(#220875,#220876),(#220877,#220878),(#220879,#220880),
(#220881,#220882),(#220883,#220884),(#220885,#220886),(#220887,#220888),
(#220889,#220890),(#220891,#220892),(#220893,#220894),(#220895,#220896),
(#220897,#220898),(#220899,#220900),(#220901,#220902),(#220903,#220904),
(#220905,#220906),(#220907,#220908),(#220909,#220910),(#220911,#220912),
(#220913,#220914),(#220915,#220916),(#220917,#220918),(#220919,#220920),
(#220921,#220922),(#220923,#220924),(#220925,#220926),(#220927,#220928),
(#220929,#220930),(#220931,#220932),(#220933,#220934),(#220935,#220936),
(#220937,#220938),(#220939,#220940),(#220941,#220942),(#220943,#220944),
(#220945,#220946),(#220947,#220948),(#220949,#220950),(#220951,#220952),
(#220953,#220954),(#220955,#220956),(#220957,#220958),(#220959,#220960),
(#220961,#220962),(#220963,#220964),(#220965,#220966),(#220967,#220968),
(#220969,#220970),(#220971,#220972),(#220973,#220974),(#220975,#220976),
(#220977,#220978),(#220979,#220980),(#220981,#220982),(#220983,#220984),
(#220985,#220986),(#220987,#220988),(#220989,#220990),(#220991,#220992),
(#220993,#220994),(#220995,#220996),(#220997,#220998),(#220999,#221000),
(#221001,#221002),(#221003,#221004),(#221005,#221006),(#221007,#221008),
(#221009,#221010),(#221011,#221012),(#221013,#221014),(#221015,#221016),
(#221017,#221018),(#221019,#221020),(#221021,#221022),(#221023,#221024),
(#221025,#221026),(#221027,#221028),(#221029,#221030),(#221031,#221032),
(#221033,#221034),(#221035,#221036),(#221037,#221038),(#221039,#221040),
(#221041,#221042),(#221043,#221044),(#221045,#221046),(#221047,#221048),
(#221049,#221050),(#221051,#221052),(#221053,#221054),(#221055,#221056),
(#221057,#221058),(#221059,#221060),(#221061,#221062),(#221063,#221064),
(#221065,#221066),(#221067,#221068),(#221069,#221070),(#221071,#221072),
(#221073,#221074),(#221075,#221076),(#221077,#221078),(#221079,#221080),
(#221081,#221082),(#221083,#221084),(#221085,#221086),(#221087,#221088),
(#221089,#221090),(#221091,#221092),(#221093,#221094),(#221095,#221096),
(#221097,#221098),(#221099,#221100),(#221101,#221102),(#221103,#221104),
(#221105,#221106),(#221107,#221108),(#221109,#221110),(#221111,#221112),
(#221113,#221114),(#221115,#221116),(#221117,#221118),(#221119,#221120),
(#221121,#221122),(#221123,#221124),(#221125,#221126),(#221127,#221128),
(#221129,#221130),(#221131,#221132),(#221133,#221134),(#221135,#221136),
(#221137,#221138),(#221139,#221140),(#221141,#221142),(#221143,#221144),
(#221145,#221146),(#221147,#221148),(#221149,#221150),(#221151,#221152),
(#221153,#221154),(#221155,#221156),(#221157,#221158),(#221159,#221160),
(#221161,#221162),(#221163,#221164),(#221165,#221166),(#221167,#221168),
(#221169,#221170),(#221171,#221172),(#221173,#221174),(#221175,#221176),
(#221177,#221178),(#221179,#221180),(#221181,#221182),(#221183,#221184),
(#221185,#221186),(#221187,#221188),(#221189,#221190),(#221191,#221192),
(#221193,#221194),(#221195,#221196),(#221197,#221198),(#221199,#221200),
(#221201,#221202),(#221203,#221204),(#221205,#221206),(#221207,#221208),
(#221209,#221210),(#221211,#221212),(#221213,#221214),(#221215,#221216),
(#221217,#221218),(#221219,#221220),(#221221,#221222),(#221223,#221224),
(#221225,#221226),(#221227,#221228),(#221229,#221230),(#221231,#221232),
(#221233,#221234),(#221235,#221236),(#221237,#221238),(#221239,#221240),
(#221241,#221242),(#221243,#221244),(#221245,#221246),(#221247,#221248),
(#221249,#221250),(#221251,#221252),(#221253,#221254),(#221255,#221256),
(#221257,#221258),(#221259,#221260),(#221261,#221262),(#221263,#221264),
(#221265,#221266),(#221267,#221268),(#221269,#221270),(#221271,#221272),
(#221273,#221274),(#221275,#221276),(#221277,#221278),(#221279,#221280),
(#221281,#221282),(#221283,#221284),(#221285,#221286),(#221287,#221288),
(#221289,#221290),(#221291,#221292),(#221293,#221294),(#221295,#221296),
(#221297,#221298),(#221299,#221300),(#221301,#221302),(#221303,#221304),
(#221305,#221306),(#221307,#221308),(#221309,#221310),(#221311,#221312),
(#221313,#221314),(#221315,#221316),(#221317,#221318),(#221319,#221320),
(#221321,#221322),(#221323,#221324),(#221325,#221326),(#221327,#221328),
(#221329,#221330),(#221331,#221332),(#221333,#221334),(#221335,#221336),
(#221337,#221338),(#221339,#221340),(#221341,#221342),(#221343,#221344),
(#221345,#221346),(#221347,#221348),(#221349,#221350),(#221351,#221352),
(#221353,#221354),(#221355,#221356),(#221357,#221358),(#221359,#221360),
(#221361,#221362),(#221363,#221364)),.UNSPECIFIED.,.F.,.F.,.F.,(6,1,1,1,
1,1,1,1,1,1,1,1,1,1,1,1,1,1,1,1,1,1,1,1,1,1,1,1,1,1,1,1,1,1,1,1,1,1,1,1,
1,1,1,1,1,1,1,1,1,1,1,1,1,1,1,1,1,1,1,1,1,1,1,1,1,1,1,1,1,1,1,1,1,1,1,1,
1,1,1,1,1,1,1,1,1,1,1,1,1,1,1,1,1,1,1,1,1,1,1,1,1,1,1,1,1,1,1,1,1,1,1,1,
1,1,1,1,1,1,1,1,1,1,1,1,1,1,1,1,1,1,1,1,1,1,1,1,1,1,1,1,1,1,1,1,1,1,1,1,
1,1,1,1,1,1,1,1,1,1,1,1,1,1,1,1,1,1,1,1,1,1,1,1,1,1,1,1,1,1,1,1,1,1,1,1,
1,1,1,1,1,1,1,1,1,1,1,1,1,1,1,1,1,1,1,1,1,1,1,1,1,1,1,1,1,1,1,1,1,1,1,1,
1,1,1,1,1,1,1,1,1,1,1,1,1,1,1,1,1,1,1,1,1,1,1,1,1,1,1,1,1,1,1,1,1,1,1,1,
1,1,1,1,1,1,1,1,1,1,1,1,1,1,1,1,1,1,1,1,1,1,1,1,1,1,1,1,1,1,1,1,1,1,1,1,
1,1,1,1,1,1,1,1,1,1,1,1,1,1,1,1,1,1,1,1,1,1,1,1,1,1,1,1,1,1,1,1,1,1,1,1,
1,1,1,1,1,1,1,1,1,1,1,1,1,1,1,1,1,1,1,1,1,1,1,1,1,1,1,1,1,1,1,1,1,1,1,1,
1,1,1,1,1,1,1,1,1,1,1,1,1,1,1,1,1,1,1,1,1,1,1,1,1,1,1,1,1,1,1,1,1,1,1,1,
1,1,1,1,1,1,1,1,1,1,1,1,1,1,1,1,1,1,1,1,1,1,1,1,1,1,1,1,1,1,1,1,1,1,1,1,
1,1,1,1,1,1,1,1,1,1,1,1,1,1,1,1,1,1,1,1,1,1,1,1,1,1,1,1,1,1,1,6),(2,2),
(0.143172103,0.144954128,0.146788991,0.148623853,0.150458716,0.152293578,
0.15412844,0.155963303,0.157798165,0.159633028,0.16146789,0.163302752,0.165137615,
0.166972477,0.168807339,0.170642202,0.172477064,0.174311927,0.176146789,
0.177981651,0.179816514,0.181651376,0.183486239,0.185321101,0.187155963,
0.188990826,0.190825688,0.19266055,0.194495413,0.196330275,0.198165138,
0.2,0.201834862,0.203669725,0.205504587,0.20733945,0.209174312,0.211009174,
0.212844037,0.214678899,0.216513761,0.218348624,0.220183486,0.222018349,
0.223853211,0.225688073,0.227522936,0.229357798,0.231192661,0.233027523,
0.234862385,0.236697248,0.23853211,0.240366972,0.242201835,0.244036697,
0.24587156,0.247706422,0.249541284,0.251376147,0.253211009,0.255045872,
0.256880734,0.258715596,0.260550459,0.262385321,0.264220183,0.266055046,
0.267889908,0.269724771,0.271559633,0.273394495,0.275229358,0.27706422,
0.278899083,0.280733945,0.282568807,0.28440367,0.286238532,0.288073394,
0.289908257,0.291743119,0.293577982,0.295412844,0.297247706,0.299082569,
0.300917431,0.302752294,0.304587156,0.306422018,0.308256881,0.310091743,
0.311926606,0.313761468,0.31559633,0.317431193,0.319266055,0.321100917,
0.32293578,0.324770642,0.326605505,0.328440367,0.330275229,0.332110092,
0.333944954,0.335779817,0.337614679,0.339449541,0.341284404,0.343119266,
0.344954128,0.346788991,0.348623853,0.350458716,0.352293578,0.35412844,
0.355963303,0.357798165,0.359633028,0.36146789,0.363302752,0.365137615,
0.366972477,0.368807339,0.370642202,0.372477064,0.374311927,0.376146789,
0.377981651,0.379816514,0.381651376,0.383486239,0.385321101,0.387155963,
0.388990826,0.390825688,0.39266055,0.394495413,0.396330275,0.398165138,
0.4,0.401834862,0.403669725,0.405504587,0.40733945,0.409174312,0.411009174,
0.412844037,0.414678899,0.416513761,0.418348624,0.420183486,0.422018349,
0.423853211,0.425688073,0.427522936,0.429357798,0.431192661,0.433027523,
0.434862385,0.436697248,0.43853211,0.440366972,0.442201835,0.444036697,
0.44587156,0.447706422,0.449541284,0.451376147,0.453211009,0.455045872,
0.456880734,0.458715596,0.460550459,0.462385321,0.464220183,0.466055046,
0.467889908,0.469724771,0.471559633,0.473394495,0.475229358,0.47706422,
0.478899083,0.480733945,0.482568807,0.48440367,0.486238532,0.488073394,
0.489908257,0.491743119,0.493577982,0.495412844,0.497247706,0.499082569,
0.500917431,0.502752294,0.504587156,0.506422018,0.508256881,0.510091743,
0.511926606,0.513761468,0.51559633,0.517431193,0.519266055,0.521100917,
0.52293578,0.524770642,0.526605505,0.528440367,0.530275229,0.532110092,
0.533944954,0.535779817,0.537614679,0.539449541,0.541284404,0.543119266,
0.544954128,0.546788991,0.548623853,0.550458716,0.552293578,0.55412844,
0.555963303,0.557798165,0.559633028,0.56146789,0.563302752,0.565137615,
0.566972477,0.568807339,0.570642202,0.572477064,0.574311927,0.576146789,
0.577981651,0.579816514,0.581651376,0.583486239,0.585321101,0.587155963,
0.588990826,0.590825688,0.59266055,0.594495413,0.596330275,0.598165138,
0.6,0.601834862,0.603669725,0.605504587,0.60733945,0.609174312,0.611009174,
0.612844037,0.614678899,0.616513761,0.618348624,0.620183486,0.622018349,
0.623853211,0.625688073,0.627522936,0.629357798,0.631192661,0.633027523,
0.634862385,0.636697248,0.63853211,0.640366972,0.642201835,0.644036697,
0.64587156,0.647706422,0.649541284,0.651376147,0.653211009,0.655045872,
0.656880734,0.658715596,0.660550459,0.662385321,0.664220183,0.666055046,
0.667889908,0.669724771,0.671559633,0.673394495,0.675229358,0.67706422,
0.678899083,0.680733945,0.682568807,0.68440367,0.686238532,0.688073394,
0.689908257,0.691743119,0.693577982,0.695412844,0.697247706,0.699082569,
0.700917431,0.702752294,0.704587156,0.706422018,0.708256881,0.710091743,
0.711926606,0.713761468,0.71559633,0.717431193,0.719266055,0.721100917,
0.72293578,0.724770642,0.726605505,0.728440367,0.730275229,0.732110092,
0.733944954,0.735779817,0.737614679,0.739449541,0.741284404,0.743119266,
0.744954128,0.746788991,0.748623853,0.750458716,0.752293578,0.75412844,
0.755963303,0.757798165,0.759633028,0.76146789,0.763302752,0.765137615,
0.766972477,0.768807339,0.770642202,0.772477064,0.774311927,0.776146789,
0.777981651,0.779816514,0.781651376,0.783486239,0.785321101,0.787155963,
0.788990826,0.790825688,0.79266055,0.794495413,0.796330275,0.798165138,
0.8,0.801834862,0.803669725,0.805504587,0.80733945,0.809174312,0.811009174,
0.812844037,0.814678899,0.816513761,0.818348624,0.820183486,0.822018349,
0.823853211,0.825688073,0.827522936,0.829357798,0.831192661,0.833027523,
0.834862385,0.836697248,0.83853211,0.840366972,0.842201835,0.844036697,
0.84587156,0.847706422,0.849541284,0.851376147,0.853211009,0.855045872,
0.856880734,0.858715596,0.860550459,0.862385321,0.864220183,0.866055046,
0.867889908,0.869724771,0.871559633,0.873394495,0.875229358,0.87706422,
0.878899083,0.880733945,0.882568807,0.88440367,0.886238532,0.888073394,
0.889908257,0.891743119,0.893577982,0.895412844,0.897247706,0.899082569,
0.900917431,0.902752294,0.904587156,0.906422018,0.908256881,0.910091743,
0.911926606,0.913761468,0.91559633,0.917431193,0.919266055,0.921100917,
0.92293578,0.924770642,0.926605505,0.928440367,0.930275229,0.932110092,
0.933944954,0.935779817,0.937614679,0.939449541,0.941284404,0.943119266,
0.944954128,0.946788991,0.948623853,0.950458716,0.952293578,0.95412844,
0.955963303,0.957798165,0.959633028,0.96146789,0.963302752,0.965137615,
0.966972477,0.968807339,0.970642202,0.972477064,0.974311927,0.976146789,
0.977981651,0.979816514,0.981651376,0.983486239,0.985321101,0.987155963,
0.988990826,0.990825688,0.99266055,0.994495413,0.996330275,0.998165138,
1.),(0.,0.36),.UNSPECIFIED.);
#6256=B_SPLINE_SURFACE_WITH_KNOTS('',5,1,((#221976,#221977),(#221978,#221979),
(#221980,#221981),(#221982,#221983),(#221984,#221985),(#221986,#221987),
(#221988,#221989),(#221990,#221991),(#221992,#221993),(#221994,#221995),
(#221996,#221997),(#221998,#221999),(#222000,#222001),(#222002,#222003),
(#222004,#222005),(#222006,#222007),(#222008,#222009),(#222010,#222011),
(#222012,#222013),(#222014,#222015),(#222016,#222017),(#222018,#222019),
(#222020,#222021),(#222022,#222023),(#222024,#222025),(#222026,#222027),
(#222028,#222029),(#222030,#222031),(#222032,#222033),(#222034,#222035),
(#222036,#222037),(#222038,#222039),(#222040,#222041),(#222042,#222043),
(#222044,#222045),(#222046,#222047),(#222048,#222049),(#222050,#222051),
(#222052,#222053),(#222054,#222055),(#222056,#222057),(#222058,#222059),
(#222060,#222061),(#222062,#222063),(#222064,#222065),(#222066,#222067),
(#222068,#222069),(#222070,#222071),(#222072,#222073),(#222074,#222075),
(#222076,#222077),(#222078,#222079),(#222080,#222081),(#222082,#222083),
(#222084,#222085),(#222086,#222087),(#222088,#222089),(#222090,#222091),
(#222092,#222093),(#222094,#222095),(#222096,#222097),(#222098,#222099),
(#222100,#222101),(#222102,#222103),(#222104,#222105),(#222106,#222107),
(#222108,#222109),(#222110,#222111),(#222112,#222113),(#222114,#222115),
(#222116,#222117),(#222118,#222119),(#222120,#222121),(#222122,#222123),
(#222124,#222125),(#222126,#222127),(#222128,#222129),(#222130,#222131),
(#222132,#222133),(#222134,#222135),(#222136,#222137),(#222138,#222139),
(#222140,#222141),(#222142,#222143),(#222144,#222145),(#222146,#222147),
(#222148,#222149),(#222150,#222151),(#222152,#222153),(#222154,#222155),
(#222156,#222157),(#222158,#222159),(#222160,#222161),(#222162,#222163),
(#222164,#222165),(#222166,#222167),(#222168,#222169),(#222170,#222171),
(#222172,#222173),(#222174,#222175),(#222176,#222177),(#222178,#222179),
(#222180,#222181),(#222182,#222183),(#222184,#222185),(#222186,#222187),
(#222188,#222189),(#222190,#222191),(#222192,#222193),(#222194,#222195),
(#222196,#222197),(#222198,#222199),(#222200,#222201),(#222202,#222203),
(#222204,#222205),(#222206,#222207),(#222208,#222209),(#222210,#222211),
(#222212,#222213),(#222214,#222215),(#222216,#222217),(#222218,#222219),
(#222220,#222221),(#222222,#222223),(#222224,#222225),(#222226,#222227),
(#222228,#222229),(#222230,#222231),(#222232,#222233),(#222234,#222235),
(#222236,#222237),(#222238,#222239),(#222240,#222241),(#222242,#222243),
(#222244,#222245),(#222246,#222247),(#222248,#222249),(#222250,#222251),
(#222252,#222253),(#222254,#222255),(#222256,#222257),(#222258,#222259),
(#222260,#222261),(#222262,#222263),(#222264,#222265),(#222266,#222267),
(#222268,#222269),(#222270,#222271),(#222272,#222273),(#222274,#222275),
(#222276,#222277),(#222278,#222279),(#222280,#222281),(#222282,#222283),
(#222284,#222285),(#222286,#222287),(#222288,#222289),(#222290,#222291),
(#222292,#222293),(#222294,#222295),(#222296,#222297),(#222298,#222299),
(#222300,#222301),(#222302,#222303),(#222304,#222305),(#222306,#222307),
(#222308,#222309),(#222310,#222311),(#222312,#222313),(#222314,#222315),
(#222316,#222317),(#222318,#222319),(#222320,#222321),(#222322,#222323),
(#222324,#222325),(#222326,#222327),(#222328,#222329),(#222330,#222331),
(#222332,#222333),(#222334,#222335),(#222336,#222337),(#222338,#222339),
(#222340,#222341),(#222342,#222343),(#222344,#222345),(#222346,#222347),
(#222348,#222349),(#222350,#222351),(#222352,#222353),(#222354,#222355),
(#222356,#222357),(#222358,#222359),(#222360,#222361),(#222362,#222363),
(#222364,#222365),(#222366,#222367),(#222368,#222369),(#222370,#222371),
(#222372,#222373),(#222374,#222375),(#222376,#222377),(#222378,#222379),
(#222380,#222381),(#222382,#222383),(#222384,#222385),(#222386,#222387),
(#222388,#222389),(#222390,#222391),(#222392,#222393),(#222394,#222395),
(#222396,#222397),(#222398,#222399),(#222400,#222401),(#222402,#222403),
(#222404,#222405),(#222406,#222407),(#222408,#222409),(#222410,#222411),
(#222412,#222413),(#222414,#222415),(#222416,#222417),(#222418,#222419),
(#222420,#222421),(#222422,#222423),(#222424,#222425),(#222426,#222427),
(#222428,#222429),(#222430,#222431),(#222432,#222433),(#222434,#222435),
(#222436,#222437),(#222438,#222439),(#222440,#222441),(#222442,#222443),
(#222444,#222445),(#222446,#222447),(#222448,#222449),(#222450,#222451),
(#222452,#222453),(#222454,#222455),(#222456,#222457),(#222458,#222459),
(#222460,#222461),(#222462,#222463),(#222464,#222465),(#222466,#222467),
(#222468,#222469),(#222470,#222471),(#222472,#222473),(#222474,#222475),
(#222476,#222477),(#222478,#222479),(#222480,#222481),(#222482,#222483),
(#222484,#222485),(#222486,#222487),(#222488,#222489),(#222490,#222491),
(#222492,#222493),(#222494,#222495),(#222496,#222497),(#222498,#222499),
(#222500,#222501),(#222502,#222503),(#222504,#222505),(#222506,#222507),
(#222508,#222509),(#222510,#222511),(#222512,#222513),(#222514,#222515),
(#222516,#222517),(#222518,#222519),(#222520,#222521),(#222522,#222523),
(#222524,#222525),(#222526,#222527),(#222528,#222529),(#222530,#222531),
(#222532,#222533),(#222534,#222535),(#222536,#222537),(#222538,#222539),
(#222540,#222541),(#222542,#222543),(#222544,#222545),(#222546,#222547),
(#222548,#222549),(#222550,#222551),(#222552,#222553),(#222554,#222555),
(#222556,#222557),(#222558,#222559),(#222560,#222561),(#222562,#222563),
(#222564,#222565),(#222566,#222567),(#222568,#222569),(#222570,#222571),
(#222572,#222573),(#222574,#222575),(#222576,#222577),(#222578,#222579),
(#222580,#222581),(#222582,#222583),(#222584,#222585),(#222586,#222587),
(#222588,#222589),(#222590,#222591),(#222592,#222593),(#222594,#222595),
(#222596,#222597),(#222598,#222599),(#222600,#222601),(#222602,#222603),
(#222604,#222605),(#222606,#222607),(#222608,#222609),(#222610,#222611),
(#222612,#222613),(#222614,#222615),(#222616,#222617),(#222618,#222619),
(#222620,#222621),(#222622,#222623),(#222624,#222625),(#222626,#222627),
(#222628,#222629),(#222630,#222631),(#222632,#222633),(#222634,#222635),
(#222636,#222637),(#222638,#222639),(#222640,#222641),(#222642,#222643),
(#222644,#222645),(#222646,#222647),(#222648,#222649),(#222650,#222651),
(#222652,#222653),(#222654,#222655),(#222656,#222657),(#222658,#222659),
(#222660,#222661),(#222662,#222663),(#222664,#222665),(#222666,#222667),
(#222668,#222669),(#222670,#222671),(#222672,#222673),(#222674,#222675),
(#222676,#222677),(#222678,#222679),(#222680,#222681),(#222682,#222683),
(#222684,#222685),(#222686,#222687),(#222688,#222689),(#222690,#222691),
(#222692,#222693),(#222694,#222695),(#222696,#222697),(#222698,#222699),
(#222700,#222701),(#222702,#222703),(#222704,#222705),(#222706,#222707),
(#222708,#222709),(#222710,#222711),(#222712,#222713),(#222714,#222715),
(#222716,#222717),(#222718,#222719),(#222720,#222721),(#222722,#222723),
(#222724,#222725),(#222726,#222727),(#222728,#222729),(#222730,#222731),
(#222732,#222733),(#222734,#222735),(#222736,#222737),(#222738,#222739),
(#222740,#222741),(#222742,#222743),(#222744,#222745),(#222746,#222747),
(#222748,#222749),(#222750,#222751),(#222752,#222753),(#222754,#222755),
(#222756,#222757),(#222758,#222759),(#222760,#222761),(#222762,#222763),
(#222764,#222765),(#222766,#222767),(#222768,#222769),(#222770,#222771),
(#222772,#222773),(#222774,#222775),(#222776,#222777),(#222778,#222779),
(#222780,#222781),(#222782,#222783),(#222784,#222785),(#222786,#222787),
(#222788,#222789),(#222790,#222791),(#222792,#222793),(#222794,#222795),
(#222796,#222797),(#222798,#222799),(#222800,#222801),(#222802,#222803),
(#222804,#222805),(#222806,#222807),(#222808,#222809),(#222810,#222811),
(#222812,#222813),(#222814,#222815),(#222816,#222817),(#222818,#222819),
(#222820,#222821),(#222822,#222823),(#222824,#222825),(#222826,#222827),
(#222828,#222829),(#222830,#222831),(#222832,#222833),(#222834,#222835),
(#222836,#222837),(#222838,#222839),(#222840,#222841),(#222842,#222843),
(#222844,#222845),(#222846,#222847),(#222848,#222849),(#222850,#222851),
(#222852,#222853),(#222854,#222855),(#222856,#222857),(#222858,#222859),
(#222860,#222861),(#222862,#222863),(#222864,#222865),(#222866,#222867),
(#222868,#222869),(#222870,#222871),(#222872,#222873),(#222874,#222875),
(#222876,#222877),(#222878,#222879),(#222880,#222881),(#222882,#222883),
(#222884,#222885),(#222886,#222887),(#222888,#222889),(#222890,#222891),
(#222892,#222893),(#222894,#222895),(#222896,#222897),(#222898,#222899),
(#222900,#222901),(#222902,#222903),(#222904,#222905),(#222906,#222907),
(#222908,#222909),(#222910,#222911),(#222912,#222913),(#222914,#222915),
(#222916,#222917),(#222918,#222919)),.UNSPECIFIED.,.F.,.F.,.F.,(6,1,1,1,
1,1,1,1,1,1,1,1,1,1,1,1,1,1,1,1,1,1,1,1,1,1,1,1,1,1,1,1,1,1,1,1,1,1,1,1,
1,1,1,1,1,1,1,1,1,1,1,1,1,1,1,1,1,1,1,1,1,1,1,1,1,1,1,1,1,1,1,1,1,1,1,1,
1,1,1,1,1,1,1,1,1,1,1,1,1,1,1,1,1,1,1,1,1,1,1,1,1,1,1,1,1,1,1,1,1,1,1,1,
1,1,1,1,1,1,1,1,1,1,1,1,1,1,1,1,1,1,1,1,1,1,1,1,1,1,1,1,1,1,1,1,1,1,1,1,
1,1,1,1,1,1,1,1,1,1,1,1,1,1,1,1,1,1,1,1,1,1,1,1,1,1,1,1,1,1,1,1,1,1,1,1,
1,1,1,1,1,1,1,1,1,1,1,1,1,1,1,1,1,1,1,1,1,1,1,1,1,1,1,1,1,1,1,1,1,1,1,1,
1,1,1,1,1,1,1,1,1,1,1,1,1,1,1,1,1,1,1,1,1,1,1,1,1,1,1,1,1,1,1,1,1,1,1,1,
1,1,1,1,1,1,1,1,1,1,1,1,1,1,1,1,1,1,1,1,1,1,1,1,1,1,1,1,1,1,1,1,1,1,1,1,
1,1,1,1,1,1,1,1,1,1,1,1,1,1,1,1,1,1,1,1,1,1,1,1,1,1,1,1,1,1,1,1,1,1,1,1,
1,1,1,1,1,1,1,1,1,1,1,1,1,1,1,1,1,1,1,1,1,1,1,1,1,1,1,1,1,1,1,1,1,1,1,1,
1,1,1,1,1,1,1,1,1,1,1,1,1,1,1,1,1,1,1,1,1,1,1,1,1,1,1,1,1,1,1,1,1,1,1,1,
1,1,1,1,1,1,1,1,1,1,1,1,1,1,1,1,1,1,1,1,1,1,1,1,1,1,1,1,1,1,1,1,1,1,1,1,
1,1,1,1,1,1,1,1,1,1,1,1,1,1,1,1,1,1,1,1,1,1,1,1,1,1,1,1,1,1,1,6),(2,2),
(-1.,-0.998165138,-0.996330275,-0.994495413,-0.99266055,-0.990825688,-0.988990826,
-0.987155963,-0.985321101,-0.983486239,-0.981651376,-0.979816514,-0.977981651,
-0.976146789,-0.974311927,-0.972477064,-0.970642202,-0.968807339,-0.966972477,
-0.965137615,-0.963302752,-0.96146789,-0.959633028,-0.957798165,-0.955963303,
-0.95412844,-0.952293578,-0.950458716,-0.948623853,-0.946788991,-0.944954128,
-0.943119266,-0.941284404,-0.939449541,-0.937614679,-0.935779817,-0.933944954,
-0.932110092,-0.930275229,-0.928440367,-0.926605505,-0.924770642,-0.92293578,
-0.921100917,-0.919266055,-0.917431193,-0.91559633,-0.913761468,-0.911926606,
-0.910091743,-0.908256881,-0.906422018,-0.904587156,-0.902752294,-0.900917431,
-0.899082569,-0.897247706,-0.895412844,-0.893577982,-0.891743119,-0.889908257,
-0.888073394,-0.886238532,-0.88440367,-0.882568807,-0.880733945,-0.878899083,
-0.87706422,-0.875229358,-0.873394495,-0.871559633,-0.869724771,-0.867889908,
-0.866055046,-0.864220183,-0.862385321,-0.860550459,-0.858715596,-0.856880734,
-0.855045872,-0.853211009,-0.851376147,-0.849541284,-0.847706422,-0.84587156,
-0.844036697,-0.842201835,-0.840366972,-0.83853211,-0.836697248,-0.834862385,
-0.833027523,-0.831192661,-0.829357798,-0.827522936,-0.825688073,-0.823853211,
-0.822018349,-0.820183486,-0.818348624,-0.816513761,-0.814678899,-0.812844037,
-0.811009174,-0.809174312,-0.80733945,-0.805504587,-0.803669725,-0.801834862,
-0.8,-0.798165138,-0.796330275,-0.794495413,-0.79266055,-0.790825688,-0.788990826,
-0.787155963,-0.785321101,-0.783486239,-0.781651376,-0.779816514,-0.777981651,
-0.776146789,-0.774311927,-0.772477064,-0.770642202,-0.768807339,-0.766972477,
-0.765137615,-0.763302752,-0.76146789,-0.759633028,-0.757798165,-0.755963303,
-0.75412844,-0.752293578,-0.750458716,-0.748623853,-0.746788991,-0.744954128,
-0.743119266,-0.741284404,-0.739449541,-0.737614679,-0.735779817,-0.733944954,
-0.732110092,-0.730275229,-0.728440367,-0.726605505,-0.724770642,-0.72293578,
-0.721100917,-0.719266055,-0.717431193,-0.71559633,-0.713761468,-0.711926606,
-0.710091743,-0.708256881,-0.706422018,-0.704587156,-0.702752294,-0.700917431,
-0.699082569,-0.697247706,-0.695412844,-0.693577982,-0.691743119,-0.689908257,
-0.688073394,-0.686238532,-0.68440367,-0.682568807,-0.680733945,-0.678899083,
-0.67706422,-0.675229358,-0.673394495,-0.671559633,-0.669724771,-0.667889908,
-0.666055046,-0.664220183,-0.662385321,-0.660550459,-0.658715596,-0.656880734,
-0.655045872,-0.653211009,-0.651376147,-0.649541284,-0.647706422,-0.64587156,
-0.644036697,-0.642201835,-0.640366972,-0.63853211,-0.636697248,-0.634862385,
-0.633027523,-0.631192661,-0.629357798,-0.627522936,-0.625688073,-0.623853211,
-0.622018349,-0.620183486,-0.618348624,-0.616513761,-0.614678899,-0.612844037,
-0.611009174,-0.609174312,-0.60733945,-0.605504587,-0.603669725,-0.601834862,
-0.6,-0.598165138,-0.596330275,-0.594495413,-0.59266055,-0.590825688,-0.588990826,
-0.587155963,-0.585321101,-0.583486239,-0.581651376,-0.579816514,-0.577981651,
-0.576146789,-0.574311927,-0.572477064,-0.570642202,-0.568807339,-0.566972477,
-0.565137615,-0.563302752,-0.56146789,-0.559633028,-0.557798165,-0.555963303,
-0.55412844,-0.552293578,-0.550458716,-0.548623853,-0.546788991,-0.544954128,
-0.543119266,-0.541284404,-0.539449541,-0.537614679,-0.535779817,-0.533944954,
-0.532110092,-0.530275229,-0.528440367,-0.526605505,-0.524770642,-0.52293578,
-0.521100917,-0.519266055,-0.517431193,-0.51559633,-0.513761468,-0.511926606,
-0.510091743,-0.508256881,-0.506422018,-0.504587156,-0.502752294,-0.500917431,
-0.499082569,-0.497247706,-0.495412844,-0.493577982,-0.491743119,-0.489908257,
-0.488073394,-0.486238532,-0.48440367,-0.482568807,-0.480733945,-0.478899083,
-0.47706422,-0.475229358,-0.473394495,-0.471559633,-0.469724771,-0.467889908,
-0.466055046,-0.464220183,-0.462385321,-0.460550459,-0.458715596,-0.456880734,
-0.455045872,-0.453211009,-0.451376147,-0.449541284,-0.447706422,-0.44587156,
-0.444036697,-0.442201835,-0.440366972,-0.43853211,-0.436697248,-0.434862385,
-0.433027523,-0.431192661,-0.429357798,-0.427522936,-0.425688073,-0.423853211,
-0.422018349,-0.420183486,-0.418348624,-0.416513761,-0.414678899,-0.412844037,
-0.411009174,-0.409174312,-0.40733945,-0.405504587,-0.403669725,-0.401834862,
-0.4,-0.398165138,-0.396330275,-0.394495413,-0.39266055,-0.390825688,-0.388990826,
-0.387155963,-0.385321101,-0.383486239,-0.381651376,-0.379816514,-0.377981651,
-0.376146789,-0.374311927,-0.372477064,-0.370642202,-0.368807339,-0.366972477,
-0.365137615,-0.363302752,-0.36146789,-0.359633028,-0.357798165,-0.355963303,
-0.35412844,-0.352293578,-0.350458716,-0.348623853,-0.346788991,-0.344954128,
-0.343119266,-0.341284404,-0.339449541,-0.337614679,-0.335779817,-0.333944954,
-0.332110092,-0.330275229,-0.328440367,-0.326605505,-0.324770642,-0.32293578,
-0.321100917,-0.319266055,-0.317431193,-0.31559633,-0.313761468,-0.311926606,
-0.310091743,-0.308256881,-0.306422018,-0.304587156,-0.302752294,-0.300917431,
-0.299082569,-0.297247706,-0.295412844,-0.293577982,-0.291743119,-0.289908257,
-0.288073394,-0.286238532,-0.28440367,-0.282568807,-0.280733945,-0.278899083,
-0.27706422,-0.275229358,-0.273394495,-0.271559633,-0.269724771,-0.267889908,
-0.266055046,-0.264220183,-0.262385321,-0.260550459,-0.258715596,-0.256880734,
-0.255045872,-0.253211009,-0.251376147,-0.249541284,-0.247706422,-0.24587156,
-0.244036697,-0.242201835,-0.240366972,-0.23853211,-0.236697248,-0.234862385,
-0.233027523,-0.231192661,-0.229357798,-0.227522936,-0.225688073,-0.223853211,
-0.222018349,-0.220183486,-0.218348624,-0.216513761,-0.214678899,-0.212844037,
-0.211009174,-0.209174312,-0.20733945,-0.205504587,-0.203669725,-0.201834862,
-0.2,-0.198165138,-0.196330275,-0.194495413,-0.19266055,-0.190825688,-0.188990826,
-0.187155963,-0.185321101,-0.183486239,-0.181651376,-0.179816514,-0.177981651,
-0.176146789,-0.174311927,-0.172477064,-0.170642202,-0.168807339,-0.166972477,
-0.165137615,-0.163302752,-0.16146789,-0.159633028,-0.157798165,-0.155963303,
-0.15412844,-0.152293578,-0.150458716,-0.148623853,-0.146788991,-0.144954128,
-0.143172103),(0.,0.36),.UNSPECIFIED.);
#6257=B_SPLINE_SURFACE_WITH_KNOTS('',5,1,((#223564,#223565),(#223566,#223567),
(#223568,#223569),(#223570,#223571),(#223572,#223573),(#223574,#223575),
(#223576,#223577),(#223578,#223579),(#223580,#223581),(#223582,#223583),
(#223584,#223585),(#223586,#223587),(#223588,#223589),(#223590,#223591),
(#223592,#223593),(#223594,#223595),(#223596,#223597),(#223598,#223599),
(#223600,#223601),(#223602,#223603),(#223604,#223605),(#223606,#223607),
(#223608,#223609),(#223610,#223611),(#223612,#223613),(#223614,#223615),
(#223616,#223617),(#223618,#223619),(#223620,#223621),(#223622,#223623),
(#223624,#223625),(#223626,#223627),(#223628,#223629),(#223630,#223631),
(#223632,#223633),(#223634,#223635),(#223636,#223637),(#223638,#223639),
(#223640,#223641),(#223642,#223643),(#223644,#223645),(#223646,#223647),
(#223648,#223649),(#223650,#223651),(#223652,#223653),(#223654,#223655),
(#223656,#223657),(#223658,#223659),(#223660,#223661),(#223662,#223663),
(#223664,#223665),(#223666,#223667),(#223668,#223669),(#223670,#223671),
(#223672,#223673),(#223674,#223675),(#223676,#223677),(#223678,#223679),
(#223680,#223681),(#223682,#223683),(#223684,#223685),(#223686,#223687),
(#223688,#223689),(#223690,#223691),(#223692,#223693),(#223694,#223695),
(#223696,#223697),(#223698,#223699),(#223700,#223701),(#223702,#223703),
(#223704,#223705),(#223706,#223707),(#223708,#223709),(#223710,#223711),
(#223712,#223713),(#223714,#223715),(#223716,#223717),(#223718,#223719),
(#223720,#223721),(#223722,#223723),(#223724,#223725),(#223726,#223727),
(#223728,#223729),(#223730,#223731),(#223732,#223733),(#223734,#223735),
(#223736,#223737),(#223738,#223739),(#223740,#223741),(#223742,#223743),
(#223744,#223745),(#223746,#223747),(#223748,#223749),(#223750,#223751),
(#223752,#223753),(#223754,#223755),(#223756,#223757),(#223758,#223759),
(#223760,#223761),(#223762,#223763),(#223764,#223765),(#223766,#223767),
(#223768,#223769),(#223770,#223771),(#223772,#223773),(#223774,#223775),
(#223776,#223777),(#223778,#223779),(#223780,#223781),(#223782,#223783),
(#223784,#223785),(#223786,#223787),(#223788,#223789),(#223790,#223791),
(#223792,#223793),(#223794,#223795),(#223796,#223797),(#223798,#223799),
(#223800,#223801),(#223802,#223803),(#223804,#223805),(#223806,#223807),
(#223808,#223809),(#223810,#223811),(#223812,#223813),(#223814,#223815),
(#223816,#223817),(#223818,#223819),(#223820,#223821),(#223822,#223823),
(#223824,#223825),(#223826,#223827),(#223828,#223829),(#223830,#223831),
(#223832,#223833),(#223834,#223835),(#223836,#223837),(#223838,#223839),
(#223840,#223841),(#223842,#223843),(#223844,#223845),(#223846,#223847),
(#223848,#223849),(#223850,#223851),(#223852,#223853),(#223854,#223855),
(#223856,#223857),(#223858,#223859),(#223860,#223861),(#223862,#223863),
(#223864,#223865),(#223866,#223867),(#223868,#223869),(#223870,#223871),
(#223872,#223873),(#223874,#223875),(#223876,#223877),(#223878,#223879),
(#223880,#223881),(#223882,#223883),(#223884,#223885),(#223886,#223887),
(#223888,#223889),(#223890,#223891),(#223892,#223893),(#223894,#223895),
(#223896,#223897),(#223898,#223899),(#223900,#223901),(#223902,#223903),
(#223904,#223905),(#223906,#223907),(#223908,#223909),(#223910,#223911),
(#223912,#223913),(#223914,#223915),(#223916,#223917),(#223918,#223919),
(#223920,#223921),(#223922,#223923),(#223924,#223925),(#223926,#223927),
(#223928,#223929),(#223930,#223931),(#223932,#223933),(#223934,#223935),
(#223936,#223937),(#223938,#223939),(#223940,#223941),(#223942,#223943),
(#223944,#223945),(#223946,#223947),(#223948,#223949),(#223950,#223951),
(#223952,#223953),(#223954,#223955),(#223956,#223957),(#223958,#223959),
(#223960,#223961),(#223962,#223963),(#223964,#223965),(#223966,#223967),
(#223968,#223969),(#223970,#223971),(#223972,#223973),(#223974,#223975),
(#223976,#223977),(#223978,#223979),(#223980,#223981),(#223982,#223983),
(#223984,#223985),(#223986,#223987),(#223988,#223989),(#223990,#223991),
(#223992,#223993),(#223994,#223995),(#223996,#223997),(#223998,#223999),
(#224000,#224001),(#224002,#224003),(#224004,#224005),(#224006,#224007),
(#224008,#224009),(#224010,#224011),(#224012,#224013),(#224014,#224015),
(#224016,#224017),(#224018,#224019),(#224020,#224021),(#224022,#224023),
(#224024,#224025),(#224026,#224027),(#224028,#224029),(#224030,#224031),
(#224032,#224033),(#224034,#224035),(#224036,#224037),(#224038,#224039),
(#224040,#224041),(#224042,#224043),(#224044,#224045),(#224046,#224047),
(#224048,#224049),(#224050,#224051),(#224052,#224053),(#224054,#224055),
(#224056,#224057),(#224058,#224059),(#224060,#224061),(#224062,#224063),
(#224064,#224065),(#224066,#224067),(#224068,#224069),(#224070,#224071),
(#224072,#224073),(#224074,#224075),(#224076,#224077),(#224078,#224079),
(#224080,#224081),(#224082,#224083),(#224084,#224085),(#224086,#224087),
(#224088,#224089),(#224090,#224091),(#224092,#224093),(#224094,#224095),
(#224096,#224097),(#224098,#224099),(#224100,#224101),(#224102,#224103),
(#224104,#224105),(#224106,#224107),(#224108,#224109),(#224110,#224111),
(#224112,#224113),(#224114,#224115),(#224116,#224117),(#224118,#224119),
(#224120,#224121),(#224122,#224123),(#224124,#224125),(#224126,#224127),
(#224128,#224129),(#224130,#224131),(#224132,#224133),(#224134,#224135),
(#224136,#224137),(#224138,#224139),(#224140,#224141),(#224142,#224143),
(#224144,#224145),(#224146,#224147),(#224148,#224149),(#224150,#224151),
(#224152,#224153),(#224154,#224155),(#224156,#224157),(#224158,#224159),
(#224160,#224161),(#224162,#224163),(#224164,#224165),(#224166,#224167),
(#224168,#224169),(#224170,#224171),(#224172,#224173),(#224174,#224175),
(#224176,#224177),(#224178,#224179),(#224180,#224181),(#224182,#224183),
(#224184,#224185),(#224186,#224187),(#224188,#224189),(#224190,#224191),
(#224192,#224193),(#224194,#224195),(#224196,#224197),(#224198,#224199),
(#224200,#224201),(#224202,#224203),(#224204,#224205),(#224206,#224207),
(#224208,#224209),(#224210,#224211),(#224212,#224213),(#224214,#224215),
(#224216,#224217),(#224218,#224219),(#224220,#224221),(#224222,#224223),
(#224224,#224225),(#224226,#224227),(#224228,#224229),(#224230,#224231),
(#224232,#224233),(#224234,#224235),(#224236,#224237),(#224238,#224239),
(#224240,#224241),(#224242,#224243),(#224244,#224245),(#224246,#224247),
(#224248,#224249),(#224250,#224251),(#224252,#224253),(#224254,#224255),
(#224256,#224257),(#224258,#224259),(#224260,#224261),(#224262,#224263),
(#224264,#224265),(#224266,#224267),(#224268,#224269),(#224270,#224271),
(#224272,#224273),(#224274,#224275),(#224276,#224277),(#224278,#224279),
(#224280,#224281),(#224282,#224283),(#224284,#224285),(#224286,#224287),
(#224288,#224289),(#224290,#224291),(#224292,#224293),(#224294,#224295),
(#224296,#224297),(#224298,#224299),(#224300,#224301),(#224302,#224303),
(#224304,#224305),(#224306,#224307),(#224308,#224309),(#224310,#224311),
(#224312,#224313),(#224314,#224315),(#224316,#224317),(#224318,#224319),
(#224320,#224321),(#224322,#224323),(#224324,#224325),(#224326,#224327),
(#224328,#224329),(#224330,#224331),(#224332,#224333),(#224334,#224335),
(#224336,#224337),(#224338,#224339),(#224340,#224341),(#224342,#224343),
(#224344,#224345),(#224346,#224347),(#224348,#224349),(#224350,#224351),
(#224352,#224353),(#224354,#224355),(#224356,#224357),(#224358,#224359),
(#224360,#224361),(#224362,#224363),(#224364,#224365),(#224366,#224367),
(#224368,#224369),(#224370,#224371),(#224372,#224373),(#224374,#224375),
(#224376,#224377),(#224378,#224379),(#224380,#224381),(#224382,#224383),
(#224384,#224385),(#224386,#224387),(#224388,#224389),(#224390,#224391),
(#224392,#224393),(#224394,#224395),(#224396,#224397),(#224398,#224399),
(#224400,#224401),(#224402,#224403),(#224404,#224405),(#224406,#224407),
(#224408,#224409),(#224410,#224411),(#224412,#224413),(#224414,#224415),
(#224416,#224417),(#224418,#224419),(#224420,#224421),(#224422,#224423),
(#224424,#224425),(#224426,#224427),(#224428,#224429),(#224430,#224431),
(#224432,#224433),(#224434,#224435),(#224436,#224437),(#224438,#224439),
(#224440,#224441),(#224442,#224443),(#224444,#224445),(#224446,#224447),
(#224448,#224449),(#224450,#224451),(#224452,#224453),(#224454,#224455),
(#224456,#224457),(#224458,#224459),(#224460,#224461),(#224462,#224463),
(#224464,#224465),(#224466,#224467),(#224468,#224469),(#224470,#224471),
(#224472,#224473),(#224474,#224475),(#224476,#224477),(#224478,#224479),
(#224480,#224481),(#224482,#224483),(#224484,#224485),(#224486,#224487),
(#224488,#224489),(#224490,#224491),(#224492,#224493),(#224494,#224495),
(#224496,#224497),(#224498,#224499),(#224500,#224501),(#224502,#224503),
(#224504,#224505),(#224506,#224507)),.UNSPECIFIED.,.F.,.F.,.F.,(6,1,1,1,
1,1,1,1,1,1,1,1,1,1,1,1,1,1,1,1,1,1,1,1,1,1,1,1,1,1,1,1,1,1,1,1,1,1,1,1,
1,1,1,1,1,1,1,1,1,1,1,1,1,1,1,1,1,1,1,1,1,1,1,1,1,1,1,1,1,1,1,1,1,1,1,1,
1,1,1,1,1,1,1,1,1,1,1,1,1,1,1,1,1,1,1,1,1,1,1,1,1,1,1,1,1,1,1,1,1,1,1,1,
1,1,1,1,1,1,1,1,1,1,1,1,1,1,1,1,1,1,1,1,1,1,1,1,1,1,1,1,1,1,1,1,1,1,1,1,
1,1,1,1,1,1,1,1,1,1,1,1,1,1,1,1,1,1,1,1,1,1,1,1,1,1,1,1,1,1,1,1,1,1,1,1,
1,1,1,1,1,1,1,1,1,1,1,1,1,1,1,1,1,1,1,1,1,1,1,1,1,1,1,1,1,1,1,1,1,1,1,1,
1,1,1,1,1,1,1,1,1,1,1,1,1,1,1,1,1,1,1,1,1,1,1,1,1,1,1,1,1,1,1,1,1,1,1,1,
1,1,1,1,1,1,1,1,1,1,1,1,1,1,1,1,1,1,1,1,1,1,1,1,1,1,1,1,1,1,1,1,1,1,1,1,
1,1,1,1,1,1,1,1,1,1,1,1,1,1,1,1,1,1,1,1,1,1,1,1,1,1,1,1,1,1,1,1,1,1,1,1,
1,1,1,1,1,1,1,1,1,1,1,1,1,1,1,1,1,1,1,1,1,1,1,1,1,1,1,1,1,1,1,1,1,1,1,1,
1,1,1,1,1,1,1,1,1,1,1,1,1,1,1,1,1,1,1,1,1,1,1,1,1,1,1,1,1,1,1,1,1,1,1,1,
1,1,1,1,1,1,1,1,1,1,1,1,1,1,1,1,1,1,1,1,1,1,1,1,1,1,1,1,1,1,1,1,1,1,1,1,
1,1,1,1,1,1,1,1,1,1,1,1,1,1,1,1,1,1,1,1,1,1,1,1,1,1,1,1,1,1,1,6),(2,2),
(-1.,-0.998165138,-0.996330275,-0.994495413,-0.99266055,-0.990825688,-0.988990826,
-0.987155963,-0.985321101,-0.983486239,-0.981651376,-0.979816514,-0.977981651,
-0.976146789,-0.974311927,-0.972477064,-0.970642202,-0.968807339,-0.966972477,
-0.965137615,-0.963302752,-0.96146789,-0.959633028,-0.957798165,-0.955963303,
-0.95412844,-0.952293578,-0.950458716,-0.948623853,-0.946788991,-0.944954128,
-0.943119266,-0.941284404,-0.939449541,-0.937614679,-0.935779817,-0.933944954,
-0.932110092,-0.930275229,-0.928440367,-0.926605505,-0.924770642,-0.92293578,
-0.921100917,-0.919266055,-0.917431193,-0.91559633,-0.913761468,-0.911926606,
-0.910091743,-0.908256881,-0.906422018,-0.904587156,-0.902752294,-0.900917431,
-0.899082569,-0.897247706,-0.895412844,-0.893577982,-0.891743119,-0.889908257,
-0.888073394,-0.886238532,-0.88440367,-0.882568807,-0.880733945,-0.878899083,
-0.87706422,-0.875229358,-0.873394495,-0.871559633,-0.869724771,-0.867889908,
-0.866055046,-0.864220183,-0.862385321,-0.860550459,-0.858715596,-0.856880734,
-0.855045872,-0.853211009,-0.851376147,-0.849541284,-0.847706422,-0.84587156,
-0.844036697,-0.842201835,-0.840366972,-0.83853211,-0.836697248,-0.834862385,
-0.833027523,-0.831192661,-0.829357798,-0.827522936,-0.825688073,-0.823853211,
-0.822018349,-0.820183486,-0.818348624,-0.816513761,-0.814678899,-0.812844037,
-0.811009174,-0.809174312,-0.80733945,-0.805504587,-0.803669725,-0.801834862,
-0.8,-0.798165138,-0.796330275,-0.794495413,-0.79266055,-0.790825688,-0.788990826,
-0.787155963,-0.785321101,-0.783486239,-0.781651376,-0.779816514,-0.777981651,
-0.776146789,-0.774311927,-0.772477064,-0.770642202,-0.768807339,-0.766972477,
-0.765137615,-0.763302752,-0.76146789,-0.759633028,-0.757798165,-0.755963303,
-0.75412844,-0.752293578,-0.750458716,-0.748623853,-0.746788991,-0.744954128,
-0.743119266,-0.741284404,-0.739449541,-0.737614679,-0.735779817,-0.733944954,
-0.732110092,-0.730275229,-0.728440367,-0.726605505,-0.724770642,-0.72293578,
-0.721100917,-0.719266055,-0.717431193,-0.71559633,-0.713761468,-0.711926606,
-0.710091743,-0.708256881,-0.706422018,-0.704587156,-0.702752294,-0.700917431,
-0.699082569,-0.697247706,-0.695412844,-0.693577982,-0.691743119,-0.689908257,
-0.688073394,-0.686238532,-0.68440367,-0.682568807,-0.680733945,-0.678899083,
-0.67706422,-0.675229358,-0.673394495,-0.671559633,-0.669724771,-0.667889908,
-0.666055046,-0.664220183,-0.662385321,-0.660550459,-0.658715596,-0.656880734,
-0.655045872,-0.653211009,-0.651376147,-0.649541284,-0.647706422,-0.64587156,
-0.644036697,-0.642201835,-0.640366972,-0.63853211,-0.636697248,-0.634862385,
-0.633027523,-0.631192661,-0.629357798,-0.627522936,-0.625688073,-0.623853211,
-0.622018349,-0.620183486,-0.618348624,-0.616513761,-0.614678899,-0.612844037,
-0.611009174,-0.609174312,-0.60733945,-0.605504587,-0.603669725,-0.601834862,
-0.6,-0.598165138,-0.596330275,-0.594495413,-0.59266055,-0.590825688,-0.588990826,
-0.587155963,-0.585321101,-0.583486239,-0.581651376,-0.579816514,-0.577981651,
-0.576146789,-0.574311927,-0.572477064,-0.570642202,-0.568807339,-0.566972477,
-0.565137615,-0.563302752,-0.56146789,-0.559633028,-0.557798165,-0.555963303,
-0.55412844,-0.552293578,-0.550458716,-0.548623853,-0.546788991,-0.544954128,
-0.543119266,-0.541284404,-0.539449541,-0.537614679,-0.535779817,-0.533944954,
-0.532110092,-0.530275229,-0.528440367,-0.526605505,-0.524770642,-0.52293578,
-0.521100917,-0.519266055,-0.517431193,-0.51559633,-0.513761468,-0.511926606,
-0.510091743,-0.508256881,-0.506422018,-0.504587156,-0.502752294,-0.500917431,
-0.499082569,-0.497247706,-0.495412844,-0.493577982,-0.491743119,-0.489908257,
-0.488073394,-0.486238532,-0.48440367,-0.482568807,-0.480733945,-0.478899083,
-0.47706422,-0.475229358,-0.473394495,-0.471559633,-0.469724771,-0.467889908,
-0.466055046,-0.464220183,-0.462385321,-0.460550459,-0.458715596,-0.456880734,
-0.455045872,-0.453211009,-0.451376147,-0.449541284,-0.447706422,-0.44587156,
-0.444036697,-0.442201835,-0.440366972,-0.43853211,-0.436697248,-0.434862385,
-0.433027523,-0.431192661,-0.429357798,-0.427522936,-0.425688073,-0.423853211,
-0.422018349,-0.420183486,-0.418348624,-0.416513761,-0.414678899,-0.412844037,
-0.411009174,-0.409174312,-0.40733945,-0.405504587,-0.403669725,-0.401834862,
-0.4,-0.398165138,-0.396330275,-0.394495413,-0.39266055,-0.390825688,-0.388990826,
-0.387155963,-0.385321101,-0.383486239,-0.381651376,-0.379816514,-0.377981651,
-0.376146789,-0.374311927,-0.372477064,-0.370642202,-0.368807339,-0.366972477,
-0.365137615,-0.363302752,-0.36146789,-0.359633028,-0.357798165,-0.355963303,
-0.35412844,-0.352293578,-0.350458716,-0.348623853,-0.346788991,-0.344954128,
-0.343119266,-0.341284404,-0.339449541,-0.337614679,-0.335779817,-0.333944954,
-0.332110092,-0.330275229,-0.328440367,-0.326605505,-0.324770642,-0.32293578,
-0.321100917,-0.319266055,-0.317431193,-0.31559633,-0.313761468,-0.311926606,
-0.310091743,-0.308256881,-0.306422018,-0.304587156,-0.302752294,-0.300917431,
-0.299082569,-0.297247706,-0.295412844,-0.293577982,-0.291743119,-0.289908257,
-0.288073394,-0.286238532,-0.28440367,-0.282568807,-0.280733945,-0.278899083,
-0.27706422,-0.275229358,-0.273394495,-0.271559633,-0.269724771,-0.267889908,
-0.266055046,-0.264220183,-0.262385321,-0.260550459,-0.258715596,-0.256880734,
-0.255045872,-0.253211009,-0.251376147,-0.249541284,-0.247706422,-0.24587156,
-0.244036697,-0.242201835,-0.240366972,-0.23853211,-0.236697248,-0.234862385,
-0.233027523,-0.231192661,-0.229357798,-0.227522936,-0.225688073,-0.223853211,
-0.222018349,-0.220183486,-0.218348624,-0.216513761,-0.214678899,-0.212844037,
-0.211009174,-0.209174312,-0.20733945,-0.205504587,-0.203669725,-0.201834862,
-0.2,-0.198165138,-0.196330275,-0.194495413,-0.19266055,-0.190825688,-0.188990826,
-0.187155963,-0.185321101,-0.183486239,-0.181651376,-0.179816514,-0.177981651,
-0.176146789,-0.174311927,-0.172477064,-0.170642202,-0.168807339,-0.166972477,
-0.165137615,-0.163302752,-0.16146789,-0.159633028,-0.157798165,-0.155963303,
-0.15412844,-0.152293578,-0.150458716,-0.148623853,-0.146788991,-0.144954128,
-0.143172103),(0.,0.36),.UNSPECIFIED.);
#6258=B_SPLINE_SURFACE_WITH_KNOTS('',5,1,((#225453,#225454),(#225455,#225456),
(#225457,#225458),(#225459,#225460),(#225461,#225462),(#225463,#225464),
(#225465,#225466),(#225467,#225468),(#225469,#225470),(#225471,#225472),
(#225473,#225474),(#225475,#225476),(#225477,#225478),(#225479,#225480),
(#225481,#225482),(#225483,#225484),(#225485,#225486),(#225487,#225488),
(#225489,#225490),(#225491,#225492),(#225493,#225494),(#225495,#225496),
(#225497,#225498),(#225499,#225500),(#225501,#225502),(#225503,#225504),
(#225505,#225506),(#225507,#225508),(#225509,#225510),(#225511,#225512),
(#225513,#225514),(#225515,#225516),(#225517,#225518),(#225519,#225520),
(#225521,#225522),(#225523,#225524),(#225525,#225526),(#225527,#225528),
(#225529,#225530),(#225531,#225532),(#225533,#225534),(#225535,#225536),
(#225537,#225538),(#225539,#225540),(#225541,#225542),(#225543,#225544),
(#225545,#225546),(#225547,#225548),(#225549,#225550),(#225551,#225552),
(#225553,#225554),(#225555,#225556),(#225557,#225558),(#225559,#225560),
(#225561,#225562),(#225563,#225564),(#225565,#225566),(#225567,#225568),
(#225569,#225570),(#225571,#225572),(#225573,#225574),(#225575,#225576),
(#225577,#225578),(#225579,#225580),(#225581,#225582),(#225583,#225584),
(#225585,#225586),(#225587,#225588),(#225589,#225590),(#225591,#225592),
(#225593,#225594),(#225595,#225596),(#225597,#225598),(#225599,#225600),
(#225601,#225602),(#225603,#225604),(#225605,#225606),(#225607,#225608),
(#225609,#225610),(#225611,#225612),(#225613,#225614),(#225615,#225616),
(#225617,#225618),(#225619,#225620),(#225621,#225622),(#225623,#225624),
(#225625,#225626),(#225627,#225628),(#225629,#225630),(#225631,#225632),
(#225633,#225634),(#225635,#225636),(#225637,#225638),(#225639,#225640),
(#225641,#225642),(#225643,#225644),(#225645,#225646),(#225647,#225648),
(#225649,#225650),(#225651,#225652),(#225653,#225654),(#225655,#225656),
(#225657,#225658),(#225659,#225660),(#225661,#225662),(#225663,#225664),
(#225665,#225666),(#225667,#225668),(#225669,#225670),(#225671,#225672),
(#225673,#225674),(#225675,#225676),(#225677,#225678),(#225679,#225680),
(#225681,#225682),(#225683,#225684),(#225685,#225686),(#225687,#225688),
(#225689,#225690),(#225691,#225692),(#225693,#225694),(#225695,#225696),
(#225697,#225698),(#225699,#225700),(#225701,#225702),(#225703,#225704),
(#225705,#225706),(#225707,#225708),(#225709,#225710),(#225711,#225712),
(#225713,#225714),(#225715,#225716),(#225717,#225718),(#225719,#225720),
(#225721,#225722),(#225723,#225724),(#225725,#225726),(#225727,#225728),
(#225729,#225730),(#225731,#225732),(#225733,#225734),(#225735,#225736),
(#225737,#225738),(#225739,#225740),(#225741,#225742),(#225743,#225744),
(#225745,#225746),(#225747,#225748),(#225749,#225750),(#225751,#225752),
(#225753,#225754),(#225755,#225756),(#225757,#225758),(#225759,#225760),
(#225761,#225762),(#225763,#225764),(#225765,#225766),(#225767,#225768),
(#225769,#225770),(#225771,#225772),(#225773,#225774),(#225775,#225776),
(#225777,#225778),(#225779,#225780),(#225781,#225782),(#225783,#225784),
(#225785,#225786),(#225787,#225788),(#225789,#225790),(#225791,#225792),
(#225793,#225794),(#225795,#225796),(#225797,#225798),(#225799,#225800),
(#225801,#225802),(#225803,#225804),(#225805,#225806),(#225807,#225808),
(#225809,#225810),(#225811,#225812),(#225813,#225814),(#225815,#225816),
(#225817,#225818),(#225819,#225820),(#225821,#225822),(#225823,#225824),
(#225825,#225826),(#225827,#225828),(#225829,#225830),(#225831,#225832),
(#225833,#225834),(#225835,#225836),(#225837,#225838),(#225839,#225840),
(#225841,#225842),(#225843,#225844),(#225845,#225846),(#225847,#225848),
(#225849,#225850),(#225851,#225852),(#225853,#225854),(#225855,#225856),
(#225857,#225858),(#225859,#225860),(#225861,#225862),(#225863,#225864),
(#225865,#225866),(#225867,#225868),(#225869,#225870),(#225871,#225872),
(#225873,#225874),(#225875,#225876),(#225877,#225878),(#225879,#225880),
(#225881,#225882),(#225883,#225884),(#225885,#225886),(#225887,#225888),
(#225889,#225890),(#225891,#225892),(#225893,#225894),(#225895,#225896),
(#225897,#225898),(#225899,#225900),(#225901,#225902),(#225903,#225904),
(#225905,#225906),(#225907,#225908),(#225909,#225910),(#225911,#225912),
(#225913,#225914),(#225915,#225916),(#225917,#225918),(#225919,#225920),
(#225921,#225922),(#225923,#225924),(#225925,#225926),(#225927,#225928),
(#225929,#225930),(#225931,#225932),(#225933,#225934),(#225935,#225936),
(#225937,#225938),(#225939,#225940),(#225941,#225942),(#225943,#225944),
(#225945,#225946),(#225947,#225948),(#225949,#225950),(#225951,#225952),
(#225953,#225954),(#225955,#225956),(#225957,#225958),(#225959,#225960),
(#225961,#225962),(#225963,#225964),(#225965,#225966),(#225967,#225968),
(#225969,#225970),(#225971,#225972),(#225973,#225974),(#225975,#225976),
(#225977,#225978),(#225979,#225980),(#225981,#225982),(#225983,#225984),
(#225985,#225986),(#225987,#225988),(#225989,#225990),(#225991,#225992),
(#225993,#225994),(#225995,#225996),(#225997,#225998),(#225999,#226000),
(#226001,#226002),(#226003,#226004),(#226005,#226006),(#226007,#226008),
(#226009,#226010),(#226011,#226012),(#226013,#226014),(#226015,#226016),
(#226017,#226018),(#226019,#226020),(#226021,#226022),(#226023,#226024),
(#226025,#226026),(#226027,#226028),(#226029,#226030),(#226031,#226032),
(#226033,#226034),(#226035,#226036),(#226037,#226038),(#226039,#226040),
(#226041,#226042),(#226043,#226044),(#226045,#226046),(#226047,#226048),
(#226049,#226050),(#226051,#226052),(#226053,#226054),(#226055,#226056),
(#226057,#226058),(#226059,#226060),(#226061,#226062),(#226063,#226064),
(#226065,#226066),(#226067,#226068),(#226069,#226070),(#226071,#226072),
(#226073,#226074),(#226075,#226076),(#226077,#226078),(#226079,#226080),
(#226081,#226082),(#226083,#226084),(#226085,#226086),(#226087,#226088),
(#226089,#226090),(#226091,#226092),(#226093,#226094),(#226095,#226096),
(#226097,#226098),(#226099,#226100),(#226101,#226102),(#226103,#226104),
(#226105,#226106),(#226107,#226108),(#226109,#226110),(#226111,#226112),
(#226113,#226114),(#226115,#226116),(#226117,#226118),(#226119,#226120),
(#226121,#226122),(#226123,#226124),(#226125,#226126),(#226127,#226128),
(#226129,#226130),(#226131,#226132),(#226133,#226134),(#226135,#226136),
(#226137,#226138),(#226139,#226140),(#226141,#226142),(#226143,#226144),
(#226145,#226146),(#226147,#226148),(#226149,#226150),(#226151,#226152),
(#226153,#226154),(#226155,#226156),(#226157,#226158),(#226159,#226160),
(#226161,#226162),(#226163,#226164),(#226165,#226166),(#226167,#226168),
(#226169,#226170),(#226171,#226172),(#226173,#226174),(#226175,#226176),
(#226177,#226178),(#226179,#226180),(#226181,#226182),(#226183,#226184),
(#226185,#226186),(#226187,#226188),(#226189,#226190),(#226191,#226192),
(#226193,#226194),(#226195,#226196),(#226197,#226198),(#226199,#226200),
(#226201,#226202),(#226203,#226204),(#226205,#226206),(#226207,#226208),
(#226209,#226210),(#226211,#226212),(#226213,#226214),(#226215,#226216),
(#226217,#226218),(#226219,#226220),(#226221,#226222),(#226223,#226224),
(#226225,#226226),(#226227,#226228),(#226229,#226230),(#226231,#226232),
(#226233,#226234),(#226235,#226236),(#226237,#226238),(#226239,#226240),
(#226241,#226242),(#226243,#226244),(#226245,#226246),(#226247,#226248),
(#226249,#226250),(#226251,#226252),(#226253,#226254),(#226255,#226256),
(#226257,#226258),(#226259,#226260),(#226261,#226262),(#226263,#226264),
(#226265,#226266),(#226267,#226268),(#226269,#226270),(#226271,#226272),
(#226273,#226274),(#226275,#226276),(#226277,#226278),(#226279,#226280),
(#226281,#226282),(#226283,#226284),(#226285,#226286),(#226287,#226288),
(#226289,#226290),(#226291,#226292),(#226293,#226294),(#226295,#226296),
(#226297,#226298),(#226299,#226300),(#226301,#226302),(#226303,#226304),
(#226305,#226306),(#226307,#226308),(#226309,#226310),(#226311,#226312),
(#226313,#226314),(#226315,#226316),(#226317,#226318),(#226319,#226320),
(#226321,#226322),(#226323,#226324),(#226325,#226326),(#226327,#226328),
(#226329,#226330),(#226331,#226332),(#226333,#226334),(#226335,#226336),
(#226337,#226338),(#226339,#226340),(#226341,#226342),(#226343,#226344),
(#226345,#226346),(#226347,#226348),(#226349,#226350),(#226351,#226352),
(#226353,#226354),(#226355,#226356),(#226357,#226358),(#226359,#226360),
(#226361,#226362),(#226363,#226364),(#226365,#226366),(#226367,#226368),
(#226369,#226370),(#226371,#226372),(#226373,#226374),(#226375,#226376),
(#226377,#226378),(#226379,#226380),(#226381,#226382),(#226383,#226384),
(#226385,#226386),(#226387,#226388),(#226389,#226390),(#226391,#226392),
(#226393,#226394),(#226395,#226396)),.UNSPECIFIED.,.F.,.F.,.F.,(6,1,1,1,
1,1,1,1,1,1,1,1,1,1,1,1,1,1,1,1,1,1,1,1,1,1,1,1,1,1,1,1,1,1,1,1,1,1,1,1,
1,1,1,1,1,1,1,1,1,1,1,1,1,1,1,1,1,1,1,1,1,1,1,1,1,1,1,1,1,1,1,1,1,1,1,1,
1,1,1,1,1,1,1,1,1,1,1,1,1,1,1,1,1,1,1,1,1,1,1,1,1,1,1,1,1,1,1,1,1,1,1,1,
1,1,1,1,1,1,1,1,1,1,1,1,1,1,1,1,1,1,1,1,1,1,1,1,1,1,1,1,1,1,1,1,1,1,1,1,
1,1,1,1,1,1,1,1,1,1,1,1,1,1,1,1,1,1,1,1,1,1,1,1,1,1,1,1,1,1,1,1,1,1,1,1,
1,1,1,1,1,1,1,1,1,1,1,1,1,1,1,1,1,1,1,1,1,1,1,1,1,1,1,1,1,1,1,1,1,1,1,1,
1,1,1,1,1,1,1,1,1,1,1,1,1,1,1,1,1,1,1,1,1,1,1,1,1,1,1,1,1,1,1,1,1,1,1,1,
1,1,1,1,1,1,1,1,1,1,1,1,1,1,1,1,1,1,1,1,1,1,1,1,1,1,1,1,1,1,1,1,1,1,1,1,
1,1,1,1,1,1,1,1,1,1,1,1,1,1,1,1,1,1,1,1,1,1,1,1,1,1,1,1,1,1,1,1,1,1,1,1,
1,1,1,1,1,1,1,1,1,1,1,1,1,1,1,1,1,1,1,1,1,1,1,1,1,1,1,1,1,1,1,1,1,1,1,1,
1,1,1,1,1,1,1,1,1,1,1,1,1,1,1,1,1,1,1,1,1,1,1,1,1,1,1,1,1,1,1,1,1,1,1,1,
1,1,1,1,1,1,1,1,1,1,1,1,1,1,1,1,1,1,1,1,1,1,1,1,1,1,1,1,1,1,1,1,1,1,1,1,
1,1,1,1,1,1,1,1,1,1,1,1,1,1,1,1,1,1,1,1,1,1,1,1,1,1,1,1,1,1,1,6),(2,2),
(0.143172104,0.144954128,0.146788991,0.148623853,0.150458716,0.152293578,
0.15412844,0.155963303,0.157798165,0.159633028,0.16146789,0.163302752,0.165137615,
0.166972477,0.168807339,0.170642202,0.172477064,0.174311927,0.176146789,
0.177981651,0.179816514,0.181651376,0.183486239,0.185321101,0.187155963,
0.188990826,0.190825688,0.19266055,0.194495413,0.196330275,0.198165138,
0.2,0.201834862,0.203669725,0.205504587,0.20733945,0.209174312,0.211009174,
0.212844037,0.214678899,0.216513761,0.218348624,0.220183486,0.222018349,
0.223853211,0.225688073,0.227522936,0.229357798,0.231192661,0.233027523,
0.234862385,0.236697248,0.23853211,0.240366972,0.242201835,0.244036697,
0.24587156,0.247706422,0.249541284,0.251376147,0.253211009,0.255045872,
0.256880734,0.258715596,0.260550459,0.262385321,0.264220183,0.266055046,
0.267889908,0.269724771,0.271559633,0.273394495,0.275229358,0.27706422,
0.278899083,0.280733945,0.282568807,0.28440367,0.286238532,0.288073394,
0.289908257,0.291743119,0.293577982,0.295412844,0.297247706,0.299082569,
0.300917431,0.302752294,0.304587156,0.306422018,0.308256881,0.310091743,
0.311926606,0.313761468,0.31559633,0.317431193,0.319266055,0.321100917,
0.32293578,0.324770642,0.326605505,0.328440367,0.330275229,0.332110092,
0.333944954,0.335779817,0.337614679,0.339449541,0.341284404,0.343119266,
0.344954128,0.346788991,0.348623853,0.350458716,0.352293578,0.35412844,
0.355963303,0.357798165,0.359633028,0.36146789,0.363302752,0.365137615,
0.366972477,0.368807339,0.370642202,0.372477064,0.374311927,0.376146789,
0.377981651,0.379816514,0.381651376,0.383486239,0.385321101,0.387155963,
0.388990826,0.390825688,0.39266055,0.394495413,0.396330275,0.398165138,
0.4,0.401834862,0.403669725,0.405504587,0.40733945,0.409174312,0.411009174,
0.412844037,0.414678899,0.416513761,0.418348624,0.420183486,0.422018349,
0.423853211,0.425688073,0.427522936,0.429357798,0.431192661,0.433027523,
0.434862385,0.436697248,0.43853211,0.440366972,0.442201835,0.444036697,
0.44587156,0.447706422,0.449541284,0.451376147,0.453211009,0.455045872,
0.456880734,0.458715596,0.460550459,0.462385321,0.464220183,0.466055046,
0.467889908,0.469724771,0.471559633,0.473394495,0.475229358,0.47706422,
0.478899083,0.480733945,0.482568807,0.48440367,0.486238532,0.488073394,
0.489908257,0.491743119,0.493577982,0.495412844,0.497247706,0.499082569,
0.500917431,0.502752294,0.504587156,0.506422018,0.508256881,0.510091743,
0.511926606,0.513761468,0.51559633,0.517431193,0.519266055,0.521100917,
0.52293578,0.524770642,0.526605505,0.528440367,0.530275229,0.532110092,
0.533944954,0.535779817,0.537614679,0.539449541,0.541284404,0.543119266,
0.544954128,0.546788991,0.548623853,0.550458716,0.552293578,0.55412844,
0.555963303,0.557798165,0.559633028,0.56146789,0.563302752,0.565137615,
0.566972477,0.568807339,0.570642202,0.572477064,0.574311927,0.576146789,
0.577981651,0.579816514,0.581651376,0.583486239,0.585321101,0.587155963,
0.588990826,0.590825688,0.59266055,0.594495413,0.596330275,0.598165138,
0.6,0.601834862,0.603669725,0.605504587,0.60733945,0.609174312,0.611009174,
0.612844037,0.614678899,0.616513761,0.618348624,0.620183486,0.622018349,
0.623853211,0.625688073,0.627522936,0.629357798,0.631192661,0.633027523,
0.634862385,0.636697248,0.63853211,0.640366972,0.642201835,0.644036697,
0.64587156,0.647706422,0.649541284,0.651376147,0.653211009,0.655045872,
0.656880734,0.658715596,0.660550459,0.662385321,0.664220183,0.666055046,
0.667889908,0.669724771,0.671559633,0.673394495,0.675229358,0.67706422,
0.678899083,0.680733945,0.682568807,0.68440367,0.686238532,0.688073394,
0.689908257,0.691743119,0.693577982,0.695412844,0.697247706,0.699082569,
0.700917431,0.702752294,0.704587156,0.706422018,0.708256881,0.710091743,
0.711926606,0.713761468,0.71559633,0.717431193,0.719266055,0.721100917,
0.72293578,0.724770642,0.726605505,0.728440367,0.730275229,0.732110092,
0.733944954,0.735779817,0.737614679,0.739449541,0.741284404,0.743119266,
0.744954128,0.746788991,0.748623853,0.750458716,0.752293578,0.75412844,
0.755963303,0.757798165,0.759633028,0.76146789,0.763302752,0.765137615,
0.766972477,0.768807339,0.770642202,0.772477064,0.774311927,0.776146789,
0.777981651,0.779816514,0.781651376,0.783486239,0.785321101,0.787155963,
0.788990826,0.790825688,0.79266055,0.794495413,0.796330275,0.798165138,
0.8,0.801834862,0.803669725,0.805504587,0.80733945,0.809174312,0.811009174,
0.812844037,0.814678899,0.816513761,0.818348624,0.820183486,0.822018349,
0.823853211,0.825688073,0.827522936,0.829357798,0.831192661,0.833027523,
0.834862385,0.836697248,0.83853211,0.840366972,0.842201835,0.844036697,
0.84587156,0.847706422,0.849541284,0.851376147,0.853211009,0.855045872,
0.856880734,0.858715596,0.860550459,0.862385321,0.864220183,0.866055046,
0.867889908,0.869724771,0.871559633,0.873394495,0.875229358,0.87706422,
0.878899083,0.880733945,0.882568807,0.88440367,0.886238532,0.888073394,
0.889908257,0.891743119,0.893577982,0.895412844,0.897247706,0.899082569,
0.900917431,0.902752294,0.904587156,0.906422018,0.908256881,0.910091743,
0.911926606,0.913761468,0.91559633,0.917431193,0.919266055,0.921100917,
0.92293578,0.924770642,0.926605505,0.928440367,0.930275229,0.932110092,
0.933944954,0.935779817,0.937614679,0.939449541,0.941284404,0.943119266,
0.944954128,0.946788991,0.948623853,0.950458716,0.952293578,0.95412844,
0.955963303,0.957798165,0.959633028,0.96146789,0.963302752,0.965137615,
0.966972477,0.968807339,0.970642202,0.972477064,0.974311927,0.976146789,
0.977981651,0.979816514,0.981651376,0.983486239,0.985321101,0.987155963,
0.988990826,0.990825688,0.99266055,0.994495413,0.996330275,0.998165138,
1.),(0.,0.36),.UNSPECIFIED.);
#6259=B_SPLINE_SURFACE_WITH_KNOTS('',5,1,((#227008,#227009),(#227010,#227011),
(#227012,#227013),(#227014,#227015),(#227016,#227017),(#227018,#227019),
(#227020,#227021),(#227022,#227023),(#227024,#227025),(#227026,#227027),
(#227028,#227029),(#227030,#227031),(#227032,#227033),(#227034,#227035),
(#227036,#227037),(#227038,#227039),(#227040,#227041),(#227042,#227043),
(#227044,#227045),(#227046,#227047),(#227048,#227049),(#227050,#227051),
(#227052,#227053),(#227054,#227055),(#227056,#227057),(#227058,#227059),
(#227060,#227061),(#227062,#227063),(#227064,#227065),(#227066,#227067),
(#227068,#227069),(#227070,#227071),(#227072,#227073),(#227074,#227075),
(#227076,#227077),(#227078,#227079),(#227080,#227081),(#227082,#227083),
(#227084,#227085),(#227086,#227087),(#227088,#227089),(#227090,#227091),
(#227092,#227093),(#227094,#227095),(#227096,#227097),(#227098,#227099),
(#227100,#227101),(#227102,#227103),(#227104,#227105),(#227106,#227107),
(#227108,#227109),(#227110,#227111),(#227112,#227113),(#227114,#227115),
(#227116,#227117),(#227118,#227119),(#227120,#227121),(#227122,#227123),
(#227124,#227125),(#227126,#227127),(#227128,#227129),(#227130,#227131),
(#227132,#227133),(#227134,#227135),(#227136,#227137),(#227138,#227139),
(#227140,#227141),(#227142,#227143),(#227144,#227145),(#227146,#227147),
(#227148,#227149),(#227150,#227151),(#227152,#227153),(#227154,#227155),
(#227156,#227157),(#227158,#227159),(#227160,#227161),(#227162,#227163),
(#227164,#227165),(#227166,#227167),(#227168,#227169),(#227170,#227171),
(#227172,#227173),(#227174,#227175),(#227176,#227177),(#227178,#227179),
(#227180,#227181),(#227182,#227183),(#227184,#227185),(#227186,#227187),
(#227188,#227189),(#227190,#227191),(#227192,#227193),(#227194,#227195),
(#227196,#227197),(#227198,#227199),(#227200,#227201),(#227202,#227203),
(#227204,#227205),(#227206,#227207),(#227208,#227209),(#227210,#227211),
(#227212,#227213),(#227214,#227215),(#227216,#227217),(#227218,#227219),
(#227220,#227221),(#227222,#227223),(#227224,#227225),(#227226,#227227),
(#227228,#227229),(#227230,#227231),(#227232,#227233),(#227234,#227235),
(#227236,#227237),(#227238,#227239),(#227240,#227241),(#227242,#227243),
(#227244,#227245),(#227246,#227247),(#227248,#227249),(#227250,#227251),
(#227252,#227253),(#227254,#227255),(#227256,#227257),(#227258,#227259),
(#227260,#227261),(#227262,#227263),(#227264,#227265),(#227266,#227267),
(#227268,#227269),(#227270,#227271),(#227272,#227273),(#227274,#227275),
(#227276,#227277),(#227278,#227279),(#227280,#227281),(#227282,#227283),
(#227284,#227285),(#227286,#227287),(#227288,#227289),(#227290,#227291),
(#227292,#227293),(#227294,#227295),(#227296,#227297),(#227298,#227299),
(#227300,#227301),(#227302,#227303),(#227304,#227305),(#227306,#227307),
(#227308,#227309),(#227310,#227311),(#227312,#227313),(#227314,#227315),
(#227316,#227317),(#227318,#227319),(#227320,#227321),(#227322,#227323),
(#227324,#227325),(#227326,#227327),(#227328,#227329),(#227330,#227331),
(#227332,#227333),(#227334,#227335),(#227336,#227337),(#227338,#227339),
(#227340,#227341),(#227342,#227343),(#227344,#227345),(#227346,#227347),
(#227348,#227349),(#227350,#227351),(#227352,#227353),(#227354,#227355),
(#227356,#227357),(#227358,#227359),(#227360,#227361),(#227362,#227363),
(#227364,#227365),(#227366,#227367),(#227368,#227369),(#227370,#227371),
(#227372,#227373),(#227374,#227375),(#227376,#227377),(#227378,#227379),
(#227380,#227381),(#227382,#227383),(#227384,#227385),(#227386,#227387),
(#227388,#227389),(#227390,#227391),(#227392,#227393),(#227394,#227395),
(#227396,#227397),(#227398,#227399),(#227400,#227401),(#227402,#227403),
(#227404,#227405),(#227406,#227407),(#227408,#227409),(#227410,#227411),
(#227412,#227413),(#227414,#227415),(#227416,#227417),(#227418,#227419),
(#227420,#227421),(#227422,#227423),(#227424,#227425),(#227426,#227427),
(#227428,#227429),(#227430,#227431),(#227432,#227433),(#227434,#227435),
(#227436,#227437),(#227438,#227439),(#227440,#227441),(#227442,#227443),
(#227444,#227445),(#227446,#227447),(#227448,#227449),(#227450,#227451),
(#227452,#227453),(#227454,#227455),(#227456,#227457),(#227458,#227459),
(#227460,#227461),(#227462,#227463),(#227464,#227465),(#227466,#227467),
(#227468,#227469),(#227470,#227471),(#227472,#227473),(#227474,#227475),
(#227476,#227477),(#227478,#227479),(#227480,#227481),(#227482,#227483),
(#227484,#227485),(#227486,#227487),(#227488,#227489),(#227490,#227491),
(#227492,#227493),(#227494,#227495),(#227496,#227497),(#227498,#227499),
(#227500,#227501),(#227502,#227503),(#227504,#227505),(#227506,#227507),
(#227508,#227509),(#227510,#227511),(#227512,#227513),(#227514,#227515),
(#227516,#227517),(#227518,#227519),(#227520,#227521),(#227522,#227523),
(#227524,#227525),(#227526,#227527),(#227528,#227529),(#227530,#227531),
(#227532,#227533),(#227534,#227535),(#227536,#227537),(#227538,#227539),
(#227540,#227541),(#227542,#227543),(#227544,#227545),(#227546,#227547),
(#227548,#227549),(#227550,#227551),(#227552,#227553),(#227554,#227555),
(#227556,#227557),(#227558,#227559),(#227560,#227561),(#227562,#227563),
(#227564,#227565),(#227566,#227567),(#227568,#227569),(#227570,#227571),
(#227572,#227573),(#227574,#227575),(#227576,#227577),(#227578,#227579),
(#227580,#227581),(#227582,#227583),(#227584,#227585),(#227586,#227587),
(#227588,#227589),(#227590,#227591),(#227592,#227593),(#227594,#227595),
(#227596,#227597),(#227598,#227599),(#227600,#227601),(#227602,#227603),
(#227604,#227605),(#227606,#227607),(#227608,#227609),(#227610,#227611),
(#227612,#227613),(#227614,#227615),(#227616,#227617),(#227618,#227619),
(#227620,#227621),(#227622,#227623),(#227624,#227625),(#227626,#227627),
(#227628,#227629),(#227630,#227631),(#227632,#227633),(#227634,#227635),
(#227636,#227637),(#227638,#227639),(#227640,#227641),(#227642,#227643),
(#227644,#227645),(#227646,#227647),(#227648,#227649),(#227650,#227651),
(#227652,#227653),(#227654,#227655),(#227656,#227657),(#227658,#227659),
(#227660,#227661),(#227662,#227663),(#227664,#227665),(#227666,#227667),
(#227668,#227669),(#227670,#227671),(#227672,#227673),(#227674,#227675),
(#227676,#227677),(#227678,#227679),(#227680,#227681),(#227682,#227683),
(#227684,#227685),(#227686,#227687),(#227688,#227689),(#227690,#227691),
(#227692,#227693),(#227694,#227695),(#227696,#227697),(#227698,#227699),
(#227700,#227701),(#227702,#227703),(#227704,#227705),(#227706,#227707),
(#227708,#227709),(#227710,#227711),(#227712,#227713),(#227714,#227715),
(#227716,#227717),(#227718,#227719),(#227720,#227721),(#227722,#227723),
(#227724,#227725),(#227726,#227727),(#227728,#227729),(#227730,#227731),
(#227732,#227733),(#227734,#227735),(#227736,#227737),(#227738,#227739),
(#227740,#227741),(#227742,#227743),(#227744,#227745),(#227746,#227747),
(#227748,#227749),(#227750,#227751),(#227752,#227753),(#227754,#227755),
(#227756,#227757),(#227758,#227759),(#227760,#227761),(#227762,#227763),
(#227764,#227765),(#227766,#227767),(#227768,#227769),(#227770,#227771),
(#227772,#227773),(#227774,#227775),(#227776,#227777),(#227778,#227779),
(#227780,#227781),(#227782,#227783),(#227784,#227785),(#227786,#227787),
(#227788,#227789),(#227790,#227791),(#227792,#227793),(#227794,#227795),
(#227796,#227797),(#227798,#227799),(#227800,#227801),(#227802,#227803),
(#227804,#227805),(#227806,#227807),(#227808,#227809),(#227810,#227811),
(#227812,#227813),(#227814,#227815),(#227816,#227817),(#227818,#227819),
(#227820,#227821),(#227822,#227823),(#227824,#227825),(#227826,#227827),
(#227828,#227829),(#227830,#227831),(#227832,#227833),(#227834,#227835),
(#227836,#227837),(#227838,#227839),(#227840,#227841),(#227842,#227843),
(#227844,#227845),(#227846,#227847),(#227848,#227849),(#227850,#227851),
(#227852,#227853),(#227854,#227855),(#227856,#227857),(#227858,#227859),
(#227860,#227861),(#227862,#227863),(#227864,#227865),(#227866,#227867),
(#227868,#227869),(#227870,#227871),(#227872,#227873),(#227874,#227875),
(#227876,#227877),(#227878,#227879),(#227880,#227881),(#227882,#227883),
(#227884,#227885),(#227886,#227887),(#227888,#227889),(#227890,#227891),
(#227892,#227893),(#227894,#227895),(#227896,#227897),(#227898,#227899),
(#227900,#227901),(#227902,#227903),(#227904,#227905),(#227906,#227907),
(#227908,#227909),(#227910,#227911),(#227912,#227913),(#227914,#227915),
(#227916,#227917),(#227918,#227919),(#227920,#227921),(#227922,#227923),
(#227924,#227925),(#227926,#227927),(#227928,#227929),(#227930,#227931),
(#227932,#227933),(#227934,#227935),(#227936,#227937),(#227938,#227939),
(#227940,#227941),(#227942,#227943),(#227944,#227945),(#227946,#227947),
(#227948,#227949),(#227950,#227951)),.UNSPECIFIED.,.F.,.F.,.F.,(6,1,1,1,
1,1,1,1,1,1,1,1,1,1,1,1,1,1,1,1,1,1,1,1,1,1,1,1,1,1,1,1,1,1,1,1,1,1,1,1,
1,1,1,1,1,1,1,1,1,1,1,1,1,1,1,1,1,1,1,1,1,1,1,1,1,1,1,1,1,1,1,1,1,1,1,1,
1,1,1,1,1,1,1,1,1,1,1,1,1,1,1,1,1,1,1,1,1,1,1,1,1,1,1,1,1,1,1,1,1,1,1,1,
1,1,1,1,1,1,1,1,1,1,1,1,1,1,1,1,1,1,1,1,1,1,1,1,1,1,1,1,1,1,1,1,1,1,1,1,
1,1,1,1,1,1,1,1,1,1,1,1,1,1,1,1,1,1,1,1,1,1,1,1,1,1,1,1,1,1,1,1,1,1,1,1,
1,1,1,1,1,1,1,1,1,1,1,1,1,1,1,1,1,1,1,1,1,1,1,1,1,1,1,1,1,1,1,1,1,1,1,1,
1,1,1,1,1,1,1,1,1,1,1,1,1,1,1,1,1,1,1,1,1,1,1,1,1,1,1,1,1,1,1,1,1,1,1,1,
1,1,1,1,1,1,1,1,1,1,1,1,1,1,1,1,1,1,1,1,1,1,1,1,1,1,1,1,1,1,1,1,1,1,1,1,
1,1,1,1,1,1,1,1,1,1,1,1,1,1,1,1,1,1,1,1,1,1,1,1,1,1,1,1,1,1,1,1,1,1,1,1,
1,1,1,1,1,1,1,1,1,1,1,1,1,1,1,1,1,1,1,1,1,1,1,1,1,1,1,1,1,1,1,1,1,1,1,1,
1,1,1,1,1,1,1,1,1,1,1,1,1,1,1,1,1,1,1,1,1,1,1,1,1,1,1,1,1,1,1,1,1,1,1,1,
1,1,1,1,1,1,1,1,1,1,1,1,1,1,1,1,1,1,1,1,1,1,1,1,1,1,1,1,1,1,1,1,1,1,1,1,
1,1,1,1,1,1,1,1,1,1,1,1,1,1,1,1,1,1,1,1,1,1,1,1,1,1,1,1,1,1,1,6),(2,2),
(0.143172103,0.144954128,0.146788991,0.148623853,0.150458716,0.152293578,
0.15412844,0.155963303,0.157798165,0.159633028,0.16146789,0.163302752,0.165137615,
0.166972477,0.168807339,0.170642202,0.172477064,0.174311927,0.176146789,
0.177981651,0.179816514,0.181651376,0.183486239,0.185321101,0.187155963,
0.188990826,0.190825688,0.19266055,0.194495413,0.196330275,0.198165138,
0.2,0.201834862,0.203669725,0.205504587,0.20733945,0.209174312,0.211009174,
0.212844037,0.214678899,0.216513761,0.218348624,0.220183486,0.222018349,
0.223853211,0.225688073,0.227522936,0.229357798,0.231192661,0.233027523,
0.234862385,0.236697248,0.23853211,0.240366972,0.242201835,0.244036697,
0.24587156,0.247706422,0.249541284,0.251376147,0.253211009,0.255045872,
0.256880734,0.258715596,0.260550459,0.262385321,0.264220183,0.266055046,
0.267889908,0.269724771,0.271559633,0.273394495,0.275229358,0.27706422,
0.278899083,0.280733945,0.282568807,0.28440367,0.286238532,0.288073394,
0.289908257,0.291743119,0.293577982,0.295412844,0.297247706,0.299082569,
0.300917431,0.302752294,0.304587156,0.306422018,0.308256881,0.310091743,
0.311926606,0.313761468,0.31559633,0.317431193,0.319266055,0.321100917,
0.32293578,0.324770642,0.326605505,0.328440367,0.330275229,0.332110092,
0.333944954,0.335779817,0.337614679,0.339449541,0.341284404,0.343119266,
0.344954128,0.346788991,0.348623853,0.350458716,0.352293578,0.35412844,
0.355963303,0.357798165,0.359633028,0.36146789,0.363302752,0.365137615,
0.366972477,0.368807339,0.370642202,0.372477064,0.374311927,0.376146789,
0.377981651,0.379816514,0.381651376,0.383486239,0.385321101,0.387155963,
0.388990826,0.390825688,0.39266055,0.394495413,0.396330275,0.398165138,
0.4,0.401834862,0.403669725,0.405504587,0.40733945,0.409174312,0.411009174,
0.412844037,0.414678899,0.416513761,0.418348624,0.420183486,0.422018349,
0.423853211,0.425688073,0.427522936,0.429357798,0.431192661,0.433027523,
0.434862385,0.436697248,0.43853211,0.440366972,0.442201835,0.444036697,
0.44587156,0.447706422,0.449541284,0.451376147,0.453211009,0.455045872,
0.456880734,0.458715596,0.460550459,0.462385321,0.464220183,0.466055046,
0.467889908,0.469724771,0.471559633,0.473394495,0.475229358,0.47706422,
0.478899083,0.480733945,0.482568807,0.48440367,0.486238532,0.488073394,
0.489908257,0.491743119,0.493577982,0.495412844,0.497247706,0.499082569,
0.500917431,0.502752294,0.504587156,0.506422018,0.508256881,0.510091743,
0.511926606,0.513761468,0.51559633,0.517431193,0.519266055,0.521100917,
0.52293578,0.524770642,0.526605505,0.528440367,0.530275229,0.532110092,
0.533944954,0.535779817,0.537614679,0.539449541,0.541284404,0.543119266,
0.544954128,0.546788991,0.548623853,0.550458716,0.552293578,0.55412844,
0.555963303,0.557798165,0.559633028,0.56146789,0.563302752,0.565137615,
0.566972477,0.568807339,0.570642202,0.572477064,0.574311927,0.576146789,
0.577981651,0.579816514,0.581651376,0.583486239,0.585321101,0.587155963,
0.588990826,0.590825688,0.59266055,0.594495413,0.596330275,0.598165138,
0.6,0.601834862,0.603669725,0.605504587,0.60733945,0.609174312,0.611009174,
0.612844037,0.614678899,0.616513761,0.618348624,0.620183486,0.622018349,
0.623853211,0.625688073,0.627522936,0.629357798,0.631192661,0.633027523,
0.634862385,0.636697248,0.63853211,0.640366972,0.642201835,0.644036697,
0.64587156,0.647706422,0.649541284,0.651376147,0.653211009,0.655045872,
0.656880734,0.658715596,0.660550459,0.662385321,0.664220183,0.666055046,
0.667889908,0.669724771,0.671559633,0.673394495,0.675229358,0.67706422,
0.678899083,0.680733945,0.682568807,0.68440367,0.686238532,0.688073394,
0.689908257,0.691743119,0.693577982,0.695412844,0.697247706,0.699082569,
0.700917431,0.702752294,0.704587156,0.706422018,0.708256881,0.710091743,
0.711926606,0.713761468,0.71559633,0.717431193,0.719266055,0.721100917,
0.72293578,0.724770642,0.726605505,0.728440367,0.730275229,0.732110092,
0.733944954,0.735779817,0.737614679,0.739449541,0.741284404,0.743119266,
0.744954128,0.746788991,0.748623853,0.750458716,0.752293578,0.75412844,
0.755963303,0.757798165,0.759633028,0.76146789,0.763302752,0.765137615,
0.766972477,0.768807339,0.770642202,0.772477064,0.774311927,0.776146789,
0.777981651,0.779816514,0.781651376,0.783486239,0.785321101,0.787155963,
0.788990826,0.790825688,0.79266055,0.794495413,0.796330275,0.798165138,
0.8,0.801834862,0.803669725,0.805504587,0.80733945,0.809174312,0.811009174,
0.812844037,0.814678899,0.816513761,0.818348624,0.820183486,0.822018349,
0.823853211,0.825688073,0.827522936,0.829357798,0.831192661,0.833027523,
0.834862385,0.836697248,0.83853211,0.840366972,0.842201835,0.844036697,
0.84587156,0.847706422,0.849541284,0.851376147,0.853211009,0.855045872,
0.856880734,0.858715596,0.860550459,0.862385321,0.864220183,0.866055046,
0.867889908,0.869724771,0.871559633,0.873394495,0.875229358,0.87706422,
0.878899083,0.880733945,0.882568807,0.88440367,0.886238532,0.888073394,
0.889908257,0.891743119,0.893577982,0.895412844,0.897247706,0.899082569,
0.900917431,0.902752294,0.904587156,0.906422018,0.908256881,0.910091743,
0.911926606,0.913761468,0.91559633,0.917431193,0.919266055,0.921100917,
0.92293578,0.924770642,0.926605505,0.928440367,0.930275229,0.932110092,
0.933944954,0.935779817,0.937614679,0.939449541,0.941284404,0.943119266,
0.944954128,0.946788991,0.948623853,0.950458716,0.952293578,0.95412844,
0.955963303,0.957798165,0.959633028,0.96146789,0.963302752,0.965137615,
0.966972477,0.968807339,0.970642202,0.972477064,0.974311927,0.976146789,
0.977981651,0.979816514,0.981651376,0.983486239,0.985321101,0.987155963,
0.988990826,0.990825688,0.99266055,0.994495413,0.996330275,0.998165138,
1.),(0.,0.36),.UNSPECIFIED.);
#6260=B_SPLINE_SURFACE_WITH_KNOTS('',5,1,((#228575,#228576),(#228577,#228578),
(#228579,#228580),(#228581,#228582),(#228583,#228584),(#228585,#228586),
(#228587,#228588),(#228589,#228590),(#228591,#228592),(#228593,#228594),
(#228595,#228596),(#228597,#228598),(#228599,#228600),(#228601,#228602),
(#228603,#228604),(#228605,#228606),(#228607,#228608),(#228609,#228610),
(#228611,#228612),(#228613,#228614),(#228615,#228616),(#228617,#228618),
(#228619,#228620),(#228621,#228622),(#228623,#228624),(#228625,#228626),
(#228627,#228628),(#228629,#228630),(#228631,#228632),(#228633,#228634),
(#228635,#228636),(#228637,#228638),(#228639,#228640),(#228641,#228642),
(#228643,#228644),(#228645,#228646),(#228647,#228648),(#228649,#228650),
(#228651,#228652),(#228653,#228654),(#228655,#228656),(#228657,#228658),
(#228659,#228660),(#228661,#228662),(#228663,#228664),(#228665,#228666),
(#228667,#228668),(#228669,#228670),(#228671,#228672),(#228673,#228674),
(#228675,#228676),(#228677,#228678),(#228679,#228680),(#228681,#228682),
(#228683,#228684),(#228685,#228686),(#228687,#228688),(#228689,#228690),
(#228691,#228692),(#228693,#228694),(#228695,#228696),(#228697,#228698),
(#228699,#228700),(#228701,#228702),(#228703,#228704),(#228705,#228706),
(#228707,#228708),(#228709,#228710),(#228711,#228712),(#228713,#228714),
(#228715,#228716),(#228717,#228718),(#228719,#228720),(#228721,#228722),
(#228723,#228724),(#228725,#228726),(#228727,#228728),(#228729,#228730),
(#228731,#228732),(#228733,#228734),(#228735,#228736),(#228737,#228738),
(#228739,#228740),(#228741,#228742),(#228743,#228744),(#228745,#228746),
(#228747,#228748),(#228749,#228750),(#228751,#228752),(#228753,#228754),
(#228755,#228756),(#228757,#228758),(#228759,#228760),(#228761,#228762),
(#228763,#228764),(#228765,#228766),(#228767,#228768),(#228769,#228770),
(#228771,#228772),(#228773,#228774),(#228775,#228776),(#228777,#228778),
(#228779,#228780),(#228781,#228782),(#228783,#228784),(#228785,#228786),
(#228787,#228788),(#228789,#228790),(#228791,#228792),(#228793,#228794),
(#228795,#228796),(#228797,#228798),(#228799,#228800),(#228801,#228802),
(#228803,#228804),(#228805,#228806),(#228807,#228808),(#228809,#228810),
(#228811,#228812),(#228813,#228814),(#228815,#228816),(#228817,#228818),
(#228819,#228820),(#228821,#228822),(#228823,#228824),(#228825,#228826),
(#228827,#228828),(#228829,#228830),(#228831,#228832),(#228833,#228834),
(#228835,#228836),(#228837,#228838),(#228839,#228840),(#228841,#228842),
(#228843,#228844),(#228845,#228846),(#228847,#228848),(#228849,#228850),
(#228851,#228852),(#228853,#228854),(#228855,#228856),(#228857,#228858),
(#228859,#228860),(#228861,#228862),(#228863,#228864),(#228865,#228866),
(#228867,#228868),(#228869,#228870),(#228871,#228872),(#228873,#228874),
(#228875,#228876),(#228877,#228878),(#228879,#228880),(#228881,#228882),
(#228883,#228884),(#228885,#228886),(#228887,#228888),(#228889,#228890),
(#228891,#228892),(#228893,#228894),(#228895,#228896),(#228897,#228898),
(#228899,#228900),(#228901,#228902),(#228903,#228904),(#228905,#228906),
(#228907,#228908),(#228909,#228910),(#228911,#228912),(#228913,#228914),
(#228915,#228916),(#228917,#228918),(#228919,#228920),(#228921,#228922),
(#228923,#228924),(#228925,#228926),(#228927,#228928),(#228929,#228930),
(#228931,#228932),(#228933,#228934),(#228935,#228936),(#228937,#228938),
(#228939,#228940),(#228941,#228942),(#228943,#228944),(#228945,#228946),
(#228947,#228948),(#228949,#228950),(#228951,#228952),(#228953,#228954),
(#228955,#228956),(#228957,#228958),(#228959,#228960),(#228961,#228962),
(#228963,#228964),(#228965,#228966),(#228967,#228968),(#228969,#228970),
(#228971,#228972),(#228973,#228974),(#228975,#228976),(#228977,#228978),
(#228979,#228980),(#228981,#228982),(#228983,#228984),(#228985,#228986),
(#228987,#228988),(#228989,#228990),(#228991,#228992),(#228993,#228994),
(#228995,#228996),(#228997,#228998),(#228999,#229000),(#229001,#229002),
(#229003,#229004),(#229005,#229006),(#229007,#229008),(#229009,#229010),
(#229011,#229012),(#229013,#229014),(#229015,#229016),(#229017,#229018),
(#229019,#229020),(#229021,#229022),(#229023,#229024),(#229025,#229026),
(#229027,#229028),(#229029,#229030),(#229031,#229032),(#229033,#229034),
(#229035,#229036),(#229037,#229038),(#229039,#229040),(#229041,#229042),
(#229043,#229044),(#229045,#229046),(#229047,#229048),(#229049,#229050),
(#229051,#229052),(#229053,#229054),(#229055,#229056),(#229057,#229058),
(#229059,#229060),(#229061,#229062),(#229063,#229064),(#229065,#229066),
(#229067,#229068),(#229069,#229070),(#229071,#229072),(#229073,#229074),
(#229075,#229076),(#229077,#229078),(#229079,#229080),(#229081,#229082),
(#229083,#229084),(#229085,#229086),(#229087,#229088),(#229089,#229090),
(#229091,#229092),(#229093,#229094),(#229095,#229096),(#229097,#229098),
(#229099,#229100),(#229101,#229102),(#229103,#229104),(#229105,#229106),
(#229107,#229108),(#229109,#229110),(#229111,#229112),(#229113,#229114),
(#229115,#229116),(#229117,#229118),(#229119,#229120),(#229121,#229122),
(#229123,#229124),(#229125,#229126),(#229127,#229128),(#229129,#229130),
(#229131,#229132),(#229133,#229134),(#229135,#229136),(#229137,#229138),
(#229139,#229140),(#229141,#229142),(#229143,#229144),(#229145,#229146),
(#229147,#229148),(#229149,#229150),(#229151,#229152),(#229153,#229154),
(#229155,#229156),(#229157,#229158),(#229159,#229160),(#229161,#229162),
(#229163,#229164),(#229165,#229166),(#229167,#229168),(#229169,#229170),
(#229171,#229172),(#229173,#229174),(#229175,#229176),(#229177,#229178),
(#229179,#229180),(#229181,#229182),(#229183,#229184),(#229185,#229186),
(#229187,#229188),(#229189,#229190),(#229191,#229192),(#229193,#229194),
(#229195,#229196),(#229197,#229198),(#229199,#229200),(#229201,#229202),
(#229203,#229204),(#229205,#229206),(#229207,#229208),(#229209,#229210),
(#229211,#229212),(#229213,#229214),(#229215,#229216),(#229217,#229218),
(#229219,#229220),(#229221,#229222),(#229223,#229224),(#229225,#229226),
(#229227,#229228),(#229229,#229230),(#229231,#229232),(#229233,#229234),
(#229235,#229236),(#229237,#229238),(#229239,#229240),(#229241,#229242),
(#229243,#229244),(#229245,#229246),(#229247,#229248),(#229249,#229250),
(#229251,#229252),(#229253,#229254),(#229255,#229256),(#229257,#229258),
(#229259,#229260),(#229261,#229262),(#229263,#229264),(#229265,#229266),
(#229267,#229268),(#229269,#229270),(#229271,#229272),(#229273,#229274),
(#229275,#229276),(#229277,#229278),(#229279,#229280),(#229281,#229282),
(#229283,#229284),(#229285,#229286),(#229287,#229288),(#229289,#229290),
(#229291,#229292),(#229293,#229294),(#229295,#229296),(#229297,#229298),
(#229299,#229300),(#229301,#229302),(#229303,#229304),(#229305,#229306),
(#229307,#229308),(#229309,#229310),(#229311,#229312),(#229313,#229314),
(#229315,#229316),(#229317,#229318),(#229319,#229320),(#229321,#229322),
(#229323,#229324),(#229325,#229326),(#229327,#229328),(#229329,#229330),
(#229331,#229332),(#229333,#229334),(#229335,#229336),(#229337,#229338),
(#229339,#229340),(#229341,#229342),(#229343,#229344),(#229345,#229346),
(#229347,#229348),(#229349,#229350),(#229351,#229352),(#229353,#229354),
(#229355,#229356),(#229357,#229358),(#229359,#229360),(#229361,#229362),
(#229363,#229364),(#229365,#229366),(#229367,#229368),(#229369,#229370),
(#229371,#229372),(#229373,#229374),(#229375,#229376),(#229377,#229378),
(#229379,#229380),(#229381,#229382),(#229383,#229384),(#229385,#229386),
(#229387,#229388),(#229389,#229390),(#229391,#229392),(#229393,#229394),
(#229395,#229396),(#229397,#229398),(#229399,#229400),(#229401,#229402),
(#229403,#229404),(#229405,#229406),(#229407,#229408),(#229409,#229410),
(#229411,#229412),(#229413,#229414),(#229415,#229416),(#229417,#229418),
(#229419,#229420),(#229421,#229422),(#229423,#229424),(#229425,#229426),
(#229427,#229428),(#229429,#229430),(#229431,#229432),(#229433,#229434),
(#229435,#229436),(#229437,#229438),(#229439,#229440),(#229441,#229442),
(#229443,#229444),(#229445,#229446),(#229447,#229448),(#229449,#229450),
(#229451,#229452),(#229453,#229454),(#229455,#229456),(#229457,#229458),
(#229459,#229460),(#229461,#229462),(#229463,#229464),(#229465,#229466),
(#229467,#229468),(#229469,#229470),(#229471,#229472),(#229473,#229474),
(#229475,#229476),(#229477,#229478),(#229479,#229480),(#229481,#229482),
(#229483,#229484),(#229485,#229486),(#229487,#229488),(#229489,#229490),
(#229491,#229492),(#229493,#229494),(#229495,#229496),(#229497,#229498),
(#229499,#229500),(#229501,#229502),(#229503,#229504),(#229505,#229506),
(#229507,#229508),(#229509,#229510),(#229511,#229512),(#229513,#229514),
(#229515,#229516),(#229517,#229518)),.UNSPECIFIED.,.F.,.F.,.F.,(6,1,1,1,
1,1,1,1,1,1,1,1,1,1,1,1,1,1,1,1,1,1,1,1,1,1,1,1,1,1,1,1,1,1,1,1,1,1,1,1,
1,1,1,1,1,1,1,1,1,1,1,1,1,1,1,1,1,1,1,1,1,1,1,1,1,1,1,1,1,1,1,1,1,1,1,1,
1,1,1,1,1,1,1,1,1,1,1,1,1,1,1,1,1,1,1,1,1,1,1,1,1,1,1,1,1,1,1,1,1,1,1,1,
1,1,1,1,1,1,1,1,1,1,1,1,1,1,1,1,1,1,1,1,1,1,1,1,1,1,1,1,1,1,1,1,1,1,1,1,
1,1,1,1,1,1,1,1,1,1,1,1,1,1,1,1,1,1,1,1,1,1,1,1,1,1,1,1,1,1,1,1,1,1,1,1,
1,1,1,1,1,1,1,1,1,1,1,1,1,1,1,1,1,1,1,1,1,1,1,1,1,1,1,1,1,1,1,1,1,1,1,1,
1,1,1,1,1,1,1,1,1,1,1,1,1,1,1,1,1,1,1,1,1,1,1,1,1,1,1,1,1,1,1,1,1,1,1,1,
1,1,1,1,1,1,1,1,1,1,1,1,1,1,1,1,1,1,1,1,1,1,1,1,1,1,1,1,1,1,1,1,1,1,1,1,
1,1,1,1,1,1,1,1,1,1,1,1,1,1,1,1,1,1,1,1,1,1,1,1,1,1,1,1,1,1,1,1,1,1,1,1,
1,1,1,1,1,1,1,1,1,1,1,1,1,1,1,1,1,1,1,1,1,1,1,1,1,1,1,1,1,1,1,1,1,1,1,1,
1,1,1,1,1,1,1,1,1,1,1,1,1,1,1,1,1,1,1,1,1,1,1,1,1,1,1,1,1,1,1,1,1,1,1,1,
1,1,1,1,1,1,1,1,1,1,1,1,1,1,1,1,1,1,1,1,1,1,1,1,1,1,1,1,1,1,1,1,1,1,1,1,
1,1,1,1,1,1,1,1,1,1,1,1,1,1,1,1,1,1,1,1,1,1,1,1,1,1,1,1,1,1,1,6),(2,2),
(-1.,-0.998165138,-0.996330275,-0.994495413,-0.99266055,-0.990825688,-0.988990826,
-0.987155963,-0.985321101,-0.983486239,-0.981651376,-0.979816514,-0.977981651,
-0.976146789,-0.974311927,-0.972477064,-0.970642202,-0.968807339,-0.966972477,
-0.965137615,-0.963302752,-0.96146789,-0.959633028,-0.957798165,-0.955963303,
-0.95412844,-0.952293578,-0.950458716,-0.948623853,-0.946788991,-0.944954128,
-0.943119266,-0.941284404,-0.939449541,-0.937614679,-0.935779817,-0.933944954,
-0.932110092,-0.930275229,-0.928440367,-0.926605505,-0.924770642,-0.92293578,
-0.921100917,-0.919266055,-0.917431193,-0.91559633,-0.913761468,-0.911926606,
-0.910091743,-0.908256881,-0.906422018,-0.904587156,-0.902752294,-0.900917431,
-0.899082569,-0.897247706,-0.895412844,-0.893577982,-0.891743119,-0.889908257,
-0.888073394,-0.886238532,-0.88440367,-0.882568807,-0.880733945,-0.878899083,
-0.87706422,-0.875229358,-0.873394495,-0.871559633,-0.869724771,-0.867889908,
-0.866055046,-0.864220183,-0.862385321,-0.860550459,-0.858715596,-0.856880734,
-0.855045872,-0.853211009,-0.851376147,-0.849541284,-0.847706422,-0.84587156,
-0.844036697,-0.842201835,-0.840366972,-0.83853211,-0.836697248,-0.834862385,
-0.833027523,-0.831192661,-0.829357798,-0.827522936,-0.825688073,-0.823853211,
-0.822018349,-0.820183486,-0.818348624,-0.816513761,-0.814678899,-0.812844037,
-0.811009174,-0.809174312,-0.80733945,-0.805504587,-0.803669725,-0.801834862,
-0.8,-0.798165138,-0.796330275,-0.794495413,-0.79266055,-0.790825688,-0.788990826,
-0.787155963,-0.785321101,-0.783486239,-0.781651376,-0.779816514,-0.777981651,
-0.776146789,-0.774311927,-0.772477064,-0.770642202,-0.768807339,-0.766972477,
-0.765137615,-0.763302752,-0.76146789,-0.759633028,-0.757798165,-0.755963303,
-0.75412844,-0.752293578,-0.750458716,-0.748623853,-0.746788991,-0.744954128,
-0.743119266,-0.741284404,-0.739449541,-0.737614679,-0.735779817,-0.733944954,
-0.732110092,-0.730275229,-0.728440367,-0.726605505,-0.724770642,-0.72293578,
-0.721100917,-0.719266055,-0.717431193,-0.71559633,-0.713761468,-0.711926606,
-0.710091743,-0.708256881,-0.706422018,-0.704587156,-0.702752294,-0.700917431,
-0.699082569,-0.697247706,-0.695412844,-0.693577982,-0.691743119,-0.689908257,
-0.688073394,-0.686238532,-0.68440367,-0.682568807,-0.680733945,-0.678899083,
-0.67706422,-0.675229358,-0.673394495,-0.671559633,-0.669724771,-0.667889908,
-0.666055046,-0.664220183,-0.662385321,-0.660550459,-0.658715596,-0.656880734,
-0.655045872,-0.653211009,-0.651376147,-0.649541284,-0.647706422,-0.64587156,
-0.644036697,-0.642201835,-0.640366972,-0.63853211,-0.636697248,-0.634862385,
-0.633027523,-0.631192661,-0.629357798,-0.627522936,-0.625688073,-0.623853211,
-0.622018349,-0.620183486,-0.618348624,-0.616513761,-0.614678899,-0.612844037,
-0.611009174,-0.609174312,-0.60733945,-0.605504587,-0.603669725,-0.601834862,
-0.6,-0.598165138,-0.596330275,-0.594495413,-0.59266055,-0.590825688,-0.588990826,
-0.587155963,-0.585321101,-0.583486239,-0.581651376,-0.579816514,-0.577981651,
-0.576146789,-0.574311927,-0.572477064,-0.570642202,-0.568807339,-0.566972477,
-0.565137615,-0.563302752,-0.56146789,-0.559633028,-0.557798165,-0.555963303,
-0.55412844,-0.552293578,-0.550458716,-0.548623853,-0.546788991,-0.544954128,
-0.543119266,-0.541284404,-0.539449541,-0.537614679,-0.535779817,-0.533944954,
-0.532110092,-0.530275229,-0.528440367,-0.526605505,-0.524770642,-0.52293578,
-0.521100917,-0.519266055,-0.517431193,-0.51559633,-0.513761468,-0.511926606,
-0.510091743,-0.508256881,-0.506422018,-0.504587156,-0.502752294,-0.500917431,
-0.499082569,-0.497247706,-0.495412844,-0.493577982,-0.491743119,-0.489908257,
-0.488073394,-0.486238532,-0.48440367,-0.482568807,-0.480733945,-0.478899083,
-0.47706422,-0.475229358,-0.473394495,-0.471559633,-0.469724771,-0.467889908,
-0.466055046,-0.464220183,-0.462385321,-0.460550459,-0.458715596,-0.456880734,
-0.455045872,-0.453211009,-0.451376147,-0.449541284,-0.447706422,-0.44587156,
-0.444036697,-0.442201835,-0.440366972,-0.43853211,-0.436697248,-0.434862385,
-0.433027523,-0.431192661,-0.429357798,-0.427522936,-0.425688073,-0.423853211,
-0.422018349,-0.420183486,-0.418348624,-0.416513761,-0.414678899,-0.412844037,
-0.411009174,-0.409174312,-0.40733945,-0.405504587,-0.403669725,-0.401834862,
-0.4,-0.398165138,-0.396330275,-0.394495413,-0.39266055,-0.390825688,-0.388990826,
-0.387155963,-0.385321101,-0.383486239,-0.381651376,-0.379816514,-0.377981651,
-0.376146789,-0.374311927,-0.372477064,-0.370642202,-0.368807339,-0.366972477,
-0.365137615,-0.363302752,-0.36146789,-0.359633028,-0.357798165,-0.355963303,
-0.35412844,-0.352293578,-0.350458716,-0.348623853,-0.346788991,-0.344954128,
-0.343119266,-0.341284404,-0.339449541,-0.337614679,-0.335779817,-0.333944954,
-0.332110092,-0.330275229,-0.328440367,-0.326605505,-0.324770642,-0.32293578,
-0.321100917,-0.319266055,-0.317431193,-0.31559633,-0.313761468,-0.311926606,
-0.310091743,-0.308256881,-0.306422018,-0.304587156,-0.302752294,-0.300917431,
-0.299082569,-0.297247706,-0.295412844,-0.293577982,-0.291743119,-0.289908257,
-0.288073394,-0.286238532,-0.28440367,-0.282568807,-0.280733945,-0.278899083,
-0.27706422,-0.275229358,-0.273394495,-0.271559633,-0.269724771,-0.267889908,
-0.266055046,-0.264220183,-0.262385321,-0.260550459,-0.258715596,-0.256880734,
-0.255045872,-0.253211009,-0.251376147,-0.249541284,-0.247706422,-0.24587156,
-0.244036697,-0.242201835,-0.240366972,-0.23853211,-0.236697248,-0.234862385,
-0.233027523,-0.231192661,-0.229357798,-0.227522936,-0.225688073,-0.223853211,
-0.222018349,-0.220183486,-0.218348624,-0.216513761,-0.214678899,-0.212844037,
-0.211009174,-0.209174312,-0.20733945,-0.205504587,-0.203669725,-0.201834862,
-0.2,-0.198165138,-0.196330275,-0.194495413,-0.19266055,-0.190825688,-0.188990826,
-0.187155963,-0.185321101,-0.183486239,-0.181651376,-0.179816514,-0.177981651,
-0.176146789,-0.174311927,-0.172477064,-0.170642202,-0.168807339,-0.166972477,
-0.165137615,-0.163302752,-0.16146789,-0.159633028,-0.157798165,-0.155963303,
-0.15412844,-0.152293578,-0.150458716,-0.148623853,-0.146788991,-0.144954128,
-0.143172103),(0.,0.36),.UNSPECIFIED.);
#6261=B_SPLINE_SURFACE_WITH_KNOTS('',5,1,((#230148,#230149),(#230150,#230151),
(#230152,#230153),(#230154,#230155),(#230156,#230157),(#230158,#230159),
(#230160,#230161),(#230162,#230163),(#230164,#230165),(#230166,#230167),
(#230168,#230169),(#230170,#230171),(#230172,#230173),(#230174,#230175),
(#230176,#230177),(#230178,#230179),(#230180,#230181),(#230182,#230183),
(#230184,#230185),(#230186,#230187),(#230188,#230189),(#230190,#230191),
(#230192,#230193),(#230194,#230195),(#230196,#230197),(#230198,#230199),
(#230200,#230201),(#230202,#230203),(#230204,#230205),(#230206,#230207),
(#230208,#230209),(#230210,#230211),(#230212,#230213),(#230214,#230215),
(#230216,#230217),(#230218,#230219),(#230220,#230221),(#230222,#230223),
(#230224,#230225),(#230226,#230227),(#230228,#230229),(#230230,#230231),
(#230232,#230233),(#230234,#230235),(#230236,#230237),(#230238,#230239),
(#230240,#230241),(#230242,#230243),(#230244,#230245),(#230246,#230247),
(#230248,#230249),(#230250,#230251),(#230252,#230253),(#230254,#230255),
(#230256,#230257),(#230258,#230259),(#230260,#230261),(#230262,#230263),
(#230264,#230265),(#230266,#230267),(#230268,#230269),(#230270,#230271),
(#230272,#230273),(#230274,#230275),(#230276,#230277),(#230278,#230279),
(#230280,#230281),(#230282,#230283),(#230284,#230285),(#230286,#230287),
(#230288,#230289),(#230290,#230291),(#230292,#230293),(#230294,#230295),
(#230296,#230297),(#230298,#230299),(#230300,#230301),(#230302,#230303),
(#230304,#230305),(#230306,#230307),(#230308,#230309),(#230310,#230311),
(#230312,#230313),(#230314,#230315),(#230316,#230317),(#230318,#230319),
(#230320,#230321),(#230322,#230323),(#230324,#230325),(#230326,#230327),
(#230328,#230329),(#230330,#230331),(#230332,#230333),(#230334,#230335),
(#230336,#230337),(#230338,#230339),(#230340,#230341),(#230342,#230343),
(#230344,#230345),(#230346,#230347),(#230348,#230349),(#230350,#230351),
(#230352,#230353),(#230354,#230355),(#230356,#230357),(#230358,#230359),
(#230360,#230361),(#230362,#230363),(#230364,#230365),(#230366,#230367),
(#230368,#230369),(#230370,#230371),(#230372,#230373),(#230374,#230375),
(#230376,#230377),(#230378,#230379),(#230380,#230381),(#230382,#230383),
(#230384,#230385),(#230386,#230387),(#230388,#230389),(#230390,#230391),
(#230392,#230393),(#230394,#230395),(#230396,#230397),(#230398,#230399),
(#230400,#230401),(#230402,#230403),(#230404,#230405),(#230406,#230407),
(#230408,#230409),(#230410,#230411),(#230412,#230413),(#230414,#230415),
(#230416,#230417),(#230418,#230419),(#230420,#230421),(#230422,#230423),
(#230424,#230425),(#230426,#230427),(#230428,#230429),(#230430,#230431),
(#230432,#230433),(#230434,#230435),(#230436,#230437),(#230438,#230439),
(#230440,#230441),(#230442,#230443),(#230444,#230445),(#230446,#230447),
(#230448,#230449),(#230450,#230451),(#230452,#230453),(#230454,#230455),
(#230456,#230457),(#230458,#230459),(#230460,#230461),(#230462,#230463),
(#230464,#230465),(#230466,#230467),(#230468,#230469),(#230470,#230471),
(#230472,#230473),(#230474,#230475),(#230476,#230477),(#230478,#230479),
(#230480,#230481),(#230482,#230483),(#230484,#230485),(#230486,#230487),
(#230488,#230489),(#230490,#230491),(#230492,#230493),(#230494,#230495),
(#230496,#230497),(#230498,#230499),(#230500,#230501),(#230502,#230503),
(#230504,#230505),(#230506,#230507),(#230508,#230509),(#230510,#230511),
(#230512,#230513),(#230514,#230515),(#230516,#230517),(#230518,#230519),
(#230520,#230521),(#230522,#230523),(#230524,#230525),(#230526,#230527),
(#230528,#230529),(#230530,#230531),(#230532,#230533),(#230534,#230535),
(#230536,#230537),(#230538,#230539),(#230540,#230541),(#230542,#230543),
(#230544,#230545),(#230546,#230547),(#230548,#230549),(#230550,#230551),
(#230552,#230553),(#230554,#230555),(#230556,#230557),(#230558,#230559),
(#230560,#230561),(#230562,#230563),(#230564,#230565),(#230566,#230567),
(#230568,#230569),(#230570,#230571),(#230572,#230573),(#230574,#230575),
(#230576,#230577),(#230578,#230579),(#230580,#230581),(#230582,#230583),
(#230584,#230585),(#230586,#230587),(#230588,#230589),(#230590,#230591),
(#230592,#230593),(#230594,#230595),(#230596,#230597),(#230598,#230599),
(#230600,#230601),(#230602,#230603),(#230604,#230605),(#230606,#230607),
(#230608,#230609),(#230610,#230611),(#230612,#230613),(#230614,#230615),
(#230616,#230617),(#230618,#230619),(#230620,#230621),(#230622,#230623),
(#230624,#230625),(#230626,#230627),(#230628,#230629),(#230630,#230631),
(#230632,#230633),(#230634,#230635),(#230636,#230637),(#230638,#230639),
(#230640,#230641),(#230642,#230643),(#230644,#230645),(#230646,#230647),
(#230648,#230649),(#230650,#230651),(#230652,#230653),(#230654,#230655),
(#230656,#230657),(#230658,#230659),(#230660,#230661),(#230662,#230663),
(#230664,#230665),(#230666,#230667),(#230668,#230669),(#230670,#230671),
(#230672,#230673),(#230674,#230675),(#230676,#230677),(#230678,#230679),
(#230680,#230681),(#230682,#230683),(#230684,#230685),(#230686,#230687),
(#230688,#230689),(#230690,#230691),(#230692,#230693),(#230694,#230695),
(#230696,#230697),(#230698,#230699),(#230700,#230701),(#230702,#230703),
(#230704,#230705),(#230706,#230707),(#230708,#230709),(#230710,#230711),
(#230712,#230713),(#230714,#230715),(#230716,#230717),(#230718,#230719),
(#230720,#230721),(#230722,#230723),(#230724,#230725),(#230726,#230727),
(#230728,#230729),(#230730,#230731),(#230732,#230733),(#230734,#230735),
(#230736,#230737),(#230738,#230739),(#230740,#230741),(#230742,#230743),
(#230744,#230745),(#230746,#230747),(#230748,#230749),(#230750,#230751),
(#230752,#230753),(#230754,#230755),(#230756,#230757),(#230758,#230759),
(#230760,#230761),(#230762,#230763),(#230764,#230765),(#230766,#230767),
(#230768,#230769),(#230770,#230771),(#230772,#230773),(#230774,#230775),
(#230776,#230777),(#230778,#230779),(#230780,#230781),(#230782,#230783),
(#230784,#230785),(#230786,#230787),(#230788,#230789),(#230790,#230791),
(#230792,#230793),(#230794,#230795),(#230796,#230797),(#230798,#230799),
(#230800,#230801),(#230802,#230803),(#230804,#230805),(#230806,#230807),
(#230808,#230809),(#230810,#230811),(#230812,#230813),(#230814,#230815),
(#230816,#230817),(#230818,#230819),(#230820,#230821),(#230822,#230823),
(#230824,#230825),(#230826,#230827),(#230828,#230829),(#230830,#230831),
(#230832,#230833),(#230834,#230835),(#230836,#230837),(#230838,#230839),
(#230840,#230841),(#230842,#230843),(#230844,#230845),(#230846,#230847),
(#230848,#230849),(#230850,#230851),(#230852,#230853),(#230854,#230855),
(#230856,#230857),(#230858,#230859),(#230860,#230861),(#230862,#230863),
(#230864,#230865),(#230866,#230867),(#230868,#230869),(#230870,#230871),
(#230872,#230873),(#230874,#230875),(#230876,#230877),(#230878,#230879),
(#230880,#230881),(#230882,#230883),(#230884,#230885),(#230886,#230887),
(#230888,#230889),(#230890,#230891),(#230892,#230893),(#230894,#230895),
(#230896,#230897),(#230898,#230899),(#230900,#230901),(#230902,#230903),
(#230904,#230905),(#230906,#230907),(#230908,#230909),(#230910,#230911),
(#230912,#230913),(#230914,#230915),(#230916,#230917),(#230918,#230919),
(#230920,#230921),(#230922,#230923),(#230924,#230925),(#230926,#230927),
(#230928,#230929),(#230930,#230931),(#230932,#230933),(#230934,#230935),
(#230936,#230937),(#230938,#230939),(#230940,#230941),(#230942,#230943),
(#230944,#230945),(#230946,#230947),(#230948,#230949),(#230950,#230951),
(#230952,#230953),(#230954,#230955),(#230956,#230957),(#230958,#230959),
(#230960,#230961),(#230962,#230963),(#230964,#230965),(#230966,#230967),
(#230968,#230969),(#230970,#230971),(#230972,#230973),(#230974,#230975),
(#230976,#230977),(#230978,#230979),(#230980,#230981),(#230982,#230983),
(#230984,#230985),(#230986,#230987),(#230988,#230989),(#230990,#230991),
(#230992,#230993),(#230994,#230995),(#230996,#230997),(#230998,#230999),
(#231000,#231001),(#231002,#231003),(#231004,#231005),(#231006,#231007),
(#231008,#231009),(#231010,#231011),(#231012,#231013),(#231014,#231015),
(#231016,#231017),(#231018,#231019),(#231020,#231021),(#231022,#231023),
(#231024,#231025),(#231026,#231027),(#231028,#231029),(#231030,#231031),
(#231032,#231033),(#231034,#231035),(#231036,#231037),(#231038,#231039),
(#231040,#231041),(#231042,#231043),(#231044,#231045),(#231046,#231047),
(#231048,#231049),(#231050,#231051),(#231052,#231053),(#231054,#231055),
(#231056,#231057),(#231058,#231059),(#231060,#231061),(#231062,#231063),
(#231064,#231065),(#231066,#231067),(#231068,#231069),(#231070,#231071),
(#231072,#231073),(#231074,#231075),(#231076,#231077),(#231078,#231079),
(#231080,#231081),(#231082,#231083),(#231084,#231085),(#231086,#231087),
(#231088,#231089),(#231090,#231091)),.UNSPECIFIED.,.F.,.F.,.F.,(6,1,1,1,
1,1,1,1,1,1,1,1,1,1,1,1,1,1,1,1,1,1,1,1,1,1,1,1,1,1,1,1,1,1,1,1,1,1,1,1,
1,1,1,1,1,1,1,1,1,1,1,1,1,1,1,1,1,1,1,1,1,1,1,1,1,1,1,1,1,1,1,1,1,1,1,1,
1,1,1,1,1,1,1,1,1,1,1,1,1,1,1,1,1,1,1,1,1,1,1,1,1,1,1,1,1,1,1,1,1,1,1,1,
1,1,1,1,1,1,1,1,1,1,1,1,1,1,1,1,1,1,1,1,1,1,1,1,1,1,1,1,1,1,1,1,1,1,1,1,
1,1,1,1,1,1,1,1,1,1,1,1,1,1,1,1,1,1,1,1,1,1,1,1,1,1,1,1,1,1,1,1,1,1,1,1,
1,1,1,1,1,1,1,1,1,1,1,1,1,1,1,1,1,1,1,1,1,1,1,1,1,1,1,1,1,1,1,1,1,1,1,1,
1,1,1,1,1,1,1,1,1,1,1,1,1,1,1,1,1,1,1,1,1,1,1,1,1,1,1,1,1,1,1,1,1,1,1,1,
1,1,1,1,1,1,1,1,1,1,1,1,1,1,1,1,1,1,1,1,1,1,1,1,1,1,1,1,1,1,1,1,1,1,1,1,
1,1,1,1,1,1,1,1,1,1,1,1,1,1,1,1,1,1,1,1,1,1,1,1,1,1,1,1,1,1,1,1,1,1,1,1,
1,1,1,1,1,1,1,1,1,1,1,1,1,1,1,1,1,1,1,1,1,1,1,1,1,1,1,1,1,1,1,1,1,1,1,1,
1,1,1,1,1,1,1,1,1,1,1,1,1,1,1,1,1,1,1,1,1,1,1,1,1,1,1,1,1,1,1,1,1,1,1,1,
1,1,1,1,1,1,1,1,1,1,1,1,1,1,1,1,1,1,1,1,1,1,1,1,1,1,1,1,1,1,1,1,1,1,1,1,
1,1,1,1,1,1,1,1,1,1,1,1,1,1,1,1,1,1,1,1,1,1,1,1,1,1,1,1,1,1,1,6),(2,2),
(-1.,-0.998165138,-0.996330275,-0.994495413,-0.99266055,-0.990825688,-0.988990826,
-0.987155963,-0.985321101,-0.983486239,-0.981651376,-0.979816514,-0.977981651,
-0.976146789,-0.974311927,-0.972477064,-0.970642202,-0.968807339,-0.966972477,
-0.965137615,-0.963302752,-0.96146789,-0.959633028,-0.957798165,-0.955963303,
-0.95412844,-0.952293578,-0.950458716,-0.948623853,-0.946788991,-0.944954128,
-0.943119266,-0.941284404,-0.939449541,-0.937614679,-0.935779817,-0.933944954,
-0.932110092,-0.930275229,-0.928440367,-0.926605505,-0.924770642,-0.92293578,
-0.921100917,-0.919266055,-0.917431193,-0.91559633,-0.913761468,-0.911926606,
-0.910091743,-0.908256881,-0.906422018,-0.904587156,-0.902752294,-0.900917431,
-0.899082569,-0.897247706,-0.895412844,-0.893577982,-0.891743119,-0.889908257,
-0.888073394,-0.886238532,-0.88440367,-0.882568807,-0.880733945,-0.878899083,
-0.87706422,-0.875229358,-0.873394495,-0.871559633,-0.869724771,-0.867889908,
-0.866055046,-0.864220183,-0.862385321,-0.860550459,-0.858715596,-0.856880734,
-0.855045872,-0.853211009,-0.851376147,-0.849541284,-0.847706422,-0.84587156,
-0.844036697,-0.842201835,-0.840366972,-0.83853211,-0.836697248,-0.834862385,
-0.833027523,-0.831192661,-0.829357798,-0.827522936,-0.825688073,-0.823853211,
-0.822018349,-0.820183486,-0.818348624,-0.816513761,-0.814678899,-0.812844037,
-0.811009174,-0.809174312,-0.80733945,-0.805504587,-0.803669725,-0.801834862,
-0.8,-0.798165138,-0.796330275,-0.794495413,-0.79266055,-0.790825688,-0.788990826,
-0.787155963,-0.785321101,-0.783486239,-0.781651376,-0.779816514,-0.777981651,
-0.776146789,-0.774311927,-0.772477064,-0.770642202,-0.768807339,-0.766972477,
-0.765137615,-0.763302752,-0.76146789,-0.759633028,-0.757798165,-0.755963303,
-0.75412844,-0.752293578,-0.750458716,-0.748623853,-0.746788991,-0.744954128,
-0.743119266,-0.741284404,-0.739449541,-0.737614679,-0.735779817,-0.733944954,
-0.732110092,-0.730275229,-0.728440367,-0.726605505,-0.724770642,-0.72293578,
-0.721100917,-0.719266055,-0.717431193,-0.71559633,-0.713761468,-0.711926606,
-0.710091743,-0.708256881,-0.706422018,-0.704587156,-0.702752294,-0.700917431,
-0.699082569,-0.697247706,-0.695412844,-0.693577982,-0.691743119,-0.689908257,
-0.688073394,-0.686238532,-0.68440367,-0.682568807,-0.680733945,-0.678899083,
-0.67706422,-0.675229358,-0.673394495,-0.671559633,-0.669724771,-0.667889908,
-0.666055046,-0.664220183,-0.662385321,-0.660550459,-0.658715596,-0.656880734,
-0.655045872,-0.653211009,-0.651376147,-0.649541284,-0.647706422,-0.64587156,
-0.644036697,-0.642201835,-0.640366972,-0.63853211,-0.636697248,-0.634862385,
-0.633027523,-0.631192661,-0.629357798,-0.627522936,-0.625688073,-0.623853211,
-0.622018349,-0.620183486,-0.618348624,-0.616513761,-0.614678899,-0.612844037,
-0.611009174,-0.609174312,-0.60733945,-0.605504587,-0.603669725,-0.601834862,
-0.6,-0.598165138,-0.596330275,-0.594495413,-0.59266055,-0.590825688,-0.588990826,
-0.587155963,-0.585321101,-0.583486239,-0.581651376,-0.579816514,-0.577981651,
-0.576146789,-0.574311927,-0.572477064,-0.570642202,-0.568807339,-0.566972477,
-0.565137615,-0.563302752,-0.56146789,-0.559633028,-0.557798165,-0.555963303,
-0.55412844,-0.552293578,-0.550458716,-0.548623853,-0.546788991,-0.544954128,
-0.543119266,-0.541284404,-0.539449541,-0.537614679,-0.535779817,-0.533944954,
-0.532110092,-0.530275229,-0.528440367,-0.526605505,-0.524770642,-0.52293578,
-0.521100917,-0.519266055,-0.517431193,-0.51559633,-0.513761468,-0.511926606,
-0.510091743,-0.508256881,-0.506422018,-0.504587156,-0.502752294,-0.500917431,
-0.499082569,-0.497247706,-0.495412844,-0.493577982,-0.491743119,-0.489908257,
-0.488073394,-0.486238532,-0.48440367,-0.482568807,-0.480733945,-0.478899083,
-0.47706422,-0.475229358,-0.473394495,-0.471559633,-0.469724771,-0.467889908,
-0.466055046,-0.464220183,-0.462385321,-0.460550459,-0.458715596,-0.456880734,
-0.455045872,-0.453211009,-0.451376147,-0.449541284,-0.447706422,-0.44587156,
-0.444036697,-0.442201835,-0.440366972,-0.43853211,-0.436697248,-0.434862385,
-0.433027523,-0.431192661,-0.429357798,-0.427522936,-0.425688073,-0.423853211,
-0.422018349,-0.420183486,-0.418348624,-0.416513761,-0.414678899,-0.412844037,
-0.411009174,-0.409174312,-0.40733945,-0.405504587,-0.403669725,-0.401834862,
-0.4,-0.398165138,-0.396330275,-0.394495413,-0.39266055,-0.390825688,-0.388990826,
-0.387155963,-0.385321101,-0.383486239,-0.381651376,-0.379816514,-0.377981651,
-0.376146789,-0.374311927,-0.372477064,-0.370642202,-0.368807339,-0.366972477,
-0.365137615,-0.363302752,-0.36146789,-0.359633028,-0.357798165,-0.355963303,
-0.35412844,-0.352293578,-0.350458716,-0.348623853,-0.346788991,-0.344954128,
-0.343119266,-0.341284404,-0.339449541,-0.337614679,-0.335779817,-0.333944954,
-0.332110092,-0.330275229,-0.328440367,-0.326605505,-0.324770642,-0.32293578,
-0.321100917,-0.319266055,-0.317431193,-0.31559633,-0.313761468,-0.311926606,
-0.310091743,-0.308256881,-0.306422018,-0.304587156,-0.302752294,-0.300917431,
-0.299082569,-0.297247706,-0.295412844,-0.293577982,-0.291743119,-0.289908257,
-0.288073394,-0.286238532,-0.28440367,-0.282568807,-0.280733945,-0.278899083,
-0.27706422,-0.275229358,-0.273394495,-0.271559633,-0.269724771,-0.267889908,
-0.266055046,-0.264220183,-0.262385321,-0.260550459,-0.258715596,-0.256880734,
-0.255045872,-0.253211009,-0.251376147,-0.249541284,-0.247706422,-0.24587156,
-0.244036697,-0.242201835,-0.240366972,-0.23853211,-0.236697248,-0.234862385,
-0.233027523,-0.231192661,-0.229357798,-0.227522936,-0.225688073,-0.223853211,
-0.222018349,-0.220183486,-0.218348624,-0.216513761,-0.214678899,-0.212844037,
-0.211009174,-0.209174312,-0.20733945,-0.205504587,-0.203669725,-0.201834862,
-0.2,-0.198165138,-0.196330275,-0.194495413,-0.19266055,-0.190825688,-0.188990826,
-0.187155963,-0.185321101,-0.183486239,-0.181651376,-0.179816514,-0.177981651,
-0.176146789,-0.174311927,-0.172477064,-0.170642202,-0.168807339,-0.166972477,
-0.165137615,-0.163302752,-0.16146789,-0.159633028,-0.157798165,-0.155963303,
-0.15412844,-0.152293578,-0.150458716,-0.148623853,-0.146788991,-0.144954128,
-0.143172104),(0.,0.36),.UNSPECIFIED.);
#6262=B_SPLINE_SURFACE_WITH_KNOTS('',5,1,((#231706,#231707),(#231708,#231709),
(#231710,#231711),(#231712,#231713),(#231714,#231715),(#231716,#231717),
(#231718,#231719),(#231720,#231721),(#231722,#231723),(#231724,#231725),
(#231726,#231727),(#231728,#231729),(#231730,#231731),(#231732,#231733),
(#231734,#231735),(#231736,#231737),(#231738,#231739),(#231740,#231741),
(#231742,#231743),(#231744,#231745),(#231746,#231747),(#231748,#231749),
(#231750,#231751),(#231752,#231753),(#231754,#231755),(#231756,#231757),
(#231758,#231759),(#231760,#231761),(#231762,#231763),(#231764,#231765),
(#231766,#231767),(#231768,#231769),(#231770,#231771),(#231772,#231773),
(#231774,#231775),(#231776,#231777),(#231778,#231779),(#231780,#231781),
(#231782,#231783),(#231784,#231785),(#231786,#231787),(#231788,#231789),
(#231790,#231791),(#231792,#231793),(#231794,#231795),(#231796,#231797),
(#231798,#231799),(#231800,#231801),(#231802,#231803),(#231804,#231805),
(#231806,#231807),(#231808,#231809),(#231810,#231811),(#231812,#231813),
(#231814,#231815),(#231816,#231817),(#231818,#231819),(#231820,#231821),
(#231822,#231823),(#231824,#231825),(#231826,#231827),(#231828,#231829),
(#231830,#231831),(#231832,#231833),(#231834,#231835),(#231836,#231837),
(#231838,#231839),(#231840,#231841),(#231842,#231843),(#231844,#231845),
(#231846,#231847),(#231848,#231849),(#231850,#231851),(#231852,#231853),
(#231854,#231855),(#231856,#231857),(#231858,#231859),(#231860,#231861),
(#231862,#231863),(#231864,#231865),(#231866,#231867),(#231868,#231869),
(#231870,#231871),(#231872,#231873),(#231874,#231875),(#231876,#231877),
(#231878,#231879),(#231880,#231881),(#231882,#231883),(#231884,#231885),
(#231886,#231887),(#231888,#231889),(#231890,#231891),(#231892,#231893),
(#231894,#231895),(#231896,#231897),(#231898,#231899),(#231900,#231901),
(#231902,#231903),(#231904,#231905),(#231906,#231907),(#231908,#231909),
(#231910,#231911),(#231912,#231913),(#231914,#231915),(#231916,#231917),
(#231918,#231919),(#231920,#231921),(#231922,#231923),(#231924,#231925),
(#231926,#231927),(#231928,#231929),(#231930,#231931),(#231932,#231933),
(#231934,#231935),(#231936,#231937),(#231938,#231939),(#231940,#231941),
(#231942,#231943),(#231944,#231945),(#231946,#231947),(#231948,#231949),
(#231950,#231951),(#231952,#231953),(#231954,#231955),(#231956,#231957),
(#231958,#231959),(#231960,#231961),(#231962,#231963),(#231964,#231965),
(#231966,#231967),(#231968,#231969),(#231970,#231971),(#231972,#231973),
(#231974,#231975),(#231976,#231977),(#231978,#231979),(#231980,#231981),
(#231982,#231983),(#231984,#231985),(#231986,#231987),(#231988,#231989),
(#231990,#231991),(#231992,#231993),(#231994,#231995),(#231996,#231997),
(#231998,#231999),(#232000,#232001),(#232002,#232003),(#232004,#232005),
(#232006,#232007),(#232008,#232009),(#232010,#232011),(#232012,#232013),
(#232014,#232015),(#232016,#232017),(#232018,#232019),(#232020,#232021),
(#232022,#232023),(#232024,#232025),(#232026,#232027),(#232028,#232029),
(#232030,#232031),(#232032,#232033),(#232034,#232035),(#232036,#232037),
(#232038,#232039),(#232040,#232041),(#232042,#232043),(#232044,#232045),
(#232046,#232047),(#232048,#232049),(#232050,#232051),(#232052,#232053),
(#232054,#232055),(#232056,#232057),(#232058,#232059),(#232060,#232061),
(#232062,#232063),(#232064,#232065),(#232066,#232067),(#232068,#232069),
(#232070,#232071),(#232072,#232073),(#232074,#232075),(#232076,#232077),
(#232078,#232079),(#232080,#232081),(#232082,#232083),(#232084,#232085),
(#232086,#232087),(#232088,#232089),(#232090,#232091),(#232092,#232093),
(#232094,#232095),(#232096,#232097),(#232098,#232099),(#232100,#232101),
(#232102,#232103),(#232104,#232105),(#232106,#232107),(#232108,#232109),
(#232110,#232111),(#232112,#232113),(#232114,#232115),(#232116,#232117),
(#232118,#232119),(#232120,#232121),(#232122,#232123),(#232124,#232125),
(#232126,#232127),(#232128,#232129),(#232130,#232131),(#232132,#232133),
(#232134,#232135),(#232136,#232137),(#232138,#232139),(#232140,#232141),
(#232142,#232143),(#232144,#232145),(#232146,#232147),(#232148,#232149),
(#232150,#232151),(#232152,#232153),(#232154,#232155),(#232156,#232157),
(#232158,#232159),(#232160,#232161),(#232162,#232163),(#232164,#232165),
(#232166,#232167),(#232168,#232169),(#232170,#232171),(#232172,#232173),
(#232174,#232175),(#232176,#232177),(#232178,#232179),(#232180,#232181),
(#232182,#232183),(#232184,#232185),(#232186,#232187),(#232188,#232189),
(#232190,#232191),(#232192,#232193),(#232194,#232195),(#232196,#232197),
(#232198,#232199),(#232200,#232201),(#232202,#232203),(#232204,#232205),
(#232206,#232207),(#232208,#232209),(#232210,#232211),(#232212,#232213),
(#232214,#232215),(#232216,#232217),(#232218,#232219),(#232220,#232221),
(#232222,#232223),(#232224,#232225),(#232226,#232227),(#232228,#232229),
(#232230,#232231),(#232232,#232233),(#232234,#232235),(#232236,#232237),
(#232238,#232239),(#232240,#232241),(#232242,#232243),(#232244,#232245),
(#232246,#232247),(#232248,#232249),(#232250,#232251),(#232252,#232253),
(#232254,#232255),(#232256,#232257),(#232258,#232259),(#232260,#232261),
(#232262,#232263),(#232264,#232265),(#232266,#232267),(#232268,#232269),
(#232270,#232271),(#232272,#232273),(#232274,#232275),(#232276,#232277),
(#232278,#232279),(#232280,#232281),(#232282,#232283),(#232284,#232285),
(#232286,#232287),(#232288,#232289),(#232290,#232291),(#232292,#232293),
(#232294,#232295),(#232296,#232297),(#232298,#232299),(#232300,#232301),
(#232302,#232303),(#232304,#232305),(#232306,#232307),(#232308,#232309),
(#232310,#232311),(#232312,#232313),(#232314,#232315),(#232316,#232317),
(#232318,#232319),(#232320,#232321),(#232322,#232323),(#232324,#232325),
(#232326,#232327),(#232328,#232329),(#232330,#232331),(#232332,#232333),
(#232334,#232335),(#232336,#232337),(#232338,#232339),(#232340,#232341),
(#232342,#232343),(#232344,#232345),(#232346,#232347),(#232348,#232349),
(#232350,#232351),(#232352,#232353),(#232354,#232355),(#232356,#232357),
(#232358,#232359),(#232360,#232361),(#232362,#232363),(#232364,#232365),
(#232366,#232367),(#232368,#232369),(#232370,#232371),(#232372,#232373),
(#232374,#232375),(#232376,#232377),(#232378,#232379),(#232380,#232381),
(#232382,#232383),(#232384,#232385),(#232386,#232387),(#232388,#232389),
(#232390,#232391),(#232392,#232393),(#232394,#232395),(#232396,#232397),
(#232398,#232399),(#232400,#232401),(#232402,#232403),(#232404,#232405),
(#232406,#232407),(#232408,#232409),(#232410,#232411),(#232412,#232413),
(#232414,#232415),(#232416,#232417),(#232418,#232419),(#232420,#232421),
(#232422,#232423),(#232424,#232425),(#232426,#232427),(#232428,#232429),
(#232430,#232431),(#232432,#232433),(#232434,#232435),(#232436,#232437),
(#232438,#232439),(#232440,#232441),(#232442,#232443),(#232444,#232445),
(#232446,#232447),(#232448,#232449),(#232450,#232451),(#232452,#232453),
(#232454,#232455),(#232456,#232457),(#232458,#232459),(#232460,#232461),
(#232462,#232463),(#232464,#232465),(#232466,#232467),(#232468,#232469),
(#232470,#232471),(#232472,#232473),(#232474,#232475),(#232476,#232477),
(#232478,#232479),(#232480,#232481),(#232482,#232483),(#232484,#232485),
(#232486,#232487),(#232488,#232489),(#232490,#232491),(#232492,#232493),
(#232494,#232495),(#232496,#232497),(#232498,#232499),(#232500,#232501),
(#232502,#232503),(#232504,#232505),(#232506,#232507),(#232508,#232509),
(#232510,#232511),(#232512,#232513),(#232514,#232515),(#232516,#232517),
(#232518,#232519),(#232520,#232521),(#232522,#232523),(#232524,#232525),
(#232526,#232527),(#232528,#232529),(#232530,#232531),(#232532,#232533),
(#232534,#232535),(#232536,#232537),(#232538,#232539),(#232540,#232541),
(#232542,#232543),(#232544,#232545),(#232546,#232547),(#232548,#232549),
(#232550,#232551),(#232552,#232553),(#232554,#232555),(#232556,#232557),
(#232558,#232559),(#232560,#232561),(#232562,#232563),(#232564,#232565),
(#232566,#232567),(#232568,#232569),(#232570,#232571),(#232572,#232573),
(#232574,#232575),(#232576,#232577),(#232578,#232579),(#232580,#232581),
(#232582,#232583),(#232584,#232585),(#232586,#232587),(#232588,#232589),
(#232590,#232591),(#232592,#232593),(#232594,#232595),(#232596,#232597),
(#232598,#232599),(#232600,#232601),(#232602,#232603),(#232604,#232605),
(#232606,#232607),(#232608,#232609),(#232610,#232611),(#232612,#232613),
(#232614,#232615),(#232616,#232617),(#232618,#232619),(#232620,#232621),
(#232622,#232623),(#232624,#232625),(#232626,#232627),(#232628,#232629),
(#232630,#232631),(#232632,#232633),(#232634,#232635),(#232636,#232637),
(#232638,#232639),(#232640,#232641),(#232642,#232643),(#232644,#232645),
(#232646,#232647),(#232648,#232649)),.UNSPECIFIED.,.F.,.F.,.F.,(6,1,1,1,
1,1,1,1,1,1,1,1,1,1,1,1,1,1,1,1,1,1,1,1,1,1,1,1,1,1,1,1,1,1,1,1,1,1,1,1,
1,1,1,1,1,1,1,1,1,1,1,1,1,1,1,1,1,1,1,1,1,1,1,1,1,1,1,1,1,1,1,1,1,1,1,1,
1,1,1,1,1,1,1,1,1,1,1,1,1,1,1,1,1,1,1,1,1,1,1,1,1,1,1,1,1,1,1,1,1,1,1,1,
1,1,1,1,1,1,1,1,1,1,1,1,1,1,1,1,1,1,1,1,1,1,1,1,1,1,1,1,1,1,1,1,1,1,1,1,
1,1,1,1,1,1,1,1,1,1,1,1,1,1,1,1,1,1,1,1,1,1,1,1,1,1,1,1,1,1,1,1,1,1,1,1,
1,1,1,1,1,1,1,1,1,1,1,1,1,1,1,1,1,1,1,1,1,1,1,1,1,1,1,1,1,1,1,1,1,1,1,1,
1,1,1,1,1,1,1,1,1,1,1,1,1,1,1,1,1,1,1,1,1,1,1,1,1,1,1,1,1,1,1,1,1,1,1,1,
1,1,1,1,1,1,1,1,1,1,1,1,1,1,1,1,1,1,1,1,1,1,1,1,1,1,1,1,1,1,1,1,1,1,1,1,
1,1,1,1,1,1,1,1,1,1,1,1,1,1,1,1,1,1,1,1,1,1,1,1,1,1,1,1,1,1,1,1,1,1,1,1,
1,1,1,1,1,1,1,1,1,1,1,1,1,1,1,1,1,1,1,1,1,1,1,1,1,1,1,1,1,1,1,1,1,1,1,1,
1,1,1,1,1,1,1,1,1,1,1,1,1,1,1,1,1,1,1,1,1,1,1,1,1,1,1,1,1,1,1,1,1,1,1,1,
1,1,1,1,1,1,1,1,1,1,1,1,1,1,1,1,1,1,1,1,1,1,1,1,1,1,1,1,1,1,1,1,1,1,1,1,
1,1,1,1,1,1,1,1,1,1,1,1,1,1,1,1,1,1,1,1,1,1,1,1,1,1,1,1,1,1,1,6),(2,2),
(0.143172105,0.144954128,0.146788991,0.148623853,0.150458716,0.152293578,
0.15412844,0.155963303,0.157798165,0.159633028,0.16146789,0.163302752,0.165137615,
0.166972477,0.168807339,0.170642202,0.172477064,0.174311927,0.176146789,
0.177981651,0.179816514,0.181651376,0.183486239,0.185321101,0.187155963,
0.188990826,0.190825688,0.19266055,0.194495413,0.196330275,0.198165138,
0.2,0.201834862,0.203669725,0.205504587,0.20733945,0.209174312,0.211009174,
0.212844037,0.214678899,0.216513761,0.218348624,0.220183486,0.222018349,
0.223853211,0.225688073,0.227522936,0.229357798,0.231192661,0.233027523,
0.234862385,0.236697248,0.23853211,0.240366972,0.242201835,0.244036697,
0.24587156,0.247706422,0.249541284,0.251376147,0.253211009,0.255045872,
0.256880734,0.258715596,0.260550459,0.262385321,0.264220183,0.266055046,
0.267889908,0.269724771,0.271559633,0.273394495,0.275229358,0.27706422,
0.278899083,0.280733945,0.282568807,0.28440367,0.286238532,0.288073394,
0.289908257,0.291743119,0.293577982,0.295412844,0.297247706,0.299082569,
0.300917431,0.302752294,0.304587156,0.306422018,0.308256881,0.310091743,
0.311926606,0.313761468,0.31559633,0.317431193,0.319266055,0.321100917,
0.32293578,0.324770642,0.326605505,0.328440367,0.330275229,0.332110092,
0.333944954,0.335779817,0.337614679,0.339449541,0.341284404,0.343119266,
0.344954128,0.346788991,0.348623853,0.350458716,0.352293578,0.35412844,
0.355963303,0.357798165,0.359633028,0.36146789,0.363302752,0.365137615,
0.366972477,0.368807339,0.370642202,0.372477064,0.374311927,0.376146789,
0.377981651,0.379816514,0.381651376,0.383486239,0.385321101,0.387155963,
0.388990826,0.390825688,0.39266055,0.394495413,0.396330275,0.398165138,
0.4,0.401834862,0.403669725,0.405504587,0.40733945,0.409174312,0.411009174,
0.412844037,0.414678899,0.416513761,0.418348624,0.420183486,0.422018349,
0.423853211,0.425688073,0.427522936,0.429357798,0.431192661,0.433027523,
0.434862385,0.436697248,0.43853211,0.440366972,0.442201835,0.444036697,
0.44587156,0.447706422,0.449541284,0.451376147,0.453211009,0.455045872,
0.456880734,0.458715596,0.460550459,0.462385321,0.464220183,0.466055046,
0.467889908,0.469724771,0.471559633,0.473394495,0.475229358,0.47706422,
0.478899083,0.480733945,0.482568807,0.48440367,0.486238532,0.488073394,
0.489908257,0.491743119,0.493577982,0.495412844,0.497247706,0.499082569,
0.500917431,0.502752294,0.504587156,0.506422018,0.508256881,0.510091743,
0.511926606,0.513761468,0.51559633,0.517431193,0.519266055,0.521100917,
0.52293578,0.524770642,0.526605505,0.528440367,0.530275229,0.532110092,
0.533944954,0.535779817,0.537614679,0.539449541,0.541284404,0.543119266,
0.544954128,0.546788991,0.548623853,0.550458716,0.552293578,0.55412844,
0.555963303,0.557798165,0.559633028,0.56146789,0.563302752,0.565137615,
0.566972477,0.568807339,0.570642202,0.572477064,0.574311927,0.576146789,
0.577981651,0.579816514,0.581651376,0.583486239,0.585321101,0.587155963,
0.588990826,0.590825688,0.59266055,0.594495413,0.596330275,0.598165138,
0.6,0.601834862,0.603669725,0.605504587,0.60733945,0.609174312,0.611009174,
0.612844037,0.614678899,0.616513761,0.618348624,0.620183486,0.622018349,
0.623853211,0.625688073,0.627522936,0.629357798,0.631192661,0.633027523,
0.634862385,0.636697248,0.63853211,0.640366972,0.642201835,0.644036697,
0.64587156,0.647706422,0.649541284,0.651376147,0.653211009,0.655045872,
0.656880734,0.658715596,0.660550459,0.662385321,0.664220183,0.666055046,
0.667889908,0.669724771,0.671559633,0.673394495,0.675229358,0.67706422,
0.678899083,0.680733945,0.682568807,0.68440367,0.686238532,0.688073394,
0.689908257,0.691743119,0.693577982,0.695412844,0.697247706,0.699082569,
0.700917431,0.702752294,0.704587156,0.706422018,0.708256881,0.710091743,
0.711926606,0.713761468,0.71559633,0.717431193,0.719266055,0.721100917,
0.72293578,0.724770642,0.726605505,0.728440367,0.730275229,0.732110092,
0.733944954,0.735779817,0.737614679,0.739449541,0.741284404,0.743119266,
0.744954128,0.746788991,0.748623853,0.750458716,0.752293578,0.75412844,
0.755963303,0.757798165,0.759633028,0.76146789,0.763302752,0.765137615,
0.766972477,0.768807339,0.770642202,0.772477064,0.774311927,0.776146789,
0.777981651,0.779816514,0.781651376,0.783486239,0.785321101,0.787155963,
0.788990826,0.790825688,0.79266055,0.794495413,0.796330275,0.798165138,
0.8,0.801834862,0.803669725,0.805504587,0.80733945,0.809174312,0.811009174,
0.812844037,0.814678899,0.816513761,0.818348624,0.820183486,0.822018349,
0.823853211,0.825688073,0.827522936,0.829357798,0.831192661,0.833027523,
0.834862385,0.836697248,0.83853211,0.840366972,0.842201835,0.844036697,
0.84587156,0.847706422,0.849541284,0.851376147,0.853211009,0.855045872,
0.856880734,0.858715596,0.860550459,0.862385321,0.864220183,0.866055046,
0.867889908,0.869724771,0.871559633,0.873394495,0.875229358,0.87706422,
0.878899083,0.880733945,0.882568807,0.88440367,0.886238532,0.888073394,
0.889908257,0.891743119,0.893577982,0.895412844,0.897247706,0.899082569,
0.900917431,0.902752294,0.904587156,0.906422018,0.908256881,0.910091743,
0.911926606,0.913761468,0.91559633,0.917431193,0.919266055,0.921100917,
0.92293578,0.924770642,0.926605505,0.928440367,0.930275229,0.932110092,
0.933944954,0.935779817,0.937614679,0.939449541,0.941284404,0.943119266,
0.944954128,0.946788991,0.948623853,0.950458716,0.952293578,0.95412844,
0.955963303,0.957798165,0.959633028,0.96146789,0.963302752,0.965137615,
0.966972477,0.968807339,0.970642202,0.972477064,0.974311927,0.976146789,
0.977981651,0.979816514,0.981651376,0.983486239,0.985321101,0.987155963,
0.988990826,0.990825688,0.99266055,0.994495413,0.996330275,0.998165138,
1.),(0.,0.36),.UNSPECIFIED.);
#6263=B_SPLINE_SURFACE_WITH_KNOTS('',5,1,((#233288,#233289),(#233290,#233291),
(#233292,#233293),(#233294,#233295),(#233296,#233297),(#233298,#233299),
(#233300,#233301),(#233302,#233303),(#233304,#233305),(#233306,#233307),
(#233308,#233309),(#233310,#233311),(#233312,#233313),(#233314,#233315),
(#233316,#233317),(#233318,#233319),(#233320,#233321),(#233322,#233323),
(#233324,#233325),(#233326,#233327),(#233328,#233329),(#233330,#233331),
(#233332,#233333),(#233334,#233335),(#233336,#233337),(#233338,#233339),
(#233340,#233341),(#233342,#233343),(#233344,#233345),(#233346,#233347),
(#233348,#233349),(#233350,#233351),(#233352,#233353),(#233354,#233355),
(#233356,#233357),(#233358,#233359),(#233360,#233361),(#233362,#233363),
(#233364,#233365),(#233366,#233367),(#233368,#233369),(#233370,#233371),
(#233372,#233373),(#233374,#233375),(#233376,#233377),(#233378,#233379),
(#233380,#233381),(#233382,#233383),(#233384,#233385),(#233386,#233387),
(#233388,#233389),(#233390,#233391),(#233392,#233393),(#233394,#233395),
(#233396,#233397),(#233398,#233399),(#233400,#233401),(#233402,#233403),
(#233404,#233405),(#233406,#233407),(#233408,#233409),(#233410,#233411),
(#233412,#233413),(#233414,#233415),(#233416,#233417),(#233418,#233419),
(#233420,#233421),(#233422,#233423),(#233424,#233425),(#233426,#233427),
(#233428,#233429),(#233430,#233431),(#233432,#233433),(#233434,#233435),
(#233436,#233437),(#233438,#233439),(#233440,#233441),(#233442,#233443),
(#233444,#233445),(#233446,#233447),(#233448,#233449),(#233450,#233451),
(#233452,#233453),(#233454,#233455),(#233456,#233457),(#233458,#233459),
(#233460,#233461),(#233462,#233463),(#233464,#233465),(#233466,#233467),
(#233468,#233469),(#233470,#233471),(#233472,#233473),(#233474,#233475),
(#233476,#233477),(#233478,#233479),(#233480,#233481),(#233482,#233483),
(#233484,#233485),(#233486,#233487),(#233488,#233489),(#233490,#233491),
(#233492,#233493),(#233494,#233495),(#233496,#233497),(#233498,#233499),
(#233500,#233501),(#233502,#233503),(#233504,#233505),(#233506,#233507),
(#233508,#233509),(#233510,#233511),(#233512,#233513),(#233514,#233515),
(#233516,#233517),(#233518,#233519),(#233520,#233521),(#233522,#233523),
(#233524,#233525),(#233526,#233527),(#233528,#233529),(#233530,#233531),
(#233532,#233533),(#233534,#233535),(#233536,#233537),(#233538,#233539),
(#233540,#233541),(#233542,#233543),(#233544,#233545),(#233546,#233547),
(#233548,#233549),(#233550,#233551),(#233552,#233553),(#233554,#233555),
(#233556,#233557),(#233558,#233559),(#233560,#233561),(#233562,#233563),
(#233564,#233565),(#233566,#233567),(#233568,#233569),(#233570,#233571),
(#233572,#233573),(#233574,#233575),(#233576,#233577),(#233578,#233579),
(#233580,#233581),(#233582,#233583),(#233584,#233585),(#233586,#233587),
(#233588,#233589),(#233590,#233591),(#233592,#233593),(#233594,#233595),
(#233596,#233597),(#233598,#233599),(#233600,#233601),(#233602,#233603),
(#233604,#233605),(#233606,#233607),(#233608,#233609),(#233610,#233611),
(#233612,#233613),(#233614,#233615),(#233616,#233617),(#233618,#233619),
(#233620,#233621),(#233622,#233623),(#233624,#233625),(#233626,#233627),
(#233628,#233629),(#233630,#233631),(#233632,#233633),(#233634,#233635),
(#233636,#233637),(#233638,#233639),(#233640,#233641),(#233642,#233643),
(#233644,#233645),(#233646,#233647),(#233648,#233649),(#233650,#233651),
(#233652,#233653),(#233654,#233655),(#233656,#233657),(#233658,#233659),
(#233660,#233661),(#233662,#233663),(#233664,#233665),(#233666,#233667),
(#233668,#233669),(#233670,#233671),(#233672,#233673),(#233674,#233675),
(#233676,#233677),(#233678,#233679),(#233680,#233681),(#233682,#233683),
(#233684,#233685),(#233686,#233687),(#233688,#233689),(#233690,#233691),
(#233692,#233693),(#233694,#233695),(#233696,#233697),(#233698,#233699),
(#233700,#233701),(#233702,#233703),(#233704,#233705),(#233706,#233707),
(#233708,#233709),(#233710,#233711),(#233712,#233713),(#233714,#233715),
(#233716,#233717),(#233718,#233719),(#233720,#233721),(#233722,#233723),
(#233724,#233725),(#233726,#233727),(#233728,#233729),(#233730,#233731),
(#233732,#233733),(#233734,#233735),(#233736,#233737),(#233738,#233739),
(#233740,#233741),(#233742,#233743),(#233744,#233745),(#233746,#233747),
(#233748,#233749),(#233750,#233751),(#233752,#233753),(#233754,#233755),
(#233756,#233757),(#233758,#233759),(#233760,#233761),(#233762,#233763),
(#233764,#233765),(#233766,#233767),(#233768,#233769),(#233770,#233771),
(#233772,#233773),(#233774,#233775),(#233776,#233777),(#233778,#233779),
(#233780,#233781),(#233782,#233783),(#233784,#233785),(#233786,#233787),
(#233788,#233789),(#233790,#233791),(#233792,#233793),(#233794,#233795),
(#233796,#233797),(#233798,#233799),(#233800,#233801),(#233802,#233803),
(#233804,#233805),(#233806,#233807),(#233808,#233809),(#233810,#233811),
(#233812,#233813),(#233814,#233815),(#233816,#233817),(#233818,#233819),
(#233820,#233821),(#233822,#233823),(#233824,#233825),(#233826,#233827),
(#233828,#233829),(#233830,#233831),(#233832,#233833),(#233834,#233835),
(#233836,#233837),(#233838,#233839),(#233840,#233841),(#233842,#233843),
(#233844,#233845),(#233846,#233847),(#233848,#233849),(#233850,#233851),
(#233852,#233853),(#233854,#233855),(#233856,#233857),(#233858,#233859),
(#233860,#233861),(#233862,#233863),(#233864,#233865),(#233866,#233867),
(#233868,#233869),(#233870,#233871),(#233872,#233873),(#233874,#233875),
(#233876,#233877),(#233878,#233879),(#233880,#233881),(#233882,#233883),
(#233884,#233885),(#233886,#233887),(#233888,#233889),(#233890,#233891),
(#233892,#233893),(#233894,#233895),(#233896,#233897),(#233898,#233899),
(#233900,#233901),(#233902,#233903),(#233904,#233905),(#233906,#233907),
(#233908,#233909),(#233910,#233911),(#233912,#233913),(#233914,#233915),
(#233916,#233917),(#233918,#233919),(#233920,#233921),(#233922,#233923),
(#233924,#233925),(#233926,#233927),(#233928,#233929),(#233930,#233931),
(#233932,#233933),(#233934,#233935),(#233936,#233937),(#233938,#233939),
(#233940,#233941),(#233942,#233943),(#233944,#233945),(#233946,#233947),
(#233948,#233949),(#233950,#233951),(#233952,#233953),(#233954,#233955),
(#233956,#233957),(#233958,#233959),(#233960,#233961),(#233962,#233963),
(#233964,#233965),(#233966,#233967),(#233968,#233969),(#233970,#233971),
(#233972,#233973),(#233974,#233975),(#233976,#233977),(#233978,#233979),
(#233980,#233981),(#233982,#233983),(#233984,#233985),(#233986,#233987),
(#233988,#233989),(#233990,#233991),(#233992,#233993),(#233994,#233995),
(#233996,#233997),(#233998,#233999),(#234000,#234001),(#234002,#234003),
(#234004,#234005),(#234006,#234007),(#234008,#234009),(#234010,#234011),
(#234012,#234013),(#234014,#234015),(#234016,#234017),(#234018,#234019),
(#234020,#234021),(#234022,#234023),(#234024,#234025),(#234026,#234027),
(#234028,#234029),(#234030,#234031),(#234032,#234033),(#234034,#234035),
(#234036,#234037),(#234038,#234039),(#234040,#234041),(#234042,#234043),
(#234044,#234045),(#234046,#234047),(#234048,#234049),(#234050,#234051),
(#234052,#234053),(#234054,#234055),(#234056,#234057),(#234058,#234059),
(#234060,#234061),(#234062,#234063),(#234064,#234065),(#234066,#234067),
(#234068,#234069),(#234070,#234071),(#234072,#234073),(#234074,#234075),
(#234076,#234077),(#234078,#234079),(#234080,#234081),(#234082,#234083),
(#234084,#234085),(#234086,#234087),(#234088,#234089),(#234090,#234091),
(#234092,#234093),(#234094,#234095),(#234096,#234097),(#234098,#234099),
(#234100,#234101),(#234102,#234103),(#234104,#234105),(#234106,#234107),
(#234108,#234109),(#234110,#234111),(#234112,#234113),(#234114,#234115),
(#234116,#234117),(#234118,#234119),(#234120,#234121),(#234122,#234123),
(#234124,#234125),(#234126,#234127),(#234128,#234129),(#234130,#234131),
(#234132,#234133),(#234134,#234135),(#234136,#234137),(#234138,#234139),
(#234140,#234141),(#234142,#234143),(#234144,#234145),(#234146,#234147),
(#234148,#234149),(#234150,#234151),(#234152,#234153),(#234154,#234155),
(#234156,#234157),(#234158,#234159),(#234160,#234161),(#234162,#234163),
(#234164,#234165),(#234166,#234167),(#234168,#234169),(#234170,#234171),
(#234172,#234173),(#234174,#234175),(#234176,#234177),(#234178,#234179),
(#234180,#234181),(#234182,#234183),(#234184,#234185),(#234186,#234187),
(#234188,#234189),(#234190,#234191),(#234192,#234193),(#234194,#234195),
(#234196,#234197),(#234198,#234199),(#234200,#234201),(#234202,#234203),
(#234204,#234205),(#234206,#234207),(#234208,#234209),(#234210,#234211),
(#234212,#234213),(#234214,#234215),(#234216,#234217),(#234218,#234219),
(#234220,#234221),(#234222,#234223),(#234224,#234225),(#234226,#234227),
(#234228,#234229),(#234230,#234231)),.UNSPECIFIED.,.F.,.F.,.F.,(6,1,1,1,
1,1,1,1,1,1,1,1,1,1,1,1,1,1,1,1,1,1,1,1,1,1,1,1,1,1,1,1,1,1,1,1,1,1,1,1,
1,1,1,1,1,1,1,1,1,1,1,1,1,1,1,1,1,1,1,1,1,1,1,1,1,1,1,1,1,1,1,1,1,1,1,1,
1,1,1,1,1,1,1,1,1,1,1,1,1,1,1,1,1,1,1,1,1,1,1,1,1,1,1,1,1,1,1,1,1,1,1,1,
1,1,1,1,1,1,1,1,1,1,1,1,1,1,1,1,1,1,1,1,1,1,1,1,1,1,1,1,1,1,1,1,1,1,1,1,
1,1,1,1,1,1,1,1,1,1,1,1,1,1,1,1,1,1,1,1,1,1,1,1,1,1,1,1,1,1,1,1,1,1,1,1,
1,1,1,1,1,1,1,1,1,1,1,1,1,1,1,1,1,1,1,1,1,1,1,1,1,1,1,1,1,1,1,1,1,1,1,1,
1,1,1,1,1,1,1,1,1,1,1,1,1,1,1,1,1,1,1,1,1,1,1,1,1,1,1,1,1,1,1,1,1,1,1,1,
1,1,1,1,1,1,1,1,1,1,1,1,1,1,1,1,1,1,1,1,1,1,1,1,1,1,1,1,1,1,1,1,1,1,1,1,
1,1,1,1,1,1,1,1,1,1,1,1,1,1,1,1,1,1,1,1,1,1,1,1,1,1,1,1,1,1,1,1,1,1,1,1,
1,1,1,1,1,1,1,1,1,1,1,1,1,1,1,1,1,1,1,1,1,1,1,1,1,1,1,1,1,1,1,1,1,1,1,1,
1,1,1,1,1,1,1,1,1,1,1,1,1,1,1,1,1,1,1,1,1,1,1,1,1,1,1,1,1,1,1,1,1,1,1,1,
1,1,1,1,1,1,1,1,1,1,1,1,1,1,1,1,1,1,1,1,1,1,1,1,1,1,1,1,1,1,1,1,1,1,1,1,
1,1,1,1,1,1,1,1,1,1,1,1,1,1,1,1,1,1,1,1,1,1,1,1,1,1,1,1,1,1,1,6),(2,2),
(0.143172104,0.144954128,0.146788991,0.148623853,0.150458716,0.152293578,
0.15412844,0.155963303,0.157798165,0.159633028,0.16146789,0.163302752,0.165137615,
0.166972477,0.168807339,0.170642202,0.172477064,0.174311927,0.176146789,
0.177981651,0.179816514,0.181651376,0.183486239,0.185321101,0.187155963,
0.188990826,0.190825688,0.19266055,0.194495413,0.196330275,0.198165138,
0.2,0.201834862,0.203669725,0.205504587,0.20733945,0.209174312,0.211009174,
0.212844037,0.214678899,0.216513761,0.218348624,0.220183486,0.222018349,
0.223853211,0.225688073,0.227522936,0.229357798,0.231192661,0.233027523,
0.234862385,0.236697248,0.23853211,0.240366972,0.242201835,0.244036697,
0.24587156,0.247706422,0.249541284,0.251376147,0.253211009,0.255045872,
0.256880734,0.258715596,0.260550459,0.262385321,0.264220183,0.266055046,
0.267889908,0.269724771,0.271559633,0.273394495,0.275229358,0.27706422,
0.278899083,0.280733945,0.282568807,0.28440367,0.286238532,0.288073394,
0.289908257,0.291743119,0.293577982,0.295412844,0.297247706,0.299082569,
0.300917431,0.302752294,0.304587156,0.306422018,0.308256881,0.310091743,
0.311926606,0.313761468,0.31559633,0.317431193,0.319266055,0.321100917,
0.32293578,0.324770642,0.326605505,0.328440367,0.330275229,0.332110092,
0.333944954,0.335779817,0.337614679,0.339449541,0.341284404,0.343119266,
0.344954128,0.346788991,0.348623853,0.350458716,0.352293578,0.35412844,
0.355963303,0.357798165,0.359633028,0.36146789,0.363302752,0.365137615,
0.366972477,0.368807339,0.370642202,0.372477064,0.374311927,0.376146789,
0.377981651,0.379816514,0.381651376,0.383486239,0.385321101,0.387155963,
0.388990826,0.390825688,0.39266055,0.394495413,0.396330275,0.398165138,
0.4,0.401834862,0.403669725,0.405504587,0.40733945,0.409174312,0.411009174,
0.412844037,0.414678899,0.416513761,0.418348624,0.420183486,0.422018349,
0.423853211,0.425688073,0.427522936,0.429357798,0.431192661,0.433027523,
0.434862385,0.436697248,0.43853211,0.440366972,0.442201835,0.444036697,
0.44587156,0.447706422,0.449541284,0.451376147,0.453211009,0.455045872,
0.456880734,0.458715596,0.460550459,0.462385321,0.464220183,0.466055046,
0.467889908,0.469724771,0.471559633,0.473394495,0.475229358,0.47706422,
0.478899083,0.480733945,0.482568807,0.48440367,0.486238532,0.488073394,
0.489908257,0.491743119,0.493577982,0.495412844,0.497247706,0.499082569,
0.500917431,0.502752294,0.504587156,0.506422018,0.508256881,0.510091743,
0.511926606,0.513761468,0.51559633,0.517431193,0.519266055,0.521100917,
0.52293578,0.524770642,0.526605505,0.528440367,0.530275229,0.532110092,
0.533944954,0.535779817,0.537614679,0.539449541,0.541284404,0.543119266,
0.544954128,0.546788991,0.548623853,0.550458716,0.552293578,0.55412844,
0.555963303,0.557798165,0.559633028,0.56146789,0.563302752,0.565137615,
0.566972477,0.568807339,0.570642202,0.572477064,0.574311927,0.576146789,
0.577981651,0.579816514,0.581651376,0.583486239,0.585321101,0.587155963,
0.588990826,0.590825688,0.59266055,0.594495413,0.596330275,0.598165138,
0.6,0.601834862,0.603669725,0.605504587,0.60733945,0.609174312,0.611009174,
0.612844037,0.614678899,0.616513761,0.618348624,0.620183486,0.622018349,
0.623853211,0.625688073,0.627522936,0.629357798,0.631192661,0.633027523,
0.634862385,0.636697248,0.63853211,0.640366972,0.642201835,0.644036697,
0.64587156,0.647706422,0.649541284,0.651376147,0.653211009,0.655045872,
0.656880734,0.658715596,0.660550459,0.662385321,0.664220183,0.666055046,
0.667889908,0.669724771,0.671559633,0.673394495,0.675229358,0.67706422,
0.678899083,0.680733945,0.682568807,0.68440367,0.686238532,0.688073394,
0.689908257,0.691743119,0.693577982,0.695412844,0.697247706,0.699082569,
0.700917431,0.702752294,0.704587156,0.706422018,0.708256881,0.710091743,
0.711926606,0.713761468,0.71559633,0.717431193,0.719266055,0.721100917,
0.72293578,0.724770642,0.726605505,0.728440367,0.730275229,0.732110092,
0.733944954,0.735779817,0.737614679,0.739449541,0.741284404,0.743119266,
0.744954128,0.746788991,0.748623853,0.750458716,0.752293578,0.75412844,
0.755963303,0.757798165,0.759633028,0.76146789,0.763302752,0.765137615,
0.766972477,0.768807339,0.770642202,0.772477064,0.774311927,0.776146789,
0.777981651,0.779816514,0.781651376,0.783486239,0.785321101,0.787155963,
0.788990826,0.790825688,0.79266055,0.794495413,0.796330275,0.798165138,
0.8,0.801834862,0.803669725,0.805504587,0.80733945,0.809174312,0.811009174,
0.812844037,0.814678899,0.816513761,0.818348624,0.820183486,0.822018349,
0.823853211,0.825688073,0.827522936,0.829357798,0.831192661,0.833027523,
0.834862385,0.836697248,0.83853211,0.840366972,0.842201835,0.844036697,
0.84587156,0.847706422,0.849541284,0.851376147,0.853211009,0.855045872,
0.856880734,0.858715596,0.860550459,0.862385321,0.864220183,0.866055046,
0.867889908,0.869724771,0.871559633,0.873394495,0.875229358,0.87706422,
0.878899083,0.880733945,0.882568807,0.88440367,0.886238532,0.888073394,
0.889908257,0.891743119,0.893577982,0.895412844,0.897247706,0.899082569,
0.900917431,0.902752294,0.904587156,0.906422018,0.908256881,0.910091743,
0.911926606,0.913761468,0.91559633,0.917431193,0.919266055,0.921100917,
0.92293578,0.924770642,0.926605505,0.928440367,0.930275229,0.932110092,
0.933944954,0.935779817,0.937614679,0.939449541,0.941284404,0.943119266,
0.944954128,0.946788991,0.948623853,0.950458716,0.952293578,0.95412844,
0.955963303,0.957798165,0.959633028,0.96146789,0.963302752,0.965137615,
0.966972477,0.968807339,0.970642202,0.972477064,0.974311927,0.976146789,
0.977981651,0.979816514,0.981651376,0.983486239,0.985321101,0.987155963,
0.988990826,0.990825688,0.99266055,0.994495413,0.996330275,0.998165138,
1.),(0.,0.36),.UNSPECIFIED.);
#6264=B_SPLINE_SURFACE_WITH_KNOTS('',5,1,((#234870,#234871),(#234872,#234873),
(#234874,#234875),(#234876,#234877),(#234878,#234879),(#234880,#234881),
(#234882,#234883),(#234884,#234885),(#234886,#234887),(#234888,#234889),
(#234890,#234891),(#234892,#234893),(#234894,#234895),(#234896,#234897),
(#234898,#234899),(#234900,#234901),(#234902,#234903),(#234904,#234905),
(#234906,#234907),(#234908,#234909),(#234910,#234911),(#234912,#234913),
(#234914,#234915),(#234916,#234917),(#234918,#234919),(#234920,#234921),
(#234922,#234923),(#234924,#234925),(#234926,#234927),(#234928,#234929),
(#234930,#234931),(#234932,#234933),(#234934,#234935),(#234936,#234937),
(#234938,#234939),(#234940,#234941),(#234942,#234943),(#234944,#234945),
(#234946,#234947),(#234948,#234949),(#234950,#234951),(#234952,#234953),
(#234954,#234955),(#234956,#234957),(#234958,#234959),(#234960,#234961),
(#234962,#234963),(#234964,#234965),(#234966,#234967),(#234968,#234969),
(#234970,#234971),(#234972,#234973),(#234974,#234975),(#234976,#234977),
(#234978,#234979),(#234980,#234981),(#234982,#234983),(#234984,#234985),
(#234986,#234987),(#234988,#234989),(#234990,#234991),(#234992,#234993),
(#234994,#234995),(#234996,#234997),(#234998,#234999),(#235000,#235001),
(#235002,#235003),(#235004,#235005),(#235006,#235007),(#235008,#235009),
(#235010,#235011),(#235012,#235013),(#235014,#235015),(#235016,#235017),
(#235018,#235019),(#235020,#235021),(#235022,#235023),(#235024,#235025),
(#235026,#235027),(#235028,#235029),(#235030,#235031),(#235032,#235033),
(#235034,#235035),(#235036,#235037),(#235038,#235039),(#235040,#235041),
(#235042,#235043),(#235044,#235045),(#235046,#235047),(#235048,#235049),
(#235050,#235051),(#235052,#235053),(#235054,#235055),(#235056,#235057),
(#235058,#235059),(#235060,#235061),(#235062,#235063),(#235064,#235065),
(#235066,#235067),(#235068,#235069),(#235070,#235071),(#235072,#235073),
(#235074,#235075),(#235076,#235077),(#235078,#235079),(#235080,#235081),
(#235082,#235083),(#235084,#235085),(#235086,#235087),(#235088,#235089),
(#235090,#235091),(#235092,#235093),(#235094,#235095),(#235096,#235097),
(#235098,#235099),(#235100,#235101),(#235102,#235103),(#235104,#235105),
(#235106,#235107),(#235108,#235109),(#235110,#235111),(#235112,#235113),
(#235114,#235115),(#235116,#235117),(#235118,#235119),(#235120,#235121),
(#235122,#235123),(#235124,#235125),(#235126,#235127),(#235128,#235129),
(#235130,#235131),(#235132,#235133),(#235134,#235135),(#235136,#235137),
(#235138,#235139),(#235140,#235141),(#235142,#235143),(#235144,#235145),
(#235146,#235147),(#235148,#235149),(#235150,#235151),(#235152,#235153),
(#235154,#235155),(#235156,#235157),(#235158,#235159),(#235160,#235161),
(#235162,#235163),(#235164,#235165),(#235166,#235167),(#235168,#235169),
(#235170,#235171),(#235172,#235173),(#235174,#235175),(#235176,#235177),
(#235178,#235179),(#235180,#235181),(#235182,#235183),(#235184,#235185),
(#235186,#235187),(#235188,#235189),(#235190,#235191),(#235192,#235193),
(#235194,#235195),(#235196,#235197),(#235198,#235199),(#235200,#235201),
(#235202,#235203),(#235204,#235205),(#235206,#235207),(#235208,#235209),
(#235210,#235211),(#235212,#235213),(#235214,#235215),(#235216,#235217),
(#235218,#235219),(#235220,#235221),(#235222,#235223),(#235224,#235225),
(#235226,#235227),(#235228,#235229),(#235230,#235231),(#235232,#235233),
(#235234,#235235),(#235236,#235237),(#235238,#235239),(#235240,#235241),
(#235242,#235243),(#235244,#235245),(#235246,#235247),(#235248,#235249),
(#235250,#235251),(#235252,#235253),(#235254,#235255),(#235256,#235257),
(#235258,#235259),(#235260,#235261),(#235262,#235263),(#235264,#235265),
(#235266,#235267),(#235268,#235269),(#235270,#235271),(#235272,#235273),
(#235274,#235275),(#235276,#235277),(#235278,#235279),(#235280,#235281),
(#235282,#235283),(#235284,#235285),(#235286,#235287),(#235288,#235289),
(#235290,#235291),(#235292,#235293),(#235294,#235295),(#235296,#235297),
(#235298,#235299),(#235300,#235301),(#235302,#235303),(#235304,#235305),
(#235306,#235307),(#235308,#235309),(#235310,#235311),(#235312,#235313),
(#235314,#235315),(#235316,#235317),(#235318,#235319),(#235320,#235321),
(#235322,#235323),(#235324,#235325),(#235326,#235327),(#235328,#235329),
(#235330,#235331),(#235332,#235333),(#235334,#235335),(#235336,#235337),
(#235338,#235339),(#235340,#235341),(#235342,#235343),(#235344,#235345),
(#235346,#235347),(#235348,#235349),(#235350,#235351),(#235352,#235353),
(#235354,#235355),(#235356,#235357),(#235358,#235359),(#235360,#235361),
(#235362,#235363),(#235364,#235365),(#235366,#235367),(#235368,#235369),
(#235370,#235371),(#235372,#235373),(#235374,#235375),(#235376,#235377),
(#235378,#235379),(#235380,#235381),(#235382,#235383),(#235384,#235385),
(#235386,#235387),(#235388,#235389),(#235390,#235391),(#235392,#235393),
(#235394,#235395),(#235396,#235397),(#235398,#235399),(#235400,#235401),
(#235402,#235403),(#235404,#235405),(#235406,#235407),(#235408,#235409),
(#235410,#235411),(#235412,#235413),(#235414,#235415),(#235416,#235417),
(#235418,#235419),(#235420,#235421),(#235422,#235423),(#235424,#235425),
(#235426,#235427),(#235428,#235429),(#235430,#235431),(#235432,#235433),
(#235434,#235435),(#235436,#235437),(#235438,#235439),(#235440,#235441),
(#235442,#235443),(#235444,#235445),(#235446,#235447),(#235448,#235449),
(#235450,#235451),(#235452,#235453),(#235454,#235455),(#235456,#235457),
(#235458,#235459),(#235460,#235461),(#235462,#235463),(#235464,#235465),
(#235466,#235467),(#235468,#235469),(#235470,#235471),(#235472,#235473),
(#235474,#235475),(#235476,#235477),(#235478,#235479),(#235480,#235481),
(#235482,#235483),(#235484,#235485),(#235486,#235487),(#235488,#235489),
(#235490,#235491),(#235492,#235493),(#235494,#235495),(#235496,#235497),
(#235498,#235499),(#235500,#235501),(#235502,#235503),(#235504,#235505),
(#235506,#235507),(#235508,#235509),(#235510,#235511),(#235512,#235513),
(#235514,#235515),(#235516,#235517),(#235518,#235519),(#235520,#235521),
(#235522,#235523),(#235524,#235525),(#235526,#235527),(#235528,#235529),
(#235530,#235531),(#235532,#235533),(#235534,#235535),(#235536,#235537),
(#235538,#235539),(#235540,#235541),(#235542,#235543),(#235544,#235545),
(#235546,#235547),(#235548,#235549),(#235550,#235551),(#235552,#235553),
(#235554,#235555),(#235556,#235557),(#235558,#235559),(#235560,#235561),
(#235562,#235563),(#235564,#235565),(#235566,#235567),(#235568,#235569),
(#235570,#235571),(#235572,#235573),(#235574,#235575),(#235576,#235577),
(#235578,#235579),(#235580,#235581),(#235582,#235583),(#235584,#235585),
(#235586,#235587),(#235588,#235589),(#235590,#235591),(#235592,#235593),
(#235594,#235595),(#235596,#235597),(#235598,#235599),(#235600,#235601),
(#235602,#235603),(#235604,#235605),(#235606,#235607),(#235608,#235609),
(#235610,#235611),(#235612,#235613),(#235614,#235615),(#235616,#235617),
(#235618,#235619),(#235620,#235621),(#235622,#235623),(#235624,#235625),
(#235626,#235627),(#235628,#235629),(#235630,#235631),(#235632,#235633),
(#235634,#235635),(#235636,#235637),(#235638,#235639),(#235640,#235641),
(#235642,#235643),(#235644,#235645),(#235646,#235647),(#235648,#235649),
(#235650,#235651),(#235652,#235653),(#235654,#235655),(#235656,#235657),
(#235658,#235659),(#235660,#235661),(#235662,#235663),(#235664,#235665),
(#235666,#235667),(#235668,#235669),(#235670,#235671),(#235672,#235673),
(#235674,#235675),(#235676,#235677),(#235678,#235679),(#235680,#235681),
(#235682,#235683),(#235684,#235685),(#235686,#235687),(#235688,#235689),
(#235690,#235691),(#235692,#235693),(#235694,#235695),(#235696,#235697),
(#235698,#235699),(#235700,#235701),(#235702,#235703),(#235704,#235705),
(#235706,#235707),(#235708,#235709),(#235710,#235711),(#235712,#235713),
(#235714,#235715),(#235716,#235717),(#235718,#235719),(#235720,#235721),
(#235722,#235723),(#235724,#235725),(#235726,#235727),(#235728,#235729),
(#235730,#235731),(#235732,#235733),(#235734,#235735),(#235736,#235737),
(#235738,#235739),(#235740,#235741),(#235742,#235743),(#235744,#235745),
(#235746,#235747),(#235748,#235749),(#235750,#235751),(#235752,#235753),
(#235754,#235755),(#235756,#235757),(#235758,#235759),(#235760,#235761),
(#235762,#235763),(#235764,#235765),(#235766,#235767),(#235768,#235769),
(#235770,#235771),(#235772,#235773),(#235774,#235775),(#235776,#235777),
(#235778,#235779),(#235780,#235781),(#235782,#235783),(#235784,#235785),
(#235786,#235787),(#235788,#235789),(#235790,#235791),(#235792,#235793),
(#235794,#235795),(#235796,#235797),(#235798,#235799),(#235800,#235801),
(#235802,#235803),(#235804,#235805),(#235806,#235807),(#235808,#235809),
(#235810,#235811),(#235812,#235813)),.UNSPECIFIED.,.F.,.F.,.F.,(6,1,1,1,
1,1,1,1,1,1,1,1,1,1,1,1,1,1,1,1,1,1,1,1,1,1,1,1,1,1,1,1,1,1,1,1,1,1,1,1,
1,1,1,1,1,1,1,1,1,1,1,1,1,1,1,1,1,1,1,1,1,1,1,1,1,1,1,1,1,1,1,1,1,1,1,1,
1,1,1,1,1,1,1,1,1,1,1,1,1,1,1,1,1,1,1,1,1,1,1,1,1,1,1,1,1,1,1,1,1,1,1,1,
1,1,1,1,1,1,1,1,1,1,1,1,1,1,1,1,1,1,1,1,1,1,1,1,1,1,1,1,1,1,1,1,1,1,1,1,
1,1,1,1,1,1,1,1,1,1,1,1,1,1,1,1,1,1,1,1,1,1,1,1,1,1,1,1,1,1,1,1,1,1,1,1,
1,1,1,1,1,1,1,1,1,1,1,1,1,1,1,1,1,1,1,1,1,1,1,1,1,1,1,1,1,1,1,1,1,1,1,1,
1,1,1,1,1,1,1,1,1,1,1,1,1,1,1,1,1,1,1,1,1,1,1,1,1,1,1,1,1,1,1,1,1,1,1,1,
1,1,1,1,1,1,1,1,1,1,1,1,1,1,1,1,1,1,1,1,1,1,1,1,1,1,1,1,1,1,1,1,1,1,1,1,
1,1,1,1,1,1,1,1,1,1,1,1,1,1,1,1,1,1,1,1,1,1,1,1,1,1,1,1,1,1,1,1,1,1,1,1,
1,1,1,1,1,1,1,1,1,1,1,1,1,1,1,1,1,1,1,1,1,1,1,1,1,1,1,1,1,1,1,1,1,1,1,1,
1,1,1,1,1,1,1,1,1,1,1,1,1,1,1,1,1,1,1,1,1,1,1,1,1,1,1,1,1,1,1,1,1,1,1,1,
1,1,1,1,1,1,1,1,1,1,1,1,1,1,1,1,1,1,1,1,1,1,1,1,1,1,1,1,1,1,1,1,1,1,1,1,
1,1,1,1,1,1,1,1,1,1,1,1,1,1,1,1,1,1,1,1,1,1,1,1,1,1,1,1,1,1,1,6),(2,2),
(-1.,-0.998165138,-0.996330275,-0.994495413,-0.99266055,-0.990825688,-0.988990826,
-0.987155963,-0.985321101,-0.983486239,-0.981651376,-0.979816514,-0.977981651,
-0.976146789,-0.974311927,-0.972477064,-0.970642202,-0.968807339,-0.966972477,
-0.965137615,-0.963302752,-0.96146789,-0.959633028,-0.957798165,-0.955963303,
-0.95412844,-0.952293578,-0.950458716,-0.948623853,-0.946788991,-0.944954128,
-0.943119266,-0.941284404,-0.939449541,-0.937614679,-0.935779817,-0.933944954,
-0.932110092,-0.930275229,-0.928440367,-0.926605505,-0.924770642,-0.92293578,
-0.921100917,-0.919266055,-0.917431193,-0.91559633,-0.913761468,-0.911926606,
-0.910091743,-0.908256881,-0.906422018,-0.904587156,-0.902752294,-0.900917431,
-0.899082569,-0.897247706,-0.895412844,-0.893577982,-0.891743119,-0.889908257,
-0.888073394,-0.886238532,-0.88440367,-0.882568807,-0.880733945,-0.878899083,
-0.87706422,-0.875229358,-0.873394495,-0.871559633,-0.869724771,-0.867889908,
-0.866055046,-0.864220183,-0.862385321,-0.860550459,-0.858715596,-0.856880734,
-0.855045872,-0.853211009,-0.851376147,-0.849541284,-0.847706422,-0.84587156,
-0.844036697,-0.842201835,-0.840366972,-0.83853211,-0.836697248,-0.834862385,
-0.833027523,-0.831192661,-0.829357798,-0.827522936,-0.825688073,-0.823853211,
-0.822018349,-0.820183486,-0.818348624,-0.816513761,-0.814678899,-0.812844037,
-0.811009174,-0.809174312,-0.80733945,-0.805504587,-0.803669725,-0.801834862,
-0.8,-0.798165138,-0.796330275,-0.794495413,-0.79266055,-0.790825688,-0.788990826,
-0.787155963,-0.785321101,-0.783486239,-0.781651376,-0.779816514,-0.777981651,
-0.776146789,-0.774311927,-0.772477064,-0.770642202,-0.768807339,-0.766972477,
-0.765137615,-0.763302752,-0.76146789,-0.759633028,-0.757798165,-0.755963303,
-0.75412844,-0.752293578,-0.750458716,-0.748623853,-0.746788991,-0.744954128,
-0.743119266,-0.741284404,-0.739449541,-0.737614679,-0.735779817,-0.733944954,
-0.732110092,-0.730275229,-0.728440367,-0.726605505,-0.724770642,-0.72293578,
-0.721100917,-0.719266055,-0.717431193,-0.71559633,-0.713761468,-0.711926606,
-0.710091743,-0.708256881,-0.706422018,-0.704587156,-0.702752294,-0.700917431,
-0.699082569,-0.697247706,-0.695412844,-0.693577982,-0.691743119,-0.689908257,
-0.688073394,-0.686238532,-0.68440367,-0.682568807,-0.680733945,-0.678899083,
-0.67706422,-0.675229358,-0.673394495,-0.671559633,-0.669724771,-0.667889908,
-0.666055046,-0.664220183,-0.662385321,-0.660550459,-0.658715596,-0.656880734,
-0.655045872,-0.653211009,-0.651376147,-0.649541284,-0.647706422,-0.64587156,
-0.644036697,-0.642201835,-0.640366972,-0.63853211,-0.636697248,-0.634862385,
-0.633027523,-0.631192661,-0.629357798,-0.627522936,-0.625688073,-0.623853211,
-0.622018349,-0.620183486,-0.618348624,-0.616513761,-0.614678899,-0.612844037,
-0.611009174,-0.609174312,-0.60733945,-0.605504587,-0.603669725,-0.601834862,
-0.6,-0.598165138,-0.596330275,-0.594495413,-0.59266055,-0.590825688,-0.588990826,
-0.587155963,-0.585321101,-0.583486239,-0.581651376,-0.579816514,-0.577981651,
-0.576146789,-0.574311927,-0.572477064,-0.570642202,-0.568807339,-0.566972477,
-0.565137615,-0.563302752,-0.56146789,-0.559633028,-0.557798165,-0.555963303,
-0.55412844,-0.552293578,-0.550458716,-0.548623853,-0.546788991,-0.544954128,
-0.543119266,-0.541284404,-0.539449541,-0.537614679,-0.535779817,-0.533944954,
-0.532110092,-0.530275229,-0.528440367,-0.526605505,-0.524770642,-0.52293578,
-0.521100917,-0.519266055,-0.517431193,-0.51559633,-0.513761468,-0.511926606,
-0.510091743,-0.508256881,-0.506422018,-0.504587156,-0.502752294,-0.500917431,
-0.499082569,-0.497247706,-0.495412844,-0.493577982,-0.491743119,-0.489908257,
-0.488073394,-0.486238532,-0.48440367,-0.482568807,-0.480733945,-0.478899083,
-0.47706422,-0.475229358,-0.473394495,-0.471559633,-0.469724771,-0.467889908,
-0.466055046,-0.464220183,-0.462385321,-0.460550459,-0.458715596,-0.456880734,
-0.455045872,-0.453211009,-0.451376147,-0.449541284,-0.447706422,-0.44587156,
-0.444036697,-0.442201835,-0.440366972,-0.43853211,-0.436697248,-0.434862385,
-0.433027523,-0.431192661,-0.429357798,-0.427522936,-0.425688073,-0.423853211,
-0.422018349,-0.420183486,-0.418348624,-0.416513761,-0.414678899,-0.412844037,
-0.411009174,-0.409174312,-0.40733945,-0.405504587,-0.403669725,-0.401834862,
-0.4,-0.398165138,-0.396330275,-0.394495413,-0.39266055,-0.390825688,-0.388990826,
-0.387155963,-0.385321101,-0.383486239,-0.381651376,-0.379816514,-0.377981651,
-0.376146789,-0.374311927,-0.372477064,-0.370642202,-0.368807339,-0.366972477,
-0.365137615,-0.363302752,-0.36146789,-0.359633028,-0.357798165,-0.355963303,
-0.35412844,-0.352293578,-0.350458716,-0.348623853,-0.346788991,-0.344954128,
-0.343119266,-0.341284404,-0.339449541,-0.337614679,-0.335779817,-0.333944954,
-0.332110092,-0.330275229,-0.328440367,-0.326605505,-0.324770642,-0.32293578,
-0.321100917,-0.319266055,-0.317431193,-0.31559633,-0.313761468,-0.311926606,
-0.310091743,-0.308256881,-0.306422018,-0.304587156,-0.302752294,-0.300917431,
-0.299082569,-0.297247706,-0.295412844,-0.293577982,-0.291743119,-0.289908257,
-0.288073394,-0.286238532,-0.28440367,-0.282568807,-0.280733945,-0.278899083,
-0.27706422,-0.275229358,-0.273394495,-0.271559633,-0.269724771,-0.267889908,
-0.266055046,-0.264220183,-0.262385321,-0.260550459,-0.258715596,-0.256880734,
-0.255045872,-0.253211009,-0.251376147,-0.249541284,-0.247706422,-0.24587156,
-0.244036697,-0.242201835,-0.240366972,-0.23853211,-0.236697248,-0.234862385,
-0.233027523,-0.231192661,-0.229357798,-0.227522936,-0.225688073,-0.223853211,
-0.222018349,-0.220183486,-0.218348624,-0.216513761,-0.214678899,-0.212844037,
-0.211009174,-0.209174312,-0.20733945,-0.205504587,-0.203669725,-0.201834862,
-0.2,-0.198165138,-0.196330275,-0.194495413,-0.19266055,-0.190825688,-0.188990826,
-0.187155963,-0.185321101,-0.183486239,-0.181651376,-0.179816514,-0.177981651,
-0.176146789,-0.174311927,-0.172477064,-0.170642202,-0.168807339,-0.166972477,
-0.165137615,-0.163302752,-0.16146789,-0.159633028,-0.157798165,-0.155963303,
-0.15412844,-0.152293578,-0.150458716,-0.148623853,-0.146788991,-0.144954128,
-0.143172104),(0.,0.36),.UNSPECIFIED.);
#6265=B_SPLINE_SURFACE_WITH_KNOTS('',5,1,((#236446,#236447),(#236448,#236449),
(#236450,#236451),(#236452,#236453),(#236454,#236455),(#236456,#236457),
(#236458,#236459),(#236460,#236461),(#236462,#236463),(#236464,#236465),
(#236466,#236467),(#236468,#236469),(#236470,#236471),(#236472,#236473),
(#236474,#236475),(#236476,#236477),(#236478,#236479),(#236480,#236481),
(#236482,#236483),(#236484,#236485),(#236486,#236487),(#236488,#236489),
(#236490,#236491),(#236492,#236493),(#236494,#236495),(#236496,#236497),
(#236498,#236499),(#236500,#236501),(#236502,#236503),(#236504,#236505),
(#236506,#236507),(#236508,#236509),(#236510,#236511),(#236512,#236513),
(#236514,#236515),(#236516,#236517),(#236518,#236519),(#236520,#236521),
(#236522,#236523),(#236524,#236525),(#236526,#236527),(#236528,#236529),
(#236530,#236531),(#236532,#236533),(#236534,#236535),(#236536,#236537),
(#236538,#236539),(#236540,#236541),(#236542,#236543),(#236544,#236545),
(#236546,#236547),(#236548,#236549),(#236550,#236551),(#236552,#236553),
(#236554,#236555),(#236556,#236557),(#236558,#236559),(#236560,#236561),
(#236562,#236563),(#236564,#236565),(#236566,#236567),(#236568,#236569),
(#236570,#236571),(#236572,#236573),(#236574,#236575),(#236576,#236577),
(#236578,#236579),(#236580,#236581),(#236582,#236583),(#236584,#236585),
(#236586,#236587),(#236588,#236589),(#236590,#236591),(#236592,#236593),
(#236594,#236595),(#236596,#236597),(#236598,#236599),(#236600,#236601),
(#236602,#236603),(#236604,#236605),(#236606,#236607),(#236608,#236609),
(#236610,#236611),(#236612,#236613),(#236614,#236615),(#236616,#236617),
(#236618,#236619),(#236620,#236621),(#236622,#236623),(#236624,#236625),
(#236626,#236627),(#236628,#236629),(#236630,#236631),(#236632,#236633),
(#236634,#236635),(#236636,#236637),(#236638,#236639),(#236640,#236641),
(#236642,#236643),(#236644,#236645),(#236646,#236647),(#236648,#236649),
(#236650,#236651),(#236652,#236653),(#236654,#236655),(#236656,#236657),
(#236658,#236659),(#236660,#236661),(#236662,#236663),(#236664,#236665),
(#236666,#236667),(#236668,#236669),(#236670,#236671),(#236672,#236673),
(#236674,#236675),(#236676,#236677),(#236678,#236679),(#236680,#236681),
(#236682,#236683),(#236684,#236685),(#236686,#236687),(#236688,#236689),
(#236690,#236691),(#236692,#236693),(#236694,#236695),(#236696,#236697),
(#236698,#236699),(#236700,#236701),(#236702,#236703),(#236704,#236705),
(#236706,#236707),(#236708,#236709),(#236710,#236711),(#236712,#236713),
(#236714,#236715),(#236716,#236717),(#236718,#236719),(#236720,#236721),
(#236722,#236723),(#236724,#236725),(#236726,#236727),(#236728,#236729),
(#236730,#236731),(#236732,#236733),(#236734,#236735),(#236736,#236737),
(#236738,#236739),(#236740,#236741),(#236742,#236743),(#236744,#236745),
(#236746,#236747),(#236748,#236749),(#236750,#236751),(#236752,#236753),
(#236754,#236755),(#236756,#236757),(#236758,#236759),(#236760,#236761),
(#236762,#236763),(#236764,#236765),(#236766,#236767),(#236768,#236769),
(#236770,#236771),(#236772,#236773),(#236774,#236775),(#236776,#236777),
(#236778,#236779),(#236780,#236781),(#236782,#236783),(#236784,#236785),
(#236786,#236787),(#236788,#236789),(#236790,#236791),(#236792,#236793),
(#236794,#236795),(#236796,#236797),(#236798,#236799),(#236800,#236801),
(#236802,#236803),(#236804,#236805),(#236806,#236807),(#236808,#236809),
(#236810,#236811),(#236812,#236813),(#236814,#236815),(#236816,#236817),
(#236818,#236819),(#236820,#236821),(#236822,#236823),(#236824,#236825),
(#236826,#236827),(#236828,#236829),(#236830,#236831),(#236832,#236833),
(#236834,#236835),(#236836,#236837),(#236838,#236839),(#236840,#236841),
(#236842,#236843),(#236844,#236845),(#236846,#236847),(#236848,#236849),
(#236850,#236851),(#236852,#236853),(#236854,#236855),(#236856,#236857),
(#236858,#236859),(#236860,#236861),(#236862,#236863),(#236864,#236865),
(#236866,#236867),(#236868,#236869),(#236870,#236871),(#236872,#236873),
(#236874,#236875),(#236876,#236877),(#236878,#236879),(#236880,#236881),
(#236882,#236883),(#236884,#236885),(#236886,#236887),(#236888,#236889),
(#236890,#236891),(#236892,#236893),(#236894,#236895),(#236896,#236897),
(#236898,#236899),(#236900,#236901),(#236902,#236903),(#236904,#236905),
(#236906,#236907),(#236908,#236909),(#236910,#236911),(#236912,#236913),
(#236914,#236915),(#236916,#236917),(#236918,#236919),(#236920,#236921),
(#236922,#236923),(#236924,#236925),(#236926,#236927),(#236928,#236929),
(#236930,#236931),(#236932,#236933),(#236934,#236935),(#236936,#236937),
(#236938,#236939),(#236940,#236941),(#236942,#236943),(#236944,#236945),
(#236946,#236947),(#236948,#236949),(#236950,#236951),(#236952,#236953),
(#236954,#236955),(#236956,#236957),(#236958,#236959),(#236960,#236961),
(#236962,#236963),(#236964,#236965),(#236966,#236967),(#236968,#236969),
(#236970,#236971),(#236972,#236973),(#236974,#236975),(#236976,#236977),
(#236978,#236979),(#236980,#236981),(#236982,#236983),(#236984,#236985),
(#236986,#236987),(#236988,#236989),(#236990,#236991),(#236992,#236993),
(#236994,#236995),(#236996,#236997),(#236998,#236999),(#237000,#237001),
(#237002,#237003),(#237004,#237005),(#237006,#237007),(#237008,#237009),
(#237010,#237011),(#237012,#237013),(#237014,#237015),(#237016,#237017),
(#237018,#237019),(#237020,#237021),(#237022,#237023),(#237024,#237025),
(#237026,#237027),(#237028,#237029),(#237030,#237031),(#237032,#237033),
(#237034,#237035),(#237036,#237037),(#237038,#237039),(#237040,#237041),
(#237042,#237043),(#237044,#237045),(#237046,#237047),(#237048,#237049),
(#237050,#237051),(#237052,#237053),(#237054,#237055),(#237056,#237057),
(#237058,#237059),(#237060,#237061),(#237062,#237063),(#237064,#237065),
(#237066,#237067),(#237068,#237069),(#237070,#237071),(#237072,#237073),
(#237074,#237075),(#237076,#237077),(#237078,#237079),(#237080,#237081),
(#237082,#237083),(#237084,#237085),(#237086,#237087),(#237088,#237089),
(#237090,#237091),(#237092,#237093),(#237094,#237095),(#237096,#237097),
(#237098,#237099),(#237100,#237101),(#237102,#237103),(#237104,#237105),
(#237106,#237107),(#237108,#237109),(#237110,#237111),(#237112,#237113),
(#237114,#237115),(#237116,#237117),(#237118,#237119),(#237120,#237121),
(#237122,#237123),(#237124,#237125),(#237126,#237127),(#237128,#237129),
(#237130,#237131),(#237132,#237133),(#237134,#237135),(#237136,#237137),
(#237138,#237139),(#237140,#237141),(#237142,#237143),(#237144,#237145),
(#237146,#237147),(#237148,#237149),(#237150,#237151),(#237152,#237153),
(#237154,#237155),(#237156,#237157),(#237158,#237159),(#237160,#237161),
(#237162,#237163),(#237164,#237165),(#237166,#237167),(#237168,#237169),
(#237170,#237171),(#237172,#237173),(#237174,#237175),(#237176,#237177),
(#237178,#237179),(#237180,#237181),(#237182,#237183),(#237184,#237185),
(#237186,#237187),(#237188,#237189),(#237190,#237191),(#237192,#237193),
(#237194,#237195),(#237196,#237197),(#237198,#237199),(#237200,#237201),
(#237202,#237203),(#237204,#237205),(#237206,#237207),(#237208,#237209),
(#237210,#237211),(#237212,#237213),(#237214,#237215),(#237216,#237217),
(#237218,#237219),(#237220,#237221),(#237222,#237223),(#237224,#237225),
(#237226,#237227),(#237228,#237229),(#237230,#237231),(#237232,#237233),
(#237234,#237235),(#237236,#237237),(#237238,#237239),(#237240,#237241),
(#237242,#237243),(#237244,#237245),(#237246,#237247),(#237248,#237249),
(#237250,#237251),(#237252,#237253),(#237254,#237255),(#237256,#237257),
(#237258,#237259),(#237260,#237261),(#237262,#237263),(#237264,#237265),
(#237266,#237267),(#237268,#237269),(#237270,#237271),(#237272,#237273),
(#237274,#237275),(#237276,#237277),(#237278,#237279),(#237280,#237281),
(#237282,#237283),(#237284,#237285),(#237286,#237287),(#237288,#237289),
(#237290,#237291),(#237292,#237293),(#237294,#237295),(#237296,#237297),
(#237298,#237299),(#237300,#237301),(#237302,#237303),(#237304,#237305),
(#237306,#237307),(#237308,#237309),(#237310,#237311),(#237312,#237313),
(#237314,#237315),(#237316,#237317),(#237318,#237319),(#237320,#237321),
(#237322,#237323),(#237324,#237325),(#237326,#237327),(#237328,#237329),
(#237330,#237331),(#237332,#237333),(#237334,#237335),(#237336,#237337),
(#237338,#237339),(#237340,#237341),(#237342,#237343),(#237344,#237345),
(#237346,#237347),(#237348,#237349),(#237350,#237351),(#237352,#237353),
(#237354,#237355),(#237356,#237357),(#237358,#237359),(#237360,#237361),
(#237362,#237363),(#237364,#237365),(#237366,#237367),(#237368,#237369),
(#237370,#237371),(#237372,#237373),(#237374,#237375),(#237376,#237377),
(#237378,#237379),(#237380,#237381),(#237382,#237383),(#237384,#237385),
(#237386,#237387),(#237388,#237389)),.UNSPECIFIED.,.F.,.F.,.F.,(6,1,1,1,
1,1,1,1,1,1,1,1,1,1,1,1,1,1,1,1,1,1,1,1,1,1,1,1,1,1,1,1,1,1,1,1,1,1,1,1,
1,1,1,1,1,1,1,1,1,1,1,1,1,1,1,1,1,1,1,1,1,1,1,1,1,1,1,1,1,1,1,1,1,1,1,1,
1,1,1,1,1,1,1,1,1,1,1,1,1,1,1,1,1,1,1,1,1,1,1,1,1,1,1,1,1,1,1,1,1,1,1,1,
1,1,1,1,1,1,1,1,1,1,1,1,1,1,1,1,1,1,1,1,1,1,1,1,1,1,1,1,1,1,1,1,1,1,1,1,
1,1,1,1,1,1,1,1,1,1,1,1,1,1,1,1,1,1,1,1,1,1,1,1,1,1,1,1,1,1,1,1,1,1,1,1,
1,1,1,1,1,1,1,1,1,1,1,1,1,1,1,1,1,1,1,1,1,1,1,1,1,1,1,1,1,1,1,1,1,1,1,1,
1,1,1,1,1,1,1,1,1,1,1,1,1,1,1,1,1,1,1,1,1,1,1,1,1,1,1,1,1,1,1,1,1,1,1,1,
1,1,1,1,1,1,1,1,1,1,1,1,1,1,1,1,1,1,1,1,1,1,1,1,1,1,1,1,1,1,1,1,1,1,1,1,
1,1,1,1,1,1,1,1,1,1,1,1,1,1,1,1,1,1,1,1,1,1,1,1,1,1,1,1,1,1,1,1,1,1,1,1,
1,1,1,1,1,1,1,1,1,1,1,1,1,1,1,1,1,1,1,1,1,1,1,1,1,1,1,1,1,1,1,1,1,1,1,1,
1,1,1,1,1,1,1,1,1,1,1,1,1,1,1,1,1,1,1,1,1,1,1,1,1,1,1,1,1,1,1,1,1,1,1,1,
1,1,1,1,1,1,1,1,1,1,1,1,1,1,1,1,1,1,1,1,1,1,1,1,1,1,1,1,1,1,1,1,1,1,1,1,
1,1,1,1,1,1,1,1,1,1,1,1,1,1,1,1,1,1,1,1,1,1,1,1,1,1,1,1,1,1,1,6),(2,2),
(-1.,-0.998165138,-0.996330275,-0.994495413,-0.99266055,-0.990825688,-0.988990826,
-0.987155963,-0.985321101,-0.983486239,-0.981651376,-0.979816514,-0.977981651,
-0.976146789,-0.974311927,-0.972477064,-0.970642202,-0.968807339,-0.966972477,
-0.965137615,-0.963302752,-0.96146789,-0.959633028,-0.957798165,-0.955963303,
-0.95412844,-0.952293578,-0.950458716,-0.948623853,-0.946788991,-0.944954128,
-0.943119266,-0.941284404,-0.939449541,-0.937614679,-0.935779817,-0.933944954,
-0.932110092,-0.930275229,-0.928440367,-0.926605505,-0.924770642,-0.92293578,
-0.921100917,-0.919266055,-0.917431193,-0.91559633,-0.913761468,-0.911926606,
-0.910091743,-0.908256881,-0.906422018,-0.904587156,-0.902752294,-0.900917431,
-0.899082569,-0.897247706,-0.895412844,-0.893577982,-0.891743119,-0.889908257,
-0.888073394,-0.886238532,-0.88440367,-0.882568807,-0.880733945,-0.878899083,
-0.87706422,-0.875229358,-0.873394495,-0.871559633,-0.869724771,-0.867889908,
-0.866055046,-0.864220183,-0.862385321,-0.860550459,-0.858715596,-0.856880734,
-0.855045872,-0.853211009,-0.851376147,-0.849541284,-0.847706422,-0.84587156,
-0.844036697,-0.842201835,-0.840366972,-0.83853211,-0.836697248,-0.834862385,
-0.833027523,-0.831192661,-0.829357798,-0.827522936,-0.825688073,-0.823853211,
-0.822018349,-0.820183486,-0.818348624,-0.816513761,-0.814678899,-0.812844037,
-0.811009174,-0.809174312,-0.80733945,-0.805504587,-0.803669725,-0.801834862,
-0.8,-0.798165138,-0.796330275,-0.794495413,-0.79266055,-0.790825688,-0.788990826,
-0.787155963,-0.785321101,-0.783486239,-0.781651376,-0.779816514,-0.777981651,
-0.776146789,-0.774311927,-0.772477064,-0.770642202,-0.768807339,-0.766972477,
-0.765137615,-0.763302752,-0.76146789,-0.759633028,-0.757798165,-0.755963303,
-0.75412844,-0.752293578,-0.750458716,-0.748623853,-0.746788991,-0.744954128,
-0.743119266,-0.741284404,-0.739449541,-0.737614679,-0.735779817,-0.733944954,
-0.732110092,-0.730275229,-0.728440367,-0.726605505,-0.724770642,-0.72293578,
-0.721100917,-0.719266055,-0.717431193,-0.71559633,-0.713761468,-0.711926606,
-0.710091743,-0.708256881,-0.706422018,-0.704587156,-0.702752294,-0.700917431,
-0.699082569,-0.697247706,-0.695412844,-0.693577982,-0.691743119,-0.689908257,
-0.688073394,-0.686238532,-0.68440367,-0.682568807,-0.680733945,-0.678899083,
-0.67706422,-0.675229358,-0.673394495,-0.671559633,-0.669724771,-0.667889908,
-0.666055046,-0.664220183,-0.662385321,-0.660550459,-0.658715596,-0.656880734,
-0.655045872,-0.653211009,-0.651376147,-0.649541284,-0.647706422,-0.64587156,
-0.644036697,-0.642201835,-0.640366972,-0.63853211,-0.636697248,-0.634862385,
-0.633027523,-0.631192661,-0.629357798,-0.627522936,-0.625688073,-0.623853211,
-0.622018349,-0.620183486,-0.618348624,-0.616513761,-0.614678899,-0.612844037,
-0.611009174,-0.609174312,-0.60733945,-0.605504587,-0.603669725,-0.601834862,
-0.6,-0.598165138,-0.596330275,-0.594495413,-0.59266055,-0.590825688,-0.588990826,
-0.587155963,-0.585321101,-0.583486239,-0.581651376,-0.579816514,-0.577981651,
-0.576146789,-0.574311927,-0.572477064,-0.570642202,-0.568807339,-0.566972477,
-0.565137615,-0.563302752,-0.56146789,-0.559633028,-0.557798165,-0.555963303,
-0.55412844,-0.552293578,-0.550458716,-0.548623853,-0.546788991,-0.544954128,
-0.543119266,-0.541284404,-0.539449541,-0.537614679,-0.535779817,-0.533944954,
-0.532110092,-0.530275229,-0.528440367,-0.526605505,-0.524770642,-0.52293578,
-0.521100917,-0.519266055,-0.517431193,-0.51559633,-0.513761468,-0.511926606,
-0.510091743,-0.508256881,-0.506422018,-0.504587156,-0.502752294,-0.500917431,
-0.499082569,-0.497247706,-0.495412844,-0.493577982,-0.491743119,-0.489908257,
-0.488073394,-0.486238532,-0.48440367,-0.482568807,-0.480733945,-0.478899083,
-0.47706422,-0.475229358,-0.473394495,-0.471559633,-0.469724771,-0.467889908,
-0.466055046,-0.464220183,-0.462385321,-0.460550459,-0.458715596,-0.456880734,
-0.455045872,-0.453211009,-0.451376147,-0.449541284,-0.447706422,-0.44587156,
-0.444036697,-0.442201835,-0.440366972,-0.43853211,-0.436697248,-0.434862385,
-0.433027523,-0.431192661,-0.429357798,-0.427522936,-0.425688073,-0.423853211,
-0.422018349,-0.420183486,-0.418348624,-0.416513761,-0.414678899,-0.412844037,
-0.411009174,-0.409174312,-0.40733945,-0.405504587,-0.403669725,-0.401834862,
-0.4,-0.398165138,-0.396330275,-0.394495413,-0.39266055,-0.390825688,-0.388990826,
-0.387155963,-0.385321101,-0.383486239,-0.381651376,-0.379816514,-0.377981651,
-0.376146789,-0.374311927,-0.372477064,-0.370642202,-0.368807339,-0.366972477,
-0.365137615,-0.363302752,-0.36146789,-0.359633028,-0.357798165,-0.355963303,
-0.35412844,-0.352293578,-0.350458716,-0.348623853,-0.346788991,-0.344954128,
-0.343119266,-0.341284404,-0.339449541,-0.337614679,-0.335779817,-0.333944954,
-0.332110092,-0.330275229,-0.328440367,-0.326605505,-0.324770642,-0.32293578,
-0.321100917,-0.319266055,-0.317431193,-0.31559633,-0.313761468,-0.311926606,
-0.310091743,-0.308256881,-0.306422018,-0.304587156,-0.302752294,-0.300917431,
-0.299082569,-0.297247706,-0.295412844,-0.293577982,-0.291743119,-0.289908257,
-0.288073394,-0.286238532,-0.28440367,-0.282568807,-0.280733945,-0.278899083,
-0.27706422,-0.275229358,-0.273394495,-0.271559633,-0.269724771,-0.267889908,
-0.266055046,-0.264220183,-0.262385321,-0.260550459,-0.258715596,-0.256880734,
-0.255045872,-0.253211009,-0.251376147,-0.249541284,-0.247706422,-0.24587156,
-0.244036697,-0.242201835,-0.240366972,-0.23853211,-0.236697248,-0.234862385,
-0.233027523,-0.231192661,-0.229357798,-0.227522936,-0.225688073,-0.223853211,
-0.222018349,-0.220183486,-0.218348624,-0.216513761,-0.214678899,-0.212844037,
-0.211009174,-0.209174312,-0.20733945,-0.205504587,-0.203669725,-0.201834862,
-0.2,-0.198165138,-0.196330275,-0.194495413,-0.19266055,-0.190825688,-0.188990826,
-0.187155963,-0.185321101,-0.183486239,-0.181651376,-0.179816514,-0.177981651,
-0.176146789,-0.174311927,-0.172477064,-0.170642202,-0.168807339,-0.166972477,
-0.165137615,-0.163302752,-0.16146789,-0.159633028,-0.157798165,-0.155963303,
-0.15412844,-0.152293578,-0.150458716,-0.148623853,-0.146788991,-0.144954128,
-0.143172103),(0.,0.36),.UNSPECIFIED.);
#6266=B_SPLINE_SURFACE_WITH_KNOTS('',5,1,((#238022,#238023),(#238024,#238025),
(#238026,#238027),(#238028,#238029),(#238030,#238031),(#238032,#238033),
(#238034,#238035),(#238036,#238037),(#238038,#238039),(#238040,#238041),
(#238042,#238043),(#238044,#238045),(#238046,#238047),(#238048,#238049),
(#238050,#238051),(#238052,#238053),(#238054,#238055),(#238056,#238057),
(#238058,#238059),(#238060,#238061),(#238062,#238063),(#238064,#238065),
(#238066,#238067),(#238068,#238069),(#238070,#238071),(#238072,#238073),
(#238074,#238075),(#238076,#238077),(#238078,#238079),(#238080,#238081),
(#238082,#238083),(#238084,#238085),(#238086,#238087),(#238088,#238089),
(#238090,#238091),(#238092,#238093),(#238094,#238095),(#238096,#238097),
(#238098,#238099),(#238100,#238101),(#238102,#238103),(#238104,#238105),
(#238106,#238107),(#238108,#238109),(#238110,#238111),(#238112,#238113),
(#238114,#238115),(#238116,#238117),(#238118,#238119),(#238120,#238121),
(#238122,#238123),(#238124,#238125),(#238126,#238127),(#238128,#238129),
(#238130,#238131),(#238132,#238133),(#238134,#238135),(#238136,#238137),
(#238138,#238139),(#238140,#238141),(#238142,#238143),(#238144,#238145),
(#238146,#238147),(#238148,#238149),(#238150,#238151),(#238152,#238153),
(#238154,#238155),(#238156,#238157),(#238158,#238159),(#238160,#238161),
(#238162,#238163),(#238164,#238165),(#238166,#238167),(#238168,#238169),
(#238170,#238171),(#238172,#238173),(#238174,#238175),(#238176,#238177),
(#238178,#238179),(#238180,#238181),(#238182,#238183),(#238184,#238185),
(#238186,#238187),(#238188,#238189),(#238190,#238191),(#238192,#238193),
(#238194,#238195),(#238196,#238197),(#238198,#238199),(#238200,#238201),
(#238202,#238203),(#238204,#238205),(#238206,#238207),(#238208,#238209),
(#238210,#238211),(#238212,#238213),(#238214,#238215),(#238216,#238217),
(#238218,#238219),(#238220,#238221),(#238222,#238223),(#238224,#238225),
(#238226,#238227),(#238228,#238229),(#238230,#238231),(#238232,#238233),
(#238234,#238235),(#238236,#238237),(#238238,#238239),(#238240,#238241),
(#238242,#238243),(#238244,#238245),(#238246,#238247),(#238248,#238249),
(#238250,#238251),(#238252,#238253),(#238254,#238255),(#238256,#238257),
(#238258,#238259),(#238260,#238261),(#238262,#238263),(#238264,#238265),
(#238266,#238267),(#238268,#238269),(#238270,#238271),(#238272,#238273),
(#238274,#238275),(#238276,#238277),(#238278,#238279),(#238280,#238281),
(#238282,#238283),(#238284,#238285),(#238286,#238287),(#238288,#238289),
(#238290,#238291),(#238292,#238293),(#238294,#238295),(#238296,#238297),
(#238298,#238299),(#238300,#238301),(#238302,#238303),(#238304,#238305),
(#238306,#238307),(#238308,#238309),(#238310,#238311),(#238312,#238313),
(#238314,#238315),(#238316,#238317),(#238318,#238319),(#238320,#238321),
(#238322,#238323),(#238324,#238325),(#238326,#238327),(#238328,#238329),
(#238330,#238331),(#238332,#238333),(#238334,#238335),(#238336,#238337),
(#238338,#238339),(#238340,#238341),(#238342,#238343),(#238344,#238345),
(#238346,#238347),(#238348,#238349),(#238350,#238351),(#238352,#238353),
(#238354,#238355),(#238356,#238357),(#238358,#238359),(#238360,#238361),
(#238362,#238363),(#238364,#238365),(#238366,#238367),(#238368,#238369),
(#238370,#238371),(#238372,#238373),(#238374,#238375),(#238376,#238377),
(#238378,#238379),(#238380,#238381),(#238382,#238383),(#238384,#238385),
(#238386,#238387),(#238388,#238389),(#238390,#238391),(#238392,#238393),
(#238394,#238395),(#238396,#238397),(#238398,#238399),(#238400,#238401),
(#238402,#238403),(#238404,#238405),(#238406,#238407),(#238408,#238409),
(#238410,#238411),(#238412,#238413),(#238414,#238415),(#238416,#238417),
(#238418,#238419),(#238420,#238421),(#238422,#238423),(#238424,#238425),
(#238426,#238427),(#238428,#238429),(#238430,#238431),(#238432,#238433),
(#238434,#238435),(#238436,#238437),(#238438,#238439),(#238440,#238441),
(#238442,#238443),(#238444,#238445),(#238446,#238447),(#238448,#238449),
(#238450,#238451),(#238452,#238453),(#238454,#238455),(#238456,#238457),
(#238458,#238459),(#238460,#238461),(#238462,#238463),(#238464,#238465),
(#238466,#238467),(#238468,#238469),(#238470,#238471),(#238472,#238473),
(#238474,#238475),(#238476,#238477),(#238478,#238479),(#238480,#238481),
(#238482,#238483),(#238484,#238485),(#238486,#238487),(#238488,#238489),
(#238490,#238491),(#238492,#238493),(#238494,#238495),(#238496,#238497),
(#238498,#238499),(#238500,#238501),(#238502,#238503),(#238504,#238505),
(#238506,#238507),(#238508,#238509),(#238510,#238511),(#238512,#238513),
(#238514,#238515),(#238516,#238517),(#238518,#238519),(#238520,#238521),
(#238522,#238523),(#238524,#238525),(#238526,#238527),(#238528,#238529),
(#238530,#238531),(#238532,#238533),(#238534,#238535),(#238536,#238537),
(#238538,#238539),(#238540,#238541),(#238542,#238543),(#238544,#238545),
(#238546,#238547),(#238548,#238549),(#238550,#238551),(#238552,#238553),
(#238554,#238555),(#238556,#238557),(#238558,#238559),(#238560,#238561),
(#238562,#238563),(#238564,#238565),(#238566,#238567),(#238568,#238569),
(#238570,#238571),(#238572,#238573),(#238574,#238575),(#238576,#238577),
(#238578,#238579),(#238580,#238581),(#238582,#238583),(#238584,#238585),
(#238586,#238587),(#238588,#238589),(#238590,#238591),(#238592,#238593),
(#238594,#238595),(#238596,#238597),(#238598,#238599),(#238600,#238601),
(#238602,#238603),(#238604,#238605),(#238606,#238607),(#238608,#238609),
(#238610,#238611),(#238612,#238613),(#238614,#238615),(#238616,#238617),
(#238618,#238619),(#238620,#238621),(#238622,#238623),(#238624,#238625),
(#238626,#238627),(#238628,#238629),(#238630,#238631),(#238632,#238633),
(#238634,#238635),(#238636,#238637),(#238638,#238639),(#238640,#238641),
(#238642,#238643),(#238644,#238645),(#238646,#238647),(#238648,#238649),
(#238650,#238651),(#238652,#238653),(#238654,#238655),(#238656,#238657),
(#238658,#238659),(#238660,#238661),(#238662,#238663),(#238664,#238665),
(#238666,#238667),(#238668,#238669),(#238670,#238671),(#238672,#238673),
(#238674,#238675),(#238676,#238677),(#238678,#238679),(#238680,#238681),
(#238682,#238683),(#238684,#238685),(#238686,#238687),(#238688,#238689),
(#238690,#238691),(#238692,#238693),(#238694,#238695),(#238696,#238697),
(#238698,#238699),(#238700,#238701),(#238702,#238703),(#238704,#238705),
(#238706,#238707),(#238708,#238709),(#238710,#238711),(#238712,#238713),
(#238714,#238715),(#238716,#238717),(#238718,#238719),(#238720,#238721),
(#238722,#238723),(#238724,#238725),(#238726,#238727),(#238728,#238729),
(#238730,#238731),(#238732,#238733),(#238734,#238735),(#238736,#238737),
(#238738,#238739),(#238740,#238741),(#238742,#238743),(#238744,#238745),
(#238746,#238747),(#238748,#238749),(#238750,#238751),(#238752,#238753),
(#238754,#238755),(#238756,#238757),(#238758,#238759),(#238760,#238761),
(#238762,#238763),(#238764,#238765),(#238766,#238767),(#238768,#238769),
(#238770,#238771),(#238772,#238773),(#238774,#238775),(#238776,#238777),
(#238778,#238779),(#238780,#238781),(#238782,#238783),(#238784,#238785),
(#238786,#238787),(#238788,#238789),(#238790,#238791),(#238792,#238793),
(#238794,#238795),(#238796,#238797),(#238798,#238799),(#238800,#238801),
(#238802,#238803),(#238804,#238805),(#238806,#238807),(#238808,#238809),
(#238810,#238811),(#238812,#238813),(#238814,#238815),(#238816,#238817),
(#238818,#238819),(#238820,#238821),(#238822,#238823),(#238824,#238825),
(#238826,#238827),(#238828,#238829),(#238830,#238831),(#238832,#238833),
(#238834,#238835),(#238836,#238837),(#238838,#238839),(#238840,#238841),
(#238842,#238843),(#238844,#238845),(#238846,#238847),(#238848,#238849),
(#238850,#238851),(#238852,#238853),(#238854,#238855),(#238856,#238857),
(#238858,#238859),(#238860,#238861),(#238862,#238863),(#238864,#238865),
(#238866,#238867),(#238868,#238869),(#238870,#238871),(#238872,#238873),
(#238874,#238875),(#238876,#238877),(#238878,#238879),(#238880,#238881),
(#238882,#238883),(#238884,#238885),(#238886,#238887),(#238888,#238889),
(#238890,#238891),(#238892,#238893),(#238894,#238895),(#238896,#238897),
(#238898,#238899),(#238900,#238901),(#238902,#238903),(#238904,#238905),
(#238906,#238907),(#238908,#238909),(#238910,#238911),(#238912,#238913),
(#238914,#238915),(#238916,#238917),(#238918,#238919),(#238920,#238921),
(#238922,#238923),(#238924,#238925),(#238926,#238927),(#238928,#238929),
(#238930,#238931),(#238932,#238933),(#238934,#238935),(#238936,#238937),
(#238938,#238939),(#238940,#238941),(#238942,#238943),(#238944,#238945),
(#238946,#238947),(#238948,#238949),(#238950,#238951),(#238952,#238953),
(#238954,#238955),(#238956,#238957),(#238958,#238959),(#238960,#238961),
(#238962,#238963),(#238964,#238965)),.UNSPECIFIED.,.F.,.F.,.F.,(6,1,1,1,
1,1,1,1,1,1,1,1,1,1,1,1,1,1,1,1,1,1,1,1,1,1,1,1,1,1,1,1,1,1,1,1,1,1,1,1,
1,1,1,1,1,1,1,1,1,1,1,1,1,1,1,1,1,1,1,1,1,1,1,1,1,1,1,1,1,1,1,1,1,1,1,1,
1,1,1,1,1,1,1,1,1,1,1,1,1,1,1,1,1,1,1,1,1,1,1,1,1,1,1,1,1,1,1,1,1,1,1,1,
1,1,1,1,1,1,1,1,1,1,1,1,1,1,1,1,1,1,1,1,1,1,1,1,1,1,1,1,1,1,1,1,1,1,1,1,
1,1,1,1,1,1,1,1,1,1,1,1,1,1,1,1,1,1,1,1,1,1,1,1,1,1,1,1,1,1,1,1,1,1,1,1,
1,1,1,1,1,1,1,1,1,1,1,1,1,1,1,1,1,1,1,1,1,1,1,1,1,1,1,1,1,1,1,1,1,1,1,1,
1,1,1,1,1,1,1,1,1,1,1,1,1,1,1,1,1,1,1,1,1,1,1,1,1,1,1,1,1,1,1,1,1,1,1,1,
1,1,1,1,1,1,1,1,1,1,1,1,1,1,1,1,1,1,1,1,1,1,1,1,1,1,1,1,1,1,1,1,1,1,1,1,
1,1,1,1,1,1,1,1,1,1,1,1,1,1,1,1,1,1,1,1,1,1,1,1,1,1,1,1,1,1,1,1,1,1,1,1,
1,1,1,1,1,1,1,1,1,1,1,1,1,1,1,1,1,1,1,1,1,1,1,1,1,1,1,1,1,1,1,1,1,1,1,1,
1,1,1,1,1,1,1,1,1,1,1,1,1,1,1,1,1,1,1,1,1,1,1,1,1,1,1,1,1,1,1,1,1,1,1,1,
1,1,1,1,1,1,1,1,1,1,1,1,1,1,1,1,1,1,1,1,1,1,1,1,1,1,1,1,1,1,1,1,1,1,1,1,
1,1,1,1,1,1,1,1,1,1,1,1,1,1,1,1,1,1,1,1,1,1,1,1,1,1,1,1,1,1,1,6),(2,2),
(0.143172104,0.144954128,0.146788991,0.148623853,0.150458716,0.152293578,
0.15412844,0.155963303,0.157798165,0.159633028,0.16146789,0.163302752,0.165137615,
0.166972477,0.168807339,0.170642202,0.172477064,0.174311927,0.176146789,
0.177981651,0.179816514,0.181651376,0.183486239,0.185321101,0.187155963,
0.188990826,0.190825688,0.19266055,0.194495413,0.196330275,0.198165138,
0.2,0.201834862,0.203669725,0.205504587,0.20733945,0.209174312,0.211009174,
0.212844037,0.214678899,0.216513761,0.218348624,0.220183486,0.222018349,
0.223853211,0.225688073,0.227522936,0.229357798,0.231192661,0.233027523,
0.234862385,0.236697248,0.23853211,0.240366972,0.242201835,0.244036697,
0.24587156,0.247706422,0.249541284,0.251376147,0.253211009,0.255045872,
0.256880734,0.258715596,0.260550459,0.262385321,0.264220183,0.266055046,
0.267889908,0.269724771,0.271559633,0.273394495,0.275229358,0.27706422,
0.278899083,0.280733945,0.282568807,0.28440367,0.286238532,0.288073394,
0.289908257,0.291743119,0.293577982,0.295412844,0.297247706,0.299082569,
0.300917431,0.302752294,0.304587156,0.306422018,0.308256881,0.310091743,
0.311926606,0.313761468,0.31559633,0.317431193,0.319266055,0.321100917,
0.32293578,0.324770642,0.326605505,0.328440367,0.330275229,0.332110092,
0.333944954,0.335779817,0.337614679,0.339449541,0.341284404,0.343119266,
0.344954128,0.346788991,0.348623853,0.350458716,0.352293578,0.35412844,
0.355963303,0.357798165,0.359633028,0.36146789,0.363302752,0.365137615,
0.366972477,0.368807339,0.370642202,0.372477064,0.374311927,0.376146789,
0.377981651,0.379816514,0.381651376,0.383486239,0.385321101,0.387155963,
0.388990826,0.390825688,0.39266055,0.394495413,0.396330275,0.398165138,
0.4,0.401834862,0.403669725,0.405504587,0.40733945,0.409174312,0.411009174,
0.412844037,0.414678899,0.416513761,0.418348624,0.420183486,0.422018349,
0.423853211,0.425688073,0.427522936,0.429357798,0.431192661,0.433027523,
0.434862385,0.436697248,0.43853211,0.440366972,0.442201835,0.444036697,
0.44587156,0.447706422,0.449541284,0.451376147,0.453211009,0.455045872,
0.456880734,0.458715596,0.460550459,0.462385321,0.464220183,0.466055046,
0.467889908,0.469724771,0.471559633,0.473394495,0.475229358,0.47706422,
0.478899083,0.480733945,0.482568807,0.48440367,0.486238532,0.488073394,
0.489908257,0.491743119,0.493577982,0.495412844,0.497247706,0.499082569,
0.500917431,0.502752294,0.504587156,0.506422018,0.508256881,0.510091743,
0.511926606,0.513761468,0.51559633,0.517431193,0.519266055,0.521100917,
0.52293578,0.524770642,0.526605505,0.528440367,0.530275229,0.532110092,
0.533944954,0.535779817,0.537614679,0.539449541,0.541284404,0.543119266,
0.544954128,0.546788991,0.548623853,0.550458716,0.552293578,0.55412844,
0.555963303,0.557798165,0.559633028,0.56146789,0.563302752,0.565137615,
0.566972477,0.568807339,0.570642202,0.572477064,0.574311927,0.576146789,
0.577981651,0.579816514,0.581651376,0.583486239,0.585321101,0.587155963,
0.588990826,0.590825688,0.59266055,0.594495413,0.596330275,0.598165138,
0.6,0.601834862,0.603669725,0.605504587,0.60733945,0.609174312,0.611009174,
0.612844037,0.614678899,0.616513761,0.618348624,0.620183486,0.622018349,
0.623853211,0.625688073,0.627522936,0.629357798,0.631192661,0.633027523,
0.634862385,0.636697248,0.63853211,0.640366972,0.642201835,0.644036697,
0.64587156,0.647706422,0.649541284,0.651376147,0.653211009,0.655045872,
0.656880734,0.658715596,0.660550459,0.662385321,0.664220183,0.666055046,
0.667889908,0.669724771,0.671559633,0.673394495,0.675229358,0.67706422,
0.678899083,0.680733945,0.682568807,0.68440367,0.686238532,0.688073394,
0.689908257,0.691743119,0.693577982,0.695412844,0.697247706,0.699082569,
0.700917431,0.702752294,0.704587156,0.706422018,0.708256881,0.710091743,
0.711926606,0.713761468,0.71559633,0.717431193,0.719266055,0.721100917,
0.72293578,0.724770642,0.726605505,0.728440367,0.730275229,0.732110092,
0.733944954,0.735779817,0.737614679,0.739449541,0.741284404,0.743119266,
0.744954128,0.746788991,0.748623853,0.750458716,0.752293578,0.75412844,
0.755963303,0.757798165,0.759633028,0.76146789,0.763302752,0.765137615,
0.766972477,0.768807339,0.770642202,0.772477064,0.774311927,0.776146789,
0.777981651,0.779816514,0.781651376,0.783486239,0.785321101,0.787155963,
0.788990826,0.790825688,0.79266055,0.794495413,0.796330275,0.798165138,
0.8,0.801834862,0.803669725,0.805504587,0.80733945,0.809174312,0.811009174,
0.812844037,0.814678899,0.816513761,0.818348624,0.820183486,0.822018349,
0.823853211,0.825688073,0.827522936,0.829357798,0.831192661,0.833027523,
0.834862385,0.836697248,0.83853211,0.840366972,0.842201835,0.844036697,
0.84587156,0.847706422,0.849541284,0.851376147,0.853211009,0.855045872,
0.856880734,0.858715596,0.860550459,0.862385321,0.864220183,0.866055046,
0.867889908,0.869724771,0.871559633,0.873394495,0.875229358,0.87706422,
0.878899083,0.880733945,0.882568807,0.88440367,0.886238532,0.888073394,
0.889908257,0.891743119,0.893577982,0.895412844,0.897247706,0.899082569,
0.900917431,0.902752294,0.904587156,0.906422018,0.908256881,0.910091743,
0.911926606,0.913761468,0.91559633,0.917431193,0.919266055,0.921100917,
0.92293578,0.924770642,0.926605505,0.928440367,0.930275229,0.932110092,
0.933944954,0.935779817,0.937614679,0.939449541,0.941284404,0.943119266,
0.944954128,0.946788991,0.948623853,0.950458716,0.952293578,0.95412844,
0.955963303,0.957798165,0.959633028,0.96146789,0.963302752,0.965137615,
0.966972477,0.968807339,0.970642202,0.972477064,0.974311927,0.976146789,
0.977981651,0.979816514,0.981651376,0.983486239,0.985321101,0.987155963,
0.988990826,0.990825688,0.99266055,0.994495413,0.996330275,0.998165138,
1.),(0.,0.36),.UNSPECIFIED.);
#6267=B_SPLINE_SURFACE_WITH_KNOTS('',5,1,((#239616,#239617),(#239618,#239619),
(#239620,#239621),(#239622,#239623),(#239624,#239625),(#239626,#239627),
(#239628,#239629),(#239630,#239631),(#239632,#239633),(#239634,#239635),
(#239636,#239637),(#239638,#239639),(#239640,#239641),(#239642,#239643),
(#239644,#239645),(#239646,#239647),(#239648,#239649),(#239650,#239651),
(#239652,#239653),(#239654,#239655),(#239656,#239657),(#239658,#239659),
(#239660,#239661),(#239662,#239663),(#239664,#239665),(#239666,#239667),
(#239668,#239669),(#239670,#239671),(#239672,#239673),(#239674,#239675),
(#239676,#239677),(#239678,#239679),(#239680,#239681),(#239682,#239683),
(#239684,#239685),(#239686,#239687),(#239688,#239689),(#239690,#239691),
(#239692,#239693),(#239694,#239695),(#239696,#239697),(#239698,#239699),
(#239700,#239701),(#239702,#239703),(#239704,#239705),(#239706,#239707),
(#239708,#239709),(#239710,#239711),(#239712,#239713),(#239714,#239715),
(#239716,#239717),(#239718,#239719),(#239720,#239721),(#239722,#239723),
(#239724,#239725),(#239726,#239727),(#239728,#239729),(#239730,#239731),
(#239732,#239733),(#239734,#239735),(#239736,#239737),(#239738,#239739),
(#239740,#239741),(#239742,#239743),(#239744,#239745),(#239746,#239747),
(#239748,#239749),(#239750,#239751),(#239752,#239753),(#239754,#239755),
(#239756,#239757),(#239758,#239759),(#239760,#239761),(#239762,#239763),
(#239764,#239765),(#239766,#239767),(#239768,#239769),(#239770,#239771),
(#239772,#239773),(#239774,#239775),(#239776,#239777),(#239778,#239779),
(#239780,#239781),(#239782,#239783),(#239784,#239785),(#239786,#239787),
(#239788,#239789),(#239790,#239791),(#239792,#239793),(#239794,#239795),
(#239796,#239797),(#239798,#239799),(#239800,#239801),(#239802,#239803),
(#239804,#239805),(#239806,#239807),(#239808,#239809),(#239810,#239811),
(#239812,#239813),(#239814,#239815),(#239816,#239817),(#239818,#239819),
(#239820,#239821),(#239822,#239823),(#239824,#239825),(#239826,#239827),
(#239828,#239829),(#239830,#239831),(#239832,#239833),(#239834,#239835),
(#239836,#239837),(#239838,#239839),(#239840,#239841),(#239842,#239843),
(#239844,#239845),(#239846,#239847),(#239848,#239849),(#239850,#239851),
(#239852,#239853),(#239854,#239855),(#239856,#239857),(#239858,#239859),
(#239860,#239861),(#239862,#239863),(#239864,#239865),(#239866,#239867),
(#239868,#239869),(#239870,#239871),(#239872,#239873),(#239874,#239875),
(#239876,#239877),(#239878,#239879),(#239880,#239881),(#239882,#239883),
(#239884,#239885),(#239886,#239887),(#239888,#239889),(#239890,#239891),
(#239892,#239893),(#239894,#239895),(#239896,#239897),(#239898,#239899),
(#239900,#239901),(#239902,#239903),(#239904,#239905),(#239906,#239907),
(#239908,#239909),(#239910,#239911),(#239912,#239913),(#239914,#239915),
(#239916,#239917),(#239918,#239919),(#239920,#239921),(#239922,#239923),
(#239924,#239925),(#239926,#239927),(#239928,#239929),(#239930,#239931),
(#239932,#239933),(#239934,#239935),(#239936,#239937),(#239938,#239939),
(#239940,#239941),(#239942,#239943),(#239944,#239945),(#239946,#239947),
(#239948,#239949),(#239950,#239951),(#239952,#239953),(#239954,#239955),
(#239956,#239957),(#239958,#239959),(#239960,#239961),(#239962,#239963),
(#239964,#239965),(#239966,#239967),(#239968,#239969),(#239970,#239971),
(#239972,#239973),(#239974,#239975),(#239976,#239977),(#239978,#239979),
(#239980,#239981),(#239982,#239983),(#239984,#239985),(#239986,#239987),
(#239988,#239989),(#239990,#239991),(#239992,#239993),(#239994,#239995),
(#239996,#239997),(#239998,#239999),(#240000,#240001),(#240002,#240003),
(#240004,#240005),(#240006,#240007),(#240008,#240009),(#240010,#240011),
(#240012,#240013),(#240014,#240015),(#240016,#240017),(#240018,#240019),
(#240020,#240021),(#240022,#240023),(#240024,#240025),(#240026,#240027),
(#240028,#240029),(#240030,#240031),(#240032,#240033),(#240034,#240035),
(#240036,#240037),(#240038,#240039),(#240040,#240041),(#240042,#240043),
(#240044,#240045),(#240046,#240047),(#240048,#240049),(#240050,#240051),
(#240052,#240053),(#240054,#240055),(#240056,#240057),(#240058,#240059),
(#240060,#240061),(#240062,#240063),(#240064,#240065),(#240066,#240067),
(#240068,#240069),(#240070,#240071),(#240072,#240073),(#240074,#240075),
(#240076,#240077),(#240078,#240079),(#240080,#240081),(#240082,#240083),
(#240084,#240085),(#240086,#240087),(#240088,#240089),(#240090,#240091),
(#240092,#240093),(#240094,#240095),(#240096,#240097),(#240098,#240099),
(#240100,#240101),(#240102,#240103),(#240104,#240105),(#240106,#240107),
(#240108,#240109),(#240110,#240111),(#240112,#240113),(#240114,#240115),
(#240116,#240117),(#240118,#240119),(#240120,#240121),(#240122,#240123),
(#240124,#240125),(#240126,#240127),(#240128,#240129),(#240130,#240131),
(#240132,#240133),(#240134,#240135),(#240136,#240137),(#240138,#240139),
(#240140,#240141),(#240142,#240143),(#240144,#240145),(#240146,#240147),
(#240148,#240149),(#240150,#240151),(#240152,#240153),(#240154,#240155),
(#240156,#240157),(#240158,#240159),(#240160,#240161),(#240162,#240163),
(#240164,#240165),(#240166,#240167),(#240168,#240169),(#240170,#240171),
(#240172,#240173),(#240174,#240175),(#240176,#240177),(#240178,#240179),
(#240180,#240181),(#240182,#240183),(#240184,#240185),(#240186,#240187),
(#240188,#240189),(#240190,#240191),(#240192,#240193),(#240194,#240195),
(#240196,#240197),(#240198,#240199),(#240200,#240201),(#240202,#240203),
(#240204,#240205),(#240206,#240207),(#240208,#240209),(#240210,#240211),
(#240212,#240213),(#240214,#240215),(#240216,#240217),(#240218,#240219),
(#240220,#240221),(#240222,#240223),(#240224,#240225),(#240226,#240227),
(#240228,#240229),(#240230,#240231),(#240232,#240233),(#240234,#240235),
(#240236,#240237),(#240238,#240239),(#240240,#240241),(#240242,#240243),
(#240244,#240245),(#240246,#240247),(#240248,#240249),(#240250,#240251),
(#240252,#240253),(#240254,#240255),(#240256,#240257),(#240258,#240259),
(#240260,#240261),(#240262,#240263),(#240264,#240265),(#240266,#240267),
(#240268,#240269),(#240270,#240271),(#240272,#240273),(#240274,#240275),
(#240276,#240277),(#240278,#240279),(#240280,#240281),(#240282,#240283),
(#240284,#240285),(#240286,#240287),(#240288,#240289),(#240290,#240291),
(#240292,#240293),(#240294,#240295),(#240296,#240297),(#240298,#240299),
(#240300,#240301),(#240302,#240303),(#240304,#240305),(#240306,#240307),
(#240308,#240309),(#240310,#240311),(#240312,#240313),(#240314,#240315),
(#240316,#240317),(#240318,#240319),(#240320,#240321),(#240322,#240323),
(#240324,#240325),(#240326,#240327),(#240328,#240329),(#240330,#240331),
(#240332,#240333),(#240334,#240335),(#240336,#240337),(#240338,#240339),
(#240340,#240341),(#240342,#240343),(#240344,#240345),(#240346,#240347),
(#240348,#240349),(#240350,#240351),(#240352,#240353),(#240354,#240355),
(#240356,#240357),(#240358,#240359),(#240360,#240361),(#240362,#240363),
(#240364,#240365),(#240366,#240367),(#240368,#240369),(#240370,#240371),
(#240372,#240373),(#240374,#240375),(#240376,#240377),(#240378,#240379),
(#240380,#240381),(#240382,#240383),(#240384,#240385),(#240386,#240387),
(#240388,#240389),(#240390,#240391),(#240392,#240393),(#240394,#240395),
(#240396,#240397),(#240398,#240399),(#240400,#240401),(#240402,#240403),
(#240404,#240405),(#240406,#240407),(#240408,#240409),(#240410,#240411),
(#240412,#240413),(#240414,#240415),(#240416,#240417),(#240418,#240419),
(#240420,#240421),(#240422,#240423),(#240424,#240425),(#240426,#240427),
(#240428,#240429),(#240430,#240431),(#240432,#240433),(#240434,#240435),
(#240436,#240437),(#240438,#240439),(#240440,#240441),(#240442,#240443),
(#240444,#240445),(#240446,#240447),(#240448,#240449),(#240450,#240451),
(#240452,#240453),(#240454,#240455),(#240456,#240457),(#240458,#240459),
(#240460,#240461),(#240462,#240463),(#240464,#240465),(#240466,#240467),
(#240468,#240469),(#240470,#240471),(#240472,#240473),(#240474,#240475),
(#240476,#240477),(#240478,#240479),(#240480,#240481),(#240482,#240483),
(#240484,#240485),(#240486,#240487),(#240488,#240489),(#240490,#240491),
(#240492,#240493),(#240494,#240495),(#240496,#240497),(#240498,#240499),
(#240500,#240501),(#240502,#240503),(#240504,#240505),(#240506,#240507),
(#240508,#240509),(#240510,#240511),(#240512,#240513),(#240514,#240515),
(#240516,#240517),(#240518,#240519),(#240520,#240521),(#240522,#240523),
(#240524,#240525),(#240526,#240527),(#240528,#240529),(#240530,#240531),
(#240532,#240533),(#240534,#240535),(#240536,#240537),(#240538,#240539),
(#240540,#240541),(#240542,#240543),(#240544,#240545),(#240546,#240547),
(#240548,#240549),(#240550,#240551),(#240552,#240553),(#240554,#240555),
(#240556,#240557),(#240558,#240559)),.UNSPECIFIED.,.F.,.F.,.F.,(6,1,1,1,
1,1,1,1,1,1,1,1,1,1,1,1,1,1,1,1,1,1,1,1,1,1,1,1,1,1,1,1,1,1,1,1,1,1,1,1,
1,1,1,1,1,1,1,1,1,1,1,1,1,1,1,1,1,1,1,1,1,1,1,1,1,1,1,1,1,1,1,1,1,1,1,1,
1,1,1,1,1,1,1,1,1,1,1,1,1,1,1,1,1,1,1,1,1,1,1,1,1,1,1,1,1,1,1,1,1,1,1,1,
1,1,1,1,1,1,1,1,1,1,1,1,1,1,1,1,1,1,1,1,1,1,1,1,1,1,1,1,1,1,1,1,1,1,1,1,
1,1,1,1,1,1,1,1,1,1,1,1,1,1,1,1,1,1,1,1,1,1,1,1,1,1,1,1,1,1,1,1,1,1,1,1,
1,1,1,1,1,1,1,1,1,1,1,1,1,1,1,1,1,1,1,1,1,1,1,1,1,1,1,1,1,1,1,1,1,1,1,1,
1,1,1,1,1,1,1,1,1,1,1,1,1,1,1,1,1,1,1,1,1,1,1,1,1,1,1,1,1,1,1,1,1,1,1,1,
1,1,1,1,1,1,1,1,1,1,1,1,1,1,1,1,1,1,1,1,1,1,1,1,1,1,1,1,1,1,1,1,1,1,1,1,
1,1,1,1,1,1,1,1,1,1,1,1,1,1,1,1,1,1,1,1,1,1,1,1,1,1,1,1,1,1,1,1,1,1,1,1,
1,1,1,1,1,1,1,1,1,1,1,1,1,1,1,1,1,1,1,1,1,1,1,1,1,1,1,1,1,1,1,1,1,1,1,1,
1,1,1,1,1,1,1,1,1,1,1,1,1,1,1,1,1,1,1,1,1,1,1,1,1,1,1,1,1,1,1,1,1,1,1,1,
1,1,1,1,1,1,1,1,1,1,1,1,1,1,1,1,1,1,1,1,1,1,1,1,1,1,1,1,1,1,1,1,1,1,1,1,
1,1,1,1,1,1,1,1,1,1,1,1,1,1,1,1,1,1,1,1,1,1,1,1,1,1,1,1,1,1,1,6),(2,2),
(0.143172103,0.144954128,0.146788991,0.148623853,0.150458716,0.152293578,
0.15412844,0.155963303,0.157798165,0.159633028,0.16146789,0.163302752,0.165137615,
0.166972477,0.168807339,0.170642202,0.172477064,0.174311927,0.176146789,
0.177981651,0.179816514,0.181651376,0.183486239,0.185321101,0.187155963,
0.188990826,0.190825688,0.19266055,0.194495413,0.196330275,0.198165138,
0.2,0.201834862,0.203669725,0.205504587,0.20733945,0.209174312,0.211009174,
0.212844037,0.214678899,0.216513761,0.218348624,0.220183486,0.222018349,
0.223853211,0.225688073,0.227522936,0.229357798,0.231192661,0.233027523,
0.234862385,0.236697248,0.23853211,0.240366972,0.242201835,0.244036697,
0.24587156,0.247706422,0.249541284,0.251376147,0.253211009,0.255045872,
0.256880734,0.258715596,0.260550459,0.262385321,0.264220183,0.266055046,
0.267889908,0.269724771,0.271559633,0.273394495,0.275229358,0.27706422,
0.278899083,0.280733945,0.282568807,0.28440367,0.286238532,0.288073394,
0.289908257,0.291743119,0.293577982,0.295412844,0.297247706,0.299082569,
0.300917431,0.302752294,0.304587156,0.306422018,0.308256881,0.310091743,
0.311926606,0.313761468,0.31559633,0.317431193,0.319266055,0.321100917,
0.32293578,0.324770642,0.326605505,0.328440367,0.330275229,0.332110092,
0.333944954,0.335779817,0.337614679,0.339449541,0.341284404,0.343119266,
0.344954128,0.346788991,0.348623853,0.350458716,0.352293578,0.35412844,
0.355963303,0.357798165,0.359633028,0.36146789,0.363302752,0.365137615,
0.366972477,0.368807339,0.370642202,0.372477064,0.374311927,0.376146789,
0.377981651,0.379816514,0.381651376,0.383486239,0.385321101,0.387155963,
0.388990826,0.390825688,0.39266055,0.394495413,0.396330275,0.398165138,
0.4,0.401834862,0.403669725,0.405504587,0.40733945,0.409174312,0.411009174,
0.412844037,0.414678899,0.416513761,0.418348624,0.420183486,0.422018349,
0.423853211,0.425688073,0.427522936,0.429357798,0.431192661,0.433027523,
0.434862385,0.436697248,0.43853211,0.440366972,0.442201835,0.444036697,
0.44587156,0.447706422,0.449541284,0.451376147,0.453211009,0.455045872,
0.456880734,0.458715596,0.460550459,0.462385321,0.464220183,0.466055046,
0.467889908,0.469724771,0.471559633,0.473394495,0.475229358,0.47706422,
0.478899083,0.480733945,0.482568807,0.48440367,0.486238532,0.488073394,
0.489908257,0.491743119,0.493577982,0.495412844,0.497247706,0.499082569,
0.500917431,0.502752294,0.504587156,0.506422018,0.508256881,0.510091743,
0.511926606,0.513761468,0.51559633,0.517431193,0.519266055,0.521100917,
0.52293578,0.524770642,0.526605505,0.528440367,0.530275229,0.532110092,
0.533944954,0.535779817,0.537614679,0.539449541,0.541284404,0.543119266,
0.544954128,0.546788991,0.548623853,0.550458716,0.552293578,0.55412844,
0.555963303,0.557798165,0.559633028,0.56146789,0.563302752,0.565137615,
0.566972477,0.568807339,0.570642202,0.572477064,0.574311927,0.576146789,
0.577981651,0.579816514,0.581651376,0.583486239,0.585321101,0.587155963,
0.588990826,0.590825688,0.59266055,0.594495413,0.596330275,0.598165138,
0.6,0.601834862,0.603669725,0.605504587,0.60733945,0.609174312,0.611009174,
0.612844037,0.614678899,0.616513761,0.618348624,0.620183486,0.622018349,
0.623853211,0.625688073,0.627522936,0.629357798,0.631192661,0.633027523,
0.634862385,0.636697248,0.63853211,0.640366972,0.642201835,0.644036697,
0.64587156,0.647706422,0.649541284,0.651376147,0.653211009,0.655045872,
0.656880734,0.658715596,0.660550459,0.662385321,0.664220183,0.666055046,
0.667889908,0.669724771,0.671559633,0.673394495,0.675229358,0.67706422,
0.678899083,0.680733945,0.682568807,0.68440367,0.686238532,0.688073394,
0.689908257,0.691743119,0.693577982,0.695412844,0.697247706,0.699082569,
0.700917431,0.702752294,0.704587156,0.706422018,0.708256881,0.710091743,
0.711926606,0.713761468,0.71559633,0.717431193,0.719266055,0.721100917,
0.72293578,0.724770642,0.726605505,0.728440367,0.730275229,0.732110092,
0.733944954,0.735779817,0.737614679,0.739449541,0.741284404,0.743119266,
0.744954128,0.746788991,0.748623853,0.750458716,0.752293578,0.75412844,
0.755963303,0.757798165,0.759633028,0.76146789,0.763302752,0.765137615,
0.766972477,0.768807339,0.770642202,0.772477064,0.774311927,0.776146789,
0.777981651,0.779816514,0.781651376,0.783486239,0.785321101,0.787155963,
0.788990826,0.790825688,0.79266055,0.794495413,0.796330275,0.798165138,
0.8,0.801834862,0.803669725,0.805504587,0.80733945,0.809174312,0.811009174,
0.812844037,0.814678899,0.816513761,0.818348624,0.820183486,0.822018349,
0.823853211,0.825688073,0.827522936,0.829357798,0.831192661,0.833027523,
0.834862385,0.836697248,0.83853211,0.840366972,0.842201835,0.844036697,
0.84587156,0.847706422,0.849541284,0.851376147,0.853211009,0.855045872,
0.856880734,0.858715596,0.860550459,0.862385321,0.864220183,0.866055046,
0.867889908,0.869724771,0.871559633,0.873394495,0.875229358,0.87706422,
0.878899083,0.880733945,0.882568807,0.88440367,0.886238532,0.888073394,
0.889908257,0.891743119,0.893577982,0.895412844,0.897247706,0.899082569,
0.900917431,0.902752294,0.904587156,0.906422018,0.908256881,0.910091743,
0.911926606,0.913761468,0.91559633,0.917431193,0.919266055,0.921100917,
0.92293578,0.924770642,0.926605505,0.928440367,0.930275229,0.932110092,
0.933944954,0.935779817,0.937614679,0.939449541,0.941284404,0.943119266,
0.944954128,0.946788991,0.948623853,0.950458716,0.952293578,0.95412844,
0.955963303,0.957798165,0.959633028,0.96146789,0.963302752,0.965137615,
0.966972477,0.968807339,0.970642202,0.972477064,0.974311927,0.976146789,
0.977981651,0.979816514,0.981651376,0.983486239,0.985321101,0.987155963,
0.988990826,0.990825688,0.99266055,0.994495413,0.996330275,0.998165138,
1.),(0.,0.36),.UNSPECIFIED.);
#6268=B_SPLINE_SURFACE_WITH_KNOTS('',5,1,((#241192,#241193),(#241194,#241195),
(#241196,#241197),(#241198,#241199),(#241200,#241201),(#241202,#241203),
(#241204,#241205),(#241206,#241207),(#241208,#241209),(#241210,#241211),
(#241212,#241213),(#241214,#241215),(#241216,#241217),(#241218,#241219),
(#241220,#241221),(#241222,#241223),(#241224,#241225),(#241226,#241227),
(#241228,#241229),(#241230,#241231),(#241232,#241233),(#241234,#241235),
(#241236,#241237),(#241238,#241239),(#241240,#241241),(#241242,#241243),
(#241244,#241245),(#241246,#241247),(#241248,#241249),(#241250,#241251),
(#241252,#241253),(#241254,#241255),(#241256,#241257),(#241258,#241259),
(#241260,#241261),(#241262,#241263),(#241264,#241265),(#241266,#241267),
(#241268,#241269),(#241270,#241271),(#241272,#241273),(#241274,#241275),
(#241276,#241277),(#241278,#241279),(#241280,#241281),(#241282,#241283),
(#241284,#241285),(#241286,#241287),(#241288,#241289),(#241290,#241291),
(#241292,#241293),(#241294,#241295),(#241296,#241297),(#241298,#241299),
(#241300,#241301),(#241302,#241303),(#241304,#241305),(#241306,#241307),
(#241308,#241309),(#241310,#241311),(#241312,#241313),(#241314,#241315),
(#241316,#241317),(#241318,#241319),(#241320,#241321),(#241322,#241323),
(#241324,#241325),(#241326,#241327),(#241328,#241329),(#241330,#241331),
(#241332,#241333),(#241334,#241335),(#241336,#241337),(#241338,#241339),
(#241340,#241341),(#241342,#241343),(#241344,#241345),(#241346,#241347),
(#241348,#241349),(#241350,#241351),(#241352,#241353),(#241354,#241355),
(#241356,#241357),(#241358,#241359),(#241360,#241361),(#241362,#241363),
(#241364,#241365),(#241366,#241367),(#241368,#241369),(#241370,#241371),
(#241372,#241373),(#241374,#241375),(#241376,#241377),(#241378,#241379),
(#241380,#241381),(#241382,#241383),(#241384,#241385),(#241386,#241387),
(#241388,#241389),(#241390,#241391),(#241392,#241393),(#241394,#241395),
(#241396,#241397),(#241398,#241399),(#241400,#241401),(#241402,#241403),
(#241404,#241405),(#241406,#241407),(#241408,#241409),(#241410,#241411),
(#241412,#241413),(#241414,#241415),(#241416,#241417),(#241418,#241419),
(#241420,#241421),(#241422,#241423),(#241424,#241425),(#241426,#241427),
(#241428,#241429),(#241430,#241431),(#241432,#241433),(#241434,#241435),
(#241436,#241437),(#241438,#241439),(#241440,#241441),(#241442,#241443),
(#241444,#241445),(#241446,#241447),(#241448,#241449),(#241450,#241451),
(#241452,#241453),(#241454,#241455),(#241456,#241457),(#241458,#241459),
(#241460,#241461),(#241462,#241463),(#241464,#241465),(#241466,#241467),
(#241468,#241469),(#241470,#241471),(#241472,#241473),(#241474,#241475),
(#241476,#241477),(#241478,#241479),(#241480,#241481),(#241482,#241483),
(#241484,#241485),(#241486,#241487),(#241488,#241489),(#241490,#241491),
(#241492,#241493),(#241494,#241495),(#241496,#241497),(#241498,#241499),
(#241500,#241501),(#241502,#241503),(#241504,#241505),(#241506,#241507),
(#241508,#241509),(#241510,#241511),(#241512,#241513),(#241514,#241515),
(#241516,#241517),(#241518,#241519),(#241520,#241521),(#241522,#241523),
(#241524,#241525),(#241526,#241527),(#241528,#241529),(#241530,#241531),
(#241532,#241533),(#241534,#241535),(#241536,#241537),(#241538,#241539),
(#241540,#241541),(#241542,#241543),(#241544,#241545),(#241546,#241547),
(#241548,#241549),(#241550,#241551),(#241552,#241553),(#241554,#241555),
(#241556,#241557),(#241558,#241559),(#241560,#241561),(#241562,#241563),
(#241564,#241565),(#241566,#241567),(#241568,#241569),(#241570,#241571),
(#241572,#241573),(#241574,#241575),(#241576,#241577),(#241578,#241579),
(#241580,#241581),(#241582,#241583),(#241584,#241585),(#241586,#241587),
(#241588,#241589),(#241590,#241591),(#241592,#241593),(#241594,#241595),
(#241596,#241597),(#241598,#241599),(#241600,#241601),(#241602,#241603),
(#241604,#241605),(#241606,#241607),(#241608,#241609),(#241610,#241611),
(#241612,#241613),(#241614,#241615),(#241616,#241617),(#241618,#241619),
(#241620,#241621),(#241622,#241623),(#241624,#241625),(#241626,#241627),
(#241628,#241629),(#241630,#241631),(#241632,#241633),(#241634,#241635),
(#241636,#241637),(#241638,#241639),(#241640,#241641),(#241642,#241643),
(#241644,#241645),(#241646,#241647),(#241648,#241649),(#241650,#241651),
(#241652,#241653),(#241654,#241655),(#241656,#241657),(#241658,#241659),
(#241660,#241661),(#241662,#241663),(#241664,#241665),(#241666,#241667),
(#241668,#241669),(#241670,#241671),(#241672,#241673),(#241674,#241675),
(#241676,#241677),(#241678,#241679),(#241680,#241681),(#241682,#241683),
(#241684,#241685),(#241686,#241687),(#241688,#241689),(#241690,#241691),
(#241692,#241693),(#241694,#241695),(#241696,#241697),(#241698,#241699),
(#241700,#241701),(#241702,#241703),(#241704,#241705),(#241706,#241707),
(#241708,#241709),(#241710,#241711),(#241712,#241713),(#241714,#241715),
(#241716,#241717),(#241718,#241719),(#241720,#241721),(#241722,#241723),
(#241724,#241725),(#241726,#241727),(#241728,#241729),(#241730,#241731),
(#241732,#241733),(#241734,#241735),(#241736,#241737),(#241738,#241739),
(#241740,#241741),(#241742,#241743),(#241744,#241745),(#241746,#241747),
(#241748,#241749),(#241750,#241751),(#241752,#241753),(#241754,#241755),
(#241756,#241757),(#241758,#241759),(#241760,#241761),(#241762,#241763),
(#241764,#241765),(#241766,#241767),(#241768,#241769),(#241770,#241771),
(#241772,#241773),(#241774,#241775),(#241776,#241777),(#241778,#241779),
(#241780,#241781),(#241782,#241783),(#241784,#241785),(#241786,#241787),
(#241788,#241789),(#241790,#241791),(#241792,#241793),(#241794,#241795),
(#241796,#241797),(#241798,#241799),(#241800,#241801),(#241802,#241803),
(#241804,#241805),(#241806,#241807),(#241808,#241809),(#241810,#241811),
(#241812,#241813),(#241814,#241815),(#241816,#241817),(#241818,#241819),
(#241820,#241821),(#241822,#241823),(#241824,#241825),(#241826,#241827),
(#241828,#241829),(#241830,#241831),(#241832,#241833),(#241834,#241835),
(#241836,#241837),(#241838,#241839),(#241840,#241841),(#241842,#241843),
(#241844,#241845),(#241846,#241847),(#241848,#241849),(#241850,#241851),
(#241852,#241853),(#241854,#241855),(#241856,#241857),(#241858,#241859),
(#241860,#241861),(#241862,#241863),(#241864,#241865),(#241866,#241867),
(#241868,#241869),(#241870,#241871),(#241872,#241873),(#241874,#241875),
(#241876,#241877),(#241878,#241879),(#241880,#241881),(#241882,#241883),
(#241884,#241885),(#241886,#241887),(#241888,#241889),(#241890,#241891),
(#241892,#241893),(#241894,#241895),(#241896,#241897),(#241898,#241899),
(#241900,#241901),(#241902,#241903),(#241904,#241905),(#241906,#241907),
(#241908,#241909),(#241910,#241911),(#241912,#241913),(#241914,#241915),
(#241916,#241917),(#241918,#241919),(#241920,#241921),(#241922,#241923),
(#241924,#241925),(#241926,#241927),(#241928,#241929),(#241930,#241931),
(#241932,#241933),(#241934,#241935),(#241936,#241937),(#241938,#241939),
(#241940,#241941),(#241942,#241943),(#241944,#241945),(#241946,#241947),
(#241948,#241949),(#241950,#241951),(#241952,#241953),(#241954,#241955),
(#241956,#241957),(#241958,#241959),(#241960,#241961),(#241962,#241963),
(#241964,#241965),(#241966,#241967),(#241968,#241969),(#241970,#241971),
(#241972,#241973),(#241974,#241975),(#241976,#241977),(#241978,#241979),
(#241980,#241981),(#241982,#241983),(#241984,#241985),(#241986,#241987),
(#241988,#241989),(#241990,#241991),(#241992,#241993),(#241994,#241995),
(#241996,#241997),(#241998,#241999),(#242000,#242001),(#242002,#242003),
(#242004,#242005),(#242006,#242007),(#242008,#242009),(#242010,#242011),
(#242012,#242013),(#242014,#242015),(#242016,#242017),(#242018,#242019),
(#242020,#242021),(#242022,#242023),(#242024,#242025),(#242026,#242027),
(#242028,#242029),(#242030,#242031),(#242032,#242033),(#242034,#242035),
(#242036,#242037),(#242038,#242039),(#242040,#242041),(#242042,#242043),
(#242044,#242045),(#242046,#242047),(#242048,#242049),(#242050,#242051),
(#242052,#242053),(#242054,#242055),(#242056,#242057),(#242058,#242059),
(#242060,#242061),(#242062,#242063),(#242064,#242065),(#242066,#242067),
(#242068,#242069),(#242070,#242071),(#242072,#242073),(#242074,#242075),
(#242076,#242077),(#242078,#242079),(#242080,#242081),(#242082,#242083),
(#242084,#242085),(#242086,#242087),(#242088,#242089),(#242090,#242091),
(#242092,#242093),(#242094,#242095),(#242096,#242097),(#242098,#242099),
(#242100,#242101),(#242102,#242103),(#242104,#242105),(#242106,#242107),
(#242108,#242109),(#242110,#242111),(#242112,#242113),(#242114,#242115),
(#242116,#242117),(#242118,#242119),(#242120,#242121),(#242122,#242123),
(#242124,#242125),(#242126,#242127),(#242128,#242129),(#242130,#242131),
(#242132,#242133),(#242134,#242135)),.UNSPECIFIED.,.F.,.F.,.F.,(6,1,1,1,
1,1,1,1,1,1,1,1,1,1,1,1,1,1,1,1,1,1,1,1,1,1,1,1,1,1,1,1,1,1,1,1,1,1,1,1,
1,1,1,1,1,1,1,1,1,1,1,1,1,1,1,1,1,1,1,1,1,1,1,1,1,1,1,1,1,1,1,1,1,1,1,1,
1,1,1,1,1,1,1,1,1,1,1,1,1,1,1,1,1,1,1,1,1,1,1,1,1,1,1,1,1,1,1,1,1,1,1,1,
1,1,1,1,1,1,1,1,1,1,1,1,1,1,1,1,1,1,1,1,1,1,1,1,1,1,1,1,1,1,1,1,1,1,1,1,
1,1,1,1,1,1,1,1,1,1,1,1,1,1,1,1,1,1,1,1,1,1,1,1,1,1,1,1,1,1,1,1,1,1,1,1,
1,1,1,1,1,1,1,1,1,1,1,1,1,1,1,1,1,1,1,1,1,1,1,1,1,1,1,1,1,1,1,1,1,1,1,1,
1,1,1,1,1,1,1,1,1,1,1,1,1,1,1,1,1,1,1,1,1,1,1,1,1,1,1,1,1,1,1,1,1,1,1,1,
1,1,1,1,1,1,1,1,1,1,1,1,1,1,1,1,1,1,1,1,1,1,1,1,1,1,1,1,1,1,1,1,1,1,1,1,
1,1,1,1,1,1,1,1,1,1,1,1,1,1,1,1,1,1,1,1,1,1,1,1,1,1,1,1,1,1,1,1,1,1,1,1,
1,1,1,1,1,1,1,1,1,1,1,1,1,1,1,1,1,1,1,1,1,1,1,1,1,1,1,1,1,1,1,1,1,1,1,1,
1,1,1,1,1,1,1,1,1,1,1,1,1,1,1,1,1,1,1,1,1,1,1,1,1,1,1,1,1,1,1,1,1,1,1,1,
1,1,1,1,1,1,1,1,1,1,1,1,1,1,1,1,1,1,1,1,1,1,1,1,1,1,1,1,1,1,1,1,1,1,1,1,
1,1,1,1,1,1,1,1,1,1,1,1,1,1,1,1,1,1,1,1,1,1,1,1,1,1,1,1,1,1,1,6),(2,2),
(-1.,-0.998165138,-0.996330275,-0.994495413,-0.99266055,-0.990825688,-0.988990826,
-0.987155963,-0.985321101,-0.983486239,-0.981651376,-0.979816514,-0.977981651,
-0.976146789,-0.974311927,-0.972477064,-0.970642202,-0.968807339,-0.966972477,
-0.965137615,-0.963302752,-0.96146789,-0.959633028,-0.957798165,-0.955963303,
-0.95412844,-0.952293578,-0.950458716,-0.948623853,-0.946788991,-0.944954128,
-0.943119266,-0.941284404,-0.939449541,-0.937614679,-0.935779817,-0.933944954,
-0.932110092,-0.930275229,-0.928440367,-0.926605505,-0.924770642,-0.92293578,
-0.921100917,-0.919266055,-0.917431193,-0.91559633,-0.913761468,-0.911926606,
-0.910091743,-0.908256881,-0.906422018,-0.904587156,-0.902752294,-0.900917431,
-0.899082569,-0.897247706,-0.895412844,-0.893577982,-0.891743119,-0.889908257,
-0.888073394,-0.886238532,-0.88440367,-0.882568807,-0.880733945,-0.878899083,
-0.87706422,-0.875229358,-0.873394495,-0.871559633,-0.869724771,-0.867889908,
-0.866055046,-0.864220183,-0.862385321,-0.860550459,-0.858715596,-0.856880734,
-0.855045872,-0.853211009,-0.851376147,-0.849541284,-0.847706422,-0.84587156,
-0.844036697,-0.842201835,-0.840366972,-0.83853211,-0.836697248,-0.834862385,
-0.833027523,-0.831192661,-0.829357798,-0.827522936,-0.825688073,-0.823853211,
-0.822018349,-0.820183486,-0.818348624,-0.816513761,-0.814678899,-0.812844037,
-0.811009174,-0.809174312,-0.80733945,-0.805504587,-0.803669725,-0.801834862,
-0.8,-0.798165138,-0.796330275,-0.794495413,-0.79266055,-0.790825688,-0.788990826,
-0.787155963,-0.785321101,-0.783486239,-0.781651376,-0.779816514,-0.777981651,
-0.776146789,-0.774311927,-0.772477064,-0.770642202,-0.768807339,-0.766972477,
-0.765137615,-0.763302752,-0.76146789,-0.759633028,-0.757798165,-0.755963303,
-0.75412844,-0.752293578,-0.750458716,-0.748623853,-0.746788991,-0.744954128,
-0.743119266,-0.741284404,-0.739449541,-0.737614679,-0.735779817,-0.733944954,
-0.732110092,-0.730275229,-0.728440367,-0.726605505,-0.724770642,-0.72293578,
-0.721100917,-0.719266055,-0.717431193,-0.71559633,-0.713761468,-0.711926606,
-0.710091743,-0.708256881,-0.706422018,-0.704587156,-0.702752294,-0.700917431,
-0.699082569,-0.697247706,-0.695412844,-0.693577982,-0.691743119,-0.689908257,
-0.688073394,-0.686238532,-0.68440367,-0.682568807,-0.680733945,-0.678899083,
-0.67706422,-0.675229358,-0.673394495,-0.671559633,-0.669724771,-0.667889908,
-0.666055046,-0.664220183,-0.662385321,-0.660550459,-0.658715596,-0.656880734,
-0.655045872,-0.653211009,-0.651376147,-0.649541284,-0.647706422,-0.64587156,
-0.644036697,-0.642201835,-0.640366972,-0.63853211,-0.636697248,-0.634862385,
-0.633027523,-0.631192661,-0.629357798,-0.627522936,-0.625688073,-0.623853211,
-0.622018349,-0.620183486,-0.618348624,-0.616513761,-0.614678899,-0.612844037,
-0.611009174,-0.609174312,-0.60733945,-0.605504587,-0.603669725,-0.601834862,
-0.6,-0.598165138,-0.596330275,-0.594495413,-0.59266055,-0.590825688,-0.588990826,
-0.587155963,-0.585321101,-0.583486239,-0.581651376,-0.579816514,-0.577981651,
-0.576146789,-0.574311927,-0.572477064,-0.570642202,-0.568807339,-0.566972477,
-0.565137615,-0.563302752,-0.56146789,-0.559633028,-0.557798165,-0.555963303,
-0.55412844,-0.552293578,-0.550458716,-0.548623853,-0.546788991,-0.544954128,
-0.543119266,-0.541284404,-0.539449541,-0.537614679,-0.535779817,-0.533944954,
-0.532110092,-0.530275229,-0.528440367,-0.526605505,-0.524770642,-0.52293578,
-0.521100917,-0.519266055,-0.517431193,-0.51559633,-0.513761468,-0.511926606,
-0.510091743,-0.508256881,-0.506422018,-0.504587156,-0.502752294,-0.500917431,
-0.499082569,-0.497247706,-0.495412844,-0.493577982,-0.491743119,-0.489908257,
-0.488073394,-0.486238532,-0.48440367,-0.482568807,-0.480733945,-0.478899083,
-0.47706422,-0.475229358,-0.473394495,-0.471559633,-0.469724771,-0.467889908,
-0.466055046,-0.464220183,-0.462385321,-0.460550459,-0.458715596,-0.456880734,
-0.455045872,-0.453211009,-0.451376147,-0.449541284,-0.447706422,-0.44587156,
-0.444036697,-0.442201835,-0.440366972,-0.43853211,-0.436697248,-0.434862385,
-0.433027523,-0.431192661,-0.429357798,-0.427522936,-0.425688073,-0.423853211,
-0.422018349,-0.420183486,-0.418348624,-0.416513761,-0.414678899,-0.412844037,
-0.411009174,-0.409174312,-0.40733945,-0.405504587,-0.403669725,-0.401834862,
-0.4,-0.398165138,-0.396330275,-0.394495413,-0.39266055,-0.390825688,-0.388990826,
-0.387155963,-0.385321101,-0.383486239,-0.381651376,-0.379816514,-0.377981651,
-0.376146789,-0.374311927,-0.372477064,-0.370642202,-0.368807339,-0.366972477,
-0.365137615,-0.363302752,-0.36146789,-0.359633028,-0.357798165,-0.355963303,
-0.35412844,-0.352293578,-0.350458716,-0.348623853,-0.346788991,-0.344954128,
-0.343119266,-0.341284404,-0.339449541,-0.337614679,-0.335779817,-0.333944954,
-0.332110092,-0.330275229,-0.328440367,-0.326605505,-0.324770642,-0.32293578,
-0.321100917,-0.319266055,-0.317431193,-0.31559633,-0.313761468,-0.311926606,
-0.310091743,-0.308256881,-0.306422018,-0.304587156,-0.302752294,-0.300917431,
-0.299082569,-0.297247706,-0.295412844,-0.293577982,-0.291743119,-0.289908257,
-0.288073394,-0.286238532,-0.28440367,-0.282568807,-0.280733945,-0.278899083,
-0.27706422,-0.275229358,-0.273394495,-0.271559633,-0.269724771,-0.267889908,
-0.266055046,-0.264220183,-0.262385321,-0.260550459,-0.258715596,-0.256880734,
-0.255045872,-0.253211009,-0.251376147,-0.249541284,-0.247706422,-0.24587156,
-0.244036697,-0.242201835,-0.240366972,-0.23853211,-0.236697248,-0.234862385,
-0.233027523,-0.231192661,-0.229357798,-0.227522936,-0.225688073,-0.223853211,
-0.222018349,-0.220183486,-0.218348624,-0.216513761,-0.214678899,-0.212844037,
-0.211009174,-0.209174312,-0.20733945,-0.205504587,-0.203669725,-0.201834862,
-0.2,-0.198165138,-0.196330275,-0.194495413,-0.19266055,-0.190825688,-0.188990826,
-0.187155963,-0.185321101,-0.183486239,-0.181651376,-0.179816514,-0.177981651,
-0.176146789,-0.174311927,-0.172477064,-0.170642202,-0.168807339,-0.166972477,
-0.165137615,-0.163302752,-0.16146789,-0.159633028,-0.157798165,-0.155963303,
-0.15412844,-0.152293578,-0.150458716,-0.148623853,-0.146788991,-0.144954128,
-0.143172103),(0.,0.36),.UNSPECIFIED.);
#6269=B_SPLINE_SURFACE_WITH_KNOTS('',5,1,((#242783,#242784),(#242785,#242786),
(#242787,#242788),(#242789,#242790),(#242791,#242792),(#242793,#242794),
(#242795,#242796),(#242797,#242798),(#242799,#242800),(#242801,#242802),
(#242803,#242804),(#242805,#242806),(#242807,#242808),(#242809,#242810),
(#242811,#242812),(#242813,#242814),(#242815,#242816),(#242817,#242818),
(#242819,#242820),(#242821,#242822),(#242823,#242824),(#242825,#242826),
(#242827,#242828),(#242829,#242830),(#242831,#242832),(#242833,#242834),
(#242835,#242836),(#242837,#242838),(#242839,#242840),(#242841,#242842),
(#242843,#242844),(#242845,#242846),(#242847,#242848),(#242849,#242850),
(#242851,#242852),(#242853,#242854),(#242855,#242856),(#242857,#242858),
(#242859,#242860),(#242861,#242862),(#242863,#242864),(#242865,#242866),
(#242867,#242868),(#242869,#242870),(#242871,#242872),(#242873,#242874),
(#242875,#242876),(#242877,#242878),(#242879,#242880),(#242881,#242882),
(#242883,#242884),(#242885,#242886),(#242887,#242888),(#242889,#242890),
(#242891,#242892),(#242893,#242894),(#242895,#242896),(#242897,#242898),
(#242899,#242900),(#242901,#242902),(#242903,#242904),(#242905,#242906),
(#242907,#242908),(#242909,#242910),(#242911,#242912),(#242913,#242914),
(#242915,#242916),(#242917,#242918),(#242919,#242920),(#242921,#242922),
(#242923,#242924),(#242925,#242926),(#242927,#242928),(#242929,#242930),
(#242931,#242932),(#242933,#242934),(#242935,#242936),(#242937,#242938),
(#242939,#242940),(#242941,#242942),(#242943,#242944),(#242945,#242946),
(#242947,#242948),(#242949,#242950),(#242951,#242952),(#242953,#242954),
(#242955,#242956),(#242957,#242958),(#242959,#242960),(#242961,#242962),
(#242963,#242964),(#242965,#242966),(#242967,#242968),(#242969,#242970),
(#242971,#242972),(#242973,#242974),(#242975,#242976),(#242977,#242978),
(#242979,#242980),(#242981,#242982),(#242983,#242984),(#242985,#242986),
(#242987,#242988),(#242989,#242990),(#242991,#242992),(#242993,#242994),
(#242995,#242996),(#242997,#242998),(#242999,#243000),(#243001,#243002),
(#243003,#243004),(#243005,#243006),(#243007,#243008),(#243009,#243010),
(#243011,#243012),(#243013,#243014),(#243015,#243016),(#243017,#243018),
(#243019,#243020),(#243021,#243022),(#243023,#243024),(#243025,#243026),
(#243027,#243028),(#243029,#243030),(#243031,#243032),(#243033,#243034),
(#243035,#243036),(#243037,#243038),(#243039,#243040),(#243041,#243042),
(#243043,#243044),(#243045,#243046),(#243047,#243048),(#243049,#243050),
(#243051,#243052),(#243053,#243054),(#243055,#243056),(#243057,#243058),
(#243059,#243060),(#243061,#243062),(#243063,#243064),(#243065,#243066),
(#243067,#243068),(#243069,#243070),(#243071,#243072),(#243073,#243074),
(#243075,#243076),(#243077,#243078),(#243079,#243080),(#243081,#243082),
(#243083,#243084),(#243085,#243086),(#243087,#243088),(#243089,#243090),
(#243091,#243092),(#243093,#243094),(#243095,#243096),(#243097,#243098),
(#243099,#243100),(#243101,#243102),(#243103,#243104),(#243105,#243106),
(#243107,#243108),(#243109,#243110),(#243111,#243112),(#243113,#243114),
(#243115,#243116),(#243117,#243118),(#243119,#243120),(#243121,#243122),
(#243123,#243124),(#243125,#243126),(#243127,#243128),(#243129,#243130),
(#243131,#243132),(#243133,#243134),(#243135,#243136),(#243137,#243138),
(#243139,#243140),(#243141,#243142),(#243143,#243144),(#243145,#243146),
(#243147,#243148),(#243149,#243150),(#243151,#243152),(#243153,#243154),
(#243155,#243156),(#243157,#243158),(#243159,#243160),(#243161,#243162),
(#243163,#243164),(#243165,#243166),(#243167,#243168),(#243169,#243170),
(#243171,#243172),(#243173,#243174),(#243175,#243176),(#243177,#243178),
(#243179,#243180),(#243181,#243182),(#243183,#243184),(#243185,#243186),
(#243187,#243188),(#243189,#243190),(#243191,#243192),(#243193,#243194),
(#243195,#243196),(#243197,#243198),(#243199,#243200),(#243201,#243202),
(#243203,#243204),(#243205,#243206),(#243207,#243208),(#243209,#243210),
(#243211,#243212),(#243213,#243214),(#243215,#243216),(#243217,#243218),
(#243219,#243220),(#243221,#243222),(#243223,#243224),(#243225,#243226),
(#243227,#243228),(#243229,#243230),(#243231,#243232),(#243233,#243234),
(#243235,#243236),(#243237,#243238),(#243239,#243240),(#243241,#243242),
(#243243,#243244),(#243245,#243246),(#243247,#243248),(#243249,#243250),
(#243251,#243252),(#243253,#243254),(#243255,#243256),(#243257,#243258),
(#243259,#243260),(#243261,#243262),(#243263,#243264),(#243265,#243266),
(#243267,#243268),(#243269,#243270),(#243271,#243272),(#243273,#243274),
(#243275,#243276),(#243277,#243278),(#243279,#243280),(#243281,#243282),
(#243283,#243284),(#243285,#243286),(#243287,#243288),(#243289,#243290),
(#243291,#243292),(#243293,#243294),(#243295,#243296),(#243297,#243298),
(#243299,#243300),(#243301,#243302),(#243303,#243304),(#243305,#243306),
(#243307,#243308),(#243309,#243310),(#243311,#243312),(#243313,#243314),
(#243315,#243316),(#243317,#243318),(#243319,#243320),(#243321,#243322),
(#243323,#243324),(#243325,#243326),(#243327,#243328),(#243329,#243330),
(#243331,#243332),(#243333,#243334),(#243335,#243336),(#243337,#243338),
(#243339,#243340),(#243341,#243342),(#243343,#243344),(#243345,#243346),
(#243347,#243348),(#243349,#243350),(#243351,#243352),(#243353,#243354),
(#243355,#243356),(#243357,#243358),(#243359,#243360),(#243361,#243362),
(#243363,#243364),(#243365,#243366),(#243367,#243368),(#243369,#243370),
(#243371,#243372),(#243373,#243374),(#243375,#243376),(#243377,#243378),
(#243379,#243380),(#243381,#243382),(#243383,#243384),(#243385,#243386),
(#243387,#243388),(#243389,#243390),(#243391,#243392),(#243393,#243394),
(#243395,#243396),(#243397,#243398),(#243399,#243400),(#243401,#243402),
(#243403,#243404),(#243405,#243406),(#243407,#243408),(#243409,#243410),
(#243411,#243412),(#243413,#243414),(#243415,#243416),(#243417,#243418),
(#243419,#243420),(#243421,#243422),(#243423,#243424),(#243425,#243426),
(#243427,#243428),(#243429,#243430),(#243431,#243432),(#243433,#243434),
(#243435,#243436),(#243437,#243438),(#243439,#243440),(#243441,#243442),
(#243443,#243444),(#243445,#243446),(#243447,#243448),(#243449,#243450),
(#243451,#243452),(#243453,#243454),(#243455,#243456),(#243457,#243458),
(#243459,#243460),(#243461,#243462),(#243463,#243464),(#243465,#243466),
(#243467,#243468),(#243469,#243470),(#243471,#243472),(#243473,#243474),
(#243475,#243476),(#243477,#243478),(#243479,#243480),(#243481,#243482),
(#243483,#243484),(#243485,#243486),(#243487,#243488),(#243489,#243490),
(#243491,#243492),(#243493,#243494),(#243495,#243496),(#243497,#243498),
(#243499,#243500),(#243501,#243502),(#243503,#243504),(#243505,#243506),
(#243507,#243508),(#243509,#243510),(#243511,#243512),(#243513,#243514),
(#243515,#243516),(#243517,#243518),(#243519,#243520),(#243521,#243522),
(#243523,#243524),(#243525,#243526),(#243527,#243528),(#243529,#243530),
(#243531,#243532),(#243533,#243534),(#243535,#243536),(#243537,#243538),
(#243539,#243540),(#243541,#243542),(#243543,#243544),(#243545,#243546),
(#243547,#243548),(#243549,#243550),(#243551,#243552),(#243553,#243554),
(#243555,#243556),(#243557,#243558),(#243559,#243560),(#243561,#243562),
(#243563,#243564),(#243565,#243566),(#243567,#243568),(#243569,#243570),
(#243571,#243572),(#243573,#243574),(#243575,#243576),(#243577,#243578),
(#243579,#243580),(#243581,#243582),(#243583,#243584),(#243585,#243586),
(#243587,#243588),(#243589,#243590),(#243591,#243592),(#243593,#243594),
(#243595,#243596),(#243597,#243598),(#243599,#243600),(#243601,#243602),
(#243603,#243604),(#243605,#243606),(#243607,#243608),(#243609,#243610),
(#243611,#243612),(#243613,#243614),(#243615,#243616),(#243617,#243618),
(#243619,#243620),(#243621,#243622),(#243623,#243624),(#243625,#243626),
(#243627,#243628),(#243629,#243630),(#243631,#243632),(#243633,#243634),
(#243635,#243636),(#243637,#243638),(#243639,#243640),(#243641,#243642),
(#243643,#243644),(#243645,#243646),(#243647,#243648),(#243649,#243650),
(#243651,#243652),(#243653,#243654),(#243655,#243656),(#243657,#243658),
(#243659,#243660),(#243661,#243662),(#243663,#243664),(#243665,#243666),
(#243667,#243668),(#243669,#243670),(#243671,#243672),(#243673,#243674),
(#243675,#243676),(#243677,#243678),(#243679,#243680),(#243681,#243682),
(#243683,#243684),(#243685,#243686),(#243687,#243688),(#243689,#243690),
(#243691,#243692),(#243693,#243694),(#243695,#243696),(#243697,#243698),
(#243699,#243700),(#243701,#243702),(#243703,#243704),(#243705,#243706),
(#243707,#243708),(#243709,#243710),(#243711,#243712),(#243713,#243714),
(#243715,#243716),(#243717,#243718),(#243719,#243720),(#243721,#243722),
(#243723,#243724),(#243725,#243726)),.UNSPECIFIED.,.F.,.F.,.F.,(6,1,1,1,
1,1,1,1,1,1,1,1,1,1,1,1,1,1,1,1,1,1,1,1,1,1,1,1,1,1,1,1,1,1,1,1,1,1,1,1,
1,1,1,1,1,1,1,1,1,1,1,1,1,1,1,1,1,1,1,1,1,1,1,1,1,1,1,1,1,1,1,1,1,1,1,1,
1,1,1,1,1,1,1,1,1,1,1,1,1,1,1,1,1,1,1,1,1,1,1,1,1,1,1,1,1,1,1,1,1,1,1,1,
1,1,1,1,1,1,1,1,1,1,1,1,1,1,1,1,1,1,1,1,1,1,1,1,1,1,1,1,1,1,1,1,1,1,1,1,
1,1,1,1,1,1,1,1,1,1,1,1,1,1,1,1,1,1,1,1,1,1,1,1,1,1,1,1,1,1,1,1,1,1,1,1,
1,1,1,1,1,1,1,1,1,1,1,1,1,1,1,1,1,1,1,1,1,1,1,1,1,1,1,1,1,1,1,1,1,1,1,1,
1,1,1,1,1,1,1,1,1,1,1,1,1,1,1,1,1,1,1,1,1,1,1,1,1,1,1,1,1,1,1,1,1,1,1,1,
1,1,1,1,1,1,1,1,1,1,1,1,1,1,1,1,1,1,1,1,1,1,1,1,1,1,1,1,1,1,1,1,1,1,1,1,
1,1,1,1,1,1,1,1,1,1,1,1,1,1,1,1,1,1,1,1,1,1,1,1,1,1,1,1,1,1,1,1,1,1,1,1,
1,1,1,1,1,1,1,1,1,1,1,1,1,1,1,1,1,1,1,1,1,1,1,1,1,1,1,1,1,1,1,1,1,1,1,1,
1,1,1,1,1,1,1,1,1,1,1,1,1,1,1,1,1,1,1,1,1,1,1,1,1,1,1,1,1,1,1,1,1,1,1,1,
1,1,1,1,1,1,1,1,1,1,1,1,1,1,1,1,1,1,1,1,1,1,1,1,1,1,1,1,1,1,1,1,1,1,1,1,
1,1,1,1,1,1,1,1,1,1,1,1,1,1,1,1,1,1,1,1,1,1,1,1,1,1,1,1,1,1,1,6),(2,2),
(-1.,-0.998165138,-0.996330275,-0.994495413,-0.99266055,-0.990825688,-0.988990826,
-0.987155963,-0.985321101,-0.983486239,-0.981651376,-0.979816514,-0.977981651,
-0.976146789,-0.974311927,-0.972477064,-0.970642202,-0.968807339,-0.966972477,
-0.965137615,-0.963302752,-0.96146789,-0.959633028,-0.957798165,-0.955963303,
-0.95412844,-0.952293578,-0.950458716,-0.948623853,-0.946788991,-0.944954128,
-0.943119266,-0.941284404,-0.939449541,-0.937614679,-0.935779817,-0.933944954,
-0.932110092,-0.930275229,-0.928440367,-0.926605505,-0.924770642,-0.92293578,
-0.921100917,-0.919266055,-0.917431193,-0.91559633,-0.913761468,-0.911926606,
-0.910091743,-0.908256881,-0.906422018,-0.904587156,-0.902752294,-0.900917431,
-0.899082569,-0.897247706,-0.895412844,-0.893577982,-0.891743119,-0.889908257,
-0.888073394,-0.886238532,-0.88440367,-0.882568807,-0.880733945,-0.878899083,
-0.87706422,-0.875229358,-0.873394495,-0.871559633,-0.869724771,-0.867889908,
-0.866055046,-0.864220183,-0.862385321,-0.860550459,-0.858715596,-0.856880734,
-0.855045872,-0.853211009,-0.851376147,-0.849541284,-0.847706422,-0.84587156,
-0.844036697,-0.842201835,-0.840366972,-0.83853211,-0.836697248,-0.834862385,
-0.833027523,-0.831192661,-0.829357798,-0.827522936,-0.825688073,-0.823853211,
-0.822018349,-0.820183486,-0.818348624,-0.816513761,-0.814678899,-0.812844037,
-0.811009174,-0.809174312,-0.80733945,-0.805504587,-0.803669725,-0.801834862,
-0.8,-0.798165138,-0.796330275,-0.794495413,-0.79266055,-0.790825688,-0.788990826,
-0.787155963,-0.785321101,-0.783486239,-0.781651376,-0.779816514,-0.777981651,
-0.776146789,-0.774311927,-0.772477064,-0.770642202,-0.768807339,-0.766972477,
-0.765137615,-0.763302752,-0.76146789,-0.759633028,-0.757798165,-0.755963303,
-0.75412844,-0.752293578,-0.750458716,-0.748623853,-0.746788991,-0.744954128,
-0.743119266,-0.741284404,-0.739449541,-0.737614679,-0.735779817,-0.733944954,
-0.732110092,-0.730275229,-0.728440367,-0.726605505,-0.724770642,-0.72293578,
-0.721100917,-0.719266055,-0.717431193,-0.71559633,-0.713761468,-0.711926606,
-0.710091743,-0.708256881,-0.706422018,-0.704587156,-0.702752294,-0.700917431,
-0.699082569,-0.697247706,-0.695412844,-0.693577982,-0.691743119,-0.689908257,
-0.688073394,-0.686238532,-0.68440367,-0.682568807,-0.680733945,-0.678899083,
-0.67706422,-0.675229358,-0.673394495,-0.671559633,-0.669724771,-0.667889908,
-0.666055046,-0.664220183,-0.662385321,-0.660550459,-0.658715596,-0.656880734,
-0.655045872,-0.653211009,-0.651376147,-0.649541284,-0.647706422,-0.64587156,
-0.644036697,-0.642201835,-0.640366972,-0.63853211,-0.636697248,-0.634862385,
-0.633027523,-0.631192661,-0.629357798,-0.627522936,-0.625688073,-0.623853211,
-0.622018349,-0.620183486,-0.618348624,-0.616513761,-0.614678899,-0.612844037,
-0.611009174,-0.609174312,-0.60733945,-0.605504587,-0.603669725,-0.601834862,
-0.6,-0.598165138,-0.596330275,-0.594495413,-0.59266055,-0.590825688,-0.588990826,
-0.587155963,-0.585321101,-0.583486239,-0.581651376,-0.579816514,-0.577981651,
-0.576146789,-0.574311927,-0.572477064,-0.570642202,-0.568807339,-0.566972477,
-0.565137615,-0.563302752,-0.56146789,-0.559633028,-0.557798165,-0.555963303,
-0.55412844,-0.552293578,-0.550458716,-0.548623853,-0.546788991,-0.544954128,
-0.543119266,-0.541284404,-0.539449541,-0.537614679,-0.535779817,-0.533944954,
-0.532110092,-0.530275229,-0.528440367,-0.526605505,-0.524770642,-0.52293578,
-0.521100917,-0.519266055,-0.517431193,-0.51559633,-0.513761468,-0.511926606,
-0.510091743,-0.508256881,-0.506422018,-0.504587156,-0.502752294,-0.500917431,
-0.499082569,-0.497247706,-0.495412844,-0.493577982,-0.491743119,-0.489908257,
-0.488073394,-0.486238532,-0.48440367,-0.482568807,-0.480733945,-0.478899083,
-0.47706422,-0.475229358,-0.473394495,-0.471559633,-0.469724771,-0.467889908,
-0.466055046,-0.464220183,-0.462385321,-0.460550459,-0.458715596,-0.456880734,
-0.455045872,-0.453211009,-0.451376147,-0.449541284,-0.447706422,-0.44587156,
-0.444036697,-0.442201835,-0.440366972,-0.43853211,-0.436697248,-0.434862385,
-0.433027523,-0.431192661,-0.429357798,-0.427522936,-0.425688073,-0.423853211,
-0.422018349,-0.420183486,-0.418348624,-0.416513761,-0.414678899,-0.412844037,
-0.411009174,-0.409174312,-0.40733945,-0.405504587,-0.403669725,-0.401834862,
-0.4,-0.398165138,-0.396330275,-0.394495413,-0.39266055,-0.390825688,-0.388990826,
-0.387155963,-0.385321101,-0.383486239,-0.381651376,-0.379816514,-0.377981651,
-0.376146789,-0.374311927,-0.372477064,-0.370642202,-0.368807339,-0.366972477,
-0.365137615,-0.363302752,-0.36146789,-0.359633028,-0.357798165,-0.355963303,
-0.35412844,-0.352293578,-0.350458716,-0.348623853,-0.346788991,-0.344954128,
-0.343119266,-0.341284404,-0.339449541,-0.337614679,-0.335779817,-0.333944954,
-0.332110092,-0.330275229,-0.328440367,-0.326605505,-0.324770642,-0.32293578,
-0.321100917,-0.319266055,-0.317431193,-0.31559633,-0.313761468,-0.311926606,
-0.310091743,-0.308256881,-0.306422018,-0.304587156,-0.302752294,-0.300917431,
-0.299082569,-0.297247706,-0.295412844,-0.293577982,-0.291743119,-0.289908257,
-0.288073394,-0.286238532,-0.28440367,-0.282568807,-0.280733945,-0.278899083,
-0.27706422,-0.275229358,-0.273394495,-0.271559633,-0.269724771,-0.267889908,
-0.266055046,-0.264220183,-0.262385321,-0.260550459,-0.258715596,-0.256880734,
-0.255045872,-0.253211009,-0.251376147,-0.249541284,-0.247706422,-0.24587156,
-0.244036697,-0.242201835,-0.240366972,-0.23853211,-0.236697248,-0.234862385,
-0.233027523,-0.231192661,-0.229357798,-0.227522936,-0.225688073,-0.223853211,
-0.222018349,-0.220183486,-0.218348624,-0.216513761,-0.214678899,-0.212844037,
-0.211009174,-0.209174312,-0.20733945,-0.205504587,-0.203669725,-0.201834862,
-0.2,-0.198165138,-0.196330275,-0.194495413,-0.19266055,-0.190825688,-0.188990826,
-0.187155963,-0.185321101,-0.183486239,-0.181651376,-0.179816514,-0.177981651,
-0.176146789,-0.174311927,-0.172477064,-0.170642202,-0.168807339,-0.166972477,
-0.165137615,-0.163302752,-0.16146789,-0.159633028,-0.157798165,-0.155963303,
-0.15412844,-0.152293578,-0.150458716,-0.148623853,-0.146788991,-0.144954128,
-0.143172103),(0.,0.36),.UNSPECIFIED.);
#6270=B_SPLINE_SURFACE_WITH_KNOTS('',5,1,((#244362,#244363),(#244364,#244365),
(#244366,#244367),(#244368,#244369),(#244370,#244371),(#244372,#244373),
(#244374,#244375),(#244376,#244377),(#244378,#244379),(#244380,#244381),
(#244382,#244383),(#244384,#244385),(#244386,#244387),(#244388,#244389),
(#244390,#244391),(#244392,#244393),(#244394,#244395),(#244396,#244397),
(#244398,#244399),(#244400,#244401),(#244402,#244403),(#244404,#244405),
(#244406,#244407),(#244408,#244409),(#244410,#244411),(#244412,#244413),
(#244414,#244415),(#244416,#244417),(#244418,#244419),(#244420,#244421),
(#244422,#244423),(#244424,#244425),(#244426,#244427),(#244428,#244429),
(#244430,#244431),(#244432,#244433),(#244434,#244435),(#244436,#244437),
(#244438,#244439),(#244440,#244441),(#244442,#244443),(#244444,#244445),
(#244446,#244447),(#244448,#244449),(#244450,#244451),(#244452,#244453),
(#244454,#244455),(#244456,#244457),(#244458,#244459),(#244460,#244461),
(#244462,#244463),(#244464,#244465),(#244466,#244467),(#244468,#244469),
(#244470,#244471),(#244472,#244473),(#244474,#244475),(#244476,#244477),
(#244478,#244479),(#244480,#244481),(#244482,#244483),(#244484,#244485),
(#244486,#244487),(#244488,#244489),(#244490,#244491),(#244492,#244493),
(#244494,#244495),(#244496,#244497),(#244498,#244499),(#244500,#244501),
(#244502,#244503),(#244504,#244505),(#244506,#244507),(#244508,#244509),
(#244510,#244511),(#244512,#244513),(#244514,#244515),(#244516,#244517),
(#244518,#244519),(#244520,#244521),(#244522,#244523),(#244524,#244525),
(#244526,#244527),(#244528,#244529),(#244530,#244531),(#244532,#244533),
(#244534,#244535),(#244536,#244537),(#244538,#244539),(#244540,#244541),
(#244542,#244543),(#244544,#244545),(#244546,#244547),(#244548,#244549),
(#244550,#244551),(#244552,#244553),(#244554,#244555),(#244556,#244557),
(#244558,#244559),(#244560,#244561),(#244562,#244563),(#244564,#244565),
(#244566,#244567),(#244568,#244569),(#244570,#244571),(#244572,#244573),
(#244574,#244575),(#244576,#244577),(#244578,#244579),(#244580,#244581),
(#244582,#244583),(#244584,#244585),(#244586,#244587),(#244588,#244589),
(#244590,#244591),(#244592,#244593),(#244594,#244595),(#244596,#244597),
(#244598,#244599),(#244600,#244601),(#244602,#244603),(#244604,#244605),
(#244606,#244607),(#244608,#244609),(#244610,#244611),(#244612,#244613),
(#244614,#244615),(#244616,#244617),(#244618,#244619),(#244620,#244621),
(#244622,#244623),(#244624,#244625),(#244626,#244627),(#244628,#244629),
(#244630,#244631),(#244632,#244633),(#244634,#244635),(#244636,#244637),
(#244638,#244639),(#244640,#244641),(#244642,#244643),(#244644,#244645),
(#244646,#244647),(#244648,#244649),(#244650,#244651),(#244652,#244653),
(#244654,#244655),(#244656,#244657),(#244658,#244659),(#244660,#244661),
(#244662,#244663),(#244664,#244665),(#244666,#244667),(#244668,#244669),
(#244670,#244671),(#244672,#244673),(#244674,#244675),(#244676,#244677),
(#244678,#244679),(#244680,#244681),(#244682,#244683),(#244684,#244685),
(#244686,#244687),(#244688,#244689),(#244690,#244691),(#244692,#244693),
(#244694,#244695),(#244696,#244697),(#244698,#244699),(#244700,#244701),
(#244702,#244703),(#244704,#244705),(#244706,#244707),(#244708,#244709),
(#244710,#244711),(#244712,#244713),(#244714,#244715),(#244716,#244717),
(#244718,#244719),(#244720,#244721),(#244722,#244723),(#244724,#244725),
(#244726,#244727),(#244728,#244729),(#244730,#244731),(#244732,#244733),
(#244734,#244735),(#244736,#244737),(#244738,#244739),(#244740,#244741),
(#244742,#244743),(#244744,#244745),(#244746,#244747),(#244748,#244749),
(#244750,#244751),(#244752,#244753),(#244754,#244755),(#244756,#244757),
(#244758,#244759),(#244760,#244761),(#244762,#244763),(#244764,#244765),
(#244766,#244767),(#244768,#244769),(#244770,#244771),(#244772,#244773),
(#244774,#244775),(#244776,#244777),(#244778,#244779),(#244780,#244781),
(#244782,#244783),(#244784,#244785),(#244786,#244787),(#244788,#244789),
(#244790,#244791),(#244792,#244793),(#244794,#244795),(#244796,#244797),
(#244798,#244799),(#244800,#244801),(#244802,#244803),(#244804,#244805),
(#244806,#244807),(#244808,#244809),(#244810,#244811),(#244812,#244813),
(#244814,#244815),(#244816,#244817),(#244818,#244819),(#244820,#244821),
(#244822,#244823),(#244824,#244825),(#244826,#244827),(#244828,#244829),
(#244830,#244831),(#244832,#244833),(#244834,#244835),(#244836,#244837),
(#244838,#244839),(#244840,#244841),(#244842,#244843),(#244844,#244845),
(#244846,#244847),(#244848,#244849),(#244850,#244851),(#244852,#244853),
(#244854,#244855),(#244856,#244857),(#244858,#244859),(#244860,#244861),
(#244862,#244863),(#244864,#244865),(#244866,#244867),(#244868,#244869),
(#244870,#244871),(#244872,#244873),(#244874,#244875),(#244876,#244877),
(#244878,#244879),(#244880,#244881),(#244882,#244883),(#244884,#244885),
(#244886,#244887),(#244888,#244889),(#244890,#244891),(#244892,#244893),
(#244894,#244895),(#244896,#244897),(#244898,#244899),(#244900,#244901),
(#244902,#244903),(#244904,#244905),(#244906,#244907),(#244908,#244909),
(#244910,#244911),(#244912,#244913),(#244914,#244915),(#244916,#244917),
(#244918,#244919),(#244920,#244921),(#244922,#244923),(#244924,#244925),
(#244926,#244927),(#244928,#244929),(#244930,#244931),(#244932,#244933),
(#244934,#244935),(#244936,#244937),(#244938,#244939),(#244940,#244941),
(#244942,#244943),(#244944,#244945),(#244946,#244947),(#244948,#244949),
(#244950,#244951),(#244952,#244953),(#244954,#244955),(#244956,#244957),
(#244958,#244959),(#244960,#244961),(#244962,#244963),(#244964,#244965),
(#244966,#244967),(#244968,#244969),(#244970,#244971),(#244972,#244973),
(#244974,#244975),(#244976,#244977),(#244978,#244979),(#244980,#244981),
(#244982,#244983),(#244984,#244985),(#244986,#244987),(#244988,#244989),
(#244990,#244991),(#244992,#244993),(#244994,#244995),(#244996,#244997),
(#244998,#244999),(#245000,#245001),(#245002,#245003),(#245004,#245005),
(#245006,#245007),(#245008,#245009),(#245010,#245011),(#245012,#245013),
(#245014,#245015),(#245016,#245017),(#245018,#245019),(#245020,#245021),
(#245022,#245023),(#245024,#245025),(#245026,#245027),(#245028,#245029),
(#245030,#245031),(#245032,#245033),(#245034,#245035),(#245036,#245037),
(#245038,#245039),(#245040,#245041),(#245042,#245043),(#245044,#245045),
(#245046,#245047),(#245048,#245049),(#245050,#245051),(#245052,#245053),
(#245054,#245055),(#245056,#245057),(#245058,#245059),(#245060,#245061),
(#245062,#245063),(#245064,#245065),(#245066,#245067),(#245068,#245069),
(#245070,#245071),(#245072,#245073),(#245074,#245075),(#245076,#245077),
(#245078,#245079),(#245080,#245081),(#245082,#245083),(#245084,#245085),
(#245086,#245087),(#245088,#245089),(#245090,#245091),(#245092,#245093),
(#245094,#245095),(#245096,#245097),(#245098,#245099),(#245100,#245101),
(#245102,#245103),(#245104,#245105),(#245106,#245107),(#245108,#245109),
(#245110,#245111),(#245112,#245113),(#245114,#245115),(#245116,#245117),
(#245118,#245119),(#245120,#245121),(#245122,#245123),(#245124,#245125),
(#245126,#245127),(#245128,#245129),(#245130,#245131),(#245132,#245133),
(#245134,#245135),(#245136,#245137),(#245138,#245139),(#245140,#245141),
(#245142,#245143),(#245144,#245145),(#245146,#245147),(#245148,#245149),
(#245150,#245151),(#245152,#245153),(#245154,#245155),(#245156,#245157),
(#245158,#245159),(#245160,#245161),(#245162,#245163),(#245164,#245165),
(#245166,#245167),(#245168,#245169),(#245170,#245171),(#245172,#245173),
(#245174,#245175),(#245176,#245177),(#245178,#245179),(#245180,#245181),
(#245182,#245183),(#245184,#245185),(#245186,#245187),(#245188,#245189),
(#245190,#245191),(#245192,#245193),(#245194,#245195),(#245196,#245197),
(#245198,#245199),(#245200,#245201),(#245202,#245203),(#245204,#245205),
(#245206,#245207),(#245208,#245209),(#245210,#245211),(#245212,#245213),
(#245214,#245215),(#245216,#245217),(#245218,#245219),(#245220,#245221),
(#245222,#245223),(#245224,#245225),(#245226,#245227),(#245228,#245229),
(#245230,#245231),(#245232,#245233),(#245234,#245235),(#245236,#245237),
(#245238,#245239),(#245240,#245241),(#245242,#245243),(#245244,#245245),
(#245246,#245247),(#245248,#245249),(#245250,#245251),(#245252,#245253),
(#245254,#245255),(#245256,#245257),(#245258,#245259),(#245260,#245261),
(#245262,#245263),(#245264,#245265),(#245266,#245267),(#245268,#245269),
(#245270,#245271),(#245272,#245273),(#245274,#245275),(#245276,#245277),
(#245278,#245279),(#245280,#245281),(#245282,#245283),(#245284,#245285),
(#245286,#245287),(#245288,#245289),(#245290,#245291),(#245292,#245293),
(#245294,#245295),(#245296,#245297),(#245298,#245299),(#245300,#245301),
(#245302,#245303),(#245304,#245305)),.UNSPECIFIED.,.F.,.F.,.F.,(6,1,1,1,
1,1,1,1,1,1,1,1,1,1,1,1,1,1,1,1,1,1,1,1,1,1,1,1,1,1,1,1,1,1,1,1,1,1,1,1,
1,1,1,1,1,1,1,1,1,1,1,1,1,1,1,1,1,1,1,1,1,1,1,1,1,1,1,1,1,1,1,1,1,1,1,1,
1,1,1,1,1,1,1,1,1,1,1,1,1,1,1,1,1,1,1,1,1,1,1,1,1,1,1,1,1,1,1,1,1,1,1,1,
1,1,1,1,1,1,1,1,1,1,1,1,1,1,1,1,1,1,1,1,1,1,1,1,1,1,1,1,1,1,1,1,1,1,1,1,
1,1,1,1,1,1,1,1,1,1,1,1,1,1,1,1,1,1,1,1,1,1,1,1,1,1,1,1,1,1,1,1,1,1,1,1,
1,1,1,1,1,1,1,1,1,1,1,1,1,1,1,1,1,1,1,1,1,1,1,1,1,1,1,1,1,1,1,1,1,1,1,1,
1,1,1,1,1,1,1,1,1,1,1,1,1,1,1,1,1,1,1,1,1,1,1,1,1,1,1,1,1,1,1,1,1,1,1,1,
1,1,1,1,1,1,1,1,1,1,1,1,1,1,1,1,1,1,1,1,1,1,1,1,1,1,1,1,1,1,1,1,1,1,1,1,
1,1,1,1,1,1,1,1,1,1,1,1,1,1,1,1,1,1,1,1,1,1,1,1,1,1,1,1,1,1,1,1,1,1,1,1,
1,1,1,1,1,1,1,1,1,1,1,1,1,1,1,1,1,1,1,1,1,1,1,1,1,1,1,1,1,1,1,1,1,1,1,1,
1,1,1,1,1,1,1,1,1,1,1,1,1,1,1,1,1,1,1,1,1,1,1,1,1,1,1,1,1,1,1,1,1,1,1,1,
1,1,1,1,1,1,1,1,1,1,1,1,1,1,1,1,1,1,1,1,1,1,1,1,1,1,1,1,1,1,1,1,1,1,1,1,
1,1,1,1,1,1,1,1,1,1,1,1,1,1,1,1,1,1,1,1,1,1,1,1,1,1,1,1,1,1,1,6),(2,2),
(0.143172104,0.144954128,0.146788991,0.148623853,0.150458716,0.152293578,
0.15412844,0.155963303,0.157798165,0.159633028,0.16146789,0.163302752,0.165137615,
0.166972477,0.168807339,0.170642202,0.172477064,0.174311927,0.176146789,
0.177981651,0.179816514,0.181651376,0.183486239,0.185321101,0.187155963,
0.188990826,0.190825688,0.19266055,0.194495413,0.196330275,0.198165138,
0.2,0.201834862,0.203669725,0.205504587,0.20733945,0.209174312,0.211009174,
0.212844037,0.214678899,0.216513761,0.218348624,0.220183486,0.222018349,
0.223853211,0.225688073,0.227522936,0.229357798,0.231192661,0.233027523,
0.234862385,0.236697248,0.23853211,0.240366972,0.242201835,0.244036697,
0.24587156,0.247706422,0.249541284,0.251376147,0.253211009,0.255045872,
0.256880734,0.258715596,0.260550459,0.262385321,0.264220183,0.266055046,
0.267889908,0.269724771,0.271559633,0.273394495,0.275229358,0.27706422,
0.278899083,0.280733945,0.282568807,0.28440367,0.286238532,0.288073394,
0.289908257,0.291743119,0.293577982,0.295412844,0.297247706,0.299082569,
0.300917431,0.302752294,0.304587156,0.306422018,0.308256881,0.310091743,
0.311926606,0.313761468,0.31559633,0.317431193,0.319266055,0.321100917,
0.32293578,0.324770642,0.326605505,0.328440367,0.330275229,0.332110092,
0.333944954,0.335779817,0.337614679,0.339449541,0.341284404,0.343119266,
0.344954128,0.346788991,0.348623853,0.350458716,0.352293578,0.35412844,
0.355963303,0.357798165,0.359633028,0.36146789,0.363302752,0.365137615,
0.366972477,0.368807339,0.370642202,0.372477064,0.374311927,0.376146789,
0.377981651,0.379816514,0.381651376,0.383486239,0.385321101,0.387155963,
0.388990826,0.390825688,0.39266055,0.394495413,0.396330275,0.398165138,
0.4,0.401834862,0.403669725,0.405504587,0.40733945,0.409174312,0.411009174,
0.412844037,0.414678899,0.416513761,0.418348624,0.420183486,0.422018349,
0.423853211,0.425688073,0.427522936,0.429357798,0.431192661,0.433027523,
0.434862385,0.436697248,0.43853211,0.440366972,0.442201835,0.444036697,
0.44587156,0.447706422,0.449541284,0.451376147,0.453211009,0.455045872,
0.456880734,0.458715596,0.460550459,0.462385321,0.464220183,0.466055046,
0.467889908,0.469724771,0.471559633,0.473394495,0.475229358,0.47706422,
0.478899083,0.480733945,0.482568807,0.48440367,0.486238532,0.488073394,
0.489908257,0.491743119,0.493577982,0.495412844,0.497247706,0.499082569,
0.500917431,0.502752294,0.504587156,0.506422018,0.508256881,0.510091743,
0.511926606,0.513761468,0.51559633,0.517431193,0.519266055,0.521100917,
0.52293578,0.524770642,0.526605505,0.528440367,0.530275229,0.532110092,
0.533944954,0.535779817,0.537614679,0.539449541,0.541284404,0.543119266,
0.544954128,0.546788991,0.548623853,0.550458716,0.552293578,0.55412844,
0.555963303,0.557798165,0.559633028,0.56146789,0.563302752,0.565137615,
0.566972477,0.568807339,0.570642202,0.572477064,0.574311927,0.576146789,
0.577981651,0.579816514,0.581651376,0.583486239,0.585321101,0.587155963,
0.588990826,0.590825688,0.59266055,0.594495413,0.596330275,0.598165138,
0.6,0.601834862,0.603669725,0.605504587,0.60733945,0.609174312,0.611009174,
0.612844037,0.614678899,0.616513761,0.618348624,0.620183486,0.622018349,
0.623853211,0.625688073,0.627522936,0.629357798,0.631192661,0.633027523,
0.634862385,0.636697248,0.63853211,0.640366972,0.642201835,0.644036697,
0.64587156,0.647706422,0.649541284,0.651376147,0.653211009,0.655045872,
0.656880734,0.658715596,0.660550459,0.662385321,0.664220183,0.666055046,
0.667889908,0.669724771,0.671559633,0.673394495,0.675229358,0.67706422,
0.678899083,0.680733945,0.682568807,0.68440367,0.686238532,0.688073394,
0.689908257,0.691743119,0.693577982,0.695412844,0.697247706,0.699082569,
0.700917431,0.702752294,0.704587156,0.706422018,0.708256881,0.710091743,
0.711926606,0.713761468,0.71559633,0.717431193,0.719266055,0.721100917,
0.72293578,0.724770642,0.726605505,0.728440367,0.730275229,0.732110092,
0.733944954,0.735779817,0.737614679,0.739449541,0.741284404,0.743119266,
0.744954128,0.746788991,0.748623853,0.750458716,0.752293578,0.75412844,
0.755963303,0.757798165,0.759633028,0.76146789,0.763302752,0.765137615,
0.766972477,0.768807339,0.770642202,0.772477064,0.774311927,0.776146789,
0.777981651,0.779816514,0.781651376,0.783486239,0.785321101,0.787155963,
0.788990826,0.790825688,0.79266055,0.794495413,0.796330275,0.798165138,
0.8,0.801834862,0.803669725,0.805504587,0.80733945,0.809174312,0.811009174,
0.812844037,0.814678899,0.816513761,0.818348624,0.820183486,0.822018349,
0.823853211,0.825688073,0.827522936,0.829357798,0.831192661,0.833027523,
0.834862385,0.836697248,0.83853211,0.840366972,0.842201835,0.844036697,
0.84587156,0.847706422,0.849541284,0.851376147,0.853211009,0.855045872,
0.856880734,0.858715596,0.860550459,0.862385321,0.864220183,0.866055046,
0.867889908,0.869724771,0.871559633,0.873394495,0.875229358,0.87706422,
0.878899083,0.880733945,0.882568807,0.88440367,0.886238532,0.888073394,
0.889908257,0.891743119,0.893577982,0.895412844,0.897247706,0.899082569,
0.900917431,0.902752294,0.904587156,0.906422018,0.908256881,0.910091743,
0.911926606,0.913761468,0.91559633,0.917431193,0.919266055,0.921100917,
0.92293578,0.924770642,0.926605505,0.928440367,0.930275229,0.932110092,
0.933944954,0.935779817,0.937614679,0.939449541,0.941284404,0.943119266,
0.944954128,0.946788991,0.948623853,0.950458716,0.952293578,0.95412844,
0.955963303,0.957798165,0.959633028,0.96146789,0.963302752,0.965137615,
0.966972477,0.968807339,0.970642202,0.972477064,0.974311927,0.976146789,
0.977981651,0.979816514,0.981651376,0.983486239,0.985321101,0.987155963,
0.988990826,0.990825688,0.99266055,0.994495413,0.996330275,0.998165138,
1.),(0.,0.36),.UNSPECIFIED.);
#6271=B_SPLINE_SURFACE_WITH_KNOTS('',5,1,((#246265,#246266),(#246267,#246268),
(#246269,#246270),(#246271,#246272),(#246273,#246274),(#246275,#246276),
(#246277,#246278),(#246279,#246280),(#246281,#246282),(#246283,#246284),
(#246285,#246286),(#246287,#246288),(#246289,#246290),(#246291,#246292),
(#246293,#246294),(#246295,#246296),(#246297,#246298),(#246299,#246300),
(#246301,#246302),(#246303,#246304),(#246305,#246306),(#246307,#246308),
(#246309,#246310),(#246311,#246312),(#246313,#246314),(#246315,#246316),
(#246317,#246318),(#246319,#246320),(#246321,#246322),(#246323,#246324),
(#246325,#246326),(#246327,#246328),(#246329,#246330),(#246331,#246332),
(#246333,#246334),(#246335,#246336),(#246337,#246338),(#246339,#246340),
(#246341,#246342),(#246343,#246344),(#246345,#246346),(#246347,#246348),
(#246349,#246350),(#246351,#246352),(#246353,#246354),(#246355,#246356),
(#246357,#246358),(#246359,#246360),(#246361,#246362),(#246363,#246364),
(#246365,#246366),(#246367,#246368),(#246369,#246370),(#246371,#246372),
(#246373,#246374),(#246375,#246376),(#246377,#246378),(#246379,#246380),
(#246381,#246382),(#246383,#246384),(#246385,#246386),(#246387,#246388),
(#246389,#246390),(#246391,#246392),(#246393,#246394),(#246395,#246396),
(#246397,#246398),(#246399,#246400),(#246401,#246402),(#246403,#246404),
(#246405,#246406),(#246407,#246408),(#246409,#246410),(#246411,#246412),
(#246413,#246414),(#246415,#246416),(#246417,#246418),(#246419,#246420),
(#246421,#246422),(#246423,#246424),(#246425,#246426),(#246427,#246428),
(#246429,#246430),(#246431,#246432),(#246433,#246434),(#246435,#246436),
(#246437,#246438),(#246439,#246440),(#246441,#246442),(#246443,#246444),
(#246445,#246446),(#246447,#246448),(#246449,#246450),(#246451,#246452),
(#246453,#246454),(#246455,#246456),(#246457,#246458),(#246459,#246460),
(#246461,#246462),(#246463,#246464),(#246465,#246466),(#246467,#246468),
(#246469,#246470),(#246471,#246472),(#246473,#246474),(#246475,#246476),
(#246477,#246478),(#246479,#246480),(#246481,#246482),(#246483,#246484),
(#246485,#246486),(#246487,#246488),(#246489,#246490),(#246491,#246492),
(#246493,#246494),(#246495,#246496),(#246497,#246498),(#246499,#246500),
(#246501,#246502),(#246503,#246504),(#246505,#246506),(#246507,#246508),
(#246509,#246510),(#246511,#246512),(#246513,#246514),(#246515,#246516),
(#246517,#246518),(#246519,#246520),(#246521,#246522),(#246523,#246524),
(#246525,#246526),(#246527,#246528),(#246529,#246530),(#246531,#246532),
(#246533,#246534),(#246535,#246536),(#246537,#246538),(#246539,#246540),
(#246541,#246542),(#246543,#246544),(#246545,#246546),(#246547,#246548),
(#246549,#246550),(#246551,#246552),(#246553,#246554),(#246555,#246556),
(#246557,#246558),(#246559,#246560),(#246561,#246562),(#246563,#246564),
(#246565,#246566),(#246567,#246568),(#246569,#246570),(#246571,#246572),
(#246573,#246574),(#246575,#246576),(#246577,#246578),(#246579,#246580),
(#246581,#246582),(#246583,#246584),(#246585,#246586),(#246587,#246588),
(#246589,#246590),(#246591,#246592),(#246593,#246594),(#246595,#246596),
(#246597,#246598),(#246599,#246600),(#246601,#246602),(#246603,#246604),
(#246605,#246606),(#246607,#246608),(#246609,#246610),(#246611,#246612),
(#246613,#246614),(#246615,#246616),(#246617,#246618),(#246619,#246620),
(#246621,#246622),(#246623,#246624),(#246625,#246626),(#246627,#246628),
(#246629,#246630),(#246631,#246632),(#246633,#246634),(#246635,#246636),
(#246637,#246638),(#246639,#246640),(#246641,#246642),(#246643,#246644),
(#246645,#246646),(#246647,#246648),(#246649,#246650),(#246651,#246652),
(#246653,#246654),(#246655,#246656),(#246657,#246658),(#246659,#246660),
(#246661,#246662),(#246663,#246664),(#246665,#246666),(#246667,#246668),
(#246669,#246670),(#246671,#246672),(#246673,#246674),(#246675,#246676),
(#246677,#246678),(#246679,#246680),(#246681,#246682),(#246683,#246684),
(#246685,#246686),(#246687,#246688),(#246689,#246690),(#246691,#246692),
(#246693,#246694),(#246695,#246696),(#246697,#246698),(#246699,#246700),
(#246701,#246702),(#246703,#246704),(#246705,#246706),(#246707,#246708),
(#246709,#246710),(#246711,#246712),(#246713,#246714),(#246715,#246716),
(#246717,#246718),(#246719,#246720),(#246721,#246722),(#246723,#246724),
(#246725,#246726),(#246727,#246728),(#246729,#246730),(#246731,#246732),
(#246733,#246734),(#246735,#246736),(#246737,#246738),(#246739,#246740),
(#246741,#246742),(#246743,#246744),(#246745,#246746),(#246747,#246748),
(#246749,#246750),(#246751,#246752),(#246753,#246754),(#246755,#246756),
(#246757,#246758),(#246759,#246760),(#246761,#246762),(#246763,#246764),
(#246765,#246766),(#246767,#246768),(#246769,#246770),(#246771,#246772),
(#246773,#246774),(#246775,#246776),(#246777,#246778),(#246779,#246780),
(#246781,#246782),(#246783,#246784),(#246785,#246786),(#246787,#246788),
(#246789,#246790),(#246791,#246792),(#246793,#246794),(#246795,#246796),
(#246797,#246798),(#246799,#246800),(#246801,#246802),(#246803,#246804),
(#246805,#246806),(#246807,#246808),(#246809,#246810),(#246811,#246812),
(#246813,#246814),(#246815,#246816),(#246817,#246818),(#246819,#246820),
(#246821,#246822),(#246823,#246824),(#246825,#246826),(#246827,#246828),
(#246829,#246830),(#246831,#246832),(#246833,#246834),(#246835,#246836),
(#246837,#246838),(#246839,#246840),(#246841,#246842),(#246843,#246844),
(#246845,#246846),(#246847,#246848),(#246849,#246850),(#246851,#246852),
(#246853,#246854),(#246855,#246856),(#246857,#246858),(#246859,#246860),
(#246861,#246862),(#246863,#246864),(#246865,#246866),(#246867,#246868),
(#246869,#246870),(#246871,#246872),(#246873,#246874),(#246875,#246876),
(#246877,#246878),(#246879,#246880),(#246881,#246882),(#246883,#246884),
(#246885,#246886),(#246887,#246888),(#246889,#246890),(#246891,#246892),
(#246893,#246894),(#246895,#246896),(#246897,#246898),(#246899,#246900),
(#246901,#246902),(#246903,#246904),(#246905,#246906),(#246907,#246908),
(#246909,#246910),(#246911,#246912),(#246913,#246914),(#246915,#246916),
(#246917,#246918),(#246919,#246920),(#246921,#246922),(#246923,#246924),
(#246925,#246926),(#246927,#246928),(#246929,#246930),(#246931,#246932),
(#246933,#246934),(#246935,#246936),(#246937,#246938),(#246939,#246940),
(#246941,#246942),(#246943,#246944),(#246945,#246946),(#246947,#246948),
(#246949,#246950),(#246951,#246952),(#246953,#246954),(#246955,#246956),
(#246957,#246958),(#246959,#246960),(#246961,#246962),(#246963,#246964),
(#246965,#246966),(#246967,#246968),(#246969,#246970),(#246971,#246972),
(#246973,#246974),(#246975,#246976),(#246977,#246978),(#246979,#246980),
(#246981,#246982),(#246983,#246984),(#246985,#246986),(#246987,#246988),
(#246989,#246990),(#246991,#246992),(#246993,#246994),(#246995,#246996),
(#246997,#246998),(#246999,#247000),(#247001,#247002),(#247003,#247004),
(#247005,#247006),(#247007,#247008),(#247009,#247010),(#247011,#247012),
(#247013,#247014),(#247015,#247016),(#247017,#247018),(#247019,#247020),
(#247021,#247022),(#247023,#247024),(#247025,#247026),(#247027,#247028),
(#247029,#247030),(#247031,#247032),(#247033,#247034),(#247035,#247036),
(#247037,#247038),(#247039,#247040),(#247041,#247042),(#247043,#247044),
(#247045,#247046),(#247047,#247048),(#247049,#247050),(#247051,#247052),
(#247053,#247054),(#247055,#247056),(#247057,#247058),(#247059,#247060),
(#247061,#247062),(#247063,#247064),(#247065,#247066),(#247067,#247068),
(#247069,#247070),(#247071,#247072),(#247073,#247074),(#247075,#247076),
(#247077,#247078),(#247079,#247080),(#247081,#247082),(#247083,#247084),
(#247085,#247086),(#247087,#247088),(#247089,#247090),(#247091,#247092),
(#247093,#247094),(#247095,#247096),(#247097,#247098),(#247099,#247100),
(#247101,#247102),(#247103,#247104),(#247105,#247106),(#247107,#247108),
(#247109,#247110),(#247111,#247112),(#247113,#247114),(#247115,#247116),
(#247117,#247118),(#247119,#247120),(#247121,#247122),(#247123,#247124),
(#247125,#247126),(#247127,#247128),(#247129,#247130),(#247131,#247132),
(#247133,#247134),(#247135,#247136),(#247137,#247138),(#247139,#247140),
(#247141,#247142),(#247143,#247144),(#247145,#247146),(#247147,#247148),
(#247149,#247150),(#247151,#247152),(#247153,#247154),(#247155,#247156),
(#247157,#247158),(#247159,#247160),(#247161,#247162),(#247163,#247164),
(#247165,#247166),(#247167,#247168),(#247169,#247170),(#247171,#247172),
(#247173,#247174),(#247175,#247176),(#247177,#247178),(#247179,#247180),
(#247181,#247182),(#247183,#247184),(#247185,#247186),(#247187,#247188),
(#247189,#247190),(#247191,#247192),(#247193,#247194),(#247195,#247196),
(#247197,#247198),(#247199,#247200),(#247201,#247202),(#247203,#247204),
(#247205,#247206),(#247207,#247208)),.UNSPECIFIED.,.F.,.F.,.F.,(6,1,1,1,
1,1,1,1,1,1,1,1,1,1,1,1,1,1,1,1,1,1,1,1,1,1,1,1,1,1,1,1,1,1,1,1,1,1,1,1,
1,1,1,1,1,1,1,1,1,1,1,1,1,1,1,1,1,1,1,1,1,1,1,1,1,1,1,1,1,1,1,1,1,1,1,1,
1,1,1,1,1,1,1,1,1,1,1,1,1,1,1,1,1,1,1,1,1,1,1,1,1,1,1,1,1,1,1,1,1,1,1,1,
1,1,1,1,1,1,1,1,1,1,1,1,1,1,1,1,1,1,1,1,1,1,1,1,1,1,1,1,1,1,1,1,1,1,1,1,
1,1,1,1,1,1,1,1,1,1,1,1,1,1,1,1,1,1,1,1,1,1,1,1,1,1,1,1,1,1,1,1,1,1,1,1,
1,1,1,1,1,1,1,1,1,1,1,1,1,1,1,1,1,1,1,1,1,1,1,1,1,1,1,1,1,1,1,1,1,1,1,1,
1,1,1,1,1,1,1,1,1,1,1,1,1,1,1,1,1,1,1,1,1,1,1,1,1,1,1,1,1,1,1,1,1,1,1,1,
1,1,1,1,1,1,1,1,1,1,1,1,1,1,1,1,1,1,1,1,1,1,1,1,1,1,1,1,1,1,1,1,1,1,1,1,
1,1,1,1,1,1,1,1,1,1,1,1,1,1,1,1,1,1,1,1,1,1,1,1,1,1,1,1,1,1,1,1,1,1,1,1,
1,1,1,1,1,1,1,1,1,1,1,1,1,1,1,1,1,1,1,1,1,1,1,1,1,1,1,1,1,1,1,1,1,1,1,1,
1,1,1,1,1,1,1,1,1,1,1,1,1,1,1,1,1,1,1,1,1,1,1,1,1,1,1,1,1,1,1,1,1,1,1,1,
1,1,1,1,1,1,1,1,1,1,1,1,1,1,1,1,1,1,1,1,1,1,1,1,1,1,1,1,1,1,1,1,1,1,1,1,
1,1,1,1,1,1,1,1,1,1,1,1,1,1,1,1,1,1,1,1,1,1,1,1,1,1,1,1,1,1,1,6),(2,2),
(0.143172103,0.144954128,0.146788991,0.148623853,0.150458716,0.152293578,
0.15412844,0.155963303,0.157798165,0.159633028,0.16146789,0.163302752,0.165137615,
0.166972477,0.168807339,0.170642202,0.172477064,0.174311927,0.176146789,
0.177981651,0.179816514,0.181651376,0.183486239,0.185321101,0.187155963,
0.188990826,0.190825688,0.19266055,0.194495413,0.196330275,0.198165138,
0.2,0.201834862,0.203669725,0.205504587,0.20733945,0.209174312,0.211009174,
0.212844037,0.214678899,0.216513761,0.218348624,0.220183486,0.222018349,
0.223853211,0.225688073,0.227522936,0.229357798,0.231192661,0.233027523,
0.234862385,0.236697248,0.23853211,0.240366972,0.242201835,0.244036697,
0.24587156,0.247706422,0.249541284,0.251376147,0.253211009,0.255045872,
0.256880734,0.258715596,0.260550459,0.262385321,0.264220183,0.266055046,
0.267889908,0.269724771,0.271559633,0.273394495,0.275229358,0.27706422,
0.278899083,0.280733945,0.282568807,0.28440367,0.286238532,0.288073394,
0.289908257,0.291743119,0.293577982,0.295412844,0.297247706,0.299082569,
0.300917431,0.302752294,0.304587156,0.306422018,0.308256881,0.310091743,
0.311926606,0.313761468,0.31559633,0.317431193,0.319266055,0.321100917,
0.32293578,0.324770642,0.326605505,0.328440367,0.330275229,0.332110092,
0.333944954,0.335779817,0.337614679,0.339449541,0.341284404,0.343119266,
0.344954128,0.346788991,0.348623853,0.350458716,0.352293578,0.35412844,
0.355963303,0.357798165,0.359633028,0.36146789,0.363302752,0.365137615,
0.366972477,0.368807339,0.370642202,0.372477064,0.374311927,0.376146789,
0.377981651,0.379816514,0.381651376,0.383486239,0.385321101,0.387155963,
0.388990826,0.390825688,0.39266055,0.394495413,0.396330275,0.398165138,
0.4,0.401834862,0.403669725,0.405504587,0.40733945,0.409174312,0.411009174,
0.412844037,0.414678899,0.416513761,0.418348624,0.420183486,0.422018349,
0.423853211,0.425688073,0.427522936,0.429357798,0.431192661,0.433027523,
0.434862385,0.436697248,0.43853211,0.440366972,0.442201835,0.444036697,
0.44587156,0.447706422,0.449541284,0.451376147,0.453211009,0.455045872,
0.456880734,0.458715596,0.460550459,0.462385321,0.464220183,0.466055046,
0.467889908,0.469724771,0.471559633,0.473394495,0.475229358,0.47706422,
0.478899083,0.480733945,0.482568807,0.48440367,0.486238532,0.488073394,
0.489908257,0.491743119,0.493577982,0.495412844,0.497247706,0.499082569,
0.500917431,0.502752294,0.504587156,0.506422018,0.508256881,0.510091743,
0.511926606,0.513761468,0.51559633,0.517431193,0.519266055,0.521100917,
0.52293578,0.524770642,0.526605505,0.528440367,0.530275229,0.532110092,
0.533944954,0.535779817,0.537614679,0.539449541,0.541284404,0.543119266,
0.544954128,0.546788991,0.548623853,0.550458716,0.552293578,0.55412844,
0.555963303,0.557798165,0.559633028,0.56146789,0.563302752,0.565137615,
0.566972477,0.568807339,0.570642202,0.572477064,0.574311927,0.576146789,
0.577981651,0.579816514,0.581651376,0.583486239,0.585321101,0.587155963,
0.588990826,0.590825688,0.59266055,0.594495413,0.596330275,0.598165138,
0.6,0.601834862,0.603669725,0.605504587,0.60733945,0.609174312,0.611009174,
0.612844037,0.614678899,0.616513761,0.618348624,0.620183486,0.622018349,
0.623853211,0.625688073,0.627522936,0.629357798,0.631192661,0.633027523,
0.634862385,0.636697248,0.63853211,0.640366972,0.642201835,0.644036697,
0.64587156,0.647706422,0.649541284,0.651376147,0.653211009,0.655045872,
0.656880734,0.658715596,0.660550459,0.662385321,0.664220183,0.666055046,
0.667889908,0.669724771,0.671559633,0.673394495,0.675229358,0.67706422,
0.678899083,0.680733945,0.682568807,0.68440367,0.686238532,0.688073394,
0.689908257,0.691743119,0.693577982,0.695412844,0.697247706,0.699082569,
0.700917431,0.702752294,0.704587156,0.706422018,0.708256881,0.710091743,
0.711926606,0.713761468,0.71559633,0.717431193,0.719266055,0.721100917,
0.72293578,0.724770642,0.726605505,0.728440367,0.730275229,0.732110092,
0.733944954,0.735779817,0.737614679,0.739449541,0.741284404,0.743119266,
0.744954128,0.746788991,0.748623853,0.750458716,0.752293578,0.75412844,
0.755963303,0.757798165,0.759633028,0.76146789,0.763302752,0.765137615,
0.766972477,0.768807339,0.770642202,0.772477064,0.774311927,0.776146789,
0.777981651,0.779816514,0.781651376,0.783486239,0.785321101,0.787155963,
0.788990826,0.790825688,0.79266055,0.794495413,0.796330275,0.798165138,
0.8,0.801834862,0.803669725,0.805504587,0.80733945,0.809174312,0.811009174,
0.812844037,0.814678899,0.816513761,0.818348624,0.820183486,0.822018349,
0.823853211,0.825688073,0.827522936,0.829357798,0.831192661,0.833027523,
0.834862385,0.836697248,0.83853211,0.840366972,0.842201835,0.844036697,
0.84587156,0.847706422,0.849541284,0.851376147,0.853211009,0.855045872,
0.856880734,0.858715596,0.860550459,0.862385321,0.864220183,0.866055046,
0.867889908,0.869724771,0.871559633,0.873394495,0.875229358,0.87706422,
0.878899083,0.880733945,0.882568807,0.88440367,0.886238532,0.888073394,
0.889908257,0.891743119,0.893577982,0.895412844,0.897247706,0.899082569,
0.900917431,0.902752294,0.904587156,0.906422018,0.908256881,0.910091743,
0.911926606,0.913761468,0.91559633,0.917431193,0.919266055,0.921100917,
0.92293578,0.924770642,0.926605505,0.928440367,0.930275229,0.932110092,
0.933944954,0.935779817,0.937614679,0.939449541,0.941284404,0.943119266,
0.944954128,0.946788991,0.948623853,0.950458716,0.952293578,0.95412844,
0.955963303,0.957798165,0.959633028,0.96146789,0.963302752,0.965137615,
0.966972477,0.968807339,0.970642202,0.972477064,0.974311927,0.976146789,
0.977981651,0.979816514,0.981651376,0.983486239,0.985321101,0.987155963,
0.988990826,0.990825688,0.99266055,0.994495413,0.996330275,0.998165138,
1.),(0.,0.36),.UNSPECIFIED.);
#6272=B_SPLINE_SURFACE_WITH_KNOTS('',5,1,((#247844,#247845),(#247846,#247847),
(#247848,#247849),(#247850,#247851),(#247852,#247853),(#247854,#247855),
(#247856,#247857),(#247858,#247859),(#247860,#247861),(#247862,#247863),
(#247864,#247865),(#247866,#247867),(#247868,#247869),(#247870,#247871),
(#247872,#247873),(#247874,#247875),(#247876,#247877),(#247878,#247879),
(#247880,#247881),(#247882,#247883),(#247884,#247885),(#247886,#247887),
(#247888,#247889),(#247890,#247891),(#247892,#247893),(#247894,#247895),
(#247896,#247897),(#247898,#247899),(#247900,#247901),(#247902,#247903),
(#247904,#247905),(#247906,#247907),(#247908,#247909),(#247910,#247911),
(#247912,#247913),(#247914,#247915),(#247916,#247917),(#247918,#247919),
(#247920,#247921),(#247922,#247923),(#247924,#247925),(#247926,#247927),
(#247928,#247929),(#247930,#247931),(#247932,#247933),(#247934,#247935),
(#247936,#247937),(#247938,#247939),(#247940,#247941),(#247942,#247943),
(#247944,#247945),(#247946,#247947),(#247948,#247949),(#247950,#247951),
(#247952,#247953),(#247954,#247955),(#247956,#247957),(#247958,#247959),
(#247960,#247961),(#247962,#247963),(#247964,#247965),(#247966,#247967),
(#247968,#247969),(#247970,#247971),(#247972,#247973),(#247974,#247975),
(#247976,#247977),(#247978,#247979),(#247980,#247981),(#247982,#247983),
(#247984,#247985),(#247986,#247987),(#247988,#247989),(#247990,#247991),
(#247992,#247993),(#247994,#247995),(#247996,#247997),(#247998,#247999),
(#248000,#248001),(#248002,#248003),(#248004,#248005),(#248006,#248007),
(#248008,#248009),(#248010,#248011),(#248012,#248013),(#248014,#248015),
(#248016,#248017),(#248018,#248019),(#248020,#248021),(#248022,#248023),
(#248024,#248025),(#248026,#248027),(#248028,#248029),(#248030,#248031),
(#248032,#248033),(#248034,#248035),(#248036,#248037),(#248038,#248039),
(#248040,#248041),(#248042,#248043),(#248044,#248045),(#248046,#248047),
(#248048,#248049),(#248050,#248051),(#248052,#248053),(#248054,#248055),
(#248056,#248057),(#248058,#248059),(#248060,#248061),(#248062,#248063),
(#248064,#248065),(#248066,#248067),(#248068,#248069),(#248070,#248071),
(#248072,#248073),(#248074,#248075),(#248076,#248077),(#248078,#248079),
(#248080,#248081),(#248082,#248083),(#248084,#248085),(#248086,#248087),
(#248088,#248089),(#248090,#248091),(#248092,#248093),(#248094,#248095),
(#248096,#248097),(#248098,#248099),(#248100,#248101),(#248102,#248103),
(#248104,#248105),(#248106,#248107),(#248108,#248109),(#248110,#248111),
(#248112,#248113),(#248114,#248115),(#248116,#248117),(#248118,#248119),
(#248120,#248121),(#248122,#248123),(#248124,#248125),(#248126,#248127),
(#248128,#248129),(#248130,#248131),(#248132,#248133),(#248134,#248135),
(#248136,#248137),(#248138,#248139),(#248140,#248141),(#248142,#248143),
(#248144,#248145),(#248146,#248147),(#248148,#248149),(#248150,#248151),
(#248152,#248153),(#248154,#248155),(#248156,#248157),(#248158,#248159),
(#248160,#248161),(#248162,#248163),(#248164,#248165),(#248166,#248167),
(#248168,#248169),(#248170,#248171),(#248172,#248173),(#248174,#248175),
(#248176,#248177),(#248178,#248179),(#248180,#248181),(#248182,#248183),
(#248184,#248185),(#248186,#248187),(#248188,#248189),(#248190,#248191),
(#248192,#248193),(#248194,#248195),(#248196,#248197),(#248198,#248199),
(#248200,#248201),(#248202,#248203),(#248204,#248205),(#248206,#248207),
(#248208,#248209),(#248210,#248211),(#248212,#248213),(#248214,#248215),
(#248216,#248217),(#248218,#248219),(#248220,#248221),(#248222,#248223),
(#248224,#248225),(#248226,#248227),(#248228,#248229),(#248230,#248231),
(#248232,#248233),(#248234,#248235),(#248236,#248237),(#248238,#248239),
(#248240,#248241),(#248242,#248243),(#248244,#248245),(#248246,#248247),
(#248248,#248249),(#248250,#248251),(#248252,#248253),(#248254,#248255),
(#248256,#248257),(#248258,#248259),(#248260,#248261),(#248262,#248263),
(#248264,#248265),(#248266,#248267),(#248268,#248269),(#248270,#248271),
(#248272,#248273),(#248274,#248275),(#248276,#248277),(#248278,#248279),
(#248280,#248281),(#248282,#248283),(#248284,#248285),(#248286,#248287),
(#248288,#248289),(#248290,#248291),(#248292,#248293),(#248294,#248295),
(#248296,#248297),(#248298,#248299),(#248300,#248301),(#248302,#248303),
(#248304,#248305),(#248306,#248307),(#248308,#248309),(#248310,#248311),
(#248312,#248313),(#248314,#248315),(#248316,#248317),(#248318,#248319),
(#248320,#248321),(#248322,#248323),(#248324,#248325),(#248326,#248327),
(#248328,#248329),(#248330,#248331),(#248332,#248333),(#248334,#248335),
(#248336,#248337),(#248338,#248339),(#248340,#248341),(#248342,#248343),
(#248344,#248345),(#248346,#248347),(#248348,#248349),(#248350,#248351),
(#248352,#248353),(#248354,#248355),(#248356,#248357),(#248358,#248359),
(#248360,#248361),(#248362,#248363),(#248364,#248365),(#248366,#248367),
(#248368,#248369),(#248370,#248371),(#248372,#248373),(#248374,#248375),
(#248376,#248377),(#248378,#248379),(#248380,#248381),(#248382,#248383),
(#248384,#248385),(#248386,#248387),(#248388,#248389),(#248390,#248391),
(#248392,#248393),(#248394,#248395),(#248396,#248397),(#248398,#248399),
(#248400,#248401),(#248402,#248403),(#248404,#248405),(#248406,#248407),
(#248408,#248409),(#248410,#248411),(#248412,#248413),(#248414,#248415),
(#248416,#248417),(#248418,#248419),(#248420,#248421),(#248422,#248423),
(#248424,#248425),(#248426,#248427),(#248428,#248429),(#248430,#248431),
(#248432,#248433),(#248434,#248435),(#248436,#248437),(#248438,#248439),
(#248440,#248441),(#248442,#248443),(#248444,#248445),(#248446,#248447),
(#248448,#248449),(#248450,#248451),(#248452,#248453),(#248454,#248455),
(#248456,#248457),(#248458,#248459),(#248460,#248461),(#248462,#248463),
(#248464,#248465),(#248466,#248467),(#248468,#248469),(#248470,#248471),
(#248472,#248473),(#248474,#248475),(#248476,#248477),(#248478,#248479),
(#248480,#248481),(#248482,#248483),(#248484,#248485),(#248486,#248487),
(#248488,#248489),(#248490,#248491),(#248492,#248493),(#248494,#248495),
(#248496,#248497),(#248498,#248499),(#248500,#248501),(#248502,#248503),
(#248504,#248505),(#248506,#248507),(#248508,#248509),(#248510,#248511),
(#248512,#248513),(#248514,#248515),(#248516,#248517),(#248518,#248519),
(#248520,#248521),(#248522,#248523),(#248524,#248525),(#248526,#248527),
(#248528,#248529),(#248530,#248531),(#248532,#248533),(#248534,#248535),
(#248536,#248537),(#248538,#248539),(#248540,#248541),(#248542,#248543),
(#248544,#248545),(#248546,#248547),(#248548,#248549),(#248550,#248551),
(#248552,#248553),(#248554,#248555),(#248556,#248557),(#248558,#248559),
(#248560,#248561),(#248562,#248563),(#248564,#248565),(#248566,#248567),
(#248568,#248569),(#248570,#248571),(#248572,#248573),(#248574,#248575),
(#248576,#248577),(#248578,#248579),(#248580,#248581),(#248582,#248583),
(#248584,#248585),(#248586,#248587),(#248588,#248589),(#248590,#248591),
(#248592,#248593),(#248594,#248595),(#248596,#248597),(#248598,#248599),
(#248600,#248601),(#248602,#248603),(#248604,#248605),(#248606,#248607),
(#248608,#248609),(#248610,#248611),(#248612,#248613),(#248614,#248615),
(#248616,#248617),(#248618,#248619),(#248620,#248621),(#248622,#248623),
(#248624,#248625),(#248626,#248627),(#248628,#248629),(#248630,#248631),
(#248632,#248633),(#248634,#248635),(#248636,#248637),(#248638,#248639),
(#248640,#248641),(#248642,#248643),(#248644,#248645),(#248646,#248647),
(#248648,#248649),(#248650,#248651),(#248652,#248653),(#248654,#248655),
(#248656,#248657),(#248658,#248659),(#248660,#248661),(#248662,#248663),
(#248664,#248665),(#248666,#248667),(#248668,#248669),(#248670,#248671),
(#248672,#248673),(#248674,#248675),(#248676,#248677),(#248678,#248679),
(#248680,#248681),(#248682,#248683),(#248684,#248685),(#248686,#248687),
(#248688,#248689),(#248690,#248691),(#248692,#248693),(#248694,#248695),
(#248696,#248697),(#248698,#248699),(#248700,#248701),(#248702,#248703),
(#248704,#248705),(#248706,#248707),(#248708,#248709),(#248710,#248711),
(#248712,#248713),(#248714,#248715),(#248716,#248717),(#248718,#248719),
(#248720,#248721),(#248722,#248723),(#248724,#248725),(#248726,#248727),
(#248728,#248729),(#248730,#248731),(#248732,#248733),(#248734,#248735),
(#248736,#248737),(#248738,#248739),(#248740,#248741),(#248742,#248743),
(#248744,#248745),(#248746,#248747),(#248748,#248749),(#248750,#248751),
(#248752,#248753),(#248754,#248755),(#248756,#248757),(#248758,#248759),
(#248760,#248761),(#248762,#248763),(#248764,#248765),(#248766,#248767),
(#248768,#248769),(#248770,#248771),(#248772,#248773),(#248774,#248775),
(#248776,#248777),(#248778,#248779),(#248780,#248781),(#248782,#248783),
(#248784,#248785),(#248786,#248787)),.UNSPECIFIED.,.F.,.F.,.F.,(6,1,1,1,
1,1,1,1,1,1,1,1,1,1,1,1,1,1,1,1,1,1,1,1,1,1,1,1,1,1,1,1,1,1,1,1,1,1,1,1,
1,1,1,1,1,1,1,1,1,1,1,1,1,1,1,1,1,1,1,1,1,1,1,1,1,1,1,1,1,1,1,1,1,1,1,1,
1,1,1,1,1,1,1,1,1,1,1,1,1,1,1,1,1,1,1,1,1,1,1,1,1,1,1,1,1,1,1,1,1,1,1,1,
1,1,1,1,1,1,1,1,1,1,1,1,1,1,1,1,1,1,1,1,1,1,1,1,1,1,1,1,1,1,1,1,1,1,1,1,
1,1,1,1,1,1,1,1,1,1,1,1,1,1,1,1,1,1,1,1,1,1,1,1,1,1,1,1,1,1,1,1,1,1,1,1,
1,1,1,1,1,1,1,1,1,1,1,1,1,1,1,1,1,1,1,1,1,1,1,1,1,1,1,1,1,1,1,1,1,1,1,1,
1,1,1,1,1,1,1,1,1,1,1,1,1,1,1,1,1,1,1,1,1,1,1,1,1,1,1,1,1,1,1,1,1,1,1,1,
1,1,1,1,1,1,1,1,1,1,1,1,1,1,1,1,1,1,1,1,1,1,1,1,1,1,1,1,1,1,1,1,1,1,1,1,
1,1,1,1,1,1,1,1,1,1,1,1,1,1,1,1,1,1,1,1,1,1,1,1,1,1,1,1,1,1,1,1,1,1,1,1,
1,1,1,1,1,1,1,1,1,1,1,1,1,1,1,1,1,1,1,1,1,1,1,1,1,1,1,1,1,1,1,1,1,1,1,1,
1,1,1,1,1,1,1,1,1,1,1,1,1,1,1,1,1,1,1,1,1,1,1,1,1,1,1,1,1,1,1,1,1,1,1,1,
1,1,1,1,1,1,1,1,1,1,1,1,1,1,1,1,1,1,1,1,1,1,1,1,1,1,1,1,1,1,1,1,1,1,1,1,
1,1,1,1,1,1,1,1,1,1,1,1,1,1,1,1,1,1,1,1,1,1,1,1,1,1,1,1,1,1,1,6),(2,2),
(-1.,-0.998165138,-0.996330275,-0.994495413,-0.99266055,-0.990825688,-0.988990826,
-0.987155963,-0.985321101,-0.983486239,-0.981651376,-0.979816514,-0.977981651,
-0.976146789,-0.974311927,-0.972477064,-0.970642202,-0.968807339,-0.966972477,
-0.965137615,-0.963302752,-0.96146789,-0.959633028,-0.957798165,-0.955963303,
-0.95412844,-0.952293578,-0.950458716,-0.948623853,-0.946788991,-0.944954128,
-0.943119266,-0.941284404,-0.939449541,-0.937614679,-0.935779817,-0.933944954,
-0.932110092,-0.930275229,-0.928440367,-0.926605505,-0.924770642,-0.92293578,
-0.921100917,-0.919266055,-0.917431193,-0.91559633,-0.913761468,-0.911926606,
-0.910091743,-0.908256881,-0.906422018,-0.904587156,-0.902752294,-0.900917431,
-0.899082569,-0.897247706,-0.895412844,-0.893577982,-0.891743119,-0.889908257,
-0.888073394,-0.886238532,-0.88440367,-0.882568807,-0.880733945,-0.878899083,
-0.87706422,-0.875229358,-0.873394495,-0.871559633,-0.869724771,-0.867889908,
-0.866055046,-0.864220183,-0.862385321,-0.860550459,-0.858715596,-0.856880734,
-0.855045872,-0.853211009,-0.851376147,-0.849541284,-0.847706422,-0.84587156,
-0.844036697,-0.842201835,-0.840366972,-0.83853211,-0.836697248,-0.834862385,
-0.833027523,-0.831192661,-0.829357798,-0.827522936,-0.825688073,-0.823853211,
-0.822018349,-0.820183486,-0.818348624,-0.816513761,-0.814678899,-0.812844037,
-0.811009174,-0.809174312,-0.80733945,-0.805504587,-0.803669725,-0.801834862,
-0.8,-0.798165138,-0.796330275,-0.794495413,-0.79266055,-0.790825688,-0.788990826,
-0.787155963,-0.785321101,-0.783486239,-0.781651376,-0.779816514,-0.777981651,
-0.776146789,-0.774311927,-0.772477064,-0.770642202,-0.768807339,-0.766972477,
-0.765137615,-0.763302752,-0.76146789,-0.759633028,-0.757798165,-0.755963303,
-0.75412844,-0.752293578,-0.750458716,-0.748623853,-0.746788991,-0.744954128,
-0.743119266,-0.741284404,-0.739449541,-0.737614679,-0.735779817,-0.733944954,
-0.732110092,-0.730275229,-0.728440367,-0.726605505,-0.724770642,-0.72293578,
-0.721100917,-0.719266055,-0.717431193,-0.71559633,-0.713761468,-0.711926606,
-0.710091743,-0.708256881,-0.706422018,-0.704587156,-0.702752294,-0.700917431,
-0.699082569,-0.697247706,-0.695412844,-0.693577982,-0.691743119,-0.689908257,
-0.688073394,-0.686238532,-0.68440367,-0.682568807,-0.680733945,-0.678899083,
-0.67706422,-0.675229358,-0.673394495,-0.671559633,-0.669724771,-0.667889908,
-0.666055046,-0.664220183,-0.662385321,-0.660550459,-0.658715596,-0.656880734,
-0.655045872,-0.653211009,-0.651376147,-0.649541284,-0.647706422,-0.64587156,
-0.644036697,-0.642201835,-0.640366972,-0.63853211,-0.636697248,-0.634862385,
-0.633027523,-0.631192661,-0.629357798,-0.627522936,-0.625688073,-0.623853211,
-0.622018349,-0.620183486,-0.618348624,-0.616513761,-0.614678899,-0.612844037,
-0.611009174,-0.609174312,-0.60733945,-0.605504587,-0.603669725,-0.601834862,
-0.6,-0.598165138,-0.596330275,-0.594495413,-0.59266055,-0.590825688,-0.588990826,
-0.587155963,-0.585321101,-0.583486239,-0.581651376,-0.579816514,-0.577981651,
-0.576146789,-0.574311927,-0.572477064,-0.570642202,-0.568807339,-0.566972477,
-0.565137615,-0.563302752,-0.56146789,-0.559633028,-0.557798165,-0.555963303,
-0.55412844,-0.552293578,-0.550458716,-0.548623853,-0.546788991,-0.544954128,
-0.543119266,-0.541284404,-0.539449541,-0.537614679,-0.535779817,-0.533944954,
-0.532110092,-0.530275229,-0.528440367,-0.526605505,-0.524770642,-0.52293578,
-0.521100917,-0.519266055,-0.517431193,-0.51559633,-0.513761468,-0.511926606,
-0.510091743,-0.508256881,-0.506422018,-0.504587156,-0.502752294,-0.500917431,
-0.499082569,-0.497247706,-0.495412844,-0.493577982,-0.491743119,-0.489908257,
-0.488073394,-0.486238532,-0.48440367,-0.482568807,-0.480733945,-0.478899083,
-0.47706422,-0.475229358,-0.473394495,-0.471559633,-0.469724771,-0.467889908,
-0.466055046,-0.464220183,-0.462385321,-0.460550459,-0.458715596,-0.456880734,
-0.455045872,-0.453211009,-0.451376147,-0.449541284,-0.447706422,-0.44587156,
-0.444036697,-0.442201835,-0.440366972,-0.43853211,-0.436697248,-0.434862385,
-0.433027523,-0.431192661,-0.429357798,-0.427522936,-0.425688073,-0.423853211,
-0.422018349,-0.420183486,-0.418348624,-0.416513761,-0.414678899,-0.412844037,
-0.411009174,-0.409174312,-0.40733945,-0.405504587,-0.403669725,-0.401834862,
-0.4,-0.398165138,-0.396330275,-0.394495413,-0.39266055,-0.390825688,-0.388990826,
-0.387155963,-0.385321101,-0.383486239,-0.381651376,-0.379816514,-0.377981651,
-0.376146789,-0.374311927,-0.372477064,-0.370642202,-0.368807339,-0.366972477,
-0.365137615,-0.363302752,-0.36146789,-0.359633028,-0.357798165,-0.355963303,
-0.35412844,-0.352293578,-0.350458716,-0.348623853,-0.346788991,-0.344954128,
-0.343119266,-0.341284404,-0.339449541,-0.337614679,-0.335779817,-0.333944954,
-0.332110092,-0.330275229,-0.328440367,-0.326605505,-0.324770642,-0.32293578,
-0.321100917,-0.319266055,-0.317431193,-0.31559633,-0.313761468,-0.311926606,
-0.310091743,-0.308256881,-0.306422018,-0.304587156,-0.302752294,-0.300917431,
-0.299082569,-0.297247706,-0.295412844,-0.293577982,-0.291743119,-0.289908257,
-0.288073394,-0.286238532,-0.28440367,-0.282568807,-0.280733945,-0.278899083,
-0.27706422,-0.275229358,-0.273394495,-0.271559633,-0.269724771,-0.267889908,
-0.266055046,-0.264220183,-0.262385321,-0.260550459,-0.258715596,-0.256880734,
-0.255045872,-0.253211009,-0.251376147,-0.249541284,-0.247706422,-0.24587156,
-0.244036697,-0.242201835,-0.240366972,-0.23853211,-0.236697248,-0.234862385,
-0.233027523,-0.231192661,-0.229357798,-0.227522936,-0.225688073,-0.223853211,
-0.222018349,-0.220183486,-0.218348624,-0.216513761,-0.214678899,-0.212844037,
-0.211009174,-0.209174312,-0.20733945,-0.205504587,-0.203669725,-0.201834862,
-0.2,-0.198165138,-0.196330275,-0.194495413,-0.19266055,-0.190825688,-0.188990826,
-0.187155963,-0.185321101,-0.183486239,-0.181651376,-0.179816514,-0.177981651,
-0.176146789,-0.174311927,-0.172477064,-0.170642202,-0.168807339,-0.166972477,
-0.165137615,-0.163302752,-0.16146789,-0.159633028,-0.157798165,-0.155963303,
-0.15412844,-0.152293578,-0.150458716,-0.148623853,-0.146788991,-0.144954128,
-0.143172103),(0.,0.36),.UNSPECIFIED.);
#6273=B_SPLINE_SURFACE_WITH_KNOTS('',5,1,((#249438,#249439),(#249440,#249441),
(#249442,#249443),(#249444,#249445),(#249446,#249447),(#249448,#249449),
(#249450,#249451),(#249452,#249453),(#249454,#249455),(#249456,#249457),
(#249458,#249459),(#249460,#249461),(#249462,#249463),(#249464,#249465),
(#249466,#249467),(#249468,#249469),(#249470,#249471),(#249472,#249473),
(#249474,#249475),(#249476,#249477),(#249478,#249479),(#249480,#249481),
(#249482,#249483),(#249484,#249485),(#249486,#249487),(#249488,#249489),
(#249490,#249491),(#249492,#249493),(#249494,#249495),(#249496,#249497),
(#249498,#249499),(#249500,#249501),(#249502,#249503),(#249504,#249505),
(#249506,#249507),(#249508,#249509),(#249510,#249511),(#249512,#249513),
(#249514,#249515),(#249516,#249517),(#249518,#249519),(#249520,#249521),
(#249522,#249523),(#249524,#249525),(#249526,#249527),(#249528,#249529),
(#249530,#249531),(#249532,#249533),(#249534,#249535),(#249536,#249537),
(#249538,#249539),(#249540,#249541),(#249542,#249543),(#249544,#249545),
(#249546,#249547),(#249548,#249549),(#249550,#249551),(#249552,#249553),
(#249554,#249555),(#249556,#249557),(#249558,#249559),(#249560,#249561),
(#249562,#249563),(#249564,#249565),(#249566,#249567),(#249568,#249569),
(#249570,#249571),(#249572,#249573),(#249574,#249575),(#249576,#249577),
(#249578,#249579),(#249580,#249581),(#249582,#249583),(#249584,#249585),
(#249586,#249587),(#249588,#249589),(#249590,#249591),(#249592,#249593),
(#249594,#249595),(#249596,#249597),(#249598,#249599),(#249600,#249601),
(#249602,#249603),(#249604,#249605),(#249606,#249607),(#249608,#249609),
(#249610,#249611),(#249612,#249613),(#249614,#249615),(#249616,#249617),
(#249618,#249619),(#249620,#249621),(#249622,#249623),(#249624,#249625),
(#249626,#249627),(#249628,#249629),(#249630,#249631),(#249632,#249633),
(#249634,#249635),(#249636,#249637),(#249638,#249639),(#249640,#249641),
(#249642,#249643),(#249644,#249645),(#249646,#249647),(#249648,#249649),
(#249650,#249651),(#249652,#249653),(#249654,#249655),(#249656,#249657),
(#249658,#249659),(#249660,#249661),(#249662,#249663),(#249664,#249665),
(#249666,#249667),(#249668,#249669),(#249670,#249671),(#249672,#249673),
(#249674,#249675),(#249676,#249677),(#249678,#249679),(#249680,#249681),
(#249682,#249683),(#249684,#249685),(#249686,#249687),(#249688,#249689),
(#249690,#249691),(#249692,#249693),(#249694,#249695),(#249696,#249697),
(#249698,#249699),(#249700,#249701),(#249702,#249703),(#249704,#249705),
(#249706,#249707),(#249708,#249709),(#249710,#249711),(#249712,#249713),
(#249714,#249715),(#249716,#249717),(#249718,#249719),(#249720,#249721),
(#249722,#249723),(#249724,#249725),(#249726,#249727),(#249728,#249729),
(#249730,#249731),(#249732,#249733),(#249734,#249735),(#249736,#249737),
(#249738,#249739),(#249740,#249741),(#249742,#249743),(#249744,#249745),
(#249746,#249747),(#249748,#249749),(#249750,#249751),(#249752,#249753),
(#249754,#249755),(#249756,#249757),(#249758,#249759),(#249760,#249761),
(#249762,#249763),(#249764,#249765),(#249766,#249767),(#249768,#249769),
(#249770,#249771),(#249772,#249773),(#249774,#249775),(#249776,#249777),
(#249778,#249779),(#249780,#249781),(#249782,#249783),(#249784,#249785),
(#249786,#249787),(#249788,#249789),(#249790,#249791),(#249792,#249793),
(#249794,#249795),(#249796,#249797),(#249798,#249799),(#249800,#249801),
(#249802,#249803),(#249804,#249805),(#249806,#249807),(#249808,#249809),
(#249810,#249811),(#249812,#249813),(#249814,#249815),(#249816,#249817),
(#249818,#249819),(#249820,#249821),(#249822,#249823),(#249824,#249825),
(#249826,#249827),(#249828,#249829),(#249830,#249831),(#249832,#249833),
(#249834,#249835),(#249836,#249837),(#249838,#249839),(#249840,#249841),
(#249842,#249843),(#249844,#249845),(#249846,#249847),(#249848,#249849),
(#249850,#249851),(#249852,#249853),(#249854,#249855),(#249856,#249857),
(#249858,#249859),(#249860,#249861),(#249862,#249863),(#249864,#249865),
(#249866,#249867),(#249868,#249869),(#249870,#249871),(#249872,#249873),
(#249874,#249875),(#249876,#249877),(#249878,#249879),(#249880,#249881),
(#249882,#249883),(#249884,#249885),(#249886,#249887),(#249888,#249889),
(#249890,#249891),(#249892,#249893),(#249894,#249895),(#249896,#249897),
(#249898,#249899),(#249900,#249901),(#249902,#249903),(#249904,#249905),
(#249906,#249907),(#249908,#249909),(#249910,#249911),(#249912,#249913),
(#249914,#249915),(#249916,#249917),(#249918,#249919),(#249920,#249921),
(#249922,#249923),(#249924,#249925),(#249926,#249927),(#249928,#249929),
(#249930,#249931),(#249932,#249933),(#249934,#249935),(#249936,#249937),
(#249938,#249939),(#249940,#249941),(#249942,#249943),(#249944,#249945),
(#249946,#249947),(#249948,#249949),(#249950,#249951),(#249952,#249953),
(#249954,#249955),(#249956,#249957),(#249958,#249959),(#249960,#249961),
(#249962,#249963),(#249964,#249965),(#249966,#249967),(#249968,#249969),
(#249970,#249971),(#249972,#249973),(#249974,#249975),(#249976,#249977),
(#249978,#249979),(#249980,#249981),(#249982,#249983),(#249984,#249985),
(#249986,#249987),(#249988,#249989),(#249990,#249991),(#249992,#249993),
(#249994,#249995),(#249996,#249997),(#249998,#249999),(#250000,#250001),
(#250002,#250003),(#250004,#250005),(#250006,#250007),(#250008,#250009),
(#250010,#250011),(#250012,#250013),(#250014,#250015),(#250016,#250017),
(#250018,#250019),(#250020,#250021),(#250022,#250023),(#250024,#250025),
(#250026,#250027),(#250028,#250029),(#250030,#250031),(#250032,#250033),
(#250034,#250035),(#250036,#250037),(#250038,#250039),(#250040,#250041),
(#250042,#250043),(#250044,#250045),(#250046,#250047),(#250048,#250049),
(#250050,#250051),(#250052,#250053),(#250054,#250055),(#250056,#250057),
(#250058,#250059),(#250060,#250061),(#250062,#250063),(#250064,#250065),
(#250066,#250067),(#250068,#250069),(#250070,#250071),(#250072,#250073),
(#250074,#250075),(#250076,#250077),(#250078,#250079),(#250080,#250081),
(#250082,#250083),(#250084,#250085),(#250086,#250087),(#250088,#250089),
(#250090,#250091),(#250092,#250093),(#250094,#250095),(#250096,#250097),
(#250098,#250099),(#250100,#250101),(#250102,#250103),(#250104,#250105),
(#250106,#250107),(#250108,#250109),(#250110,#250111),(#250112,#250113),
(#250114,#250115),(#250116,#250117),(#250118,#250119),(#250120,#250121),
(#250122,#250123),(#250124,#250125),(#250126,#250127),(#250128,#250129),
(#250130,#250131),(#250132,#250133),(#250134,#250135),(#250136,#250137),
(#250138,#250139),(#250140,#250141),(#250142,#250143),(#250144,#250145),
(#250146,#250147),(#250148,#250149),(#250150,#250151),(#250152,#250153),
(#250154,#250155),(#250156,#250157),(#250158,#250159),(#250160,#250161),
(#250162,#250163),(#250164,#250165),(#250166,#250167),(#250168,#250169),
(#250170,#250171),(#250172,#250173),(#250174,#250175),(#250176,#250177),
(#250178,#250179),(#250180,#250181),(#250182,#250183),(#250184,#250185),
(#250186,#250187),(#250188,#250189),(#250190,#250191),(#250192,#250193),
(#250194,#250195),(#250196,#250197),(#250198,#250199),(#250200,#250201),
(#250202,#250203),(#250204,#250205),(#250206,#250207),(#250208,#250209),
(#250210,#250211),(#250212,#250213),(#250214,#250215),(#250216,#250217),
(#250218,#250219),(#250220,#250221),(#250222,#250223),(#250224,#250225),
(#250226,#250227),(#250228,#250229),(#250230,#250231),(#250232,#250233),
(#250234,#250235),(#250236,#250237),(#250238,#250239),(#250240,#250241),
(#250242,#250243),(#250244,#250245),(#250246,#250247),(#250248,#250249),
(#250250,#250251),(#250252,#250253),(#250254,#250255),(#250256,#250257),
(#250258,#250259),(#250260,#250261),(#250262,#250263),(#250264,#250265),
(#250266,#250267),(#250268,#250269),(#250270,#250271),(#250272,#250273),
(#250274,#250275),(#250276,#250277),(#250278,#250279),(#250280,#250281),
(#250282,#250283),(#250284,#250285),(#250286,#250287),(#250288,#250289),
(#250290,#250291),(#250292,#250293),(#250294,#250295),(#250296,#250297),
(#250298,#250299),(#250300,#250301),(#250302,#250303),(#250304,#250305),
(#250306,#250307),(#250308,#250309),(#250310,#250311),(#250312,#250313),
(#250314,#250315),(#250316,#250317),(#250318,#250319),(#250320,#250321),
(#250322,#250323),(#250324,#250325),(#250326,#250327),(#250328,#250329),
(#250330,#250331),(#250332,#250333),(#250334,#250335),(#250336,#250337),
(#250338,#250339),(#250340,#250341),(#250342,#250343),(#250344,#250345),
(#250346,#250347),(#250348,#250349),(#250350,#250351),(#250352,#250353),
(#250354,#250355),(#250356,#250357),(#250358,#250359),(#250360,#250361),
(#250362,#250363),(#250364,#250365),(#250366,#250367),(#250368,#250369),
(#250370,#250371),(#250372,#250373),(#250374,#250375),(#250376,#250377),
(#250378,#250379),(#250380,#250381)),.UNSPECIFIED.,.F.,.F.,.F.,(6,1,1,1,
1,1,1,1,1,1,1,1,1,1,1,1,1,1,1,1,1,1,1,1,1,1,1,1,1,1,1,1,1,1,1,1,1,1,1,1,
1,1,1,1,1,1,1,1,1,1,1,1,1,1,1,1,1,1,1,1,1,1,1,1,1,1,1,1,1,1,1,1,1,1,1,1,
1,1,1,1,1,1,1,1,1,1,1,1,1,1,1,1,1,1,1,1,1,1,1,1,1,1,1,1,1,1,1,1,1,1,1,1,
1,1,1,1,1,1,1,1,1,1,1,1,1,1,1,1,1,1,1,1,1,1,1,1,1,1,1,1,1,1,1,1,1,1,1,1,
1,1,1,1,1,1,1,1,1,1,1,1,1,1,1,1,1,1,1,1,1,1,1,1,1,1,1,1,1,1,1,1,1,1,1,1,
1,1,1,1,1,1,1,1,1,1,1,1,1,1,1,1,1,1,1,1,1,1,1,1,1,1,1,1,1,1,1,1,1,1,1,1,
1,1,1,1,1,1,1,1,1,1,1,1,1,1,1,1,1,1,1,1,1,1,1,1,1,1,1,1,1,1,1,1,1,1,1,1,
1,1,1,1,1,1,1,1,1,1,1,1,1,1,1,1,1,1,1,1,1,1,1,1,1,1,1,1,1,1,1,1,1,1,1,1,
1,1,1,1,1,1,1,1,1,1,1,1,1,1,1,1,1,1,1,1,1,1,1,1,1,1,1,1,1,1,1,1,1,1,1,1,
1,1,1,1,1,1,1,1,1,1,1,1,1,1,1,1,1,1,1,1,1,1,1,1,1,1,1,1,1,1,1,1,1,1,1,1,
1,1,1,1,1,1,1,1,1,1,1,1,1,1,1,1,1,1,1,1,1,1,1,1,1,1,1,1,1,1,1,1,1,1,1,1,
1,1,1,1,1,1,1,1,1,1,1,1,1,1,1,1,1,1,1,1,1,1,1,1,1,1,1,1,1,1,1,1,1,1,1,1,
1,1,1,1,1,1,1,1,1,1,1,1,1,1,1,1,1,1,1,1,1,1,1,1,1,1,1,1,1,1,1,6),(2,2),
(-1.,-0.998165138,-0.996330275,-0.994495413,-0.99266055,-0.990825688,-0.988990826,
-0.987155963,-0.985321101,-0.983486239,-0.981651376,-0.979816514,-0.977981651,
-0.976146789,-0.974311927,-0.972477064,-0.970642202,-0.968807339,-0.966972477,
-0.965137615,-0.963302752,-0.96146789,-0.959633028,-0.957798165,-0.955963303,
-0.95412844,-0.952293578,-0.950458716,-0.948623853,-0.946788991,-0.944954128,
-0.943119266,-0.941284404,-0.939449541,-0.937614679,-0.935779817,-0.933944954,
-0.932110092,-0.930275229,-0.928440367,-0.926605505,-0.924770642,-0.92293578,
-0.921100917,-0.919266055,-0.917431193,-0.91559633,-0.913761468,-0.911926606,
-0.910091743,-0.908256881,-0.906422018,-0.904587156,-0.902752294,-0.900917431,
-0.899082569,-0.897247706,-0.895412844,-0.893577982,-0.891743119,-0.889908257,
-0.888073394,-0.886238532,-0.88440367,-0.882568807,-0.880733945,-0.878899083,
-0.87706422,-0.875229358,-0.873394495,-0.871559633,-0.869724771,-0.867889908,
-0.866055046,-0.864220183,-0.862385321,-0.860550459,-0.858715596,-0.856880734,
-0.855045872,-0.853211009,-0.851376147,-0.849541284,-0.847706422,-0.84587156,
-0.844036697,-0.842201835,-0.840366972,-0.83853211,-0.836697248,-0.834862385,
-0.833027523,-0.831192661,-0.829357798,-0.827522936,-0.825688073,-0.823853211,
-0.822018349,-0.820183486,-0.818348624,-0.816513761,-0.814678899,-0.812844037,
-0.811009174,-0.809174312,-0.80733945,-0.805504587,-0.803669725,-0.801834862,
-0.8,-0.798165138,-0.796330275,-0.794495413,-0.79266055,-0.790825688,-0.788990826,
-0.787155963,-0.785321101,-0.783486239,-0.781651376,-0.779816514,-0.777981651,
-0.776146789,-0.774311927,-0.772477064,-0.770642202,-0.768807339,-0.766972477,
-0.765137615,-0.763302752,-0.76146789,-0.759633028,-0.757798165,-0.755963303,
-0.75412844,-0.752293578,-0.750458716,-0.748623853,-0.746788991,-0.744954128,
-0.743119266,-0.741284404,-0.739449541,-0.737614679,-0.735779817,-0.733944954,
-0.732110092,-0.730275229,-0.728440367,-0.726605505,-0.724770642,-0.72293578,
-0.721100917,-0.719266055,-0.717431193,-0.71559633,-0.713761468,-0.711926606,
-0.710091743,-0.708256881,-0.706422018,-0.704587156,-0.702752294,-0.700917431,
-0.699082569,-0.697247706,-0.695412844,-0.693577982,-0.691743119,-0.689908257,
-0.688073394,-0.686238532,-0.68440367,-0.682568807,-0.680733945,-0.678899083,
-0.67706422,-0.675229358,-0.673394495,-0.671559633,-0.669724771,-0.667889908,
-0.666055046,-0.664220183,-0.662385321,-0.660550459,-0.658715596,-0.656880734,
-0.655045872,-0.653211009,-0.651376147,-0.649541284,-0.647706422,-0.64587156,
-0.644036697,-0.642201835,-0.640366972,-0.63853211,-0.636697248,-0.634862385,
-0.633027523,-0.631192661,-0.629357798,-0.627522936,-0.625688073,-0.623853211,
-0.622018349,-0.620183486,-0.618348624,-0.616513761,-0.614678899,-0.612844037,
-0.611009174,-0.609174312,-0.60733945,-0.605504587,-0.603669725,-0.601834862,
-0.6,-0.598165138,-0.596330275,-0.594495413,-0.59266055,-0.590825688,-0.588990826,
-0.587155963,-0.585321101,-0.583486239,-0.581651376,-0.579816514,-0.577981651,
-0.576146789,-0.574311927,-0.572477064,-0.570642202,-0.568807339,-0.566972477,
-0.565137615,-0.563302752,-0.56146789,-0.559633028,-0.557798165,-0.555963303,
-0.55412844,-0.552293578,-0.550458716,-0.548623853,-0.546788991,-0.544954128,
-0.543119266,-0.541284404,-0.539449541,-0.537614679,-0.535779817,-0.533944954,
-0.532110092,-0.530275229,-0.528440367,-0.526605505,-0.524770642,-0.52293578,
-0.521100917,-0.519266055,-0.517431193,-0.51559633,-0.513761468,-0.511926606,
-0.510091743,-0.508256881,-0.506422018,-0.504587156,-0.502752294,-0.500917431,
-0.499082569,-0.497247706,-0.495412844,-0.493577982,-0.491743119,-0.489908257,
-0.488073394,-0.486238532,-0.48440367,-0.482568807,-0.480733945,-0.478899083,
-0.47706422,-0.475229358,-0.473394495,-0.471559633,-0.469724771,-0.467889908,
-0.466055046,-0.464220183,-0.462385321,-0.460550459,-0.458715596,-0.456880734,
-0.455045872,-0.453211009,-0.451376147,-0.449541284,-0.447706422,-0.44587156,
-0.444036697,-0.442201835,-0.440366972,-0.43853211,-0.436697248,-0.434862385,
-0.433027523,-0.431192661,-0.429357798,-0.427522936,-0.425688073,-0.423853211,
-0.422018349,-0.420183486,-0.418348624,-0.416513761,-0.414678899,-0.412844037,
-0.411009174,-0.409174312,-0.40733945,-0.405504587,-0.403669725,-0.401834862,
-0.4,-0.398165138,-0.396330275,-0.394495413,-0.39266055,-0.390825688,-0.388990826,
-0.387155963,-0.385321101,-0.383486239,-0.381651376,-0.379816514,-0.377981651,
-0.376146789,-0.374311927,-0.372477064,-0.370642202,-0.368807339,-0.366972477,
-0.365137615,-0.363302752,-0.36146789,-0.359633028,-0.357798165,-0.355963303,
-0.35412844,-0.352293578,-0.350458716,-0.348623853,-0.346788991,-0.344954128,
-0.343119266,-0.341284404,-0.339449541,-0.337614679,-0.335779817,-0.333944954,
-0.332110092,-0.330275229,-0.328440367,-0.326605505,-0.324770642,-0.32293578,
-0.321100917,-0.319266055,-0.317431193,-0.31559633,-0.313761468,-0.311926606,
-0.310091743,-0.308256881,-0.306422018,-0.304587156,-0.302752294,-0.300917431,
-0.299082569,-0.297247706,-0.295412844,-0.293577982,-0.291743119,-0.289908257,
-0.288073394,-0.286238532,-0.28440367,-0.282568807,-0.280733945,-0.278899083,
-0.27706422,-0.275229358,-0.273394495,-0.271559633,-0.269724771,-0.267889908,
-0.266055046,-0.264220183,-0.262385321,-0.260550459,-0.258715596,-0.256880734,
-0.255045872,-0.253211009,-0.251376147,-0.249541284,-0.247706422,-0.24587156,
-0.244036697,-0.242201835,-0.240366972,-0.23853211,-0.236697248,-0.234862385,
-0.233027523,-0.231192661,-0.229357798,-0.227522936,-0.225688073,-0.223853211,
-0.222018349,-0.220183486,-0.218348624,-0.216513761,-0.214678899,-0.212844037,
-0.211009174,-0.209174312,-0.20733945,-0.205504587,-0.203669725,-0.201834862,
-0.2,-0.198165138,-0.196330275,-0.194495413,-0.19266055,-0.190825688,-0.188990826,
-0.187155963,-0.185321101,-0.183486239,-0.181651376,-0.179816514,-0.177981651,
-0.176146789,-0.174311927,-0.172477064,-0.170642202,-0.168807339,-0.166972477,
-0.165137615,-0.163302752,-0.16146789,-0.159633028,-0.157798165,-0.155963303,
-0.15412844,-0.152293578,-0.150458716,-0.148623853,-0.146788991,-0.144954128,
-0.143172103),(0.,0.36),.UNSPECIFIED.);
#6274=B_SPLINE_SURFACE_WITH_KNOTS('',5,1,((#251023,#251024),(#251025,#251026),
(#251027,#251028),(#251029,#251030),(#251031,#251032),(#251033,#251034),
(#251035,#251036),(#251037,#251038),(#251039,#251040),(#251041,#251042),
(#251043,#251044),(#251045,#251046),(#251047,#251048),(#251049,#251050),
(#251051,#251052),(#251053,#251054),(#251055,#251056),(#251057,#251058),
(#251059,#251060),(#251061,#251062),(#251063,#251064),(#251065,#251066),
(#251067,#251068),(#251069,#251070),(#251071,#251072),(#251073,#251074),
(#251075,#251076),(#251077,#251078),(#251079,#251080),(#251081,#251082),
(#251083,#251084),(#251085,#251086),(#251087,#251088),(#251089,#251090),
(#251091,#251092),(#251093,#251094),(#251095,#251096),(#251097,#251098),
(#251099,#251100),(#251101,#251102),(#251103,#251104),(#251105,#251106),
(#251107,#251108),(#251109,#251110),(#251111,#251112),(#251113,#251114),
(#251115,#251116),(#251117,#251118),(#251119,#251120),(#251121,#251122),
(#251123,#251124),(#251125,#251126),(#251127,#251128),(#251129,#251130),
(#251131,#251132),(#251133,#251134),(#251135,#251136),(#251137,#251138),
(#251139,#251140),(#251141,#251142),(#251143,#251144),(#251145,#251146),
(#251147,#251148),(#251149,#251150),(#251151,#251152),(#251153,#251154),
(#251155,#251156),(#251157,#251158),(#251159,#251160),(#251161,#251162),
(#251163,#251164),(#251165,#251166),(#251167,#251168),(#251169,#251170),
(#251171,#251172),(#251173,#251174),(#251175,#251176),(#251177,#251178),
(#251179,#251180),(#251181,#251182),(#251183,#251184),(#251185,#251186),
(#251187,#251188),(#251189,#251190),(#251191,#251192),(#251193,#251194),
(#251195,#251196),(#251197,#251198),(#251199,#251200),(#251201,#251202),
(#251203,#251204),(#251205,#251206),(#251207,#251208),(#251209,#251210),
(#251211,#251212),(#251213,#251214),(#251215,#251216),(#251217,#251218),
(#251219,#251220),(#251221,#251222),(#251223,#251224),(#251225,#251226),
(#251227,#251228),(#251229,#251230),(#251231,#251232),(#251233,#251234),
(#251235,#251236),(#251237,#251238),(#251239,#251240),(#251241,#251242),
(#251243,#251244),(#251245,#251246),(#251247,#251248),(#251249,#251250),
(#251251,#251252),(#251253,#251254),(#251255,#251256),(#251257,#251258),
(#251259,#251260),(#251261,#251262),(#251263,#251264),(#251265,#251266),
(#251267,#251268),(#251269,#251270),(#251271,#251272),(#251273,#251274),
(#251275,#251276),(#251277,#251278),(#251279,#251280),(#251281,#251282),
(#251283,#251284),(#251285,#251286),(#251287,#251288),(#251289,#251290),
(#251291,#251292),(#251293,#251294),(#251295,#251296),(#251297,#251298),
(#251299,#251300),(#251301,#251302),(#251303,#251304),(#251305,#251306),
(#251307,#251308),(#251309,#251310),(#251311,#251312),(#251313,#251314),
(#251315,#251316),(#251317,#251318),(#251319,#251320),(#251321,#251322),
(#251323,#251324),(#251325,#251326),(#251327,#251328),(#251329,#251330),
(#251331,#251332),(#251333,#251334),(#251335,#251336),(#251337,#251338),
(#251339,#251340),(#251341,#251342),(#251343,#251344),(#251345,#251346),
(#251347,#251348),(#251349,#251350),(#251351,#251352),(#251353,#251354),
(#251355,#251356),(#251357,#251358),(#251359,#251360),(#251361,#251362),
(#251363,#251364),(#251365,#251366),(#251367,#251368),(#251369,#251370),
(#251371,#251372),(#251373,#251374),(#251375,#251376),(#251377,#251378),
(#251379,#251380),(#251381,#251382),(#251383,#251384),(#251385,#251386),
(#251387,#251388),(#251389,#251390),(#251391,#251392),(#251393,#251394),
(#251395,#251396),(#251397,#251398),(#251399,#251400),(#251401,#251402),
(#251403,#251404),(#251405,#251406),(#251407,#251408),(#251409,#251410),
(#251411,#251412),(#251413,#251414),(#251415,#251416),(#251417,#251418),
(#251419,#251420),(#251421,#251422),(#251423,#251424),(#251425,#251426),
(#251427,#251428),(#251429,#251430),(#251431,#251432),(#251433,#251434),
(#251435,#251436),(#251437,#251438),(#251439,#251440),(#251441,#251442),
(#251443,#251444),(#251445,#251446),(#251447,#251448),(#251449,#251450),
(#251451,#251452),(#251453,#251454),(#251455,#251456),(#251457,#251458),
(#251459,#251460),(#251461,#251462),(#251463,#251464),(#251465,#251466),
(#251467,#251468),(#251469,#251470),(#251471,#251472),(#251473,#251474),
(#251475,#251476),(#251477,#251478),(#251479,#251480),(#251481,#251482),
(#251483,#251484),(#251485,#251486),(#251487,#251488),(#251489,#251490),
(#251491,#251492),(#251493,#251494),(#251495,#251496),(#251497,#251498),
(#251499,#251500),(#251501,#251502),(#251503,#251504),(#251505,#251506),
(#251507,#251508),(#251509,#251510),(#251511,#251512),(#251513,#251514),
(#251515,#251516),(#251517,#251518),(#251519,#251520),(#251521,#251522),
(#251523,#251524),(#251525,#251526),(#251527,#251528),(#251529,#251530),
(#251531,#251532),(#251533,#251534),(#251535,#251536),(#251537,#251538),
(#251539,#251540),(#251541,#251542),(#251543,#251544),(#251545,#251546),
(#251547,#251548),(#251549,#251550),(#251551,#251552),(#251553,#251554),
(#251555,#251556),(#251557,#251558),(#251559,#251560),(#251561,#251562),
(#251563,#251564),(#251565,#251566),(#251567,#251568),(#251569,#251570),
(#251571,#251572),(#251573,#251574),(#251575,#251576),(#251577,#251578),
(#251579,#251580),(#251581,#251582),(#251583,#251584),(#251585,#251586),
(#251587,#251588),(#251589,#251590),(#251591,#251592),(#251593,#251594),
(#251595,#251596),(#251597,#251598),(#251599,#251600),(#251601,#251602),
(#251603,#251604),(#251605,#251606),(#251607,#251608),(#251609,#251610),
(#251611,#251612),(#251613,#251614),(#251615,#251616),(#251617,#251618),
(#251619,#251620),(#251621,#251622),(#251623,#251624),(#251625,#251626),
(#251627,#251628),(#251629,#251630),(#251631,#251632),(#251633,#251634),
(#251635,#251636),(#251637,#251638),(#251639,#251640),(#251641,#251642),
(#251643,#251644),(#251645,#251646),(#251647,#251648),(#251649,#251650),
(#251651,#251652),(#251653,#251654),(#251655,#251656),(#251657,#251658),
(#251659,#251660),(#251661,#251662),(#251663,#251664),(#251665,#251666),
(#251667,#251668),(#251669,#251670),(#251671,#251672),(#251673,#251674),
(#251675,#251676),(#251677,#251678),(#251679,#251680),(#251681,#251682),
(#251683,#251684),(#251685,#251686),(#251687,#251688),(#251689,#251690),
(#251691,#251692),(#251693,#251694),(#251695,#251696),(#251697,#251698),
(#251699,#251700),(#251701,#251702),(#251703,#251704),(#251705,#251706),
(#251707,#251708),(#251709,#251710),(#251711,#251712),(#251713,#251714),
(#251715,#251716),(#251717,#251718),(#251719,#251720),(#251721,#251722),
(#251723,#251724),(#251725,#251726),(#251727,#251728),(#251729,#251730),
(#251731,#251732),(#251733,#251734),(#251735,#251736),(#251737,#251738),
(#251739,#251740),(#251741,#251742),(#251743,#251744),(#251745,#251746),
(#251747,#251748),(#251749,#251750),(#251751,#251752),(#251753,#251754),
(#251755,#251756),(#251757,#251758),(#251759,#251760),(#251761,#251762),
(#251763,#251764),(#251765,#251766),(#251767,#251768),(#251769,#251770),
(#251771,#251772),(#251773,#251774),(#251775,#251776),(#251777,#251778),
(#251779,#251780),(#251781,#251782),(#251783,#251784),(#251785,#251786),
(#251787,#251788),(#251789,#251790),(#251791,#251792),(#251793,#251794),
(#251795,#251796),(#251797,#251798),(#251799,#251800),(#251801,#251802),
(#251803,#251804),(#251805,#251806),(#251807,#251808),(#251809,#251810),
(#251811,#251812),(#251813,#251814),(#251815,#251816),(#251817,#251818),
(#251819,#251820),(#251821,#251822),(#251823,#251824),(#251825,#251826),
(#251827,#251828),(#251829,#251830),(#251831,#251832),(#251833,#251834),
(#251835,#251836),(#251837,#251838),(#251839,#251840),(#251841,#251842),
(#251843,#251844),(#251845,#251846),(#251847,#251848),(#251849,#251850),
(#251851,#251852),(#251853,#251854),(#251855,#251856),(#251857,#251858),
(#251859,#251860),(#251861,#251862),(#251863,#251864),(#251865,#251866),
(#251867,#251868),(#251869,#251870),(#251871,#251872),(#251873,#251874),
(#251875,#251876),(#251877,#251878),(#251879,#251880),(#251881,#251882),
(#251883,#251884),(#251885,#251886),(#251887,#251888),(#251889,#251890),
(#251891,#251892),(#251893,#251894),(#251895,#251896),(#251897,#251898),
(#251899,#251900),(#251901,#251902),(#251903,#251904),(#251905,#251906),
(#251907,#251908),(#251909,#251910),(#251911,#251912),(#251913,#251914),
(#251915,#251916),(#251917,#251918),(#251919,#251920),(#251921,#251922),
(#251923,#251924),(#251925,#251926),(#251927,#251928),(#251929,#251930),
(#251931,#251932),(#251933,#251934),(#251935,#251936),(#251937,#251938),
(#251939,#251940),(#251941,#251942),(#251943,#251944),(#251945,#251946),
(#251947,#251948),(#251949,#251950),(#251951,#251952),(#251953,#251954),
(#251955,#251956),(#251957,#251958),(#251959,#251960),(#251961,#251962),
(#251963,#251964),(#251965,#251966)),.UNSPECIFIED.,.F.,.F.,.F.,(6,1,1,1,
1,1,1,1,1,1,1,1,1,1,1,1,1,1,1,1,1,1,1,1,1,1,1,1,1,1,1,1,1,1,1,1,1,1,1,1,
1,1,1,1,1,1,1,1,1,1,1,1,1,1,1,1,1,1,1,1,1,1,1,1,1,1,1,1,1,1,1,1,1,1,1,1,
1,1,1,1,1,1,1,1,1,1,1,1,1,1,1,1,1,1,1,1,1,1,1,1,1,1,1,1,1,1,1,1,1,1,1,1,
1,1,1,1,1,1,1,1,1,1,1,1,1,1,1,1,1,1,1,1,1,1,1,1,1,1,1,1,1,1,1,1,1,1,1,1,
1,1,1,1,1,1,1,1,1,1,1,1,1,1,1,1,1,1,1,1,1,1,1,1,1,1,1,1,1,1,1,1,1,1,1,1,
1,1,1,1,1,1,1,1,1,1,1,1,1,1,1,1,1,1,1,1,1,1,1,1,1,1,1,1,1,1,1,1,1,1,1,1,
1,1,1,1,1,1,1,1,1,1,1,1,1,1,1,1,1,1,1,1,1,1,1,1,1,1,1,1,1,1,1,1,1,1,1,1,
1,1,1,1,1,1,1,1,1,1,1,1,1,1,1,1,1,1,1,1,1,1,1,1,1,1,1,1,1,1,1,1,1,1,1,1,
1,1,1,1,1,1,1,1,1,1,1,1,1,1,1,1,1,1,1,1,1,1,1,1,1,1,1,1,1,1,1,1,1,1,1,1,
1,1,1,1,1,1,1,1,1,1,1,1,1,1,1,1,1,1,1,1,1,1,1,1,1,1,1,1,1,1,1,1,1,1,1,1,
1,1,1,1,1,1,1,1,1,1,1,1,1,1,1,1,1,1,1,1,1,1,1,1,1,1,1,1,1,1,1,1,1,1,1,1,
1,1,1,1,1,1,1,1,1,1,1,1,1,1,1,1,1,1,1,1,1,1,1,1,1,1,1,1,1,1,1,1,1,1,1,1,
1,1,1,1,1,1,1,1,1,1,1,1,1,1,1,1,1,1,1,1,1,1,1,1,1,1,1,1,1,1,1,6),(2,2),
(0.143172104,0.144954128,0.146788991,0.148623853,0.150458716,0.152293578,
0.15412844,0.155963303,0.157798165,0.159633028,0.16146789,0.163302752,0.165137615,
0.166972477,0.168807339,0.170642202,0.172477064,0.174311927,0.176146789,
0.177981651,0.179816514,0.181651376,0.183486239,0.185321101,0.187155963,
0.188990826,0.190825688,0.19266055,0.194495413,0.196330275,0.198165138,
0.2,0.201834862,0.203669725,0.205504587,0.20733945,0.209174312,0.211009174,
0.212844037,0.214678899,0.216513761,0.218348624,0.220183486,0.222018349,
0.223853211,0.225688073,0.227522936,0.229357798,0.231192661,0.233027523,
0.234862385,0.236697248,0.23853211,0.240366972,0.242201835,0.244036697,
0.24587156,0.247706422,0.249541284,0.251376147,0.253211009,0.255045872,
0.256880734,0.258715596,0.260550459,0.262385321,0.264220183,0.266055046,
0.267889908,0.269724771,0.271559633,0.273394495,0.275229358,0.27706422,
0.278899083,0.280733945,0.282568807,0.28440367,0.286238532,0.288073394,
0.289908257,0.291743119,0.293577982,0.295412844,0.297247706,0.299082569,
0.300917431,0.302752294,0.304587156,0.306422018,0.308256881,0.310091743,
0.311926606,0.313761468,0.31559633,0.317431193,0.319266055,0.321100917,
0.32293578,0.324770642,0.326605505,0.328440367,0.330275229,0.332110092,
0.333944954,0.335779817,0.337614679,0.339449541,0.341284404,0.343119266,
0.344954128,0.346788991,0.348623853,0.350458716,0.352293578,0.35412844,
0.355963303,0.357798165,0.359633028,0.36146789,0.363302752,0.365137615,
0.366972477,0.368807339,0.370642202,0.372477064,0.374311927,0.376146789,
0.377981651,0.379816514,0.381651376,0.383486239,0.385321101,0.387155963,
0.388990826,0.390825688,0.39266055,0.394495413,0.396330275,0.398165138,
0.4,0.401834862,0.403669725,0.405504587,0.40733945,0.409174312,0.411009174,
0.412844037,0.414678899,0.416513761,0.418348624,0.420183486,0.422018349,
0.423853211,0.425688073,0.427522936,0.429357798,0.431192661,0.433027523,
0.434862385,0.436697248,0.43853211,0.440366972,0.442201835,0.444036697,
0.44587156,0.447706422,0.449541284,0.451376147,0.453211009,0.455045872,
0.456880734,0.458715596,0.460550459,0.462385321,0.464220183,0.466055046,
0.467889908,0.469724771,0.471559633,0.473394495,0.475229358,0.47706422,
0.478899083,0.480733945,0.482568807,0.48440367,0.486238532,0.488073394,
0.489908257,0.491743119,0.493577982,0.495412844,0.497247706,0.499082569,
0.500917431,0.502752294,0.504587156,0.506422018,0.508256881,0.510091743,
0.511926606,0.513761468,0.51559633,0.517431193,0.519266055,0.521100917,
0.52293578,0.524770642,0.526605505,0.528440367,0.530275229,0.532110092,
0.533944954,0.535779817,0.537614679,0.539449541,0.541284404,0.543119266,
0.544954128,0.546788991,0.548623853,0.550458716,0.552293578,0.55412844,
0.555963303,0.557798165,0.559633028,0.56146789,0.563302752,0.565137615,
0.566972477,0.568807339,0.570642202,0.572477064,0.574311927,0.576146789,
0.577981651,0.579816514,0.581651376,0.583486239,0.585321101,0.587155963,
0.588990826,0.590825688,0.59266055,0.594495413,0.596330275,0.598165138,
0.6,0.601834862,0.603669725,0.605504587,0.60733945,0.609174312,0.611009174,
0.612844037,0.614678899,0.616513761,0.618348624,0.620183486,0.622018349,
0.623853211,0.625688073,0.627522936,0.629357798,0.631192661,0.633027523,
0.634862385,0.636697248,0.63853211,0.640366972,0.642201835,0.644036697,
0.64587156,0.647706422,0.649541284,0.651376147,0.653211009,0.655045872,
0.656880734,0.658715596,0.660550459,0.662385321,0.664220183,0.666055046,
0.667889908,0.669724771,0.671559633,0.673394495,0.675229358,0.67706422,
0.678899083,0.680733945,0.682568807,0.68440367,0.686238532,0.688073394,
0.689908257,0.691743119,0.693577982,0.695412844,0.697247706,0.699082569,
0.700917431,0.702752294,0.704587156,0.706422018,0.708256881,0.710091743,
0.711926606,0.713761468,0.71559633,0.717431193,0.719266055,0.721100917,
0.72293578,0.724770642,0.726605505,0.728440367,0.730275229,0.732110092,
0.733944954,0.735779817,0.737614679,0.739449541,0.741284404,0.743119266,
0.744954128,0.746788991,0.748623853,0.750458716,0.752293578,0.75412844,
0.755963303,0.757798165,0.759633028,0.76146789,0.763302752,0.765137615,
0.766972477,0.768807339,0.770642202,0.772477064,0.774311927,0.776146789,
0.777981651,0.779816514,0.781651376,0.783486239,0.785321101,0.787155963,
0.788990826,0.790825688,0.79266055,0.794495413,0.796330275,0.798165138,
0.8,0.801834862,0.803669725,0.805504587,0.80733945,0.809174312,0.811009174,
0.812844037,0.814678899,0.816513761,0.818348624,0.820183486,0.822018349,
0.823853211,0.825688073,0.827522936,0.829357798,0.831192661,0.833027523,
0.834862385,0.836697248,0.83853211,0.840366972,0.842201835,0.844036697,
0.84587156,0.847706422,0.849541284,0.851376147,0.853211009,0.855045872,
0.856880734,0.858715596,0.860550459,0.862385321,0.864220183,0.866055046,
0.867889908,0.869724771,0.871559633,0.873394495,0.875229358,0.87706422,
0.878899083,0.880733945,0.882568807,0.88440367,0.886238532,0.888073394,
0.889908257,0.891743119,0.893577982,0.895412844,0.897247706,0.899082569,
0.900917431,0.902752294,0.904587156,0.906422018,0.908256881,0.910091743,
0.911926606,0.913761468,0.91559633,0.917431193,0.919266055,0.921100917,
0.92293578,0.924770642,0.926605505,0.928440367,0.930275229,0.932110092,
0.933944954,0.935779817,0.937614679,0.939449541,0.941284404,0.943119266,
0.944954128,0.946788991,0.948623853,0.950458716,0.952293578,0.95412844,
0.955963303,0.957798165,0.959633028,0.96146789,0.963302752,0.965137615,
0.966972477,0.968807339,0.970642202,0.972477064,0.974311927,0.976146789,
0.977981651,0.979816514,0.981651376,0.983486239,0.985321101,0.987155963,
0.988990826,0.990825688,0.99266055,0.994495413,0.996330275,0.998165138,
1.),(0.,0.36),.UNSPECIFIED.);
#6275=B_SPLINE_SURFACE_WITH_KNOTS('',5,1,((#252611,#252612),(#252613,#252614),
(#252615,#252616),(#252617,#252618),(#252619,#252620),(#252621,#252622),
(#252623,#252624),(#252625,#252626),(#252627,#252628),(#252629,#252630),
(#252631,#252632),(#252633,#252634),(#252635,#252636),(#252637,#252638),
(#252639,#252640),(#252641,#252642),(#252643,#252644),(#252645,#252646),
(#252647,#252648),(#252649,#252650),(#252651,#252652),(#252653,#252654),
(#252655,#252656),(#252657,#252658),(#252659,#252660),(#252661,#252662),
(#252663,#252664),(#252665,#252666),(#252667,#252668),(#252669,#252670),
(#252671,#252672),(#252673,#252674),(#252675,#252676),(#252677,#252678),
(#252679,#252680),(#252681,#252682),(#252683,#252684),(#252685,#252686),
(#252687,#252688),(#252689,#252690),(#252691,#252692),(#252693,#252694),
(#252695,#252696),(#252697,#252698),(#252699,#252700),(#252701,#252702),
(#252703,#252704),(#252705,#252706),(#252707,#252708),(#252709,#252710),
(#252711,#252712),(#252713,#252714),(#252715,#252716),(#252717,#252718),
(#252719,#252720),(#252721,#252722),(#252723,#252724),(#252725,#252726),
(#252727,#252728),(#252729,#252730),(#252731,#252732),(#252733,#252734),
(#252735,#252736),(#252737,#252738),(#252739,#252740),(#252741,#252742),
(#252743,#252744),(#252745,#252746),(#252747,#252748),(#252749,#252750),
(#252751,#252752),(#252753,#252754),(#252755,#252756),(#252757,#252758),
(#252759,#252760),(#252761,#252762),(#252763,#252764),(#252765,#252766),
(#252767,#252768),(#252769,#252770),(#252771,#252772),(#252773,#252774),
(#252775,#252776),(#252777,#252778),(#252779,#252780),(#252781,#252782),
(#252783,#252784),(#252785,#252786),(#252787,#252788),(#252789,#252790),
(#252791,#252792),(#252793,#252794),(#252795,#252796),(#252797,#252798),
(#252799,#252800),(#252801,#252802),(#252803,#252804),(#252805,#252806),
(#252807,#252808),(#252809,#252810),(#252811,#252812),(#252813,#252814),
(#252815,#252816),(#252817,#252818),(#252819,#252820),(#252821,#252822),
(#252823,#252824),(#252825,#252826),(#252827,#252828),(#252829,#252830),
(#252831,#252832),(#252833,#252834),(#252835,#252836),(#252837,#252838),
(#252839,#252840),(#252841,#252842),(#252843,#252844),(#252845,#252846),
(#252847,#252848),(#252849,#252850),(#252851,#252852),(#252853,#252854),
(#252855,#252856),(#252857,#252858),(#252859,#252860),(#252861,#252862),
(#252863,#252864),(#252865,#252866),(#252867,#252868),(#252869,#252870),
(#252871,#252872),(#252873,#252874),(#252875,#252876),(#252877,#252878),
(#252879,#252880),(#252881,#252882),(#252883,#252884),(#252885,#252886),
(#252887,#252888),(#252889,#252890),(#252891,#252892),(#252893,#252894),
(#252895,#252896),(#252897,#252898),(#252899,#252900),(#252901,#252902),
(#252903,#252904),(#252905,#252906),(#252907,#252908),(#252909,#252910),
(#252911,#252912),(#252913,#252914),(#252915,#252916),(#252917,#252918),
(#252919,#252920),(#252921,#252922),(#252923,#252924),(#252925,#252926),
(#252927,#252928),(#252929,#252930),(#252931,#252932),(#252933,#252934),
(#252935,#252936),(#252937,#252938),(#252939,#252940),(#252941,#252942),
(#252943,#252944),(#252945,#252946),(#252947,#252948),(#252949,#252950),
(#252951,#252952),(#252953,#252954),(#252955,#252956),(#252957,#252958),
(#252959,#252960),(#252961,#252962),(#252963,#252964),(#252965,#252966),
(#252967,#252968),(#252969,#252970),(#252971,#252972),(#252973,#252974),
(#252975,#252976),(#252977,#252978),(#252979,#252980),(#252981,#252982),
(#252983,#252984),(#252985,#252986),(#252987,#252988),(#252989,#252990),
(#252991,#252992),(#252993,#252994),(#252995,#252996),(#252997,#252998),
(#252999,#253000),(#253001,#253002),(#253003,#253004),(#253005,#253006),
(#253007,#253008),(#253009,#253010),(#253011,#253012),(#253013,#253014),
(#253015,#253016),(#253017,#253018),(#253019,#253020),(#253021,#253022),
(#253023,#253024),(#253025,#253026),(#253027,#253028),(#253029,#253030),
(#253031,#253032),(#253033,#253034),(#253035,#253036),(#253037,#253038),
(#253039,#253040),(#253041,#253042),(#253043,#253044),(#253045,#253046),
(#253047,#253048),(#253049,#253050),(#253051,#253052),(#253053,#253054),
(#253055,#253056),(#253057,#253058),(#253059,#253060),(#253061,#253062),
(#253063,#253064),(#253065,#253066),(#253067,#253068),(#253069,#253070),
(#253071,#253072),(#253073,#253074),(#253075,#253076),(#253077,#253078),
(#253079,#253080),(#253081,#253082),(#253083,#253084),(#253085,#253086),
(#253087,#253088),(#253089,#253090),(#253091,#253092),(#253093,#253094),
(#253095,#253096),(#253097,#253098),(#253099,#253100),(#253101,#253102),
(#253103,#253104),(#253105,#253106),(#253107,#253108),(#253109,#253110),
(#253111,#253112),(#253113,#253114),(#253115,#253116),(#253117,#253118),
(#253119,#253120),(#253121,#253122),(#253123,#253124),(#253125,#253126),
(#253127,#253128),(#253129,#253130),(#253131,#253132),(#253133,#253134),
(#253135,#253136),(#253137,#253138),(#253139,#253140),(#253141,#253142),
(#253143,#253144),(#253145,#253146),(#253147,#253148),(#253149,#253150),
(#253151,#253152),(#253153,#253154),(#253155,#253156),(#253157,#253158),
(#253159,#253160),(#253161,#253162),(#253163,#253164),(#253165,#253166),
(#253167,#253168),(#253169,#253170),(#253171,#253172),(#253173,#253174),
(#253175,#253176),(#253177,#253178),(#253179,#253180),(#253181,#253182),
(#253183,#253184),(#253185,#253186),(#253187,#253188),(#253189,#253190),
(#253191,#253192),(#253193,#253194),(#253195,#253196),(#253197,#253198),
(#253199,#253200),(#253201,#253202),(#253203,#253204),(#253205,#253206),
(#253207,#253208),(#253209,#253210),(#253211,#253212),(#253213,#253214),
(#253215,#253216),(#253217,#253218),(#253219,#253220),(#253221,#253222),
(#253223,#253224),(#253225,#253226),(#253227,#253228),(#253229,#253230),
(#253231,#253232),(#253233,#253234),(#253235,#253236),(#253237,#253238),
(#253239,#253240),(#253241,#253242),(#253243,#253244),(#253245,#253246),
(#253247,#253248),(#253249,#253250),(#253251,#253252),(#253253,#253254),
(#253255,#253256),(#253257,#253258),(#253259,#253260),(#253261,#253262),
(#253263,#253264),(#253265,#253266),(#253267,#253268),(#253269,#253270),
(#253271,#253272),(#253273,#253274),(#253275,#253276),(#253277,#253278),
(#253279,#253280),(#253281,#253282),(#253283,#253284),(#253285,#253286),
(#253287,#253288),(#253289,#253290),(#253291,#253292),(#253293,#253294),
(#253295,#253296),(#253297,#253298),(#253299,#253300),(#253301,#253302),
(#253303,#253304),(#253305,#253306),(#253307,#253308),(#253309,#253310),
(#253311,#253312),(#253313,#253314),(#253315,#253316),(#253317,#253318),
(#253319,#253320),(#253321,#253322),(#253323,#253324),(#253325,#253326),
(#253327,#253328),(#253329,#253330),(#253331,#253332),(#253333,#253334),
(#253335,#253336),(#253337,#253338),(#253339,#253340),(#253341,#253342),
(#253343,#253344),(#253345,#253346),(#253347,#253348),(#253349,#253350),
(#253351,#253352),(#253353,#253354),(#253355,#253356),(#253357,#253358),
(#253359,#253360),(#253361,#253362),(#253363,#253364),(#253365,#253366),
(#253367,#253368),(#253369,#253370),(#253371,#253372),(#253373,#253374),
(#253375,#253376),(#253377,#253378),(#253379,#253380),(#253381,#253382),
(#253383,#253384),(#253385,#253386),(#253387,#253388),(#253389,#253390),
(#253391,#253392),(#253393,#253394),(#253395,#253396),(#253397,#253398),
(#253399,#253400),(#253401,#253402),(#253403,#253404),(#253405,#253406),
(#253407,#253408),(#253409,#253410),(#253411,#253412),(#253413,#253414),
(#253415,#253416),(#253417,#253418),(#253419,#253420),(#253421,#253422),
(#253423,#253424),(#253425,#253426),(#253427,#253428),(#253429,#253430),
(#253431,#253432),(#253433,#253434),(#253435,#253436),(#253437,#253438),
(#253439,#253440),(#253441,#253442),(#253443,#253444),(#253445,#253446),
(#253447,#253448),(#253449,#253450),(#253451,#253452),(#253453,#253454),
(#253455,#253456),(#253457,#253458),(#253459,#253460),(#253461,#253462),
(#253463,#253464),(#253465,#253466),(#253467,#253468),(#253469,#253470),
(#253471,#253472),(#253473,#253474),(#253475,#253476),(#253477,#253478),
(#253479,#253480),(#253481,#253482),(#253483,#253484),(#253485,#253486),
(#253487,#253488),(#253489,#253490),(#253491,#253492),(#253493,#253494),
(#253495,#253496),(#253497,#253498),(#253499,#253500),(#253501,#253502),
(#253503,#253504),(#253505,#253506),(#253507,#253508),(#253509,#253510),
(#253511,#253512),(#253513,#253514),(#253515,#253516),(#253517,#253518),
(#253519,#253520),(#253521,#253522),(#253523,#253524),(#253525,#253526),
(#253527,#253528),(#253529,#253530),(#253531,#253532),(#253533,#253534),
(#253535,#253536),(#253537,#253538),(#253539,#253540),(#253541,#253542),
(#253543,#253544),(#253545,#253546),(#253547,#253548),(#253549,#253550),
(#253551,#253552),(#253553,#253554)),.UNSPECIFIED.,.F.,.F.,.F.,(6,1,1,1,
1,1,1,1,1,1,1,1,1,1,1,1,1,1,1,1,1,1,1,1,1,1,1,1,1,1,1,1,1,1,1,1,1,1,1,1,
1,1,1,1,1,1,1,1,1,1,1,1,1,1,1,1,1,1,1,1,1,1,1,1,1,1,1,1,1,1,1,1,1,1,1,1,
1,1,1,1,1,1,1,1,1,1,1,1,1,1,1,1,1,1,1,1,1,1,1,1,1,1,1,1,1,1,1,1,1,1,1,1,
1,1,1,1,1,1,1,1,1,1,1,1,1,1,1,1,1,1,1,1,1,1,1,1,1,1,1,1,1,1,1,1,1,1,1,1,
1,1,1,1,1,1,1,1,1,1,1,1,1,1,1,1,1,1,1,1,1,1,1,1,1,1,1,1,1,1,1,1,1,1,1,1,
1,1,1,1,1,1,1,1,1,1,1,1,1,1,1,1,1,1,1,1,1,1,1,1,1,1,1,1,1,1,1,1,1,1,1,1,
1,1,1,1,1,1,1,1,1,1,1,1,1,1,1,1,1,1,1,1,1,1,1,1,1,1,1,1,1,1,1,1,1,1,1,1,
1,1,1,1,1,1,1,1,1,1,1,1,1,1,1,1,1,1,1,1,1,1,1,1,1,1,1,1,1,1,1,1,1,1,1,1,
1,1,1,1,1,1,1,1,1,1,1,1,1,1,1,1,1,1,1,1,1,1,1,1,1,1,1,1,1,1,1,1,1,1,1,1,
1,1,1,1,1,1,1,1,1,1,1,1,1,1,1,1,1,1,1,1,1,1,1,1,1,1,1,1,1,1,1,1,1,1,1,1,
1,1,1,1,1,1,1,1,1,1,1,1,1,1,1,1,1,1,1,1,1,1,1,1,1,1,1,1,1,1,1,1,1,1,1,1,
1,1,1,1,1,1,1,1,1,1,1,1,1,1,1,1,1,1,1,1,1,1,1,1,1,1,1,1,1,1,1,1,1,1,1,1,
1,1,1,1,1,1,1,1,1,1,1,1,1,1,1,1,1,1,1,1,1,1,1,1,1,1,1,1,1,1,1,6),(2,2),
(0.143172103,0.144954128,0.146788991,0.148623853,0.150458716,0.152293578,
0.15412844,0.155963303,0.157798165,0.159633028,0.16146789,0.163302752,0.165137615,
0.166972477,0.168807339,0.170642202,0.172477064,0.174311927,0.176146789,
0.177981651,0.179816514,0.181651376,0.183486239,0.185321101,0.187155963,
0.188990826,0.190825688,0.19266055,0.194495413,0.196330275,0.198165138,
0.2,0.201834862,0.203669725,0.205504587,0.20733945,0.209174312,0.211009174,
0.212844037,0.214678899,0.216513761,0.218348624,0.220183486,0.222018349,
0.223853211,0.225688073,0.227522936,0.229357798,0.231192661,0.233027523,
0.234862385,0.236697248,0.23853211,0.240366972,0.242201835,0.244036697,
0.24587156,0.247706422,0.249541284,0.251376147,0.253211009,0.255045872,
0.256880734,0.258715596,0.260550459,0.262385321,0.264220183,0.266055046,
0.267889908,0.269724771,0.271559633,0.273394495,0.275229358,0.27706422,
0.278899083,0.280733945,0.282568807,0.28440367,0.286238532,0.288073394,
0.289908257,0.291743119,0.293577982,0.295412844,0.297247706,0.299082569,
0.300917431,0.302752294,0.304587156,0.306422018,0.308256881,0.310091743,
0.311926606,0.313761468,0.31559633,0.317431193,0.319266055,0.321100917,
0.32293578,0.324770642,0.326605505,0.328440367,0.330275229,0.332110092,
0.333944954,0.335779817,0.337614679,0.339449541,0.341284404,0.343119266,
0.344954128,0.346788991,0.348623853,0.350458716,0.352293578,0.35412844,
0.355963303,0.357798165,0.359633028,0.36146789,0.363302752,0.365137615,
0.366972477,0.368807339,0.370642202,0.372477064,0.374311927,0.376146789,
0.377981651,0.379816514,0.381651376,0.383486239,0.385321101,0.387155963,
0.388990826,0.390825688,0.39266055,0.394495413,0.396330275,0.398165138,
0.4,0.401834862,0.403669725,0.405504587,0.40733945,0.409174312,0.411009174,
0.412844037,0.414678899,0.416513761,0.418348624,0.420183486,0.422018349,
0.423853211,0.425688073,0.427522936,0.429357798,0.431192661,0.433027523,
0.434862385,0.436697248,0.43853211,0.440366972,0.442201835,0.444036697,
0.44587156,0.447706422,0.449541284,0.451376147,0.453211009,0.455045872,
0.456880734,0.458715596,0.460550459,0.462385321,0.464220183,0.466055046,
0.467889908,0.469724771,0.471559633,0.473394495,0.475229358,0.47706422,
0.478899083,0.480733945,0.482568807,0.48440367,0.486238532,0.488073394,
0.489908257,0.491743119,0.493577982,0.495412844,0.497247706,0.499082569,
0.500917431,0.502752294,0.504587156,0.506422018,0.508256881,0.510091743,
0.511926606,0.513761468,0.51559633,0.517431193,0.519266055,0.521100917,
0.52293578,0.524770642,0.526605505,0.528440367,0.530275229,0.532110092,
0.533944954,0.535779817,0.537614679,0.539449541,0.541284404,0.543119266,
0.544954128,0.546788991,0.548623853,0.550458716,0.552293578,0.55412844,
0.555963303,0.557798165,0.559633028,0.56146789,0.563302752,0.565137615,
0.566972477,0.568807339,0.570642202,0.572477064,0.574311927,0.576146789,
0.577981651,0.579816514,0.581651376,0.583486239,0.585321101,0.587155963,
0.588990826,0.590825688,0.59266055,0.594495413,0.596330275,0.598165138,
0.6,0.601834862,0.603669725,0.605504587,0.60733945,0.609174312,0.611009174,
0.612844037,0.614678899,0.616513761,0.618348624,0.620183486,0.622018349,
0.623853211,0.625688073,0.627522936,0.629357798,0.631192661,0.633027523,
0.634862385,0.636697248,0.63853211,0.640366972,0.642201835,0.644036697,
0.64587156,0.647706422,0.649541284,0.651376147,0.653211009,0.655045872,
0.656880734,0.658715596,0.660550459,0.662385321,0.664220183,0.666055046,
0.667889908,0.669724771,0.671559633,0.673394495,0.675229358,0.67706422,
0.678899083,0.680733945,0.682568807,0.68440367,0.686238532,0.688073394,
0.689908257,0.691743119,0.693577982,0.695412844,0.697247706,0.699082569,
0.700917431,0.702752294,0.704587156,0.706422018,0.708256881,0.710091743,
0.711926606,0.713761468,0.71559633,0.717431193,0.719266055,0.721100917,
0.72293578,0.724770642,0.726605505,0.728440367,0.730275229,0.732110092,
0.733944954,0.735779817,0.737614679,0.739449541,0.741284404,0.743119266,
0.744954128,0.746788991,0.748623853,0.750458716,0.752293578,0.75412844,
0.755963303,0.757798165,0.759633028,0.76146789,0.763302752,0.765137615,
0.766972477,0.768807339,0.770642202,0.772477064,0.774311927,0.776146789,
0.777981651,0.779816514,0.781651376,0.783486239,0.785321101,0.787155963,
0.788990826,0.790825688,0.79266055,0.794495413,0.796330275,0.798165138,
0.8,0.801834862,0.803669725,0.805504587,0.80733945,0.809174312,0.811009174,
0.812844037,0.814678899,0.816513761,0.818348624,0.820183486,0.822018349,
0.823853211,0.825688073,0.827522936,0.829357798,0.831192661,0.833027523,
0.834862385,0.836697248,0.83853211,0.840366972,0.842201835,0.844036697,
0.84587156,0.847706422,0.849541284,0.851376147,0.853211009,0.855045872,
0.856880734,0.858715596,0.860550459,0.862385321,0.864220183,0.866055046,
0.867889908,0.869724771,0.871559633,0.873394495,0.875229358,0.87706422,
0.878899083,0.880733945,0.882568807,0.88440367,0.886238532,0.888073394,
0.889908257,0.891743119,0.893577982,0.895412844,0.897247706,0.899082569,
0.900917431,0.902752294,0.904587156,0.906422018,0.908256881,0.910091743,
0.911926606,0.913761468,0.91559633,0.917431193,0.919266055,0.921100917,
0.92293578,0.924770642,0.926605505,0.928440367,0.930275229,0.932110092,
0.933944954,0.935779817,0.937614679,0.939449541,0.941284404,0.943119266,
0.944954128,0.946788991,0.948623853,0.950458716,0.952293578,0.95412844,
0.955963303,0.957798165,0.959633028,0.96146789,0.963302752,0.965137615,
0.966972477,0.968807339,0.970642202,0.972477064,0.974311927,0.976146789,
0.977981651,0.979816514,0.981651376,0.983486239,0.985321101,0.987155963,
0.988990826,0.990825688,0.99266055,0.994495413,0.996330275,0.998165138,
1.),(0.,0.36),.UNSPECIFIED.);
#6276=B_SPLINE_SURFACE_WITH_KNOTS('',5,1,((#254166,#254167),(#254168,#254169),
(#254170,#254171),(#254172,#254173),(#254174,#254175),(#254176,#254177),
(#254178,#254179),(#254180,#254181),(#254182,#254183),(#254184,#254185),
(#254186,#254187),(#254188,#254189),(#254190,#254191),(#254192,#254193),
(#254194,#254195),(#254196,#254197),(#254198,#254199),(#254200,#254201),
(#254202,#254203),(#254204,#254205),(#254206,#254207),(#254208,#254209),
(#254210,#254211),(#254212,#254213),(#254214,#254215),(#254216,#254217),
(#254218,#254219),(#254220,#254221),(#254222,#254223),(#254224,#254225),
(#254226,#254227),(#254228,#254229),(#254230,#254231),(#254232,#254233),
(#254234,#254235),(#254236,#254237),(#254238,#254239),(#254240,#254241),
(#254242,#254243),(#254244,#254245),(#254246,#254247),(#254248,#254249),
(#254250,#254251),(#254252,#254253),(#254254,#254255),(#254256,#254257),
(#254258,#254259),(#254260,#254261),(#254262,#254263),(#254264,#254265),
(#254266,#254267),(#254268,#254269),(#254270,#254271),(#254272,#254273),
(#254274,#254275),(#254276,#254277),(#254278,#254279),(#254280,#254281),
(#254282,#254283),(#254284,#254285),(#254286,#254287),(#254288,#254289),
(#254290,#254291),(#254292,#254293),(#254294,#254295),(#254296,#254297),
(#254298,#254299),(#254300,#254301),(#254302,#254303),(#254304,#254305),
(#254306,#254307),(#254308,#254309),(#254310,#254311),(#254312,#254313),
(#254314,#254315),(#254316,#254317),(#254318,#254319),(#254320,#254321),
(#254322,#254323),(#254324,#254325),(#254326,#254327),(#254328,#254329),
(#254330,#254331),(#254332,#254333),(#254334,#254335),(#254336,#254337),
(#254338,#254339),(#254340,#254341),(#254342,#254343),(#254344,#254345),
(#254346,#254347),(#254348,#254349),(#254350,#254351),(#254352,#254353),
(#254354,#254355),(#254356,#254357),(#254358,#254359),(#254360,#254361),
(#254362,#254363),(#254364,#254365),(#254366,#254367),(#254368,#254369),
(#254370,#254371),(#254372,#254373),(#254374,#254375),(#254376,#254377),
(#254378,#254379),(#254380,#254381),(#254382,#254383),(#254384,#254385),
(#254386,#254387),(#254388,#254389),(#254390,#254391),(#254392,#254393),
(#254394,#254395),(#254396,#254397),(#254398,#254399),(#254400,#254401),
(#254402,#254403),(#254404,#254405),(#254406,#254407),(#254408,#254409),
(#254410,#254411),(#254412,#254413),(#254414,#254415),(#254416,#254417),
(#254418,#254419),(#254420,#254421),(#254422,#254423),(#254424,#254425),
(#254426,#254427),(#254428,#254429),(#254430,#254431),(#254432,#254433),
(#254434,#254435),(#254436,#254437),(#254438,#254439),(#254440,#254441),
(#254442,#254443),(#254444,#254445),(#254446,#254447),(#254448,#254449),
(#254450,#254451),(#254452,#254453),(#254454,#254455),(#254456,#254457),
(#254458,#254459),(#254460,#254461),(#254462,#254463),(#254464,#254465),
(#254466,#254467),(#254468,#254469),(#254470,#254471),(#254472,#254473),
(#254474,#254475),(#254476,#254477),(#254478,#254479),(#254480,#254481),
(#254482,#254483),(#254484,#254485),(#254486,#254487),(#254488,#254489),
(#254490,#254491),(#254492,#254493),(#254494,#254495),(#254496,#254497),
(#254498,#254499),(#254500,#254501),(#254502,#254503),(#254504,#254505),
(#254506,#254507),(#254508,#254509),(#254510,#254511),(#254512,#254513),
(#254514,#254515),(#254516,#254517),(#254518,#254519),(#254520,#254521),
(#254522,#254523),(#254524,#254525),(#254526,#254527),(#254528,#254529),
(#254530,#254531),(#254532,#254533),(#254534,#254535),(#254536,#254537),
(#254538,#254539),(#254540,#254541),(#254542,#254543),(#254544,#254545),
(#254546,#254547),(#254548,#254549),(#254550,#254551),(#254552,#254553),
(#254554,#254555),(#254556,#254557),(#254558,#254559),(#254560,#254561),
(#254562,#254563),(#254564,#254565),(#254566,#254567),(#254568,#254569),
(#254570,#254571),(#254572,#254573),(#254574,#254575),(#254576,#254577),
(#254578,#254579),(#254580,#254581),(#254582,#254583),(#254584,#254585),
(#254586,#254587),(#254588,#254589),(#254590,#254591),(#254592,#254593),
(#254594,#254595),(#254596,#254597),(#254598,#254599),(#254600,#254601),
(#254602,#254603),(#254604,#254605),(#254606,#254607),(#254608,#254609),
(#254610,#254611),(#254612,#254613),(#254614,#254615),(#254616,#254617),
(#254618,#254619),(#254620,#254621),(#254622,#254623),(#254624,#254625),
(#254626,#254627),(#254628,#254629),(#254630,#254631),(#254632,#254633),
(#254634,#254635),(#254636,#254637),(#254638,#254639),(#254640,#254641),
(#254642,#254643),(#254644,#254645),(#254646,#254647),(#254648,#254649),
(#254650,#254651),(#254652,#254653),(#254654,#254655),(#254656,#254657),
(#254658,#254659),(#254660,#254661),(#254662,#254663),(#254664,#254665),
(#254666,#254667),(#254668,#254669),(#254670,#254671),(#254672,#254673),
(#254674,#254675),(#254676,#254677),(#254678,#254679),(#254680,#254681),
(#254682,#254683),(#254684,#254685),(#254686,#254687),(#254688,#254689),
(#254690,#254691),(#254692,#254693),(#254694,#254695),(#254696,#254697),
(#254698,#254699),(#254700,#254701),(#254702,#254703),(#254704,#254705),
(#254706,#254707),(#254708,#254709),(#254710,#254711),(#254712,#254713),
(#254714,#254715),(#254716,#254717),(#254718,#254719),(#254720,#254721),
(#254722,#254723),(#254724,#254725),(#254726,#254727),(#254728,#254729),
(#254730,#254731),(#254732,#254733),(#254734,#254735),(#254736,#254737),
(#254738,#254739),(#254740,#254741),(#254742,#254743),(#254744,#254745),
(#254746,#254747),(#254748,#254749),(#254750,#254751),(#254752,#254753),
(#254754,#254755),(#254756,#254757),(#254758,#254759),(#254760,#254761),
(#254762,#254763),(#254764,#254765),(#254766,#254767),(#254768,#254769),
(#254770,#254771),(#254772,#254773),(#254774,#254775),(#254776,#254777),
(#254778,#254779),(#254780,#254781),(#254782,#254783),(#254784,#254785),
(#254786,#254787),(#254788,#254789),(#254790,#254791),(#254792,#254793),
(#254794,#254795),(#254796,#254797),(#254798,#254799),(#254800,#254801),
(#254802,#254803),(#254804,#254805),(#254806,#254807),(#254808,#254809),
(#254810,#254811),(#254812,#254813),(#254814,#254815),(#254816,#254817),
(#254818,#254819),(#254820,#254821),(#254822,#254823),(#254824,#254825),
(#254826,#254827),(#254828,#254829),(#254830,#254831),(#254832,#254833),
(#254834,#254835),(#254836,#254837),(#254838,#254839),(#254840,#254841),
(#254842,#254843),(#254844,#254845),(#254846,#254847),(#254848,#254849),
(#254850,#254851),(#254852,#254853),(#254854,#254855),(#254856,#254857),
(#254858,#254859),(#254860,#254861),(#254862,#254863),(#254864,#254865),
(#254866,#254867),(#254868,#254869),(#254870,#254871),(#254872,#254873),
(#254874,#254875),(#254876,#254877),(#254878,#254879),(#254880,#254881),
(#254882,#254883),(#254884,#254885),(#254886,#254887),(#254888,#254889),
(#254890,#254891),(#254892,#254893),(#254894,#254895),(#254896,#254897),
(#254898,#254899),(#254900,#254901),(#254902,#254903),(#254904,#254905),
(#254906,#254907),(#254908,#254909),(#254910,#254911),(#254912,#254913),
(#254914,#254915),(#254916,#254917),(#254918,#254919),(#254920,#254921),
(#254922,#254923),(#254924,#254925),(#254926,#254927),(#254928,#254929),
(#254930,#254931),(#254932,#254933),(#254934,#254935),(#254936,#254937),
(#254938,#254939),(#254940,#254941),(#254942,#254943),(#254944,#254945),
(#254946,#254947),(#254948,#254949),(#254950,#254951),(#254952,#254953),
(#254954,#254955),(#254956,#254957),(#254958,#254959),(#254960,#254961),
(#254962,#254963),(#254964,#254965),(#254966,#254967),(#254968,#254969),
(#254970,#254971),(#254972,#254973),(#254974,#254975),(#254976,#254977),
(#254978,#254979),(#254980,#254981),(#254982,#254983),(#254984,#254985),
(#254986,#254987),(#254988,#254989),(#254990,#254991),(#254992,#254993),
(#254994,#254995),(#254996,#254997),(#254998,#254999),(#255000,#255001),
(#255002,#255003),(#255004,#255005),(#255006,#255007),(#255008,#255009),
(#255010,#255011),(#255012,#255013),(#255014,#255015),(#255016,#255017),
(#255018,#255019),(#255020,#255021),(#255022,#255023),(#255024,#255025),
(#255026,#255027),(#255028,#255029),(#255030,#255031),(#255032,#255033),
(#255034,#255035),(#255036,#255037),(#255038,#255039),(#255040,#255041),
(#255042,#255043),(#255044,#255045),(#255046,#255047),(#255048,#255049),
(#255050,#255051),(#255052,#255053),(#255054,#255055),(#255056,#255057),
(#255058,#255059),(#255060,#255061),(#255062,#255063),(#255064,#255065),
(#255066,#255067),(#255068,#255069),(#255070,#255071),(#255072,#255073),
(#255074,#255075),(#255076,#255077),(#255078,#255079),(#255080,#255081),
(#255082,#255083),(#255084,#255085),(#255086,#255087),(#255088,#255089),
(#255090,#255091),(#255092,#255093),(#255094,#255095),(#255096,#255097),
(#255098,#255099),(#255100,#255101),(#255102,#255103),(#255104,#255105),
(#255106,#255107),(#255108,#255109)),.UNSPECIFIED.,.F.,.F.,.F.,(6,1,1,1,
1,1,1,1,1,1,1,1,1,1,1,1,1,1,1,1,1,1,1,1,1,1,1,1,1,1,1,1,1,1,1,1,1,1,1,1,
1,1,1,1,1,1,1,1,1,1,1,1,1,1,1,1,1,1,1,1,1,1,1,1,1,1,1,1,1,1,1,1,1,1,1,1,
1,1,1,1,1,1,1,1,1,1,1,1,1,1,1,1,1,1,1,1,1,1,1,1,1,1,1,1,1,1,1,1,1,1,1,1,
1,1,1,1,1,1,1,1,1,1,1,1,1,1,1,1,1,1,1,1,1,1,1,1,1,1,1,1,1,1,1,1,1,1,1,1,
1,1,1,1,1,1,1,1,1,1,1,1,1,1,1,1,1,1,1,1,1,1,1,1,1,1,1,1,1,1,1,1,1,1,1,1,
1,1,1,1,1,1,1,1,1,1,1,1,1,1,1,1,1,1,1,1,1,1,1,1,1,1,1,1,1,1,1,1,1,1,1,1,
1,1,1,1,1,1,1,1,1,1,1,1,1,1,1,1,1,1,1,1,1,1,1,1,1,1,1,1,1,1,1,1,1,1,1,1,
1,1,1,1,1,1,1,1,1,1,1,1,1,1,1,1,1,1,1,1,1,1,1,1,1,1,1,1,1,1,1,1,1,1,1,1,
1,1,1,1,1,1,1,1,1,1,1,1,1,1,1,1,1,1,1,1,1,1,1,1,1,1,1,1,1,1,1,1,1,1,1,1,
1,1,1,1,1,1,1,1,1,1,1,1,1,1,1,1,1,1,1,1,1,1,1,1,1,1,1,1,1,1,1,1,1,1,1,1,
1,1,1,1,1,1,1,1,1,1,1,1,1,1,1,1,1,1,1,1,1,1,1,1,1,1,1,1,1,1,1,1,1,1,1,1,
1,1,1,1,1,1,1,1,1,1,1,1,1,1,1,1,1,1,1,1,1,1,1,1,1,1,1,1,1,1,1,1,1,1,1,1,
1,1,1,1,1,1,1,1,1,1,1,1,1,1,1,1,1,1,1,1,1,1,1,1,1,1,1,1,1,1,1,6),(2,2),
(-1.,-0.998165138,-0.996330275,-0.994495413,-0.99266055,-0.990825688,-0.988990826,
-0.987155963,-0.985321101,-0.983486239,-0.981651376,-0.979816514,-0.977981651,
-0.976146789,-0.974311927,-0.972477064,-0.970642202,-0.968807339,-0.966972477,
-0.965137615,-0.963302752,-0.96146789,-0.959633028,-0.957798165,-0.955963303,
-0.95412844,-0.952293578,-0.950458716,-0.948623853,-0.946788991,-0.944954128,
-0.943119266,-0.941284404,-0.939449541,-0.937614679,-0.935779817,-0.933944954,
-0.932110092,-0.930275229,-0.928440367,-0.926605505,-0.924770642,-0.92293578,
-0.921100917,-0.919266055,-0.917431193,-0.91559633,-0.913761468,-0.911926606,
-0.910091743,-0.908256881,-0.906422018,-0.904587156,-0.902752294,-0.900917431,
-0.899082569,-0.897247706,-0.895412844,-0.893577982,-0.891743119,-0.889908257,
-0.888073394,-0.886238532,-0.88440367,-0.882568807,-0.880733945,-0.878899083,
-0.87706422,-0.875229358,-0.873394495,-0.871559633,-0.869724771,-0.867889908,
-0.866055046,-0.864220183,-0.862385321,-0.860550459,-0.858715596,-0.856880734,
-0.855045872,-0.853211009,-0.851376147,-0.849541284,-0.847706422,-0.84587156,
-0.844036697,-0.842201835,-0.840366972,-0.83853211,-0.836697248,-0.834862385,
-0.833027523,-0.831192661,-0.829357798,-0.827522936,-0.825688073,-0.823853211,
-0.822018349,-0.820183486,-0.818348624,-0.816513761,-0.814678899,-0.812844037,
-0.811009174,-0.809174312,-0.80733945,-0.805504587,-0.803669725,-0.801834862,
-0.8,-0.798165138,-0.796330275,-0.794495413,-0.79266055,-0.790825688,-0.788990826,
-0.787155963,-0.785321101,-0.783486239,-0.781651376,-0.779816514,-0.777981651,
-0.776146789,-0.774311927,-0.772477064,-0.770642202,-0.768807339,-0.766972477,
-0.765137615,-0.763302752,-0.76146789,-0.759633028,-0.757798165,-0.755963303,
-0.75412844,-0.752293578,-0.750458716,-0.748623853,-0.746788991,-0.744954128,
-0.743119266,-0.741284404,-0.739449541,-0.737614679,-0.735779817,-0.733944954,
-0.732110092,-0.730275229,-0.728440367,-0.726605505,-0.724770642,-0.72293578,
-0.721100917,-0.719266055,-0.717431193,-0.71559633,-0.713761468,-0.711926606,
-0.710091743,-0.708256881,-0.706422018,-0.704587156,-0.702752294,-0.700917431,
-0.699082569,-0.697247706,-0.695412844,-0.693577982,-0.691743119,-0.689908257,
-0.688073394,-0.686238532,-0.68440367,-0.682568807,-0.680733945,-0.678899083,
-0.67706422,-0.675229358,-0.673394495,-0.671559633,-0.669724771,-0.667889908,
-0.666055046,-0.664220183,-0.662385321,-0.660550459,-0.658715596,-0.656880734,
-0.655045872,-0.653211009,-0.651376147,-0.649541284,-0.647706422,-0.64587156,
-0.644036697,-0.642201835,-0.640366972,-0.63853211,-0.636697248,-0.634862385,
-0.633027523,-0.631192661,-0.629357798,-0.627522936,-0.625688073,-0.623853211,
-0.622018349,-0.620183486,-0.618348624,-0.616513761,-0.614678899,-0.612844037,
-0.611009174,-0.609174312,-0.60733945,-0.605504587,-0.603669725,-0.601834862,
-0.6,-0.598165138,-0.596330275,-0.594495413,-0.59266055,-0.590825688,-0.588990826,
-0.587155963,-0.585321101,-0.583486239,-0.581651376,-0.579816514,-0.577981651,
-0.576146789,-0.574311927,-0.572477064,-0.570642202,-0.568807339,-0.566972477,
-0.565137615,-0.563302752,-0.56146789,-0.559633028,-0.557798165,-0.555963303,
-0.55412844,-0.552293578,-0.550458716,-0.548623853,-0.546788991,-0.544954128,
-0.543119266,-0.541284404,-0.539449541,-0.537614679,-0.535779817,-0.533944954,
-0.532110092,-0.530275229,-0.528440367,-0.526605505,-0.524770642,-0.52293578,
-0.521100917,-0.519266055,-0.517431193,-0.51559633,-0.513761468,-0.511926606,
-0.510091743,-0.508256881,-0.506422018,-0.504587156,-0.502752294,-0.500917431,
-0.499082569,-0.497247706,-0.495412844,-0.493577982,-0.491743119,-0.489908257,
-0.488073394,-0.486238532,-0.48440367,-0.482568807,-0.480733945,-0.478899083,
-0.47706422,-0.475229358,-0.473394495,-0.471559633,-0.469724771,-0.467889908,
-0.466055046,-0.464220183,-0.462385321,-0.460550459,-0.458715596,-0.456880734,
-0.455045872,-0.453211009,-0.451376147,-0.449541284,-0.447706422,-0.44587156,
-0.444036697,-0.442201835,-0.440366972,-0.43853211,-0.436697248,-0.434862385,
-0.433027523,-0.431192661,-0.429357798,-0.427522936,-0.425688073,-0.423853211,
-0.422018349,-0.420183486,-0.418348624,-0.416513761,-0.414678899,-0.412844037,
-0.411009174,-0.409174312,-0.40733945,-0.405504587,-0.403669725,-0.401834862,
-0.4,-0.398165138,-0.396330275,-0.394495413,-0.39266055,-0.390825688,-0.388990826,
-0.387155963,-0.385321101,-0.383486239,-0.381651376,-0.379816514,-0.377981651,
-0.376146789,-0.374311927,-0.372477064,-0.370642202,-0.368807339,-0.366972477,
-0.365137615,-0.363302752,-0.36146789,-0.359633028,-0.357798165,-0.355963303,
-0.35412844,-0.352293578,-0.350458716,-0.348623853,-0.346788991,-0.344954128,
-0.343119266,-0.341284404,-0.339449541,-0.337614679,-0.335779817,-0.333944954,
-0.332110092,-0.330275229,-0.328440367,-0.326605505,-0.324770642,-0.32293578,
-0.321100917,-0.319266055,-0.317431193,-0.31559633,-0.313761468,-0.311926606,
-0.310091743,-0.308256881,-0.306422018,-0.304587156,-0.302752294,-0.300917431,
-0.299082569,-0.297247706,-0.295412844,-0.293577982,-0.291743119,-0.289908257,
-0.288073394,-0.286238532,-0.28440367,-0.282568807,-0.280733945,-0.278899083,
-0.27706422,-0.275229358,-0.273394495,-0.271559633,-0.269724771,-0.267889908,
-0.266055046,-0.264220183,-0.262385321,-0.260550459,-0.258715596,-0.256880734,
-0.255045872,-0.253211009,-0.251376147,-0.249541284,-0.247706422,-0.24587156,
-0.244036697,-0.242201835,-0.240366972,-0.23853211,-0.236697248,-0.234862385,
-0.233027523,-0.231192661,-0.229357798,-0.227522936,-0.225688073,-0.223853211,
-0.222018349,-0.220183486,-0.218348624,-0.216513761,-0.214678899,-0.212844037,
-0.211009174,-0.209174312,-0.20733945,-0.205504587,-0.203669725,-0.201834862,
-0.2,-0.198165138,-0.196330275,-0.194495413,-0.19266055,-0.190825688,-0.188990826,
-0.187155963,-0.185321101,-0.183486239,-0.181651376,-0.179816514,-0.177981651,
-0.176146789,-0.174311927,-0.172477064,-0.170642202,-0.168807339,-0.166972477,
-0.165137615,-0.163302752,-0.16146789,-0.159633028,-0.157798165,-0.155963303,
-0.15412844,-0.152293578,-0.150458716,-0.148623853,-0.146788991,-0.144954128,
-0.143172103),(0.,0.36),.UNSPECIFIED.);
#6277=B_SPLINE_SURFACE_WITH_KNOTS('',5,1,((#255763,#255764),(#255765,#255766),
(#255767,#255768),(#255769,#255770),(#255771,#255772),(#255773,#255774),
(#255775,#255776),(#255777,#255778),(#255779,#255780),(#255781,#255782),
(#255783,#255784),(#255785,#255786),(#255787,#255788),(#255789,#255790),
(#255791,#255792),(#255793,#255794),(#255795,#255796),(#255797,#255798),
(#255799,#255800),(#255801,#255802),(#255803,#255804),(#255805,#255806),
(#255807,#255808),(#255809,#255810),(#255811,#255812),(#255813,#255814),
(#255815,#255816),(#255817,#255818),(#255819,#255820),(#255821,#255822),
(#255823,#255824),(#255825,#255826),(#255827,#255828),(#255829,#255830),
(#255831,#255832),(#255833,#255834),(#255835,#255836),(#255837,#255838),
(#255839,#255840),(#255841,#255842),(#255843,#255844),(#255845,#255846),
(#255847,#255848),(#255849,#255850),(#255851,#255852),(#255853,#255854),
(#255855,#255856),(#255857,#255858),(#255859,#255860),(#255861,#255862),
(#255863,#255864),(#255865,#255866),(#255867,#255868),(#255869,#255870),
(#255871,#255872),(#255873,#255874),(#255875,#255876),(#255877,#255878),
(#255879,#255880),(#255881,#255882),(#255883,#255884),(#255885,#255886),
(#255887,#255888),(#255889,#255890),(#255891,#255892),(#255893,#255894),
(#255895,#255896),(#255897,#255898),(#255899,#255900),(#255901,#255902),
(#255903,#255904),(#255905,#255906),(#255907,#255908),(#255909,#255910),
(#255911,#255912),(#255913,#255914),(#255915,#255916),(#255917,#255918),
(#255919,#255920),(#255921,#255922),(#255923,#255924),(#255925,#255926),
(#255927,#255928),(#255929,#255930),(#255931,#255932),(#255933,#255934),
(#255935,#255936),(#255937,#255938),(#255939,#255940),(#255941,#255942),
(#255943,#255944),(#255945,#255946),(#255947,#255948),(#255949,#255950),
(#255951,#255952),(#255953,#255954),(#255955,#255956),(#255957,#255958),
(#255959,#255960),(#255961,#255962),(#255963,#255964),(#255965,#255966),
(#255967,#255968),(#255969,#255970),(#255971,#255972),(#255973,#255974),
(#255975,#255976),(#255977,#255978),(#255979,#255980),(#255981,#255982),
(#255983,#255984),(#255985,#255986),(#255987,#255988),(#255989,#255990),
(#255991,#255992),(#255993,#255994),(#255995,#255996),(#255997,#255998),
(#255999,#256000),(#256001,#256002),(#256003,#256004),(#256005,#256006),
(#256007,#256008),(#256009,#256010),(#256011,#256012),(#256013,#256014),
(#256015,#256016),(#256017,#256018),(#256019,#256020),(#256021,#256022),
(#256023,#256024),(#256025,#256026),(#256027,#256028),(#256029,#256030),
(#256031,#256032),(#256033,#256034),(#256035,#256036),(#256037,#256038),
(#256039,#256040),(#256041,#256042),(#256043,#256044),(#256045,#256046),
(#256047,#256048),(#256049,#256050),(#256051,#256052),(#256053,#256054),
(#256055,#256056),(#256057,#256058),(#256059,#256060),(#256061,#256062),
(#256063,#256064),(#256065,#256066),(#256067,#256068),(#256069,#256070),
(#256071,#256072),(#256073,#256074),(#256075,#256076),(#256077,#256078),
(#256079,#256080),(#256081,#256082),(#256083,#256084),(#256085,#256086),
(#256087,#256088),(#256089,#256090),(#256091,#256092),(#256093,#256094),
(#256095,#256096),(#256097,#256098),(#256099,#256100),(#256101,#256102),
(#256103,#256104),(#256105,#256106),(#256107,#256108),(#256109,#256110),
(#256111,#256112),(#256113,#256114),(#256115,#256116),(#256117,#256118),
(#256119,#256120),(#256121,#256122),(#256123,#256124),(#256125,#256126),
(#256127,#256128),(#256129,#256130),(#256131,#256132),(#256133,#256134),
(#256135,#256136),(#256137,#256138),(#256139,#256140),(#256141,#256142),
(#256143,#256144),(#256145,#256146),(#256147,#256148),(#256149,#256150),
(#256151,#256152),(#256153,#256154),(#256155,#256156),(#256157,#256158),
(#256159,#256160),(#256161,#256162),(#256163,#256164),(#256165,#256166),
(#256167,#256168),(#256169,#256170),(#256171,#256172),(#256173,#256174),
(#256175,#256176),(#256177,#256178),(#256179,#256180),(#256181,#256182),
(#256183,#256184),(#256185,#256186),(#256187,#256188),(#256189,#256190),
(#256191,#256192),(#256193,#256194),(#256195,#256196),(#256197,#256198),
(#256199,#256200),(#256201,#256202),(#256203,#256204),(#256205,#256206),
(#256207,#256208),(#256209,#256210),(#256211,#256212),(#256213,#256214),
(#256215,#256216),(#256217,#256218),(#256219,#256220),(#256221,#256222),
(#256223,#256224),(#256225,#256226),(#256227,#256228),(#256229,#256230),
(#256231,#256232),(#256233,#256234),(#256235,#256236),(#256237,#256238),
(#256239,#256240),(#256241,#256242),(#256243,#256244),(#256245,#256246),
(#256247,#256248),(#256249,#256250),(#256251,#256252),(#256253,#256254),
(#256255,#256256),(#256257,#256258),(#256259,#256260),(#256261,#256262),
(#256263,#256264),(#256265,#256266),(#256267,#256268),(#256269,#256270),
(#256271,#256272),(#256273,#256274),(#256275,#256276),(#256277,#256278),
(#256279,#256280),(#256281,#256282),(#256283,#256284),(#256285,#256286),
(#256287,#256288),(#256289,#256290),(#256291,#256292),(#256293,#256294),
(#256295,#256296),(#256297,#256298),(#256299,#256300),(#256301,#256302),
(#256303,#256304),(#256305,#256306),(#256307,#256308),(#256309,#256310),
(#256311,#256312),(#256313,#256314),(#256315,#256316),(#256317,#256318),
(#256319,#256320),(#256321,#256322),(#256323,#256324),(#256325,#256326),
(#256327,#256328),(#256329,#256330),(#256331,#256332),(#256333,#256334),
(#256335,#256336),(#256337,#256338),(#256339,#256340),(#256341,#256342),
(#256343,#256344),(#256345,#256346),(#256347,#256348),(#256349,#256350),
(#256351,#256352),(#256353,#256354),(#256355,#256356),(#256357,#256358),
(#256359,#256360),(#256361,#256362),(#256363,#256364),(#256365,#256366),
(#256367,#256368),(#256369,#256370),(#256371,#256372),(#256373,#256374),
(#256375,#256376),(#256377,#256378),(#256379,#256380),(#256381,#256382),
(#256383,#256384),(#256385,#256386),(#256387,#256388),(#256389,#256390),
(#256391,#256392),(#256393,#256394),(#256395,#256396),(#256397,#256398),
(#256399,#256400),(#256401,#256402),(#256403,#256404),(#256405,#256406),
(#256407,#256408),(#256409,#256410),(#256411,#256412),(#256413,#256414),
(#256415,#256416),(#256417,#256418),(#256419,#256420),(#256421,#256422),
(#256423,#256424),(#256425,#256426),(#256427,#256428),(#256429,#256430),
(#256431,#256432),(#256433,#256434),(#256435,#256436),(#256437,#256438),
(#256439,#256440),(#256441,#256442),(#256443,#256444),(#256445,#256446),
(#256447,#256448),(#256449,#256450),(#256451,#256452),(#256453,#256454),
(#256455,#256456),(#256457,#256458),(#256459,#256460),(#256461,#256462),
(#256463,#256464),(#256465,#256466),(#256467,#256468),(#256469,#256470),
(#256471,#256472),(#256473,#256474),(#256475,#256476),(#256477,#256478),
(#256479,#256480),(#256481,#256482),(#256483,#256484),(#256485,#256486),
(#256487,#256488),(#256489,#256490),(#256491,#256492),(#256493,#256494),
(#256495,#256496),(#256497,#256498),(#256499,#256500),(#256501,#256502),
(#256503,#256504),(#256505,#256506),(#256507,#256508),(#256509,#256510),
(#256511,#256512),(#256513,#256514),(#256515,#256516),(#256517,#256518),
(#256519,#256520),(#256521,#256522),(#256523,#256524),(#256525,#256526),
(#256527,#256528),(#256529,#256530),(#256531,#256532),(#256533,#256534),
(#256535,#256536),(#256537,#256538),(#256539,#256540),(#256541,#256542),
(#256543,#256544),(#256545,#256546),(#256547,#256548),(#256549,#256550),
(#256551,#256552),(#256553,#256554),(#256555,#256556),(#256557,#256558),
(#256559,#256560),(#256561,#256562),(#256563,#256564),(#256565,#256566),
(#256567,#256568),(#256569,#256570),(#256571,#256572),(#256573,#256574),
(#256575,#256576),(#256577,#256578),(#256579,#256580),(#256581,#256582),
(#256583,#256584),(#256585,#256586),(#256587,#256588),(#256589,#256590),
(#256591,#256592),(#256593,#256594),(#256595,#256596),(#256597,#256598),
(#256599,#256600),(#256601,#256602),(#256603,#256604),(#256605,#256606),
(#256607,#256608),(#256609,#256610),(#256611,#256612),(#256613,#256614),
(#256615,#256616),(#256617,#256618),(#256619,#256620),(#256621,#256622),
(#256623,#256624),(#256625,#256626),(#256627,#256628),(#256629,#256630),
(#256631,#256632),(#256633,#256634),(#256635,#256636),(#256637,#256638),
(#256639,#256640),(#256641,#256642),(#256643,#256644),(#256645,#256646),
(#256647,#256648),(#256649,#256650),(#256651,#256652),(#256653,#256654),
(#256655,#256656),(#256657,#256658),(#256659,#256660),(#256661,#256662),
(#256663,#256664),(#256665,#256666),(#256667,#256668),(#256669,#256670),
(#256671,#256672),(#256673,#256674),(#256675,#256676),(#256677,#256678),
(#256679,#256680),(#256681,#256682),(#256683,#256684),(#256685,#256686),
(#256687,#256688),(#256689,#256690),(#256691,#256692),(#256693,#256694),
(#256695,#256696),(#256697,#256698),(#256699,#256700),(#256701,#256702),
(#256703,#256704),(#256705,#256706)),.UNSPECIFIED.,.F.,.F.,.F.,(6,1,1,1,
1,1,1,1,1,1,1,1,1,1,1,1,1,1,1,1,1,1,1,1,1,1,1,1,1,1,1,1,1,1,1,1,1,1,1,1,
1,1,1,1,1,1,1,1,1,1,1,1,1,1,1,1,1,1,1,1,1,1,1,1,1,1,1,1,1,1,1,1,1,1,1,1,
1,1,1,1,1,1,1,1,1,1,1,1,1,1,1,1,1,1,1,1,1,1,1,1,1,1,1,1,1,1,1,1,1,1,1,1,
1,1,1,1,1,1,1,1,1,1,1,1,1,1,1,1,1,1,1,1,1,1,1,1,1,1,1,1,1,1,1,1,1,1,1,1,
1,1,1,1,1,1,1,1,1,1,1,1,1,1,1,1,1,1,1,1,1,1,1,1,1,1,1,1,1,1,1,1,1,1,1,1,
1,1,1,1,1,1,1,1,1,1,1,1,1,1,1,1,1,1,1,1,1,1,1,1,1,1,1,1,1,1,1,1,1,1,1,1,
1,1,1,1,1,1,1,1,1,1,1,1,1,1,1,1,1,1,1,1,1,1,1,1,1,1,1,1,1,1,1,1,1,1,1,1,
1,1,1,1,1,1,1,1,1,1,1,1,1,1,1,1,1,1,1,1,1,1,1,1,1,1,1,1,1,1,1,1,1,1,1,1,
1,1,1,1,1,1,1,1,1,1,1,1,1,1,1,1,1,1,1,1,1,1,1,1,1,1,1,1,1,1,1,1,1,1,1,1,
1,1,1,1,1,1,1,1,1,1,1,1,1,1,1,1,1,1,1,1,1,1,1,1,1,1,1,1,1,1,1,1,1,1,1,1,
1,1,1,1,1,1,1,1,1,1,1,1,1,1,1,1,1,1,1,1,1,1,1,1,1,1,1,1,1,1,1,1,1,1,1,1,
1,1,1,1,1,1,1,1,1,1,1,1,1,1,1,1,1,1,1,1,1,1,1,1,1,1,1,1,1,1,1,1,1,1,1,1,
1,1,1,1,1,1,1,1,1,1,1,1,1,1,1,1,1,1,1,1,1,1,1,1,1,1,1,1,1,1,1,6),(2,2),
(-1.,-0.998165138,-0.996330275,-0.994495413,-0.99266055,-0.990825688,-0.988990826,
-0.987155963,-0.985321101,-0.983486239,-0.981651376,-0.979816514,-0.977981651,
-0.976146789,-0.974311927,-0.972477064,-0.970642202,-0.968807339,-0.966972477,
-0.965137615,-0.963302752,-0.96146789,-0.959633028,-0.957798165,-0.955963303,
-0.95412844,-0.952293578,-0.950458716,-0.948623853,-0.946788991,-0.944954128,
-0.943119266,-0.941284404,-0.939449541,-0.937614679,-0.935779817,-0.933944954,
-0.932110092,-0.930275229,-0.928440367,-0.926605505,-0.924770642,-0.92293578,
-0.921100917,-0.919266055,-0.917431193,-0.91559633,-0.913761468,-0.911926606,
-0.910091743,-0.908256881,-0.906422018,-0.904587156,-0.902752294,-0.900917431,
-0.899082569,-0.897247706,-0.895412844,-0.893577982,-0.891743119,-0.889908257,
-0.888073394,-0.886238532,-0.88440367,-0.882568807,-0.880733945,-0.878899083,
-0.87706422,-0.875229358,-0.873394495,-0.871559633,-0.869724771,-0.867889908,
-0.866055046,-0.864220183,-0.862385321,-0.860550459,-0.858715596,-0.856880734,
-0.855045872,-0.853211009,-0.851376147,-0.849541284,-0.847706422,-0.84587156,
-0.844036697,-0.842201835,-0.840366972,-0.83853211,-0.836697248,-0.834862385,
-0.833027523,-0.831192661,-0.829357798,-0.827522936,-0.825688073,-0.823853211,
-0.822018349,-0.820183486,-0.818348624,-0.816513761,-0.814678899,-0.812844037,
-0.811009174,-0.809174312,-0.80733945,-0.805504587,-0.803669725,-0.801834862,
-0.8,-0.798165138,-0.796330275,-0.794495413,-0.79266055,-0.790825688,-0.788990826,
-0.787155963,-0.785321101,-0.783486239,-0.781651376,-0.779816514,-0.777981651,
-0.776146789,-0.774311927,-0.772477064,-0.770642202,-0.768807339,-0.766972477,
-0.765137615,-0.763302752,-0.76146789,-0.759633028,-0.757798165,-0.755963303,
-0.75412844,-0.752293578,-0.750458716,-0.748623853,-0.746788991,-0.744954128,
-0.743119266,-0.741284404,-0.739449541,-0.737614679,-0.735779817,-0.733944954,
-0.732110092,-0.730275229,-0.728440367,-0.726605505,-0.724770642,-0.72293578,
-0.721100917,-0.719266055,-0.717431193,-0.71559633,-0.713761468,-0.711926606,
-0.710091743,-0.708256881,-0.706422018,-0.704587156,-0.702752294,-0.700917431,
-0.699082569,-0.697247706,-0.695412844,-0.693577982,-0.691743119,-0.689908257,
-0.688073394,-0.686238532,-0.68440367,-0.682568807,-0.680733945,-0.678899083,
-0.67706422,-0.675229358,-0.673394495,-0.671559633,-0.669724771,-0.667889908,
-0.666055046,-0.664220183,-0.662385321,-0.660550459,-0.658715596,-0.656880734,
-0.655045872,-0.653211009,-0.651376147,-0.649541284,-0.647706422,-0.64587156,
-0.644036697,-0.642201835,-0.640366972,-0.63853211,-0.636697248,-0.634862385,
-0.633027523,-0.631192661,-0.629357798,-0.627522936,-0.625688073,-0.623853211,
-0.622018349,-0.620183486,-0.618348624,-0.616513761,-0.614678899,-0.612844037,
-0.611009174,-0.609174312,-0.60733945,-0.605504587,-0.603669725,-0.601834862,
-0.6,-0.598165138,-0.596330275,-0.594495413,-0.59266055,-0.590825688,-0.588990826,
-0.587155963,-0.585321101,-0.583486239,-0.581651376,-0.579816514,-0.577981651,
-0.576146789,-0.574311927,-0.572477064,-0.570642202,-0.568807339,-0.566972477,
-0.565137615,-0.563302752,-0.56146789,-0.559633028,-0.557798165,-0.555963303,
-0.55412844,-0.552293578,-0.550458716,-0.548623853,-0.546788991,-0.544954128,
-0.543119266,-0.541284404,-0.539449541,-0.537614679,-0.535779817,-0.533944954,
-0.532110092,-0.530275229,-0.528440367,-0.526605505,-0.524770642,-0.52293578,
-0.521100917,-0.519266055,-0.517431193,-0.51559633,-0.513761468,-0.511926606,
-0.510091743,-0.508256881,-0.506422018,-0.504587156,-0.502752294,-0.500917431,
-0.499082569,-0.497247706,-0.495412844,-0.493577982,-0.491743119,-0.489908257,
-0.488073394,-0.486238532,-0.48440367,-0.482568807,-0.480733945,-0.478899083,
-0.47706422,-0.475229358,-0.473394495,-0.471559633,-0.469724771,-0.467889908,
-0.466055046,-0.464220183,-0.462385321,-0.460550459,-0.458715596,-0.456880734,
-0.455045872,-0.453211009,-0.451376147,-0.449541284,-0.447706422,-0.44587156,
-0.444036697,-0.442201835,-0.440366972,-0.43853211,-0.436697248,-0.434862385,
-0.433027523,-0.431192661,-0.429357798,-0.427522936,-0.425688073,-0.423853211,
-0.422018349,-0.420183486,-0.418348624,-0.416513761,-0.414678899,-0.412844037,
-0.411009174,-0.409174312,-0.40733945,-0.405504587,-0.403669725,-0.401834862,
-0.4,-0.398165138,-0.396330275,-0.394495413,-0.39266055,-0.390825688,-0.388990826,
-0.387155963,-0.385321101,-0.383486239,-0.381651376,-0.379816514,-0.377981651,
-0.376146789,-0.374311927,-0.372477064,-0.370642202,-0.368807339,-0.366972477,
-0.365137615,-0.363302752,-0.36146789,-0.359633028,-0.357798165,-0.355963303,
-0.35412844,-0.352293578,-0.350458716,-0.348623853,-0.346788991,-0.344954128,
-0.343119266,-0.341284404,-0.339449541,-0.337614679,-0.335779817,-0.333944954,
-0.332110092,-0.330275229,-0.328440367,-0.326605505,-0.324770642,-0.32293578,
-0.321100917,-0.319266055,-0.317431193,-0.31559633,-0.313761468,-0.311926606,
-0.310091743,-0.308256881,-0.306422018,-0.304587156,-0.302752294,-0.300917431,
-0.299082569,-0.297247706,-0.295412844,-0.293577982,-0.291743119,-0.289908257,
-0.288073394,-0.286238532,-0.28440367,-0.282568807,-0.280733945,-0.278899083,
-0.27706422,-0.275229358,-0.273394495,-0.271559633,-0.269724771,-0.267889908,
-0.266055046,-0.264220183,-0.262385321,-0.260550459,-0.258715596,-0.256880734,
-0.255045872,-0.253211009,-0.251376147,-0.249541284,-0.247706422,-0.24587156,
-0.244036697,-0.242201835,-0.240366972,-0.23853211,-0.236697248,-0.234862385,
-0.233027523,-0.231192661,-0.229357798,-0.227522936,-0.225688073,-0.223853211,
-0.222018349,-0.220183486,-0.218348624,-0.216513761,-0.214678899,-0.212844037,
-0.211009174,-0.209174312,-0.20733945,-0.205504587,-0.203669725,-0.201834862,
-0.2,-0.198165138,-0.196330275,-0.194495413,-0.19266055,-0.190825688,-0.188990826,
-0.187155963,-0.185321101,-0.183486239,-0.181651376,-0.179816514,-0.177981651,
-0.176146789,-0.174311927,-0.172477064,-0.170642202,-0.168807339,-0.166972477,
-0.165137615,-0.163302752,-0.16146789,-0.159633028,-0.157798165,-0.155963303,
-0.15412844,-0.152293578,-0.150458716,-0.148623853,-0.146788991,-0.144954128,
-0.143172103),(0.,0.36),.UNSPECIFIED.);
#6278=B_SPLINE_SURFACE_WITH_KNOTS('',5,1,((#257339,#257340),(#257341,#257342),
(#257343,#257344),(#257345,#257346),(#257347,#257348),(#257349,#257350),
(#257351,#257352),(#257353,#257354),(#257355,#257356),(#257357,#257358),
(#257359,#257360),(#257361,#257362),(#257363,#257364),(#257365,#257366),
(#257367,#257368),(#257369,#257370),(#257371,#257372),(#257373,#257374),
(#257375,#257376),(#257377,#257378),(#257379,#257380),(#257381,#257382),
(#257383,#257384),(#257385,#257386),(#257387,#257388),(#257389,#257390),
(#257391,#257392),(#257393,#257394),(#257395,#257396),(#257397,#257398),
(#257399,#257400),(#257401,#257402),(#257403,#257404),(#257405,#257406),
(#257407,#257408),(#257409,#257410),(#257411,#257412),(#257413,#257414),
(#257415,#257416),(#257417,#257418),(#257419,#257420),(#257421,#257422),
(#257423,#257424),(#257425,#257426),(#257427,#257428),(#257429,#257430),
(#257431,#257432),(#257433,#257434),(#257435,#257436),(#257437,#257438),
(#257439,#257440),(#257441,#257442),(#257443,#257444),(#257445,#257446),
(#257447,#257448),(#257449,#257450),(#257451,#257452),(#257453,#257454),
(#257455,#257456),(#257457,#257458),(#257459,#257460),(#257461,#257462),
(#257463,#257464),(#257465,#257466),(#257467,#257468),(#257469,#257470),
(#257471,#257472),(#257473,#257474),(#257475,#257476),(#257477,#257478),
(#257479,#257480),(#257481,#257482),(#257483,#257484),(#257485,#257486),
(#257487,#257488),(#257489,#257490),(#257491,#257492),(#257493,#257494),
(#257495,#257496),(#257497,#257498),(#257499,#257500),(#257501,#257502),
(#257503,#257504),(#257505,#257506),(#257507,#257508),(#257509,#257510),
(#257511,#257512),(#257513,#257514),(#257515,#257516),(#257517,#257518),
(#257519,#257520),(#257521,#257522),(#257523,#257524),(#257525,#257526),
(#257527,#257528),(#257529,#257530),(#257531,#257532),(#257533,#257534),
(#257535,#257536),(#257537,#257538),(#257539,#257540),(#257541,#257542),
(#257543,#257544),(#257545,#257546),(#257547,#257548),(#257549,#257550),
(#257551,#257552),(#257553,#257554),(#257555,#257556),(#257557,#257558),
(#257559,#257560),(#257561,#257562),(#257563,#257564),(#257565,#257566),
(#257567,#257568),(#257569,#257570),(#257571,#257572),(#257573,#257574),
(#257575,#257576),(#257577,#257578),(#257579,#257580),(#257581,#257582),
(#257583,#257584),(#257585,#257586),(#257587,#257588),(#257589,#257590),
(#257591,#257592),(#257593,#257594),(#257595,#257596),(#257597,#257598),
(#257599,#257600),(#257601,#257602),(#257603,#257604),(#257605,#257606),
(#257607,#257608),(#257609,#257610),(#257611,#257612),(#257613,#257614),
(#257615,#257616),(#257617,#257618),(#257619,#257620),(#257621,#257622),
(#257623,#257624),(#257625,#257626),(#257627,#257628),(#257629,#257630),
(#257631,#257632),(#257633,#257634),(#257635,#257636),(#257637,#257638),
(#257639,#257640),(#257641,#257642),(#257643,#257644),(#257645,#257646),
(#257647,#257648),(#257649,#257650),(#257651,#257652),(#257653,#257654),
(#257655,#257656),(#257657,#257658),(#257659,#257660),(#257661,#257662),
(#257663,#257664),(#257665,#257666),(#257667,#257668),(#257669,#257670),
(#257671,#257672),(#257673,#257674),(#257675,#257676),(#257677,#257678),
(#257679,#257680),(#257681,#257682),(#257683,#257684),(#257685,#257686),
(#257687,#257688),(#257689,#257690),(#257691,#257692),(#257693,#257694),
(#257695,#257696),(#257697,#257698),(#257699,#257700),(#257701,#257702),
(#257703,#257704),(#257705,#257706),(#257707,#257708),(#257709,#257710),
(#257711,#257712),(#257713,#257714),(#257715,#257716),(#257717,#257718),
(#257719,#257720),(#257721,#257722),(#257723,#257724),(#257725,#257726),
(#257727,#257728),(#257729,#257730),(#257731,#257732),(#257733,#257734),
(#257735,#257736),(#257737,#257738),(#257739,#257740),(#257741,#257742),
(#257743,#257744),(#257745,#257746),(#257747,#257748),(#257749,#257750),
(#257751,#257752),(#257753,#257754),(#257755,#257756),(#257757,#257758),
(#257759,#257760),(#257761,#257762),(#257763,#257764),(#257765,#257766),
(#257767,#257768),(#257769,#257770),(#257771,#257772),(#257773,#257774),
(#257775,#257776),(#257777,#257778),(#257779,#257780),(#257781,#257782),
(#257783,#257784),(#257785,#257786),(#257787,#257788),(#257789,#257790),
(#257791,#257792),(#257793,#257794),(#257795,#257796),(#257797,#257798),
(#257799,#257800),(#257801,#257802),(#257803,#257804),(#257805,#257806),
(#257807,#257808),(#257809,#257810),(#257811,#257812),(#257813,#257814),
(#257815,#257816),(#257817,#257818),(#257819,#257820),(#257821,#257822),
(#257823,#257824),(#257825,#257826),(#257827,#257828),(#257829,#257830),
(#257831,#257832),(#257833,#257834),(#257835,#257836),(#257837,#257838),
(#257839,#257840),(#257841,#257842),(#257843,#257844),(#257845,#257846),
(#257847,#257848),(#257849,#257850),(#257851,#257852),(#257853,#257854),
(#257855,#257856),(#257857,#257858),(#257859,#257860),(#257861,#257862),
(#257863,#257864),(#257865,#257866),(#257867,#257868),(#257869,#257870),
(#257871,#257872),(#257873,#257874),(#257875,#257876),(#257877,#257878),
(#257879,#257880),(#257881,#257882),(#257883,#257884),(#257885,#257886),
(#257887,#257888),(#257889,#257890),(#257891,#257892),(#257893,#257894),
(#257895,#257896),(#257897,#257898),(#257899,#257900),(#257901,#257902),
(#257903,#257904),(#257905,#257906),(#257907,#257908),(#257909,#257910),
(#257911,#257912),(#257913,#257914),(#257915,#257916),(#257917,#257918),
(#257919,#257920),(#257921,#257922),(#257923,#257924),(#257925,#257926),
(#257927,#257928),(#257929,#257930),(#257931,#257932),(#257933,#257934),
(#257935,#257936),(#257937,#257938),(#257939,#257940),(#257941,#257942),
(#257943,#257944),(#257945,#257946),(#257947,#257948),(#257949,#257950),
(#257951,#257952),(#257953,#257954),(#257955,#257956),(#257957,#257958),
(#257959,#257960),(#257961,#257962),(#257963,#257964),(#257965,#257966),
(#257967,#257968),(#257969,#257970),(#257971,#257972),(#257973,#257974),
(#257975,#257976),(#257977,#257978),(#257979,#257980),(#257981,#257982),
(#257983,#257984),(#257985,#257986),(#257987,#257988),(#257989,#257990),
(#257991,#257992),(#257993,#257994),(#257995,#257996),(#257997,#257998),
(#257999,#258000),(#258001,#258002),(#258003,#258004),(#258005,#258006),
(#258007,#258008),(#258009,#258010),(#258011,#258012),(#258013,#258014),
(#258015,#258016),(#258017,#258018),(#258019,#258020),(#258021,#258022),
(#258023,#258024),(#258025,#258026),(#258027,#258028),(#258029,#258030),
(#258031,#258032),(#258033,#258034),(#258035,#258036),(#258037,#258038),
(#258039,#258040),(#258041,#258042),(#258043,#258044),(#258045,#258046),
(#258047,#258048),(#258049,#258050),(#258051,#258052),(#258053,#258054),
(#258055,#258056),(#258057,#258058),(#258059,#258060),(#258061,#258062),
(#258063,#258064),(#258065,#258066),(#258067,#258068),(#258069,#258070),
(#258071,#258072),(#258073,#258074),(#258075,#258076),(#258077,#258078),
(#258079,#258080),(#258081,#258082),(#258083,#258084),(#258085,#258086),
(#258087,#258088),(#258089,#258090),(#258091,#258092),(#258093,#258094),
(#258095,#258096),(#258097,#258098),(#258099,#258100),(#258101,#258102),
(#258103,#258104),(#258105,#258106),(#258107,#258108),(#258109,#258110),
(#258111,#258112),(#258113,#258114),(#258115,#258116),(#258117,#258118),
(#258119,#258120),(#258121,#258122),(#258123,#258124),(#258125,#258126),
(#258127,#258128),(#258129,#258130),(#258131,#258132),(#258133,#258134),
(#258135,#258136),(#258137,#258138),(#258139,#258140),(#258141,#258142),
(#258143,#258144),(#258145,#258146),(#258147,#258148),(#258149,#258150),
(#258151,#258152),(#258153,#258154),(#258155,#258156),(#258157,#258158),
(#258159,#258160),(#258161,#258162),(#258163,#258164),(#258165,#258166),
(#258167,#258168),(#258169,#258170),(#258171,#258172),(#258173,#258174),
(#258175,#258176),(#258177,#258178),(#258179,#258180),(#258181,#258182),
(#258183,#258184),(#258185,#258186),(#258187,#258188),(#258189,#258190),
(#258191,#258192),(#258193,#258194),(#258195,#258196),(#258197,#258198),
(#258199,#258200),(#258201,#258202),(#258203,#258204),(#258205,#258206),
(#258207,#258208),(#258209,#258210),(#258211,#258212),(#258213,#258214),
(#258215,#258216),(#258217,#258218),(#258219,#258220),(#258221,#258222),
(#258223,#258224),(#258225,#258226),(#258227,#258228),(#258229,#258230),
(#258231,#258232),(#258233,#258234),(#258235,#258236),(#258237,#258238),
(#258239,#258240),(#258241,#258242),(#258243,#258244),(#258245,#258246),
(#258247,#258248),(#258249,#258250),(#258251,#258252),(#258253,#258254),
(#258255,#258256),(#258257,#258258),(#258259,#258260),(#258261,#258262),
(#258263,#258264),(#258265,#258266),(#258267,#258268),(#258269,#258270),
(#258271,#258272),(#258273,#258274),(#258275,#258276),(#258277,#258278),
(#258279,#258280),(#258281,#258282)),.UNSPECIFIED.,.F.,.F.,.F.,(6,1,1,1,
1,1,1,1,1,1,1,1,1,1,1,1,1,1,1,1,1,1,1,1,1,1,1,1,1,1,1,1,1,1,1,1,1,1,1,1,
1,1,1,1,1,1,1,1,1,1,1,1,1,1,1,1,1,1,1,1,1,1,1,1,1,1,1,1,1,1,1,1,1,1,1,1,
1,1,1,1,1,1,1,1,1,1,1,1,1,1,1,1,1,1,1,1,1,1,1,1,1,1,1,1,1,1,1,1,1,1,1,1,
1,1,1,1,1,1,1,1,1,1,1,1,1,1,1,1,1,1,1,1,1,1,1,1,1,1,1,1,1,1,1,1,1,1,1,1,
1,1,1,1,1,1,1,1,1,1,1,1,1,1,1,1,1,1,1,1,1,1,1,1,1,1,1,1,1,1,1,1,1,1,1,1,
1,1,1,1,1,1,1,1,1,1,1,1,1,1,1,1,1,1,1,1,1,1,1,1,1,1,1,1,1,1,1,1,1,1,1,1,
1,1,1,1,1,1,1,1,1,1,1,1,1,1,1,1,1,1,1,1,1,1,1,1,1,1,1,1,1,1,1,1,1,1,1,1,
1,1,1,1,1,1,1,1,1,1,1,1,1,1,1,1,1,1,1,1,1,1,1,1,1,1,1,1,1,1,1,1,1,1,1,1,
1,1,1,1,1,1,1,1,1,1,1,1,1,1,1,1,1,1,1,1,1,1,1,1,1,1,1,1,1,1,1,1,1,1,1,1,
1,1,1,1,1,1,1,1,1,1,1,1,1,1,1,1,1,1,1,1,1,1,1,1,1,1,1,1,1,1,1,1,1,1,1,1,
1,1,1,1,1,1,1,1,1,1,1,1,1,1,1,1,1,1,1,1,1,1,1,1,1,1,1,1,1,1,1,1,1,1,1,1,
1,1,1,1,1,1,1,1,1,1,1,1,1,1,1,1,1,1,1,1,1,1,1,1,1,1,1,1,1,1,1,1,1,1,1,1,
1,1,1,1,1,1,1,1,1,1,1,1,1,1,1,1,1,1,1,1,1,1,1,1,1,1,1,1,1,1,1,6),(2,2),
(0.143172104,0.144954128,0.146788991,0.148623853,0.150458716,0.152293578,
0.15412844,0.155963303,0.157798165,0.159633028,0.16146789,0.163302752,0.165137615,
0.166972477,0.168807339,0.170642202,0.172477064,0.174311927,0.176146789,
0.177981651,0.179816514,0.181651376,0.183486239,0.185321101,0.187155963,
0.188990826,0.190825688,0.19266055,0.194495413,0.196330275,0.198165138,
0.2,0.201834862,0.203669725,0.205504587,0.20733945,0.209174312,0.211009174,
0.212844037,0.214678899,0.216513761,0.218348624,0.220183486,0.222018349,
0.223853211,0.225688073,0.227522936,0.229357798,0.231192661,0.233027523,
0.234862385,0.236697248,0.23853211,0.240366972,0.242201835,0.244036697,
0.24587156,0.247706422,0.249541284,0.251376147,0.253211009,0.255045872,
0.256880734,0.258715596,0.260550459,0.262385321,0.264220183,0.266055046,
0.267889908,0.269724771,0.271559633,0.273394495,0.275229358,0.27706422,
0.278899083,0.280733945,0.282568807,0.28440367,0.286238532,0.288073394,
0.289908257,0.291743119,0.293577982,0.295412844,0.297247706,0.299082569,
0.300917431,0.302752294,0.304587156,0.306422018,0.308256881,0.310091743,
0.311926606,0.313761468,0.31559633,0.317431193,0.319266055,0.321100917,
0.32293578,0.324770642,0.326605505,0.328440367,0.330275229,0.332110092,
0.333944954,0.335779817,0.337614679,0.339449541,0.341284404,0.343119266,
0.344954128,0.346788991,0.348623853,0.350458716,0.352293578,0.35412844,
0.355963303,0.357798165,0.359633028,0.36146789,0.363302752,0.365137615,
0.366972477,0.368807339,0.370642202,0.372477064,0.374311927,0.376146789,
0.377981651,0.379816514,0.381651376,0.383486239,0.385321101,0.387155963,
0.388990826,0.390825688,0.39266055,0.394495413,0.396330275,0.398165138,
0.4,0.401834862,0.403669725,0.405504587,0.40733945,0.409174312,0.411009174,
0.412844037,0.414678899,0.416513761,0.418348624,0.420183486,0.422018349,
0.423853211,0.425688073,0.427522936,0.429357798,0.431192661,0.433027523,
0.434862385,0.436697248,0.43853211,0.440366972,0.442201835,0.444036697,
0.44587156,0.447706422,0.449541284,0.451376147,0.453211009,0.455045872,
0.456880734,0.458715596,0.460550459,0.462385321,0.464220183,0.466055046,
0.467889908,0.469724771,0.471559633,0.473394495,0.475229358,0.47706422,
0.478899083,0.480733945,0.482568807,0.48440367,0.486238532,0.488073394,
0.489908257,0.491743119,0.493577982,0.495412844,0.497247706,0.499082569,
0.500917431,0.502752294,0.504587156,0.506422018,0.508256881,0.510091743,
0.511926606,0.513761468,0.51559633,0.517431193,0.519266055,0.521100917,
0.52293578,0.524770642,0.526605505,0.528440367,0.530275229,0.532110092,
0.533944954,0.535779817,0.537614679,0.539449541,0.541284404,0.543119266,
0.544954128,0.546788991,0.548623853,0.550458716,0.552293578,0.55412844,
0.555963303,0.557798165,0.559633028,0.56146789,0.563302752,0.565137615,
0.566972477,0.568807339,0.570642202,0.572477064,0.574311927,0.576146789,
0.577981651,0.579816514,0.581651376,0.583486239,0.585321101,0.587155963,
0.588990826,0.590825688,0.59266055,0.594495413,0.596330275,0.598165138,
0.6,0.601834862,0.603669725,0.605504587,0.60733945,0.609174312,0.611009174,
0.612844037,0.614678899,0.616513761,0.618348624,0.620183486,0.622018349,
0.623853211,0.625688073,0.627522936,0.629357798,0.631192661,0.633027523,
0.634862385,0.636697248,0.63853211,0.640366972,0.642201835,0.644036697,
0.64587156,0.647706422,0.649541284,0.651376147,0.653211009,0.655045872,
0.656880734,0.658715596,0.660550459,0.662385321,0.664220183,0.666055046,
0.667889908,0.669724771,0.671559633,0.673394495,0.675229358,0.67706422,
0.678899083,0.680733945,0.682568807,0.68440367,0.686238532,0.688073394,
0.689908257,0.691743119,0.693577982,0.695412844,0.697247706,0.699082569,
0.700917431,0.702752294,0.704587156,0.706422018,0.708256881,0.710091743,
0.711926606,0.713761468,0.71559633,0.717431193,0.719266055,0.721100917,
0.72293578,0.724770642,0.726605505,0.728440367,0.730275229,0.732110092,
0.733944954,0.735779817,0.737614679,0.739449541,0.741284404,0.743119266,
0.744954128,0.746788991,0.748623853,0.750458716,0.752293578,0.75412844,
0.755963303,0.757798165,0.759633028,0.76146789,0.763302752,0.765137615,
0.766972477,0.768807339,0.770642202,0.772477064,0.774311927,0.776146789,
0.777981651,0.779816514,0.781651376,0.783486239,0.785321101,0.787155963,
0.788990826,0.790825688,0.79266055,0.794495413,0.796330275,0.798165138,
0.8,0.801834862,0.803669725,0.805504587,0.80733945,0.809174312,0.811009174,
0.812844037,0.814678899,0.816513761,0.818348624,0.820183486,0.822018349,
0.823853211,0.825688073,0.827522936,0.829357798,0.831192661,0.833027523,
0.834862385,0.836697248,0.83853211,0.840366972,0.842201835,0.844036697,
0.84587156,0.847706422,0.849541284,0.851376147,0.853211009,0.855045872,
0.856880734,0.858715596,0.860550459,0.862385321,0.864220183,0.866055046,
0.867889908,0.869724771,0.871559633,0.873394495,0.875229358,0.87706422,
0.878899083,0.880733945,0.882568807,0.88440367,0.886238532,0.888073394,
0.889908257,0.891743119,0.893577982,0.895412844,0.897247706,0.899082569,
0.900917431,0.902752294,0.904587156,0.906422018,0.908256881,0.910091743,
0.911926606,0.913761468,0.91559633,0.917431193,0.919266055,0.921100917,
0.92293578,0.924770642,0.926605505,0.928440367,0.930275229,0.932110092,
0.933944954,0.935779817,0.937614679,0.939449541,0.941284404,0.943119266,
0.944954128,0.946788991,0.948623853,0.950458716,0.952293578,0.95412844,
0.955963303,0.957798165,0.959633028,0.96146789,0.963302752,0.965137615,
0.966972477,0.968807339,0.970642202,0.972477064,0.974311927,0.976146789,
0.977981651,0.979816514,0.981651376,0.983486239,0.985321101,0.987155963,
0.988990826,0.990825688,0.99266055,0.994495413,0.996330275,0.998165138,
1.),(0.,0.36),.UNSPECIFIED.);
#6279=B_SPLINE_SURFACE_WITH_KNOTS('',5,1,((#258912,#258913),(#258914,#258915),
(#258916,#258917),(#258918,#258919),(#258920,#258921),(#258922,#258923),
(#258924,#258925),(#258926,#258927),(#258928,#258929),(#258930,#258931),
(#258932,#258933),(#258934,#258935),(#258936,#258937),(#258938,#258939),
(#258940,#258941),(#258942,#258943),(#258944,#258945),(#258946,#258947),
(#258948,#258949),(#258950,#258951),(#258952,#258953),(#258954,#258955),
(#258956,#258957),(#258958,#258959),(#258960,#258961),(#258962,#258963),
(#258964,#258965),(#258966,#258967),(#258968,#258969),(#258970,#258971),
(#258972,#258973),(#258974,#258975),(#258976,#258977),(#258978,#258979),
(#258980,#258981),(#258982,#258983),(#258984,#258985),(#258986,#258987),
(#258988,#258989),(#258990,#258991),(#258992,#258993),(#258994,#258995),
(#258996,#258997),(#258998,#258999),(#259000,#259001),(#259002,#259003),
(#259004,#259005),(#259006,#259007),(#259008,#259009),(#259010,#259011),
(#259012,#259013),(#259014,#259015),(#259016,#259017),(#259018,#259019),
(#259020,#259021),(#259022,#259023),(#259024,#259025),(#259026,#259027),
(#259028,#259029),(#259030,#259031),(#259032,#259033),(#259034,#259035),
(#259036,#259037),(#259038,#259039),(#259040,#259041),(#259042,#259043),
(#259044,#259045),(#259046,#259047),(#259048,#259049),(#259050,#259051),
(#259052,#259053),(#259054,#259055),(#259056,#259057),(#259058,#259059),
(#259060,#259061),(#259062,#259063),(#259064,#259065),(#259066,#259067),
(#259068,#259069),(#259070,#259071),(#259072,#259073),(#259074,#259075),
(#259076,#259077),(#259078,#259079),(#259080,#259081),(#259082,#259083),
(#259084,#259085),(#259086,#259087),(#259088,#259089),(#259090,#259091),
(#259092,#259093),(#259094,#259095),(#259096,#259097),(#259098,#259099),
(#259100,#259101),(#259102,#259103),(#259104,#259105),(#259106,#259107),
(#259108,#259109),(#259110,#259111),(#259112,#259113),(#259114,#259115),
(#259116,#259117),(#259118,#259119),(#259120,#259121),(#259122,#259123),
(#259124,#259125),(#259126,#259127),(#259128,#259129),(#259130,#259131),
(#259132,#259133),(#259134,#259135),(#259136,#259137),(#259138,#259139),
(#259140,#259141),(#259142,#259143),(#259144,#259145),(#259146,#259147),
(#259148,#259149),(#259150,#259151),(#259152,#259153),(#259154,#259155),
(#259156,#259157),(#259158,#259159),(#259160,#259161),(#259162,#259163),
(#259164,#259165),(#259166,#259167),(#259168,#259169),(#259170,#259171),
(#259172,#259173),(#259174,#259175),(#259176,#259177),(#259178,#259179),
(#259180,#259181),(#259182,#259183),(#259184,#259185),(#259186,#259187),
(#259188,#259189),(#259190,#259191),(#259192,#259193),(#259194,#259195),
(#259196,#259197),(#259198,#259199),(#259200,#259201),(#259202,#259203),
(#259204,#259205),(#259206,#259207),(#259208,#259209),(#259210,#259211),
(#259212,#259213),(#259214,#259215),(#259216,#259217),(#259218,#259219),
(#259220,#259221),(#259222,#259223),(#259224,#259225),(#259226,#259227),
(#259228,#259229),(#259230,#259231),(#259232,#259233),(#259234,#259235),
(#259236,#259237),(#259238,#259239),(#259240,#259241),(#259242,#259243),
(#259244,#259245),(#259246,#259247),(#259248,#259249),(#259250,#259251),
(#259252,#259253),(#259254,#259255),(#259256,#259257),(#259258,#259259),
(#259260,#259261),(#259262,#259263),(#259264,#259265),(#259266,#259267),
(#259268,#259269),(#259270,#259271),(#259272,#259273),(#259274,#259275),
(#259276,#259277),(#259278,#259279),(#259280,#259281),(#259282,#259283),
(#259284,#259285),(#259286,#259287),(#259288,#259289),(#259290,#259291),
(#259292,#259293),(#259294,#259295),(#259296,#259297),(#259298,#259299),
(#259300,#259301),(#259302,#259303),(#259304,#259305),(#259306,#259307),
(#259308,#259309),(#259310,#259311),(#259312,#259313),(#259314,#259315),
(#259316,#259317),(#259318,#259319),(#259320,#259321),(#259322,#259323),
(#259324,#259325),(#259326,#259327),(#259328,#259329),(#259330,#259331),
(#259332,#259333),(#259334,#259335),(#259336,#259337),(#259338,#259339),
(#259340,#259341),(#259342,#259343),(#259344,#259345),(#259346,#259347),
(#259348,#259349),(#259350,#259351),(#259352,#259353),(#259354,#259355),
(#259356,#259357),(#259358,#259359),(#259360,#259361),(#259362,#259363),
(#259364,#259365),(#259366,#259367),(#259368,#259369),(#259370,#259371),
(#259372,#259373),(#259374,#259375),(#259376,#259377),(#259378,#259379),
(#259380,#259381),(#259382,#259383),(#259384,#259385),(#259386,#259387),
(#259388,#259389),(#259390,#259391),(#259392,#259393),(#259394,#259395),
(#259396,#259397),(#259398,#259399),(#259400,#259401),(#259402,#259403),
(#259404,#259405),(#259406,#259407),(#259408,#259409),(#259410,#259411),
(#259412,#259413),(#259414,#259415),(#259416,#259417),(#259418,#259419),
(#259420,#259421),(#259422,#259423),(#259424,#259425),(#259426,#259427),
(#259428,#259429),(#259430,#259431),(#259432,#259433),(#259434,#259435),
(#259436,#259437),(#259438,#259439),(#259440,#259441),(#259442,#259443),
(#259444,#259445),(#259446,#259447),(#259448,#259449),(#259450,#259451),
(#259452,#259453),(#259454,#259455),(#259456,#259457),(#259458,#259459),
(#259460,#259461),(#259462,#259463),(#259464,#259465),(#259466,#259467),
(#259468,#259469),(#259470,#259471),(#259472,#259473),(#259474,#259475),
(#259476,#259477),(#259478,#259479),(#259480,#259481),(#259482,#259483),
(#259484,#259485),(#259486,#259487),(#259488,#259489),(#259490,#259491),
(#259492,#259493),(#259494,#259495),(#259496,#259497),(#259498,#259499),
(#259500,#259501),(#259502,#259503),(#259504,#259505),(#259506,#259507),
(#259508,#259509),(#259510,#259511),(#259512,#259513),(#259514,#259515),
(#259516,#259517),(#259518,#259519),(#259520,#259521),(#259522,#259523),
(#259524,#259525),(#259526,#259527),(#259528,#259529),(#259530,#259531),
(#259532,#259533),(#259534,#259535),(#259536,#259537),(#259538,#259539),
(#259540,#259541),(#259542,#259543),(#259544,#259545),(#259546,#259547),
(#259548,#259549),(#259550,#259551),(#259552,#259553),(#259554,#259555),
(#259556,#259557),(#259558,#259559),(#259560,#259561),(#259562,#259563),
(#259564,#259565),(#259566,#259567),(#259568,#259569),(#259570,#259571),
(#259572,#259573),(#259574,#259575),(#259576,#259577),(#259578,#259579),
(#259580,#259581),(#259582,#259583),(#259584,#259585),(#259586,#259587),
(#259588,#259589),(#259590,#259591),(#259592,#259593),(#259594,#259595),
(#259596,#259597),(#259598,#259599),(#259600,#259601),(#259602,#259603),
(#259604,#259605),(#259606,#259607),(#259608,#259609),(#259610,#259611),
(#259612,#259613),(#259614,#259615),(#259616,#259617),(#259618,#259619),
(#259620,#259621),(#259622,#259623),(#259624,#259625),(#259626,#259627),
(#259628,#259629),(#259630,#259631),(#259632,#259633),(#259634,#259635),
(#259636,#259637),(#259638,#259639),(#259640,#259641),(#259642,#259643),
(#259644,#259645),(#259646,#259647),(#259648,#259649),(#259650,#259651),
(#259652,#259653),(#259654,#259655),(#259656,#259657),(#259658,#259659),
(#259660,#259661),(#259662,#259663),(#259664,#259665),(#259666,#259667),
(#259668,#259669),(#259670,#259671),(#259672,#259673),(#259674,#259675),
(#259676,#259677),(#259678,#259679),(#259680,#259681),(#259682,#259683),
(#259684,#259685),(#259686,#259687),(#259688,#259689),(#259690,#259691),
(#259692,#259693),(#259694,#259695),(#259696,#259697),(#259698,#259699),
(#259700,#259701),(#259702,#259703),(#259704,#259705),(#259706,#259707),
(#259708,#259709),(#259710,#259711),(#259712,#259713),(#259714,#259715),
(#259716,#259717),(#259718,#259719),(#259720,#259721),(#259722,#259723),
(#259724,#259725),(#259726,#259727),(#259728,#259729),(#259730,#259731),
(#259732,#259733),(#259734,#259735),(#259736,#259737),(#259738,#259739),
(#259740,#259741),(#259742,#259743),(#259744,#259745),(#259746,#259747),
(#259748,#259749),(#259750,#259751),(#259752,#259753),(#259754,#259755),
(#259756,#259757),(#259758,#259759),(#259760,#259761),(#259762,#259763),
(#259764,#259765),(#259766,#259767),(#259768,#259769),(#259770,#259771),
(#259772,#259773),(#259774,#259775),(#259776,#259777),(#259778,#259779),
(#259780,#259781),(#259782,#259783),(#259784,#259785),(#259786,#259787),
(#259788,#259789),(#259790,#259791),(#259792,#259793),(#259794,#259795),
(#259796,#259797),(#259798,#259799),(#259800,#259801),(#259802,#259803),
(#259804,#259805),(#259806,#259807),(#259808,#259809),(#259810,#259811),
(#259812,#259813),(#259814,#259815),(#259816,#259817),(#259818,#259819),
(#259820,#259821),(#259822,#259823),(#259824,#259825),(#259826,#259827),
(#259828,#259829),(#259830,#259831),(#259832,#259833),(#259834,#259835),
(#259836,#259837),(#259838,#259839),(#259840,#259841),(#259842,#259843),
(#259844,#259845),(#259846,#259847),(#259848,#259849),(#259850,#259851),
(#259852,#259853),(#259854,#259855)),.UNSPECIFIED.,.F.,.F.,.F.,(6,1,1,1,
1,1,1,1,1,1,1,1,1,1,1,1,1,1,1,1,1,1,1,1,1,1,1,1,1,1,1,1,1,1,1,1,1,1,1,1,
1,1,1,1,1,1,1,1,1,1,1,1,1,1,1,1,1,1,1,1,1,1,1,1,1,1,1,1,1,1,1,1,1,1,1,1,
1,1,1,1,1,1,1,1,1,1,1,1,1,1,1,1,1,1,1,1,1,1,1,1,1,1,1,1,1,1,1,1,1,1,1,1,
1,1,1,1,1,1,1,1,1,1,1,1,1,1,1,1,1,1,1,1,1,1,1,1,1,1,1,1,1,1,1,1,1,1,1,1,
1,1,1,1,1,1,1,1,1,1,1,1,1,1,1,1,1,1,1,1,1,1,1,1,1,1,1,1,1,1,1,1,1,1,1,1,
1,1,1,1,1,1,1,1,1,1,1,1,1,1,1,1,1,1,1,1,1,1,1,1,1,1,1,1,1,1,1,1,1,1,1,1,
1,1,1,1,1,1,1,1,1,1,1,1,1,1,1,1,1,1,1,1,1,1,1,1,1,1,1,1,1,1,1,1,1,1,1,1,
1,1,1,1,1,1,1,1,1,1,1,1,1,1,1,1,1,1,1,1,1,1,1,1,1,1,1,1,1,1,1,1,1,1,1,1,
1,1,1,1,1,1,1,1,1,1,1,1,1,1,1,1,1,1,1,1,1,1,1,1,1,1,1,1,1,1,1,1,1,1,1,1,
1,1,1,1,1,1,1,1,1,1,1,1,1,1,1,1,1,1,1,1,1,1,1,1,1,1,1,1,1,1,1,1,1,1,1,1,
1,1,1,1,1,1,1,1,1,1,1,1,1,1,1,1,1,1,1,1,1,1,1,1,1,1,1,1,1,1,1,1,1,1,1,1,
1,1,1,1,1,1,1,1,1,1,1,1,1,1,1,1,1,1,1,1,1,1,1,1,1,1,1,1,1,1,1,1,1,1,1,1,
1,1,1,1,1,1,1,1,1,1,1,1,1,1,1,1,1,1,1,1,1,1,1,1,1,1,1,1,1,1,1,6),(2,2),
(0.143172104,0.144954128,0.146788991,0.148623853,0.150458716,0.152293578,
0.15412844,0.155963303,0.157798165,0.159633028,0.16146789,0.163302752,0.165137615,
0.166972477,0.168807339,0.170642202,0.172477064,0.174311927,0.176146789,
0.177981651,0.179816514,0.181651376,0.183486239,0.185321101,0.187155963,
0.188990826,0.190825688,0.19266055,0.194495413,0.196330275,0.198165138,
0.2,0.201834862,0.203669725,0.205504587,0.20733945,0.209174312,0.211009174,
0.212844037,0.214678899,0.216513761,0.218348624,0.220183486,0.222018349,
0.223853211,0.225688073,0.227522936,0.229357798,0.231192661,0.233027523,
0.234862385,0.236697248,0.23853211,0.240366972,0.242201835,0.244036697,
0.24587156,0.247706422,0.249541284,0.251376147,0.253211009,0.255045872,
0.256880734,0.258715596,0.260550459,0.262385321,0.264220183,0.266055046,
0.267889908,0.269724771,0.271559633,0.273394495,0.275229358,0.27706422,
0.278899083,0.280733945,0.282568807,0.28440367,0.286238532,0.288073394,
0.289908257,0.291743119,0.293577982,0.295412844,0.297247706,0.299082569,
0.300917431,0.302752294,0.304587156,0.306422018,0.308256881,0.310091743,
0.311926606,0.313761468,0.31559633,0.317431193,0.319266055,0.321100917,
0.32293578,0.324770642,0.326605505,0.328440367,0.330275229,0.332110092,
0.333944954,0.335779817,0.337614679,0.339449541,0.341284404,0.343119266,
0.344954128,0.346788991,0.348623853,0.350458716,0.352293578,0.35412844,
0.355963303,0.357798165,0.359633028,0.36146789,0.363302752,0.365137615,
0.366972477,0.368807339,0.370642202,0.372477064,0.374311927,0.376146789,
0.377981651,0.379816514,0.381651376,0.383486239,0.385321101,0.387155963,
0.388990826,0.390825688,0.39266055,0.394495413,0.396330275,0.398165138,
0.4,0.401834862,0.403669725,0.405504587,0.40733945,0.409174312,0.411009174,
0.412844037,0.414678899,0.416513761,0.418348624,0.420183486,0.422018349,
0.423853211,0.425688073,0.427522936,0.429357798,0.431192661,0.433027523,
0.434862385,0.436697248,0.43853211,0.440366972,0.442201835,0.444036697,
0.44587156,0.447706422,0.449541284,0.451376147,0.453211009,0.455045872,
0.456880734,0.458715596,0.460550459,0.462385321,0.464220183,0.466055046,
0.467889908,0.469724771,0.471559633,0.473394495,0.475229358,0.47706422,
0.478899083,0.480733945,0.482568807,0.48440367,0.486238532,0.488073394,
0.489908257,0.491743119,0.493577982,0.495412844,0.497247706,0.499082569,
0.500917431,0.502752294,0.504587156,0.506422018,0.508256881,0.510091743,
0.511926606,0.513761468,0.51559633,0.517431193,0.519266055,0.521100917,
0.52293578,0.524770642,0.526605505,0.528440367,0.530275229,0.532110092,
0.533944954,0.535779817,0.537614679,0.539449541,0.541284404,0.543119266,
0.544954128,0.546788991,0.548623853,0.550458716,0.552293578,0.55412844,
0.555963303,0.557798165,0.559633028,0.56146789,0.563302752,0.565137615,
0.566972477,0.568807339,0.570642202,0.572477064,0.574311927,0.576146789,
0.577981651,0.579816514,0.581651376,0.583486239,0.585321101,0.587155963,
0.588990826,0.590825688,0.59266055,0.594495413,0.596330275,0.598165138,
0.6,0.601834862,0.603669725,0.605504587,0.60733945,0.609174312,0.611009174,
0.612844037,0.614678899,0.616513761,0.618348624,0.620183486,0.622018349,
0.623853211,0.625688073,0.627522936,0.629357798,0.631192661,0.633027523,
0.634862385,0.636697248,0.63853211,0.640366972,0.642201835,0.644036697,
0.64587156,0.647706422,0.649541284,0.651376147,0.653211009,0.655045872,
0.656880734,0.658715596,0.660550459,0.662385321,0.664220183,0.666055046,
0.667889908,0.669724771,0.671559633,0.673394495,0.675229358,0.67706422,
0.678899083,0.680733945,0.682568807,0.68440367,0.686238532,0.688073394,
0.689908257,0.691743119,0.693577982,0.695412844,0.697247706,0.699082569,
0.700917431,0.702752294,0.704587156,0.706422018,0.708256881,0.710091743,
0.711926606,0.713761468,0.71559633,0.717431193,0.719266055,0.721100917,
0.72293578,0.724770642,0.726605505,0.728440367,0.730275229,0.732110092,
0.733944954,0.735779817,0.737614679,0.739449541,0.741284404,0.743119266,
0.744954128,0.746788991,0.748623853,0.750458716,0.752293578,0.75412844,
0.755963303,0.757798165,0.759633028,0.76146789,0.763302752,0.765137615,
0.766972477,0.768807339,0.770642202,0.772477064,0.774311927,0.776146789,
0.777981651,0.779816514,0.781651376,0.783486239,0.785321101,0.787155963,
0.788990826,0.790825688,0.79266055,0.794495413,0.796330275,0.798165138,
0.8,0.801834862,0.803669725,0.805504587,0.80733945,0.809174312,0.811009174,
0.812844037,0.814678899,0.816513761,0.818348624,0.820183486,0.822018349,
0.823853211,0.825688073,0.827522936,0.829357798,0.831192661,0.833027523,
0.834862385,0.836697248,0.83853211,0.840366972,0.842201835,0.844036697,
0.84587156,0.847706422,0.849541284,0.851376147,0.853211009,0.855045872,
0.856880734,0.858715596,0.860550459,0.862385321,0.864220183,0.866055046,
0.867889908,0.869724771,0.871559633,0.873394495,0.875229358,0.87706422,
0.878899083,0.880733945,0.882568807,0.88440367,0.886238532,0.888073394,
0.889908257,0.891743119,0.893577982,0.895412844,0.897247706,0.899082569,
0.900917431,0.902752294,0.904587156,0.906422018,0.908256881,0.910091743,
0.911926606,0.913761468,0.91559633,0.917431193,0.919266055,0.921100917,
0.92293578,0.924770642,0.926605505,0.928440367,0.930275229,0.932110092,
0.933944954,0.935779817,0.937614679,0.939449541,0.941284404,0.943119266,
0.944954128,0.946788991,0.948623853,0.950458716,0.952293578,0.95412844,
0.955963303,0.957798165,0.959633028,0.96146789,0.963302752,0.965137615,
0.966972477,0.968807339,0.970642202,0.972477064,0.974311927,0.976146789,
0.977981651,0.979816514,0.981651376,0.983486239,0.985321101,0.987155963,
0.988990826,0.990825688,0.99266055,0.994495413,0.996330275,0.998165138,
1.),(0.,0.36),.UNSPECIFIED.);
#6280=B_SPLINE_SURFACE_WITH_KNOTS('',5,1,((#260798,#260799),(#260800,#260801),
(#260802,#260803),(#260804,#260805),(#260806,#260807),(#260808,#260809),
(#260810,#260811),(#260812,#260813),(#260814,#260815),(#260816,#260817),
(#260818,#260819),(#260820,#260821),(#260822,#260823),(#260824,#260825),
(#260826,#260827),(#260828,#260829),(#260830,#260831),(#260832,#260833),
(#260834,#260835),(#260836,#260837),(#260838,#260839),(#260840,#260841),
(#260842,#260843),(#260844,#260845),(#260846,#260847),(#260848,#260849),
(#260850,#260851),(#260852,#260853),(#260854,#260855),(#260856,#260857),
(#260858,#260859),(#260860,#260861),(#260862,#260863),(#260864,#260865),
(#260866,#260867),(#260868,#260869),(#260870,#260871),(#260872,#260873),
(#260874,#260875),(#260876,#260877),(#260878,#260879),(#260880,#260881),
(#260882,#260883),(#260884,#260885),(#260886,#260887),(#260888,#260889),
(#260890,#260891),(#260892,#260893),(#260894,#260895),(#260896,#260897),
(#260898,#260899),(#260900,#260901),(#260902,#260903),(#260904,#260905),
(#260906,#260907),(#260908,#260909),(#260910,#260911),(#260912,#260913),
(#260914,#260915),(#260916,#260917),(#260918,#260919),(#260920,#260921),
(#260922,#260923),(#260924,#260925),(#260926,#260927),(#260928,#260929),
(#260930,#260931),(#260932,#260933),(#260934,#260935),(#260936,#260937),
(#260938,#260939),(#260940,#260941),(#260942,#260943),(#260944,#260945),
(#260946,#260947),(#260948,#260949),(#260950,#260951),(#260952,#260953),
(#260954,#260955),(#260956,#260957),(#260958,#260959),(#260960,#260961),
(#260962,#260963),(#260964,#260965),(#260966,#260967),(#260968,#260969),
(#260970,#260971),(#260972,#260973),(#260974,#260975),(#260976,#260977),
(#260978,#260979),(#260980,#260981),(#260982,#260983),(#260984,#260985),
(#260986,#260987),(#260988,#260989),(#260990,#260991),(#260992,#260993),
(#260994,#260995),(#260996,#260997),(#260998,#260999),(#261000,#261001),
(#261002,#261003),(#261004,#261005),(#261006,#261007),(#261008,#261009),
(#261010,#261011),(#261012,#261013),(#261014,#261015),(#261016,#261017),
(#261018,#261019),(#261020,#261021),(#261022,#261023),(#261024,#261025),
(#261026,#261027),(#261028,#261029),(#261030,#261031),(#261032,#261033),
(#261034,#261035),(#261036,#261037),(#261038,#261039),(#261040,#261041),
(#261042,#261043),(#261044,#261045),(#261046,#261047),(#261048,#261049),
(#261050,#261051),(#261052,#261053),(#261054,#261055),(#261056,#261057),
(#261058,#261059),(#261060,#261061),(#261062,#261063),(#261064,#261065),
(#261066,#261067),(#261068,#261069),(#261070,#261071),(#261072,#261073),
(#261074,#261075),(#261076,#261077),(#261078,#261079),(#261080,#261081),
(#261082,#261083),(#261084,#261085),(#261086,#261087),(#261088,#261089),
(#261090,#261091),(#261092,#261093),(#261094,#261095),(#261096,#261097),
(#261098,#261099),(#261100,#261101),(#261102,#261103),(#261104,#261105),
(#261106,#261107),(#261108,#261109),(#261110,#261111),(#261112,#261113),
(#261114,#261115),(#261116,#261117),(#261118,#261119),(#261120,#261121),
(#261122,#261123),(#261124,#261125),(#261126,#261127),(#261128,#261129),
(#261130,#261131),(#261132,#261133),(#261134,#261135),(#261136,#261137),
(#261138,#261139),(#261140,#261141),(#261142,#261143),(#261144,#261145),
(#261146,#261147),(#261148,#261149),(#261150,#261151),(#261152,#261153),
(#261154,#261155),(#261156,#261157),(#261158,#261159),(#261160,#261161),
(#261162,#261163),(#261164,#261165),(#261166,#261167),(#261168,#261169),
(#261170,#261171),(#261172,#261173),(#261174,#261175),(#261176,#261177),
(#261178,#261179),(#261180,#261181),(#261182,#261183),(#261184,#261185),
(#261186,#261187),(#261188,#261189),(#261190,#261191),(#261192,#261193),
(#261194,#261195),(#261196,#261197),(#261198,#261199),(#261200,#261201),
(#261202,#261203),(#261204,#261205),(#261206,#261207),(#261208,#261209),
(#261210,#261211),(#261212,#261213),(#261214,#261215),(#261216,#261217),
(#261218,#261219),(#261220,#261221),(#261222,#261223),(#261224,#261225),
(#261226,#261227),(#261228,#261229),(#261230,#261231),(#261232,#261233),
(#261234,#261235),(#261236,#261237),(#261238,#261239),(#261240,#261241),
(#261242,#261243),(#261244,#261245),(#261246,#261247),(#261248,#261249),
(#261250,#261251),(#261252,#261253),(#261254,#261255),(#261256,#261257),
(#261258,#261259),(#261260,#261261),(#261262,#261263),(#261264,#261265),
(#261266,#261267),(#261268,#261269),(#261270,#261271),(#261272,#261273),
(#261274,#261275),(#261276,#261277),(#261278,#261279),(#261280,#261281),
(#261282,#261283),(#261284,#261285),(#261286,#261287),(#261288,#261289),
(#261290,#261291),(#261292,#261293),(#261294,#261295),(#261296,#261297),
(#261298,#261299),(#261300,#261301),(#261302,#261303),(#261304,#261305),
(#261306,#261307),(#261308,#261309),(#261310,#261311),(#261312,#261313),
(#261314,#261315),(#261316,#261317),(#261318,#261319),(#261320,#261321),
(#261322,#261323),(#261324,#261325),(#261326,#261327),(#261328,#261329),
(#261330,#261331),(#261332,#261333),(#261334,#261335),(#261336,#261337),
(#261338,#261339),(#261340,#261341),(#261342,#261343),(#261344,#261345),
(#261346,#261347),(#261348,#261349),(#261350,#261351),(#261352,#261353),
(#261354,#261355),(#261356,#261357),(#261358,#261359),(#261360,#261361),
(#261362,#261363),(#261364,#261365),(#261366,#261367),(#261368,#261369),
(#261370,#261371),(#261372,#261373),(#261374,#261375),(#261376,#261377),
(#261378,#261379),(#261380,#261381),(#261382,#261383),(#261384,#261385),
(#261386,#261387),(#261388,#261389),(#261390,#261391),(#261392,#261393),
(#261394,#261395),(#261396,#261397),(#261398,#261399),(#261400,#261401),
(#261402,#261403),(#261404,#261405),(#261406,#261407),(#261408,#261409),
(#261410,#261411),(#261412,#261413),(#261414,#261415),(#261416,#261417),
(#261418,#261419),(#261420,#261421),(#261422,#261423),(#261424,#261425),
(#261426,#261427),(#261428,#261429),(#261430,#261431),(#261432,#261433),
(#261434,#261435),(#261436,#261437),(#261438,#261439),(#261440,#261441),
(#261442,#261443),(#261444,#261445),(#261446,#261447),(#261448,#261449),
(#261450,#261451),(#261452,#261453),(#261454,#261455),(#261456,#261457),
(#261458,#261459),(#261460,#261461),(#261462,#261463),(#261464,#261465),
(#261466,#261467),(#261468,#261469),(#261470,#261471),(#261472,#261473),
(#261474,#261475),(#261476,#261477),(#261478,#261479),(#261480,#261481),
(#261482,#261483),(#261484,#261485),(#261486,#261487),(#261488,#261489),
(#261490,#261491),(#261492,#261493),(#261494,#261495),(#261496,#261497),
(#261498,#261499),(#261500,#261501),(#261502,#261503),(#261504,#261505),
(#261506,#261507),(#261508,#261509),(#261510,#261511),(#261512,#261513),
(#261514,#261515),(#261516,#261517),(#261518,#261519),(#261520,#261521),
(#261522,#261523),(#261524,#261525),(#261526,#261527),(#261528,#261529),
(#261530,#261531),(#261532,#261533),(#261534,#261535),(#261536,#261537),
(#261538,#261539),(#261540,#261541),(#261542,#261543),(#261544,#261545),
(#261546,#261547),(#261548,#261549),(#261550,#261551),(#261552,#261553),
(#261554,#261555),(#261556,#261557),(#261558,#261559),(#261560,#261561),
(#261562,#261563),(#261564,#261565),(#261566,#261567),(#261568,#261569),
(#261570,#261571),(#261572,#261573),(#261574,#261575),(#261576,#261577),
(#261578,#261579),(#261580,#261581),(#261582,#261583),(#261584,#261585),
(#261586,#261587),(#261588,#261589),(#261590,#261591),(#261592,#261593),
(#261594,#261595),(#261596,#261597),(#261598,#261599),(#261600,#261601),
(#261602,#261603),(#261604,#261605),(#261606,#261607),(#261608,#261609),
(#261610,#261611),(#261612,#261613),(#261614,#261615),(#261616,#261617),
(#261618,#261619),(#261620,#261621),(#261622,#261623),(#261624,#261625),
(#261626,#261627),(#261628,#261629),(#261630,#261631),(#261632,#261633),
(#261634,#261635),(#261636,#261637),(#261638,#261639),(#261640,#261641),
(#261642,#261643),(#261644,#261645),(#261646,#261647),(#261648,#261649),
(#261650,#261651),(#261652,#261653),(#261654,#261655),(#261656,#261657),
(#261658,#261659),(#261660,#261661),(#261662,#261663),(#261664,#261665),
(#261666,#261667),(#261668,#261669),(#261670,#261671),(#261672,#261673),
(#261674,#261675),(#261676,#261677),(#261678,#261679),(#261680,#261681),
(#261682,#261683),(#261684,#261685),(#261686,#261687),(#261688,#261689),
(#261690,#261691),(#261692,#261693),(#261694,#261695),(#261696,#261697),
(#261698,#261699),(#261700,#261701),(#261702,#261703),(#261704,#261705),
(#261706,#261707),(#261708,#261709),(#261710,#261711),(#261712,#261713),
(#261714,#261715),(#261716,#261717),(#261718,#261719),(#261720,#261721),
(#261722,#261723),(#261724,#261725),(#261726,#261727),(#261728,#261729),
(#261730,#261731),(#261732,#261733),(#261734,#261735),(#261736,#261737),
(#261738,#261739),(#261740,#261741)),.UNSPECIFIED.,.F.,.F.,.F.,(6,1,1,1,
1,1,1,1,1,1,1,1,1,1,1,1,1,1,1,1,1,1,1,1,1,1,1,1,1,1,1,1,1,1,1,1,1,1,1,1,
1,1,1,1,1,1,1,1,1,1,1,1,1,1,1,1,1,1,1,1,1,1,1,1,1,1,1,1,1,1,1,1,1,1,1,1,
1,1,1,1,1,1,1,1,1,1,1,1,1,1,1,1,1,1,1,1,1,1,1,1,1,1,1,1,1,1,1,1,1,1,1,1,
1,1,1,1,1,1,1,1,1,1,1,1,1,1,1,1,1,1,1,1,1,1,1,1,1,1,1,1,1,1,1,1,1,1,1,1,
1,1,1,1,1,1,1,1,1,1,1,1,1,1,1,1,1,1,1,1,1,1,1,1,1,1,1,1,1,1,1,1,1,1,1,1,
1,1,1,1,1,1,1,1,1,1,1,1,1,1,1,1,1,1,1,1,1,1,1,1,1,1,1,1,1,1,1,1,1,1,1,1,
1,1,1,1,1,1,1,1,1,1,1,1,1,1,1,1,1,1,1,1,1,1,1,1,1,1,1,1,1,1,1,1,1,1,1,1,
1,1,1,1,1,1,1,1,1,1,1,1,1,1,1,1,1,1,1,1,1,1,1,1,1,1,1,1,1,1,1,1,1,1,1,1,
1,1,1,1,1,1,1,1,1,1,1,1,1,1,1,1,1,1,1,1,1,1,1,1,1,1,1,1,1,1,1,1,1,1,1,1,
1,1,1,1,1,1,1,1,1,1,1,1,1,1,1,1,1,1,1,1,1,1,1,1,1,1,1,1,1,1,1,1,1,1,1,1,
1,1,1,1,1,1,1,1,1,1,1,1,1,1,1,1,1,1,1,1,1,1,1,1,1,1,1,1,1,1,1,1,1,1,1,1,
1,1,1,1,1,1,1,1,1,1,1,1,1,1,1,1,1,1,1,1,1,1,1,1,1,1,1,1,1,1,1,1,1,1,1,1,
1,1,1,1,1,1,1,1,1,1,1,1,1,1,1,1,1,1,1,1,1,1,1,1,1,1,1,1,1,1,1,6),(2,2),
(-1.,-0.998165138,-0.996330275,-0.994495413,-0.99266055,-0.990825688,-0.988990826,
-0.987155963,-0.985321101,-0.983486239,-0.981651376,-0.979816514,-0.977981651,
-0.976146789,-0.974311927,-0.972477064,-0.970642202,-0.968807339,-0.966972477,
-0.965137615,-0.963302752,-0.96146789,-0.959633028,-0.957798165,-0.955963303,
-0.95412844,-0.952293578,-0.950458716,-0.948623853,-0.946788991,-0.944954128,
-0.943119266,-0.941284404,-0.939449541,-0.937614679,-0.935779817,-0.933944954,
-0.932110092,-0.930275229,-0.928440367,-0.926605505,-0.924770642,-0.92293578,
-0.921100917,-0.919266055,-0.917431193,-0.91559633,-0.913761468,-0.911926606,
-0.910091743,-0.908256881,-0.906422018,-0.904587156,-0.902752294,-0.900917431,
-0.899082569,-0.897247706,-0.895412844,-0.893577982,-0.891743119,-0.889908257,
-0.888073394,-0.886238532,-0.88440367,-0.882568807,-0.880733945,-0.878899083,
-0.87706422,-0.875229358,-0.873394495,-0.871559633,-0.869724771,-0.867889908,
-0.866055046,-0.864220183,-0.862385321,-0.860550459,-0.858715596,-0.856880734,
-0.855045872,-0.853211009,-0.851376147,-0.849541284,-0.847706422,-0.84587156,
-0.844036697,-0.842201835,-0.840366972,-0.83853211,-0.836697248,-0.834862385,
-0.833027523,-0.831192661,-0.829357798,-0.827522936,-0.825688073,-0.823853211,
-0.822018349,-0.820183486,-0.818348624,-0.816513761,-0.814678899,-0.812844037,
-0.811009174,-0.809174312,-0.80733945,-0.805504587,-0.803669725,-0.801834862,
-0.8,-0.798165138,-0.796330275,-0.794495413,-0.79266055,-0.790825688,-0.788990826,
-0.787155963,-0.785321101,-0.783486239,-0.781651376,-0.779816514,-0.777981651,
-0.776146789,-0.774311927,-0.772477064,-0.770642202,-0.768807339,-0.766972477,
-0.765137615,-0.763302752,-0.76146789,-0.759633028,-0.757798165,-0.755963303,
-0.75412844,-0.752293578,-0.750458716,-0.748623853,-0.746788991,-0.744954128,
-0.743119266,-0.741284404,-0.739449541,-0.737614679,-0.735779817,-0.733944954,
-0.732110092,-0.730275229,-0.728440367,-0.726605505,-0.724770642,-0.72293578,
-0.721100917,-0.719266055,-0.717431193,-0.71559633,-0.713761468,-0.711926606,
-0.710091743,-0.708256881,-0.706422018,-0.704587156,-0.702752294,-0.700917431,
-0.699082569,-0.697247706,-0.695412844,-0.693577982,-0.691743119,-0.689908257,
-0.688073394,-0.686238532,-0.68440367,-0.682568807,-0.680733945,-0.678899083,
-0.67706422,-0.675229358,-0.673394495,-0.671559633,-0.669724771,-0.667889908,
-0.666055046,-0.664220183,-0.662385321,-0.660550459,-0.658715596,-0.656880734,
-0.655045872,-0.653211009,-0.651376147,-0.649541284,-0.647706422,-0.64587156,
-0.644036697,-0.642201835,-0.640366972,-0.63853211,-0.636697248,-0.634862385,
-0.633027523,-0.631192661,-0.629357798,-0.627522936,-0.625688073,-0.623853211,
-0.622018349,-0.620183486,-0.618348624,-0.616513761,-0.614678899,-0.612844037,
-0.611009174,-0.609174312,-0.60733945,-0.605504587,-0.603669725,-0.601834862,
-0.6,-0.598165138,-0.596330275,-0.594495413,-0.59266055,-0.590825688,-0.588990826,
-0.587155963,-0.585321101,-0.583486239,-0.581651376,-0.579816514,-0.577981651,
-0.576146789,-0.574311927,-0.572477064,-0.570642202,-0.568807339,-0.566972477,
-0.565137615,-0.563302752,-0.56146789,-0.559633028,-0.557798165,-0.555963303,
-0.55412844,-0.552293578,-0.550458716,-0.548623853,-0.546788991,-0.544954128,
-0.543119266,-0.541284404,-0.539449541,-0.537614679,-0.535779817,-0.533944954,
-0.532110092,-0.530275229,-0.528440367,-0.526605505,-0.524770642,-0.52293578,
-0.521100917,-0.519266055,-0.517431193,-0.51559633,-0.513761468,-0.511926606,
-0.510091743,-0.508256881,-0.506422018,-0.504587156,-0.502752294,-0.500917431,
-0.499082569,-0.497247706,-0.495412844,-0.493577982,-0.491743119,-0.489908257,
-0.488073394,-0.486238532,-0.48440367,-0.482568807,-0.480733945,-0.478899083,
-0.47706422,-0.475229358,-0.473394495,-0.471559633,-0.469724771,-0.467889908,
-0.466055046,-0.464220183,-0.462385321,-0.460550459,-0.458715596,-0.456880734,
-0.455045872,-0.453211009,-0.451376147,-0.449541284,-0.447706422,-0.44587156,
-0.444036697,-0.442201835,-0.440366972,-0.43853211,-0.436697248,-0.434862385,
-0.433027523,-0.431192661,-0.429357798,-0.427522936,-0.425688073,-0.423853211,
-0.422018349,-0.420183486,-0.418348624,-0.416513761,-0.414678899,-0.412844037,
-0.411009174,-0.409174312,-0.40733945,-0.405504587,-0.403669725,-0.401834862,
-0.4,-0.398165138,-0.396330275,-0.394495413,-0.39266055,-0.390825688,-0.388990826,
-0.387155963,-0.385321101,-0.383486239,-0.381651376,-0.379816514,-0.377981651,
-0.376146789,-0.374311927,-0.372477064,-0.370642202,-0.368807339,-0.366972477,
-0.365137615,-0.363302752,-0.36146789,-0.359633028,-0.357798165,-0.355963303,
-0.35412844,-0.352293578,-0.350458716,-0.348623853,-0.346788991,-0.344954128,
-0.343119266,-0.341284404,-0.339449541,-0.337614679,-0.335779817,-0.333944954,
-0.332110092,-0.330275229,-0.328440367,-0.326605505,-0.324770642,-0.32293578,
-0.321100917,-0.319266055,-0.317431193,-0.31559633,-0.313761468,-0.311926606,
-0.310091743,-0.308256881,-0.306422018,-0.304587156,-0.302752294,-0.300917431,
-0.299082569,-0.297247706,-0.295412844,-0.293577982,-0.291743119,-0.289908257,
-0.288073394,-0.286238532,-0.28440367,-0.282568807,-0.280733945,-0.278899083,
-0.27706422,-0.275229358,-0.273394495,-0.271559633,-0.269724771,-0.267889908,
-0.266055046,-0.264220183,-0.262385321,-0.260550459,-0.258715596,-0.256880734,
-0.255045872,-0.253211009,-0.251376147,-0.249541284,-0.247706422,-0.24587156,
-0.244036697,-0.242201835,-0.240366972,-0.23853211,-0.236697248,-0.234862385,
-0.233027523,-0.231192661,-0.229357798,-0.227522936,-0.225688073,-0.223853211,
-0.222018349,-0.220183486,-0.218348624,-0.216513761,-0.214678899,-0.212844037,
-0.211009174,-0.209174312,-0.20733945,-0.205504587,-0.203669725,-0.201834862,
-0.2,-0.198165138,-0.196330275,-0.194495413,-0.19266055,-0.190825688,-0.188990826,
-0.187155963,-0.185321101,-0.183486239,-0.181651376,-0.179816514,-0.177981651,
-0.176146789,-0.174311927,-0.172477064,-0.170642202,-0.168807339,-0.166972477,
-0.165137615,-0.163302752,-0.16146789,-0.159633028,-0.157798165,-0.155963303,
-0.15412844,-0.152293578,-0.150458716,-0.148623853,-0.146788991,-0.144954128,
-0.143172103),(0.,0.36),.UNSPECIFIED.);
#6281=B_SPLINE_SURFACE_WITH_KNOTS('',5,1,((#262704,#262705),(#262706,#262707),
(#262708,#262709),(#262710,#262711),(#262712,#262713),(#262714,#262715),
(#262716,#262717),(#262718,#262719),(#262720,#262721),(#262722,#262723),
(#262724,#262725),(#262726,#262727),(#262728,#262729),(#262730,#262731),
(#262732,#262733),(#262734,#262735),(#262736,#262737),(#262738,#262739),
(#262740,#262741),(#262742,#262743),(#262744,#262745),(#262746,#262747),
(#262748,#262749),(#262750,#262751),(#262752,#262753),(#262754,#262755),
(#262756,#262757),(#262758,#262759),(#262760,#262761),(#262762,#262763),
(#262764,#262765),(#262766,#262767),(#262768,#262769),(#262770,#262771),
(#262772,#262773),(#262774,#262775),(#262776,#262777),(#262778,#262779),
(#262780,#262781),(#262782,#262783),(#262784,#262785),(#262786,#262787),
(#262788,#262789),(#262790,#262791),(#262792,#262793),(#262794,#262795),
(#262796,#262797),(#262798,#262799),(#262800,#262801),(#262802,#262803),
(#262804,#262805),(#262806,#262807),(#262808,#262809),(#262810,#262811),
(#262812,#262813),(#262814,#262815),(#262816,#262817),(#262818,#262819),
(#262820,#262821),(#262822,#262823),(#262824,#262825),(#262826,#262827),
(#262828,#262829),(#262830,#262831),(#262832,#262833),(#262834,#262835),
(#262836,#262837),(#262838,#262839),(#262840,#262841),(#262842,#262843),
(#262844,#262845),(#262846,#262847),(#262848,#262849),(#262850,#262851),
(#262852,#262853),(#262854,#262855),(#262856,#262857),(#262858,#262859),
(#262860,#262861),(#262862,#262863),(#262864,#262865),(#262866,#262867),
(#262868,#262869),(#262870,#262871),(#262872,#262873),(#262874,#262875),
(#262876,#262877),(#262878,#262879),(#262880,#262881),(#262882,#262883),
(#262884,#262885),(#262886,#262887),(#262888,#262889),(#262890,#262891),
(#262892,#262893),(#262894,#262895),(#262896,#262897),(#262898,#262899),
(#262900,#262901),(#262902,#262903),(#262904,#262905),(#262906,#262907),
(#262908,#262909),(#262910,#262911),(#262912,#262913),(#262914,#262915),
(#262916,#262917),(#262918,#262919),(#262920,#262921),(#262922,#262923),
(#262924,#262925),(#262926,#262927),(#262928,#262929),(#262930,#262931),
(#262932,#262933),(#262934,#262935),(#262936,#262937),(#262938,#262939),
(#262940,#262941),(#262942,#262943),(#262944,#262945),(#262946,#262947),
(#262948,#262949),(#262950,#262951),(#262952,#262953),(#262954,#262955),
(#262956,#262957),(#262958,#262959),(#262960,#262961),(#262962,#262963),
(#262964,#262965),(#262966,#262967),(#262968,#262969),(#262970,#262971),
(#262972,#262973),(#262974,#262975),(#262976,#262977),(#262978,#262979),
(#262980,#262981),(#262982,#262983),(#262984,#262985),(#262986,#262987),
(#262988,#262989),(#262990,#262991),(#262992,#262993),(#262994,#262995),
(#262996,#262997),(#262998,#262999),(#263000,#263001),(#263002,#263003),
(#263004,#263005),(#263006,#263007),(#263008,#263009),(#263010,#263011),
(#263012,#263013),(#263014,#263015),(#263016,#263017),(#263018,#263019),
(#263020,#263021),(#263022,#263023),(#263024,#263025),(#263026,#263027),
(#263028,#263029),(#263030,#263031),(#263032,#263033),(#263034,#263035),
(#263036,#263037),(#263038,#263039),(#263040,#263041),(#263042,#263043),
(#263044,#263045),(#263046,#263047),(#263048,#263049),(#263050,#263051),
(#263052,#263053),(#263054,#263055),(#263056,#263057),(#263058,#263059),
(#263060,#263061),(#263062,#263063),(#263064,#263065),(#263066,#263067),
(#263068,#263069),(#263070,#263071),(#263072,#263073),(#263074,#263075),
(#263076,#263077),(#263078,#263079),(#263080,#263081),(#263082,#263083),
(#263084,#263085),(#263086,#263087),(#263088,#263089),(#263090,#263091),
(#263092,#263093),(#263094,#263095),(#263096,#263097),(#263098,#263099),
(#263100,#263101),(#263102,#263103),(#263104,#263105),(#263106,#263107),
(#263108,#263109),(#263110,#263111),(#263112,#263113),(#263114,#263115),
(#263116,#263117),(#263118,#263119),(#263120,#263121),(#263122,#263123),
(#263124,#263125),(#263126,#263127),(#263128,#263129),(#263130,#263131),
(#263132,#263133),(#263134,#263135),(#263136,#263137),(#263138,#263139),
(#263140,#263141),(#263142,#263143),(#263144,#263145),(#263146,#263147),
(#263148,#263149),(#263150,#263151),(#263152,#263153),(#263154,#263155),
(#263156,#263157),(#263158,#263159),(#263160,#263161),(#263162,#263163),
(#263164,#263165),(#263166,#263167),(#263168,#263169),(#263170,#263171),
(#263172,#263173),(#263174,#263175),(#263176,#263177),(#263178,#263179),
(#263180,#263181),(#263182,#263183),(#263184,#263185),(#263186,#263187),
(#263188,#263189),(#263190,#263191),(#263192,#263193),(#263194,#263195),
(#263196,#263197),(#263198,#263199),(#263200,#263201),(#263202,#263203),
(#263204,#263205),(#263206,#263207),(#263208,#263209),(#263210,#263211),
(#263212,#263213),(#263214,#263215),(#263216,#263217),(#263218,#263219),
(#263220,#263221),(#263222,#263223),(#263224,#263225),(#263226,#263227),
(#263228,#263229),(#263230,#263231),(#263232,#263233),(#263234,#263235),
(#263236,#263237),(#263238,#263239),(#263240,#263241),(#263242,#263243),
(#263244,#263245),(#263246,#263247),(#263248,#263249),(#263250,#263251),
(#263252,#263253),(#263254,#263255),(#263256,#263257),(#263258,#263259),
(#263260,#263261),(#263262,#263263),(#263264,#263265),(#263266,#263267),
(#263268,#263269),(#263270,#263271),(#263272,#263273),(#263274,#263275),
(#263276,#263277),(#263278,#263279),(#263280,#263281),(#263282,#263283),
(#263284,#263285),(#263286,#263287),(#263288,#263289),(#263290,#263291),
(#263292,#263293),(#263294,#263295),(#263296,#263297),(#263298,#263299),
(#263300,#263301),(#263302,#263303),(#263304,#263305),(#263306,#263307),
(#263308,#263309),(#263310,#263311),(#263312,#263313),(#263314,#263315),
(#263316,#263317),(#263318,#263319),(#263320,#263321),(#263322,#263323),
(#263324,#263325),(#263326,#263327),(#263328,#263329),(#263330,#263331),
(#263332,#263333),(#263334,#263335),(#263336,#263337),(#263338,#263339),
(#263340,#263341),(#263342,#263343),(#263344,#263345),(#263346,#263347),
(#263348,#263349),(#263350,#263351),(#263352,#263353),(#263354,#263355),
(#263356,#263357),(#263358,#263359),(#263360,#263361),(#263362,#263363),
(#263364,#263365),(#263366,#263367),(#263368,#263369),(#263370,#263371),
(#263372,#263373),(#263374,#263375),(#263376,#263377),(#263378,#263379),
(#263380,#263381),(#263382,#263383),(#263384,#263385),(#263386,#263387),
(#263388,#263389),(#263390,#263391),(#263392,#263393),(#263394,#263395),
(#263396,#263397),(#263398,#263399),(#263400,#263401),(#263402,#263403),
(#263404,#263405),(#263406,#263407),(#263408,#263409),(#263410,#263411),
(#263412,#263413),(#263414,#263415),(#263416,#263417),(#263418,#263419),
(#263420,#263421),(#263422,#263423),(#263424,#263425),(#263426,#263427),
(#263428,#263429),(#263430,#263431),(#263432,#263433),(#263434,#263435),
(#263436,#263437),(#263438,#263439),(#263440,#263441),(#263442,#263443),
(#263444,#263445),(#263446,#263447),(#263448,#263449),(#263450,#263451),
(#263452,#263453),(#263454,#263455),(#263456,#263457),(#263458,#263459),
(#263460,#263461),(#263462,#263463),(#263464,#263465),(#263466,#263467),
(#263468,#263469),(#263470,#263471),(#263472,#263473),(#263474,#263475),
(#263476,#263477),(#263478,#263479),(#263480,#263481),(#263482,#263483),
(#263484,#263485),(#263486,#263487),(#263488,#263489),(#263490,#263491),
(#263492,#263493),(#263494,#263495),(#263496,#263497),(#263498,#263499),
(#263500,#263501),(#263502,#263503),(#263504,#263505),(#263506,#263507),
(#263508,#263509),(#263510,#263511),(#263512,#263513),(#263514,#263515),
(#263516,#263517),(#263518,#263519),(#263520,#263521),(#263522,#263523),
(#263524,#263525),(#263526,#263527),(#263528,#263529),(#263530,#263531),
(#263532,#263533),(#263534,#263535),(#263536,#263537),(#263538,#263539),
(#263540,#263541),(#263542,#263543),(#263544,#263545),(#263546,#263547),
(#263548,#263549),(#263550,#263551),(#263552,#263553),(#263554,#263555),
(#263556,#263557),(#263558,#263559),(#263560,#263561),(#263562,#263563),
(#263564,#263565),(#263566,#263567),(#263568,#263569),(#263570,#263571),
(#263572,#263573),(#263574,#263575),(#263576,#263577),(#263578,#263579),
(#263580,#263581),(#263582,#263583),(#263584,#263585),(#263586,#263587),
(#263588,#263589),(#263590,#263591),(#263592,#263593),(#263594,#263595),
(#263596,#263597),(#263598,#263599),(#263600,#263601),(#263602,#263603),
(#263604,#263605),(#263606,#263607),(#263608,#263609),(#263610,#263611),
(#263612,#263613),(#263614,#263615),(#263616,#263617),(#263618,#263619),
(#263620,#263621),(#263622,#263623),(#263624,#263625),(#263626,#263627),
(#263628,#263629),(#263630,#263631),(#263632,#263633),(#263634,#263635),
(#263636,#263637),(#263638,#263639),(#263640,#263641),(#263642,#263643),
(#263644,#263645),(#263646,#263647)),.UNSPECIFIED.,.F.,.F.,.F.,(6,1,1,1,
1,1,1,1,1,1,1,1,1,1,1,1,1,1,1,1,1,1,1,1,1,1,1,1,1,1,1,1,1,1,1,1,1,1,1,1,
1,1,1,1,1,1,1,1,1,1,1,1,1,1,1,1,1,1,1,1,1,1,1,1,1,1,1,1,1,1,1,1,1,1,1,1,
1,1,1,1,1,1,1,1,1,1,1,1,1,1,1,1,1,1,1,1,1,1,1,1,1,1,1,1,1,1,1,1,1,1,1,1,
1,1,1,1,1,1,1,1,1,1,1,1,1,1,1,1,1,1,1,1,1,1,1,1,1,1,1,1,1,1,1,1,1,1,1,1,
1,1,1,1,1,1,1,1,1,1,1,1,1,1,1,1,1,1,1,1,1,1,1,1,1,1,1,1,1,1,1,1,1,1,1,1,
1,1,1,1,1,1,1,1,1,1,1,1,1,1,1,1,1,1,1,1,1,1,1,1,1,1,1,1,1,1,1,1,1,1,1,1,
1,1,1,1,1,1,1,1,1,1,1,1,1,1,1,1,1,1,1,1,1,1,1,1,1,1,1,1,1,1,1,1,1,1,1,1,
1,1,1,1,1,1,1,1,1,1,1,1,1,1,1,1,1,1,1,1,1,1,1,1,1,1,1,1,1,1,1,1,1,1,1,1,
1,1,1,1,1,1,1,1,1,1,1,1,1,1,1,1,1,1,1,1,1,1,1,1,1,1,1,1,1,1,1,1,1,1,1,1,
1,1,1,1,1,1,1,1,1,1,1,1,1,1,1,1,1,1,1,1,1,1,1,1,1,1,1,1,1,1,1,1,1,1,1,1,
1,1,1,1,1,1,1,1,1,1,1,1,1,1,1,1,1,1,1,1,1,1,1,1,1,1,1,1,1,1,1,1,1,1,1,1,
1,1,1,1,1,1,1,1,1,1,1,1,1,1,1,1,1,1,1,1,1,1,1,1,1,1,1,1,1,1,1,1,1,1,1,1,
1,1,1,1,1,1,1,1,1,1,1,1,1,1,1,1,1,1,1,1,1,1,1,1,1,1,1,1,1,1,1,6),(2,2),
(-1.,-0.998165138,-0.996330275,-0.994495413,-0.99266055,-0.990825688,-0.988990826,
-0.987155963,-0.985321101,-0.983486239,-0.981651376,-0.979816514,-0.977981651,
-0.976146789,-0.974311927,-0.972477064,-0.970642202,-0.968807339,-0.966972477,
-0.965137615,-0.963302752,-0.96146789,-0.959633028,-0.957798165,-0.955963303,
-0.95412844,-0.952293578,-0.950458716,-0.948623853,-0.946788991,-0.944954128,
-0.943119266,-0.941284404,-0.939449541,-0.937614679,-0.935779817,-0.933944954,
-0.932110092,-0.930275229,-0.928440367,-0.926605505,-0.924770642,-0.92293578,
-0.921100917,-0.919266055,-0.917431193,-0.91559633,-0.913761468,-0.911926606,
-0.910091743,-0.908256881,-0.906422018,-0.904587156,-0.902752294,-0.900917431,
-0.899082569,-0.897247706,-0.895412844,-0.893577982,-0.891743119,-0.889908257,
-0.888073394,-0.886238532,-0.88440367,-0.882568807,-0.880733945,-0.878899083,
-0.87706422,-0.875229358,-0.873394495,-0.871559633,-0.869724771,-0.867889908,
-0.866055046,-0.864220183,-0.862385321,-0.860550459,-0.858715596,-0.856880734,
-0.855045872,-0.853211009,-0.851376147,-0.849541284,-0.847706422,-0.84587156,
-0.844036697,-0.842201835,-0.840366972,-0.83853211,-0.836697248,-0.834862385,
-0.833027523,-0.831192661,-0.829357798,-0.827522936,-0.825688073,-0.823853211,
-0.822018349,-0.820183486,-0.818348624,-0.816513761,-0.814678899,-0.812844037,
-0.811009174,-0.809174312,-0.80733945,-0.805504587,-0.803669725,-0.801834862,
-0.8,-0.798165138,-0.796330275,-0.794495413,-0.79266055,-0.790825688,-0.788990826,
-0.787155963,-0.785321101,-0.783486239,-0.781651376,-0.779816514,-0.777981651,
-0.776146789,-0.774311927,-0.772477064,-0.770642202,-0.768807339,-0.766972477,
-0.765137615,-0.763302752,-0.76146789,-0.759633028,-0.757798165,-0.755963303,
-0.75412844,-0.752293578,-0.750458716,-0.748623853,-0.746788991,-0.744954128,
-0.743119266,-0.741284404,-0.739449541,-0.737614679,-0.735779817,-0.733944954,
-0.732110092,-0.730275229,-0.728440367,-0.726605505,-0.724770642,-0.72293578,
-0.721100917,-0.719266055,-0.717431193,-0.71559633,-0.713761468,-0.711926606,
-0.710091743,-0.708256881,-0.706422018,-0.704587156,-0.702752294,-0.700917431,
-0.699082569,-0.697247706,-0.695412844,-0.693577982,-0.691743119,-0.689908257,
-0.688073394,-0.686238532,-0.68440367,-0.682568807,-0.680733945,-0.678899083,
-0.67706422,-0.675229358,-0.673394495,-0.671559633,-0.669724771,-0.667889908,
-0.666055046,-0.664220183,-0.662385321,-0.660550459,-0.658715596,-0.656880734,
-0.655045872,-0.653211009,-0.651376147,-0.649541284,-0.647706422,-0.64587156,
-0.644036697,-0.642201835,-0.640366972,-0.63853211,-0.636697248,-0.634862385,
-0.633027523,-0.631192661,-0.629357798,-0.627522936,-0.625688073,-0.623853211,
-0.622018349,-0.620183486,-0.618348624,-0.616513761,-0.614678899,-0.612844037,
-0.611009174,-0.609174312,-0.60733945,-0.605504587,-0.603669725,-0.601834862,
-0.6,-0.598165138,-0.596330275,-0.594495413,-0.59266055,-0.590825688,-0.588990826,
-0.587155963,-0.585321101,-0.583486239,-0.581651376,-0.579816514,-0.577981651,
-0.576146789,-0.574311927,-0.572477064,-0.570642202,-0.568807339,-0.566972477,
-0.565137615,-0.563302752,-0.56146789,-0.559633028,-0.557798165,-0.555963303,
-0.55412844,-0.552293578,-0.550458716,-0.548623853,-0.546788991,-0.544954128,
-0.543119266,-0.541284404,-0.539449541,-0.537614679,-0.535779817,-0.533944954,
-0.532110092,-0.530275229,-0.528440367,-0.526605505,-0.524770642,-0.52293578,
-0.521100917,-0.519266055,-0.517431193,-0.51559633,-0.513761468,-0.511926606,
-0.510091743,-0.508256881,-0.506422018,-0.504587156,-0.502752294,-0.500917431,
-0.499082569,-0.497247706,-0.495412844,-0.493577982,-0.491743119,-0.489908257,
-0.488073394,-0.486238532,-0.48440367,-0.482568807,-0.480733945,-0.478899083,
-0.47706422,-0.475229358,-0.473394495,-0.471559633,-0.469724771,-0.467889908,
-0.466055046,-0.464220183,-0.462385321,-0.460550459,-0.458715596,-0.456880734,
-0.455045872,-0.453211009,-0.451376147,-0.449541284,-0.447706422,-0.44587156,
-0.444036697,-0.442201835,-0.440366972,-0.43853211,-0.436697248,-0.434862385,
-0.433027523,-0.431192661,-0.429357798,-0.427522936,-0.425688073,-0.423853211,
-0.422018349,-0.420183486,-0.418348624,-0.416513761,-0.414678899,-0.412844037,
-0.411009174,-0.409174312,-0.40733945,-0.405504587,-0.403669725,-0.401834862,
-0.4,-0.398165138,-0.396330275,-0.394495413,-0.39266055,-0.390825688,-0.388990826,
-0.387155963,-0.385321101,-0.383486239,-0.381651376,-0.379816514,-0.377981651,
-0.376146789,-0.374311927,-0.372477064,-0.370642202,-0.368807339,-0.366972477,
-0.365137615,-0.363302752,-0.36146789,-0.359633028,-0.357798165,-0.355963303,
-0.35412844,-0.352293578,-0.350458716,-0.348623853,-0.346788991,-0.344954128,
-0.343119266,-0.341284404,-0.339449541,-0.337614679,-0.335779817,-0.333944954,
-0.332110092,-0.330275229,-0.328440367,-0.326605505,-0.324770642,-0.32293578,
-0.321100917,-0.319266055,-0.317431193,-0.31559633,-0.313761468,-0.311926606,
-0.310091743,-0.308256881,-0.306422018,-0.304587156,-0.302752294,-0.300917431,
-0.299082569,-0.297247706,-0.295412844,-0.293577982,-0.291743119,-0.289908257,
-0.288073394,-0.286238532,-0.28440367,-0.282568807,-0.280733945,-0.278899083,
-0.27706422,-0.275229358,-0.273394495,-0.271559633,-0.269724771,-0.267889908,
-0.266055046,-0.264220183,-0.262385321,-0.260550459,-0.258715596,-0.256880734,
-0.255045872,-0.253211009,-0.251376147,-0.249541284,-0.247706422,-0.24587156,
-0.244036697,-0.242201835,-0.240366972,-0.23853211,-0.236697248,-0.234862385,
-0.233027523,-0.231192661,-0.229357798,-0.227522936,-0.225688073,-0.223853211,
-0.222018349,-0.220183486,-0.218348624,-0.216513761,-0.214678899,-0.212844037,
-0.211009174,-0.209174312,-0.20733945,-0.205504587,-0.203669725,-0.201834862,
-0.2,-0.198165138,-0.196330275,-0.194495413,-0.19266055,-0.190825688,-0.188990826,
-0.187155963,-0.185321101,-0.183486239,-0.181651376,-0.179816514,-0.177981651,
-0.176146789,-0.174311927,-0.172477064,-0.170642202,-0.168807339,-0.166972477,
-0.165137615,-0.163302752,-0.16146789,-0.159633028,-0.157798165,-0.155963303,
-0.15412844,-0.152293578,-0.150458716,-0.148623853,-0.146788991,-0.144954128,
-0.143172103),(0.,0.36),.UNSPECIFIED.);
#6282=B_SPLINE_SURFACE_WITH_KNOTS('',5,1,((#264259,#264260),(#264261,#264262),
(#264263,#264264),(#264265,#264266),(#264267,#264268),(#264269,#264270),
(#264271,#264272),(#264273,#264274),(#264275,#264276),(#264277,#264278),
(#264279,#264280),(#264281,#264282),(#264283,#264284),(#264285,#264286),
(#264287,#264288),(#264289,#264290),(#264291,#264292),(#264293,#264294),
(#264295,#264296),(#264297,#264298),(#264299,#264300),(#264301,#264302),
(#264303,#264304),(#264305,#264306),(#264307,#264308),(#264309,#264310),
(#264311,#264312),(#264313,#264314),(#264315,#264316),(#264317,#264318),
(#264319,#264320),(#264321,#264322),(#264323,#264324),(#264325,#264326),
(#264327,#264328),(#264329,#264330),(#264331,#264332),(#264333,#264334),
(#264335,#264336),(#264337,#264338),(#264339,#264340),(#264341,#264342),
(#264343,#264344),(#264345,#264346),(#264347,#264348),(#264349,#264350),
(#264351,#264352),(#264353,#264354),(#264355,#264356),(#264357,#264358),
(#264359,#264360),(#264361,#264362),(#264363,#264364),(#264365,#264366),
(#264367,#264368),(#264369,#264370),(#264371,#264372),(#264373,#264374),
(#264375,#264376),(#264377,#264378),(#264379,#264380),(#264381,#264382),
(#264383,#264384),(#264385,#264386),(#264387,#264388),(#264389,#264390),
(#264391,#264392),(#264393,#264394),(#264395,#264396),(#264397,#264398),
(#264399,#264400),(#264401,#264402),(#264403,#264404),(#264405,#264406),
(#264407,#264408),(#264409,#264410),(#264411,#264412),(#264413,#264414),
(#264415,#264416),(#264417,#264418),(#264419,#264420),(#264421,#264422),
(#264423,#264424),(#264425,#264426),(#264427,#264428),(#264429,#264430),
(#264431,#264432),(#264433,#264434),(#264435,#264436),(#264437,#264438),
(#264439,#264440),(#264441,#264442),(#264443,#264444),(#264445,#264446),
(#264447,#264448),(#264449,#264450),(#264451,#264452),(#264453,#264454),
(#264455,#264456),(#264457,#264458),(#264459,#264460),(#264461,#264462),
(#264463,#264464),(#264465,#264466),(#264467,#264468),(#264469,#264470),
(#264471,#264472),(#264473,#264474),(#264475,#264476),(#264477,#264478),
(#264479,#264480),(#264481,#264482),(#264483,#264484),(#264485,#264486),
(#264487,#264488),(#264489,#264490),(#264491,#264492),(#264493,#264494),
(#264495,#264496),(#264497,#264498),(#264499,#264500),(#264501,#264502),
(#264503,#264504),(#264505,#264506),(#264507,#264508),(#264509,#264510),
(#264511,#264512),(#264513,#264514),(#264515,#264516),(#264517,#264518),
(#264519,#264520),(#264521,#264522),(#264523,#264524),(#264525,#264526),
(#264527,#264528),(#264529,#264530),(#264531,#264532),(#264533,#264534),
(#264535,#264536),(#264537,#264538),(#264539,#264540),(#264541,#264542),
(#264543,#264544),(#264545,#264546),(#264547,#264548),(#264549,#264550),
(#264551,#264552),(#264553,#264554),(#264555,#264556),(#264557,#264558),
(#264559,#264560),(#264561,#264562),(#264563,#264564),(#264565,#264566),
(#264567,#264568),(#264569,#264570),(#264571,#264572),(#264573,#264574),
(#264575,#264576),(#264577,#264578),(#264579,#264580),(#264581,#264582),
(#264583,#264584),(#264585,#264586),(#264587,#264588),(#264589,#264590),
(#264591,#264592),(#264593,#264594),(#264595,#264596),(#264597,#264598),
(#264599,#264600),(#264601,#264602),(#264603,#264604),(#264605,#264606),
(#264607,#264608),(#264609,#264610),(#264611,#264612),(#264613,#264614),
(#264615,#264616),(#264617,#264618),(#264619,#264620),(#264621,#264622),
(#264623,#264624),(#264625,#264626),(#264627,#264628),(#264629,#264630),
(#264631,#264632),(#264633,#264634),(#264635,#264636),(#264637,#264638),
(#264639,#264640),(#264641,#264642),(#264643,#264644),(#264645,#264646),
(#264647,#264648),(#264649,#264650),(#264651,#264652),(#264653,#264654),
(#264655,#264656),(#264657,#264658),(#264659,#264660),(#264661,#264662),
(#264663,#264664),(#264665,#264666),(#264667,#264668),(#264669,#264670),
(#264671,#264672),(#264673,#264674),(#264675,#264676),(#264677,#264678),
(#264679,#264680),(#264681,#264682),(#264683,#264684),(#264685,#264686),
(#264687,#264688),(#264689,#264690),(#264691,#264692),(#264693,#264694),
(#264695,#264696),(#264697,#264698),(#264699,#264700),(#264701,#264702),
(#264703,#264704),(#264705,#264706),(#264707,#264708),(#264709,#264710),
(#264711,#264712),(#264713,#264714),(#264715,#264716),(#264717,#264718),
(#264719,#264720),(#264721,#264722),(#264723,#264724),(#264725,#264726),
(#264727,#264728),(#264729,#264730),(#264731,#264732),(#264733,#264734),
(#264735,#264736),(#264737,#264738),(#264739,#264740),(#264741,#264742),
(#264743,#264744),(#264745,#264746),(#264747,#264748),(#264749,#264750),
(#264751,#264752),(#264753,#264754),(#264755,#264756),(#264757,#264758),
(#264759,#264760),(#264761,#264762),(#264763,#264764),(#264765,#264766),
(#264767,#264768),(#264769,#264770),(#264771,#264772),(#264773,#264774),
(#264775,#264776),(#264777,#264778),(#264779,#264780),(#264781,#264782),
(#264783,#264784),(#264785,#264786),(#264787,#264788),(#264789,#264790),
(#264791,#264792),(#264793,#264794),(#264795,#264796),(#264797,#264798),
(#264799,#264800),(#264801,#264802),(#264803,#264804),(#264805,#264806),
(#264807,#264808),(#264809,#264810),(#264811,#264812),(#264813,#264814),
(#264815,#264816),(#264817,#264818),(#264819,#264820),(#264821,#264822),
(#264823,#264824),(#264825,#264826),(#264827,#264828),(#264829,#264830),
(#264831,#264832),(#264833,#264834),(#264835,#264836),(#264837,#264838),
(#264839,#264840),(#264841,#264842),(#264843,#264844),(#264845,#264846),
(#264847,#264848),(#264849,#264850),(#264851,#264852),(#264853,#264854),
(#264855,#264856),(#264857,#264858),(#264859,#264860),(#264861,#264862),
(#264863,#264864),(#264865,#264866),(#264867,#264868),(#264869,#264870),
(#264871,#264872),(#264873,#264874),(#264875,#264876),(#264877,#264878),
(#264879,#264880),(#264881,#264882),(#264883,#264884),(#264885,#264886),
(#264887,#264888),(#264889,#264890),(#264891,#264892),(#264893,#264894),
(#264895,#264896),(#264897,#264898),(#264899,#264900),(#264901,#264902),
(#264903,#264904),(#264905,#264906),(#264907,#264908),(#264909,#264910),
(#264911,#264912),(#264913,#264914),(#264915,#264916),(#264917,#264918),
(#264919,#264920),(#264921,#264922),(#264923,#264924),(#264925,#264926),
(#264927,#264928),(#264929,#264930),(#264931,#264932),(#264933,#264934),
(#264935,#264936),(#264937,#264938),(#264939,#264940),(#264941,#264942),
(#264943,#264944),(#264945,#264946),(#264947,#264948),(#264949,#264950),
(#264951,#264952),(#264953,#264954),(#264955,#264956),(#264957,#264958),
(#264959,#264960),(#264961,#264962),(#264963,#264964),(#264965,#264966),
(#264967,#264968),(#264969,#264970),(#264971,#264972),(#264973,#264974),
(#264975,#264976),(#264977,#264978),(#264979,#264980),(#264981,#264982),
(#264983,#264984),(#264985,#264986),(#264987,#264988),(#264989,#264990),
(#264991,#264992),(#264993,#264994),(#264995,#264996),(#264997,#264998),
(#264999,#265000),(#265001,#265002),(#265003,#265004),(#265005,#265006),
(#265007,#265008),(#265009,#265010),(#265011,#265012),(#265013,#265014),
(#265015,#265016),(#265017,#265018),(#265019,#265020),(#265021,#265022),
(#265023,#265024),(#265025,#265026),(#265027,#265028),(#265029,#265030),
(#265031,#265032),(#265033,#265034),(#265035,#265036),(#265037,#265038),
(#265039,#265040),(#265041,#265042),(#265043,#265044),(#265045,#265046),
(#265047,#265048),(#265049,#265050),(#265051,#265052),(#265053,#265054),
(#265055,#265056),(#265057,#265058),(#265059,#265060),(#265061,#265062),
(#265063,#265064),(#265065,#265066),(#265067,#265068),(#265069,#265070),
(#265071,#265072),(#265073,#265074),(#265075,#265076),(#265077,#265078),
(#265079,#265080),(#265081,#265082),(#265083,#265084),(#265085,#265086),
(#265087,#265088),(#265089,#265090),(#265091,#265092),(#265093,#265094),
(#265095,#265096),(#265097,#265098),(#265099,#265100),(#265101,#265102),
(#265103,#265104),(#265105,#265106),(#265107,#265108),(#265109,#265110),
(#265111,#265112),(#265113,#265114),(#265115,#265116),(#265117,#265118),
(#265119,#265120),(#265121,#265122),(#265123,#265124),(#265125,#265126),
(#265127,#265128),(#265129,#265130),(#265131,#265132),(#265133,#265134),
(#265135,#265136),(#265137,#265138),(#265139,#265140),(#265141,#265142),
(#265143,#265144),(#265145,#265146),(#265147,#265148),(#265149,#265150),
(#265151,#265152),(#265153,#265154),(#265155,#265156),(#265157,#265158),
(#265159,#265160),(#265161,#265162),(#265163,#265164),(#265165,#265166),
(#265167,#265168),(#265169,#265170),(#265171,#265172),(#265173,#265174),
(#265175,#265176),(#265177,#265178),(#265179,#265180),(#265181,#265182),
(#265183,#265184),(#265185,#265186),(#265187,#265188),(#265189,#265190),
(#265191,#265192),(#265193,#265194),(#265195,#265196),(#265197,#265198),
(#265199,#265200),(#265201,#265202)),.UNSPECIFIED.,.F.,.F.,.F.,(6,1,1,1,
1,1,1,1,1,1,1,1,1,1,1,1,1,1,1,1,1,1,1,1,1,1,1,1,1,1,1,1,1,1,1,1,1,1,1,1,
1,1,1,1,1,1,1,1,1,1,1,1,1,1,1,1,1,1,1,1,1,1,1,1,1,1,1,1,1,1,1,1,1,1,1,1,
1,1,1,1,1,1,1,1,1,1,1,1,1,1,1,1,1,1,1,1,1,1,1,1,1,1,1,1,1,1,1,1,1,1,1,1,
1,1,1,1,1,1,1,1,1,1,1,1,1,1,1,1,1,1,1,1,1,1,1,1,1,1,1,1,1,1,1,1,1,1,1,1,
1,1,1,1,1,1,1,1,1,1,1,1,1,1,1,1,1,1,1,1,1,1,1,1,1,1,1,1,1,1,1,1,1,1,1,1,
1,1,1,1,1,1,1,1,1,1,1,1,1,1,1,1,1,1,1,1,1,1,1,1,1,1,1,1,1,1,1,1,1,1,1,1,
1,1,1,1,1,1,1,1,1,1,1,1,1,1,1,1,1,1,1,1,1,1,1,1,1,1,1,1,1,1,1,1,1,1,1,1,
1,1,1,1,1,1,1,1,1,1,1,1,1,1,1,1,1,1,1,1,1,1,1,1,1,1,1,1,1,1,1,1,1,1,1,1,
1,1,1,1,1,1,1,1,1,1,1,1,1,1,1,1,1,1,1,1,1,1,1,1,1,1,1,1,1,1,1,1,1,1,1,1,
1,1,1,1,1,1,1,1,1,1,1,1,1,1,1,1,1,1,1,1,1,1,1,1,1,1,1,1,1,1,1,1,1,1,1,1,
1,1,1,1,1,1,1,1,1,1,1,1,1,1,1,1,1,1,1,1,1,1,1,1,1,1,1,1,1,1,1,1,1,1,1,1,
1,1,1,1,1,1,1,1,1,1,1,1,1,1,1,1,1,1,1,1,1,1,1,1,1,1,1,1,1,1,1,1,1,1,1,1,
1,1,1,1,1,1,1,1,1,1,1,1,1,1,1,1,1,1,1,1,1,1,1,1,1,1,1,1,1,1,1,6),(2,2),
(0.143172103,0.144954128,0.146788991,0.148623853,0.150458716,0.152293578,
0.15412844,0.155963303,0.157798165,0.159633028,0.16146789,0.163302752,0.165137615,
0.166972477,0.168807339,0.170642202,0.172477064,0.174311927,0.176146789,
0.177981651,0.179816514,0.181651376,0.183486239,0.185321101,0.187155963,
0.188990826,0.190825688,0.19266055,0.194495413,0.196330275,0.198165138,
0.2,0.201834862,0.203669725,0.205504587,0.20733945,0.209174312,0.211009174,
0.212844037,0.214678899,0.216513761,0.218348624,0.220183486,0.222018349,
0.223853211,0.225688073,0.227522936,0.229357798,0.231192661,0.233027523,
0.234862385,0.236697248,0.23853211,0.240366972,0.242201835,0.244036697,
0.24587156,0.247706422,0.249541284,0.251376147,0.253211009,0.255045872,
0.256880734,0.258715596,0.260550459,0.262385321,0.264220183,0.266055046,
0.267889908,0.269724771,0.271559633,0.273394495,0.275229358,0.27706422,
0.278899083,0.280733945,0.282568807,0.28440367,0.286238532,0.288073394,
0.289908257,0.291743119,0.293577982,0.295412844,0.297247706,0.299082569,
0.300917431,0.302752294,0.304587156,0.306422018,0.308256881,0.310091743,
0.311926606,0.313761468,0.31559633,0.317431193,0.319266055,0.321100917,
0.32293578,0.324770642,0.326605505,0.328440367,0.330275229,0.332110092,
0.333944954,0.335779817,0.337614679,0.339449541,0.341284404,0.343119266,
0.344954128,0.346788991,0.348623853,0.350458716,0.352293578,0.35412844,
0.355963303,0.357798165,0.359633028,0.36146789,0.363302752,0.365137615,
0.366972477,0.368807339,0.370642202,0.372477064,0.374311927,0.376146789,
0.377981651,0.379816514,0.381651376,0.383486239,0.385321101,0.387155963,
0.388990826,0.390825688,0.39266055,0.394495413,0.396330275,0.398165138,
0.4,0.401834862,0.403669725,0.405504587,0.40733945,0.409174312,0.411009174,
0.412844037,0.414678899,0.416513761,0.418348624,0.420183486,0.422018349,
0.423853211,0.425688073,0.427522936,0.429357798,0.431192661,0.433027523,
0.434862385,0.436697248,0.43853211,0.440366972,0.442201835,0.444036697,
0.44587156,0.447706422,0.449541284,0.451376147,0.453211009,0.455045872,
0.456880734,0.458715596,0.460550459,0.462385321,0.464220183,0.466055046,
0.467889908,0.469724771,0.471559633,0.473394495,0.475229358,0.47706422,
0.478899083,0.480733945,0.482568807,0.48440367,0.486238532,0.488073394,
0.489908257,0.491743119,0.493577982,0.495412844,0.497247706,0.499082569,
0.500917431,0.502752294,0.504587156,0.506422018,0.508256881,0.510091743,
0.511926606,0.513761468,0.51559633,0.517431193,0.519266055,0.521100917,
0.52293578,0.524770642,0.526605505,0.528440367,0.530275229,0.532110092,
0.533944954,0.535779817,0.537614679,0.539449541,0.541284404,0.543119266,
0.544954128,0.546788991,0.548623853,0.550458716,0.552293578,0.55412844,
0.555963303,0.557798165,0.559633028,0.56146789,0.563302752,0.565137615,
0.566972477,0.568807339,0.570642202,0.572477064,0.574311927,0.576146789,
0.577981651,0.579816514,0.581651376,0.583486239,0.585321101,0.587155963,
0.588990826,0.590825688,0.59266055,0.594495413,0.596330275,0.598165138,
0.6,0.601834862,0.603669725,0.605504587,0.60733945,0.609174312,0.611009174,
0.612844037,0.614678899,0.616513761,0.618348624,0.620183486,0.622018349,
0.623853211,0.625688073,0.627522936,0.629357798,0.631192661,0.633027523,
0.634862385,0.636697248,0.63853211,0.640366972,0.642201835,0.644036697,
0.64587156,0.647706422,0.649541284,0.651376147,0.653211009,0.655045872,
0.656880734,0.658715596,0.660550459,0.662385321,0.664220183,0.666055046,
0.667889908,0.669724771,0.671559633,0.673394495,0.675229358,0.67706422,
0.678899083,0.680733945,0.682568807,0.68440367,0.686238532,0.688073394,
0.689908257,0.691743119,0.693577982,0.695412844,0.697247706,0.699082569,
0.700917431,0.702752294,0.704587156,0.706422018,0.708256881,0.710091743,
0.711926606,0.713761468,0.71559633,0.717431193,0.719266055,0.721100917,
0.72293578,0.724770642,0.726605505,0.728440367,0.730275229,0.732110092,
0.733944954,0.735779817,0.737614679,0.739449541,0.741284404,0.743119266,
0.744954128,0.746788991,0.748623853,0.750458716,0.752293578,0.75412844,
0.755963303,0.757798165,0.759633028,0.76146789,0.763302752,0.765137615,
0.766972477,0.768807339,0.770642202,0.772477064,0.774311927,0.776146789,
0.777981651,0.779816514,0.781651376,0.783486239,0.785321101,0.787155963,
0.788990826,0.790825688,0.79266055,0.794495413,0.796330275,0.798165138,
0.8,0.801834862,0.803669725,0.805504587,0.80733945,0.809174312,0.811009174,
0.812844037,0.814678899,0.816513761,0.818348624,0.820183486,0.822018349,
0.823853211,0.825688073,0.827522936,0.829357798,0.831192661,0.833027523,
0.834862385,0.836697248,0.83853211,0.840366972,0.842201835,0.844036697,
0.84587156,0.847706422,0.849541284,0.851376147,0.853211009,0.855045872,
0.856880734,0.858715596,0.860550459,0.862385321,0.864220183,0.866055046,
0.867889908,0.869724771,0.871559633,0.873394495,0.875229358,0.87706422,
0.878899083,0.880733945,0.882568807,0.88440367,0.886238532,0.888073394,
0.889908257,0.891743119,0.893577982,0.895412844,0.897247706,0.899082569,
0.900917431,0.902752294,0.904587156,0.906422018,0.908256881,0.910091743,
0.911926606,0.913761468,0.91559633,0.917431193,0.919266055,0.921100917,
0.92293578,0.924770642,0.926605505,0.928440367,0.930275229,0.932110092,
0.933944954,0.935779817,0.937614679,0.939449541,0.941284404,0.943119266,
0.944954128,0.946788991,0.948623853,0.950458716,0.952293578,0.95412844,
0.955963303,0.957798165,0.959633028,0.96146789,0.963302752,0.965137615,
0.966972477,0.968807339,0.970642202,0.972477064,0.974311927,0.976146789,
0.977981651,0.979816514,0.981651376,0.983486239,0.985321101,0.987155963,
0.988990826,0.990825688,0.99266055,0.994495413,0.996330275,0.998165138,
1.),(0.,0.36),.UNSPECIFIED.);
#6283=B_SPLINE_SURFACE_WITH_KNOTS('',5,1,((#266158,#266159),(#266160,#266161),
(#266162,#266163),(#266164,#266165),(#266166,#266167),(#266168,#266169),
(#266170,#266171),(#266172,#266173),(#266174,#266175),(#266176,#266177),
(#266178,#266179),(#266180,#266181),(#266182,#266183),(#266184,#266185),
(#266186,#266187),(#266188,#266189),(#266190,#266191),(#266192,#266193),
(#266194,#266195),(#266196,#266197),(#266198,#266199),(#266200,#266201),
(#266202,#266203),(#266204,#266205),(#266206,#266207),(#266208,#266209),
(#266210,#266211),(#266212,#266213),(#266214,#266215),(#266216,#266217),
(#266218,#266219),(#266220,#266221),(#266222,#266223),(#266224,#266225),
(#266226,#266227),(#266228,#266229),(#266230,#266231),(#266232,#266233),
(#266234,#266235),(#266236,#266237),(#266238,#266239),(#266240,#266241),
(#266242,#266243),(#266244,#266245),(#266246,#266247),(#266248,#266249),
(#266250,#266251),(#266252,#266253),(#266254,#266255),(#266256,#266257),
(#266258,#266259),(#266260,#266261),(#266262,#266263),(#266264,#266265),
(#266266,#266267),(#266268,#266269),(#266270,#266271),(#266272,#266273),
(#266274,#266275),(#266276,#266277),(#266278,#266279),(#266280,#266281),
(#266282,#266283),(#266284,#266285),(#266286,#266287),(#266288,#266289),
(#266290,#266291),(#266292,#266293),(#266294,#266295),(#266296,#266297),
(#266298,#266299),(#266300,#266301),(#266302,#266303),(#266304,#266305),
(#266306,#266307),(#266308,#266309),(#266310,#266311),(#266312,#266313),
(#266314,#266315),(#266316,#266317),(#266318,#266319),(#266320,#266321),
(#266322,#266323),(#266324,#266325),(#266326,#266327),(#266328,#266329),
(#266330,#266331),(#266332,#266333),(#266334,#266335),(#266336,#266337),
(#266338,#266339),(#266340,#266341),(#266342,#266343),(#266344,#266345),
(#266346,#266347),(#266348,#266349),(#266350,#266351),(#266352,#266353),
(#266354,#266355),(#266356,#266357),(#266358,#266359),(#266360,#266361),
(#266362,#266363),(#266364,#266365),(#266366,#266367),(#266368,#266369),
(#266370,#266371),(#266372,#266373),(#266374,#266375),(#266376,#266377),
(#266378,#266379),(#266380,#266381),(#266382,#266383),(#266384,#266385),
(#266386,#266387),(#266388,#266389),(#266390,#266391),(#266392,#266393),
(#266394,#266395),(#266396,#266397),(#266398,#266399),(#266400,#266401),
(#266402,#266403),(#266404,#266405),(#266406,#266407),(#266408,#266409),
(#266410,#266411),(#266412,#266413),(#266414,#266415),(#266416,#266417),
(#266418,#266419),(#266420,#266421),(#266422,#266423),(#266424,#266425),
(#266426,#266427),(#266428,#266429),(#266430,#266431),(#266432,#266433),
(#266434,#266435),(#266436,#266437),(#266438,#266439),(#266440,#266441),
(#266442,#266443),(#266444,#266445),(#266446,#266447),(#266448,#266449),
(#266450,#266451),(#266452,#266453),(#266454,#266455),(#266456,#266457),
(#266458,#266459),(#266460,#266461),(#266462,#266463),(#266464,#266465),
(#266466,#266467),(#266468,#266469),(#266470,#266471),(#266472,#266473),
(#266474,#266475),(#266476,#266477),(#266478,#266479),(#266480,#266481),
(#266482,#266483),(#266484,#266485),(#266486,#266487),(#266488,#266489),
(#266490,#266491),(#266492,#266493),(#266494,#266495),(#266496,#266497),
(#266498,#266499),(#266500,#266501),(#266502,#266503),(#266504,#266505),
(#266506,#266507),(#266508,#266509),(#266510,#266511),(#266512,#266513),
(#266514,#266515),(#266516,#266517),(#266518,#266519),(#266520,#266521),
(#266522,#266523),(#266524,#266525),(#266526,#266527),(#266528,#266529),
(#266530,#266531),(#266532,#266533),(#266534,#266535),(#266536,#266537),
(#266538,#266539),(#266540,#266541),(#266542,#266543),(#266544,#266545),
(#266546,#266547),(#266548,#266549),(#266550,#266551),(#266552,#266553),
(#266554,#266555),(#266556,#266557),(#266558,#266559),(#266560,#266561),
(#266562,#266563),(#266564,#266565),(#266566,#266567),(#266568,#266569),
(#266570,#266571),(#266572,#266573),(#266574,#266575),(#266576,#266577),
(#266578,#266579),(#266580,#266581),(#266582,#266583),(#266584,#266585),
(#266586,#266587),(#266588,#266589),(#266590,#266591),(#266592,#266593),
(#266594,#266595),(#266596,#266597),(#266598,#266599),(#266600,#266601),
(#266602,#266603),(#266604,#266605),(#266606,#266607),(#266608,#266609),
(#266610,#266611),(#266612,#266613),(#266614,#266615),(#266616,#266617),
(#266618,#266619),(#266620,#266621),(#266622,#266623),(#266624,#266625),
(#266626,#266627),(#266628,#266629),(#266630,#266631),(#266632,#266633),
(#266634,#266635),(#266636,#266637),(#266638,#266639),(#266640,#266641),
(#266642,#266643),(#266644,#266645),(#266646,#266647),(#266648,#266649),
(#266650,#266651),(#266652,#266653),(#266654,#266655),(#266656,#266657),
(#266658,#266659),(#266660,#266661),(#266662,#266663),(#266664,#266665),
(#266666,#266667),(#266668,#266669),(#266670,#266671),(#266672,#266673),
(#266674,#266675),(#266676,#266677),(#266678,#266679),(#266680,#266681),
(#266682,#266683),(#266684,#266685),(#266686,#266687),(#266688,#266689),
(#266690,#266691),(#266692,#266693),(#266694,#266695),(#266696,#266697),
(#266698,#266699),(#266700,#266701),(#266702,#266703),(#266704,#266705),
(#266706,#266707),(#266708,#266709),(#266710,#266711),(#266712,#266713),
(#266714,#266715),(#266716,#266717),(#266718,#266719),(#266720,#266721),
(#266722,#266723),(#266724,#266725),(#266726,#266727),(#266728,#266729),
(#266730,#266731),(#266732,#266733),(#266734,#266735),(#266736,#266737),
(#266738,#266739),(#266740,#266741),(#266742,#266743),(#266744,#266745),
(#266746,#266747),(#266748,#266749),(#266750,#266751),(#266752,#266753),
(#266754,#266755),(#266756,#266757),(#266758,#266759),(#266760,#266761),
(#266762,#266763),(#266764,#266765),(#266766,#266767),(#266768,#266769),
(#266770,#266771),(#266772,#266773),(#266774,#266775),(#266776,#266777),
(#266778,#266779),(#266780,#266781),(#266782,#266783),(#266784,#266785),
(#266786,#266787),(#266788,#266789),(#266790,#266791),(#266792,#266793),
(#266794,#266795),(#266796,#266797),(#266798,#266799),(#266800,#266801),
(#266802,#266803),(#266804,#266805),(#266806,#266807),(#266808,#266809),
(#266810,#266811),(#266812,#266813),(#266814,#266815),(#266816,#266817),
(#266818,#266819),(#266820,#266821),(#266822,#266823),(#266824,#266825),
(#266826,#266827),(#266828,#266829),(#266830,#266831),(#266832,#266833),
(#266834,#266835),(#266836,#266837),(#266838,#266839),(#266840,#266841),
(#266842,#266843),(#266844,#266845),(#266846,#266847),(#266848,#266849),
(#266850,#266851),(#266852,#266853),(#266854,#266855),(#266856,#266857),
(#266858,#266859),(#266860,#266861),(#266862,#266863),(#266864,#266865),
(#266866,#266867),(#266868,#266869),(#266870,#266871),(#266872,#266873),
(#266874,#266875),(#266876,#266877),(#266878,#266879),(#266880,#266881),
(#266882,#266883),(#266884,#266885),(#266886,#266887),(#266888,#266889),
(#266890,#266891),(#266892,#266893),(#266894,#266895),(#266896,#266897),
(#266898,#266899),(#266900,#266901),(#266902,#266903),(#266904,#266905),
(#266906,#266907),(#266908,#266909),(#266910,#266911),(#266912,#266913),
(#266914,#266915),(#266916,#266917),(#266918,#266919),(#266920,#266921),
(#266922,#266923),(#266924,#266925),(#266926,#266927),(#266928,#266929),
(#266930,#266931),(#266932,#266933),(#266934,#266935),(#266936,#266937),
(#266938,#266939),(#266940,#266941),(#266942,#266943),(#266944,#266945),
(#266946,#266947),(#266948,#266949),(#266950,#266951),(#266952,#266953),
(#266954,#266955),(#266956,#266957),(#266958,#266959),(#266960,#266961),
(#266962,#266963),(#266964,#266965),(#266966,#266967),(#266968,#266969),
(#266970,#266971),(#266972,#266973),(#266974,#266975),(#266976,#266977),
(#266978,#266979),(#266980,#266981),(#266982,#266983),(#266984,#266985),
(#266986,#266987),(#266988,#266989),(#266990,#266991),(#266992,#266993),
(#266994,#266995),(#266996,#266997),(#266998,#266999),(#267000,#267001),
(#267002,#267003),(#267004,#267005),(#267006,#267007),(#267008,#267009),
(#267010,#267011),(#267012,#267013),(#267014,#267015),(#267016,#267017),
(#267018,#267019),(#267020,#267021),(#267022,#267023),(#267024,#267025),
(#267026,#267027),(#267028,#267029),(#267030,#267031),(#267032,#267033),
(#267034,#267035),(#267036,#267037),(#267038,#267039),(#267040,#267041),
(#267042,#267043),(#267044,#267045),(#267046,#267047),(#267048,#267049),
(#267050,#267051),(#267052,#267053),(#267054,#267055),(#267056,#267057),
(#267058,#267059),(#267060,#267061),(#267062,#267063),(#267064,#267065),
(#267066,#267067),(#267068,#267069),(#267070,#267071),(#267072,#267073),
(#267074,#267075),(#267076,#267077),(#267078,#267079),(#267080,#267081),
(#267082,#267083),(#267084,#267085),(#267086,#267087),(#267088,#267089),
(#267090,#267091),(#267092,#267093),(#267094,#267095),(#267096,#267097),
(#267098,#267099),(#267100,#267101)),.UNSPECIFIED.,.F.,.F.,.F.,(6,1,1,1,
1,1,1,1,1,1,1,1,1,1,1,1,1,1,1,1,1,1,1,1,1,1,1,1,1,1,1,1,1,1,1,1,1,1,1,1,
1,1,1,1,1,1,1,1,1,1,1,1,1,1,1,1,1,1,1,1,1,1,1,1,1,1,1,1,1,1,1,1,1,1,1,1,
1,1,1,1,1,1,1,1,1,1,1,1,1,1,1,1,1,1,1,1,1,1,1,1,1,1,1,1,1,1,1,1,1,1,1,1,
1,1,1,1,1,1,1,1,1,1,1,1,1,1,1,1,1,1,1,1,1,1,1,1,1,1,1,1,1,1,1,1,1,1,1,1,
1,1,1,1,1,1,1,1,1,1,1,1,1,1,1,1,1,1,1,1,1,1,1,1,1,1,1,1,1,1,1,1,1,1,1,1,
1,1,1,1,1,1,1,1,1,1,1,1,1,1,1,1,1,1,1,1,1,1,1,1,1,1,1,1,1,1,1,1,1,1,1,1,
1,1,1,1,1,1,1,1,1,1,1,1,1,1,1,1,1,1,1,1,1,1,1,1,1,1,1,1,1,1,1,1,1,1,1,1,
1,1,1,1,1,1,1,1,1,1,1,1,1,1,1,1,1,1,1,1,1,1,1,1,1,1,1,1,1,1,1,1,1,1,1,1,
1,1,1,1,1,1,1,1,1,1,1,1,1,1,1,1,1,1,1,1,1,1,1,1,1,1,1,1,1,1,1,1,1,1,1,1,
1,1,1,1,1,1,1,1,1,1,1,1,1,1,1,1,1,1,1,1,1,1,1,1,1,1,1,1,1,1,1,1,1,1,1,1,
1,1,1,1,1,1,1,1,1,1,1,1,1,1,1,1,1,1,1,1,1,1,1,1,1,1,1,1,1,1,1,1,1,1,1,1,
1,1,1,1,1,1,1,1,1,1,1,1,1,1,1,1,1,1,1,1,1,1,1,1,1,1,1,1,1,1,1,1,1,1,1,1,
1,1,1,1,1,1,1,1,1,1,1,1,1,1,1,1,1,1,1,1,1,1,1,1,1,1,1,1,1,1,1,6),(2,2),
(0.143172103,0.144954128,0.146788991,0.148623853,0.150458716,0.152293578,
0.15412844,0.155963303,0.157798165,0.159633028,0.16146789,0.163302752,0.165137615,
0.166972477,0.168807339,0.170642202,0.172477064,0.174311927,0.176146789,
0.177981651,0.179816514,0.181651376,0.183486239,0.185321101,0.187155963,
0.188990826,0.190825688,0.19266055,0.194495413,0.196330275,0.198165138,
0.2,0.201834862,0.203669725,0.205504587,0.20733945,0.209174312,0.211009174,
0.212844037,0.214678899,0.216513761,0.218348624,0.220183486,0.222018349,
0.223853211,0.225688073,0.227522936,0.229357798,0.231192661,0.233027523,
0.234862385,0.236697248,0.23853211,0.240366972,0.242201835,0.244036697,
0.24587156,0.247706422,0.249541284,0.251376147,0.253211009,0.255045872,
0.256880734,0.258715596,0.260550459,0.262385321,0.264220183,0.266055046,
0.267889908,0.269724771,0.271559633,0.273394495,0.275229358,0.27706422,
0.278899083,0.280733945,0.282568807,0.28440367,0.286238532,0.288073394,
0.289908257,0.291743119,0.293577982,0.295412844,0.297247706,0.299082569,
0.300917431,0.302752294,0.304587156,0.306422018,0.308256881,0.310091743,
0.311926606,0.313761468,0.31559633,0.317431193,0.319266055,0.321100917,
0.32293578,0.324770642,0.326605505,0.328440367,0.330275229,0.332110092,
0.333944954,0.335779817,0.337614679,0.339449541,0.341284404,0.343119266,
0.344954128,0.346788991,0.348623853,0.350458716,0.352293578,0.35412844,
0.355963303,0.357798165,0.359633028,0.36146789,0.363302752,0.365137615,
0.366972477,0.368807339,0.370642202,0.372477064,0.374311927,0.376146789,
0.377981651,0.379816514,0.381651376,0.383486239,0.385321101,0.387155963,
0.388990826,0.390825688,0.39266055,0.394495413,0.396330275,0.398165138,
0.4,0.401834862,0.403669725,0.405504587,0.40733945,0.409174312,0.411009174,
0.412844037,0.414678899,0.416513761,0.418348624,0.420183486,0.422018349,
0.423853211,0.425688073,0.427522936,0.429357798,0.431192661,0.433027523,
0.434862385,0.436697248,0.43853211,0.440366972,0.442201835,0.444036697,
0.44587156,0.447706422,0.449541284,0.451376147,0.453211009,0.455045872,
0.456880734,0.458715596,0.460550459,0.462385321,0.464220183,0.466055046,
0.467889908,0.469724771,0.471559633,0.473394495,0.475229358,0.47706422,
0.478899083,0.480733945,0.482568807,0.48440367,0.486238532,0.488073394,
0.489908257,0.491743119,0.493577982,0.495412844,0.497247706,0.499082569,
0.500917431,0.502752294,0.504587156,0.506422018,0.508256881,0.510091743,
0.511926606,0.513761468,0.51559633,0.517431193,0.519266055,0.521100917,
0.52293578,0.524770642,0.526605505,0.528440367,0.530275229,0.532110092,
0.533944954,0.535779817,0.537614679,0.539449541,0.541284404,0.543119266,
0.544954128,0.546788991,0.548623853,0.550458716,0.552293578,0.55412844,
0.555963303,0.557798165,0.559633028,0.56146789,0.563302752,0.565137615,
0.566972477,0.568807339,0.570642202,0.572477064,0.574311927,0.576146789,
0.577981651,0.579816514,0.581651376,0.583486239,0.585321101,0.587155963,
0.588990826,0.590825688,0.59266055,0.594495413,0.596330275,0.598165138,
0.6,0.601834862,0.603669725,0.605504587,0.60733945,0.609174312,0.611009174,
0.612844037,0.614678899,0.616513761,0.618348624,0.620183486,0.622018349,
0.623853211,0.625688073,0.627522936,0.629357798,0.631192661,0.633027523,
0.634862385,0.636697248,0.63853211,0.640366972,0.642201835,0.644036697,
0.64587156,0.647706422,0.649541284,0.651376147,0.653211009,0.655045872,
0.656880734,0.658715596,0.660550459,0.662385321,0.664220183,0.666055046,
0.667889908,0.669724771,0.671559633,0.673394495,0.675229358,0.67706422,
0.678899083,0.680733945,0.682568807,0.68440367,0.686238532,0.688073394,
0.689908257,0.691743119,0.693577982,0.695412844,0.697247706,0.699082569,
0.700917431,0.702752294,0.704587156,0.706422018,0.708256881,0.710091743,
0.711926606,0.713761468,0.71559633,0.717431193,0.719266055,0.721100917,
0.72293578,0.724770642,0.726605505,0.728440367,0.730275229,0.732110092,
0.733944954,0.735779817,0.737614679,0.739449541,0.741284404,0.743119266,
0.744954128,0.746788991,0.748623853,0.750458716,0.752293578,0.75412844,
0.755963303,0.757798165,0.759633028,0.76146789,0.763302752,0.765137615,
0.766972477,0.768807339,0.770642202,0.772477064,0.774311927,0.776146789,
0.777981651,0.779816514,0.781651376,0.783486239,0.785321101,0.787155963,
0.788990826,0.790825688,0.79266055,0.794495413,0.796330275,0.798165138,
0.8,0.801834862,0.803669725,0.805504587,0.80733945,0.809174312,0.811009174,
0.812844037,0.814678899,0.816513761,0.818348624,0.820183486,0.822018349,
0.823853211,0.825688073,0.827522936,0.829357798,0.831192661,0.833027523,
0.834862385,0.836697248,0.83853211,0.840366972,0.842201835,0.844036697,
0.84587156,0.847706422,0.849541284,0.851376147,0.853211009,0.855045872,
0.856880734,0.858715596,0.860550459,0.862385321,0.864220183,0.866055046,
0.867889908,0.869724771,0.871559633,0.873394495,0.875229358,0.87706422,
0.878899083,0.880733945,0.882568807,0.88440367,0.886238532,0.888073394,
0.889908257,0.891743119,0.893577982,0.895412844,0.897247706,0.899082569,
0.900917431,0.902752294,0.904587156,0.906422018,0.908256881,0.910091743,
0.911926606,0.913761468,0.91559633,0.917431193,0.919266055,0.921100917,
0.92293578,0.924770642,0.926605505,0.928440367,0.930275229,0.932110092,
0.933944954,0.935779817,0.937614679,0.939449541,0.941284404,0.943119266,
0.944954128,0.946788991,0.948623853,0.950458716,0.952293578,0.95412844,
0.955963303,0.957798165,0.959633028,0.96146789,0.963302752,0.965137615,
0.966972477,0.968807339,0.970642202,0.972477064,0.974311927,0.976146789,
0.977981651,0.979816514,0.981651376,0.983486239,0.985321101,0.987155963,
0.988990826,0.990825688,0.99266055,0.994495413,0.996330275,0.998165138,
1.),(0.,0.36),.UNSPECIFIED.);
#6284=B_SPLINE_SURFACE_WITH_KNOTS('',5,1,((#267743,#267744),(#267745,#267746),
(#267747,#267748),(#267749,#267750),(#267751,#267752),(#267753,#267754),
(#267755,#267756),(#267757,#267758),(#267759,#267760),(#267761,#267762),
(#267763,#267764),(#267765,#267766),(#267767,#267768),(#267769,#267770),
(#267771,#267772),(#267773,#267774),(#267775,#267776),(#267777,#267778),
(#267779,#267780),(#267781,#267782),(#267783,#267784),(#267785,#267786),
(#267787,#267788),(#267789,#267790),(#267791,#267792),(#267793,#267794),
(#267795,#267796),(#267797,#267798),(#267799,#267800),(#267801,#267802),
(#267803,#267804),(#267805,#267806),(#267807,#267808),(#267809,#267810),
(#267811,#267812),(#267813,#267814),(#267815,#267816),(#267817,#267818),
(#267819,#267820),(#267821,#267822),(#267823,#267824),(#267825,#267826),
(#267827,#267828),(#267829,#267830),(#267831,#267832),(#267833,#267834),
(#267835,#267836),(#267837,#267838),(#267839,#267840),(#267841,#267842),
(#267843,#267844),(#267845,#267846),(#267847,#267848),(#267849,#267850),
(#267851,#267852),(#267853,#267854),(#267855,#267856),(#267857,#267858),
(#267859,#267860),(#267861,#267862),(#267863,#267864),(#267865,#267866),
(#267867,#267868),(#267869,#267870),(#267871,#267872),(#267873,#267874),
(#267875,#267876),(#267877,#267878),(#267879,#267880),(#267881,#267882),
(#267883,#267884),(#267885,#267886),(#267887,#267888),(#267889,#267890),
(#267891,#267892),(#267893,#267894),(#267895,#267896),(#267897,#267898),
(#267899,#267900),(#267901,#267902),(#267903,#267904),(#267905,#267906),
(#267907,#267908),(#267909,#267910),(#267911,#267912),(#267913,#267914),
(#267915,#267916),(#267917,#267918),(#267919,#267920),(#267921,#267922),
(#267923,#267924),(#267925,#267926),(#267927,#267928),(#267929,#267930),
(#267931,#267932),(#267933,#267934),(#267935,#267936),(#267937,#267938),
(#267939,#267940),(#267941,#267942),(#267943,#267944),(#267945,#267946),
(#267947,#267948),(#267949,#267950),(#267951,#267952),(#267953,#267954),
(#267955,#267956),(#267957,#267958),(#267959,#267960),(#267961,#267962),
(#267963,#267964),(#267965,#267966),(#267967,#267968),(#267969,#267970),
(#267971,#267972),(#267973,#267974),(#267975,#267976),(#267977,#267978),
(#267979,#267980),(#267981,#267982),(#267983,#267984),(#267985,#267986),
(#267987,#267988),(#267989,#267990),(#267991,#267992),(#267993,#267994),
(#267995,#267996),(#267997,#267998),(#267999,#268000),(#268001,#268002),
(#268003,#268004),(#268005,#268006),(#268007,#268008),(#268009,#268010),
(#268011,#268012),(#268013,#268014),(#268015,#268016),(#268017,#268018),
(#268019,#268020),(#268021,#268022),(#268023,#268024),(#268025,#268026),
(#268027,#268028),(#268029,#268030),(#268031,#268032),(#268033,#268034),
(#268035,#268036),(#268037,#268038),(#268039,#268040),(#268041,#268042),
(#268043,#268044),(#268045,#268046),(#268047,#268048),(#268049,#268050),
(#268051,#268052),(#268053,#268054),(#268055,#268056),(#268057,#268058),
(#268059,#268060),(#268061,#268062),(#268063,#268064),(#268065,#268066),
(#268067,#268068),(#268069,#268070),(#268071,#268072),(#268073,#268074),
(#268075,#268076),(#268077,#268078),(#268079,#268080),(#268081,#268082),
(#268083,#268084),(#268085,#268086),(#268087,#268088),(#268089,#268090),
(#268091,#268092),(#268093,#268094),(#268095,#268096),(#268097,#268098),
(#268099,#268100),(#268101,#268102),(#268103,#268104),(#268105,#268106),
(#268107,#268108),(#268109,#268110),(#268111,#268112),(#268113,#268114),
(#268115,#268116),(#268117,#268118),(#268119,#268120),(#268121,#268122),
(#268123,#268124),(#268125,#268126),(#268127,#268128),(#268129,#268130),
(#268131,#268132),(#268133,#268134),(#268135,#268136),(#268137,#268138),
(#268139,#268140),(#268141,#268142),(#268143,#268144),(#268145,#268146),
(#268147,#268148),(#268149,#268150),(#268151,#268152),(#268153,#268154),
(#268155,#268156),(#268157,#268158),(#268159,#268160),(#268161,#268162),
(#268163,#268164),(#268165,#268166),(#268167,#268168),(#268169,#268170),
(#268171,#268172),(#268173,#268174),(#268175,#268176),(#268177,#268178),
(#268179,#268180),(#268181,#268182),(#268183,#268184),(#268185,#268186),
(#268187,#268188),(#268189,#268190),(#268191,#268192),(#268193,#268194),
(#268195,#268196),(#268197,#268198),(#268199,#268200),(#268201,#268202),
(#268203,#268204),(#268205,#268206),(#268207,#268208),(#268209,#268210),
(#268211,#268212),(#268213,#268214),(#268215,#268216),(#268217,#268218),
(#268219,#268220),(#268221,#268222),(#268223,#268224),(#268225,#268226),
(#268227,#268228),(#268229,#268230),(#268231,#268232),(#268233,#268234),
(#268235,#268236),(#268237,#268238),(#268239,#268240),(#268241,#268242),
(#268243,#268244),(#268245,#268246),(#268247,#268248),(#268249,#268250),
(#268251,#268252),(#268253,#268254),(#268255,#268256),(#268257,#268258),
(#268259,#268260),(#268261,#268262),(#268263,#268264),(#268265,#268266),
(#268267,#268268),(#268269,#268270),(#268271,#268272),(#268273,#268274),
(#268275,#268276),(#268277,#268278),(#268279,#268280),(#268281,#268282),
(#268283,#268284),(#268285,#268286),(#268287,#268288),(#268289,#268290),
(#268291,#268292),(#268293,#268294),(#268295,#268296),(#268297,#268298),
(#268299,#268300),(#268301,#268302),(#268303,#268304),(#268305,#268306),
(#268307,#268308),(#268309,#268310),(#268311,#268312),(#268313,#268314),
(#268315,#268316),(#268317,#268318),(#268319,#268320),(#268321,#268322),
(#268323,#268324),(#268325,#268326),(#268327,#268328),(#268329,#268330),
(#268331,#268332),(#268333,#268334),(#268335,#268336),(#268337,#268338),
(#268339,#268340),(#268341,#268342),(#268343,#268344),(#268345,#268346),
(#268347,#268348),(#268349,#268350),(#268351,#268352),(#268353,#268354),
(#268355,#268356),(#268357,#268358),(#268359,#268360),(#268361,#268362),
(#268363,#268364),(#268365,#268366),(#268367,#268368),(#268369,#268370),
(#268371,#268372),(#268373,#268374),(#268375,#268376),(#268377,#268378),
(#268379,#268380),(#268381,#268382),(#268383,#268384),(#268385,#268386),
(#268387,#268388),(#268389,#268390),(#268391,#268392),(#268393,#268394),
(#268395,#268396),(#268397,#268398),(#268399,#268400),(#268401,#268402),
(#268403,#268404),(#268405,#268406),(#268407,#268408),(#268409,#268410),
(#268411,#268412),(#268413,#268414),(#268415,#268416),(#268417,#268418),
(#268419,#268420),(#268421,#268422),(#268423,#268424),(#268425,#268426),
(#268427,#268428),(#268429,#268430),(#268431,#268432),(#268433,#268434),
(#268435,#268436),(#268437,#268438),(#268439,#268440),(#268441,#268442),
(#268443,#268444),(#268445,#268446),(#268447,#268448),(#268449,#268450),
(#268451,#268452),(#268453,#268454),(#268455,#268456),(#268457,#268458),
(#268459,#268460),(#268461,#268462),(#268463,#268464),(#268465,#268466),
(#268467,#268468),(#268469,#268470),(#268471,#268472),(#268473,#268474),
(#268475,#268476),(#268477,#268478),(#268479,#268480),(#268481,#268482),
(#268483,#268484),(#268485,#268486),(#268487,#268488),(#268489,#268490),
(#268491,#268492),(#268493,#268494),(#268495,#268496),(#268497,#268498),
(#268499,#268500),(#268501,#268502),(#268503,#268504),(#268505,#268506),
(#268507,#268508),(#268509,#268510),(#268511,#268512),(#268513,#268514),
(#268515,#268516),(#268517,#268518),(#268519,#268520),(#268521,#268522),
(#268523,#268524),(#268525,#268526),(#268527,#268528),(#268529,#268530),
(#268531,#268532),(#268533,#268534),(#268535,#268536),(#268537,#268538),
(#268539,#268540),(#268541,#268542),(#268543,#268544),(#268545,#268546),
(#268547,#268548),(#268549,#268550),(#268551,#268552),(#268553,#268554),
(#268555,#268556),(#268557,#268558),(#268559,#268560),(#268561,#268562),
(#268563,#268564),(#268565,#268566),(#268567,#268568),(#268569,#268570),
(#268571,#268572),(#268573,#268574),(#268575,#268576),(#268577,#268578),
(#268579,#268580),(#268581,#268582),(#268583,#268584),(#268585,#268586),
(#268587,#268588),(#268589,#268590),(#268591,#268592),(#268593,#268594),
(#268595,#268596),(#268597,#268598),(#268599,#268600),(#268601,#268602),
(#268603,#268604),(#268605,#268606),(#268607,#268608),(#268609,#268610),
(#268611,#268612),(#268613,#268614),(#268615,#268616),(#268617,#268618),
(#268619,#268620),(#268621,#268622),(#268623,#268624),(#268625,#268626),
(#268627,#268628),(#268629,#268630),(#268631,#268632),(#268633,#268634),
(#268635,#268636),(#268637,#268638),(#268639,#268640),(#268641,#268642),
(#268643,#268644),(#268645,#268646),(#268647,#268648),(#268649,#268650),
(#268651,#268652),(#268653,#268654),(#268655,#268656),(#268657,#268658),
(#268659,#268660),(#268661,#268662),(#268663,#268664),(#268665,#268666),
(#268667,#268668),(#268669,#268670),(#268671,#268672),(#268673,#268674),
(#268675,#268676),(#268677,#268678),(#268679,#268680),(#268681,#268682),
(#268683,#268684),(#268685,#268686)),.UNSPECIFIED.,.F.,.F.,.F.,(6,1,1,1,
1,1,1,1,1,1,1,1,1,1,1,1,1,1,1,1,1,1,1,1,1,1,1,1,1,1,1,1,1,1,1,1,1,1,1,1,
1,1,1,1,1,1,1,1,1,1,1,1,1,1,1,1,1,1,1,1,1,1,1,1,1,1,1,1,1,1,1,1,1,1,1,1,
1,1,1,1,1,1,1,1,1,1,1,1,1,1,1,1,1,1,1,1,1,1,1,1,1,1,1,1,1,1,1,1,1,1,1,1,
1,1,1,1,1,1,1,1,1,1,1,1,1,1,1,1,1,1,1,1,1,1,1,1,1,1,1,1,1,1,1,1,1,1,1,1,
1,1,1,1,1,1,1,1,1,1,1,1,1,1,1,1,1,1,1,1,1,1,1,1,1,1,1,1,1,1,1,1,1,1,1,1,
1,1,1,1,1,1,1,1,1,1,1,1,1,1,1,1,1,1,1,1,1,1,1,1,1,1,1,1,1,1,1,1,1,1,1,1,
1,1,1,1,1,1,1,1,1,1,1,1,1,1,1,1,1,1,1,1,1,1,1,1,1,1,1,1,1,1,1,1,1,1,1,1,
1,1,1,1,1,1,1,1,1,1,1,1,1,1,1,1,1,1,1,1,1,1,1,1,1,1,1,1,1,1,1,1,1,1,1,1,
1,1,1,1,1,1,1,1,1,1,1,1,1,1,1,1,1,1,1,1,1,1,1,1,1,1,1,1,1,1,1,1,1,1,1,1,
1,1,1,1,1,1,1,1,1,1,1,1,1,1,1,1,1,1,1,1,1,1,1,1,1,1,1,1,1,1,1,1,1,1,1,1,
1,1,1,1,1,1,1,1,1,1,1,1,1,1,1,1,1,1,1,1,1,1,1,1,1,1,1,1,1,1,1,1,1,1,1,1,
1,1,1,1,1,1,1,1,1,1,1,1,1,1,1,1,1,1,1,1,1,1,1,1,1,1,1,1,1,1,1,1,1,1,1,1,
1,1,1,1,1,1,1,1,1,1,1,1,1,1,1,1,1,1,1,1,1,1,1,1,1,1,1,1,1,1,1,6),(2,2),
(-1.,-0.998165138,-0.996330275,-0.994495413,-0.99266055,-0.990825688,-0.988990826,
-0.987155963,-0.985321101,-0.983486239,-0.981651376,-0.979816514,-0.977981651,
-0.976146789,-0.974311927,-0.972477064,-0.970642202,-0.968807339,-0.966972477,
-0.965137615,-0.963302752,-0.96146789,-0.959633028,-0.957798165,-0.955963303,
-0.95412844,-0.952293578,-0.950458716,-0.948623853,-0.946788991,-0.944954128,
-0.943119266,-0.941284404,-0.939449541,-0.937614679,-0.935779817,-0.933944954,
-0.932110092,-0.930275229,-0.928440367,-0.926605505,-0.924770642,-0.92293578,
-0.921100917,-0.919266055,-0.917431193,-0.91559633,-0.913761468,-0.911926606,
-0.910091743,-0.908256881,-0.906422018,-0.904587156,-0.902752294,-0.900917431,
-0.899082569,-0.897247706,-0.895412844,-0.893577982,-0.891743119,-0.889908257,
-0.888073394,-0.886238532,-0.88440367,-0.882568807,-0.880733945,-0.878899083,
-0.87706422,-0.875229358,-0.873394495,-0.871559633,-0.869724771,-0.867889908,
-0.866055046,-0.864220183,-0.862385321,-0.860550459,-0.858715596,-0.856880734,
-0.855045872,-0.853211009,-0.851376147,-0.849541284,-0.847706422,-0.84587156,
-0.844036697,-0.842201835,-0.840366972,-0.83853211,-0.836697248,-0.834862385,
-0.833027523,-0.831192661,-0.829357798,-0.827522936,-0.825688073,-0.823853211,
-0.822018349,-0.820183486,-0.818348624,-0.816513761,-0.814678899,-0.812844037,
-0.811009174,-0.809174312,-0.80733945,-0.805504587,-0.803669725,-0.801834862,
-0.8,-0.798165138,-0.796330275,-0.794495413,-0.79266055,-0.790825688,-0.788990826,
-0.787155963,-0.785321101,-0.783486239,-0.781651376,-0.779816514,-0.777981651,
-0.776146789,-0.774311927,-0.772477064,-0.770642202,-0.768807339,-0.766972477,
-0.765137615,-0.763302752,-0.76146789,-0.759633028,-0.757798165,-0.755963303,
-0.75412844,-0.752293578,-0.750458716,-0.748623853,-0.746788991,-0.744954128,
-0.743119266,-0.741284404,-0.739449541,-0.737614679,-0.735779817,-0.733944954,
-0.732110092,-0.730275229,-0.728440367,-0.726605505,-0.724770642,-0.72293578,
-0.721100917,-0.719266055,-0.717431193,-0.71559633,-0.713761468,-0.711926606,
-0.710091743,-0.708256881,-0.706422018,-0.704587156,-0.702752294,-0.700917431,
-0.699082569,-0.697247706,-0.695412844,-0.693577982,-0.691743119,-0.689908257,
-0.688073394,-0.686238532,-0.68440367,-0.682568807,-0.680733945,-0.678899083,
-0.67706422,-0.675229358,-0.673394495,-0.671559633,-0.669724771,-0.667889908,
-0.666055046,-0.664220183,-0.662385321,-0.660550459,-0.658715596,-0.656880734,
-0.655045872,-0.653211009,-0.651376147,-0.649541284,-0.647706422,-0.64587156,
-0.644036697,-0.642201835,-0.640366972,-0.63853211,-0.636697248,-0.634862385,
-0.633027523,-0.631192661,-0.629357798,-0.627522936,-0.625688073,-0.623853211,
-0.622018349,-0.620183486,-0.618348624,-0.616513761,-0.614678899,-0.612844037,
-0.611009174,-0.609174312,-0.60733945,-0.605504587,-0.603669725,-0.601834862,
-0.6,-0.598165138,-0.596330275,-0.594495413,-0.59266055,-0.590825688,-0.588990826,
-0.587155963,-0.585321101,-0.583486239,-0.581651376,-0.579816514,-0.577981651,
-0.576146789,-0.574311927,-0.572477064,-0.570642202,-0.568807339,-0.566972477,
-0.565137615,-0.563302752,-0.56146789,-0.559633028,-0.557798165,-0.555963303,
-0.55412844,-0.552293578,-0.550458716,-0.548623853,-0.546788991,-0.544954128,
-0.543119266,-0.541284404,-0.539449541,-0.537614679,-0.535779817,-0.533944954,
-0.532110092,-0.530275229,-0.528440367,-0.526605505,-0.524770642,-0.52293578,
-0.521100917,-0.519266055,-0.517431193,-0.51559633,-0.513761468,-0.511926606,
-0.510091743,-0.508256881,-0.506422018,-0.504587156,-0.502752294,-0.500917431,
-0.499082569,-0.497247706,-0.495412844,-0.493577982,-0.491743119,-0.489908257,
-0.488073394,-0.486238532,-0.48440367,-0.482568807,-0.480733945,-0.478899083,
-0.47706422,-0.475229358,-0.473394495,-0.471559633,-0.469724771,-0.467889908,
-0.466055046,-0.464220183,-0.462385321,-0.460550459,-0.458715596,-0.456880734,
-0.455045872,-0.453211009,-0.451376147,-0.449541284,-0.447706422,-0.44587156,
-0.444036697,-0.442201835,-0.440366972,-0.43853211,-0.436697248,-0.434862385,
-0.433027523,-0.431192661,-0.429357798,-0.427522936,-0.425688073,-0.423853211,
-0.422018349,-0.420183486,-0.418348624,-0.416513761,-0.414678899,-0.412844037,
-0.411009174,-0.409174312,-0.40733945,-0.405504587,-0.403669725,-0.401834862,
-0.4,-0.398165138,-0.396330275,-0.394495413,-0.39266055,-0.390825688,-0.388990826,
-0.387155963,-0.385321101,-0.383486239,-0.381651376,-0.379816514,-0.377981651,
-0.376146789,-0.374311927,-0.372477064,-0.370642202,-0.368807339,-0.366972477,
-0.365137615,-0.363302752,-0.36146789,-0.359633028,-0.357798165,-0.355963303,
-0.35412844,-0.352293578,-0.350458716,-0.348623853,-0.346788991,-0.344954128,
-0.343119266,-0.341284404,-0.339449541,-0.337614679,-0.335779817,-0.333944954,
-0.332110092,-0.330275229,-0.328440367,-0.326605505,-0.324770642,-0.32293578,
-0.321100917,-0.319266055,-0.317431193,-0.31559633,-0.313761468,-0.311926606,
-0.310091743,-0.308256881,-0.306422018,-0.304587156,-0.302752294,-0.300917431,
-0.299082569,-0.297247706,-0.295412844,-0.293577982,-0.291743119,-0.289908257,
-0.288073394,-0.286238532,-0.28440367,-0.282568807,-0.280733945,-0.278899083,
-0.27706422,-0.275229358,-0.273394495,-0.271559633,-0.269724771,-0.267889908,
-0.266055046,-0.264220183,-0.262385321,-0.260550459,-0.258715596,-0.256880734,
-0.255045872,-0.253211009,-0.251376147,-0.249541284,-0.247706422,-0.24587156,
-0.244036697,-0.242201835,-0.240366972,-0.23853211,-0.236697248,-0.234862385,
-0.233027523,-0.231192661,-0.229357798,-0.227522936,-0.225688073,-0.223853211,
-0.222018349,-0.220183486,-0.218348624,-0.216513761,-0.214678899,-0.212844037,
-0.211009174,-0.209174312,-0.20733945,-0.205504587,-0.203669725,-0.201834862,
-0.2,-0.198165138,-0.196330275,-0.194495413,-0.19266055,-0.190825688,-0.188990826,
-0.187155963,-0.185321101,-0.183486239,-0.181651376,-0.179816514,-0.177981651,
-0.176146789,-0.174311927,-0.172477064,-0.170642202,-0.168807339,-0.166972477,
-0.165137615,-0.163302752,-0.16146789,-0.159633028,-0.157798165,-0.155963303,
-0.15412844,-0.152293578,-0.150458716,-0.148623853,-0.146788991,-0.144954128,
-0.143172103),(0.,0.36),.UNSPECIFIED.);
#6285=B_SPLINE_SURFACE_WITH_KNOTS('',5,1,((#269647,#269648),(#269649,#269650),
(#269651,#269652),(#269653,#269654),(#269655,#269656),(#269657,#269658),
(#269659,#269660),(#269661,#269662),(#269663,#269664),(#269665,#269666),
(#269667,#269668),(#269669,#269670),(#269671,#269672),(#269673,#269674),
(#269675,#269676),(#269677,#269678),(#269679,#269680),(#269681,#269682),
(#269683,#269684),(#269685,#269686),(#269687,#269688),(#269689,#269690),
(#269691,#269692),(#269693,#269694),(#269695,#269696),(#269697,#269698),
(#269699,#269700),(#269701,#269702),(#269703,#269704),(#269705,#269706),
(#269707,#269708),(#269709,#269710),(#269711,#269712),(#269713,#269714),
(#269715,#269716),(#269717,#269718),(#269719,#269720),(#269721,#269722),
(#269723,#269724),(#269725,#269726),(#269727,#269728),(#269729,#269730),
(#269731,#269732),(#269733,#269734),(#269735,#269736),(#269737,#269738),
(#269739,#269740),(#269741,#269742),(#269743,#269744),(#269745,#269746),
(#269747,#269748),(#269749,#269750),(#269751,#269752),(#269753,#269754),
(#269755,#269756),(#269757,#269758),(#269759,#269760),(#269761,#269762),
(#269763,#269764),(#269765,#269766),(#269767,#269768),(#269769,#269770),
(#269771,#269772),(#269773,#269774),(#269775,#269776),(#269777,#269778),
(#269779,#269780),(#269781,#269782),(#269783,#269784),(#269785,#269786),
(#269787,#269788),(#269789,#269790),(#269791,#269792),(#269793,#269794),
(#269795,#269796),(#269797,#269798),(#269799,#269800),(#269801,#269802),
(#269803,#269804),(#269805,#269806),(#269807,#269808),(#269809,#269810),
(#269811,#269812),(#269813,#269814),(#269815,#269816),(#269817,#269818),
(#269819,#269820),(#269821,#269822),(#269823,#269824),(#269825,#269826),
(#269827,#269828),(#269829,#269830),(#269831,#269832),(#269833,#269834),
(#269835,#269836),(#269837,#269838),(#269839,#269840),(#269841,#269842),
(#269843,#269844),(#269845,#269846),(#269847,#269848),(#269849,#269850),
(#269851,#269852),(#269853,#269854),(#269855,#269856),(#269857,#269858),
(#269859,#269860),(#269861,#269862),(#269863,#269864),(#269865,#269866),
(#269867,#269868),(#269869,#269870),(#269871,#269872),(#269873,#269874),
(#269875,#269876),(#269877,#269878),(#269879,#269880),(#269881,#269882),
(#269883,#269884),(#269885,#269886),(#269887,#269888),(#269889,#269890),
(#269891,#269892),(#269893,#269894),(#269895,#269896),(#269897,#269898),
(#269899,#269900),(#269901,#269902),(#269903,#269904),(#269905,#269906),
(#269907,#269908),(#269909,#269910),(#269911,#269912),(#269913,#269914),
(#269915,#269916),(#269917,#269918),(#269919,#269920),(#269921,#269922),
(#269923,#269924),(#269925,#269926),(#269927,#269928),(#269929,#269930),
(#269931,#269932),(#269933,#269934),(#269935,#269936),(#269937,#269938),
(#269939,#269940),(#269941,#269942),(#269943,#269944),(#269945,#269946),
(#269947,#269948),(#269949,#269950),(#269951,#269952),(#269953,#269954),
(#269955,#269956),(#269957,#269958),(#269959,#269960),(#269961,#269962),
(#269963,#269964),(#269965,#269966),(#269967,#269968),(#269969,#269970),
(#269971,#269972),(#269973,#269974),(#269975,#269976),(#269977,#269978),
(#269979,#269980),(#269981,#269982),(#269983,#269984),(#269985,#269986),
(#269987,#269988),(#269989,#269990),(#269991,#269992),(#269993,#269994),
(#269995,#269996),(#269997,#269998),(#269999,#270000),(#270001,#270002),
(#270003,#270004),(#270005,#270006),(#270007,#270008),(#270009,#270010),
(#270011,#270012),(#270013,#270014),(#270015,#270016),(#270017,#270018),
(#270019,#270020),(#270021,#270022),(#270023,#270024),(#270025,#270026),
(#270027,#270028),(#270029,#270030),(#270031,#270032),(#270033,#270034),
(#270035,#270036),(#270037,#270038),(#270039,#270040),(#270041,#270042),
(#270043,#270044),(#270045,#270046),(#270047,#270048),(#270049,#270050),
(#270051,#270052),(#270053,#270054),(#270055,#270056),(#270057,#270058),
(#270059,#270060),(#270061,#270062),(#270063,#270064),(#270065,#270066),
(#270067,#270068),(#270069,#270070),(#270071,#270072),(#270073,#270074),
(#270075,#270076),(#270077,#270078),(#270079,#270080),(#270081,#270082),
(#270083,#270084),(#270085,#270086),(#270087,#270088),(#270089,#270090),
(#270091,#270092),(#270093,#270094),(#270095,#270096),(#270097,#270098),
(#270099,#270100),(#270101,#270102),(#270103,#270104),(#270105,#270106),
(#270107,#270108),(#270109,#270110),(#270111,#270112),(#270113,#270114),
(#270115,#270116),(#270117,#270118),(#270119,#270120),(#270121,#270122),
(#270123,#270124),(#270125,#270126),(#270127,#270128),(#270129,#270130),
(#270131,#270132),(#270133,#270134),(#270135,#270136),(#270137,#270138),
(#270139,#270140),(#270141,#270142),(#270143,#270144),(#270145,#270146),
(#270147,#270148),(#270149,#270150),(#270151,#270152),(#270153,#270154),
(#270155,#270156),(#270157,#270158),(#270159,#270160),(#270161,#270162),
(#270163,#270164),(#270165,#270166),(#270167,#270168),(#270169,#270170),
(#270171,#270172),(#270173,#270174),(#270175,#270176),(#270177,#270178),
(#270179,#270180),(#270181,#270182),(#270183,#270184),(#270185,#270186),
(#270187,#270188),(#270189,#270190),(#270191,#270192),(#270193,#270194),
(#270195,#270196),(#270197,#270198),(#270199,#270200),(#270201,#270202),
(#270203,#270204),(#270205,#270206),(#270207,#270208),(#270209,#270210),
(#270211,#270212),(#270213,#270214),(#270215,#270216),(#270217,#270218),
(#270219,#270220),(#270221,#270222),(#270223,#270224),(#270225,#270226),
(#270227,#270228),(#270229,#270230),(#270231,#270232),(#270233,#270234),
(#270235,#270236),(#270237,#270238),(#270239,#270240),(#270241,#270242),
(#270243,#270244),(#270245,#270246),(#270247,#270248),(#270249,#270250),
(#270251,#270252),(#270253,#270254),(#270255,#270256),(#270257,#270258),
(#270259,#270260),(#270261,#270262),(#270263,#270264),(#270265,#270266),
(#270267,#270268),(#270269,#270270),(#270271,#270272),(#270273,#270274),
(#270275,#270276),(#270277,#270278),(#270279,#270280),(#270281,#270282),
(#270283,#270284),(#270285,#270286),(#270287,#270288),(#270289,#270290),
(#270291,#270292),(#270293,#270294),(#270295,#270296),(#270297,#270298),
(#270299,#270300),(#270301,#270302),(#270303,#270304),(#270305,#270306),
(#270307,#270308),(#270309,#270310),(#270311,#270312),(#270313,#270314),
(#270315,#270316),(#270317,#270318),(#270319,#270320),(#270321,#270322),
(#270323,#270324),(#270325,#270326),(#270327,#270328),(#270329,#270330),
(#270331,#270332),(#270333,#270334),(#270335,#270336),(#270337,#270338),
(#270339,#270340),(#270341,#270342),(#270343,#270344),(#270345,#270346),
(#270347,#270348),(#270349,#270350),(#270351,#270352),(#270353,#270354),
(#270355,#270356),(#270357,#270358),(#270359,#270360),(#270361,#270362),
(#270363,#270364),(#270365,#270366),(#270367,#270368),(#270369,#270370),
(#270371,#270372),(#270373,#270374),(#270375,#270376),(#270377,#270378),
(#270379,#270380),(#270381,#270382),(#270383,#270384),(#270385,#270386),
(#270387,#270388),(#270389,#270390),(#270391,#270392),(#270393,#270394),
(#270395,#270396),(#270397,#270398),(#270399,#270400),(#270401,#270402),
(#270403,#270404),(#270405,#270406),(#270407,#270408),(#270409,#270410),
(#270411,#270412),(#270413,#270414),(#270415,#270416),(#270417,#270418),
(#270419,#270420),(#270421,#270422),(#270423,#270424),(#270425,#270426),
(#270427,#270428),(#270429,#270430),(#270431,#270432),(#270433,#270434),
(#270435,#270436),(#270437,#270438),(#270439,#270440),(#270441,#270442),
(#270443,#270444),(#270445,#270446),(#270447,#270448),(#270449,#270450),
(#270451,#270452),(#270453,#270454),(#270455,#270456),(#270457,#270458),
(#270459,#270460),(#270461,#270462),(#270463,#270464),(#270465,#270466),
(#270467,#270468),(#270469,#270470),(#270471,#270472),(#270473,#270474),
(#270475,#270476),(#270477,#270478),(#270479,#270480),(#270481,#270482),
(#270483,#270484),(#270485,#270486),(#270487,#270488),(#270489,#270490),
(#270491,#270492),(#270493,#270494),(#270495,#270496),(#270497,#270498),
(#270499,#270500),(#270501,#270502),(#270503,#270504),(#270505,#270506),
(#270507,#270508),(#270509,#270510),(#270511,#270512),(#270513,#270514),
(#270515,#270516),(#270517,#270518),(#270519,#270520),(#270521,#270522),
(#270523,#270524),(#270525,#270526),(#270527,#270528),(#270529,#270530),
(#270531,#270532),(#270533,#270534),(#270535,#270536),(#270537,#270538),
(#270539,#270540),(#270541,#270542),(#270543,#270544),(#270545,#270546),
(#270547,#270548),(#270549,#270550),(#270551,#270552),(#270553,#270554),
(#270555,#270556),(#270557,#270558),(#270559,#270560),(#270561,#270562),
(#270563,#270564),(#270565,#270566),(#270567,#270568),(#270569,#270570),
(#270571,#270572),(#270573,#270574),(#270575,#270576),(#270577,#270578),
(#270579,#270580),(#270581,#270582),(#270583,#270584),(#270585,#270586),
(#270587,#270588),(#270589,#270590)),.UNSPECIFIED.,.F.,.F.,.F.,(6,1,1,1,
1,1,1,1,1,1,1,1,1,1,1,1,1,1,1,1,1,1,1,1,1,1,1,1,1,1,1,1,1,1,1,1,1,1,1,1,
1,1,1,1,1,1,1,1,1,1,1,1,1,1,1,1,1,1,1,1,1,1,1,1,1,1,1,1,1,1,1,1,1,1,1,1,
1,1,1,1,1,1,1,1,1,1,1,1,1,1,1,1,1,1,1,1,1,1,1,1,1,1,1,1,1,1,1,1,1,1,1,1,
1,1,1,1,1,1,1,1,1,1,1,1,1,1,1,1,1,1,1,1,1,1,1,1,1,1,1,1,1,1,1,1,1,1,1,1,
1,1,1,1,1,1,1,1,1,1,1,1,1,1,1,1,1,1,1,1,1,1,1,1,1,1,1,1,1,1,1,1,1,1,1,1,
1,1,1,1,1,1,1,1,1,1,1,1,1,1,1,1,1,1,1,1,1,1,1,1,1,1,1,1,1,1,1,1,1,1,1,1,
1,1,1,1,1,1,1,1,1,1,1,1,1,1,1,1,1,1,1,1,1,1,1,1,1,1,1,1,1,1,1,1,1,1,1,1,
1,1,1,1,1,1,1,1,1,1,1,1,1,1,1,1,1,1,1,1,1,1,1,1,1,1,1,1,1,1,1,1,1,1,1,1,
1,1,1,1,1,1,1,1,1,1,1,1,1,1,1,1,1,1,1,1,1,1,1,1,1,1,1,1,1,1,1,1,1,1,1,1,
1,1,1,1,1,1,1,1,1,1,1,1,1,1,1,1,1,1,1,1,1,1,1,1,1,1,1,1,1,1,1,1,1,1,1,1,
1,1,1,1,1,1,1,1,1,1,1,1,1,1,1,1,1,1,1,1,1,1,1,1,1,1,1,1,1,1,1,1,1,1,1,1,
1,1,1,1,1,1,1,1,1,1,1,1,1,1,1,1,1,1,1,1,1,1,1,1,1,1,1,1,1,1,1,1,1,1,1,1,
1,1,1,1,1,1,1,1,1,1,1,1,1,1,1,1,1,1,1,1,1,1,1,1,1,1,1,1,1,1,1,6),(2,2),
(-1.,-0.998165138,-0.996330275,-0.994495413,-0.99266055,-0.990825688,-0.988990826,
-0.987155963,-0.985321101,-0.983486239,-0.981651376,-0.979816514,-0.977981651,
-0.976146789,-0.974311927,-0.972477064,-0.970642202,-0.968807339,-0.966972477,
-0.965137615,-0.963302752,-0.96146789,-0.959633028,-0.957798165,-0.955963303,
-0.95412844,-0.952293578,-0.950458716,-0.948623853,-0.946788991,-0.944954128,
-0.943119266,-0.941284404,-0.939449541,-0.937614679,-0.935779817,-0.933944954,
-0.932110092,-0.930275229,-0.928440367,-0.926605505,-0.924770642,-0.92293578,
-0.921100917,-0.919266055,-0.917431193,-0.91559633,-0.913761468,-0.911926606,
-0.910091743,-0.908256881,-0.906422018,-0.904587156,-0.902752294,-0.900917431,
-0.899082569,-0.897247706,-0.895412844,-0.893577982,-0.891743119,-0.889908257,
-0.888073394,-0.886238532,-0.88440367,-0.882568807,-0.880733945,-0.878899083,
-0.87706422,-0.875229358,-0.873394495,-0.871559633,-0.869724771,-0.867889908,
-0.866055046,-0.864220183,-0.862385321,-0.860550459,-0.858715596,-0.856880734,
-0.855045872,-0.853211009,-0.851376147,-0.849541284,-0.847706422,-0.84587156,
-0.844036697,-0.842201835,-0.840366972,-0.83853211,-0.836697248,-0.834862385,
-0.833027523,-0.831192661,-0.829357798,-0.827522936,-0.825688073,-0.823853211,
-0.822018349,-0.820183486,-0.818348624,-0.816513761,-0.814678899,-0.812844037,
-0.811009174,-0.809174312,-0.80733945,-0.805504587,-0.803669725,-0.801834862,
-0.8,-0.798165138,-0.796330275,-0.794495413,-0.79266055,-0.790825688,-0.788990826,
-0.787155963,-0.785321101,-0.783486239,-0.781651376,-0.779816514,-0.777981651,
-0.776146789,-0.774311927,-0.772477064,-0.770642202,-0.768807339,-0.766972477,
-0.765137615,-0.763302752,-0.76146789,-0.759633028,-0.757798165,-0.755963303,
-0.75412844,-0.752293578,-0.750458716,-0.748623853,-0.746788991,-0.744954128,
-0.743119266,-0.741284404,-0.739449541,-0.737614679,-0.735779817,-0.733944954,
-0.732110092,-0.730275229,-0.728440367,-0.726605505,-0.724770642,-0.72293578,
-0.721100917,-0.719266055,-0.717431193,-0.71559633,-0.713761468,-0.711926606,
-0.710091743,-0.708256881,-0.706422018,-0.704587156,-0.702752294,-0.700917431,
-0.699082569,-0.697247706,-0.695412844,-0.693577982,-0.691743119,-0.689908257,
-0.688073394,-0.686238532,-0.68440367,-0.682568807,-0.680733945,-0.678899083,
-0.67706422,-0.675229358,-0.673394495,-0.671559633,-0.669724771,-0.667889908,
-0.666055046,-0.664220183,-0.662385321,-0.660550459,-0.658715596,-0.656880734,
-0.655045872,-0.653211009,-0.651376147,-0.649541284,-0.647706422,-0.64587156,
-0.644036697,-0.642201835,-0.640366972,-0.63853211,-0.636697248,-0.634862385,
-0.633027523,-0.631192661,-0.629357798,-0.627522936,-0.625688073,-0.623853211,
-0.622018349,-0.620183486,-0.618348624,-0.616513761,-0.614678899,-0.612844037,
-0.611009174,-0.609174312,-0.60733945,-0.605504587,-0.603669725,-0.601834862,
-0.6,-0.598165138,-0.596330275,-0.594495413,-0.59266055,-0.590825688,-0.588990826,
-0.587155963,-0.585321101,-0.583486239,-0.581651376,-0.579816514,-0.577981651,
-0.576146789,-0.574311927,-0.572477064,-0.570642202,-0.568807339,-0.566972477,
-0.565137615,-0.563302752,-0.56146789,-0.559633028,-0.557798165,-0.555963303,
-0.55412844,-0.552293578,-0.550458716,-0.548623853,-0.546788991,-0.544954128,
-0.543119266,-0.541284404,-0.539449541,-0.537614679,-0.535779817,-0.533944954,
-0.532110092,-0.530275229,-0.528440367,-0.526605505,-0.524770642,-0.52293578,
-0.521100917,-0.519266055,-0.517431193,-0.51559633,-0.513761468,-0.511926606,
-0.510091743,-0.508256881,-0.506422018,-0.504587156,-0.502752294,-0.500917431,
-0.499082569,-0.497247706,-0.495412844,-0.493577982,-0.491743119,-0.489908257,
-0.488073394,-0.486238532,-0.48440367,-0.482568807,-0.480733945,-0.478899083,
-0.47706422,-0.475229358,-0.473394495,-0.471559633,-0.469724771,-0.467889908,
-0.466055046,-0.464220183,-0.462385321,-0.460550459,-0.458715596,-0.456880734,
-0.455045872,-0.453211009,-0.451376147,-0.449541284,-0.447706422,-0.44587156,
-0.444036697,-0.442201835,-0.440366972,-0.43853211,-0.436697248,-0.434862385,
-0.433027523,-0.431192661,-0.429357798,-0.427522936,-0.425688073,-0.423853211,
-0.422018349,-0.420183486,-0.418348624,-0.416513761,-0.414678899,-0.412844037,
-0.411009174,-0.409174312,-0.40733945,-0.405504587,-0.403669725,-0.401834862,
-0.4,-0.398165138,-0.396330275,-0.394495413,-0.39266055,-0.390825688,-0.388990826,
-0.387155963,-0.385321101,-0.383486239,-0.381651376,-0.379816514,-0.377981651,
-0.376146789,-0.374311927,-0.372477064,-0.370642202,-0.368807339,-0.366972477,
-0.365137615,-0.363302752,-0.36146789,-0.359633028,-0.357798165,-0.355963303,
-0.35412844,-0.352293578,-0.350458716,-0.348623853,-0.346788991,-0.344954128,
-0.343119266,-0.341284404,-0.339449541,-0.337614679,-0.335779817,-0.333944954,
-0.332110092,-0.330275229,-0.328440367,-0.326605505,-0.324770642,-0.32293578,
-0.321100917,-0.319266055,-0.317431193,-0.31559633,-0.313761468,-0.311926606,
-0.310091743,-0.308256881,-0.306422018,-0.304587156,-0.302752294,-0.300917431,
-0.299082569,-0.297247706,-0.295412844,-0.293577982,-0.291743119,-0.289908257,
-0.288073394,-0.286238532,-0.28440367,-0.282568807,-0.280733945,-0.278899083,
-0.27706422,-0.275229358,-0.273394495,-0.271559633,-0.269724771,-0.267889908,
-0.266055046,-0.264220183,-0.262385321,-0.260550459,-0.258715596,-0.256880734,
-0.255045872,-0.253211009,-0.251376147,-0.249541284,-0.247706422,-0.24587156,
-0.244036697,-0.242201835,-0.240366972,-0.23853211,-0.236697248,-0.234862385,
-0.233027523,-0.231192661,-0.229357798,-0.227522936,-0.225688073,-0.223853211,
-0.222018349,-0.220183486,-0.218348624,-0.216513761,-0.214678899,-0.212844037,
-0.211009174,-0.209174312,-0.20733945,-0.205504587,-0.203669725,-0.201834862,
-0.2,-0.198165138,-0.196330275,-0.194495413,-0.19266055,-0.190825688,-0.188990826,
-0.187155963,-0.185321101,-0.183486239,-0.181651376,-0.179816514,-0.177981651,
-0.176146789,-0.174311927,-0.172477064,-0.170642202,-0.168807339,-0.166972477,
-0.165137615,-0.163302752,-0.16146789,-0.159633028,-0.157798165,-0.155963303,
-0.15412844,-0.152293578,-0.150458716,-0.148623853,-0.146788991,-0.144954128,
-0.143172103),(0.,0.36),.UNSPECIFIED.);
#6286=B_SPLINE_SURFACE_WITH_KNOTS('',5,1,((#271235,#271236),(#271237,#271238),
(#271239,#271240),(#271241,#271242),(#271243,#271244),(#271245,#271246),
(#271247,#271248),(#271249,#271250),(#271251,#271252),(#271253,#271254),
(#271255,#271256),(#271257,#271258),(#271259,#271260),(#271261,#271262),
(#271263,#271264),(#271265,#271266),(#271267,#271268),(#271269,#271270),
(#271271,#271272),(#271273,#271274),(#271275,#271276),(#271277,#271278),
(#271279,#271280),(#271281,#271282),(#271283,#271284),(#271285,#271286),
(#271287,#271288),(#271289,#271290),(#271291,#271292),(#271293,#271294),
(#271295,#271296),(#271297,#271298),(#271299,#271300),(#271301,#271302),
(#271303,#271304),(#271305,#271306),(#271307,#271308),(#271309,#271310),
(#271311,#271312),(#271313,#271314),(#271315,#271316),(#271317,#271318),
(#271319,#271320),(#271321,#271322),(#271323,#271324),(#271325,#271326),
(#271327,#271328),(#271329,#271330),(#271331,#271332),(#271333,#271334),
(#271335,#271336),(#271337,#271338),(#271339,#271340),(#271341,#271342),
(#271343,#271344),(#271345,#271346),(#271347,#271348),(#271349,#271350),
(#271351,#271352),(#271353,#271354),(#271355,#271356),(#271357,#271358),
(#271359,#271360),(#271361,#271362),(#271363,#271364),(#271365,#271366),
(#271367,#271368),(#271369,#271370),(#271371,#271372),(#271373,#271374),
(#271375,#271376),(#271377,#271378),(#271379,#271380),(#271381,#271382),
(#271383,#271384),(#271385,#271386),(#271387,#271388),(#271389,#271390),
(#271391,#271392),(#271393,#271394),(#271395,#271396),(#271397,#271398),
(#271399,#271400),(#271401,#271402),(#271403,#271404),(#271405,#271406),
(#271407,#271408),(#271409,#271410),(#271411,#271412),(#271413,#271414),
(#271415,#271416),(#271417,#271418),(#271419,#271420),(#271421,#271422),
(#271423,#271424),(#271425,#271426),(#271427,#271428),(#271429,#271430),
(#271431,#271432),(#271433,#271434),(#271435,#271436),(#271437,#271438),
(#271439,#271440),(#271441,#271442),(#271443,#271444),(#271445,#271446),
(#271447,#271448),(#271449,#271450),(#271451,#271452),(#271453,#271454),
(#271455,#271456),(#271457,#271458),(#271459,#271460),(#271461,#271462),
(#271463,#271464),(#271465,#271466),(#271467,#271468),(#271469,#271470),
(#271471,#271472),(#271473,#271474),(#271475,#271476),(#271477,#271478),
(#271479,#271480),(#271481,#271482),(#271483,#271484),(#271485,#271486),
(#271487,#271488),(#271489,#271490),(#271491,#271492),(#271493,#271494),
(#271495,#271496),(#271497,#271498),(#271499,#271500),(#271501,#271502),
(#271503,#271504),(#271505,#271506),(#271507,#271508),(#271509,#271510),
(#271511,#271512),(#271513,#271514),(#271515,#271516),(#271517,#271518),
(#271519,#271520),(#271521,#271522),(#271523,#271524),(#271525,#271526),
(#271527,#271528),(#271529,#271530),(#271531,#271532),(#271533,#271534),
(#271535,#271536),(#271537,#271538),(#271539,#271540),(#271541,#271542),
(#271543,#271544),(#271545,#271546),(#271547,#271548),(#271549,#271550),
(#271551,#271552),(#271553,#271554),(#271555,#271556),(#271557,#271558),
(#271559,#271560),(#271561,#271562),(#271563,#271564),(#271565,#271566),
(#271567,#271568),(#271569,#271570),(#271571,#271572),(#271573,#271574),
(#271575,#271576),(#271577,#271578),(#271579,#271580),(#271581,#271582),
(#271583,#271584),(#271585,#271586),(#271587,#271588),(#271589,#271590),
(#271591,#271592),(#271593,#271594),(#271595,#271596),(#271597,#271598),
(#271599,#271600),(#271601,#271602),(#271603,#271604),(#271605,#271606),
(#271607,#271608),(#271609,#271610),(#271611,#271612),(#271613,#271614),
(#271615,#271616),(#271617,#271618),(#271619,#271620),(#271621,#271622),
(#271623,#271624),(#271625,#271626),(#271627,#271628),(#271629,#271630),
(#271631,#271632),(#271633,#271634),(#271635,#271636),(#271637,#271638),
(#271639,#271640),(#271641,#271642),(#271643,#271644),(#271645,#271646),
(#271647,#271648),(#271649,#271650),(#271651,#271652),(#271653,#271654),
(#271655,#271656),(#271657,#271658),(#271659,#271660),(#271661,#271662),
(#271663,#271664),(#271665,#271666),(#271667,#271668),(#271669,#271670),
(#271671,#271672),(#271673,#271674),(#271675,#271676),(#271677,#271678),
(#271679,#271680),(#271681,#271682),(#271683,#271684),(#271685,#271686),
(#271687,#271688),(#271689,#271690),(#271691,#271692),(#271693,#271694),
(#271695,#271696),(#271697,#271698),(#271699,#271700),(#271701,#271702),
(#271703,#271704),(#271705,#271706),(#271707,#271708),(#271709,#271710),
(#271711,#271712),(#271713,#271714),(#271715,#271716),(#271717,#271718),
(#271719,#271720),(#271721,#271722),(#271723,#271724),(#271725,#271726),
(#271727,#271728),(#271729,#271730),(#271731,#271732),(#271733,#271734),
(#271735,#271736),(#271737,#271738),(#271739,#271740),(#271741,#271742),
(#271743,#271744),(#271745,#271746),(#271747,#271748),(#271749,#271750),
(#271751,#271752),(#271753,#271754),(#271755,#271756),(#271757,#271758),
(#271759,#271760),(#271761,#271762),(#271763,#271764),(#271765,#271766),
(#271767,#271768),(#271769,#271770),(#271771,#271772),(#271773,#271774),
(#271775,#271776),(#271777,#271778),(#271779,#271780),(#271781,#271782),
(#271783,#271784),(#271785,#271786),(#271787,#271788),(#271789,#271790),
(#271791,#271792),(#271793,#271794),(#271795,#271796),(#271797,#271798),
(#271799,#271800),(#271801,#271802),(#271803,#271804),(#271805,#271806),
(#271807,#271808),(#271809,#271810),(#271811,#271812),(#271813,#271814),
(#271815,#271816),(#271817,#271818),(#271819,#271820),(#271821,#271822),
(#271823,#271824),(#271825,#271826),(#271827,#271828),(#271829,#271830),
(#271831,#271832),(#271833,#271834),(#271835,#271836),(#271837,#271838),
(#271839,#271840),(#271841,#271842),(#271843,#271844),(#271845,#271846),
(#271847,#271848),(#271849,#271850),(#271851,#271852),(#271853,#271854),
(#271855,#271856),(#271857,#271858),(#271859,#271860),(#271861,#271862),
(#271863,#271864),(#271865,#271866),(#271867,#271868),(#271869,#271870),
(#271871,#271872),(#271873,#271874),(#271875,#271876),(#271877,#271878),
(#271879,#271880),(#271881,#271882),(#271883,#271884),(#271885,#271886),
(#271887,#271888),(#271889,#271890),(#271891,#271892),(#271893,#271894),
(#271895,#271896),(#271897,#271898),(#271899,#271900),(#271901,#271902),
(#271903,#271904),(#271905,#271906),(#271907,#271908),(#271909,#271910),
(#271911,#271912),(#271913,#271914),(#271915,#271916),(#271917,#271918),
(#271919,#271920),(#271921,#271922),(#271923,#271924),(#271925,#271926),
(#271927,#271928),(#271929,#271930),(#271931,#271932),(#271933,#271934),
(#271935,#271936),(#271937,#271938),(#271939,#271940),(#271941,#271942),
(#271943,#271944),(#271945,#271946),(#271947,#271948),(#271949,#271950),
(#271951,#271952),(#271953,#271954),(#271955,#271956),(#271957,#271958),
(#271959,#271960),(#271961,#271962),(#271963,#271964),(#271965,#271966),
(#271967,#271968),(#271969,#271970),(#271971,#271972),(#271973,#271974),
(#271975,#271976),(#271977,#271978),(#271979,#271980),(#271981,#271982),
(#271983,#271984),(#271985,#271986),(#271987,#271988),(#271989,#271990),
(#271991,#271992),(#271993,#271994),(#271995,#271996),(#271997,#271998),
(#271999,#272000),(#272001,#272002),(#272003,#272004),(#272005,#272006),
(#272007,#272008),(#272009,#272010),(#272011,#272012),(#272013,#272014),
(#272015,#272016),(#272017,#272018),(#272019,#272020),(#272021,#272022),
(#272023,#272024),(#272025,#272026),(#272027,#272028),(#272029,#272030),
(#272031,#272032),(#272033,#272034),(#272035,#272036),(#272037,#272038),
(#272039,#272040),(#272041,#272042),(#272043,#272044),(#272045,#272046),
(#272047,#272048),(#272049,#272050),(#272051,#272052),(#272053,#272054),
(#272055,#272056),(#272057,#272058),(#272059,#272060),(#272061,#272062),
(#272063,#272064),(#272065,#272066),(#272067,#272068),(#272069,#272070),
(#272071,#272072),(#272073,#272074),(#272075,#272076),(#272077,#272078),
(#272079,#272080),(#272081,#272082),(#272083,#272084),(#272085,#272086),
(#272087,#272088),(#272089,#272090),(#272091,#272092),(#272093,#272094),
(#272095,#272096),(#272097,#272098),(#272099,#272100),(#272101,#272102),
(#272103,#272104),(#272105,#272106),(#272107,#272108),(#272109,#272110),
(#272111,#272112),(#272113,#272114),(#272115,#272116),(#272117,#272118),
(#272119,#272120),(#272121,#272122),(#272123,#272124),(#272125,#272126),
(#272127,#272128),(#272129,#272130),(#272131,#272132),(#272133,#272134),
(#272135,#272136),(#272137,#272138),(#272139,#272140),(#272141,#272142),
(#272143,#272144),(#272145,#272146),(#272147,#272148),(#272149,#272150),
(#272151,#272152),(#272153,#272154),(#272155,#272156),(#272157,#272158),
(#272159,#272160),(#272161,#272162),(#272163,#272164),(#272165,#272166),
(#272167,#272168),(#272169,#272170),(#272171,#272172),(#272173,#272174),
(#272175,#272176),(#272177,#272178)),.UNSPECIFIED.,.F.,.F.,.F.,(6,1,1,1,
1,1,1,1,1,1,1,1,1,1,1,1,1,1,1,1,1,1,1,1,1,1,1,1,1,1,1,1,1,1,1,1,1,1,1,1,
1,1,1,1,1,1,1,1,1,1,1,1,1,1,1,1,1,1,1,1,1,1,1,1,1,1,1,1,1,1,1,1,1,1,1,1,
1,1,1,1,1,1,1,1,1,1,1,1,1,1,1,1,1,1,1,1,1,1,1,1,1,1,1,1,1,1,1,1,1,1,1,1,
1,1,1,1,1,1,1,1,1,1,1,1,1,1,1,1,1,1,1,1,1,1,1,1,1,1,1,1,1,1,1,1,1,1,1,1,
1,1,1,1,1,1,1,1,1,1,1,1,1,1,1,1,1,1,1,1,1,1,1,1,1,1,1,1,1,1,1,1,1,1,1,1,
1,1,1,1,1,1,1,1,1,1,1,1,1,1,1,1,1,1,1,1,1,1,1,1,1,1,1,1,1,1,1,1,1,1,1,1,
1,1,1,1,1,1,1,1,1,1,1,1,1,1,1,1,1,1,1,1,1,1,1,1,1,1,1,1,1,1,1,1,1,1,1,1,
1,1,1,1,1,1,1,1,1,1,1,1,1,1,1,1,1,1,1,1,1,1,1,1,1,1,1,1,1,1,1,1,1,1,1,1,
1,1,1,1,1,1,1,1,1,1,1,1,1,1,1,1,1,1,1,1,1,1,1,1,1,1,1,1,1,1,1,1,1,1,1,1,
1,1,1,1,1,1,1,1,1,1,1,1,1,1,1,1,1,1,1,1,1,1,1,1,1,1,1,1,1,1,1,1,1,1,1,1,
1,1,1,1,1,1,1,1,1,1,1,1,1,1,1,1,1,1,1,1,1,1,1,1,1,1,1,1,1,1,1,1,1,1,1,1,
1,1,1,1,1,1,1,1,1,1,1,1,1,1,1,1,1,1,1,1,1,1,1,1,1,1,1,1,1,1,1,1,1,1,1,1,
1,1,1,1,1,1,1,1,1,1,1,1,1,1,1,1,1,1,1,1,1,1,1,1,1,1,1,1,1,1,1,6),(2,2),
(0.143172103,0.144954128,0.146788991,0.148623853,0.150458716,0.152293578,
0.15412844,0.155963303,0.157798165,0.159633028,0.16146789,0.163302752,0.165137615,
0.166972477,0.168807339,0.170642202,0.172477064,0.174311927,0.176146789,
0.177981651,0.179816514,0.181651376,0.183486239,0.185321101,0.187155963,
0.188990826,0.190825688,0.19266055,0.194495413,0.196330275,0.198165138,
0.2,0.201834862,0.203669725,0.205504587,0.20733945,0.209174312,0.211009174,
0.212844037,0.214678899,0.216513761,0.218348624,0.220183486,0.222018349,
0.223853211,0.225688073,0.227522936,0.229357798,0.231192661,0.233027523,
0.234862385,0.236697248,0.23853211,0.240366972,0.242201835,0.244036697,
0.24587156,0.247706422,0.249541284,0.251376147,0.253211009,0.255045872,
0.256880734,0.258715596,0.260550459,0.262385321,0.264220183,0.266055046,
0.267889908,0.269724771,0.271559633,0.273394495,0.275229358,0.27706422,
0.278899083,0.280733945,0.282568807,0.28440367,0.286238532,0.288073394,
0.289908257,0.291743119,0.293577982,0.295412844,0.297247706,0.299082569,
0.300917431,0.302752294,0.304587156,0.306422018,0.308256881,0.310091743,
0.311926606,0.313761468,0.31559633,0.317431193,0.319266055,0.321100917,
0.32293578,0.324770642,0.326605505,0.328440367,0.330275229,0.332110092,
0.333944954,0.335779817,0.337614679,0.339449541,0.341284404,0.343119266,
0.344954128,0.346788991,0.348623853,0.350458716,0.352293578,0.35412844,
0.355963303,0.357798165,0.359633028,0.36146789,0.363302752,0.365137615,
0.366972477,0.368807339,0.370642202,0.372477064,0.374311927,0.376146789,
0.377981651,0.379816514,0.381651376,0.383486239,0.385321101,0.387155963,
0.388990826,0.390825688,0.39266055,0.394495413,0.396330275,0.398165138,
0.4,0.401834862,0.403669725,0.405504587,0.40733945,0.409174312,0.411009174,
0.412844037,0.414678899,0.416513761,0.418348624,0.420183486,0.422018349,
0.423853211,0.425688073,0.427522936,0.429357798,0.431192661,0.433027523,
0.434862385,0.436697248,0.43853211,0.440366972,0.442201835,0.444036697,
0.44587156,0.447706422,0.449541284,0.451376147,0.453211009,0.455045872,
0.456880734,0.458715596,0.460550459,0.462385321,0.464220183,0.466055046,
0.467889908,0.469724771,0.471559633,0.473394495,0.475229358,0.47706422,
0.478899083,0.480733945,0.482568807,0.48440367,0.486238532,0.488073394,
0.489908257,0.491743119,0.493577982,0.495412844,0.497247706,0.499082569,
0.500917431,0.502752294,0.504587156,0.506422018,0.508256881,0.510091743,
0.511926606,0.513761468,0.51559633,0.517431193,0.519266055,0.521100917,
0.52293578,0.524770642,0.526605505,0.528440367,0.530275229,0.532110092,
0.533944954,0.535779817,0.537614679,0.539449541,0.541284404,0.543119266,
0.544954128,0.546788991,0.548623853,0.550458716,0.552293578,0.55412844,
0.555963303,0.557798165,0.559633028,0.56146789,0.563302752,0.565137615,
0.566972477,0.568807339,0.570642202,0.572477064,0.574311927,0.576146789,
0.577981651,0.579816514,0.581651376,0.583486239,0.585321101,0.587155963,
0.588990826,0.590825688,0.59266055,0.594495413,0.596330275,0.598165138,
0.6,0.601834862,0.603669725,0.605504587,0.60733945,0.609174312,0.611009174,
0.612844037,0.614678899,0.616513761,0.618348624,0.620183486,0.622018349,
0.623853211,0.625688073,0.627522936,0.629357798,0.631192661,0.633027523,
0.634862385,0.636697248,0.63853211,0.640366972,0.642201835,0.644036697,
0.64587156,0.647706422,0.649541284,0.651376147,0.653211009,0.655045872,
0.656880734,0.658715596,0.660550459,0.662385321,0.664220183,0.666055046,
0.667889908,0.669724771,0.671559633,0.673394495,0.675229358,0.67706422,
0.678899083,0.680733945,0.682568807,0.68440367,0.686238532,0.688073394,
0.689908257,0.691743119,0.693577982,0.695412844,0.697247706,0.699082569,
0.700917431,0.702752294,0.704587156,0.706422018,0.708256881,0.710091743,
0.711926606,0.713761468,0.71559633,0.717431193,0.719266055,0.721100917,
0.72293578,0.724770642,0.726605505,0.728440367,0.730275229,0.732110092,
0.733944954,0.735779817,0.737614679,0.739449541,0.741284404,0.743119266,
0.744954128,0.746788991,0.748623853,0.750458716,0.752293578,0.75412844,
0.755963303,0.757798165,0.759633028,0.76146789,0.763302752,0.765137615,
0.766972477,0.768807339,0.770642202,0.772477064,0.774311927,0.776146789,
0.777981651,0.779816514,0.781651376,0.783486239,0.785321101,0.787155963,
0.788990826,0.790825688,0.79266055,0.794495413,0.796330275,0.798165138,
0.8,0.801834862,0.803669725,0.805504587,0.80733945,0.809174312,0.811009174,
0.812844037,0.814678899,0.816513761,0.818348624,0.820183486,0.822018349,
0.823853211,0.825688073,0.827522936,0.829357798,0.831192661,0.833027523,
0.834862385,0.836697248,0.83853211,0.840366972,0.842201835,0.844036697,
0.84587156,0.847706422,0.849541284,0.851376147,0.853211009,0.855045872,
0.856880734,0.858715596,0.860550459,0.862385321,0.864220183,0.866055046,
0.867889908,0.869724771,0.871559633,0.873394495,0.875229358,0.87706422,
0.878899083,0.880733945,0.882568807,0.88440367,0.886238532,0.888073394,
0.889908257,0.891743119,0.893577982,0.895412844,0.897247706,0.899082569,
0.900917431,0.902752294,0.904587156,0.906422018,0.908256881,0.910091743,
0.911926606,0.913761468,0.91559633,0.917431193,0.919266055,0.921100917,
0.92293578,0.924770642,0.926605505,0.928440367,0.930275229,0.932110092,
0.933944954,0.935779817,0.937614679,0.939449541,0.941284404,0.943119266,
0.944954128,0.946788991,0.948623853,0.950458716,0.952293578,0.95412844,
0.955963303,0.957798165,0.959633028,0.96146789,0.963302752,0.965137615,
0.966972477,0.968807339,0.970642202,0.972477064,0.974311927,0.976146789,
0.977981651,0.979816514,0.981651376,0.983486239,0.985321101,0.987155963,
0.988990826,0.990825688,0.99266055,0.994495413,0.996330275,0.998165138,
1.),(0.,0.36),.UNSPECIFIED.);
#6287=B_SPLINE_SURFACE_WITH_KNOTS('',5,1,((#272844,#272845),(#272846,#272847),
(#272848,#272849),(#272850,#272851),(#272852,#272853),(#272854,#272855),
(#272856,#272857),(#272858,#272859),(#272860,#272861),(#272862,#272863),
(#272864,#272865),(#272866,#272867),(#272868,#272869),(#272870,#272871),
(#272872,#272873),(#272874,#272875),(#272876,#272877),(#272878,#272879),
(#272880,#272881),(#272882,#272883),(#272884,#272885),(#272886,#272887),
(#272888,#272889),(#272890,#272891),(#272892,#272893),(#272894,#272895),
(#272896,#272897),(#272898,#272899),(#272900,#272901),(#272902,#272903),
(#272904,#272905),(#272906,#272907),(#272908,#272909),(#272910,#272911),
(#272912,#272913),(#272914,#272915),(#272916,#272917),(#272918,#272919),
(#272920,#272921),(#272922,#272923),(#272924,#272925),(#272926,#272927),
(#272928,#272929),(#272930,#272931),(#272932,#272933),(#272934,#272935),
(#272936,#272937),(#272938,#272939),(#272940,#272941),(#272942,#272943),
(#272944,#272945),(#272946,#272947),(#272948,#272949),(#272950,#272951),
(#272952,#272953),(#272954,#272955),(#272956,#272957),(#272958,#272959),
(#272960,#272961),(#272962,#272963),(#272964,#272965),(#272966,#272967),
(#272968,#272969),(#272970,#272971),(#272972,#272973),(#272974,#272975),
(#272976,#272977),(#272978,#272979),(#272980,#272981),(#272982,#272983),
(#272984,#272985),(#272986,#272987),(#272988,#272989),(#272990,#272991),
(#272992,#272993),(#272994,#272995),(#272996,#272997),(#272998,#272999),
(#273000,#273001),(#273002,#273003),(#273004,#273005),(#273006,#273007),
(#273008,#273009),(#273010,#273011),(#273012,#273013),(#273014,#273015),
(#273016,#273017),(#273018,#273019),(#273020,#273021),(#273022,#273023),
(#273024,#273025),(#273026,#273027),(#273028,#273029),(#273030,#273031),
(#273032,#273033),(#273034,#273035),(#273036,#273037),(#273038,#273039),
(#273040,#273041),(#273042,#273043),(#273044,#273045),(#273046,#273047),
(#273048,#273049),(#273050,#273051),(#273052,#273053),(#273054,#273055),
(#273056,#273057),(#273058,#273059),(#273060,#273061),(#273062,#273063),
(#273064,#273065),(#273066,#273067),(#273068,#273069),(#273070,#273071),
(#273072,#273073),(#273074,#273075),(#273076,#273077),(#273078,#273079),
(#273080,#273081),(#273082,#273083),(#273084,#273085),(#273086,#273087),
(#273088,#273089),(#273090,#273091),(#273092,#273093),(#273094,#273095),
(#273096,#273097),(#273098,#273099),(#273100,#273101),(#273102,#273103),
(#273104,#273105),(#273106,#273107),(#273108,#273109),(#273110,#273111),
(#273112,#273113),(#273114,#273115),(#273116,#273117),(#273118,#273119),
(#273120,#273121),(#273122,#273123),(#273124,#273125),(#273126,#273127),
(#273128,#273129),(#273130,#273131),(#273132,#273133),(#273134,#273135),
(#273136,#273137),(#273138,#273139),(#273140,#273141),(#273142,#273143),
(#273144,#273145),(#273146,#273147),(#273148,#273149),(#273150,#273151),
(#273152,#273153),(#273154,#273155),(#273156,#273157),(#273158,#273159),
(#273160,#273161),(#273162,#273163),(#273164,#273165),(#273166,#273167),
(#273168,#273169),(#273170,#273171),(#273172,#273173),(#273174,#273175),
(#273176,#273177),(#273178,#273179),(#273180,#273181),(#273182,#273183),
(#273184,#273185),(#273186,#273187),(#273188,#273189),(#273190,#273191),
(#273192,#273193),(#273194,#273195),(#273196,#273197),(#273198,#273199),
(#273200,#273201),(#273202,#273203),(#273204,#273205),(#273206,#273207),
(#273208,#273209),(#273210,#273211),(#273212,#273213),(#273214,#273215),
(#273216,#273217),(#273218,#273219),(#273220,#273221),(#273222,#273223),
(#273224,#273225),(#273226,#273227),(#273228,#273229),(#273230,#273231),
(#273232,#273233),(#273234,#273235),(#273236,#273237),(#273238,#273239),
(#273240,#273241),(#273242,#273243),(#273244,#273245),(#273246,#273247),
(#273248,#273249),(#273250,#273251),(#273252,#273253),(#273254,#273255),
(#273256,#273257),(#273258,#273259),(#273260,#273261),(#273262,#273263),
(#273264,#273265),(#273266,#273267),(#273268,#273269),(#273270,#273271),
(#273272,#273273),(#273274,#273275),(#273276,#273277),(#273278,#273279),
(#273280,#273281),(#273282,#273283),(#273284,#273285),(#273286,#273287),
(#273288,#273289),(#273290,#273291),(#273292,#273293),(#273294,#273295),
(#273296,#273297),(#273298,#273299),(#273300,#273301),(#273302,#273303),
(#273304,#273305),(#273306,#273307),(#273308,#273309),(#273310,#273311),
(#273312,#273313),(#273314,#273315),(#273316,#273317),(#273318,#273319),
(#273320,#273321),(#273322,#273323),(#273324,#273325),(#273326,#273327),
(#273328,#273329),(#273330,#273331),(#273332,#273333),(#273334,#273335),
(#273336,#273337),(#273338,#273339),(#273340,#273341),(#273342,#273343),
(#273344,#273345),(#273346,#273347),(#273348,#273349),(#273350,#273351),
(#273352,#273353),(#273354,#273355),(#273356,#273357),(#273358,#273359),
(#273360,#273361),(#273362,#273363),(#273364,#273365),(#273366,#273367),
(#273368,#273369),(#273370,#273371),(#273372,#273373),(#273374,#273375),
(#273376,#273377),(#273378,#273379),(#273380,#273381),(#273382,#273383),
(#273384,#273385),(#273386,#273387),(#273388,#273389),(#273390,#273391),
(#273392,#273393),(#273394,#273395),(#273396,#273397),(#273398,#273399),
(#273400,#273401),(#273402,#273403),(#273404,#273405),(#273406,#273407),
(#273408,#273409),(#273410,#273411),(#273412,#273413),(#273414,#273415),
(#273416,#273417),(#273418,#273419),(#273420,#273421),(#273422,#273423),
(#273424,#273425),(#273426,#273427),(#273428,#273429),(#273430,#273431),
(#273432,#273433),(#273434,#273435),(#273436,#273437),(#273438,#273439),
(#273440,#273441),(#273442,#273443),(#273444,#273445),(#273446,#273447),
(#273448,#273449),(#273450,#273451),(#273452,#273453),(#273454,#273455),
(#273456,#273457),(#273458,#273459),(#273460,#273461),(#273462,#273463),
(#273464,#273465),(#273466,#273467),(#273468,#273469),(#273470,#273471),
(#273472,#273473),(#273474,#273475),(#273476,#273477),(#273478,#273479),
(#273480,#273481),(#273482,#273483),(#273484,#273485),(#273486,#273487),
(#273488,#273489),(#273490,#273491),(#273492,#273493),(#273494,#273495),
(#273496,#273497),(#273498,#273499),(#273500,#273501),(#273502,#273503),
(#273504,#273505),(#273506,#273507),(#273508,#273509),(#273510,#273511),
(#273512,#273513),(#273514,#273515),(#273516,#273517),(#273518,#273519),
(#273520,#273521),(#273522,#273523),(#273524,#273525),(#273526,#273527),
(#273528,#273529),(#273530,#273531),(#273532,#273533),(#273534,#273535),
(#273536,#273537),(#273538,#273539),(#273540,#273541),(#273542,#273543),
(#273544,#273545),(#273546,#273547),(#273548,#273549),(#273550,#273551),
(#273552,#273553),(#273554,#273555),(#273556,#273557),(#273558,#273559),
(#273560,#273561),(#273562,#273563),(#273564,#273565),(#273566,#273567),
(#273568,#273569),(#273570,#273571),(#273572,#273573),(#273574,#273575),
(#273576,#273577),(#273578,#273579),(#273580,#273581),(#273582,#273583),
(#273584,#273585),(#273586,#273587),(#273588,#273589),(#273590,#273591),
(#273592,#273593),(#273594,#273595),(#273596,#273597),(#273598,#273599),
(#273600,#273601),(#273602,#273603),(#273604,#273605),(#273606,#273607),
(#273608,#273609),(#273610,#273611),(#273612,#273613),(#273614,#273615),
(#273616,#273617),(#273618,#273619),(#273620,#273621),(#273622,#273623),
(#273624,#273625),(#273626,#273627),(#273628,#273629),(#273630,#273631),
(#273632,#273633),(#273634,#273635),(#273636,#273637),(#273638,#273639),
(#273640,#273641),(#273642,#273643),(#273644,#273645),(#273646,#273647),
(#273648,#273649),(#273650,#273651),(#273652,#273653),(#273654,#273655),
(#273656,#273657),(#273658,#273659),(#273660,#273661),(#273662,#273663),
(#273664,#273665),(#273666,#273667),(#273668,#273669),(#273670,#273671),
(#273672,#273673),(#273674,#273675),(#273676,#273677),(#273678,#273679),
(#273680,#273681),(#273682,#273683),(#273684,#273685),(#273686,#273687),
(#273688,#273689),(#273690,#273691),(#273692,#273693),(#273694,#273695),
(#273696,#273697),(#273698,#273699),(#273700,#273701),(#273702,#273703),
(#273704,#273705),(#273706,#273707),(#273708,#273709),(#273710,#273711),
(#273712,#273713),(#273714,#273715),(#273716,#273717),(#273718,#273719),
(#273720,#273721),(#273722,#273723),(#273724,#273725),(#273726,#273727),
(#273728,#273729),(#273730,#273731),(#273732,#273733),(#273734,#273735),
(#273736,#273737),(#273738,#273739),(#273740,#273741),(#273742,#273743),
(#273744,#273745),(#273746,#273747),(#273748,#273749),(#273750,#273751),
(#273752,#273753),(#273754,#273755),(#273756,#273757),(#273758,#273759),
(#273760,#273761),(#273762,#273763),(#273764,#273765),(#273766,#273767),
(#273768,#273769),(#273770,#273771),(#273772,#273773),(#273774,#273775),
(#273776,#273777),(#273778,#273779),(#273780,#273781),(#273782,#273783),
(#273784,#273785),(#273786,#273787)),.UNSPECIFIED.,.F.,.F.,.F.,(6,1,1,1,
1,1,1,1,1,1,1,1,1,1,1,1,1,1,1,1,1,1,1,1,1,1,1,1,1,1,1,1,1,1,1,1,1,1,1,1,
1,1,1,1,1,1,1,1,1,1,1,1,1,1,1,1,1,1,1,1,1,1,1,1,1,1,1,1,1,1,1,1,1,1,1,1,
1,1,1,1,1,1,1,1,1,1,1,1,1,1,1,1,1,1,1,1,1,1,1,1,1,1,1,1,1,1,1,1,1,1,1,1,
1,1,1,1,1,1,1,1,1,1,1,1,1,1,1,1,1,1,1,1,1,1,1,1,1,1,1,1,1,1,1,1,1,1,1,1,
1,1,1,1,1,1,1,1,1,1,1,1,1,1,1,1,1,1,1,1,1,1,1,1,1,1,1,1,1,1,1,1,1,1,1,1,
1,1,1,1,1,1,1,1,1,1,1,1,1,1,1,1,1,1,1,1,1,1,1,1,1,1,1,1,1,1,1,1,1,1,1,1,
1,1,1,1,1,1,1,1,1,1,1,1,1,1,1,1,1,1,1,1,1,1,1,1,1,1,1,1,1,1,1,1,1,1,1,1,
1,1,1,1,1,1,1,1,1,1,1,1,1,1,1,1,1,1,1,1,1,1,1,1,1,1,1,1,1,1,1,1,1,1,1,1,
1,1,1,1,1,1,1,1,1,1,1,1,1,1,1,1,1,1,1,1,1,1,1,1,1,1,1,1,1,1,1,1,1,1,1,1,
1,1,1,1,1,1,1,1,1,1,1,1,1,1,1,1,1,1,1,1,1,1,1,1,1,1,1,1,1,1,1,1,1,1,1,1,
1,1,1,1,1,1,1,1,1,1,1,1,1,1,1,1,1,1,1,1,1,1,1,1,1,1,1,1,1,1,1,1,1,1,1,1,
1,1,1,1,1,1,1,1,1,1,1,1,1,1,1,1,1,1,1,1,1,1,1,1,1,1,1,1,1,1,1,1,1,1,1,1,
1,1,1,1,1,1,1,1,1,1,1,1,1,1,1,1,1,1,1,1,1,1,1,1,1,1,1,1,1,1,1,6),(2,2),
(0.143172103,0.144954128,0.146788991,0.148623853,0.150458716,0.152293578,
0.15412844,0.155963303,0.157798165,0.159633028,0.16146789,0.163302752,0.165137615,
0.166972477,0.168807339,0.170642202,0.172477064,0.174311927,0.176146789,
0.177981651,0.179816514,0.181651376,0.183486239,0.185321101,0.187155963,
0.188990826,0.190825688,0.19266055,0.194495413,0.196330275,0.198165138,
0.2,0.201834862,0.203669725,0.205504587,0.20733945,0.209174312,0.211009174,
0.212844037,0.214678899,0.216513761,0.218348624,0.220183486,0.222018349,
0.223853211,0.225688073,0.227522936,0.229357798,0.231192661,0.233027523,
0.234862385,0.236697248,0.23853211,0.240366972,0.242201835,0.244036697,
0.24587156,0.247706422,0.249541284,0.251376147,0.253211009,0.255045872,
0.256880734,0.258715596,0.260550459,0.262385321,0.264220183,0.266055046,
0.267889908,0.269724771,0.271559633,0.273394495,0.275229358,0.27706422,
0.278899083,0.280733945,0.282568807,0.28440367,0.286238532,0.288073394,
0.289908257,0.291743119,0.293577982,0.295412844,0.297247706,0.299082569,
0.300917431,0.302752294,0.304587156,0.306422018,0.308256881,0.310091743,
0.311926606,0.313761468,0.31559633,0.317431193,0.319266055,0.321100917,
0.32293578,0.324770642,0.326605505,0.328440367,0.330275229,0.332110092,
0.333944954,0.335779817,0.337614679,0.339449541,0.341284404,0.343119266,
0.344954128,0.346788991,0.348623853,0.350458716,0.352293578,0.35412844,
0.355963303,0.357798165,0.359633028,0.36146789,0.363302752,0.365137615,
0.366972477,0.368807339,0.370642202,0.372477064,0.374311927,0.376146789,
0.377981651,0.379816514,0.381651376,0.383486239,0.385321101,0.387155963,
0.388990826,0.390825688,0.39266055,0.394495413,0.396330275,0.398165138,
0.4,0.401834862,0.403669725,0.405504587,0.40733945,0.409174312,0.411009174,
0.412844037,0.414678899,0.416513761,0.418348624,0.420183486,0.422018349,
0.423853211,0.425688073,0.427522936,0.429357798,0.431192661,0.433027523,
0.434862385,0.436697248,0.43853211,0.440366972,0.442201835,0.444036697,
0.44587156,0.447706422,0.449541284,0.451376147,0.453211009,0.455045872,
0.456880734,0.458715596,0.460550459,0.462385321,0.464220183,0.466055046,
0.467889908,0.469724771,0.471559633,0.473394495,0.475229358,0.47706422,
0.478899083,0.480733945,0.482568807,0.48440367,0.486238532,0.488073394,
0.489908257,0.491743119,0.493577982,0.495412844,0.497247706,0.499082569,
0.500917431,0.502752294,0.504587156,0.506422018,0.508256881,0.510091743,
0.511926606,0.513761468,0.51559633,0.517431193,0.519266055,0.521100917,
0.52293578,0.524770642,0.526605505,0.528440367,0.530275229,0.532110092,
0.533944954,0.535779817,0.537614679,0.539449541,0.541284404,0.543119266,
0.544954128,0.546788991,0.548623853,0.550458716,0.552293578,0.55412844,
0.555963303,0.557798165,0.559633028,0.56146789,0.563302752,0.565137615,
0.566972477,0.568807339,0.570642202,0.572477064,0.574311927,0.576146789,
0.577981651,0.579816514,0.581651376,0.583486239,0.585321101,0.587155963,
0.588990826,0.590825688,0.59266055,0.594495413,0.596330275,0.598165138,
0.6,0.601834862,0.603669725,0.605504587,0.60733945,0.609174312,0.611009174,
0.612844037,0.614678899,0.616513761,0.618348624,0.620183486,0.622018349,
0.623853211,0.625688073,0.627522936,0.629357798,0.631192661,0.633027523,
0.634862385,0.636697248,0.63853211,0.640366972,0.642201835,0.644036697,
0.64587156,0.647706422,0.649541284,0.651376147,0.653211009,0.655045872,
0.656880734,0.658715596,0.660550459,0.662385321,0.664220183,0.666055046,
0.667889908,0.669724771,0.671559633,0.673394495,0.675229358,0.67706422,
0.678899083,0.680733945,0.682568807,0.68440367,0.686238532,0.688073394,
0.689908257,0.691743119,0.693577982,0.695412844,0.697247706,0.699082569,
0.700917431,0.702752294,0.704587156,0.706422018,0.708256881,0.710091743,
0.711926606,0.713761468,0.71559633,0.717431193,0.719266055,0.721100917,
0.72293578,0.724770642,0.726605505,0.728440367,0.730275229,0.732110092,
0.733944954,0.735779817,0.737614679,0.739449541,0.741284404,0.743119266,
0.744954128,0.746788991,0.748623853,0.750458716,0.752293578,0.75412844,
0.755963303,0.757798165,0.759633028,0.76146789,0.763302752,0.765137615,
0.766972477,0.768807339,0.770642202,0.772477064,0.774311927,0.776146789,
0.777981651,0.779816514,0.781651376,0.783486239,0.785321101,0.787155963,
0.788990826,0.790825688,0.79266055,0.794495413,0.796330275,0.798165138,
0.8,0.801834862,0.803669725,0.805504587,0.80733945,0.809174312,0.811009174,
0.812844037,0.814678899,0.816513761,0.818348624,0.820183486,0.822018349,
0.823853211,0.825688073,0.827522936,0.829357798,0.831192661,0.833027523,
0.834862385,0.836697248,0.83853211,0.840366972,0.842201835,0.844036697,
0.84587156,0.847706422,0.849541284,0.851376147,0.853211009,0.855045872,
0.856880734,0.858715596,0.860550459,0.862385321,0.864220183,0.866055046,
0.867889908,0.869724771,0.871559633,0.873394495,0.875229358,0.87706422,
0.878899083,0.880733945,0.882568807,0.88440367,0.886238532,0.888073394,
0.889908257,0.891743119,0.893577982,0.895412844,0.897247706,0.899082569,
0.900917431,0.902752294,0.904587156,0.906422018,0.908256881,0.910091743,
0.911926606,0.913761468,0.91559633,0.917431193,0.919266055,0.921100917,
0.92293578,0.924770642,0.926605505,0.928440367,0.930275229,0.932110092,
0.933944954,0.935779817,0.937614679,0.939449541,0.941284404,0.943119266,
0.944954128,0.946788991,0.948623853,0.950458716,0.952293578,0.95412844,
0.955963303,0.957798165,0.959633028,0.96146789,0.963302752,0.965137615,
0.966972477,0.968807339,0.970642202,0.972477064,0.974311927,0.976146789,
0.977981651,0.979816514,0.981651376,0.983486239,0.985321101,0.987155963,
0.988990826,0.990825688,0.99266055,0.994495413,0.996330275,0.998165138,
1.),(0.,0.36),.UNSPECIFIED.);
#6288=B_SPLINE_SURFACE_WITH_KNOTS('',5,1,((#274438,#274439),(#274440,#274441),
(#274442,#274443),(#274444,#274445),(#274446,#274447),(#274448,#274449),
(#274450,#274451),(#274452,#274453),(#274454,#274455),(#274456,#274457),
(#274458,#274459),(#274460,#274461),(#274462,#274463),(#274464,#274465),
(#274466,#274467),(#274468,#274469),(#274470,#274471),(#274472,#274473),
(#274474,#274475),(#274476,#274477),(#274478,#274479),(#274480,#274481),
(#274482,#274483),(#274484,#274485),(#274486,#274487),(#274488,#274489),
(#274490,#274491),(#274492,#274493),(#274494,#274495),(#274496,#274497),
(#274498,#274499),(#274500,#274501),(#274502,#274503),(#274504,#274505),
(#274506,#274507),(#274508,#274509),(#274510,#274511),(#274512,#274513),
(#274514,#274515),(#274516,#274517),(#274518,#274519),(#274520,#274521),
(#274522,#274523),(#274524,#274525),(#274526,#274527),(#274528,#274529),
(#274530,#274531),(#274532,#274533),(#274534,#274535),(#274536,#274537),
(#274538,#274539),(#274540,#274541),(#274542,#274543),(#274544,#274545),
(#274546,#274547),(#274548,#274549),(#274550,#274551),(#274552,#274553),
(#274554,#274555),(#274556,#274557),(#274558,#274559),(#274560,#274561),
(#274562,#274563),(#274564,#274565),(#274566,#274567),(#274568,#274569),
(#274570,#274571),(#274572,#274573),(#274574,#274575),(#274576,#274577),
(#274578,#274579),(#274580,#274581),(#274582,#274583),(#274584,#274585),
(#274586,#274587),(#274588,#274589),(#274590,#274591),(#274592,#274593),
(#274594,#274595),(#274596,#274597),(#274598,#274599),(#274600,#274601),
(#274602,#274603),(#274604,#274605),(#274606,#274607),(#274608,#274609),
(#274610,#274611),(#274612,#274613),(#274614,#274615),(#274616,#274617),
(#274618,#274619),(#274620,#274621),(#274622,#274623),(#274624,#274625),
(#274626,#274627),(#274628,#274629),(#274630,#274631),(#274632,#274633),
(#274634,#274635),(#274636,#274637),(#274638,#274639),(#274640,#274641),
(#274642,#274643),(#274644,#274645),(#274646,#274647),(#274648,#274649),
(#274650,#274651),(#274652,#274653),(#274654,#274655),(#274656,#274657),
(#274658,#274659),(#274660,#274661),(#274662,#274663),(#274664,#274665),
(#274666,#274667),(#274668,#274669),(#274670,#274671),(#274672,#274673),
(#274674,#274675),(#274676,#274677),(#274678,#274679),(#274680,#274681),
(#274682,#274683),(#274684,#274685),(#274686,#274687),(#274688,#274689),
(#274690,#274691),(#274692,#274693),(#274694,#274695),(#274696,#274697),
(#274698,#274699),(#274700,#274701),(#274702,#274703),(#274704,#274705),
(#274706,#274707),(#274708,#274709),(#274710,#274711),(#274712,#274713),
(#274714,#274715),(#274716,#274717),(#274718,#274719),(#274720,#274721),
(#274722,#274723),(#274724,#274725),(#274726,#274727),(#274728,#274729),
(#274730,#274731),(#274732,#274733),(#274734,#274735),(#274736,#274737),
(#274738,#274739),(#274740,#274741),(#274742,#274743),(#274744,#274745),
(#274746,#274747),(#274748,#274749),(#274750,#274751),(#274752,#274753),
(#274754,#274755),(#274756,#274757),(#274758,#274759),(#274760,#274761),
(#274762,#274763),(#274764,#274765),(#274766,#274767),(#274768,#274769),
(#274770,#274771),(#274772,#274773),(#274774,#274775),(#274776,#274777),
(#274778,#274779),(#274780,#274781),(#274782,#274783),(#274784,#274785),
(#274786,#274787),(#274788,#274789),(#274790,#274791),(#274792,#274793),
(#274794,#274795),(#274796,#274797),(#274798,#274799),(#274800,#274801),
(#274802,#274803),(#274804,#274805),(#274806,#274807),(#274808,#274809),
(#274810,#274811),(#274812,#274813),(#274814,#274815),(#274816,#274817),
(#274818,#274819),(#274820,#274821),(#274822,#274823),(#274824,#274825),
(#274826,#274827),(#274828,#274829),(#274830,#274831),(#274832,#274833),
(#274834,#274835),(#274836,#274837),(#274838,#274839),(#274840,#274841),
(#274842,#274843),(#274844,#274845),(#274846,#274847),(#274848,#274849),
(#274850,#274851),(#274852,#274853),(#274854,#274855),(#274856,#274857),
(#274858,#274859),(#274860,#274861),(#274862,#274863),(#274864,#274865),
(#274866,#274867),(#274868,#274869),(#274870,#274871),(#274872,#274873),
(#274874,#274875),(#274876,#274877),(#274878,#274879),(#274880,#274881),
(#274882,#274883),(#274884,#274885),(#274886,#274887),(#274888,#274889),
(#274890,#274891),(#274892,#274893),(#274894,#274895),(#274896,#274897),
(#274898,#274899),(#274900,#274901),(#274902,#274903),(#274904,#274905),
(#274906,#274907),(#274908,#274909),(#274910,#274911),(#274912,#274913),
(#274914,#274915),(#274916,#274917),(#274918,#274919),(#274920,#274921),
(#274922,#274923),(#274924,#274925),(#274926,#274927),(#274928,#274929),
(#274930,#274931),(#274932,#274933),(#274934,#274935),(#274936,#274937),
(#274938,#274939),(#274940,#274941),(#274942,#274943),(#274944,#274945),
(#274946,#274947),(#274948,#274949),(#274950,#274951),(#274952,#274953),
(#274954,#274955),(#274956,#274957),(#274958,#274959),(#274960,#274961),
(#274962,#274963),(#274964,#274965),(#274966,#274967),(#274968,#274969),
(#274970,#274971),(#274972,#274973),(#274974,#274975),(#274976,#274977),
(#274978,#274979),(#274980,#274981),(#274982,#274983),(#274984,#274985),
(#274986,#274987),(#274988,#274989),(#274990,#274991),(#274992,#274993),
(#274994,#274995),(#274996,#274997),(#274998,#274999),(#275000,#275001),
(#275002,#275003),(#275004,#275005),(#275006,#275007),(#275008,#275009),
(#275010,#275011),(#275012,#275013),(#275014,#275015),(#275016,#275017),
(#275018,#275019),(#275020,#275021),(#275022,#275023),(#275024,#275025),
(#275026,#275027),(#275028,#275029),(#275030,#275031),(#275032,#275033),
(#275034,#275035),(#275036,#275037),(#275038,#275039),(#275040,#275041),
(#275042,#275043),(#275044,#275045),(#275046,#275047),(#275048,#275049),
(#275050,#275051),(#275052,#275053),(#275054,#275055),(#275056,#275057),
(#275058,#275059),(#275060,#275061),(#275062,#275063),(#275064,#275065),
(#275066,#275067),(#275068,#275069),(#275070,#275071),(#275072,#275073),
(#275074,#275075),(#275076,#275077),(#275078,#275079),(#275080,#275081),
(#275082,#275083),(#275084,#275085),(#275086,#275087),(#275088,#275089),
(#275090,#275091),(#275092,#275093),(#275094,#275095),(#275096,#275097),
(#275098,#275099),(#275100,#275101),(#275102,#275103),(#275104,#275105),
(#275106,#275107),(#275108,#275109),(#275110,#275111),(#275112,#275113),
(#275114,#275115),(#275116,#275117),(#275118,#275119),(#275120,#275121),
(#275122,#275123),(#275124,#275125),(#275126,#275127),(#275128,#275129),
(#275130,#275131),(#275132,#275133),(#275134,#275135),(#275136,#275137),
(#275138,#275139),(#275140,#275141),(#275142,#275143),(#275144,#275145),
(#275146,#275147),(#275148,#275149),(#275150,#275151),(#275152,#275153),
(#275154,#275155),(#275156,#275157),(#275158,#275159),(#275160,#275161),
(#275162,#275163),(#275164,#275165),(#275166,#275167),(#275168,#275169),
(#275170,#275171),(#275172,#275173),(#275174,#275175),(#275176,#275177),
(#275178,#275179),(#275180,#275181),(#275182,#275183),(#275184,#275185),
(#275186,#275187),(#275188,#275189),(#275190,#275191),(#275192,#275193),
(#275194,#275195),(#275196,#275197),(#275198,#275199),(#275200,#275201),
(#275202,#275203),(#275204,#275205),(#275206,#275207),(#275208,#275209),
(#275210,#275211),(#275212,#275213),(#275214,#275215),(#275216,#275217),
(#275218,#275219),(#275220,#275221),(#275222,#275223),(#275224,#275225),
(#275226,#275227),(#275228,#275229),(#275230,#275231),(#275232,#275233),
(#275234,#275235),(#275236,#275237),(#275238,#275239),(#275240,#275241),
(#275242,#275243),(#275244,#275245),(#275246,#275247),(#275248,#275249),
(#275250,#275251),(#275252,#275253),(#275254,#275255),(#275256,#275257),
(#275258,#275259),(#275260,#275261),(#275262,#275263),(#275264,#275265),
(#275266,#275267),(#275268,#275269),(#275270,#275271),(#275272,#275273),
(#275274,#275275),(#275276,#275277),(#275278,#275279),(#275280,#275281),
(#275282,#275283),(#275284,#275285),(#275286,#275287),(#275288,#275289),
(#275290,#275291),(#275292,#275293),(#275294,#275295),(#275296,#275297),
(#275298,#275299),(#275300,#275301),(#275302,#275303),(#275304,#275305),
(#275306,#275307),(#275308,#275309),(#275310,#275311),(#275312,#275313),
(#275314,#275315),(#275316,#275317),(#275318,#275319),(#275320,#275321),
(#275322,#275323),(#275324,#275325),(#275326,#275327),(#275328,#275329),
(#275330,#275331),(#275332,#275333),(#275334,#275335),(#275336,#275337),
(#275338,#275339),(#275340,#275341),(#275342,#275343),(#275344,#275345),
(#275346,#275347),(#275348,#275349),(#275350,#275351),(#275352,#275353),
(#275354,#275355),(#275356,#275357),(#275358,#275359),(#275360,#275361),
(#275362,#275363),(#275364,#275365),(#275366,#275367),(#275368,#275369),
(#275370,#275371),(#275372,#275373),(#275374,#275375),(#275376,#275377),
(#275378,#275379),(#275380,#275381)),.UNSPECIFIED.,.F.,.F.,.F.,(6,1,1,1,
1,1,1,1,1,1,1,1,1,1,1,1,1,1,1,1,1,1,1,1,1,1,1,1,1,1,1,1,1,1,1,1,1,1,1,1,
1,1,1,1,1,1,1,1,1,1,1,1,1,1,1,1,1,1,1,1,1,1,1,1,1,1,1,1,1,1,1,1,1,1,1,1,
1,1,1,1,1,1,1,1,1,1,1,1,1,1,1,1,1,1,1,1,1,1,1,1,1,1,1,1,1,1,1,1,1,1,1,1,
1,1,1,1,1,1,1,1,1,1,1,1,1,1,1,1,1,1,1,1,1,1,1,1,1,1,1,1,1,1,1,1,1,1,1,1,
1,1,1,1,1,1,1,1,1,1,1,1,1,1,1,1,1,1,1,1,1,1,1,1,1,1,1,1,1,1,1,1,1,1,1,1,
1,1,1,1,1,1,1,1,1,1,1,1,1,1,1,1,1,1,1,1,1,1,1,1,1,1,1,1,1,1,1,1,1,1,1,1,
1,1,1,1,1,1,1,1,1,1,1,1,1,1,1,1,1,1,1,1,1,1,1,1,1,1,1,1,1,1,1,1,1,1,1,1,
1,1,1,1,1,1,1,1,1,1,1,1,1,1,1,1,1,1,1,1,1,1,1,1,1,1,1,1,1,1,1,1,1,1,1,1,
1,1,1,1,1,1,1,1,1,1,1,1,1,1,1,1,1,1,1,1,1,1,1,1,1,1,1,1,1,1,1,1,1,1,1,1,
1,1,1,1,1,1,1,1,1,1,1,1,1,1,1,1,1,1,1,1,1,1,1,1,1,1,1,1,1,1,1,1,1,1,1,1,
1,1,1,1,1,1,1,1,1,1,1,1,1,1,1,1,1,1,1,1,1,1,1,1,1,1,1,1,1,1,1,1,1,1,1,1,
1,1,1,1,1,1,1,1,1,1,1,1,1,1,1,1,1,1,1,1,1,1,1,1,1,1,1,1,1,1,1,1,1,1,1,1,
1,1,1,1,1,1,1,1,1,1,1,1,1,1,1,1,1,1,1,1,1,1,1,1,1,1,1,1,1,1,1,6),(2,2),
(-1.,-0.998165138,-0.996330275,-0.994495413,-0.99266055,-0.990825688,-0.988990826,
-0.987155963,-0.985321101,-0.983486239,-0.981651376,-0.979816514,-0.977981651,
-0.976146789,-0.974311927,-0.972477064,-0.970642202,-0.968807339,-0.966972477,
-0.965137615,-0.963302752,-0.96146789,-0.959633028,-0.957798165,-0.955963303,
-0.95412844,-0.952293578,-0.950458716,-0.948623853,-0.946788991,-0.944954128,
-0.943119266,-0.941284404,-0.939449541,-0.937614679,-0.935779817,-0.933944954,
-0.932110092,-0.930275229,-0.928440367,-0.926605505,-0.924770642,-0.92293578,
-0.921100917,-0.919266055,-0.917431193,-0.91559633,-0.913761468,-0.911926606,
-0.910091743,-0.908256881,-0.906422018,-0.904587156,-0.902752294,-0.900917431,
-0.899082569,-0.897247706,-0.895412844,-0.893577982,-0.891743119,-0.889908257,
-0.888073394,-0.886238532,-0.88440367,-0.882568807,-0.880733945,-0.878899083,
-0.87706422,-0.875229358,-0.873394495,-0.871559633,-0.869724771,-0.867889908,
-0.866055046,-0.864220183,-0.862385321,-0.860550459,-0.858715596,-0.856880734,
-0.855045872,-0.853211009,-0.851376147,-0.849541284,-0.847706422,-0.84587156,
-0.844036697,-0.842201835,-0.840366972,-0.83853211,-0.836697248,-0.834862385,
-0.833027523,-0.831192661,-0.829357798,-0.827522936,-0.825688073,-0.823853211,
-0.822018349,-0.820183486,-0.818348624,-0.816513761,-0.814678899,-0.812844037,
-0.811009174,-0.809174312,-0.80733945,-0.805504587,-0.803669725,-0.801834862,
-0.8,-0.798165138,-0.796330275,-0.794495413,-0.79266055,-0.790825688,-0.788990826,
-0.787155963,-0.785321101,-0.783486239,-0.781651376,-0.779816514,-0.777981651,
-0.776146789,-0.774311927,-0.772477064,-0.770642202,-0.768807339,-0.766972477,
-0.765137615,-0.763302752,-0.76146789,-0.759633028,-0.757798165,-0.755963303,
-0.75412844,-0.752293578,-0.750458716,-0.748623853,-0.746788991,-0.744954128,
-0.743119266,-0.741284404,-0.739449541,-0.737614679,-0.735779817,-0.733944954,
-0.732110092,-0.730275229,-0.728440367,-0.726605505,-0.724770642,-0.72293578,
-0.721100917,-0.719266055,-0.717431193,-0.71559633,-0.713761468,-0.711926606,
-0.710091743,-0.708256881,-0.706422018,-0.704587156,-0.702752294,-0.700917431,
-0.699082569,-0.697247706,-0.695412844,-0.693577982,-0.691743119,-0.689908257,
-0.688073394,-0.686238532,-0.68440367,-0.682568807,-0.680733945,-0.678899083,
-0.67706422,-0.675229358,-0.673394495,-0.671559633,-0.669724771,-0.667889908,
-0.666055046,-0.664220183,-0.662385321,-0.660550459,-0.658715596,-0.656880734,
-0.655045872,-0.653211009,-0.651376147,-0.649541284,-0.647706422,-0.64587156,
-0.644036697,-0.642201835,-0.640366972,-0.63853211,-0.636697248,-0.634862385,
-0.633027523,-0.631192661,-0.629357798,-0.627522936,-0.625688073,-0.623853211,
-0.622018349,-0.620183486,-0.618348624,-0.616513761,-0.614678899,-0.612844037,
-0.611009174,-0.609174312,-0.60733945,-0.605504587,-0.603669725,-0.601834862,
-0.6,-0.598165138,-0.596330275,-0.594495413,-0.59266055,-0.590825688,-0.588990826,
-0.587155963,-0.585321101,-0.583486239,-0.581651376,-0.579816514,-0.577981651,
-0.576146789,-0.574311927,-0.572477064,-0.570642202,-0.568807339,-0.566972477,
-0.565137615,-0.563302752,-0.56146789,-0.559633028,-0.557798165,-0.555963303,
-0.55412844,-0.552293578,-0.550458716,-0.548623853,-0.546788991,-0.544954128,
-0.543119266,-0.541284404,-0.539449541,-0.537614679,-0.535779817,-0.533944954,
-0.532110092,-0.530275229,-0.528440367,-0.526605505,-0.524770642,-0.52293578,
-0.521100917,-0.519266055,-0.517431193,-0.51559633,-0.513761468,-0.511926606,
-0.510091743,-0.508256881,-0.506422018,-0.504587156,-0.502752294,-0.500917431,
-0.499082569,-0.497247706,-0.495412844,-0.493577982,-0.491743119,-0.489908257,
-0.488073394,-0.486238532,-0.48440367,-0.482568807,-0.480733945,-0.478899083,
-0.47706422,-0.475229358,-0.473394495,-0.471559633,-0.469724771,-0.467889908,
-0.466055046,-0.464220183,-0.462385321,-0.460550459,-0.458715596,-0.456880734,
-0.455045872,-0.453211009,-0.451376147,-0.449541284,-0.447706422,-0.44587156,
-0.444036697,-0.442201835,-0.440366972,-0.43853211,-0.436697248,-0.434862385,
-0.433027523,-0.431192661,-0.429357798,-0.427522936,-0.425688073,-0.423853211,
-0.422018349,-0.420183486,-0.418348624,-0.416513761,-0.414678899,-0.412844037,
-0.411009174,-0.409174312,-0.40733945,-0.405504587,-0.403669725,-0.401834862,
-0.4,-0.398165138,-0.396330275,-0.394495413,-0.39266055,-0.390825688,-0.388990826,
-0.387155963,-0.385321101,-0.383486239,-0.381651376,-0.379816514,-0.377981651,
-0.376146789,-0.374311927,-0.372477064,-0.370642202,-0.368807339,-0.366972477,
-0.365137615,-0.363302752,-0.36146789,-0.359633028,-0.357798165,-0.355963303,
-0.35412844,-0.352293578,-0.350458716,-0.348623853,-0.346788991,-0.344954128,
-0.343119266,-0.341284404,-0.339449541,-0.337614679,-0.335779817,-0.333944954,
-0.332110092,-0.330275229,-0.328440367,-0.326605505,-0.324770642,-0.32293578,
-0.321100917,-0.319266055,-0.317431193,-0.31559633,-0.313761468,-0.311926606,
-0.310091743,-0.308256881,-0.306422018,-0.304587156,-0.302752294,-0.300917431,
-0.299082569,-0.297247706,-0.295412844,-0.293577982,-0.291743119,-0.289908257,
-0.288073394,-0.286238532,-0.28440367,-0.282568807,-0.280733945,-0.278899083,
-0.27706422,-0.275229358,-0.273394495,-0.271559633,-0.269724771,-0.267889908,
-0.266055046,-0.264220183,-0.262385321,-0.260550459,-0.258715596,-0.256880734,
-0.255045872,-0.253211009,-0.251376147,-0.249541284,-0.247706422,-0.24587156,
-0.244036697,-0.242201835,-0.240366972,-0.23853211,-0.236697248,-0.234862385,
-0.233027523,-0.231192661,-0.229357798,-0.227522936,-0.225688073,-0.223853211,
-0.222018349,-0.220183486,-0.218348624,-0.216513761,-0.214678899,-0.212844037,
-0.211009174,-0.209174312,-0.20733945,-0.205504587,-0.203669725,-0.201834862,
-0.2,-0.198165138,-0.196330275,-0.194495413,-0.19266055,-0.190825688,-0.188990826,
-0.187155963,-0.185321101,-0.183486239,-0.181651376,-0.179816514,-0.177981651,
-0.176146789,-0.174311927,-0.172477064,-0.170642202,-0.168807339,-0.166972477,
-0.165137615,-0.163302752,-0.16146789,-0.159633028,-0.157798165,-0.155963303,
-0.15412844,-0.152293578,-0.150458716,-0.148623853,-0.146788991,-0.144954128,
-0.143172103),(0.,0.36),.UNSPECIFIED.);
#6289=B_SPLINE_SURFACE_WITH_KNOTS('',5,1,((#276047,#276048),(#276049,#276050),
(#276051,#276052),(#276053,#276054),(#276055,#276056),(#276057,#276058),
(#276059,#276060),(#276061,#276062),(#276063,#276064),(#276065,#276066),
(#276067,#276068),(#276069,#276070),(#276071,#276072),(#276073,#276074),
(#276075,#276076),(#276077,#276078),(#276079,#276080),(#276081,#276082),
(#276083,#276084),(#276085,#276086),(#276087,#276088),(#276089,#276090),
(#276091,#276092),(#276093,#276094),(#276095,#276096),(#276097,#276098),
(#276099,#276100),(#276101,#276102),(#276103,#276104),(#276105,#276106),
(#276107,#276108),(#276109,#276110),(#276111,#276112),(#276113,#276114),
(#276115,#276116),(#276117,#276118),(#276119,#276120),(#276121,#276122),
(#276123,#276124),(#276125,#276126),(#276127,#276128),(#276129,#276130),
(#276131,#276132),(#276133,#276134),(#276135,#276136),(#276137,#276138),
(#276139,#276140),(#276141,#276142),(#276143,#276144),(#276145,#276146),
(#276147,#276148),(#276149,#276150),(#276151,#276152),(#276153,#276154),
(#276155,#276156),(#276157,#276158),(#276159,#276160),(#276161,#276162),
(#276163,#276164),(#276165,#276166),(#276167,#276168),(#276169,#276170),
(#276171,#276172),(#276173,#276174),(#276175,#276176),(#276177,#276178),
(#276179,#276180),(#276181,#276182),(#276183,#276184),(#276185,#276186),
(#276187,#276188),(#276189,#276190),(#276191,#276192),(#276193,#276194),
(#276195,#276196),(#276197,#276198),(#276199,#276200),(#276201,#276202),
(#276203,#276204),(#276205,#276206),(#276207,#276208),(#276209,#276210),
(#276211,#276212),(#276213,#276214),(#276215,#276216),(#276217,#276218),
(#276219,#276220),(#276221,#276222),(#276223,#276224),(#276225,#276226),
(#276227,#276228),(#276229,#276230),(#276231,#276232),(#276233,#276234),
(#276235,#276236),(#276237,#276238),(#276239,#276240),(#276241,#276242),
(#276243,#276244),(#276245,#276246),(#276247,#276248),(#276249,#276250),
(#276251,#276252),(#276253,#276254),(#276255,#276256),(#276257,#276258),
(#276259,#276260),(#276261,#276262),(#276263,#276264),(#276265,#276266),
(#276267,#276268),(#276269,#276270),(#276271,#276272),(#276273,#276274),
(#276275,#276276),(#276277,#276278),(#276279,#276280),(#276281,#276282),
(#276283,#276284),(#276285,#276286),(#276287,#276288),(#276289,#276290),
(#276291,#276292),(#276293,#276294),(#276295,#276296),(#276297,#276298),
(#276299,#276300),(#276301,#276302),(#276303,#276304),(#276305,#276306),
(#276307,#276308),(#276309,#276310),(#276311,#276312),(#276313,#276314),
(#276315,#276316),(#276317,#276318),(#276319,#276320),(#276321,#276322),
(#276323,#276324),(#276325,#276326),(#276327,#276328),(#276329,#276330),
(#276331,#276332),(#276333,#276334),(#276335,#276336),(#276337,#276338),
(#276339,#276340),(#276341,#276342),(#276343,#276344),(#276345,#276346),
(#276347,#276348),(#276349,#276350),(#276351,#276352),(#276353,#276354),
(#276355,#276356),(#276357,#276358),(#276359,#276360),(#276361,#276362),
(#276363,#276364),(#276365,#276366),(#276367,#276368),(#276369,#276370),
(#276371,#276372),(#276373,#276374),(#276375,#276376),(#276377,#276378),
(#276379,#276380),(#276381,#276382),(#276383,#276384),(#276385,#276386),
(#276387,#276388),(#276389,#276390),(#276391,#276392),(#276393,#276394),
(#276395,#276396),(#276397,#276398),(#276399,#276400),(#276401,#276402),
(#276403,#276404),(#276405,#276406),(#276407,#276408),(#276409,#276410),
(#276411,#276412),(#276413,#276414),(#276415,#276416),(#276417,#276418),
(#276419,#276420),(#276421,#276422),(#276423,#276424),(#276425,#276426),
(#276427,#276428),(#276429,#276430),(#276431,#276432),(#276433,#276434),
(#276435,#276436),(#276437,#276438),(#276439,#276440),(#276441,#276442),
(#276443,#276444),(#276445,#276446),(#276447,#276448),(#276449,#276450),
(#276451,#276452),(#276453,#276454),(#276455,#276456),(#276457,#276458),
(#276459,#276460),(#276461,#276462),(#276463,#276464),(#276465,#276466),
(#276467,#276468),(#276469,#276470),(#276471,#276472),(#276473,#276474),
(#276475,#276476),(#276477,#276478),(#276479,#276480),(#276481,#276482),
(#276483,#276484),(#276485,#276486),(#276487,#276488),(#276489,#276490),
(#276491,#276492),(#276493,#276494),(#276495,#276496),(#276497,#276498),
(#276499,#276500),(#276501,#276502),(#276503,#276504),(#276505,#276506),
(#276507,#276508),(#276509,#276510),(#276511,#276512),(#276513,#276514),
(#276515,#276516),(#276517,#276518),(#276519,#276520),(#276521,#276522),
(#276523,#276524),(#276525,#276526),(#276527,#276528),(#276529,#276530),
(#276531,#276532),(#276533,#276534),(#276535,#276536),(#276537,#276538),
(#276539,#276540),(#276541,#276542),(#276543,#276544),(#276545,#276546),
(#276547,#276548),(#276549,#276550),(#276551,#276552),(#276553,#276554),
(#276555,#276556),(#276557,#276558),(#276559,#276560),(#276561,#276562),
(#276563,#276564),(#276565,#276566),(#276567,#276568),(#276569,#276570),
(#276571,#276572),(#276573,#276574),(#276575,#276576),(#276577,#276578),
(#276579,#276580),(#276581,#276582),(#276583,#276584),(#276585,#276586),
(#276587,#276588),(#276589,#276590),(#276591,#276592),(#276593,#276594),
(#276595,#276596),(#276597,#276598),(#276599,#276600),(#276601,#276602),
(#276603,#276604),(#276605,#276606),(#276607,#276608),(#276609,#276610),
(#276611,#276612),(#276613,#276614),(#276615,#276616),(#276617,#276618),
(#276619,#276620),(#276621,#276622),(#276623,#276624),(#276625,#276626),
(#276627,#276628),(#276629,#276630),(#276631,#276632),(#276633,#276634),
(#276635,#276636),(#276637,#276638),(#276639,#276640),(#276641,#276642),
(#276643,#276644),(#276645,#276646),(#276647,#276648),(#276649,#276650),
(#276651,#276652),(#276653,#276654),(#276655,#276656),(#276657,#276658),
(#276659,#276660),(#276661,#276662),(#276663,#276664),(#276665,#276666),
(#276667,#276668),(#276669,#276670),(#276671,#276672),(#276673,#276674),
(#276675,#276676),(#276677,#276678),(#276679,#276680),(#276681,#276682),
(#276683,#276684),(#276685,#276686),(#276687,#276688),(#276689,#276690),
(#276691,#276692),(#276693,#276694),(#276695,#276696),(#276697,#276698),
(#276699,#276700),(#276701,#276702),(#276703,#276704),(#276705,#276706),
(#276707,#276708),(#276709,#276710),(#276711,#276712),(#276713,#276714),
(#276715,#276716),(#276717,#276718),(#276719,#276720),(#276721,#276722),
(#276723,#276724),(#276725,#276726),(#276727,#276728),(#276729,#276730),
(#276731,#276732),(#276733,#276734),(#276735,#276736),(#276737,#276738),
(#276739,#276740),(#276741,#276742),(#276743,#276744),(#276745,#276746),
(#276747,#276748),(#276749,#276750),(#276751,#276752),(#276753,#276754),
(#276755,#276756),(#276757,#276758),(#276759,#276760),(#276761,#276762),
(#276763,#276764),(#276765,#276766),(#276767,#276768),(#276769,#276770),
(#276771,#276772),(#276773,#276774),(#276775,#276776),(#276777,#276778),
(#276779,#276780),(#276781,#276782),(#276783,#276784),(#276785,#276786),
(#276787,#276788),(#276789,#276790),(#276791,#276792),(#276793,#276794),
(#276795,#276796),(#276797,#276798),(#276799,#276800),(#276801,#276802),
(#276803,#276804),(#276805,#276806),(#276807,#276808),(#276809,#276810),
(#276811,#276812),(#276813,#276814),(#276815,#276816),(#276817,#276818),
(#276819,#276820),(#276821,#276822),(#276823,#276824),(#276825,#276826),
(#276827,#276828),(#276829,#276830),(#276831,#276832),(#276833,#276834),
(#276835,#276836),(#276837,#276838),(#276839,#276840),(#276841,#276842),
(#276843,#276844),(#276845,#276846),(#276847,#276848),(#276849,#276850),
(#276851,#276852),(#276853,#276854),(#276855,#276856),(#276857,#276858),
(#276859,#276860),(#276861,#276862),(#276863,#276864),(#276865,#276866),
(#276867,#276868),(#276869,#276870),(#276871,#276872),(#276873,#276874),
(#276875,#276876),(#276877,#276878),(#276879,#276880),(#276881,#276882),
(#276883,#276884),(#276885,#276886),(#276887,#276888),(#276889,#276890),
(#276891,#276892),(#276893,#276894),(#276895,#276896),(#276897,#276898),
(#276899,#276900),(#276901,#276902),(#276903,#276904),(#276905,#276906),
(#276907,#276908),(#276909,#276910),(#276911,#276912),(#276913,#276914),
(#276915,#276916),(#276917,#276918),(#276919,#276920),(#276921,#276922),
(#276923,#276924),(#276925,#276926),(#276927,#276928),(#276929,#276930),
(#276931,#276932),(#276933,#276934),(#276935,#276936),(#276937,#276938),
(#276939,#276940),(#276941,#276942),(#276943,#276944),(#276945,#276946),
(#276947,#276948),(#276949,#276950),(#276951,#276952),(#276953,#276954),
(#276955,#276956),(#276957,#276958),(#276959,#276960),(#276961,#276962),
(#276963,#276964),(#276965,#276966),(#276967,#276968),(#276969,#276970),
(#276971,#276972),(#276973,#276974),(#276975,#276976),(#276977,#276978),
(#276979,#276980),(#276981,#276982),(#276983,#276984),(#276985,#276986),
(#276987,#276988),(#276989,#276990)),.UNSPECIFIED.,.F.,.F.,.F.,(6,1,1,1,
1,1,1,1,1,1,1,1,1,1,1,1,1,1,1,1,1,1,1,1,1,1,1,1,1,1,1,1,1,1,1,1,1,1,1,1,
1,1,1,1,1,1,1,1,1,1,1,1,1,1,1,1,1,1,1,1,1,1,1,1,1,1,1,1,1,1,1,1,1,1,1,1,
1,1,1,1,1,1,1,1,1,1,1,1,1,1,1,1,1,1,1,1,1,1,1,1,1,1,1,1,1,1,1,1,1,1,1,1,
1,1,1,1,1,1,1,1,1,1,1,1,1,1,1,1,1,1,1,1,1,1,1,1,1,1,1,1,1,1,1,1,1,1,1,1,
1,1,1,1,1,1,1,1,1,1,1,1,1,1,1,1,1,1,1,1,1,1,1,1,1,1,1,1,1,1,1,1,1,1,1,1,
1,1,1,1,1,1,1,1,1,1,1,1,1,1,1,1,1,1,1,1,1,1,1,1,1,1,1,1,1,1,1,1,1,1,1,1,
1,1,1,1,1,1,1,1,1,1,1,1,1,1,1,1,1,1,1,1,1,1,1,1,1,1,1,1,1,1,1,1,1,1,1,1,
1,1,1,1,1,1,1,1,1,1,1,1,1,1,1,1,1,1,1,1,1,1,1,1,1,1,1,1,1,1,1,1,1,1,1,1,
1,1,1,1,1,1,1,1,1,1,1,1,1,1,1,1,1,1,1,1,1,1,1,1,1,1,1,1,1,1,1,1,1,1,1,1,
1,1,1,1,1,1,1,1,1,1,1,1,1,1,1,1,1,1,1,1,1,1,1,1,1,1,1,1,1,1,1,1,1,1,1,1,
1,1,1,1,1,1,1,1,1,1,1,1,1,1,1,1,1,1,1,1,1,1,1,1,1,1,1,1,1,1,1,1,1,1,1,1,
1,1,1,1,1,1,1,1,1,1,1,1,1,1,1,1,1,1,1,1,1,1,1,1,1,1,1,1,1,1,1,1,1,1,1,1,
1,1,1,1,1,1,1,1,1,1,1,1,1,1,1,1,1,1,1,1,1,1,1,1,1,1,1,1,1,1,1,6),(2,2),
(-1.,-0.998165138,-0.996330275,-0.994495413,-0.99266055,-0.990825688,-0.988990826,
-0.987155963,-0.985321101,-0.983486239,-0.981651376,-0.979816514,-0.977981651,
-0.976146789,-0.974311927,-0.972477064,-0.970642202,-0.968807339,-0.966972477,
-0.965137615,-0.963302752,-0.96146789,-0.959633028,-0.957798165,-0.955963303,
-0.95412844,-0.952293578,-0.950458716,-0.948623853,-0.946788991,-0.944954128,
-0.943119266,-0.941284404,-0.939449541,-0.937614679,-0.935779817,-0.933944954,
-0.932110092,-0.930275229,-0.928440367,-0.926605505,-0.924770642,-0.92293578,
-0.921100917,-0.919266055,-0.917431193,-0.91559633,-0.913761468,-0.911926606,
-0.910091743,-0.908256881,-0.906422018,-0.904587156,-0.902752294,-0.900917431,
-0.899082569,-0.897247706,-0.895412844,-0.893577982,-0.891743119,-0.889908257,
-0.888073394,-0.886238532,-0.88440367,-0.882568807,-0.880733945,-0.878899083,
-0.87706422,-0.875229358,-0.873394495,-0.871559633,-0.869724771,-0.867889908,
-0.866055046,-0.864220183,-0.862385321,-0.860550459,-0.858715596,-0.856880734,
-0.855045872,-0.853211009,-0.851376147,-0.849541284,-0.847706422,-0.84587156,
-0.844036697,-0.842201835,-0.840366972,-0.83853211,-0.836697248,-0.834862385,
-0.833027523,-0.831192661,-0.829357798,-0.827522936,-0.825688073,-0.823853211,
-0.822018349,-0.820183486,-0.818348624,-0.816513761,-0.814678899,-0.812844037,
-0.811009174,-0.809174312,-0.80733945,-0.805504587,-0.803669725,-0.801834862,
-0.8,-0.798165138,-0.796330275,-0.794495413,-0.79266055,-0.790825688,-0.788990826,
-0.787155963,-0.785321101,-0.783486239,-0.781651376,-0.779816514,-0.777981651,
-0.776146789,-0.774311927,-0.772477064,-0.770642202,-0.768807339,-0.766972477,
-0.765137615,-0.763302752,-0.76146789,-0.759633028,-0.757798165,-0.755963303,
-0.75412844,-0.752293578,-0.750458716,-0.748623853,-0.746788991,-0.744954128,
-0.743119266,-0.741284404,-0.739449541,-0.737614679,-0.735779817,-0.733944954,
-0.732110092,-0.730275229,-0.728440367,-0.726605505,-0.724770642,-0.72293578,
-0.721100917,-0.719266055,-0.717431193,-0.71559633,-0.713761468,-0.711926606,
-0.710091743,-0.708256881,-0.706422018,-0.704587156,-0.702752294,-0.700917431,
-0.699082569,-0.697247706,-0.695412844,-0.693577982,-0.691743119,-0.689908257,
-0.688073394,-0.686238532,-0.68440367,-0.682568807,-0.680733945,-0.678899083,
-0.67706422,-0.675229358,-0.673394495,-0.671559633,-0.669724771,-0.667889908,
-0.666055046,-0.664220183,-0.662385321,-0.660550459,-0.658715596,-0.656880734,
-0.655045872,-0.653211009,-0.651376147,-0.649541284,-0.647706422,-0.64587156,
-0.644036697,-0.642201835,-0.640366972,-0.63853211,-0.636697248,-0.634862385,
-0.633027523,-0.631192661,-0.629357798,-0.627522936,-0.625688073,-0.623853211,
-0.622018349,-0.620183486,-0.618348624,-0.616513761,-0.614678899,-0.612844037,
-0.611009174,-0.609174312,-0.60733945,-0.605504587,-0.603669725,-0.601834862,
-0.6,-0.598165138,-0.596330275,-0.594495413,-0.59266055,-0.590825688,-0.588990826,
-0.587155963,-0.585321101,-0.583486239,-0.581651376,-0.579816514,-0.577981651,
-0.576146789,-0.574311927,-0.572477064,-0.570642202,-0.568807339,-0.566972477,
-0.565137615,-0.563302752,-0.56146789,-0.559633028,-0.557798165,-0.555963303,
-0.55412844,-0.552293578,-0.550458716,-0.548623853,-0.546788991,-0.544954128,
-0.543119266,-0.541284404,-0.539449541,-0.537614679,-0.535779817,-0.533944954,
-0.532110092,-0.530275229,-0.528440367,-0.526605505,-0.524770642,-0.52293578,
-0.521100917,-0.519266055,-0.517431193,-0.51559633,-0.513761468,-0.511926606,
-0.510091743,-0.508256881,-0.506422018,-0.504587156,-0.502752294,-0.500917431,
-0.499082569,-0.497247706,-0.495412844,-0.493577982,-0.491743119,-0.489908257,
-0.488073394,-0.486238532,-0.48440367,-0.482568807,-0.480733945,-0.478899083,
-0.47706422,-0.475229358,-0.473394495,-0.471559633,-0.469724771,-0.467889908,
-0.466055046,-0.464220183,-0.462385321,-0.460550459,-0.458715596,-0.456880734,
-0.455045872,-0.453211009,-0.451376147,-0.449541284,-0.447706422,-0.44587156,
-0.444036697,-0.442201835,-0.440366972,-0.43853211,-0.436697248,-0.434862385,
-0.433027523,-0.431192661,-0.429357798,-0.427522936,-0.425688073,-0.423853211,
-0.422018349,-0.420183486,-0.418348624,-0.416513761,-0.414678899,-0.412844037,
-0.411009174,-0.409174312,-0.40733945,-0.405504587,-0.403669725,-0.401834862,
-0.4,-0.398165138,-0.396330275,-0.394495413,-0.39266055,-0.390825688,-0.388990826,
-0.387155963,-0.385321101,-0.383486239,-0.381651376,-0.379816514,-0.377981651,
-0.376146789,-0.374311927,-0.372477064,-0.370642202,-0.368807339,-0.366972477,
-0.365137615,-0.363302752,-0.36146789,-0.359633028,-0.357798165,-0.355963303,
-0.35412844,-0.352293578,-0.350458716,-0.348623853,-0.346788991,-0.344954128,
-0.343119266,-0.341284404,-0.339449541,-0.337614679,-0.335779817,-0.333944954,
-0.332110092,-0.330275229,-0.328440367,-0.326605505,-0.324770642,-0.32293578,
-0.321100917,-0.319266055,-0.317431193,-0.31559633,-0.313761468,-0.311926606,
-0.310091743,-0.308256881,-0.306422018,-0.304587156,-0.302752294,-0.300917431,
-0.299082569,-0.297247706,-0.295412844,-0.293577982,-0.291743119,-0.289908257,
-0.288073394,-0.286238532,-0.28440367,-0.282568807,-0.280733945,-0.278899083,
-0.27706422,-0.275229358,-0.273394495,-0.271559633,-0.269724771,-0.267889908,
-0.266055046,-0.264220183,-0.262385321,-0.260550459,-0.258715596,-0.256880734,
-0.255045872,-0.253211009,-0.251376147,-0.249541284,-0.247706422,-0.24587156,
-0.244036697,-0.242201835,-0.240366972,-0.23853211,-0.236697248,-0.234862385,
-0.233027523,-0.231192661,-0.229357798,-0.227522936,-0.225688073,-0.223853211,
-0.222018349,-0.220183486,-0.218348624,-0.216513761,-0.214678899,-0.212844037,
-0.211009174,-0.209174312,-0.20733945,-0.205504587,-0.203669725,-0.201834862,
-0.2,-0.198165138,-0.196330275,-0.194495413,-0.19266055,-0.190825688,-0.188990826,
-0.187155963,-0.185321101,-0.183486239,-0.181651376,-0.179816514,-0.177981651,
-0.176146789,-0.174311927,-0.172477064,-0.170642202,-0.168807339,-0.166972477,
-0.165137615,-0.163302752,-0.16146789,-0.159633028,-0.157798165,-0.155963303,
-0.15412844,-0.152293578,-0.150458716,-0.148623853,-0.146788991,-0.144954128,
-0.143172103),(0.,0.36),.UNSPECIFIED.);
#6290=B_SPLINE_SURFACE_WITH_KNOTS('',5,1,((#277936,#277937),(#277938,#277939),
(#277940,#277941),(#277942,#277943),(#277944,#277945),(#277946,#277947),
(#277948,#277949),(#277950,#277951),(#277952,#277953),(#277954,#277955),
(#277956,#277957),(#277958,#277959),(#277960,#277961),(#277962,#277963),
(#277964,#277965),(#277966,#277967),(#277968,#277969),(#277970,#277971),
(#277972,#277973),(#277974,#277975),(#277976,#277977),(#277978,#277979),
(#277980,#277981),(#277982,#277983),(#277984,#277985),(#277986,#277987),
(#277988,#277989),(#277990,#277991),(#277992,#277993),(#277994,#277995),
(#277996,#277997),(#277998,#277999),(#278000,#278001),(#278002,#278003),
(#278004,#278005),(#278006,#278007),(#278008,#278009),(#278010,#278011),
(#278012,#278013),(#278014,#278015),(#278016,#278017),(#278018,#278019),
(#278020,#278021),(#278022,#278023),(#278024,#278025),(#278026,#278027),
(#278028,#278029),(#278030,#278031),(#278032,#278033),(#278034,#278035),
(#278036,#278037),(#278038,#278039),(#278040,#278041),(#278042,#278043),
(#278044,#278045),(#278046,#278047),(#278048,#278049),(#278050,#278051),
(#278052,#278053),(#278054,#278055),(#278056,#278057),(#278058,#278059),
(#278060,#278061),(#278062,#278063),(#278064,#278065),(#278066,#278067),
(#278068,#278069),(#278070,#278071),(#278072,#278073),(#278074,#278075),
(#278076,#278077),(#278078,#278079),(#278080,#278081),(#278082,#278083),
(#278084,#278085),(#278086,#278087),(#278088,#278089),(#278090,#278091),
(#278092,#278093),(#278094,#278095),(#278096,#278097),(#278098,#278099),
(#278100,#278101),(#278102,#278103),(#278104,#278105),(#278106,#278107),
(#278108,#278109),(#278110,#278111),(#278112,#278113),(#278114,#278115),
(#278116,#278117),(#278118,#278119),(#278120,#278121),(#278122,#278123),
(#278124,#278125),(#278126,#278127),(#278128,#278129),(#278130,#278131),
(#278132,#278133),(#278134,#278135),(#278136,#278137),(#278138,#278139),
(#278140,#278141),(#278142,#278143),(#278144,#278145),(#278146,#278147),
(#278148,#278149),(#278150,#278151),(#278152,#278153),(#278154,#278155),
(#278156,#278157),(#278158,#278159),(#278160,#278161),(#278162,#278163),
(#278164,#278165),(#278166,#278167),(#278168,#278169),(#278170,#278171),
(#278172,#278173),(#278174,#278175),(#278176,#278177),(#278178,#278179),
(#278180,#278181),(#278182,#278183),(#278184,#278185),(#278186,#278187),
(#278188,#278189),(#278190,#278191),(#278192,#278193),(#278194,#278195),
(#278196,#278197),(#278198,#278199),(#278200,#278201),(#278202,#278203),
(#278204,#278205),(#278206,#278207),(#278208,#278209),(#278210,#278211),
(#278212,#278213),(#278214,#278215),(#278216,#278217),(#278218,#278219),
(#278220,#278221),(#278222,#278223),(#278224,#278225),(#278226,#278227),
(#278228,#278229),(#278230,#278231),(#278232,#278233),(#278234,#278235),
(#278236,#278237),(#278238,#278239),(#278240,#278241),(#278242,#278243),
(#278244,#278245),(#278246,#278247),(#278248,#278249),(#278250,#278251),
(#278252,#278253),(#278254,#278255),(#278256,#278257),(#278258,#278259),
(#278260,#278261),(#278262,#278263),(#278264,#278265),(#278266,#278267),
(#278268,#278269),(#278270,#278271),(#278272,#278273),(#278274,#278275),
(#278276,#278277),(#278278,#278279),(#278280,#278281),(#278282,#278283),
(#278284,#278285),(#278286,#278287),(#278288,#278289),(#278290,#278291),
(#278292,#278293),(#278294,#278295),(#278296,#278297),(#278298,#278299),
(#278300,#278301),(#278302,#278303),(#278304,#278305),(#278306,#278307),
(#278308,#278309),(#278310,#278311),(#278312,#278313),(#278314,#278315),
(#278316,#278317),(#278318,#278319),(#278320,#278321),(#278322,#278323),
(#278324,#278325),(#278326,#278327),(#278328,#278329),(#278330,#278331),
(#278332,#278333),(#278334,#278335),(#278336,#278337),(#278338,#278339),
(#278340,#278341),(#278342,#278343),(#278344,#278345),(#278346,#278347),
(#278348,#278349),(#278350,#278351),(#278352,#278353),(#278354,#278355),
(#278356,#278357),(#278358,#278359),(#278360,#278361),(#278362,#278363),
(#278364,#278365),(#278366,#278367),(#278368,#278369),(#278370,#278371),
(#278372,#278373),(#278374,#278375),(#278376,#278377),(#278378,#278379),
(#278380,#278381),(#278382,#278383),(#278384,#278385),(#278386,#278387),
(#278388,#278389),(#278390,#278391),(#278392,#278393),(#278394,#278395),
(#278396,#278397),(#278398,#278399),(#278400,#278401),(#278402,#278403),
(#278404,#278405),(#278406,#278407),(#278408,#278409),(#278410,#278411),
(#278412,#278413),(#278414,#278415),(#278416,#278417),(#278418,#278419),
(#278420,#278421),(#278422,#278423),(#278424,#278425),(#278426,#278427),
(#278428,#278429),(#278430,#278431),(#278432,#278433),(#278434,#278435),
(#278436,#278437),(#278438,#278439),(#278440,#278441),(#278442,#278443),
(#278444,#278445),(#278446,#278447),(#278448,#278449),(#278450,#278451),
(#278452,#278453),(#278454,#278455),(#278456,#278457),(#278458,#278459),
(#278460,#278461),(#278462,#278463),(#278464,#278465),(#278466,#278467),
(#278468,#278469),(#278470,#278471),(#278472,#278473),(#278474,#278475),
(#278476,#278477),(#278478,#278479),(#278480,#278481),(#278482,#278483),
(#278484,#278485),(#278486,#278487),(#278488,#278489),(#278490,#278491),
(#278492,#278493),(#278494,#278495),(#278496,#278497),(#278498,#278499),
(#278500,#278501),(#278502,#278503),(#278504,#278505),(#278506,#278507),
(#278508,#278509),(#278510,#278511),(#278512,#278513),(#278514,#278515),
(#278516,#278517),(#278518,#278519),(#278520,#278521),(#278522,#278523),
(#278524,#278525),(#278526,#278527),(#278528,#278529),(#278530,#278531),
(#278532,#278533),(#278534,#278535),(#278536,#278537),(#278538,#278539),
(#278540,#278541),(#278542,#278543),(#278544,#278545),(#278546,#278547),
(#278548,#278549),(#278550,#278551),(#278552,#278553),(#278554,#278555),
(#278556,#278557),(#278558,#278559),(#278560,#278561),(#278562,#278563),
(#278564,#278565),(#278566,#278567),(#278568,#278569),(#278570,#278571),
(#278572,#278573),(#278574,#278575),(#278576,#278577),(#278578,#278579),
(#278580,#278581),(#278582,#278583),(#278584,#278585),(#278586,#278587),
(#278588,#278589),(#278590,#278591),(#278592,#278593),(#278594,#278595),
(#278596,#278597),(#278598,#278599),(#278600,#278601),(#278602,#278603),
(#278604,#278605),(#278606,#278607),(#278608,#278609),(#278610,#278611),
(#278612,#278613),(#278614,#278615),(#278616,#278617),(#278618,#278619),
(#278620,#278621),(#278622,#278623),(#278624,#278625),(#278626,#278627),
(#278628,#278629),(#278630,#278631),(#278632,#278633),(#278634,#278635),
(#278636,#278637),(#278638,#278639),(#278640,#278641),(#278642,#278643),
(#278644,#278645),(#278646,#278647),(#278648,#278649),(#278650,#278651),
(#278652,#278653),(#278654,#278655),(#278656,#278657),(#278658,#278659),
(#278660,#278661),(#278662,#278663),(#278664,#278665),(#278666,#278667),
(#278668,#278669),(#278670,#278671),(#278672,#278673),(#278674,#278675),
(#278676,#278677),(#278678,#278679),(#278680,#278681),(#278682,#278683),
(#278684,#278685),(#278686,#278687),(#278688,#278689),(#278690,#278691),
(#278692,#278693),(#278694,#278695),(#278696,#278697),(#278698,#278699),
(#278700,#278701),(#278702,#278703),(#278704,#278705),(#278706,#278707),
(#278708,#278709),(#278710,#278711),(#278712,#278713),(#278714,#278715),
(#278716,#278717),(#278718,#278719),(#278720,#278721),(#278722,#278723),
(#278724,#278725),(#278726,#278727),(#278728,#278729),(#278730,#278731),
(#278732,#278733),(#278734,#278735),(#278736,#278737),(#278738,#278739),
(#278740,#278741),(#278742,#278743),(#278744,#278745),(#278746,#278747),
(#278748,#278749),(#278750,#278751),(#278752,#278753),(#278754,#278755),
(#278756,#278757),(#278758,#278759),(#278760,#278761),(#278762,#278763),
(#278764,#278765),(#278766,#278767),(#278768,#278769),(#278770,#278771),
(#278772,#278773),(#278774,#278775),(#278776,#278777),(#278778,#278779),
(#278780,#278781),(#278782,#278783),(#278784,#278785),(#278786,#278787),
(#278788,#278789),(#278790,#278791),(#278792,#278793),(#278794,#278795),
(#278796,#278797),(#278798,#278799),(#278800,#278801),(#278802,#278803),
(#278804,#278805),(#278806,#278807),(#278808,#278809),(#278810,#278811),
(#278812,#278813),(#278814,#278815),(#278816,#278817),(#278818,#278819),
(#278820,#278821),(#278822,#278823),(#278824,#278825),(#278826,#278827),
(#278828,#278829),(#278830,#278831),(#278832,#278833),(#278834,#278835),
(#278836,#278837),(#278838,#278839),(#278840,#278841),(#278842,#278843),
(#278844,#278845),(#278846,#278847),(#278848,#278849),(#278850,#278851),
(#278852,#278853),(#278854,#278855),(#278856,#278857),(#278858,#278859),
(#278860,#278861),(#278862,#278863),(#278864,#278865),(#278866,#278867),
(#278868,#278869),(#278870,#278871),(#278872,#278873),(#278874,#278875),
(#278876,#278877),(#278878,#278879)),.UNSPECIFIED.,.F.,.F.,.F.,(6,1,1,1,
1,1,1,1,1,1,1,1,1,1,1,1,1,1,1,1,1,1,1,1,1,1,1,1,1,1,1,1,1,1,1,1,1,1,1,1,
1,1,1,1,1,1,1,1,1,1,1,1,1,1,1,1,1,1,1,1,1,1,1,1,1,1,1,1,1,1,1,1,1,1,1,1,
1,1,1,1,1,1,1,1,1,1,1,1,1,1,1,1,1,1,1,1,1,1,1,1,1,1,1,1,1,1,1,1,1,1,1,1,
1,1,1,1,1,1,1,1,1,1,1,1,1,1,1,1,1,1,1,1,1,1,1,1,1,1,1,1,1,1,1,1,1,1,1,1,
1,1,1,1,1,1,1,1,1,1,1,1,1,1,1,1,1,1,1,1,1,1,1,1,1,1,1,1,1,1,1,1,1,1,1,1,
1,1,1,1,1,1,1,1,1,1,1,1,1,1,1,1,1,1,1,1,1,1,1,1,1,1,1,1,1,1,1,1,1,1,1,1,
1,1,1,1,1,1,1,1,1,1,1,1,1,1,1,1,1,1,1,1,1,1,1,1,1,1,1,1,1,1,1,1,1,1,1,1,
1,1,1,1,1,1,1,1,1,1,1,1,1,1,1,1,1,1,1,1,1,1,1,1,1,1,1,1,1,1,1,1,1,1,1,1,
1,1,1,1,1,1,1,1,1,1,1,1,1,1,1,1,1,1,1,1,1,1,1,1,1,1,1,1,1,1,1,1,1,1,1,1,
1,1,1,1,1,1,1,1,1,1,1,1,1,1,1,1,1,1,1,1,1,1,1,1,1,1,1,1,1,1,1,1,1,1,1,1,
1,1,1,1,1,1,1,1,1,1,1,1,1,1,1,1,1,1,1,1,1,1,1,1,1,1,1,1,1,1,1,1,1,1,1,1,
1,1,1,1,1,1,1,1,1,1,1,1,1,1,1,1,1,1,1,1,1,1,1,1,1,1,1,1,1,1,1,1,1,1,1,1,
1,1,1,1,1,1,1,1,1,1,1,1,1,1,1,1,1,1,1,1,1,1,1,1,1,1,1,1,1,1,1,6),(2,2),
(0.143172103,0.144954128,0.146788991,0.148623853,0.150458716,0.152293578,
0.15412844,0.155963303,0.157798165,0.159633028,0.16146789,0.163302752,0.165137615,
0.166972477,0.168807339,0.170642202,0.172477064,0.174311927,0.176146789,
0.177981651,0.179816514,0.181651376,0.183486239,0.185321101,0.187155963,
0.188990826,0.190825688,0.19266055,0.194495413,0.196330275,0.198165138,
0.2,0.201834862,0.203669725,0.205504587,0.20733945,0.209174312,0.211009174,
0.212844037,0.214678899,0.216513761,0.218348624,0.220183486,0.222018349,
0.223853211,0.225688073,0.227522936,0.229357798,0.231192661,0.233027523,
0.234862385,0.236697248,0.23853211,0.240366972,0.242201835,0.244036697,
0.24587156,0.247706422,0.249541284,0.251376147,0.253211009,0.255045872,
0.256880734,0.258715596,0.260550459,0.262385321,0.264220183,0.266055046,
0.267889908,0.269724771,0.271559633,0.273394495,0.275229358,0.27706422,
0.278899083,0.280733945,0.282568807,0.28440367,0.286238532,0.288073394,
0.289908257,0.291743119,0.293577982,0.295412844,0.297247706,0.299082569,
0.300917431,0.302752294,0.304587156,0.306422018,0.308256881,0.310091743,
0.311926606,0.313761468,0.31559633,0.317431193,0.319266055,0.321100917,
0.32293578,0.324770642,0.326605505,0.328440367,0.330275229,0.332110092,
0.333944954,0.335779817,0.337614679,0.339449541,0.341284404,0.343119266,
0.344954128,0.346788991,0.348623853,0.350458716,0.352293578,0.35412844,
0.355963303,0.357798165,0.359633028,0.36146789,0.363302752,0.365137615,
0.366972477,0.368807339,0.370642202,0.372477064,0.374311927,0.376146789,
0.377981651,0.379816514,0.381651376,0.383486239,0.385321101,0.387155963,
0.388990826,0.390825688,0.39266055,0.394495413,0.396330275,0.398165138,
0.4,0.401834862,0.403669725,0.405504587,0.40733945,0.409174312,0.411009174,
0.412844037,0.414678899,0.416513761,0.418348624,0.420183486,0.422018349,
0.423853211,0.425688073,0.427522936,0.429357798,0.431192661,0.433027523,
0.434862385,0.436697248,0.43853211,0.440366972,0.442201835,0.444036697,
0.44587156,0.447706422,0.449541284,0.451376147,0.453211009,0.455045872,
0.456880734,0.458715596,0.460550459,0.462385321,0.464220183,0.466055046,
0.467889908,0.469724771,0.471559633,0.473394495,0.475229358,0.47706422,
0.478899083,0.480733945,0.482568807,0.48440367,0.486238532,0.488073394,
0.489908257,0.491743119,0.493577982,0.495412844,0.497247706,0.499082569,
0.500917431,0.502752294,0.504587156,0.506422018,0.508256881,0.510091743,
0.511926606,0.513761468,0.51559633,0.517431193,0.519266055,0.521100917,
0.52293578,0.524770642,0.526605505,0.528440367,0.530275229,0.532110092,
0.533944954,0.535779817,0.537614679,0.539449541,0.541284404,0.543119266,
0.544954128,0.546788991,0.548623853,0.550458716,0.552293578,0.55412844,
0.555963303,0.557798165,0.559633028,0.56146789,0.563302752,0.565137615,
0.566972477,0.568807339,0.570642202,0.572477064,0.574311927,0.576146789,
0.577981651,0.579816514,0.581651376,0.583486239,0.585321101,0.587155963,
0.588990826,0.590825688,0.59266055,0.594495413,0.596330275,0.598165138,
0.6,0.601834862,0.603669725,0.605504587,0.60733945,0.609174312,0.611009174,
0.612844037,0.614678899,0.616513761,0.618348624,0.620183486,0.622018349,
0.623853211,0.625688073,0.627522936,0.629357798,0.631192661,0.633027523,
0.634862385,0.636697248,0.63853211,0.640366972,0.642201835,0.644036697,
0.64587156,0.647706422,0.649541284,0.651376147,0.653211009,0.655045872,
0.656880734,0.658715596,0.660550459,0.662385321,0.664220183,0.666055046,
0.667889908,0.669724771,0.671559633,0.673394495,0.675229358,0.67706422,
0.678899083,0.680733945,0.682568807,0.68440367,0.686238532,0.688073394,
0.689908257,0.691743119,0.693577982,0.695412844,0.697247706,0.699082569,
0.700917431,0.702752294,0.704587156,0.706422018,0.708256881,0.710091743,
0.711926606,0.713761468,0.71559633,0.717431193,0.719266055,0.721100917,
0.72293578,0.724770642,0.726605505,0.728440367,0.730275229,0.732110092,
0.733944954,0.735779817,0.737614679,0.739449541,0.741284404,0.743119266,
0.744954128,0.746788991,0.748623853,0.750458716,0.752293578,0.75412844,
0.755963303,0.757798165,0.759633028,0.76146789,0.763302752,0.765137615,
0.766972477,0.768807339,0.770642202,0.772477064,0.774311927,0.776146789,
0.777981651,0.779816514,0.781651376,0.783486239,0.785321101,0.787155963,
0.788990826,0.790825688,0.79266055,0.794495413,0.796330275,0.798165138,
0.8,0.801834862,0.803669725,0.805504587,0.80733945,0.809174312,0.811009174,
0.812844037,0.814678899,0.816513761,0.818348624,0.820183486,0.822018349,
0.823853211,0.825688073,0.827522936,0.829357798,0.831192661,0.833027523,
0.834862385,0.836697248,0.83853211,0.840366972,0.842201835,0.844036697,
0.84587156,0.847706422,0.849541284,0.851376147,0.853211009,0.855045872,
0.856880734,0.858715596,0.860550459,0.862385321,0.864220183,0.866055046,
0.867889908,0.869724771,0.871559633,0.873394495,0.875229358,0.87706422,
0.878899083,0.880733945,0.882568807,0.88440367,0.886238532,0.888073394,
0.889908257,0.891743119,0.893577982,0.895412844,0.897247706,0.899082569,
0.900917431,0.902752294,0.904587156,0.906422018,0.908256881,0.910091743,
0.911926606,0.913761468,0.91559633,0.917431193,0.919266055,0.921100917,
0.92293578,0.924770642,0.926605505,0.928440367,0.930275229,0.932110092,
0.933944954,0.935779817,0.937614679,0.939449541,0.941284404,0.943119266,
0.944954128,0.946788991,0.948623853,0.950458716,0.952293578,0.95412844,
0.955963303,0.957798165,0.959633028,0.96146789,0.963302752,0.965137615,
0.966972477,0.968807339,0.970642202,0.972477064,0.974311927,0.976146789,
0.977981651,0.979816514,0.981651376,0.983486239,0.985321101,0.987155963,
0.988990826,0.990825688,0.99266055,0.994495413,0.996330275,0.998165138,
1.),(0.,0.36),.UNSPECIFIED.);
#6291=B_SPLINE_SURFACE_WITH_KNOTS('',5,1,((#279542,#279543),(#279544,#279545),
(#279546,#279547),(#279548,#279549),(#279550,#279551),(#279552,#279553),
(#279554,#279555),(#279556,#279557),(#279558,#279559),(#279560,#279561),
(#279562,#279563),(#279564,#279565),(#279566,#279567),(#279568,#279569),
(#279570,#279571),(#279572,#279573),(#279574,#279575),(#279576,#279577),
(#279578,#279579),(#279580,#279581),(#279582,#279583),(#279584,#279585),
(#279586,#279587),(#279588,#279589),(#279590,#279591),(#279592,#279593),
(#279594,#279595),(#279596,#279597),(#279598,#279599),(#279600,#279601),
(#279602,#279603),(#279604,#279605),(#279606,#279607),(#279608,#279609),
(#279610,#279611),(#279612,#279613),(#279614,#279615),(#279616,#279617),
(#279618,#279619),(#279620,#279621),(#279622,#279623),(#279624,#279625),
(#279626,#279627),(#279628,#279629),(#279630,#279631),(#279632,#279633),
(#279634,#279635),(#279636,#279637),(#279638,#279639),(#279640,#279641),
(#279642,#279643),(#279644,#279645),(#279646,#279647),(#279648,#279649),
(#279650,#279651),(#279652,#279653),(#279654,#279655),(#279656,#279657),
(#279658,#279659),(#279660,#279661),(#279662,#279663),(#279664,#279665),
(#279666,#279667),(#279668,#279669),(#279670,#279671),(#279672,#279673),
(#279674,#279675),(#279676,#279677),(#279678,#279679),(#279680,#279681),
(#279682,#279683),(#279684,#279685),(#279686,#279687),(#279688,#279689),
(#279690,#279691),(#279692,#279693),(#279694,#279695),(#279696,#279697),
(#279698,#279699),(#279700,#279701),(#279702,#279703),(#279704,#279705),
(#279706,#279707),(#279708,#279709),(#279710,#279711),(#279712,#279713),
(#279714,#279715),(#279716,#279717),(#279718,#279719),(#279720,#279721),
(#279722,#279723),(#279724,#279725),(#279726,#279727),(#279728,#279729),
(#279730,#279731),(#279732,#279733),(#279734,#279735),(#279736,#279737),
(#279738,#279739),(#279740,#279741),(#279742,#279743),(#279744,#279745),
(#279746,#279747),(#279748,#279749),(#279750,#279751),(#279752,#279753),
(#279754,#279755),(#279756,#279757),(#279758,#279759),(#279760,#279761),
(#279762,#279763),(#279764,#279765),(#279766,#279767),(#279768,#279769),
(#279770,#279771),(#279772,#279773),(#279774,#279775),(#279776,#279777),
(#279778,#279779),(#279780,#279781),(#279782,#279783),(#279784,#279785),
(#279786,#279787),(#279788,#279789),(#279790,#279791),(#279792,#279793),
(#279794,#279795),(#279796,#279797),(#279798,#279799),(#279800,#279801),
(#279802,#279803),(#279804,#279805),(#279806,#279807),(#279808,#279809),
(#279810,#279811),(#279812,#279813),(#279814,#279815),(#279816,#279817),
(#279818,#279819),(#279820,#279821),(#279822,#279823),(#279824,#279825),
(#279826,#279827),(#279828,#279829),(#279830,#279831),(#279832,#279833),
(#279834,#279835),(#279836,#279837),(#279838,#279839),(#279840,#279841),
(#279842,#279843),(#279844,#279845),(#279846,#279847),(#279848,#279849),
(#279850,#279851),(#279852,#279853),(#279854,#279855),(#279856,#279857),
(#279858,#279859),(#279860,#279861),(#279862,#279863),(#279864,#279865),
(#279866,#279867),(#279868,#279869),(#279870,#279871),(#279872,#279873),
(#279874,#279875),(#279876,#279877),(#279878,#279879),(#279880,#279881),
(#279882,#279883),(#279884,#279885),(#279886,#279887),(#279888,#279889),
(#279890,#279891),(#279892,#279893),(#279894,#279895),(#279896,#279897),
(#279898,#279899),(#279900,#279901),(#279902,#279903),(#279904,#279905),
(#279906,#279907),(#279908,#279909),(#279910,#279911),(#279912,#279913),
(#279914,#279915),(#279916,#279917),(#279918,#279919),(#279920,#279921),
(#279922,#279923),(#279924,#279925),(#279926,#279927),(#279928,#279929),
(#279930,#279931),(#279932,#279933),(#279934,#279935),(#279936,#279937),
(#279938,#279939),(#279940,#279941),(#279942,#279943),(#279944,#279945),
(#279946,#279947),(#279948,#279949),(#279950,#279951),(#279952,#279953),
(#279954,#279955),(#279956,#279957),(#279958,#279959),(#279960,#279961),
(#279962,#279963),(#279964,#279965),(#279966,#279967),(#279968,#279969),
(#279970,#279971),(#279972,#279973),(#279974,#279975),(#279976,#279977),
(#279978,#279979),(#279980,#279981),(#279982,#279983),(#279984,#279985),
(#279986,#279987),(#279988,#279989),(#279990,#279991),(#279992,#279993),
(#279994,#279995),(#279996,#279997),(#279998,#279999),(#280000,#280001),
(#280002,#280003),(#280004,#280005),(#280006,#280007),(#280008,#280009),
(#280010,#280011),(#280012,#280013),(#280014,#280015),(#280016,#280017),
(#280018,#280019),(#280020,#280021),(#280022,#280023),(#280024,#280025),
(#280026,#280027),(#280028,#280029),(#280030,#280031),(#280032,#280033),
(#280034,#280035),(#280036,#280037),(#280038,#280039),(#280040,#280041),
(#280042,#280043),(#280044,#280045),(#280046,#280047),(#280048,#280049),
(#280050,#280051),(#280052,#280053),(#280054,#280055),(#280056,#280057),
(#280058,#280059),(#280060,#280061),(#280062,#280063),(#280064,#280065),
(#280066,#280067),(#280068,#280069),(#280070,#280071),(#280072,#280073),
(#280074,#280075),(#280076,#280077),(#280078,#280079),(#280080,#280081),
(#280082,#280083),(#280084,#280085),(#280086,#280087),(#280088,#280089),
(#280090,#280091),(#280092,#280093),(#280094,#280095),(#280096,#280097),
(#280098,#280099),(#280100,#280101),(#280102,#280103),(#280104,#280105),
(#280106,#280107),(#280108,#280109),(#280110,#280111),(#280112,#280113),
(#280114,#280115),(#280116,#280117),(#280118,#280119),(#280120,#280121),
(#280122,#280123),(#280124,#280125),(#280126,#280127),(#280128,#280129),
(#280130,#280131),(#280132,#280133),(#280134,#280135),(#280136,#280137),
(#280138,#280139),(#280140,#280141),(#280142,#280143),(#280144,#280145),
(#280146,#280147),(#280148,#280149),(#280150,#280151),(#280152,#280153),
(#280154,#280155),(#280156,#280157),(#280158,#280159),(#280160,#280161),
(#280162,#280163),(#280164,#280165),(#280166,#280167),(#280168,#280169),
(#280170,#280171),(#280172,#280173),(#280174,#280175),(#280176,#280177),
(#280178,#280179),(#280180,#280181),(#280182,#280183),(#280184,#280185),
(#280186,#280187),(#280188,#280189),(#280190,#280191),(#280192,#280193),
(#280194,#280195),(#280196,#280197),(#280198,#280199),(#280200,#280201),
(#280202,#280203),(#280204,#280205),(#280206,#280207),(#280208,#280209),
(#280210,#280211),(#280212,#280213),(#280214,#280215),(#280216,#280217),
(#280218,#280219),(#280220,#280221),(#280222,#280223),(#280224,#280225),
(#280226,#280227),(#280228,#280229),(#280230,#280231),(#280232,#280233),
(#280234,#280235),(#280236,#280237),(#280238,#280239),(#280240,#280241),
(#280242,#280243),(#280244,#280245),(#280246,#280247),(#280248,#280249),
(#280250,#280251),(#280252,#280253),(#280254,#280255),(#280256,#280257),
(#280258,#280259),(#280260,#280261),(#280262,#280263),(#280264,#280265),
(#280266,#280267),(#280268,#280269),(#280270,#280271),(#280272,#280273),
(#280274,#280275),(#280276,#280277),(#280278,#280279),(#280280,#280281),
(#280282,#280283),(#280284,#280285),(#280286,#280287),(#280288,#280289),
(#280290,#280291),(#280292,#280293),(#280294,#280295),(#280296,#280297),
(#280298,#280299),(#280300,#280301),(#280302,#280303),(#280304,#280305),
(#280306,#280307),(#280308,#280309),(#280310,#280311),(#280312,#280313),
(#280314,#280315),(#280316,#280317),(#280318,#280319),(#280320,#280321),
(#280322,#280323),(#280324,#280325),(#280326,#280327),(#280328,#280329),
(#280330,#280331),(#280332,#280333),(#280334,#280335),(#280336,#280337),
(#280338,#280339),(#280340,#280341),(#280342,#280343),(#280344,#280345),
(#280346,#280347),(#280348,#280349),(#280350,#280351),(#280352,#280353),
(#280354,#280355),(#280356,#280357),(#280358,#280359),(#280360,#280361),
(#280362,#280363),(#280364,#280365),(#280366,#280367),(#280368,#280369),
(#280370,#280371),(#280372,#280373),(#280374,#280375),(#280376,#280377),
(#280378,#280379),(#280380,#280381),(#280382,#280383),(#280384,#280385),
(#280386,#280387),(#280388,#280389),(#280390,#280391),(#280392,#280393),
(#280394,#280395),(#280396,#280397),(#280398,#280399),(#280400,#280401),
(#280402,#280403),(#280404,#280405),(#280406,#280407),(#280408,#280409),
(#280410,#280411),(#280412,#280413),(#280414,#280415),(#280416,#280417),
(#280418,#280419),(#280420,#280421),(#280422,#280423),(#280424,#280425),
(#280426,#280427),(#280428,#280429),(#280430,#280431),(#280432,#280433),
(#280434,#280435),(#280436,#280437),(#280438,#280439),(#280440,#280441),
(#280442,#280443),(#280444,#280445),(#280446,#280447),(#280448,#280449),
(#280450,#280451),(#280452,#280453),(#280454,#280455),(#280456,#280457),
(#280458,#280459),(#280460,#280461),(#280462,#280463),(#280464,#280465),
(#280466,#280467),(#280468,#280469),(#280470,#280471),(#280472,#280473),
(#280474,#280475),(#280476,#280477),(#280478,#280479),(#280480,#280481),
(#280482,#280483),(#280484,#280485)),.UNSPECIFIED.,.F.,.F.,.F.,(6,1,1,1,
1,1,1,1,1,1,1,1,1,1,1,1,1,1,1,1,1,1,1,1,1,1,1,1,1,1,1,1,1,1,1,1,1,1,1,1,
1,1,1,1,1,1,1,1,1,1,1,1,1,1,1,1,1,1,1,1,1,1,1,1,1,1,1,1,1,1,1,1,1,1,1,1,
1,1,1,1,1,1,1,1,1,1,1,1,1,1,1,1,1,1,1,1,1,1,1,1,1,1,1,1,1,1,1,1,1,1,1,1,
1,1,1,1,1,1,1,1,1,1,1,1,1,1,1,1,1,1,1,1,1,1,1,1,1,1,1,1,1,1,1,1,1,1,1,1,
1,1,1,1,1,1,1,1,1,1,1,1,1,1,1,1,1,1,1,1,1,1,1,1,1,1,1,1,1,1,1,1,1,1,1,1,
1,1,1,1,1,1,1,1,1,1,1,1,1,1,1,1,1,1,1,1,1,1,1,1,1,1,1,1,1,1,1,1,1,1,1,1,
1,1,1,1,1,1,1,1,1,1,1,1,1,1,1,1,1,1,1,1,1,1,1,1,1,1,1,1,1,1,1,1,1,1,1,1,
1,1,1,1,1,1,1,1,1,1,1,1,1,1,1,1,1,1,1,1,1,1,1,1,1,1,1,1,1,1,1,1,1,1,1,1,
1,1,1,1,1,1,1,1,1,1,1,1,1,1,1,1,1,1,1,1,1,1,1,1,1,1,1,1,1,1,1,1,1,1,1,1,
1,1,1,1,1,1,1,1,1,1,1,1,1,1,1,1,1,1,1,1,1,1,1,1,1,1,1,1,1,1,1,1,1,1,1,1,
1,1,1,1,1,1,1,1,1,1,1,1,1,1,1,1,1,1,1,1,1,1,1,1,1,1,1,1,1,1,1,1,1,1,1,1,
1,1,1,1,1,1,1,1,1,1,1,1,1,1,1,1,1,1,1,1,1,1,1,1,1,1,1,1,1,1,1,1,1,1,1,1,
1,1,1,1,1,1,1,1,1,1,1,1,1,1,1,1,1,1,1,1,1,1,1,1,1,1,1,1,1,1,1,6),(2,2),
(0.143172103,0.144954128,0.146788991,0.148623853,0.150458716,0.152293578,
0.15412844,0.155963303,0.157798165,0.159633028,0.16146789,0.163302752,0.165137615,
0.166972477,0.168807339,0.170642202,0.172477064,0.174311927,0.176146789,
0.177981651,0.179816514,0.181651376,0.183486239,0.185321101,0.187155963,
0.188990826,0.190825688,0.19266055,0.194495413,0.196330275,0.198165138,
0.2,0.201834862,0.203669725,0.205504587,0.20733945,0.209174312,0.211009174,
0.212844037,0.214678899,0.216513761,0.218348624,0.220183486,0.222018349,
0.223853211,0.225688073,0.227522936,0.229357798,0.231192661,0.233027523,
0.234862385,0.236697248,0.23853211,0.240366972,0.242201835,0.244036697,
0.24587156,0.247706422,0.249541284,0.251376147,0.253211009,0.255045872,
0.256880734,0.258715596,0.260550459,0.262385321,0.264220183,0.266055046,
0.267889908,0.269724771,0.271559633,0.273394495,0.275229358,0.27706422,
0.278899083,0.280733945,0.282568807,0.28440367,0.286238532,0.288073394,
0.289908257,0.291743119,0.293577982,0.295412844,0.297247706,0.299082569,
0.300917431,0.302752294,0.304587156,0.306422018,0.308256881,0.310091743,
0.311926606,0.313761468,0.31559633,0.317431193,0.319266055,0.321100917,
0.32293578,0.324770642,0.326605505,0.328440367,0.330275229,0.332110092,
0.333944954,0.335779817,0.337614679,0.339449541,0.341284404,0.343119266,
0.344954128,0.346788991,0.348623853,0.350458716,0.352293578,0.35412844,
0.355963303,0.357798165,0.359633028,0.36146789,0.363302752,0.365137615,
0.366972477,0.368807339,0.370642202,0.372477064,0.374311927,0.376146789,
0.377981651,0.379816514,0.381651376,0.383486239,0.385321101,0.387155963,
0.388990826,0.390825688,0.39266055,0.394495413,0.396330275,0.398165138,
0.4,0.401834862,0.403669725,0.405504587,0.40733945,0.409174312,0.411009174,
0.412844037,0.414678899,0.416513761,0.418348624,0.420183486,0.422018349,
0.423853211,0.425688073,0.427522936,0.429357798,0.431192661,0.433027523,
0.434862385,0.436697248,0.43853211,0.440366972,0.442201835,0.444036697,
0.44587156,0.447706422,0.449541284,0.451376147,0.453211009,0.455045872,
0.456880734,0.458715596,0.460550459,0.462385321,0.464220183,0.466055046,
0.467889908,0.469724771,0.471559633,0.473394495,0.475229358,0.47706422,
0.478899083,0.480733945,0.482568807,0.48440367,0.486238532,0.488073394,
0.489908257,0.491743119,0.493577982,0.495412844,0.497247706,0.499082569,
0.500917431,0.502752294,0.504587156,0.506422018,0.508256881,0.510091743,
0.511926606,0.513761468,0.51559633,0.517431193,0.519266055,0.521100917,
0.52293578,0.524770642,0.526605505,0.528440367,0.530275229,0.532110092,
0.533944954,0.535779817,0.537614679,0.539449541,0.541284404,0.543119266,
0.544954128,0.546788991,0.548623853,0.550458716,0.552293578,0.55412844,
0.555963303,0.557798165,0.559633028,0.56146789,0.563302752,0.565137615,
0.566972477,0.568807339,0.570642202,0.572477064,0.574311927,0.576146789,
0.577981651,0.579816514,0.581651376,0.583486239,0.585321101,0.587155963,
0.588990826,0.590825688,0.59266055,0.594495413,0.596330275,0.598165138,
0.6,0.601834862,0.603669725,0.605504587,0.60733945,0.609174312,0.611009174,
0.612844037,0.614678899,0.616513761,0.618348624,0.620183486,0.622018349,
0.623853211,0.625688073,0.627522936,0.629357798,0.631192661,0.633027523,
0.634862385,0.636697248,0.63853211,0.640366972,0.642201835,0.644036697,
0.64587156,0.647706422,0.649541284,0.651376147,0.653211009,0.655045872,
0.656880734,0.658715596,0.660550459,0.662385321,0.664220183,0.666055046,
0.667889908,0.669724771,0.671559633,0.673394495,0.675229358,0.67706422,
0.678899083,0.680733945,0.682568807,0.68440367,0.686238532,0.688073394,
0.689908257,0.691743119,0.693577982,0.695412844,0.697247706,0.699082569,
0.700917431,0.702752294,0.704587156,0.706422018,0.708256881,0.710091743,
0.711926606,0.713761468,0.71559633,0.717431193,0.719266055,0.721100917,
0.72293578,0.724770642,0.726605505,0.728440367,0.730275229,0.732110092,
0.733944954,0.735779817,0.737614679,0.739449541,0.741284404,0.743119266,
0.744954128,0.746788991,0.748623853,0.750458716,0.752293578,0.75412844,
0.755963303,0.757798165,0.759633028,0.76146789,0.763302752,0.765137615,
0.766972477,0.768807339,0.770642202,0.772477064,0.774311927,0.776146789,
0.777981651,0.779816514,0.781651376,0.783486239,0.785321101,0.787155963,
0.788990826,0.790825688,0.79266055,0.794495413,0.796330275,0.798165138,
0.8,0.801834862,0.803669725,0.805504587,0.80733945,0.809174312,0.811009174,
0.812844037,0.814678899,0.816513761,0.818348624,0.820183486,0.822018349,
0.823853211,0.825688073,0.827522936,0.829357798,0.831192661,0.833027523,
0.834862385,0.836697248,0.83853211,0.840366972,0.842201835,0.844036697,
0.84587156,0.847706422,0.849541284,0.851376147,0.853211009,0.855045872,
0.856880734,0.858715596,0.860550459,0.862385321,0.864220183,0.866055046,
0.867889908,0.869724771,0.871559633,0.873394495,0.875229358,0.87706422,
0.878899083,0.880733945,0.882568807,0.88440367,0.886238532,0.888073394,
0.889908257,0.891743119,0.893577982,0.895412844,0.897247706,0.899082569,
0.900917431,0.902752294,0.904587156,0.906422018,0.908256881,0.910091743,
0.911926606,0.913761468,0.91559633,0.917431193,0.919266055,0.921100917,
0.92293578,0.924770642,0.926605505,0.928440367,0.930275229,0.932110092,
0.933944954,0.935779817,0.937614679,0.939449541,0.941284404,0.943119266,
0.944954128,0.946788991,0.948623853,0.950458716,0.952293578,0.95412844,
0.955963303,0.957798165,0.959633028,0.96146789,0.963302752,0.965137615,
0.966972477,0.968807339,0.970642202,0.972477064,0.974311927,0.976146789,
0.977981651,0.979816514,0.981651376,0.983486239,0.985321101,0.987155963,
0.988990826,0.990825688,0.99266055,0.994495413,0.996330275,0.998165138,
1.),(0.,0.36),.UNSPECIFIED.);
#6292=B_SPLINE_SURFACE_WITH_KNOTS('',5,1,((#281133,#281134),(#281135,#281136),
(#281137,#281138),(#281139,#281140),(#281141,#281142),(#281143,#281144),
(#281145,#281146),(#281147,#281148),(#281149,#281150),(#281151,#281152),
(#281153,#281154),(#281155,#281156),(#281157,#281158),(#281159,#281160),
(#281161,#281162),(#281163,#281164),(#281165,#281166),(#281167,#281168),
(#281169,#281170),(#281171,#281172),(#281173,#281174),(#281175,#281176),
(#281177,#281178),(#281179,#281180),(#281181,#281182),(#281183,#281184),
(#281185,#281186),(#281187,#281188),(#281189,#281190),(#281191,#281192),
(#281193,#281194),(#281195,#281196),(#281197,#281198),(#281199,#281200),
(#281201,#281202),(#281203,#281204),(#281205,#281206),(#281207,#281208),
(#281209,#281210),(#281211,#281212),(#281213,#281214),(#281215,#281216),
(#281217,#281218),(#281219,#281220),(#281221,#281222),(#281223,#281224),
(#281225,#281226),(#281227,#281228),(#281229,#281230),(#281231,#281232),
(#281233,#281234),(#281235,#281236),(#281237,#281238),(#281239,#281240),
(#281241,#281242),(#281243,#281244),(#281245,#281246),(#281247,#281248),
(#281249,#281250),(#281251,#281252),(#281253,#281254),(#281255,#281256),
(#281257,#281258),(#281259,#281260),(#281261,#281262),(#281263,#281264),
(#281265,#281266),(#281267,#281268),(#281269,#281270),(#281271,#281272),
(#281273,#281274),(#281275,#281276),(#281277,#281278),(#281279,#281280),
(#281281,#281282),(#281283,#281284),(#281285,#281286),(#281287,#281288),
(#281289,#281290),(#281291,#281292),(#281293,#281294),(#281295,#281296),
(#281297,#281298),(#281299,#281300),(#281301,#281302),(#281303,#281304),
(#281305,#281306),(#281307,#281308),(#281309,#281310),(#281311,#281312),
(#281313,#281314),(#281315,#281316),(#281317,#281318),(#281319,#281320),
(#281321,#281322),(#281323,#281324),(#281325,#281326),(#281327,#281328),
(#281329,#281330),(#281331,#281332),(#281333,#281334),(#281335,#281336),
(#281337,#281338),(#281339,#281340),(#281341,#281342),(#281343,#281344),
(#281345,#281346),(#281347,#281348),(#281349,#281350),(#281351,#281352),
(#281353,#281354),(#281355,#281356),(#281357,#281358),(#281359,#281360),
(#281361,#281362),(#281363,#281364),(#281365,#281366),(#281367,#281368),
(#281369,#281370),(#281371,#281372),(#281373,#281374),(#281375,#281376),
(#281377,#281378),(#281379,#281380),(#281381,#281382),(#281383,#281384),
(#281385,#281386),(#281387,#281388),(#281389,#281390),(#281391,#281392),
(#281393,#281394),(#281395,#281396),(#281397,#281398),(#281399,#281400),
(#281401,#281402),(#281403,#281404),(#281405,#281406),(#281407,#281408),
(#281409,#281410),(#281411,#281412),(#281413,#281414),(#281415,#281416),
(#281417,#281418),(#281419,#281420),(#281421,#281422),(#281423,#281424),
(#281425,#281426),(#281427,#281428),(#281429,#281430),(#281431,#281432),
(#281433,#281434),(#281435,#281436),(#281437,#281438),(#281439,#281440),
(#281441,#281442),(#281443,#281444),(#281445,#281446),(#281447,#281448),
(#281449,#281450),(#281451,#281452),(#281453,#281454),(#281455,#281456),
(#281457,#281458),(#281459,#281460),(#281461,#281462),(#281463,#281464),
(#281465,#281466),(#281467,#281468),(#281469,#281470),(#281471,#281472),
(#281473,#281474),(#281475,#281476),(#281477,#281478),(#281479,#281480),
(#281481,#281482),(#281483,#281484),(#281485,#281486),(#281487,#281488),
(#281489,#281490),(#281491,#281492),(#281493,#281494),(#281495,#281496),
(#281497,#281498),(#281499,#281500),(#281501,#281502),(#281503,#281504),
(#281505,#281506),(#281507,#281508),(#281509,#281510),(#281511,#281512),
(#281513,#281514),(#281515,#281516),(#281517,#281518),(#281519,#281520),
(#281521,#281522),(#281523,#281524),(#281525,#281526),(#281527,#281528),
(#281529,#281530),(#281531,#281532),(#281533,#281534),(#281535,#281536),
(#281537,#281538),(#281539,#281540),(#281541,#281542),(#281543,#281544),
(#281545,#281546),(#281547,#281548),(#281549,#281550),(#281551,#281552),
(#281553,#281554),(#281555,#281556),(#281557,#281558),(#281559,#281560),
(#281561,#281562),(#281563,#281564),(#281565,#281566),(#281567,#281568),
(#281569,#281570),(#281571,#281572),(#281573,#281574),(#281575,#281576),
(#281577,#281578),(#281579,#281580),(#281581,#281582),(#281583,#281584),
(#281585,#281586),(#281587,#281588),(#281589,#281590),(#281591,#281592),
(#281593,#281594),(#281595,#281596),(#281597,#281598),(#281599,#281600),
(#281601,#281602),(#281603,#281604),(#281605,#281606),(#281607,#281608),
(#281609,#281610),(#281611,#281612),(#281613,#281614),(#281615,#281616),
(#281617,#281618),(#281619,#281620),(#281621,#281622),(#281623,#281624),
(#281625,#281626),(#281627,#281628),(#281629,#281630),(#281631,#281632),
(#281633,#281634),(#281635,#281636),(#281637,#281638),(#281639,#281640),
(#281641,#281642),(#281643,#281644),(#281645,#281646),(#281647,#281648),
(#281649,#281650),(#281651,#281652),(#281653,#281654),(#281655,#281656),
(#281657,#281658),(#281659,#281660),(#281661,#281662),(#281663,#281664),
(#281665,#281666),(#281667,#281668),(#281669,#281670),(#281671,#281672),
(#281673,#281674),(#281675,#281676),(#281677,#281678),(#281679,#281680),
(#281681,#281682),(#281683,#281684),(#281685,#281686),(#281687,#281688),
(#281689,#281690),(#281691,#281692),(#281693,#281694),(#281695,#281696),
(#281697,#281698),(#281699,#281700),(#281701,#281702),(#281703,#281704),
(#281705,#281706),(#281707,#281708),(#281709,#281710),(#281711,#281712),
(#281713,#281714),(#281715,#281716),(#281717,#281718),(#281719,#281720),
(#281721,#281722),(#281723,#281724),(#281725,#281726),(#281727,#281728),
(#281729,#281730),(#281731,#281732),(#281733,#281734),(#281735,#281736),
(#281737,#281738),(#281739,#281740),(#281741,#281742),(#281743,#281744),
(#281745,#281746),(#281747,#281748),(#281749,#281750),(#281751,#281752),
(#281753,#281754),(#281755,#281756),(#281757,#281758),(#281759,#281760),
(#281761,#281762),(#281763,#281764),(#281765,#281766),(#281767,#281768),
(#281769,#281770),(#281771,#281772),(#281773,#281774),(#281775,#281776),
(#281777,#281778),(#281779,#281780),(#281781,#281782),(#281783,#281784),
(#281785,#281786),(#281787,#281788),(#281789,#281790),(#281791,#281792),
(#281793,#281794),(#281795,#281796),(#281797,#281798),(#281799,#281800),
(#281801,#281802),(#281803,#281804),(#281805,#281806),(#281807,#281808),
(#281809,#281810),(#281811,#281812),(#281813,#281814),(#281815,#281816),
(#281817,#281818),(#281819,#281820),(#281821,#281822),(#281823,#281824),
(#281825,#281826),(#281827,#281828),(#281829,#281830),(#281831,#281832),
(#281833,#281834),(#281835,#281836),(#281837,#281838),(#281839,#281840),
(#281841,#281842),(#281843,#281844),(#281845,#281846),(#281847,#281848),
(#281849,#281850),(#281851,#281852),(#281853,#281854),(#281855,#281856),
(#281857,#281858),(#281859,#281860),(#281861,#281862),(#281863,#281864),
(#281865,#281866),(#281867,#281868),(#281869,#281870),(#281871,#281872),
(#281873,#281874),(#281875,#281876),(#281877,#281878),(#281879,#281880),
(#281881,#281882),(#281883,#281884),(#281885,#281886),(#281887,#281888),
(#281889,#281890),(#281891,#281892),(#281893,#281894),(#281895,#281896),
(#281897,#281898),(#281899,#281900),(#281901,#281902),(#281903,#281904),
(#281905,#281906),(#281907,#281908),(#281909,#281910),(#281911,#281912),
(#281913,#281914),(#281915,#281916),(#281917,#281918),(#281919,#281920),
(#281921,#281922),(#281923,#281924),(#281925,#281926),(#281927,#281928),
(#281929,#281930),(#281931,#281932),(#281933,#281934),(#281935,#281936),
(#281937,#281938),(#281939,#281940),(#281941,#281942),(#281943,#281944),
(#281945,#281946),(#281947,#281948),(#281949,#281950),(#281951,#281952),
(#281953,#281954),(#281955,#281956),(#281957,#281958),(#281959,#281960),
(#281961,#281962),(#281963,#281964),(#281965,#281966),(#281967,#281968),
(#281969,#281970),(#281971,#281972),(#281973,#281974),(#281975,#281976),
(#281977,#281978),(#281979,#281980),(#281981,#281982),(#281983,#281984),
(#281985,#281986),(#281987,#281988),(#281989,#281990),(#281991,#281992),
(#281993,#281994),(#281995,#281996),(#281997,#281998),(#281999,#282000),
(#282001,#282002),(#282003,#282004),(#282005,#282006),(#282007,#282008),
(#282009,#282010),(#282011,#282012),(#282013,#282014),(#282015,#282016),
(#282017,#282018),(#282019,#282020),(#282021,#282022),(#282023,#282024),
(#282025,#282026),(#282027,#282028),(#282029,#282030),(#282031,#282032),
(#282033,#282034),(#282035,#282036),(#282037,#282038),(#282039,#282040),
(#282041,#282042),(#282043,#282044),(#282045,#282046),(#282047,#282048),
(#282049,#282050),(#282051,#282052),(#282053,#282054),(#282055,#282056),
(#282057,#282058),(#282059,#282060),(#282061,#282062),(#282063,#282064),
(#282065,#282066),(#282067,#282068),(#282069,#282070),(#282071,#282072),
(#282073,#282074),(#282075,#282076)),.UNSPECIFIED.,.F.,.F.,.F.,(6,1,1,1,
1,1,1,1,1,1,1,1,1,1,1,1,1,1,1,1,1,1,1,1,1,1,1,1,1,1,1,1,1,1,1,1,1,1,1,1,
1,1,1,1,1,1,1,1,1,1,1,1,1,1,1,1,1,1,1,1,1,1,1,1,1,1,1,1,1,1,1,1,1,1,1,1,
1,1,1,1,1,1,1,1,1,1,1,1,1,1,1,1,1,1,1,1,1,1,1,1,1,1,1,1,1,1,1,1,1,1,1,1,
1,1,1,1,1,1,1,1,1,1,1,1,1,1,1,1,1,1,1,1,1,1,1,1,1,1,1,1,1,1,1,1,1,1,1,1,
1,1,1,1,1,1,1,1,1,1,1,1,1,1,1,1,1,1,1,1,1,1,1,1,1,1,1,1,1,1,1,1,1,1,1,1,
1,1,1,1,1,1,1,1,1,1,1,1,1,1,1,1,1,1,1,1,1,1,1,1,1,1,1,1,1,1,1,1,1,1,1,1,
1,1,1,1,1,1,1,1,1,1,1,1,1,1,1,1,1,1,1,1,1,1,1,1,1,1,1,1,1,1,1,1,1,1,1,1,
1,1,1,1,1,1,1,1,1,1,1,1,1,1,1,1,1,1,1,1,1,1,1,1,1,1,1,1,1,1,1,1,1,1,1,1,
1,1,1,1,1,1,1,1,1,1,1,1,1,1,1,1,1,1,1,1,1,1,1,1,1,1,1,1,1,1,1,1,1,1,1,1,
1,1,1,1,1,1,1,1,1,1,1,1,1,1,1,1,1,1,1,1,1,1,1,1,1,1,1,1,1,1,1,1,1,1,1,1,
1,1,1,1,1,1,1,1,1,1,1,1,1,1,1,1,1,1,1,1,1,1,1,1,1,1,1,1,1,1,1,1,1,1,1,1,
1,1,1,1,1,1,1,1,1,1,1,1,1,1,1,1,1,1,1,1,1,1,1,1,1,1,1,1,1,1,1,1,1,1,1,1,
1,1,1,1,1,1,1,1,1,1,1,1,1,1,1,1,1,1,1,1,1,1,1,1,1,1,1,1,1,1,1,6),(2,2),
(-1.,-0.998165138,-0.996330275,-0.994495413,-0.99266055,-0.990825688,-0.988990826,
-0.987155963,-0.985321101,-0.983486239,-0.981651376,-0.979816514,-0.977981651,
-0.976146789,-0.974311927,-0.972477064,-0.970642202,-0.968807339,-0.966972477,
-0.965137615,-0.963302752,-0.96146789,-0.959633028,-0.957798165,-0.955963303,
-0.95412844,-0.952293578,-0.950458716,-0.948623853,-0.946788991,-0.944954128,
-0.943119266,-0.941284404,-0.939449541,-0.937614679,-0.935779817,-0.933944954,
-0.932110092,-0.930275229,-0.928440367,-0.926605505,-0.924770642,-0.92293578,
-0.921100917,-0.919266055,-0.917431193,-0.91559633,-0.913761468,-0.911926606,
-0.910091743,-0.908256881,-0.906422018,-0.904587156,-0.902752294,-0.900917431,
-0.899082569,-0.897247706,-0.895412844,-0.893577982,-0.891743119,-0.889908257,
-0.888073394,-0.886238532,-0.88440367,-0.882568807,-0.880733945,-0.878899083,
-0.87706422,-0.875229358,-0.873394495,-0.871559633,-0.869724771,-0.867889908,
-0.866055046,-0.864220183,-0.862385321,-0.860550459,-0.858715596,-0.856880734,
-0.855045872,-0.853211009,-0.851376147,-0.849541284,-0.847706422,-0.84587156,
-0.844036697,-0.842201835,-0.840366972,-0.83853211,-0.836697248,-0.834862385,
-0.833027523,-0.831192661,-0.829357798,-0.827522936,-0.825688073,-0.823853211,
-0.822018349,-0.820183486,-0.818348624,-0.816513761,-0.814678899,-0.812844037,
-0.811009174,-0.809174312,-0.80733945,-0.805504587,-0.803669725,-0.801834862,
-0.8,-0.798165138,-0.796330275,-0.794495413,-0.79266055,-0.790825688,-0.788990826,
-0.787155963,-0.785321101,-0.783486239,-0.781651376,-0.779816514,-0.777981651,
-0.776146789,-0.774311927,-0.772477064,-0.770642202,-0.768807339,-0.766972477,
-0.765137615,-0.763302752,-0.76146789,-0.759633028,-0.757798165,-0.755963303,
-0.75412844,-0.752293578,-0.750458716,-0.748623853,-0.746788991,-0.744954128,
-0.743119266,-0.741284404,-0.739449541,-0.737614679,-0.735779817,-0.733944954,
-0.732110092,-0.730275229,-0.728440367,-0.726605505,-0.724770642,-0.72293578,
-0.721100917,-0.719266055,-0.717431193,-0.71559633,-0.713761468,-0.711926606,
-0.710091743,-0.708256881,-0.706422018,-0.704587156,-0.702752294,-0.700917431,
-0.699082569,-0.697247706,-0.695412844,-0.693577982,-0.691743119,-0.689908257,
-0.688073394,-0.686238532,-0.68440367,-0.682568807,-0.680733945,-0.678899083,
-0.67706422,-0.675229358,-0.673394495,-0.671559633,-0.669724771,-0.667889908,
-0.666055046,-0.664220183,-0.662385321,-0.660550459,-0.658715596,-0.656880734,
-0.655045872,-0.653211009,-0.651376147,-0.649541284,-0.647706422,-0.64587156,
-0.644036697,-0.642201835,-0.640366972,-0.63853211,-0.636697248,-0.634862385,
-0.633027523,-0.631192661,-0.629357798,-0.627522936,-0.625688073,-0.623853211,
-0.622018349,-0.620183486,-0.618348624,-0.616513761,-0.614678899,-0.612844037,
-0.611009174,-0.609174312,-0.60733945,-0.605504587,-0.603669725,-0.601834862,
-0.6,-0.598165138,-0.596330275,-0.594495413,-0.59266055,-0.590825688,-0.588990826,
-0.587155963,-0.585321101,-0.583486239,-0.581651376,-0.579816514,-0.577981651,
-0.576146789,-0.574311927,-0.572477064,-0.570642202,-0.568807339,-0.566972477,
-0.565137615,-0.563302752,-0.56146789,-0.559633028,-0.557798165,-0.555963303,
-0.55412844,-0.552293578,-0.550458716,-0.548623853,-0.546788991,-0.544954128,
-0.543119266,-0.541284404,-0.539449541,-0.537614679,-0.535779817,-0.533944954,
-0.532110092,-0.530275229,-0.528440367,-0.526605505,-0.524770642,-0.52293578,
-0.521100917,-0.519266055,-0.517431193,-0.51559633,-0.513761468,-0.511926606,
-0.510091743,-0.508256881,-0.506422018,-0.504587156,-0.502752294,-0.500917431,
-0.499082569,-0.497247706,-0.495412844,-0.493577982,-0.491743119,-0.489908257,
-0.488073394,-0.486238532,-0.48440367,-0.482568807,-0.480733945,-0.478899083,
-0.47706422,-0.475229358,-0.473394495,-0.471559633,-0.469724771,-0.467889908,
-0.466055046,-0.464220183,-0.462385321,-0.460550459,-0.458715596,-0.456880734,
-0.455045872,-0.453211009,-0.451376147,-0.449541284,-0.447706422,-0.44587156,
-0.444036697,-0.442201835,-0.440366972,-0.43853211,-0.436697248,-0.434862385,
-0.433027523,-0.431192661,-0.429357798,-0.427522936,-0.425688073,-0.423853211,
-0.422018349,-0.420183486,-0.418348624,-0.416513761,-0.414678899,-0.412844037,
-0.411009174,-0.409174312,-0.40733945,-0.405504587,-0.403669725,-0.401834862,
-0.4,-0.398165138,-0.396330275,-0.394495413,-0.39266055,-0.390825688,-0.388990826,
-0.387155963,-0.385321101,-0.383486239,-0.381651376,-0.379816514,-0.377981651,
-0.376146789,-0.374311927,-0.372477064,-0.370642202,-0.368807339,-0.366972477,
-0.365137615,-0.363302752,-0.36146789,-0.359633028,-0.357798165,-0.355963303,
-0.35412844,-0.352293578,-0.350458716,-0.348623853,-0.346788991,-0.344954128,
-0.343119266,-0.341284404,-0.339449541,-0.337614679,-0.335779817,-0.333944954,
-0.332110092,-0.330275229,-0.328440367,-0.326605505,-0.324770642,-0.32293578,
-0.321100917,-0.319266055,-0.317431193,-0.31559633,-0.313761468,-0.311926606,
-0.310091743,-0.308256881,-0.306422018,-0.304587156,-0.302752294,-0.300917431,
-0.299082569,-0.297247706,-0.295412844,-0.293577982,-0.291743119,-0.289908257,
-0.288073394,-0.286238532,-0.28440367,-0.282568807,-0.280733945,-0.278899083,
-0.27706422,-0.275229358,-0.273394495,-0.271559633,-0.269724771,-0.267889908,
-0.266055046,-0.264220183,-0.262385321,-0.260550459,-0.258715596,-0.256880734,
-0.255045872,-0.253211009,-0.251376147,-0.249541284,-0.247706422,-0.24587156,
-0.244036697,-0.242201835,-0.240366972,-0.23853211,-0.236697248,-0.234862385,
-0.233027523,-0.231192661,-0.229357798,-0.227522936,-0.225688073,-0.223853211,
-0.222018349,-0.220183486,-0.218348624,-0.216513761,-0.214678899,-0.212844037,
-0.211009174,-0.209174312,-0.20733945,-0.205504587,-0.203669725,-0.201834862,
-0.2,-0.198165138,-0.196330275,-0.194495413,-0.19266055,-0.190825688,-0.188990826,
-0.187155963,-0.185321101,-0.183486239,-0.181651376,-0.179816514,-0.177981651,
-0.176146789,-0.174311927,-0.172477064,-0.170642202,-0.168807339,-0.166972477,
-0.165137615,-0.163302752,-0.16146789,-0.159633028,-0.157798165,-0.155963303,
-0.15412844,-0.152293578,-0.150458716,-0.148623853,-0.146788991,-0.144954128,
-0.143172103),(0.,0.36),.UNSPECIFIED.);
#6293=B_SPLINE_SURFACE_WITH_KNOTS('',5,1,((#282751,#282752),(#282753,#282754),
(#282755,#282756),(#282757,#282758),(#282759,#282760),(#282761,#282762),
(#282763,#282764),(#282765,#282766),(#282767,#282768),(#282769,#282770),
(#282771,#282772),(#282773,#282774),(#282775,#282776),(#282777,#282778),
(#282779,#282780),(#282781,#282782),(#282783,#282784),(#282785,#282786),
(#282787,#282788),(#282789,#282790),(#282791,#282792),(#282793,#282794),
(#282795,#282796),(#282797,#282798),(#282799,#282800),(#282801,#282802),
(#282803,#282804),(#282805,#282806),(#282807,#282808),(#282809,#282810),
(#282811,#282812),(#282813,#282814),(#282815,#282816),(#282817,#282818),
(#282819,#282820),(#282821,#282822),(#282823,#282824),(#282825,#282826),
(#282827,#282828),(#282829,#282830),(#282831,#282832),(#282833,#282834),
(#282835,#282836),(#282837,#282838),(#282839,#282840),(#282841,#282842),
(#282843,#282844),(#282845,#282846),(#282847,#282848),(#282849,#282850),
(#282851,#282852),(#282853,#282854),(#282855,#282856),(#282857,#282858),
(#282859,#282860),(#282861,#282862),(#282863,#282864),(#282865,#282866),
(#282867,#282868),(#282869,#282870),(#282871,#282872),(#282873,#282874),
(#282875,#282876),(#282877,#282878),(#282879,#282880),(#282881,#282882),
(#282883,#282884),(#282885,#282886),(#282887,#282888),(#282889,#282890),
(#282891,#282892),(#282893,#282894),(#282895,#282896),(#282897,#282898),
(#282899,#282900),(#282901,#282902),(#282903,#282904),(#282905,#282906),
(#282907,#282908),(#282909,#282910),(#282911,#282912),(#282913,#282914),
(#282915,#282916),(#282917,#282918),(#282919,#282920),(#282921,#282922),
(#282923,#282924),(#282925,#282926),(#282927,#282928),(#282929,#282930),
(#282931,#282932),(#282933,#282934),(#282935,#282936),(#282937,#282938),
(#282939,#282940),(#282941,#282942),(#282943,#282944),(#282945,#282946),
(#282947,#282948),(#282949,#282950),(#282951,#282952),(#282953,#282954),
(#282955,#282956),(#282957,#282958),(#282959,#282960),(#282961,#282962),
(#282963,#282964),(#282965,#282966),(#282967,#282968),(#282969,#282970),
(#282971,#282972),(#282973,#282974),(#282975,#282976),(#282977,#282978),
(#282979,#282980),(#282981,#282982),(#282983,#282984),(#282985,#282986),
(#282987,#282988),(#282989,#282990),(#282991,#282992),(#282993,#282994),
(#282995,#282996),(#282997,#282998),(#282999,#283000),(#283001,#283002),
(#283003,#283004),(#283005,#283006),(#283007,#283008),(#283009,#283010),
(#283011,#283012),(#283013,#283014),(#283015,#283016),(#283017,#283018),
(#283019,#283020),(#283021,#283022),(#283023,#283024),(#283025,#283026),
(#283027,#283028),(#283029,#283030),(#283031,#283032),(#283033,#283034),
(#283035,#283036),(#283037,#283038),(#283039,#283040),(#283041,#283042),
(#283043,#283044),(#283045,#283046),(#283047,#283048),(#283049,#283050),
(#283051,#283052),(#283053,#283054),(#283055,#283056),(#283057,#283058),
(#283059,#283060),(#283061,#283062),(#283063,#283064),(#283065,#283066),
(#283067,#283068),(#283069,#283070),(#283071,#283072),(#283073,#283074),
(#283075,#283076),(#283077,#283078),(#283079,#283080),(#283081,#283082),
(#283083,#283084),(#283085,#283086),(#283087,#283088),(#283089,#283090),
(#283091,#283092),(#283093,#283094),(#283095,#283096),(#283097,#283098),
(#283099,#283100),(#283101,#283102),(#283103,#283104),(#283105,#283106),
(#283107,#283108),(#283109,#283110),(#283111,#283112),(#283113,#283114),
(#283115,#283116),(#283117,#283118),(#283119,#283120),(#283121,#283122),
(#283123,#283124),(#283125,#283126),(#283127,#283128),(#283129,#283130),
(#283131,#283132),(#283133,#283134),(#283135,#283136),(#283137,#283138),
(#283139,#283140),(#283141,#283142),(#283143,#283144),(#283145,#283146),
(#283147,#283148),(#283149,#283150),(#283151,#283152),(#283153,#283154),
(#283155,#283156),(#283157,#283158),(#283159,#283160),(#283161,#283162),
(#283163,#283164),(#283165,#283166),(#283167,#283168),(#283169,#283170),
(#283171,#283172),(#283173,#283174),(#283175,#283176),(#283177,#283178),
(#283179,#283180),(#283181,#283182),(#283183,#283184),(#283185,#283186),
(#283187,#283188),(#283189,#283190),(#283191,#283192),(#283193,#283194),
(#283195,#283196),(#283197,#283198),(#283199,#283200),(#283201,#283202),
(#283203,#283204),(#283205,#283206),(#283207,#283208),(#283209,#283210),
(#283211,#283212),(#283213,#283214),(#283215,#283216),(#283217,#283218),
(#283219,#283220),(#283221,#283222),(#283223,#283224),(#283225,#283226),
(#283227,#283228),(#283229,#283230),(#283231,#283232),(#283233,#283234),
(#283235,#283236),(#283237,#283238),(#283239,#283240),(#283241,#283242),
(#283243,#283244),(#283245,#283246),(#283247,#283248),(#283249,#283250),
(#283251,#283252),(#283253,#283254),(#283255,#283256),(#283257,#283258),
(#283259,#283260),(#283261,#283262),(#283263,#283264),(#283265,#283266),
(#283267,#283268),(#283269,#283270),(#283271,#283272),(#283273,#283274),
(#283275,#283276),(#283277,#283278),(#283279,#283280),(#283281,#283282),
(#283283,#283284),(#283285,#283286),(#283287,#283288),(#283289,#283290),
(#283291,#283292),(#283293,#283294),(#283295,#283296),(#283297,#283298),
(#283299,#283300),(#283301,#283302),(#283303,#283304),(#283305,#283306),
(#283307,#283308),(#283309,#283310),(#283311,#283312),(#283313,#283314),
(#283315,#283316),(#283317,#283318),(#283319,#283320),(#283321,#283322),
(#283323,#283324),(#283325,#283326),(#283327,#283328),(#283329,#283330),
(#283331,#283332),(#283333,#283334),(#283335,#283336),(#283337,#283338),
(#283339,#283340),(#283341,#283342),(#283343,#283344),(#283345,#283346),
(#283347,#283348),(#283349,#283350),(#283351,#283352),(#283353,#283354),
(#283355,#283356),(#283357,#283358),(#283359,#283360),(#283361,#283362),
(#283363,#283364),(#283365,#283366),(#283367,#283368),(#283369,#283370),
(#283371,#283372),(#283373,#283374),(#283375,#283376),(#283377,#283378),
(#283379,#283380),(#283381,#283382),(#283383,#283384),(#283385,#283386),
(#283387,#283388),(#283389,#283390),(#283391,#283392),(#283393,#283394),
(#283395,#283396),(#283397,#283398),(#283399,#283400),(#283401,#283402),
(#283403,#283404),(#283405,#283406),(#283407,#283408),(#283409,#283410),
(#283411,#283412),(#283413,#283414),(#283415,#283416),(#283417,#283418),
(#283419,#283420),(#283421,#283422),(#283423,#283424),(#283425,#283426),
(#283427,#283428),(#283429,#283430),(#283431,#283432),(#283433,#283434),
(#283435,#283436),(#283437,#283438),(#283439,#283440),(#283441,#283442),
(#283443,#283444),(#283445,#283446),(#283447,#283448),(#283449,#283450),
(#283451,#283452),(#283453,#283454),(#283455,#283456),(#283457,#283458),
(#283459,#283460),(#283461,#283462),(#283463,#283464),(#283465,#283466),
(#283467,#283468),(#283469,#283470),(#283471,#283472),(#283473,#283474),
(#283475,#283476),(#283477,#283478),(#283479,#283480),(#283481,#283482),
(#283483,#283484),(#283485,#283486),(#283487,#283488),(#283489,#283490),
(#283491,#283492),(#283493,#283494),(#283495,#283496),(#283497,#283498),
(#283499,#283500),(#283501,#283502),(#283503,#283504),(#283505,#283506),
(#283507,#283508),(#283509,#283510),(#283511,#283512),(#283513,#283514),
(#283515,#283516),(#283517,#283518),(#283519,#283520),(#283521,#283522),
(#283523,#283524),(#283525,#283526),(#283527,#283528),(#283529,#283530),
(#283531,#283532),(#283533,#283534),(#283535,#283536),(#283537,#283538),
(#283539,#283540),(#283541,#283542),(#283543,#283544),(#283545,#283546),
(#283547,#283548),(#283549,#283550),(#283551,#283552),(#283553,#283554),
(#283555,#283556),(#283557,#283558),(#283559,#283560),(#283561,#283562),
(#283563,#283564),(#283565,#283566),(#283567,#283568),(#283569,#283570),
(#283571,#283572),(#283573,#283574),(#283575,#283576),(#283577,#283578),
(#283579,#283580),(#283581,#283582),(#283583,#283584),(#283585,#283586),
(#283587,#283588),(#283589,#283590),(#283591,#283592),(#283593,#283594),
(#283595,#283596),(#283597,#283598),(#283599,#283600),(#283601,#283602),
(#283603,#283604),(#283605,#283606),(#283607,#283608),(#283609,#283610),
(#283611,#283612),(#283613,#283614),(#283615,#283616),(#283617,#283618),
(#283619,#283620),(#283621,#283622),(#283623,#283624),(#283625,#283626),
(#283627,#283628),(#283629,#283630),(#283631,#283632),(#283633,#283634),
(#283635,#283636),(#283637,#283638),(#283639,#283640),(#283641,#283642),
(#283643,#283644),(#283645,#283646),(#283647,#283648),(#283649,#283650),
(#283651,#283652),(#283653,#283654),(#283655,#283656),(#283657,#283658),
(#283659,#283660),(#283661,#283662),(#283663,#283664),(#283665,#283666),
(#283667,#283668),(#283669,#283670),(#283671,#283672),(#283673,#283674),
(#283675,#283676),(#283677,#283678),(#283679,#283680),(#283681,#283682),
(#283683,#283684),(#283685,#283686),(#283687,#283688),(#283689,#283690),
(#283691,#283692),(#283693,#283694)),.UNSPECIFIED.,.F.,.F.,.F.,(6,1,1,1,
1,1,1,1,1,1,1,1,1,1,1,1,1,1,1,1,1,1,1,1,1,1,1,1,1,1,1,1,1,1,1,1,1,1,1,1,
1,1,1,1,1,1,1,1,1,1,1,1,1,1,1,1,1,1,1,1,1,1,1,1,1,1,1,1,1,1,1,1,1,1,1,1,
1,1,1,1,1,1,1,1,1,1,1,1,1,1,1,1,1,1,1,1,1,1,1,1,1,1,1,1,1,1,1,1,1,1,1,1,
1,1,1,1,1,1,1,1,1,1,1,1,1,1,1,1,1,1,1,1,1,1,1,1,1,1,1,1,1,1,1,1,1,1,1,1,
1,1,1,1,1,1,1,1,1,1,1,1,1,1,1,1,1,1,1,1,1,1,1,1,1,1,1,1,1,1,1,1,1,1,1,1,
1,1,1,1,1,1,1,1,1,1,1,1,1,1,1,1,1,1,1,1,1,1,1,1,1,1,1,1,1,1,1,1,1,1,1,1,
1,1,1,1,1,1,1,1,1,1,1,1,1,1,1,1,1,1,1,1,1,1,1,1,1,1,1,1,1,1,1,1,1,1,1,1,
1,1,1,1,1,1,1,1,1,1,1,1,1,1,1,1,1,1,1,1,1,1,1,1,1,1,1,1,1,1,1,1,1,1,1,1,
1,1,1,1,1,1,1,1,1,1,1,1,1,1,1,1,1,1,1,1,1,1,1,1,1,1,1,1,1,1,1,1,1,1,1,1,
1,1,1,1,1,1,1,1,1,1,1,1,1,1,1,1,1,1,1,1,1,1,1,1,1,1,1,1,1,1,1,1,1,1,1,1,
1,1,1,1,1,1,1,1,1,1,1,1,1,1,1,1,1,1,1,1,1,1,1,1,1,1,1,1,1,1,1,1,1,1,1,1,
1,1,1,1,1,1,1,1,1,1,1,1,1,1,1,1,1,1,1,1,1,1,1,1,1,1,1,1,1,1,1,1,1,1,1,1,
1,1,1,1,1,1,1,1,1,1,1,1,1,1,1,1,1,1,1,1,1,1,1,1,1,1,1,1,1,1,1,6),(2,2),
(-1.,-0.998165138,-0.996330275,-0.994495413,-0.99266055,-0.990825688,-0.988990826,
-0.987155963,-0.985321101,-0.983486239,-0.981651376,-0.979816514,-0.977981651,
-0.976146789,-0.974311927,-0.972477064,-0.970642202,-0.968807339,-0.966972477,
-0.965137615,-0.963302752,-0.96146789,-0.959633028,-0.957798165,-0.955963303,
-0.95412844,-0.952293578,-0.950458716,-0.948623853,-0.946788991,-0.944954128,
-0.943119266,-0.941284404,-0.939449541,-0.937614679,-0.935779817,-0.933944954,
-0.932110092,-0.930275229,-0.928440367,-0.926605505,-0.924770642,-0.92293578,
-0.921100917,-0.919266055,-0.917431193,-0.91559633,-0.913761468,-0.911926606,
-0.910091743,-0.908256881,-0.906422018,-0.904587156,-0.902752294,-0.900917431,
-0.899082569,-0.897247706,-0.895412844,-0.893577982,-0.891743119,-0.889908257,
-0.888073394,-0.886238532,-0.88440367,-0.882568807,-0.880733945,-0.878899083,
-0.87706422,-0.875229358,-0.873394495,-0.871559633,-0.869724771,-0.867889908,
-0.866055046,-0.864220183,-0.862385321,-0.860550459,-0.858715596,-0.856880734,
-0.855045872,-0.853211009,-0.851376147,-0.849541284,-0.847706422,-0.84587156,
-0.844036697,-0.842201835,-0.840366972,-0.83853211,-0.836697248,-0.834862385,
-0.833027523,-0.831192661,-0.829357798,-0.827522936,-0.825688073,-0.823853211,
-0.822018349,-0.820183486,-0.818348624,-0.816513761,-0.814678899,-0.812844037,
-0.811009174,-0.809174312,-0.80733945,-0.805504587,-0.803669725,-0.801834862,
-0.8,-0.798165138,-0.796330275,-0.794495413,-0.79266055,-0.790825688,-0.788990826,
-0.787155963,-0.785321101,-0.783486239,-0.781651376,-0.779816514,-0.777981651,
-0.776146789,-0.774311927,-0.772477064,-0.770642202,-0.768807339,-0.766972477,
-0.765137615,-0.763302752,-0.76146789,-0.759633028,-0.757798165,-0.755963303,
-0.75412844,-0.752293578,-0.750458716,-0.748623853,-0.746788991,-0.744954128,
-0.743119266,-0.741284404,-0.739449541,-0.737614679,-0.735779817,-0.733944954,
-0.732110092,-0.730275229,-0.728440367,-0.726605505,-0.724770642,-0.72293578,
-0.721100917,-0.719266055,-0.717431193,-0.71559633,-0.713761468,-0.711926606,
-0.710091743,-0.708256881,-0.706422018,-0.704587156,-0.702752294,-0.700917431,
-0.699082569,-0.697247706,-0.695412844,-0.693577982,-0.691743119,-0.689908257,
-0.688073394,-0.686238532,-0.68440367,-0.682568807,-0.680733945,-0.678899083,
-0.67706422,-0.675229358,-0.673394495,-0.671559633,-0.669724771,-0.667889908,
-0.666055046,-0.664220183,-0.662385321,-0.660550459,-0.658715596,-0.656880734,
-0.655045872,-0.653211009,-0.651376147,-0.649541284,-0.647706422,-0.64587156,
-0.644036697,-0.642201835,-0.640366972,-0.63853211,-0.636697248,-0.634862385,
-0.633027523,-0.631192661,-0.629357798,-0.627522936,-0.625688073,-0.623853211,
-0.622018349,-0.620183486,-0.618348624,-0.616513761,-0.614678899,-0.612844037,
-0.611009174,-0.609174312,-0.60733945,-0.605504587,-0.603669725,-0.601834862,
-0.6,-0.598165138,-0.596330275,-0.594495413,-0.59266055,-0.590825688,-0.588990826,
-0.587155963,-0.585321101,-0.583486239,-0.581651376,-0.579816514,-0.577981651,
-0.576146789,-0.574311927,-0.572477064,-0.570642202,-0.568807339,-0.566972477,
-0.565137615,-0.563302752,-0.56146789,-0.559633028,-0.557798165,-0.555963303,
-0.55412844,-0.552293578,-0.550458716,-0.548623853,-0.546788991,-0.544954128,
-0.543119266,-0.541284404,-0.539449541,-0.537614679,-0.535779817,-0.533944954,
-0.532110092,-0.530275229,-0.528440367,-0.526605505,-0.524770642,-0.52293578,
-0.521100917,-0.519266055,-0.517431193,-0.51559633,-0.513761468,-0.511926606,
-0.510091743,-0.508256881,-0.506422018,-0.504587156,-0.502752294,-0.500917431,
-0.499082569,-0.497247706,-0.495412844,-0.493577982,-0.491743119,-0.489908257,
-0.488073394,-0.486238532,-0.48440367,-0.482568807,-0.480733945,-0.478899083,
-0.47706422,-0.475229358,-0.473394495,-0.471559633,-0.469724771,-0.467889908,
-0.466055046,-0.464220183,-0.462385321,-0.460550459,-0.458715596,-0.456880734,
-0.455045872,-0.453211009,-0.451376147,-0.449541284,-0.447706422,-0.44587156,
-0.444036697,-0.442201835,-0.440366972,-0.43853211,-0.436697248,-0.434862385,
-0.433027523,-0.431192661,-0.429357798,-0.427522936,-0.425688073,-0.423853211,
-0.422018349,-0.420183486,-0.418348624,-0.416513761,-0.414678899,-0.412844037,
-0.411009174,-0.409174312,-0.40733945,-0.405504587,-0.403669725,-0.401834862,
-0.4,-0.398165138,-0.396330275,-0.394495413,-0.39266055,-0.390825688,-0.388990826,
-0.387155963,-0.385321101,-0.383486239,-0.381651376,-0.379816514,-0.377981651,
-0.376146789,-0.374311927,-0.372477064,-0.370642202,-0.368807339,-0.366972477,
-0.365137615,-0.363302752,-0.36146789,-0.359633028,-0.357798165,-0.355963303,
-0.35412844,-0.352293578,-0.350458716,-0.348623853,-0.346788991,-0.344954128,
-0.343119266,-0.341284404,-0.339449541,-0.337614679,-0.335779817,-0.333944954,
-0.332110092,-0.330275229,-0.328440367,-0.326605505,-0.324770642,-0.32293578,
-0.321100917,-0.319266055,-0.317431193,-0.31559633,-0.313761468,-0.311926606,
-0.310091743,-0.308256881,-0.306422018,-0.304587156,-0.302752294,-0.300917431,
-0.299082569,-0.297247706,-0.295412844,-0.293577982,-0.291743119,-0.289908257,
-0.288073394,-0.286238532,-0.28440367,-0.282568807,-0.280733945,-0.278899083,
-0.27706422,-0.275229358,-0.273394495,-0.271559633,-0.269724771,-0.267889908,
-0.266055046,-0.264220183,-0.262385321,-0.260550459,-0.258715596,-0.256880734,
-0.255045872,-0.253211009,-0.251376147,-0.249541284,-0.247706422,-0.24587156,
-0.244036697,-0.242201835,-0.240366972,-0.23853211,-0.236697248,-0.234862385,
-0.233027523,-0.231192661,-0.229357798,-0.227522936,-0.225688073,-0.223853211,
-0.222018349,-0.220183486,-0.218348624,-0.216513761,-0.214678899,-0.212844037,
-0.211009174,-0.209174312,-0.20733945,-0.205504587,-0.203669725,-0.201834862,
-0.2,-0.198165138,-0.196330275,-0.194495413,-0.19266055,-0.190825688,-0.188990826,
-0.187155963,-0.185321101,-0.183486239,-0.181651376,-0.179816514,-0.177981651,
-0.176146789,-0.174311927,-0.172477064,-0.170642202,-0.168807339,-0.166972477,
-0.165137615,-0.163302752,-0.16146789,-0.159633028,-0.157798165,-0.155963303,
-0.15412844,-0.152293578,-0.150458716,-0.148623853,-0.146788991,-0.144954128,
-0.143172103),(0.,0.36),.UNSPECIFIED.);
#6294=B_SPLINE_SURFACE_WITH_KNOTS('',5,1,((#284642,#284643),(#284644,#284645),
(#284646,#284647),(#284648,#284649),(#284650,#284651),(#284652,#284653),
(#284654,#284655),(#284656,#284657),(#284658,#284659),(#284660,#284661),
(#284662,#284663),(#284664,#284665),(#284666,#284667),(#284668,#284669),
(#284670,#284671),(#284672,#284673),(#284674,#284675),(#284676,#284677),
(#284678,#284679),(#284680,#284681),(#284682,#284683),(#284684,#284685),
(#284686,#284687),(#284688,#284689),(#284690,#284691),(#284692,#284693),
(#284694,#284695),(#284696,#284697),(#284698,#284699),(#284700,#284701),
(#284702,#284703),(#284704,#284705),(#284706,#284707),(#284708,#284709),
(#284710,#284711),(#284712,#284713),(#284714,#284715),(#284716,#284717),
(#284718,#284719),(#284720,#284721),(#284722,#284723),(#284724,#284725),
(#284726,#284727),(#284728,#284729),(#284730,#284731),(#284732,#284733),
(#284734,#284735),(#284736,#284737),(#284738,#284739),(#284740,#284741),
(#284742,#284743),(#284744,#284745),(#284746,#284747),(#284748,#284749),
(#284750,#284751),(#284752,#284753),(#284754,#284755),(#284756,#284757),
(#284758,#284759),(#284760,#284761),(#284762,#284763),(#284764,#284765),
(#284766,#284767),(#284768,#284769),(#284770,#284771),(#284772,#284773),
(#284774,#284775),(#284776,#284777),(#284778,#284779),(#284780,#284781),
(#284782,#284783),(#284784,#284785),(#284786,#284787),(#284788,#284789),
(#284790,#284791),(#284792,#284793),(#284794,#284795),(#284796,#284797),
(#284798,#284799),(#284800,#284801),(#284802,#284803),(#284804,#284805),
(#284806,#284807),(#284808,#284809),(#284810,#284811),(#284812,#284813),
(#284814,#284815),(#284816,#284817),(#284818,#284819),(#284820,#284821),
(#284822,#284823),(#284824,#284825),(#284826,#284827),(#284828,#284829),
(#284830,#284831),(#284832,#284833),(#284834,#284835),(#284836,#284837),
(#284838,#284839),(#284840,#284841),(#284842,#284843),(#284844,#284845),
(#284846,#284847),(#284848,#284849),(#284850,#284851),(#284852,#284853),
(#284854,#284855),(#284856,#284857),(#284858,#284859),(#284860,#284861),
(#284862,#284863),(#284864,#284865),(#284866,#284867),(#284868,#284869),
(#284870,#284871),(#284872,#284873),(#284874,#284875),(#284876,#284877),
(#284878,#284879),(#284880,#284881),(#284882,#284883),(#284884,#284885),
(#284886,#284887),(#284888,#284889),(#284890,#284891),(#284892,#284893),
(#284894,#284895),(#284896,#284897),(#284898,#284899),(#284900,#284901),
(#284902,#284903),(#284904,#284905),(#284906,#284907),(#284908,#284909),
(#284910,#284911),(#284912,#284913),(#284914,#284915),(#284916,#284917),
(#284918,#284919),(#284920,#284921),(#284922,#284923),(#284924,#284925),
(#284926,#284927),(#284928,#284929),(#284930,#284931),(#284932,#284933),
(#284934,#284935),(#284936,#284937),(#284938,#284939),(#284940,#284941),
(#284942,#284943),(#284944,#284945),(#284946,#284947),(#284948,#284949),
(#284950,#284951),(#284952,#284953),(#284954,#284955),(#284956,#284957),
(#284958,#284959),(#284960,#284961),(#284962,#284963),(#284964,#284965),
(#284966,#284967),(#284968,#284969),(#284970,#284971),(#284972,#284973),
(#284974,#284975),(#284976,#284977),(#284978,#284979),(#284980,#284981),
(#284982,#284983),(#284984,#284985),(#284986,#284987),(#284988,#284989),
(#284990,#284991),(#284992,#284993),(#284994,#284995),(#284996,#284997),
(#284998,#284999),(#285000,#285001),(#285002,#285003),(#285004,#285005),
(#285006,#285007),(#285008,#285009),(#285010,#285011),(#285012,#285013),
(#285014,#285015),(#285016,#285017),(#285018,#285019),(#285020,#285021),
(#285022,#285023),(#285024,#285025),(#285026,#285027),(#285028,#285029),
(#285030,#285031),(#285032,#285033),(#285034,#285035),(#285036,#285037),
(#285038,#285039),(#285040,#285041),(#285042,#285043),(#285044,#285045),
(#285046,#285047),(#285048,#285049),(#285050,#285051),(#285052,#285053),
(#285054,#285055),(#285056,#285057),(#285058,#285059),(#285060,#285061),
(#285062,#285063),(#285064,#285065),(#285066,#285067),(#285068,#285069),
(#285070,#285071),(#285072,#285073),(#285074,#285075),(#285076,#285077),
(#285078,#285079),(#285080,#285081),(#285082,#285083),(#285084,#285085),
(#285086,#285087),(#285088,#285089),(#285090,#285091),(#285092,#285093),
(#285094,#285095),(#285096,#285097),(#285098,#285099),(#285100,#285101),
(#285102,#285103),(#285104,#285105),(#285106,#285107),(#285108,#285109),
(#285110,#285111),(#285112,#285113),(#285114,#285115),(#285116,#285117),
(#285118,#285119),(#285120,#285121),(#285122,#285123),(#285124,#285125),
(#285126,#285127),(#285128,#285129),(#285130,#285131),(#285132,#285133),
(#285134,#285135),(#285136,#285137),(#285138,#285139),(#285140,#285141),
(#285142,#285143),(#285144,#285145),(#285146,#285147),(#285148,#285149),
(#285150,#285151),(#285152,#285153),(#285154,#285155),(#285156,#285157),
(#285158,#285159),(#285160,#285161),(#285162,#285163),(#285164,#285165),
(#285166,#285167),(#285168,#285169),(#285170,#285171),(#285172,#285173),
(#285174,#285175),(#285176,#285177),(#285178,#285179),(#285180,#285181),
(#285182,#285183),(#285184,#285185),(#285186,#285187),(#285188,#285189),
(#285190,#285191),(#285192,#285193),(#285194,#285195),(#285196,#285197),
(#285198,#285199),(#285200,#285201),(#285202,#285203),(#285204,#285205),
(#285206,#285207),(#285208,#285209),(#285210,#285211),(#285212,#285213),
(#285214,#285215),(#285216,#285217),(#285218,#285219),(#285220,#285221),
(#285222,#285223),(#285224,#285225),(#285226,#285227),(#285228,#285229),
(#285230,#285231),(#285232,#285233),(#285234,#285235),(#285236,#285237),
(#285238,#285239),(#285240,#285241),(#285242,#285243),(#285244,#285245),
(#285246,#285247),(#285248,#285249),(#285250,#285251),(#285252,#285253),
(#285254,#285255),(#285256,#285257),(#285258,#285259),(#285260,#285261),
(#285262,#285263),(#285264,#285265),(#285266,#285267),(#285268,#285269),
(#285270,#285271),(#285272,#285273),(#285274,#285275),(#285276,#285277),
(#285278,#285279),(#285280,#285281),(#285282,#285283),(#285284,#285285),
(#285286,#285287),(#285288,#285289),(#285290,#285291),(#285292,#285293),
(#285294,#285295),(#285296,#285297),(#285298,#285299),(#285300,#285301),
(#285302,#285303),(#285304,#285305),(#285306,#285307),(#285308,#285309),
(#285310,#285311),(#285312,#285313),(#285314,#285315),(#285316,#285317),
(#285318,#285319),(#285320,#285321),(#285322,#285323),(#285324,#285325),
(#285326,#285327),(#285328,#285329),(#285330,#285331),(#285332,#285333),
(#285334,#285335),(#285336,#285337),(#285338,#285339),(#285340,#285341),
(#285342,#285343),(#285344,#285345),(#285346,#285347),(#285348,#285349),
(#285350,#285351),(#285352,#285353),(#285354,#285355),(#285356,#285357),
(#285358,#285359),(#285360,#285361),(#285362,#285363),(#285364,#285365),
(#285366,#285367),(#285368,#285369),(#285370,#285371),(#285372,#285373),
(#285374,#285375),(#285376,#285377),(#285378,#285379),(#285380,#285381),
(#285382,#285383),(#285384,#285385),(#285386,#285387),(#285388,#285389),
(#285390,#285391),(#285392,#285393),(#285394,#285395),(#285396,#285397),
(#285398,#285399),(#285400,#285401),(#285402,#285403),(#285404,#285405),
(#285406,#285407),(#285408,#285409),(#285410,#285411),(#285412,#285413),
(#285414,#285415),(#285416,#285417),(#285418,#285419),(#285420,#285421),
(#285422,#285423),(#285424,#285425),(#285426,#285427),(#285428,#285429),
(#285430,#285431),(#285432,#285433),(#285434,#285435),(#285436,#285437),
(#285438,#285439),(#285440,#285441),(#285442,#285443),(#285444,#285445),
(#285446,#285447),(#285448,#285449),(#285450,#285451),(#285452,#285453),
(#285454,#285455),(#285456,#285457),(#285458,#285459),(#285460,#285461),
(#285462,#285463),(#285464,#285465),(#285466,#285467),(#285468,#285469),
(#285470,#285471),(#285472,#285473),(#285474,#285475),(#285476,#285477),
(#285478,#285479),(#285480,#285481),(#285482,#285483),(#285484,#285485),
(#285486,#285487),(#285488,#285489),(#285490,#285491),(#285492,#285493),
(#285494,#285495),(#285496,#285497),(#285498,#285499),(#285500,#285501),
(#285502,#285503),(#285504,#285505),(#285506,#285507),(#285508,#285509),
(#285510,#285511),(#285512,#285513),(#285514,#285515),(#285516,#285517),
(#285518,#285519),(#285520,#285521),(#285522,#285523),(#285524,#285525),
(#285526,#285527),(#285528,#285529),(#285530,#285531),(#285532,#285533),
(#285534,#285535),(#285536,#285537),(#285538,#285539),(#285540,#285541),
(#285542,#285543),(#285544,#285545),(#285546,#285547),(#285548,#285549),
(#285550,#285551),(#285552,#285553),(#285554,#285555),(#285556,#285557),
(#285558,#285559),(#285560,#285561),(#285562,#285563),(#285564,#285565),
(#285566,#285567),(#285568,#285569),(#285570,#285571),(#285572,#285573),
(#285574,#285575),(#285576,#285577),(#285578,#285579),(#285580,#285581),
(#285582,#285583),(#285584,#285585)),.UNSPECIFIED.,.F.,.F.,.F.,(6,1,1,1,
1,1,1,1,1,1,1,1,1,1,1,1,1,1,1,1,1,1,1,1,1,1,1,1,1,1,1,1,1,1,1,1,1,1,1,1,
1,1,1,1,1,1,1,1,1,1,1,1,1,1,1,1,1,1,1,1,1,1,1,1,1,1,1,1,1,1,1,1,1,1,1,1,
1,1,1,1,1,1,1,1,1,1,1,1,1,1,1,1,1,1,1,1,1,1,1,1,1,1,1,1,1,1,1,1,1,1,1,1,
1,1,1,1,1,1,1,1,1,1,1,1,1,1,1,1,1,1,1,1,1,1,1,1,1,1,1,1,1,1,1,1,1,1,1,1,
1,1,1,1,1,1,1,1,1,1,1,1,1,1,1,1,1,1,1,1,1,1,1,1,1,1,1,1,1,1,1,1,1,1,1,1,
1,1,1,1,1,1,1,1,1,1,1,1,1,1,1,1,1,1,1,1,1,1,1,1,1,1,1,1,1,1,1,1,1,1,1,1,
1,1,1,1,1,1,1,1,1,1,1,1,1,1,1,1,1,1,1,1,1,1,1,1,1,1,1,1,1,1,1,1,1,1,1,1,
1,1,1,1,1,1,1,1,1,1,1,1,1,1,1,1,1,1,1,1,1,1,1,1,1,1,1,1,1,1,1,1,1,1,1,1,
1,1,1,1,1,1,1,1,1,1,1,1,1,1,1,1,1,1,1,1,1,1,1,1,1,1,1,1,1,1,1,1,1,1,1,1,
1,1,1,1,1,1,1,1,1,1,1,1,1,1,1,1,1,1,1,1,1,1,1,1,1,1,1,1,1,1,1,1,1,1,1,1,
1,1,1,1,1,1,1,1,1,1,1,1,1,1,1,1,1,1,1,1,1,1,1,1,1,1,1,1,1,1,1,1,1,1,1,1,
1,1,1,1,1,1,1,1,1,1,1,1,1,1,1,1,1,1,1,1,1,1,1,1,1,1,1,1,1,1,1,1,1,1,1,1,
1,1,1,1,1,1,1,1,1,1,1,1,1,1,1,1,1,1,1,1,1,1,1,1,1,1,1,1,1,1,1,6),(2,2),
(0.143172103,0.144954128,0.146788991,0.148623853,0.150458716,0.152293578,
0.15412844,0.155963303,0.157798165,0.159633028,0.16146789,0.163302752,0.165137615,
0.166972477,0.168807339,0.170642202,0.172477064,0.174311927,0.176146789,
0.177981651,0.179816514,0.181651376,0.183486239,0.185321101,0.187155963,
0.188990826,0.190825688,0.19266055,0.194495413,0.196330275,0.198165138,
0.2,0.201834862,0.203669725,0.205504587,0.20733945,0.209174312,0.211009174,
0.212844037,0.214678899,0.216513761,0.218348624,0.220183486,0.222018349,
0.223853211,0.225688073,0.227522936,0.229357798,0.231192661,0.233027523,
0.234862385,0.236697248,0.23853211,0.240366972,0.242201835,0.244036697,
0.24587156,0.247706422,0.249541284,0.251376147,0.253211009,0.255045872,
0.256880734,0.258715596,0.260550459,0.262385321,0.264220183,0.266055046,
0.267889908,0.269724771,0.271559633,0.273394495,0.275229358,0.27706422,
0.278899083,0.280733945,0.282568807,0.28440367,0.286238532,0.288073394,
0.289908257,0.291743119,0.293577982,0.295412844,0.297247706,0.299082569,
0.300917431,0.302752294,0.304587156,0.306422018,0.308256881,0.310091743,
0.311926606,0.313761468,0.31559633,0.317431193,0.319266055,0.321100917,
0.32293578,0.324770642,0.326605505,0.328440367,0.330275229,0.332110092,
0.333944954,0.335779817,0.337614679,0.339449541,0.341284404,0.343119266,
0.344954128,0.346788991,0.348623853,0.350458716,0.352293578,0.35412844,
0.355963303,0.357798165,0.359633028,0.36146789,0.363302752,0.365137615,
0.366972477,0.368807339,0.370642202,0.372477064,0.374311927,0.376146789,
0.377981651,0.379816514,0.381651376,0.383486239,0.385321101,0.387155963,
0.388990826,0.390825688,0.39266055,0.394495413,0.396330275,0.398165138,
0.4,0.401834862,0.403669725,0.405504587,0.40733945,0.409174312,0.411009174,
0.412844037,0.414678899,0.416513761,0.418348624,0.420183486,0.422018349,
0.423853211,0.425688073,0.427522936,0.429357798,0.431192661,0.433027523,
0.434862385,0.436697248,0.43853211,0.440366972,0.442201835,0.444036697,
0.44587156,0.447706422,0.449541284,0.451376147,0.453211009,0.455045872,
0.456880734,0.458715596,0.460550459,0.462385321,0.464220183,0.466055046,
0.467889908,0.469724771,0.471559633,0.473394495,0.475229358,0.47706422,
0.478899083,0.480733945,0.482568807,0.48440367,0.486238532,0.488073394,
0.489908257,0.491743119,0.493577982,0.495412844,0.497247706,0.499082569,
0.500917431,0.502752294,0.504587156,0.506422018,0.508256881,0.510091743,
0.511926606,0.513761468,0.51559633,0.517431193,0.519266055,0.521100917,
0.52293578,0.524770642,0.526605505,0.528440367,0.530275229,0.532110092,
0.533944954,0.535779817,0.537614679,0.539449541,0.541284404,0.543119266,
0.544954128,0.546788991,0.548623853,0.550458716,0.552293578,0.55412844,
0.555963303,0.557798165,0.559633028,0.56146789,0.563302752,0.565137615,
0.566972477,0.568807339,0.570642202,0.572477064,0.574311927,0.576146789,
0.577981651,0.579816514,0.581651376,0.583486239,0.585321101,0.587155963,
0.588990826,0.590825688,0.59266055,0.594495413,0.596330275,0.598165138,
0.6,0.601834862,0.603669725,0.605504587,0.60733945,0.609174312,0.611009174,
0.612844037,0.614678899,0.616513761,0.618348624,0.620183486,0.622018349,
0.623853211,0.625688073,0.627522936,0.629357798,0.631192661,0.633027523,
0.634862385,0.636697248,0.63853211,0.640366972,0.642201835,0.644036697,
0.64587156,0.647706422,0.649541284,0.651376147,0.653211009,0.655045872,
0.656880734,0.658715596,0.660550459,0.662385321,0.664220183,0.666055046,
0.667889908,0.669724771,0.671559633,0.673394495,0.675229358,0.67706422,
0.678899083,0.680733945,0.682568807,0.68440367,0.686238532,0.688073394,
0.689908257,0.691743119,0.693577982,0.695412844,0.697247706,0.699082569,
0.700917431,0.702752294,0.704587156,0.706422018,0.708256881,0.710091743,
0.711926606,0.713761468,0.71559633,0.717431193,0.719266055,0.721100917,
0.72293578,0.724770642,0.726605505,0.728440367,0.730275229,0.732110092,
0.733944954,0.735779817,0.737614679,0.739449541,0.741284404,0.743119266,
0.744954128,0.746788991,0.748623853,0.750458716,0.752293578,0.75412844,
0.755963303,0.757798165,0.759633028,0.76146789,0.763302752,0.765137615,
0.766972477,0.768807339,0.770642202,0.772477064,0.774311927,0.776146789,
0.777981651,0.779816514,0.781651376,0.783486239,0.785321101,0.787155963,
0.788990826,0.790825688,0.79266055,0.794495413,0.796330275,0.798165138,
0.8,0.801834862,0.803669725,0.805504587,0.80733945,0.809174312,0.811009174,
0.812844037,0.814678899,0.816513761,0.818348624,0.820183486,0.822018349,
0.823853211,0.825688073,0.827522936,0.829357798,0.831192661,0.833027523,
0.834862385,0.836697248,0.83853211,0.840366972,0.842201835,0.844036697,
0.84587156,0.847706422,0.849541284,0.851376147,0.853211009,0.855045872,
0.856880734,0.858715596,0.860550459,0.862385321,0.864220183,0.866055046,
0.867889908,0.869724771,0.871559633,0.873394495,0.875229358,0.87706422,
0.878899083,0.880733945,0.882568807,0.88440367,0.886238532,0.888073394,
0.889908257,0.891743119,0.893577982,0.895412844,0.897247706,0.899082569,
0.900917431,0.902752294,0.904587156,0.906422018,0.908256881,0.910091743,
0.911926606,0.913761468,0.91559633,0.917431193,0.919266055,0.921100917,
0.92293578,0.924770642,0.926605505,0.928440367,0.930275229,0.932110092,
0.933944954,0.935779817,0.937614679,0.939449541,0.941284404,0.943119266,
0.944954128,0.946788991,0.948623853,0.950458716,0.952293578,0.95412844,
0.955963303,0.957798165,0.959633028,0.96146789,0.963302752,0.965137615,
0.966972477,0.968807339,0.970642202,0.972477064,0.974311927,0.976146789,
0.977981651,0.979816514,0.981651376,0.983486239,0.985321101,0.987155963,
0.988990826,0.990825688,0.99266055,0.994495413,0.996330275,0.998165138,
1.),(0.,0.36),.UNSPECIFIED.);
#6295=B_SPLINE_SURFACE_WITH_KNOTS('',5,1,((#286545,#286546),(#286547,#286548),
(#286549,#286550),(#286551,#286552),(#286553,#286554),(#286555,#286556),
(#286557,#286558),(#286559,#286560),(#286561,#286562),(#286563,#286564),
(#286565,#286566),(#286567,#286568),(#286569,#286570),(#286571,#286572),
(#286573,#286574),(#286575,#286576),(#286577,#286578),(#286579,#286580),
(#286581,#286582),(#286583,#286584),(#286585,#286586),(#286587,#286588),
(#286589,#286590),(#286591,#286592),(#286593,#286594),(#286595,#286596),
(#286597,#286598),(#286599,#286600),(#286601,#286602),(#286603,#286604),
(#286605,#286606),(#286607,#286608),(#286609,#286610),(#286611,#286612),
(#286613,#286614),(#286615,#286616),(#286617,#286618),(#286619,#286620),
(#286621,#286622),(#286623,#286624),(#286625,#286626),(#286627,#286628),
(#286629,#286630),(#286631,#286632),(#286633,#286634),(#286635,#286636),
(#286637,#286638),(#286639,#286640),(#286641,#286642),(#286643,#286644),
(#286645,#286646),(#286647,#286648),(#286649,#286650),(#286651,#286652),
(#286653,#286654),(#286655,#286656),(#286657,#286658),(#286659,#286660),
(#286661,#286662),(#286663,#286664),(#286665,#286666),(#286667,#286668),
(#286669,#286670),(#286671,#286672),(#286673,#286674),(#286675,#286676),
(#286677,#286678),(#286679,#286680),(#286681,#286682),(#286683,#286684),
(#286685,#286686),(#286687,#286688),(#286689,#286690),(#286691,#286692),
(#286693,#286694),(#286695,#286696),(#286697,#286698),(#286699,#286700),
(#286701,#286702),(#286703,#286704),(#286705,#286706),(#286707,#286708),
(#286709,#286710),(#286711,#286712),(#286713,#286714),(#286715,#286716),
(#286717,#286718),(#286719,#286720),(#286721,#286722),(#286723,#286724),
(#286725,#286726),(#286727,#286728),(#286729,#286730),(#286731,#286732),
(#286733,#286734),(#286735,#286736),(#286737,#286738),(#286739,#286740),
(#286741,#286742),(#286743,#286744),(#286745,#286746),(#286747,#286748),
(#286749,#286750),(#286751,#286752),(#286753,#286754),(#286755,#286756),
(#286757,#286758),(#286759,#286760),(#286761,#286762),(#286763,#286764),
(#286765,#286766),(#286767,#286768),(#286769,#286770),(#286771,#286772),
(#286773,#286774),(#286775,#286776),(#286777,#286778),(#286779,#286780),
(#286781,#286782),(#286783,#286784),(#286785,#286786),(#286787,#286788),
(#286789,#286790),(#286791,#286792),(#286793,#286794),(#286795,#286796),
(#286797,#286798),(#286799,#286800),(#286801,#286802),(#286803,#286804),
(#286805,#286806),(#286807,#286808),(#286809,#286810),(#286811,#286812),
(#286813,#286814),(#286815,#286816),(#286817,#286818),(#286819,#286820),
(#286821,#286822),(#286823,#286824),(#286825,#286826),(#286827,#286828),
(#286829,#286830),(#286831,#286832),(#286833,#286834),(#286835,#286836),
(#286837,#286838),(#286839,#286840),(#286841,#286842),(#286843,#286844),
(#286845,#286846),(#286847,#286848),(#286849,#286850),(#286851,#286852),
(#286853,#286854),(#286855,#286856),(#286857,#286858),(#286859,#286860),
(#286861,#286862),(#286863,#286864),(#286865,#286866),(#286867,#286868),
(#286869,#286870),(#286871,#286872),(#286873,#286874),(#286875,#286876),
(#286877,#286878),(#286879,#286880),(#286881,#286882),(#286883,#286884),
(#286885,#286886),(#286887,#286888),(#286889,#286890),(#286891,#286892),
(#286893,#286894),(#286895,#286896),(#286897,#286898),(#286899,#286900),
(#286901,#286902),(#286903,#286904),(#286905,#286906),(#286907,#286908),
(#286909,#286910),(#286911,#286912),(#286913,#286914),(#286915,#286916),
(#286917,#286918),(#286919,#286920),(#286921,#286922),(#286923,#286924),
(#286925,#286926),(#286927,#286928),(#286929,#286930),(#286931,#286932),
(#286933,#286934),(#286935,#286936),(#286937,#286938),(#286939,#286940),
(#286941,#286942),(#286943,#286944),(#286945,#286946),(#286947,#286948),
(#286949,#286950),(#286951,#286952),(#286953,#286954),(#286955,#286956),
(#286957,#286958),(#286959,#286960),(#286961,#286962),(#286963,#286964),
(#286965,#286966),(#286967,#286968),(#286969,#286970),(#286971,#286972),
(#286973,#286974),(#286975,#286976),(#286977,#286978),(#286979,#286980),
(#286981,#286982),(#286983,#286984),(#286985,#286986),(#286987,#286988),
(#286989,#286990),(#286991,#286992),(#286993,#286994),(#286995,#286996),
(#286997,#286998),(#286999,#287000),(#287001,#287002),(#287003,#287004),
(#287005,#287006),(#287007,#287008),(#287009,#287010),(#287011,#287012),
(#287013,#287014),(#287015,#287016),(#287017,#287018),(#287019,#287020),
(#287021,#287022),(#287023,#287024),(#287025,#287026),(#287027,#287028),
(#287029,#287030),(#287031,#287032),(#287033,#287034),(#287035,#287036),
(#287037,#287038),(#287039,#287040),(#287041,#287042),(#287043,#287044),
(#287045,#287046),(#287047,#287048),(#287049,#287050),(#287051,#287052),
(#287053,#287054),(#287055,#287056),(#287057,#287058),(#287059,#287060),
(#287061,#287062),(#287063,#287064),(#287065,#287066),(#287067,#287068),
(#287069,#287070),(#287071,#287072),(#287073,#287074),(#287075,#287076),
(#287077,#287078),(#287079,#287080),(#287081,#287082),(#287083,#287084),
(#287085,#287086),(#287087,#287088),(#287089,#287090),(#287091,#287092),
(#287093,#287094),(#287095,#287096),(#287097,#287098),(#287099,#287100),
(#287101,#287102),(#287103,#287104),(#287105,#287106),(#287107,#287108),
(#287109,#287110),(#287111,#287112),(#287113,#287114),(#287115,#287116),
(#287117,#287118),(#287119,#287120),(#287121,#287122),(#287123,#287124),
(#287125,#287126),(#287127,#287128),(#287129,#287130),(#287131,#287132),
(#287133,#287134),(#287135,#287136),(#287137,#287138),(#287139,#287140),
(#287141,#287142),(#287143,#287144),(#287145,#287146),(#287147,#287148),
(#287149,#287150),(#287151,#287152),(#287153,#287154),(#287155,#287156),
(#287157,#287158),(#287159,#287160),(#287161,#287162),(#287163,#287164),
(#287165,#287166),(#287167,#287168),(#287169,#287170),(#287171,#287172),
(#287173,#287174),(#287175,#287176),(#287177,#287178),(#287179,#287180),
(#287181,#287182),(#287183,#287184),(#287185,#287186),(#287187,#287188),
(#287189,#287190),(#287191,#287192),(#287193,#287194),(#287195,#287196),
(#287197,#287198),(#287199,#287200),(#287201,#287202),(#287203,#287204),
(#287205,#287206),(#287207,#287208),(#287209,#287210),(#287211,#287212),
(#287213,#287214),(#287215,#287216),(#287217,#287218),(#287219,#287220),
(#287221,#287222),(#287223,#287224),(#287225,#287226),(#287227,#287228),
(#287229,#287230),(#287231,#287232),(#287233,#287234),(#287235,#287236),
(#287237,#287238),(#287239,#287240),(#287241,#287242),(#287243,#287244),
(#287245,#287246),(#287247,#287248),(#287249,#287250),(#287251,#287252),
(#287253,#287254),(#287255,#287256),(#287257,#287258),(#287259,#287260),
(#287261,#287262),(#287263,#287264),(#287265,#287266),(#287267,#287268),
(#287269,#287270),(#287271,#287272),(#287273,#287274),(#287275,#287276),
(#287277,#287278),(#287279,#287280),(#287281,#287282),(#287283,#287284),
(#287285,#287286),(#287287,#287288),(#287289,#287290),(#287291,#287292),
(#287293,#287294),(#287295,#287296),(#287297,#287298),(#287299,#287300),
(#287301,#287302),(#287303,#287304),(#287305,#287306),(#287307,#287308),
(#287309,#287310),(#287311,#287312),(#287313,#287314),(#287315,#287316),
(#287317,#287318),(#287319,#287320),(#287321,#287322),(#287323,#287324),
(#287325,#287326),(#287327,#287328),(#287329,#287330),(#287331,#287332),
(#287333,#287334),(#287335,#287336),(#287337,#287338),(#287339,#287340),
(#287341,#287342),(#287343,#287344),(#287345,#287346),(#287347,#287348),
(#287349,#287350),(#287351,#287352),(#287353,#287354),(#287355,#287356),
(#287357,#287358),(#287359,#287360),(#287361,#287362),(#287363,#287364),
(#287365,#287366),(#287367,#287368),(#287369,#287370),(#287371,#287372),
(#287373,#287374),(#287375,#287376),(#287377,#287378),(#287379,#287380),
(#287381,#287382),(#287383,#287384),(#287385,#287386),(#287387,#287388),
(#287389,#287390),(#287391,#287392),(#287393,#287394),(#287395,#287396),
(#287397,#287398),(#287399,#287400),(#287401,#287402),(#287403,#287404),
(#287405,#287406),(#287407,#287408),(#287409,#287410),(#287411,#287412),
(#287413,#287414),(#287415,#287416),(#287417,#287418),(#287419,#287420),
(#287421,#287422),(#287423,#287424),(#287425,#287426),(#287427,#287428),
(#287429,#287430),(#287431,#287432),(#287433,#287434),(#287435,#287436),
(#287437,#287438),(#287439,#287440),(#287441,#287442),(#287443,#287444),
(#287445,#287446),(#287447,#287448),(#287449,#287450),(#287451,#287452),
(#287453,#287454),(#287455,#287456),(#287457,#287458),(#287459,#287460),
(#287461,#287462),(#287463,#287464),(#287465,#287466),(#287467,#287468),
(#287469,#287470),(#287471,#287472),(#287473,#287474),(#287475,#287476),
(#287477,#287478),(#287479,#287480),(#287481,#287482),(#287483,#287484),
(#287485,#287486),(#287487,#287488)),.UNSPECIFIED.,.F.,.F.,.F.,(6,1,1,1,
1,1,1,1,1,1,1,1,1,1,1,1,1,1,1,1,1,1,1,1,1,1,1,1,1,1,1,1,1,1,1,1,1,1,1,1,
1,1,1,1,1,1,1,1,1,1,1,1,1,1,1,1,1,1,1,1,1,1,1,1,1,1,1,1,1,1,1,1,1,1,1,1,
1,1,1,1,1,1,1,1,1,1,1,1,1,1,1,1,1,1,1,1,1,1,1,1,1,1,1,1,1,1,1,1,1,1,1,1,
1,1,1,1,1,1,1,1,1,1,1,1,1,1,1,1,1,1,1,1,1,1,1,1,1,1,1,1,1,1,1,1,1,1,1,1,
1,1,1,1,1,1,1,1,1,1,1,1,1,1,1,1,1,1,1,1,1,1,1,1,1,1,1,1,1,1,1,1,1,1,1,1,
1,1,1,1,1,1,1,1,1,1,1,1,1,1,1,1,1,1,1,1,1,1,1,1,1,1,1,1,1,1,1,1,1,1,1,1,
1,1,1,1,1,1,1,1,1,1,1,1,1,1,1,1,1,1,1,1,1,1,1,1,1,1,1,1,1,1,1,1,1,1,1,1,
1,1,1,1,1,1,1,1,1,1,1,1,1,1,1,1,1,1,1,1,1,1,1,1,1,1,1,1,1,1,1,1,1,1,1,1,
1,1,1,1,1,1,1,1,1,1,1,1,1,1,1,1,1,1,1,1,1,1,1,1,1,1,1,1,1,1,1,1,1,1,1,1,
1,1,1,1,1,1,1,1,1,1,1,1,1,1,1,1,1,1,1,1,1,1,1,1,1,1,1,1,1,1,1,1,1,1,1,1,
1,1,1,1,1,1,1,1,1,1,1,1,1,1,1,1,1,1,1,1,1,1,1,1,1,1,1,1,1,1,1,1,1,1,1,1,
1,1,1,1,1,1,1,1,1,1,1,1,1,1,1,1,1,1,1,1,1,1,1,1,1,1,1,1,1,1,1,1,1,1,1,1,
1,1,1,1,1,1,1,1,1,1,1,1,1,1,1,1,1,1,1,1,1,1,1,1,1,1,1,1,1,1,1,6),(2,2),
(0.143172104,0.144954128,0.146788991,0.148623853,0.150458716,0.152293578,
0.15412844,0.155963303,0.157798165,0.159633028,0.16146789,0.163302752,0.165137615,
0.166972477,0.168807339,0.170642202,0.172477064,0.174311927,0.176146789,
0.177981651,0.179816514,0.181651376,0.183486239,0.185321101,0.187155963,
0.188990826,0.190825688,0.19266055,0.194495413,0.196330275,0.198165138,
0.2,0.201834862,0.203669725,0.205504587,0.20733945,0.209174312,0.211009174,
0.212844037,0.214678899,0.216513761,0.218348624,0.220183486,0.222018349,
0.223853211,0.225688073,0.227522936,0.229357798,0.231192661,0.233027523,
0.234862385,0.236697248,0.23853211,0.240366972,0.242201835,0.244036697,
0.24587156,0.247706422,0.249541284,0.251376147,0.253211009,0.255045872,
0.256880734,0.258715596,0.260550459,0.262385321,0.264220183,0.266055046,
0.267889908,0.269724771,0.271559633,0.273394495,0.275229358,0.27706422,
0.278899083,0.280733945,0.282568807,0.28440367,0.286238532,0.288073394,
0.289908257,0.291743119,0.293577982,0.295412844,0.297247706,0.299082569,
0.300917431,0.302752294,0.304587156,0.306422018,0.308256881,0.310091743,
0.311926606,0.313761468,0.31559633,0.317431193,0.319266055,0.321100917,
0.32293578,0.324770642,0.326605505,0.328440367,0.330275229,0.332110092,
0.333944954,0.335779817,0.337614679,0.339449541,0.341284404,0.343119266,
0.344954128,0.346788991,0.348623853,0.350458716,0.352293578,0.35412844,
0.355963303,0.357798165,0.359633028,0.36146789,0.363302752,0.365137615,
0.366972477,0.368807339,0.370642202,0.372477064,0.374311927,0.376146789,
0.377981651,0.379816514,0.381651376,0.383486239,0.385321101,0.387155963,
0.388990826,0.390825688,0.39266055,0.394495413,0.396330275,0.398165138,
0.4,0.401834862,0.403669725,0.405504587,0.40733945,0.409174312,0.411009174,
0.412844037,0.414678899,0.416513761,0.418348624,0.420183486,0.422018349,
0.423853211,0.425688073,0.427522936,0.429357798,0.431192661,0.433027523,
0.434862385,0.436697248,0.43853211,0.440366972,0.442201835,0.444036697,
0.44587156,0.447706422,0.449541284,0.451376147,0.453211009,0.455045872,
0.456880734,0.458715596,0.460550459,0.462385321,0.464220183,0.466055046,
0.467889908,0.469724771,0.471559633,0.473394495,0.475229358,0.47706422,
0.478899083,0.480733945,0.482568807,0.48440367,0.486238532,0.488073394,
0.489908257,0.491743119,0.493577982,0.495412844,0.497247706,0.499082569,
0.500917431,0.502752294,0.504587156,0.506422018,0.508256881,0.510091743,
0.511926606,0.513761468,0.51559633,0.517431193,0.519266055,0.521100917,
0.52293578,0.524770642,0.526605505,0.528440367,0.530275229,0.532110092,
0.533944954,0.535779817,0.537614679,0.539449541,0.541284404,0.543119266,
0.544954128,0.546788991,0.548623853,0.550458716,0.552293578,0.55412844,
0.555963303,0.557798165,0.559633028,0.56146789,0.563302752,0.565137615,
0.566972477,0.568807339,0.570642202,0.572477064,0.574311927,0.576146789,
0.577981651,0.579816514,0.581651376,0.583486239,0.585321101,0.587155963,
0.588990826,0.590825688,0.59266055,0.594495413,0.596330275,0.598165138,
0.6,0.601834862,0.603669725,0.605504587,0.60733945,0.609174312,0.611009174,
0.612844037,0.614678899,0.616513761,0.618348624,0.620183486,0.622018349,
0.623853211,0.625688073,0.627522936,0.629357798,0.631192661,0.633027523,
0.634862385,0.636697248,0.63853211,0.640366972,0.642201835,0.644036697,
0.64587156,0.647706422,0.649541284,0.651376147,0.653211009,0.655045872,
0.656880734,0.658715596,0.660550459,0.662385321,0.664220183,0.666055046,
0.667889908,0.669724771,0.671559633,0.673394495,0.675229358,0.67706422,
0.678899083,0.680733945,0.682568807,0.68440367,0.686238532,0.688073394,
0.689908257,0.691743119,0.693577982,0.695412844,0.697247706,0.699082569,
0.700917431,0.702752294,0.704587156,0.706422018,0.708256881,0.710091743,
0.711926606,0.713761468,0.71559633,0.717431193,0.719266055,0.721100917,
0.72293578,0.724770642,0.726605505,0.728440367,0.730275229,0.732110092,
0.733944954,0.735779817,0.737614679,0.739449541,0.741284404,0.743119266,
0.744954128,0.746788991,0.748623853,0.750458716,0.752293578,0.75412844,
0.755963303,0.757798165,0.759633028,0.76146789,0.763302752,0.765137615,
0.766972477,0.768807339,0.770642202,0.772477064,0.774311927,0.776146789,
0.777981651,0.779816514,0.781651376,0.783486239,0.785321101,0.787155963,
0.788990826,0.790825688,0.79266055,0.794495413,0.796330275,0.798165138,
0.8,0.801834862,0.803669725,0.805504587,0.80733945,0.809174312,0.811009174,
0.812844037,0.814678899,0.816513761,0.818348624,0.820183486,0.822018349,
0.823853211,0.825688073,0.827522936,0.829357798,0.831192661,0.833027523,
0.834862385,0.836697248,0.83853211,0.840366972,0.842201835,0.844036697,
0.84587156,0.847706422,0.849541284,0.851376147,0.853211009,0.855045872,
0.856880734,0.858715596,0.860550459,0.862385321,0.864220183,0.866055046,
0.867889908,0.869724771,0.871559633,0.873394495,0.875229358,0.87706422,
0.878899083,0.880733945,0.882568807,0.88440367,0.886238532,0.888073394,
0.889908257,0.891743119,0.893577982,0.895412844,0.897247706,0.899082569,
0.900917431,0.902752294,0.904587156,0.906422018,0.908256881,0.910091743,
0.911926606,0.913761468,0.91559633,0.917431193,0.919266055,0.921100917,
0.92293578,0.924770642,0.926605505,0.928440367,0.930275229,0.932110092,
0.933944954,0.935779817,0.937614679,0.939449541,0.941284404,0.943119266,
0.944954128,0.946788991,0.948623853,0.950458716,0.952293578,0.95412844,
0.955963303,0.957798165,0.959633028,0.96146789,0.963302752,0.965137615,
0.966972477,0.968807339,0.970642202,0.972477064,0.974311927,0.976146789,
0.977981651,0.979816514,0.981651376,0.983486239,0.985321101,0.987155963,
0.988990826,0.990825688,0.99266055,0.994495413,0.996330275,0.998165138,
1.),(0.,0.36),.UNSPECIFIED.);
#6296=B_SPLINE_SURFACE_WITH_KNOTS('',5,1,((#288431,#288432),(#288433,#288434),
(#288435,#288436),(#288437,#288438),(#288439,#288440),(#288441,#288442),
(#288443,#288444),(#288445,#288446),(#288447,#288448),(#288449,#288450),
(#288451,#288452),(#288453,#288454),(#288455,#288456),(#288457,#288458),
(#288459,#288460),(#288461,#288462),(#288463,#288464),(#288465,#288466),
(#288467,#288468),(#288469,#288470),(#288471,#288472),(#288473,#288474),
(#288475,#288476),(#288477,#288478),(#288479,#288480),(#288481,#288482),
(#288483,#288484),(#288485,#288486),(#288487,#288488),(#288489,#288490),
(#288491,#288492),(#288493,#288494),(#288495,#288496),(#288497,#288498),
(#288499,#288500),(#288501,#288502),(#288503,#288504),(#288505,#288506),
(#288507,#288508),(#288509,#288510),(#288511,#288512),(#288513,#288514),
(#288515,#288516),(#288517,#288518),(#288519,#288520),(#288521,#288522),
(#288523,#288524),(#288525,#288526),(#288527,#288528),(#288529,#288530),
(#288531,#288532),(#288533,#288534),(#288535,#288536),(#288537,#288538),
(#288539,#288540),(#288541,#288542),(#288543,#288544),(#288545,#288546),
(#288547,#288548),(#288549,#288550),(#288551,#288552),(#288553,#288554),
(#288555,#288556),(#288557,#288558),(#288559,#288560),(#288561,#288562),
(#288563,#288564),(#288565,#288566),(#288567,#288568),(#288569,#288570),
(#288571,#288572),(#288573,#288574),(#288575,#288576),(#288577,#288578),
(#288579,#288580),(#288581,#288582),(#288583,#288584),(#288585,#288586),
(#288587,#288588),(#288589,#288590),(#288591,#288592),(#288593,#288594),
(#288595,#288596),(#288597,#288598),(#288599,#288600),(#288601,#288602),
(#288603,#288604),(#288605,#288606),(#288607,#288608),(#288609,#288610),
(#288611,#288612),(#288613,#288614),(#288615,#288616),(#288617,#288618),
(#288619,#288620),(#288621,#288622),(#288623,#288624),(#288625,#288626),
(#288627,#288628),(#288629,#288630),(#288631,#288632),(#288633,#288634),
(#288635,#288636),(#288637,#288638),(#288639,#288640),(#288641,#288642),
(#288643,#288644),(#288645,#288646),(#288647,#288648),(#288649,#288650),
(#288651,#288652),(#288653,#288654),(#288655,#288656),(#288657,#288658),
(#288659,#288660),(#288661,#288662),(#288663,#288664),(#288665,#288666),
(#288667,#288668),(#288669,#288670),(#288671,#288672),(#288673,#288674),
(#288675,#288676),(#288677,#288678),(#288679,#288680),(#288681,#288682),
(#288683,#288684),(#288685,#288686),(#288687,#288688),(#288689,#288690),
(#288691,#288692),(#288693,#288694),(#288695,#288696),(#288697,#288698),
(#288699,#288700),(#288701,#288702),(#288703,#288704),(#288705,#288706),
(#288707,#288708),(#288709,#288710),(#288711,#288712),(#288713,#288714),
(#288715,#288716),(#288717,#288718),(#288719,#288720),(#288721,#288722),
(#288723,#288724),(#288725,#288726),(#288727,#288728),(#288729,#288730),
(#288731,#288732),(#288733,#288734),(#288735,#288736),(#288737,#288738),
(#288739,#288740),(#288741,#288742),(#288743,#288744),(#288745,#288746),
(#288747,#288748),(#288749,#288750),(#288751,#288752),(#288753,#288754),
(#288755,#288756),(#288757,#288758),(#288759,#288760),(#288761,#288762),
(#288763,#288764),(#288765,#288766),(#288767,#288768),(#288769,#288770),
(#288771,#288772),(#288773,#288774),(#288775,#288776),(#288777,#288778),
(#288779,#288780),(#288781,#288782),(#288783,#288784),(#288785,#288786),
(#288787,#288788),(#288789,#288790),(#288791,#288792),(#288793,#288794),
(#288795,#288796),(#288797,#288798),(#288799,#288800),(#288801,#288802),
(#288803,#288804),(#288805,#288806),(#288807,#288808),(#288809,#288810),
(#288811,#288812),(#288813,#288814),(#288815,#288816),(#288817,#288818),
(#288819,#288820),(#288821,#288822),(#288823,#288824),(#288825,#288826),
(#288827,#288828),(#288829,#288830),(#288831,#288832),(#288833,#288834),
(#288835,#288836),(#288837,#288838),(#288839,#288840),(#288841,#288842),
(#288843,#288844),(#288845,#288846),(#288847,#288848),(#288849,#288850),
(#288851,#288852),(#288853,#288854),(#288855,#288856),(#288857,#288858),
(#288859,#288860),(#288861,#288862),(#288863,#288864),(#288865,#288866),
(#288867,#288868),(#288869,#288870),(#288871,#288872),(#288873,#288874),
(#288875,#288876),(#288877,#288878),(#288879,#288880),(#288881,#288882),
(#288883,#288884),(#288885,#288886),(#288887,#288888),(#288889,#288890),
(#288891,#288892),(#288893,#288894),(#288895,#288896),(#288897,#288898),
(#288899,#288900),(#288901,#288902),(#288903,#288904),(#288905,#288906),
(#288907,#288908),(#288909,#288910),(#288911,#288912),(#288913,#288914),
(#288915,#288916),(#288917,#288918),(#288919,#288920),(#288921,#288922),
(#288923,#288924),(#288925,#288926),(#288927,#288928),(#288929,#288930),
(#288931,#288932),(#288933,#288934),(#288935,#288936),(#288937,#288938),
(#288939,#288940),(#288941,#288942),(#288943,#288944),(#288945,#288946),
(#288947,#288948),(#288949,#288950),(#288951,#288952),(#288953,#288954),
(#288955,#288956),(#288957,#288958),(#288959,#288960),(#288961,#288962),
(#288963,#288964),(#288965,#288966),(#288967,#288968),(#288969,#288970),
(#288971,#288972),(#288973,#288974),(#288975,#288976),(#288977,#288978),
(#288979,#288980),(#288981,#288982),(#288983,#288984),(#288985,#288986),
(#288987,#288988),(#288989,#288990),(#288991,#288992),(#288993,#288994),
(#288995,#288996),(#288997,#288998),(#288999,#289000),(#289001,#289002),
(#289003,#289004),(#289005,#289006),(#289007,#289008),(#289009,#289010),
(#289011,#289012),(#289013,#289014),(#289015,#289016),(#289017,#289018),
(#289019,#289020),(#289021,#289022),(#289023,#289024),(#289025,#289026),
(#289027,#289028),(#289029,#289030),(#289031,#289032),(#289033,#289034),
(#289035,#289036),(#289037,#289038),(#289039,#289040),(#289041,#289042),
(#289043,#289044),(#289045,#289046),(#289047,#289048),(#289049,#289050),
(#289051,#289052),(#289053,#289054),(#289055,#289056),(#289057,#289058),
(#289059,#289060),(#289061,#289062),(#289063,#289064),(#289065,#289066),
(#289067,#289068),(#289069,#289070),(#289071,#289072),(#289073,#289074),
(#289075,#289076),(#289077,#289078),(#289079,#289080),(#289081,#289082),
(#289083,#289084),(#289085,#289086),(#289087,#289088),(#289089,#289090),
(#289091,#289092),(#289093,#289094),(#289095,#289096),(#289097,#289098),
(#289099,#289100),(#289101,#289102),(#289103,#289104),(#289105,#289106),
(#289107,#289108),(#289109,#289110),(#289111,#289112),(#289113,#289114),
(#289115,#289116),(#289117,#289118),(#289119,#289120),(#289121,#289122),
(#289123,#289124),(#289125,#289126),(#289127,#289128),(#289129,#289130),
(#289131,#289132),(#289133,#289134),(#289135,#289136),(#289137,#289138),
(#289139,#289140),(#289141,#289142),(#289143,#289144),(#289145,#289146),
(#289147,#289148),(#289149,#289150),(#289151,#289152),(#289153,#289154),
(#289155,#289156),(#289157,#289158),(#289159,#289160),(#289161,#289162),
(#289163,#289164),(#289165,#289166),(#289167,#289168),(#289169,#289170),
(#289171,#289172),(#289173,#289174),(#289175,#289176),(#289177,#289178),
(#289179,#289180),(#289181,#289182),(#289183,#289184),(#289185,#289186),
(#289187,#289188),(#289189,#289190),(#289191,#289192),(#289193,#289194),
(#289195,#289196),(#289197,#289198),(#289199,#289200),(#289201,#289202),
(#289203,#289204),(#289205,#289206),(#289207,#289208),(#289209,#289210),
(#289211,#289212),(#289213,#289214),(#289215,#289216),(#289217,#289218),
(#289219,#289220),(#289221,#289222),(#289223,#289224),(#289225,#289226),
(#289227,#289228),(#289229,#289230),(#289231,#289232),(#289233,#289234),
(#289235,#289236),(#289237,#289238),(#289239,#289240),(#289241,#289242),
(#289243,#289244),(#289245,#289246),(#289247,#289248),(#289249,#289250),
(#289251,#289252),(#289253,#289254),(#289255,#289256),(#289257,#289258),
(#289259,#289260),(#289261,#289262),(#289263,#289264),(#289265,#289266),
(#289267,#289268),(#289269,#289270),(#289271,#289272),(#289273,#289274),
(#289275,#289276),(#289277,#289278),(#289279,#289280),(#289281,#289282),
(#289283,#289284),(#289285,#289286),(#289287,#289288),(#289289,#289290),
(#289291,#289292),(#289293,#289294),(#289295,#289296),(#289297,#289298),
(#289299,#289300),(#289301,#289302),(#289303,#289304),(#289305,#289306),
(#289307,#289308),(#289309,#289310),(#289311,#289312),(#289313,#289314),
(#289315,#289316),(#289317,#289318),(#289319,#289320),(#289321,#289322),
(#289323,#289324),(#289325,#289326),(#289327,#289328),(#289329,#289330),
(#289331,#289332),(#289333,#289334),(#289335,#289336),(#289337,#289338),
(#289339,#289340),(#289341,#289342),(#289343,#289344),(#289345,#289346),
(#289347,#289348),(#289349,#289350),(#289351,#289352),(#289353,#289354),
(#289355,#289356),(#289357,#289358),(#289359,#289360),(#289361,#289362),
(#289363,#289364),(#289365,#289366),(#289367,#289368),(#289369,#289370),
(#289371,#289372),(#289373,#289374)),.UNSPECIFIED.,.F.,.F.,.F.,(6,1,1,1,
1,1,1,1,1,1,1,1,1,1,1,1,1,1,1,1,1,1,1,1,1,1,1,1,1,1,1,1,1,1,1,1,1,1,1,1,
1,1,1,1,1,1,1,1,1,1,1,1,1,1,1,1,1,1,1,1,1,1,1,1,1,1,1,1,1,1,1,1,1,1,1,1,
1,1,1,1,1,1,1,1,1,1,1,1,1,1,1,1,1,1,1,1,1,1,1,1,1,1,1,1,1,1,1,1,1,1,1,1,
1,1,1,1,1,1,1,1,1,1,1,1,1,1,1,1,1,1,1,1,1,1,1,1,1,1,1,1,1,1,1,1,1,1,1,1,
1,1,1,1,1,1,1,1,1,1,1,1,1,1,1,1,1,1,1,1,1,1,1,1,1,1,1,1,1,1,1,1,1,1,1,1,
1,1,1,1,1,1,1,1,1,1,1,1,1,1,1,1,1,1,1,1,1,1,1,1,1,1,1,1,1,1,1,1,1,1,1,1,
1,1,1,1,1,1,1,1,1,1,1,1,1,1,1,1,1,1,1,1,1,1,1,1,1,1,1,1,1,1,1,1,1,1,1,1,
1,1,1,1,1,1,1,1,1,1,1,1,1,1,1,1,1,1,1,1,1,1,1,1,1,1,1,1,1,1,1,1,1,1,1,1,
1,1,1,1,1,1,1,1,1,1,1,1,1,1,1,1,1,1,1,1,1,1,1,1,1,1,1,1,1,1,1,1,1,1,1,1,
1,1,1,1,1,1,1,1,1,1,1,1,1,1,1,1,1,1,1,1,1,1,1,1,1,1,1,1,1,1,1,1,1,1,1,1,
1,1,1,1,1,1,1,1,1,1,1,1,1,1,1,1,1,1,1,1,1,1,1,1,1,1,1,1,1,1,1,1,1,1,1,1,
1,1,1,1,1,1,1,1,1,1,1,1,1,1,1,1,1,1,1,1,1,1,1,1,1,1,1,1,1,1,1,1,1,1,1,1,
1,1,1,1,1,1,1,1,1,1,1,1,1,1,1,1,1,1,1,1,1,1,1,1,1,1,1,1,1,1,1,6),(2,2),
(-1.,-0.998165138,-0.996330275,-0.994495413,-0.99266055,-0.990825688,-0.988990826,
-0.987155963,-0.985321101,-0.983486239,-0.981651376,-0.979816514,-0.977981651,
-0.976146789,-0.974311927,-0.972477064,-0.970642202,-0.968807339,-0.966972477,
-0.965137615,-0.963302752,-0.96146789,-0.959633028,-0.957798165,-0.955963303,
-0.95412844,-0.952293578,-0.950458716,-0.948623853,-0.946788991,-0.944954128,
-0.943119266,-0.941284404,-0.939449541,-0.937614679,-0.935779817,-0.933944954,
-0.932110092,-0.930275229,-0.928440367,-0.926605505,-0.924770642,-0.92293578,
-0.921100917,-0.919266055,-0.917431193,-0.91559633,-0.913761468,-0.911926606,
-0.910091743,-0.908256881,-0.906422018,-0.904587156,-0.902752294,-0.900917431,
-0.899082569,-0.897247706,-0.895412844,-0.893577982,-0.891743119,-0.889908257,
-0.888073394,-0.886238532,-0.88440367,-0.882568807,-0.880733945,-0.878899083,
-0.87706422,-0.875229358,-0.873394495,-0.871559633,-0.869724771,-0.867889908,
-0.866055046,-0.864220183,-0.862385321,-0.860550459,-0.858715596,-0.856880734,
-0.855045872,-0.853211009,-0.851376147,-0.849541284,-0.847706422,-0.84587156,
-0.844036697,-0.842201835,-0.840366972,-0.83853211,-0.836697248,-0.834862385,
-0.833027523,-0.831192661,-0.829357798,-0.827522936,-0.825688073,-0.823853211,
-0.822018349,-0.820183486,-0.818348624,-0.816513761,-0.814678899,-0.812844037,
-0.811009174,-0.809174312,-0.80733945,-0.805504587,-0.803669725,-0.801834862,
-0.8,-0.798165138,-0.796330275,-0.794495413,-0.79266055,-0.790825688,-0.788990826,
-0.787155963,-0.785321101,-0.783486239,-0.781651376,-0.779816514,-0.777981651,
-0.776146789,-0.774311927,-0.772477064,-0.770642202,-0.768807339,-0.766972477,
-0.765137615,-0.763302752,-0.76146789,-0.759633028,-0.757798165,-0.755963303,
-0.75412844,-0.752293578,-0.750458716,-0.748623853,-0.746788991,-0.744954128,
-0.743119266,-0.741284404,-0.739449541,-0.737614679,-0.735779817,-0.733944954,
-0.732110092,-0.730275229,-0.728440367,-0.726605505,-0.724770642,-0.72293578,
-0.721100917,-0.719266055,-0.717431193,-0.71559633,-0.713761468,-0.711926606,
-0.710091743,-0.708256881,-0.706422018,-0.704587156,-0.702752294,-0.700917431,
-0.699082569,-0.697247706,-0.695412844,-0.693577982,-0.691743119,-0.689908257,
-0.688073394,-0.686238532,-0.68440367,-0.682568807,-0.680733945,-0.678899083,
-0.67706422,-0.675229358,-0.673394495,-0.671559633,-0.669724771,-0.667889908,
-0.666055046,-0.664220183,-0.662385321,-0.660550459,-0.658715596,-0.656880734,
-0.655045872,-0.653211009,-0.651376147,-0.649541284,-0.647706422,-0.64587156,
-0.644036697,-0.642201835,-0.640366972,-0.63853211,-0.636697248,-0.634862385,
-0.633027523,-0.631192661,-0.629357798,-0.627522936,-0.625688073,-0.623853211,
-0.622018349,-0.620183486,-0.618348624,-0.616513761,-0.614678899,-0.612844037,
-0.611009174,-0.609174312,-0.60733945,-0.605504587,-0.603669725,-0.601834862,
-0.6,-0.598165138,-0.596330275,-0.594495413,-0.59266055,-0.590825688,-0.588990826,
-0.587155963,-0.585321101,-0.583486239,-0.581651376,-0.579816514,-0.577981651,
-0.576146789,-0.574311927,-0.572477064,-0.570642202,-0.568807339,-0.566972477,
-0.565137615,-0.563302752,-0.56146789,-0.559633028,-0.557798165,-0.555963303,
-0.55412844,-0.552293578,-0.550458716,-0.548623853,-0.546788991,-0.544954128,
-0.543119266,-0.541284404,-0.539449541,-0.537614679,-0.535779817,-0.533944954,
-0.532110092,-0.530275229,-0.528440367,-0.526605505,-0.524770642,-0.52293578,
-0.521100917,-0.519266055,-0.517431193,-0.51559633,-0.513761468,-0.511926606,
-0.510091743,-0.508256881,-0.506422018,-0.504587156,-0.502752294,-0.500917431,
-0.499082569,-0.497247706,-0.495412844,-0.493577982,-0.491743119,-0.489908257,
-0.488073394,-0.486238532,-0.48440367,-0.482568807,-0.480733945,-0.478899083,
-0.47706422,-0.475229358,-0.473394495,-0.471559633,-0.469724771,-0.467889908,
-0.466055046,-0.464220183,-0.462385321,-0.460550459,-0.458715596,-0.456880734,
-0.455045872,-0.453211009,-0.451376147,-0.449541284,-0.447706422,-0.44587156,
-0.444036697,-0.442201835,-0.440366972,-0.43853211,-0.436697248,-0.434862385,
-0.433027523,-0.431192661,-0.429357798,-0.427522936,-0.425688073,-0.423853211,
-0.422018349,-0.420183486,-0.418348624,-0.416513761,-0.414678899,-0.412844037,
-0.411009174,-0.409174312,-0.40733945,-0.405504587,-0.403669725,-0.401834862,
-0.4,-0.398165138,-0.396330275,-0.394495413,-0.39266055,-0.390825688,-0.388990826,
-0.387155963,-0.385321101,-0.383486239,-0.381651376,-0.379816514,-0.377981651,
-0.376146789,-0.374311927,-0.372477064,-0.370642202,-0.368807339,-0.366972477,
-0.365137615,-0.363302752,-0.36146789,-0.359633028,-0.357798165,-0.355963303,
-0.35412844,-0.352293578,-0.350458716,-0.348623853,-0.346788991,-0.344954128,
-0.343119266,-0.341284404,-0.339449541,-0.337614679,-0.335779817,-0.333944954,
-0.332110092,-0.330275229,-0.328440367,-0.326605505,-0.324770642,-0.32293578,
-0.321100917,-0.319266055,-0.317431193,-0.31559633,-0.313761468,-0.311926606,
-0.310091743,-0.308256881,-0.306422018,-0.304587156,-0.302752294,-0.300917431,
-0.299082569,-0.297247706,-0.295412844,-0.293577982,-0.291743119,-0.289908257,
-0.288073394,-0.286238532,-0.28440367,-0.282568807,-0.280733945,-0.278899083,
-0.27706422,-0.275229358,-0.273394495,-0.271559633,-0.269724771,-0.267889908,
-0.266055046,-0.264220183,-0.262385321,-0.260550459,-0.258715596,-0.256880734,
-0.255045872,-0.253211009,-0.251376147,-0.249541284,-0.247706422,-0.24587156,
-0.244036697,-0.242201835,-0.240366972,-0.23853211,-0.236697248,-0.234862385,
-0.233027523,-0.231192661,-0.229357798,-0.227522936,-0.225688073,-0.223853211,
-0.222018349,-0.220183486,-0.218348624,-0.216513761,-0.214678899,-0.212844037,
-0.211009174,-0.209174312,-0.20733945,-0.205504587,-0.203669725,-0.201834862,
-0.2,-0.198165138,-0.196330275,-0.194495413,-0.19266055,-0.190825688,-0.188990826,
-0.187155963,-0.185321101,-0.183486239,-0.181651376,-0.179816514,-0.177981651,
-0.176146789,-0.174311927,-0.172477064,-0.170642202,-0.168807339,-0.166972477,
-0.165137615,-0.163302752,-0.16146789,-0.159633028,-0.157798165,-0.155963303,
-0.15412844,-0.152293578,-0.150458716,-0.148623853,-0.146788991,-0.144954128,
-0.143172103),(0.,0.36),.UNSPECIFIED.);
#6297=B_SPLINE_SURFACE_WITH_KNOTS('',5,1,((#290040,#290041),(#290042,#290043),
(#290044,#290045),(#290046,#290047),(#290048,#290049),(#290050,#290051),
(#290052,#290053),(#290054,#290055),(#290056,#290057),(#290058,#290059),
(#290060,#290061),(#290062,#290063),(#290064,#290065),(#290066,#290067),
(#290068,#290069),(#290070,#290071),(#290072,#290073),(#290074,#290075),
(#290076,#290077),(#290078,#290079),(#290080,#290081),(#290082,#290083),
(#290084,#290085),(#290086,#290087),(#290088,#290089),(#290090,#290091),
(#290092,#290093),(#290094,#290095),(#290096,#290097),(#290098,#290099),
(#290100,#290101),(#290102,#290103),(#290104,#290105),(#290106,#290107),
(#290108,#290109),(#290110,#290111),(#290112,#290113),(#290114,#290115),
(#290116,#290117),(#290118,#290119),(#290120,#290121),(#290122,#290123),
(#290124,#290125),(#290126,#290127),(#290128,#290129),(#290130,#290131),
(#290132,#290133),(#290134,#290135),(#290136,#290137),(#290138,#290139),
(#290140,#290141),(#290142,#290143),(#290144,#290145),(#290146,#290147),
(#290148,#290149),(#290150,#290151),(#290152,#290153),(#290154,#290155),
(#290156,#290157),(#290158,#290159),(#290160,#290161),(#290162,#290163),
(#290164,#290165),(#290166,#290167),(#290168,#290169),(#290170,#290171),
(#290172,#290173),(#290174,#290175),(#290176,#290177),(#290178,#290179),
(#290180,#290181),(#290182,#290183),(#290184,#290185),(#290186,#290187),
(#290188,#290189),(#290190,#290191),(#290192,#290193),(#290194,#290195),
(#290196,#290197),(#290198,#290199),(#290200,#290201),(#290202,#290203),
(#290204,#290205),(#290206,#290207),(#290208,#290209),(#290210,#290211),
(#290212,#290213),(#290214,#290215),(#290216,#290217),(#290218,#290219),
(#290220,#290221),(#290222,#290223),(#290224,#290225),(#290226,#290227),
(#290228,#290229),(#290230,#290231),(#290232,#290233),(#290234,#290235),
(#290236,#290237),(#290238,#290239),(#290240,#290241),(#290242,#290243),
(#290244,#290245),(#290246,#290247),(#290248,#290249),(#290250,#290251),
(#290252,#290253),(#290254,#290255),(#290256,#290257),(#290258,#290259),
(#290260,#290261),(#290262,#290263),(#290264,#290265),(#290266,#290267),
(#290268,#290269),(#290270,#290271),(#290272,#290273),(#290274,#290275),
(#290276,#290277),(#290278,#290279),(#290280,#290281),(#290282,#290283),
(#290284,#290285),(#290286,#290287),(#290288,#290289),(#290290,#290291),
(#290292,#290293),(#290294,#290295),(#290296,#290297),(#290298,#290299),
(#290300,#290301),(#290302,#290303),(#290304,#290305),(#290306,#290307),
(#290308,#290309),(#290310,#290311),(#290312,#290313),(#290314,#290315),
(#290316,#290317),(#290318,#290319),(#290320,#290321),(#290322,#290323),
(#290324,#290325),(#290326,#290327),(#290328,#290329),(#290330,#290331),
(#290332,#290333),(#290334,#290335),(#290336,#290337),(#290338,#290339),
(#290340,#290341),(#290342,#290343),(#290344,#290345),(#290346,#290347),
(#290348,#290349),(#290350,#290351),(#290352,#290353),(#290354,#290355),
(#290356,#290357),(#290358,#290359),(#290360,#290361),(#290362,#290363),
(#290364,#290365),(#290366,#290367),(#290368,#290369),(#290370,#290371),
(#290372,#290373),(#290374,#290375),(#290376,#290377),(#290378,#290379),
(#290380,#290381),(#290382,#290383),(#290384,#290385),(#290386,#290387),
(#290388,#290389),(#290390,#290391),(#290392,#290393),(#290394,#290395),
(#290396,#290397),(#290398,#290399),(#290400,#290401),(#290402,#290403),
(#290404,#290405),(#290406,#290407),(#290408,#290409),(#290410,#290411),
(#290412,#290413),(#290414,#290415),(#290416,#290417),(#290418,#290419),
(#290420,#290421),(#290422,#290423),(#290424,#290425),(#290426,#290427),
(#290428,#290429),(#290430,#290431),(#290432,#290433),(#290434,#290435),
(#290436,#290437),(#290438,#290439),(#290440,#290441),(#290442,#290443),
(#290444,#290445),(#290446,#290447),(#290448,#290449),(#290450,#290451),
(#290452,#290453),(#290454,#290455),(#290456,#290457),(#290458,#290459),
(#290460,#290461),(#290462,#290463),(#290464,#290465),(#290466,#290467),
(#290468,#290469),(#290470,#290471),(#290472,#290473),(#290474,#290475),
(#290476,#290477),(#290478,#290479),(#290480,#290481),(#290482,#290483),
(#290484,#290485),(#290486,#290487),(#290488,#290489),(#290490,#290491),
(#290492,#290493),(#290494,#290495),(#290496,#290497),(#290498,#290499),
(#290500,#290501),(#290502,#290503),(#290504,#290505),(#290506,#290507),
(#290508,#290509),(#290510,#290511),(#290512,#290513),(#290514,#290515),
(#290516,#290517),(#290518,#290519),(#290520,#290521),(#290522,#290523),
(#290524,#290525),(#290526,#290527),(#290528,#290529),(#290530,#290531),
(#290532,#290533),(#290534,#290535),(#290536,#290537),(#290538,#290539),
(#290540,#290541),(#290542,#290543),(#290544,#290545),(#290546,#290547),
(#290548,#290549),(#290550,#290551),(#290552,#290553),(#290554,#290555),
(#290556,#290557),(#290558,#290559),(#290560,#290561),(#290562,#290563),
(#290564,#290565),(#290566,#290567),(#290568,#290569),(#290570,#290571),
(#290572,#290573),(#290574,#290575),(#290576,#290577),(#290578,#290579),
(#290580,#290581),(#290582,#290583),(#290584,#290585),(#290586,#290587),
(#290588,#290589),(#290590,#290591),(#290592,#290593),(#290594,#290595),
(#290596,#290597),(#290598,#290599),(#290600,#290601),(#290602,#290603),
(#290604,#290605),(#290606,#290607),(#290608,#290609),(#290610,#290611),
(#290612,#290613),(#290614,#290615),(#290616,#290617),(#290618,#290619),
(#290620,#290621),(#290622,#290623),(#290624,#290625),(#290626,#290627),
(#290628,#290629),(#290630,#290631),(#290632,#290633),(#290634,#290635),
(#290636,#290637),(#290638,#290639),(#290640,#290641),(#290642,#290643),
(#290644,#290645),(#290646,#290647),(#290648,#290649),(#290650,#290651),
(#290652,#290653),(#290654,#290655),(#290656,#290657),(#290658,#290659),
(#290660,#290661),(#290662,#290663),(#290664,#290665),(#290666,#290667),
(#290668,#290669),(#290670,#290671),(#290672,#290673),(#290674,#290675),
(#290676,#290677),(#290678,#290679),(#290680,#290681),(#290682,#290683),
(#290684,#290685),(#290686,#290687),(#290688,#290689),(#290690,#290691),
(#290692,#290693),(#290694,#290695),(#290696,#290697),(#290698,#290699),
(#290700,#290701),(#290702,#290703),(#290704,#290705),(#290706,#290707),
(#290708,#290709),(#290710,#290711),(#290712,#290713),(#290714,#290715),
(#290716,#290717),(#290718,#290719),(#290720,#290721),(#290722,#290723),
(#290724,#290725),(#290726,#290727),(#290728,#290729),(#290730,#290731),
(#290732,#290733),(#290734,#290735),(#290736,#290737),(#290738,#290739),
(#290740,#290741),(#290742,#290743),(#290744,#290745),(#290746,#290747),
(#290748,#290749),(#290750,#290751),(#290752,#290753),(#290754,#290755),
(#290756,#290757),(#290758,#290759),(#290760,#290761),(#290762,#290763),
(#290764,#290765),(#290766,#290767),(#290768,#290769),(#290770,#290771),
(#290772,#290773),(#290774,#290775),(#290776,#290777),(#290778,#290779),
(#290780,#290781),(#290782,#290783),(#290784,#290785),(#290786,#290787),
(#290788,#290789),(#290790,#290791),(#290792,#290793),(#290794,#290795),
(#290796,#290797),(#290798,#290799),(#290800,#290801),(#290802,#290803),
(#290804,#290805),(#290806,#290807),(#290808,#290809),(#290810,#290811),
(#290812,#290813),(#290814,#290815),(#290816,#290817),(#290818,#290819),
(#290820,#290821),(#290822,#290823),(#290824,#290825),(#290826,#290827),
(#290828,#290829),(#290830,#290831),(#290832,#290833),(#290834,#290835),
(#290836,#290837),(#290838,#290839),(#290840,#290841),(#290842,#290843),
(#290844,#290845),(#290846,#290847),(#290848,#290849),(#290850,#290851),
(#290852,#290853),(#290854,#290855),(#290856,#290857),(#290858,#290859),
(#290860,#290861),(#290862,#290863),(#290864,#290865),(#290866,#290867),
(#290868,#290869),(#290870,#290871),(#290872,#290873),(#290874,#290875),
(#290876,#290877),(#290878,#290879),(#290880,#290881),(#290882,#290883),
(#290884,#290885),(#290886,#290887),(#290888,#290889),(#290890,#290891),
(#290892,#290893),(#290894,#290895),(#290896,#290897),(#290898,#290899),
(#290900,#290901),(#290902,#290903),(#290904,#290905),(#290906,#290907),
(#290908,#290909),(#290910,#290911),(#290912,#290913),(#290914,#290915),
(#290916,#290917),(#290918,#290919),(#290920,#290921),(#290922,#290923),
(#290924,#290925),(#290926,#290927),(#290928,#290929),(#290930,#290931),
(#290932,#290933),(#290934,#290935),(#290936,#290937),(#290938,#290939),
(#290940,#290941),(#290942,#290943),(#290944,#290945),(#290946,#290947),
(#290948,#290949),(#290950,#290951),(#290952,#290953),(#290954,#290955),
(#290956,#290957),(#290958,#290959),(#290960,#290961),(#290962,#290963),
(#290964,#290965),(#290966,#290967),(#290968,#290969),(#290970,#290971),
(#290972,#290973),(#290974,#290975),(#290976,#290977),(#290978,#290979),
(#290980,#290981),(#290982,#290983)),.UNSPECIFIED.,.F.,.F.,.F.,(6,1,1,1,
1,1,1,1,1,1,1,1,1,1,1,1,1,1,1,1,1,1,1,1,1,1,1,1,1,1,1,1,1,1,1,1,1,1,1,1,
1,1,1,1,1,1,1,1,1,1,1,1,1,1,1,1,1,1,1,1,1,1,1,1,1,1,1,1,1,1,1,1,1,1,1,1,
1,1,1,1,1,1,1,1,1,1,1,1,1,1,1,1,1,1,1,1,1,1,1,1,1,1,1,1,1,1,1,1,1,1,1,1,
1,1,1,1,1,1,1,1,1,1,1,1,1,1,1,1,1,1,1,1,1,1,1,1,1,1,1,1,1,1,1,1,1,1,1,1,
1,1,1,1,1,1,1,1,1,1,1,1,1,1,1,1,1,1,1,1,1,1,1,1,1,1,1,1,1,1,1,1,1,1,1,1,
1,1,1,1,1,1,1,1,1,1,1,1,1,1,1,1,1,1,1,1,1,1,1,1,1,1,1,1,1,1,1,1,1,1,1,1,
1,1,1,1,1,1,1,1,1,1,1,1,1,1,1,1,1,1,1,1,1,1,1,1,1,1,1,1,1,1,1,1,1,1,1,1,
1,1,1,1,1,1,1,1,1,1,1,1,1,1,1,1,1,1,1,1,1,1,1,1,1,1,1,1,1,1,1,1,1,1,1,1,
1,1,1,1,1,1,1,1,1,1,1,1,1,1,1,1,1,1,1,1,1,1,1,1,1,1,1,1,1,1,1,1,1,1,1,1,
1,1,1,1,1,1,1,1,1,1,1,1,1,1,1,1,1,1,1,1,1,1,1,1,1,1,1,1,1,1,1,1,1,1,1,1,
1,1,1,1,1,1,1,1,1,1,1,1,1,1,1,1,1,1,1,1,1,1,1,1,1,1,1,1,1,1,1,1,1,1,1,1,
1,1,1,1,1,1,1,1,1,1,1,1,1,1,1,1,1,1,1,1,1,1,1,1,1,1,1,1,1,1,1,1,1,1,1,1,
1,1,1,1,1,1,1,1,1,1,1,1,1,1,1,1,1,1,1,1,1,1,1,1,1,1,1,1,1,1,1,6),(2,2),
(-1.,-0.998165138,-0.996330275,-0.994495413,-0.99266055,-0.990825688,-0.988990826,
-0.987155963,-0.985321101,-0.983486239,-0.981651376,-0.979816514,-0.977981651,
-0.976146789,-0.974311927,-0.972477064,-0.970642202,-0.968807339,-0.966972477,
-0.965137615,-0.963302752,-0.96146789,-0.959633028,-0.957798165,-0.955963303,
-0.95412844,-0.952293578,-0.950458716,-0.948623853,-0.946788991,-0.944954128,
-0.943119266,-0.941284404,-0.939449541,-0.937614679,-0.935779817,-0.933944954,
-0.932110092,-0.930275229,-0.928440367,-0.926605505,-0.924770642,-0.92293578,
-0.921100917,-0.919266055,-0.917431193,-0.91559633,-0.913761468,-0.911926606,
-0.910091743,-0.908256881,-0.906422018,-0.904587156,-0.902752294,-0.900917431,
-0.899082569,-0.897247706,-0.895412844,-0.893577982,-0.891743119,-0.889908257,
-0.888073394,-0.886238532,-0.88440367,-0.882568807,-0.880733945,-0.878899083,
-0.87706422,-0.875229358,-0.873394495,-0.871559633,-0.869724771,-0.867889908,
-0.866055046,-0.864220183,-0.862385321,-0.860550459,-0.858715596,-0.856880734,
-0.855045872,-0.853211009,-0.851376147,-0.849541284,-0.847706422,-0.84587156,
-0.844036697,-0.842201835,-0.840366972,-0.83853211,-0.836697248,-0.834862385,
-0.833027523,-0.831192661,-0.829357798,-0.827522936,-0.825688073,-0.823853211,
-0.822018349,-0.820183486,-0.818348624,-0.816513761,-0.814678899,-0.812844037,
-0.811009174,-0.809174312,-0.80733945,-0.805504587,-0.803669725,-0.801834862,
-0.8,-0.798165138,-0.796330275,-0.794495413,-0.79266055,-0.790825688,-0.788990826,
-0.787155963,-0.785321101,-0.783486239,-0.781651376,-0.779816514,-0.777981651,
-0.776146789,-0.774311927,-0.772477064,-0.770642202,-0.768807339,-0.766972477,
-0.765137615,-0.763302752,-0.76146789,-0.759633028,-0.757798165,-0.755963303,
-0.75412844,-0.752293578,-0.750458716,-0.748623853,-0.746788991,-0.744954128,
-0.743119266,-0.741284404,-0.739449541,-0.737614679,-0.735779817,-0.733944954,
-0.732110092,-0.730275229,-0.728440367,-0.726605505,-0.724770642,-0.72293578,
-0.721100917,-0.719266055,-0.717431193,-0.71559633,-0.713761468,-0.711926606,
-0.710091743,-0.708256881,-0.706422018,-0.704587156,-0.702752294,-0.700917431,
-0.699082569,-0.697247706,-0.695412844,-0.693577982,-0.691743119,-0.689908257,
-0.688073394,-0.686238532,-0.68440367,-0.682568807,-0.680733945,-0.678899083,
-0.67706422,-0.675229358,-0.673394495,-0.671559633,-0.669724771,-0.667889908,
-0.666055046,-0.664220183,-0.662385321,-0.660550459,-0.658715596,-0.656880734,
-0.655045872,-0.653211009,-0.651376147,-0.649541284,-0.647706422,-0.64587156,
-0.644036697,-0.642201835,-0.640366972,-0.63853211,-0.636697248,-0.634862385,
-0.633027523,-0.631192661,-0.629357798,-0.627522936,-0.625688073,-0.623853211,
-0.622018349,-0.620183486,-0.618348624,-0.616513761,-0.614678899,-0.612844037,
-0.611009174,-0.609174312,-0.60733945,-0.605504587,-0.603669725,-0.601834862,
-0.6,-0.598165138,-0.596330275,-0.594495413,-0.59266055,-0.590825688,-0.588990826,
-0.587155963,-0.585321101,-0.583486239,-0.581651376,-0.579816514,-0.577981651,
-0.576146789,-0.574311927,-0.572477064,-0.570642202,-0.568807339,-0.566972477,
-0.565137615,-0.563302752,-0.56146789,-0.559633028,-0.557798165,-0.555963303,
-0.55412844,-0.552293578,-0.550458716,-0.548623853,-0.546788991,-0.544954128,
-0.543119266,-0.541284404,-0.539449541,-0.537614679,-0.535779817,-0.533944954,
-0.532110092,-0.530275229,-0.528440367,-0.526605505,-0.524770642,-0.52293578,
-0.521100917,-0.519266055,-0.517431193,-0.51559633,-0.513761468,-0.511926606,
-0.510091743,-0.508256881,-0.506422018,-0.504587156,-0.502752294,-0.500917431,
-0.499082569,-0.497247706,-0.495412844,-0.493577982,-0.491743119,-0.489908257,
-0.488073394,-0.486238532,-0.48440367,-0.482568807,-0.480733945,-0.478899083,
-0.47706422,-0.475229358,-0.473394495,-0.471559633,-0.469724771,-0.467889908,
-0.466055046,-0.464220183,-0.462385321,-0.460550459,-0.458715596,-0.456880734,
-0.455045872,-0.453211009,-0.451376147,-0.449541284,-0.447706422,-0.44587156,
-0.444036697,-0.442201835,-0.440366972,-0.43853211,-0.436697248,-0.434862385,
-0.433027523,-0.431192661,-0.429357798,-0.427522936,-0.425688073,-0.423853211,
-0.422018349,-0.420183486,-0.418348624,-0.416513761,-0.414678899,-0.412844037,
-0.411009174,-0.409174312,-0.40733945,-0.405504587,-0.403669725,-0.401834862,
-0.4,-0.398165138,-0.396330275,-0.394495413,-0.39266055,-0.390825688,-0.388990826,
-0.387155963,-0.385321101,-0.383486239,-0.381651376,-0.379816514,-0.377981651,
-0.376146789,-0.374311927,-0.372477064,-0.370642202,-0.368807339,-0.366972477,
-0.365137615,-0.363302752,-0.36146789,-0.359633028,-0.357798165,-0.355963303,
-0.35412844,-0.352293578,-0.350458716,-0.348623853,-0.346788991,-0.344954128,
-0.343119266,-0.341284404,-0.339449541,-0.337614679,-0.335779817,-0.333944954,
-0.332110092,-0.330275229,-0.328440367,-0.326605505,-0.324770642,-0.32293578,
-0.321100917,-0.319266055,-0.317431193,-0.31559633,-0.313761468,-0.311926606,
-0.310091743,-0.308256881,-0.306422018,-0.304587156,-0.302752294,-0.300917431,
-0.299082569,-0.297247706,-0.295412844,-0.293577982,-0.291743119,-0.289908257,
-0.288073394,-0.286238532,-0.28440367,-0.282568807,-0.280733945,-0.278899083,
-0.27706422,-0.275229358,-0.273394495,-0.271559633,-0.269724771,-0.267889908,
-0.266055046,-0.264220183,-0.262385321,-0.260550459,-0.258715596,-0.256880734,
-0.255045872,-0.253211009,-0.251376147,-0.249541284,-0.247706422,-0.24587156,
-0.244036697,-0.242201835,-0.240366972,-0.23853211,-0.236697248,-0.234862385,
-0.233027523,-0.231192661,-0.229357798,-0.227522936,-0.225688073,-0.223853211,
-0.222018349,-0.220183486,-0.218348624,-0.216513761,-0.214678899,-0.212844037,
-0.211009174,-0.209174312,-0.20733945,-0.205504587,-0.203669725,-0.201834862,
-0.2,-0.198165138,-0.196330275,-0.194495413,-0.19266055,-0.190825688,-0.188990826,
-0.187155963,-0.185321101,-0.183486239,-0.181651376,-0.179816514,-0.177981651,
-0.176146789,-0.174311927,-0.172477064,-0.170642202,-0.168807339,-0.166972477,
-0.165137615,-0.163302752,-0.16146789,-0.159633028,-0.157798165,-0.155963303,
-0.15412844,-0.152293578,-0.150458716,-0.148623853,-0.146788991,-0.144954128,
-0.143172103),(0.,0.36),.UNSPECIFIED.);
#6298=B_SPLINE_SURFACE_WITH_KNOTS('',5,1,((#291634,#291635),(#291636,#291637),
(#291638,#291639),(#291640,#291641),(#291642,#291643),(#291644,#291645),
(#291646,#291647),(#291648,#291649),(#291650,#291651),(#291652,#291653),
(#291654,#291655),(#291656,#291657),(#291658,#291659),(#291660,#291661),
(#291662,#291663),(#291664,#291665),(#291666,#291667),(#291668,#291669),
(#291670,#291671),(#291672,#291673),(#291674,#291675),(#291676,#291677),
(#291678,#291679),(#291680,#291681),(#291682,#291683),(#291684,#291685),
(#291686,#291687),(#291688,#291689),(#291690,#291691),(#291692,#291693),
(#291694,#291695),(#291696,#291697),(#291698,#291699),(#291700,#291701),
(#291702,#291703),(#291704,#291705),(#291706,#291707),(#291708,#291709),
(#291710,#291711),(#291712,#291713),(#291714,#291715),(#291716,#291717),
(#291718,#291719),(#291720,#291721),(#291722,#291723),(#291724,#291725),
(#291726,#291727),(#291728,#291729),(#291730,#291731),(#291732,#291733),
(#291734,#291735),(#291736,#291737),(#291738,#291739),(#291740,#291741),
(#291742,#291743),(#291744,#291745),(#291746,#291747),(#291748,#291749),
(#291750,#291751),(#291752,#291753),(#291754,#291755),(#291756,#291757),
(#291758,#291759),(#291760,#291761),(#291762,#291763),(#291764,#291765),
(#291766,#291767),(#291768,#291769),(#291770,#291771),(#291772,#291773),
(#291774,#291775),(#291776,#291777),(#291778,#291779),(#291780,#291781),
(#291782,#291783),(#291784,#291785),(#291786,#291787),(#291788,#291789),
(#291790,#291791),(#291792,#291793),(#291794,#291795),(#291796,#291797),
(#291798,#291799),(#291800,#291801),(#291802,#291803),(#291804,#291805),
(#291806,#291807),(#291808,#291809),(#291810,#291811),(#291812,#291813),
(#291814,#291815),(#291816,#291817),(#291818,#291819),(#291820,#291821),
(#291822,#291823),(#291824,#291825),(#291826,#291827),(#291828,#291829),
(#291830,#291831),(#291832,#291833),(#291834,#291835),(#291836,#291837),
(#291838,#291839),(#291840,#291841),(#291842,#291843),(#291844,#291845),
(#291846,#291847),(#291848,#291849),(#291850,#291851),(#291852,#291853),
(#291854,#291855),(#291856,#291857),(#291858,#291859),(#291860,#291861),
(#291862,#291863),(#291864,#291865),(#291866,#291867),(#291868,#291869),
(#291870,#291871),(#291872,#291873),(#291874,#291875),(#291876,#291877),
(#291878,#291879),(#291880,#291881),(#291882,#291883),(#291884,#291885),
(#291886,#291887),(#291888,#291889),(#291890,#291891),(#291892,#291893),
(#291894,#291895),(#291896,#291897),(#291898,#291899),(#291900,#291901),
(#291902,#291903),(#291904,#291905),(#291906,#291907),(#291908,#291909),
(#291910,#291911),(#291912,#291913),(#291914,#291915),(#291916,#291917),
(#291918,#291919),(#291920,#291921),(#291922,#291923),(#291924,#291925),
(#291926,#291927),(#291928,#291929),(#291930,#291931),(#291932,#291933),
(#291934,#291935),(#291936,#291937),(#291938,#291939),(#291940,#291941),
(#291942,#291943),(#291944,#291945),(#291946,#291947),(#291948,#291949),
(#291950,#291951),(#291952,#291953),(#291954,#291955),(#291956,#291957),
(#291958,#291959),(#291960,#291961),(#291962,#291963),(#291964,#291965),
(#291966,#291967),(#291968,#291969),(#291970,#291971),(#291972,#291973),
(#291974,#291975),(#291976,#291977),(#291978,#291979),(#291980,#291981),
(#291982,#291983),(#291984,#291985),(#291986,#291987),(#291988,#291989),
(#291990,#291991),(#291992,#291993),(#291994,#291995),(#291996,#291997),
(#291998,#291999),(#292000,#292001),(#292002,#292003),(#292004,#292005),
(#292006,#292007),(#292008,#292009),(#292010,#292011),(#292012,#292013),
(#292014,#292015),(#292016,#292017),(#292018,#292019),(#292020,#292021),
(#292022,#292023),(#292024,#292025),(#292026,#292027),(#292028,#292029),
(#292030,#292031),(#292032,#292033),(#292034,#292035),(#292036,#292037),
(#292038,#292039),(#292040,#292041),(#292042,#292043),(#292044,#292045),
(#292046,#292047),(#292048,#292049),(#292050,#292051),(#292052,#292053),
(#292054,#292055),(#292056,#292057),(#292058,#292059),(#292060,#292061),
(#292062,#292063),(#292064,#292065),(#292066,#292067),(#292068,#292069),
(#292070,#292071),(#292072,#292073),(#292074,#292075),(#292076,#292077),
(#292078,#292079),(#292080,#292081),(#292082,#292083),(#292084,#292085),
(#292086,#292087),(#292088,#292089),(#292090,#292091),(#292092,#292093),
(#292094,#292095),(#292096,#292097),(#292098,#292099),(#292100,#292101),
(#292102,#292103),(#292104,#292105),(#292106,#292107),(#292108,#292109),
(#292110,#292111),(#292112,#292113),(#292114,#292115),(#292116,#292117),
(#292118,#292119),(#292120,#292121),(#292122,#292123),(#292124,#292125),
(#292126,#292127),(#292128,#292129),(#292130,#292131),(#292132,#292133),
(#292134,#292135),(#292136,#292137),(#292138,#292139),(#292140,#292141),
(#292142,#292143),(#292144,#292145),(#292146,#292147),(#292148,#292149),
(#292150,#292151),(#292152,#292153),(#292154,#292155),(#292156,#292157),
(#292158,#292159),(#292160,#292161),(#292162,#292163),(#292164,#292165),
(#292166,#292167),(#292168,#292169),(#292170,#292171),(#292172,#292173),
(#292174,#292175),(#292176,#292177),(#292178,#292179),(#292180,#292181),
(#292182,#292183),(#292184,#292185),(#292186,#292187),(#292188,#292189),
(#292190,#292191),(#292192,#292193),(#292194,#292195),(#292196,#292197),
(#292198,#292199),(#292200,#292201),(#292202,#292203),(#292204,#292205),
(#292206,#292207),(#292208,#292209),(#292210,#292211),(#292212,#292213),
(#292214,#292215),(#292216,#292217),(#292218,#292219),(#292220,#292221),
(#292222,#292223),(#292224,#292225),(#292226,#292227),(#292228,#292229),
(#292230,#292231),(#292232,#292233),(#292234,#292235),(#292236,#292237),
(#292238,#292239),(#292240,#292241),(#292242,#292243),(#292244,#292245),
(#292246,#292247),(#292248,#292249),(#292250,#292251),(#292252,#292253),
(#292254,#292255),(#292256,#292257),(#292258,#292259),(#292260,#292261),
(#292262,#292263),(#292264,#292265),(#292266,#292267),(#292268,#292269),
(#292270,#292271),(#292272,#292273),(#292274,#292275),(#292276,#292277),
(#292278,#292279),(#292280,#292281),(#292282,#292283),(#292284,#292285),
(#292286,#292287),(#292288,#292289),(#292290,#292291),(#292292,#292293),
(#292294,#292295),(#292296,#292297),(#292298,#292299),(#292300,#292301),
(#292302,#292303),(#292304,#292305),(#292306,#292307),(#292308,#292309),
(#292310,#292311),(#292312,#292313),(#292314,#292315),(#292316,#292317),
(#292318,#292319),(#292320,#292321),(#292322,#292323),(#292324,#292325),
(#292326,#292327),(#292328,#292329),(#292330,#292331),(#292332,#292333),
(#292334,#292335),(#292336,#292337),(#292338,#292339),(#292340,#292341),
(#292342,#292343),(#292344,#292345),(#292346,#292347),(#292348,#292349),
(#292350,#292351),(#292352,#292353),(#292354,#292355),(#292356,#292357),
(#292358,#292359),(#292360,#292361),(#292362,#292363),(#292364,#292365),
(#292366,#292367),(#292368,#292369),(#292370,#292371),(#292372,#292373),
(#292374,#292375),(#292376,#292377),(#292378,#292379),(#292380,#292381),
(#292382,#292383),(#292384,#292385),(#292386,#292387),(#292388,#292389),
(#292390,#292391),(#292392,#292393),(#292394,#292395),(#292396,#292397),
(#292398,#292399),(#292400,#292401),(#292402,#292403),(#292404,#292405),
(#292406,#292407),(#292408,#292409),(#292410,#292411),(#292412,#292413),
(#292414,#292415),(#292416,#292417),(#292418,#292419),(#292420,#292421),
(#292422,#292423),(#292424,#292425),(#292426,#292427),(#292428,#292429),
(#292430,#292431),(#292432,#292433),(#292434,#292435),(#292436,#292437),
(#292438,#292439),(#292440,#292441),(#292442,#292443),(#292444,#292445),
(#292446,#292447),(#292448,#292449),(#292450,#292451),(#292452,#292453),
(#292454,#292455),(#292456,#292457),(#292458,#292459),(#292460,#292461),
(#292462,#292463),(#292464,#292465),(#292466,#292467),(#292468,#292469),
(#292470,#292471),(#292472,#292473),(#292474,#292475),(#292476,#292477),
(#292478,#292479),(#292480,#292481),(#292482,#292483),(#292484,#292485),
(#292486,#292487),(#292488,#292489),(#292490,#292491),(#292492,#292493),
(#292494,#292495),(#292496,#292497),(#292498,#292499),(#292500,#292501),
(#292502,#292503),(#292504,#292505),(#292506,#292507),(#292508,#292509),
(#292510,#292511),(#292512,#292513),(#292514,#292515),(#292516,#292517),
(#292518,#292519),(#292520,#292521),(#292522,#292523),(#292524,#292525),
(#292526,#292527),(#292528,#292529),(#292530,#292531),(#292532,#292533),
(#292534,#292535),(#292536,#292537),(#292538,#292539),(#292540,#292541),
(#292542,#292543),(#292544,#292545),(#292546,#292547),(#292548,#292549),
(#292550,#292551),(#292552,#292553),(#292554,#292555),(#292556,#292557),
(#292558,#292559),(#292560,#292561),(#292562,#292563),(#292564,#292565),
(#292566,#292567),(#292568,#292569),(#292570,#292571),(#292572,#292573),
(#292574,#292575),(#292576,#292577)),.UNSPECIFIED.,.F.,.F.,.F.,(6,1,1,1,
1,1,1,1,1,1,1,1,1,1,1,1,1,1,1,1,1,1,1,1,1,1,1,1,1,1,1,1,1,1,1,1,1,1,1,1,
1,1,1,1,1,1,1,1,1,1,1,1,1,1,1,1,1,1,1,1,1,1,1,1,1,1,1,1,1,1,1,1,1,1,1,1,
1,1,1,1,1,1,1,1,1,1,1,1,1,1,1,1,1,1,1,1,1,1,1,1,1,1,1,1,1,1,1,1,1,1,1,1,
1,1,1,1,1,1,1,1,1,1,1,1,1,1,1,1,1,1,1,1,1,1,1,1,1,1,1,1,1,1,1,1,1,1,1,1,
1,1,1,1,1,1,1,1,1,1,1,1,1,1,1,1,1,1,1,1,1,1,1,1,1,1,1,1,1,1,1,1,1,1,1,1,
1,1,1,1,1,1,1,1,1,1,1,1,1,1,1,1,1,1,1,1,1,1,1,1,1,1,1,1,1,1,1,1,1,1,1,1,
1,1,1,1,1,1,1,1,1,1,1,1,1,1,1,1,1,1,1,1,1,1,1,1,1,1,1,1,1,1,1,1,1,1,1,1,
1,1,1,1,1,1,1,1,1,1,1,1,1,1,1,1,1,1,1,1,1,1,1,1,1,1,1,1,1,1,1,1,1,1,1,1,
1,1,1,1,1,1,1,1,1,1,1,1,1,1,1,1,1,1,1,1,1,1,1,1,1,1,1,1,1,1,1,1,1,1,1,1,
1,1,1,1,1,1,1,1,1,1,1,1,1,1,1,1,1,1,1,1,1,1,1,1,1,1,1,1,1,1,1,1,1,1,1,1,
1,1,1,1,1,1,1,1,1,1,1,1,1,1,1,1,1,1,1,1,1,1,1,1,1,1,1,1,1,1,1,1,1,1,1,1,
1,1,1,1,1,1,1,1,1,1,1,1,1,1,1,1,1,1,1,1,1,1,1,1,1,1,1,1,1,1,1,1,1,1,1,1,
1,1,1,1,1,1,1,1,1,1,1,1,1,1,1,1,1,1,1,1,1,1,1,1,1,1,1,1,1,1,1,6),(2,2),
(0.143172103,0.144954128,0.146788991,0.148623853,0.150458716,0.152293578,
0.15412844,0.155963303,0.157798165,0.159633028,0.16146789,0.163302752,0.165137615,
0.166972477,0.168807339,0.170642202,0.172477064,0.174311927,0.176146789,
0.177981651,0.179816514,0.181651376,0.183486239,0.185321101,0.187155963,
0.188990826,0.190825688,0.19266055,0.194495413,0.196330275,0.198165138,
0.2,0.201834862,0.203669725,0.205504587,0.20733945,0.209174312,0.211009174,
0.212844037,0.214678899,0.216513761,0.218348624,0.220183486,0.222018349,
0.223853211,0.225688073,0.227522936,0.229357798,0.231192661,0.233027523,
0.234862385,0.236697248,0.23853211,0.240366972,0.242201835,0.244036697,
0.24587156,0.247706422,0.249541284,0.251376147,0.253211009,0.255045872,
0.256880734,0.258715596,0.260550459,0.262385321,0.264220183,0.266055046,
0.267889908,0.269724771,0.271559633,0.273394495,0.275229358,0.27706422,
0.278899083,0.280733945,0.282568807,0.28440367,0.286238532,0.288073394,
0.289908257,0.291743119,0.293577982,0.295412844,0.297247706,0.299082569,
0.300917431,0.302752294,0.304587156,0.306422018,0.308256881,0.310091743,
0.311926606,0.313761468,0.31559633,0.317431193,0.319266055,0.321100917,
0.32293578,0.324770642,0.326605505,0.328440367,0.330275229,0.332110092,
0.333944954,0.335779817,0.337614679,0.339449541,0.341284404,0.343119266,
0.344954128,0.346788991,0.348623853,0.350458716,0.352293578,0.35412844,
0.355963303,0.357798165,0.359633028,0.36146789,0.363302752,0.365137615,
0.366972477,0.368807339,0.370642202,0.372477064,0.374311927,0.376146789,
0.377981651,0.379816514,0.381651376,0.383486239,0.385321101,0.387155963,
0.388990826,0.390825688,0.39266055,0.394495413,0.396330275,0.398165138,
0.4,0.401834862,0.403669725,0.405504587,0.40733945,0.409174312,0.411009174,
0.412844037,0.414678899,0.416513761,0.418348624,0.420183486,0.422018349,
0.423853211,0.425688073,0.427522936,0.429357798,0.431192661,0.433027523,
0.434862385,0.436697248,0.43853211,0.440366972,0.442201835,0.444036697,
0.44587156,0.447706422,0.449541284,0.451376147,0.453211009,0.455045872,
0.456880734,0.458715596,0.460550459,0.462385321,0.464220183,0.466055046,
0.467889908,0.469724771,0.471559633,0.473394495,0.475229358,0.47706422,
0.478899083,0.480733945,0.482568807,0.48440367,0.486238532,0.488073394,
0.489908257,0.491743119,0.493577982,0.495412844,0.497247706,0.499082569,
0.500917431,0.502752294,0.504587156,0.506422018,0.508256881,0.510091743,
0.511926606,0.513761468,0.51559633,0.517431193,0.519266055,0.521100917,
0.52293578,0.524770642,0.526605505,0.528440367,0.530275229,0.532110092,
0.533944954,0.535779817,0.537614679,0.539449541,0.541284404,0.543119266,
0.544954128,0.546788991,0.548623853,0.550458716,0.552293578,0.55412844,
0.555963303,0.557798165,0.559633028,0.56146789,0.563302752,0.565137615,
0.566972477,0.568807339,0.570642202,0.572477064,0.574311927,0.576146789,
0.577981651,0.579816514,0.581651376,0.583486239,0.585321101,0.587155963,
0.588990826,0.590825688,0.59266055,0.594495413,0.596330275,0.598165138,
0.6,0.601834862,0.603669725,0.605504587,0.60733945,0.609174312,0.611009174,
0.612844037,0.614678899,0.616513761,0.618348624,0.620183486,0.622018349,
0.623853211,0.625688073,0.627522936,0.629357798,0.631192661,0.633027523,
0.634862385,0.636697248,0.63853211,0.640366972,0.642201835,0.644036697,
0.64587156,0.647706422,0.649541284,0.651376147,0.653211009,0.655045872,
0.656880734,0.658715596,0.660550459,0.662385321,0.664220183,0.666055046,
0.667889908,0.669724771,0.671559633,0.673394495,0.675229358,0.67706422,
0.678899083,0.680733945,0.682568807,0.68440367,0.686238532,0.688073394,
0.689908257,0.691743119,0.693577982,0.695412844,0.697247706,0.699082569,
0.700917431,0.702752294,0.704587156,0.706422018,0.708256881,0.710091743,
0.711926606,0.713761468,0.71559633,0.717431193,0.719266055,0.721100917,
0.72293578,0.724770642,0.726605505,0.728440367,0.730275229,0.732110092,
0.733944954,0.735779817,0.737614679,0.739449541,0.741284404,0.743119266,
0.744954128,0.746788991,0.748623853,0.750458716,0.752293578,0.75412844,
0.755963303,0.757798165,0.759633028,0.76146789,0.763302752,0.765137615,
0.766972477,0.768807339,0.770642202,0.772477064,0.774311927,0.776146789,
0.777981651,0.779816514,0.781651376,0.783486239,0.785321101,0.787155963,
0.788990826,0.790825688,0.79266055,0.794495413,0.796330275,0.798165138,
0.8,0.801834862,0.803669725,0.805504587,0.80733945,0.809174312,0.811009174,
0.812844037,0.814678899,0.816513761,0.818348624,0.820183486,0.822018349,
0.823853211,0.825688073,0.827522936,0.829357798,0.831192661,0.833027523,
0.834862385,0.836697248,0.83853211,0.840366972,0.842201835,0.844036697,
0.84587156,0.847706422,0.849541284,0.851376147,0.853211009,0.855045872,
0.856880734,0.858715596,0.860550459,0.862385321,0.864220183,0.866055046,
0.867889908,0.869724771,0.871559633,0.873394495,0.875229358,0.87706422,
0.878899083,0.880733945,0.882568807,0.88440367,0.886238532,0.888073394,
0.889908257,0.891743119,0.893577982,0.895412844,0.897247706,0.899082569,
0.900917431,0.902752294,0.904587156,0.906422018,0.908256881,0.910091743,
0.911926606,0.913761468,0.91559633,0.917431193,0.919266055,0.921100917,
0.92293578,0.924770642,0.926605505,0.928440367,0.930275229,0.932110092,
0.933944954,0.935779817,0.937614679,0.939449541,0.941284404,0.943119266,
0.944954128,0.946788991,0.948623853,0.950458716,0.952293578,0.95412844,
0.955963303,0.957798165,0.959633028,0.96146789,0.963302752,0.965137615,
0.966972477,0.968807339,0.970642202,0.972477064,0.974311927,0.976146789,
0.977981651,0.979816514,0.981651376,0.983486239,0.985321101,0.987155963,
0.988990826,0.990825688,0.99266055,0.994495413,0.996330275,0.998165138,
1.),(0.,0.36),.UNSPECIFIED.);
#6299=B_SPLINE_SURFACE_WITH_KNOTS('',5,1,((#293228,#293229),(#293230,#293231),
(#293232,#293233),(#293234,#293235),(#293236,#293237),(#293238,#293239),
(#293240,#293241),(#293242,#293243),(#293244,#293245),(#293246,#293247),
(#293248,#293249),(#293250,#293251),(#293252,#293253),(#293254,#293255),
(#293256,#293257),(#293258,#293259),(#293260,#293261),(#293262,#293263),
(#293264,#293265),(#293266,#293267),(#293268,#293269),(#293270,#293271),
(#293272,#293273),(#293274,#293275),(#293276,#293277),(#293278,#293279),
(#293280,#293281),(#293282,#293283),(#293284,#293285),(#293286,#293287),
(#293288,#293289),(#293290,#293291),(#293292,#293293),(#293294,#293295),
(#293296,#293297),(#293298,#293299),(#293300,#293301),(#293302,#293303),
(#293304,#293305),(#293306,#293307),(#293308,#293309),(#293310,#293311),
(#293312,#293313),(#293314,#293315),(#293316,#293317),(#293318,#293319),
(#293320,#293321),(#293322,#293323),(#293324,#293325),(#293326,#293327),
(#293328,#293329),(#293330,#293331),(#293332,#293333),(#293334,#293335),
(#293336,#293337),(#293338,#293339),(#293340,#293341),(#293342,#293343),
(#293344,#293345),(#293346,#293347),(#293348,#293349),(#293350,#293351),
(#293352,#293353),(#293354,#293355),(#293356,#293357),(#293358,#293359),
(#293360,#293361),(#293362,#293363),(#293364,#293365),(#293366,#293367),
(#293368,#293369),(#293370,#293371),(#293372,#293373),(#293374,#293375),
(#293376,#293377),(#293378,#293379),(#293380,#293381),(#293382,#293383),
(#293384,#293385),(#293386,#293387),(#293388,#293389),(#293390,#293391),
(#293392,#293393),(#293394,#293395),(#293396,#293397),(#293398,#293399),
(#293400,#293401),(#293402,#293403),(#293404,#293405),(#293406,#293407),
(#293408,#293409),(#293410,#293411),(#293412,#293413),(#293414,#293415),
(#293416,#293417),(#293418,#293419),(#293420,#293421),(#293422,#293423),
(#293424,#293425),(#293426,#293427),(#293428,#293429),(#293430,#293431),
(#293432,#293433),(#293434,#293435),(#293436,#293437),(#293438,#293439),
(#293440,#293441),(#293442,#293443),(#293444,#293445),(#293446,#293447),
(#293448,#293449),(#293450,#293451),(#293452,#293453),(#293454,#293455),
(#293456,#293457),(#293458,#293459),(#293460,#293461),(#293462,#293463),
(#293464,#293465),(#293466,#293467),(#293468,#293469),(#293470,#293471),
(#293472,#293473),(#293474,#293475),(#293476,#293477),(#293478,#293479),
(#293480,#293481),(#293482,#293483),(#293484,#293485),(#293486,#293487),
(#293488,#293489),(#293490,#293491),(#293492,#293493),(#293494,#293495),
(#293496,#293497),(#293498,#293499),(#293500,#293501),(#293502,#293503),
(#293504,#293505),(#293506,#293507),(#293508,#293509),(#293510,#293511),
(#293512,#293513),(#293514,#293515),(#293516,#293517),(#293518,#293519),
(#293520,#293521),(#293522,#293523),(#293524,#293525),(#293526,#293527),
(#293528,#293529),(#293530,#293531),(#293532,#293533),(#293534,#293535),
(#293536,#293537),(#293538,#293539),(#293540,#293541),(#293542,#293543),
(#293544,#293545),(#293546,#293547),(#293548,#293549),(#293550,#293551),
(#293552,#293553),(#293554,#293555),(#293556,#293557),(#293558,#293559),
(#293560,#293561),(#293562,#293563),(#293564,#293565),(#293566,#293567),
(#293568,#293569),(#293570,#293571),(#293572,#293573),(#293574,#293575),
(#293576,#293577),(#293578,#293579),(#293580,#293581),(#293582,#293583),
(#293584,#293585),(#293586,#293587),(#293588,#293589),(#293590,#293591),
(#293592,#293593),(#293594,#293595),(#293596,#293597),(#293598,#293599),
(#293600,#293601),(#293602,#293603),(#293604,#293605),(#293606,#293607),
(#293608,#293609),(#293610,#293611),(#293612,#293613),(#293614,#293615),
(#293616,#293617),(#293618,#293619),(#293620,#293621),(#293622,#293623),
(#293624,#293625),(#293626,#293627),(#293628,#293629),(#293630,#293631),
(#293632,#293633),(#293634,#293635),(#293636,#293637),(#293638,#293639),
(#293640,#293641),(#293642,#293643),(#293644,#293645),(#293646,#293647),
(#293648,#293649),(#293650,#293651),(#293652,#293653),(#293654,#293655),
(#293656,#293657),(#293658,#293659),(#293660,#293661),(#293662,#293663),
(#293664,#293665),(#293666,#293667),(#293668,#293669),(#293670,#293671),
(#293672,#293673),(#293674,#293675),(#293676,#293677),(#293678,#293679),
(#293680,#293681),(#293682,#293683),(#293684,#293685),(#293686,#293687),
(#293688,#293689),(#293690,#293691),(#293692,#293693),(#293694,#293695),
(#293696,#293697),(#293698,#293699),(#293700,#293701),(#293702,#293703),
(#293704,#293705),(#293706,#293707),(#293708,#293709),(#293710,#293711),
(#293712,#293713),(#293714,#293715),(#293716,#293717),(#293718,#293719),
(#293720,#293721),(#293722,#293723),(#293724,#293725),(#293726,#293727),
(#293728,#293729),(#293730,#293731),(#293732,#293733),(#293734,#293735),
(#293736,#293737),(#293738,#293739),(#293740,#293741),(#293742,#293743),
(#293744,#293745),(#293746,#293747),(#293748,#293749),(#293750,#293751),
(#293752,#293753),(#293754,#293755),(#293756,#293757),(#293758,#293759),
(#293760,#293761),(#293762,#293763),(#293764,#293765),(#293766,#293767),
(#293768,#293769),(#293770,#293771),(#293772,#293773),(#293774,#293775),
(#293776,#293777),(#293778,#293779),(#293780,#293781),(#293782,#293783),
(#293784,#293785),(#293786,#293787),(#293788,#293789),(#293790,#293791),
(#293792,#293793),(#293794,#293795),(#293796,#293797),(#293798,#293799),
(#293800,#293801),(#293802,#293803),(#293804,#293805),(#293806,#293807),
(#293808,#293809),(#293810,#293811),(#293812,#293813),(#293814,#293815),
(#293816,#293817),(#293818,#293819),(#293820,#293821),(#293822,#293823),
(#293824,#293825),(#293826,#293827),(#293828,#293829),(#293830,#293831),
(#293832,#293833),(#293834,#293835),(#293836,#293837),(#293838,#293839),
(#293840,#293841),(#293842,#293843),(#293844,#293845),(#293846,#293847),
(#293848,#293849),(#293850,#293851),(#293852,#293853),(#293854,#293855),
(#293856,#293857),(#293858,#293859),(#293860,#293861),(#293862,#293863),
(#293864,#293865),(#293866,#293867),(#293868,#293869),(#293870,#293871),
(#293872,#293873),(#293874,#293875),(#293876,#293877),(#293878,#293879),
(#293880,#293881),(#293882,#293883),(#293884,#293885),(#293886,#293887),
(#293888,#293889),(#293890,#293891),(#293892,#293893),(#293894,#293895),
(#293896,#293897),(#293898,#293899),(#293900,#293901),(#293902,#293903),
(#293904,#293905),(#293906,#293907),(#293908,#293909),(#293910,#293911),
(#293912,#293913),(#293914,#293915),(#293916,#293917),(#293918,#293919),
(#293920,#293921),(#293922,#293923),(#293924,#293925),(#293926,#293927),
(#293928,#293929),(#293930,#293931),(#293932,#293933),(#293934,#293935),
(#293936,#293937),(#293938,#293939),(#293940,#293941),(#293942,#293943),
(#293944,#293945),(#293946,#293947),(#293948,#293949),(#293950,#293951),
(#293952,#293953),(#293954,#293955),(#293956,#293957),(#293958,#293959),
(#293960,#293961),(#293962,#293963),(#293964,#293965),(#293966,#293967),
(#293968,#293969),(#293970,#293971),(#293972,#293973),(#293974,#293975),
(#293976,#293977),(#293978,#293979),(#293980,#293981),(#293982,#293983),
(#293984,#293985),(#293986,#293987),(#293988,#293989),(#293990,#293991),
(#293992,#293993),(#293994,#293995),(#293996,#293997),(#293998,#293999),
(#294000,#294001),(#294002,#294003),(#294004,#294005),(#294006,#294007),
(#294008,#294009),(#294010,#294011),(#294012,#294013),(#294014,#294015),
(#294016,#294017),(#294018,#294019),(#294020,#294021),(#294022,#294023),
(#294024,#294025),(#294026,#294027),(#294028,#294029),(#294030,#294031),
(#294032,#294033),(#294034,#294035),(#294036,#294037),(#294038,#294039),
(#294040,#294041),(#294042,#294043),(#294044,#294045),(#294046,#294047),
(#294048,#294049),(#294050,#294051),(#294052,#294053),(#294054,#294055),
(#294056,#294057),(#294058,#294059),(#294060,#294061),(#294062,#294063),
(#294064,#294065),(#294066,#294067),(#294068,#294069),(#294070,#294071),
(#294072,#294073),(#294074,#294075),(#294076,#294077),(#294078,#294079),
(#294080,#294081),(#294082,#294083),(#294084,#294085),(#294086,#294087),
(#294088,#294089),(#294090,#294091),(#294092,#294093),(#294094,#294095),
(#294096,#294097),(#294098,#294099),(#294100,#294101),(#294102,#294103),
(#294104,#294105),(#294106,#294107),(#294108,#294109),(#294110,#294111),
(#294112,#294113),(#294114,#294115),(#294116,#294117),(#294118,#294119),
(#294120,#294121),(#294122,#294123),(#294124,#294125),(#294126,#294127),
(#294128,#294129),(#294130,#294131),(#294132,#294133),(#294134,#294135),
(#294136,#294137),(#294138,#294139),(#294140,#294141),(#294142,#294143),
(#294144,#294145),(#294146,#294147),(#294148,#294149),(#294150,#294151),
(#294152,#294153),(#294154,#294155),(#294156,#294157),(#294158,#294159),
(#294160,#294161),(#294162,#294163),(#294164,#294165),(#294166,#294167),
(#294168,#294169),(#294170,#294171)),.UNSPECIFIED.,.F.,.F.,.F.,(6,1,1,1,
1,1,1,1,1,1,1,1,1,1,1,1,1,1,1,1,1,1,1,1,1,1,1,1,1,1,1,1,1,1,1,1,1,1,1,1,
1,1,1,1,1,1,1,1,1,1,1,1,1,1,1,1,1,1,1,1,1,1,1,1,1,1,1,1,1,1,1,1,1,1,1,1,
1,1,1,1,1,1,1,1,1,1,1,1,1,1,1,1,1,1,1,1,1,1,1,1,1,1,1,1,1,1,1,1,1,1,1,1,
1,1,1,1,1,1,1,1,1,1,1,1,1,1,1,1,1,1,1,1,1,1,1,1,1,1,1,1,1,1,1,1,1,1,1,1,
1,1,1,1,1,1,1,1,1,1,1,1,1,1,1,1,1,1,1,1,1,1,1,1,1,1,1,1,1,1,1,1,1,1,1,1,
1,1,1,1,1,1,1,1,1,1,1,1,1,1,1,1,1,1,1,1,1,1,1,1,1,1,1,1,1,1,1,1,1,1,1,1,
1,1,1,1,1,1,1,1,1,1,1,1,1,1,1,1,1,1,1,1,1,1,1,1,1,1,1,1,1,1,1,1,1,1,1,1,
1,1,1,1,1,1,1,1,1,1,1,1,1,1,1,1,1,1,1,1,1,1,1,1,1,1,1,1,1,1,1,1,1,1,1,1,
1,1,1,1,1,1,1,1,1,1,1,1,1,1,1,1,1,1,1,1,1,1,1,1,1,1,1,1,1,1,1,1,1,1,1,1,
1,1,1,1,1,1,1,1,1,1,1,1,1,1,1,1,1,1,1,1,1,1,1,1,1,1,1,1,1,1,1,1,1,1,1,1,
1,1,1,1,1,1,1,1,1,1,1,1,1,1,1,1,1,1,1,1,1,1,1,1,1,1,1,1,1,1,1,1,1,1,1,1,
1,1,1,1,1,1,1,1,1,1,1,1,1,1,1,1,1,1,1,1,1,1,1,1,1,1,1,1,1,1,1,1,1,1,1,1,
1,1,1,1,1,1,1,1,1,1,1,1,1,1,1,1,1,1,1,1,1,1,1,1,1,1,1,1,1,1,1,6),(2,2),
(0.143172103,0.144954128,0.146788991,0.148623853,0.150458716,0.152293578,
0.15412844,0.155963303,0.157798165,0.159633028,0.16146789,0.163302752,0.165137615,
0.166972477,0.168807339,0.170642202,0.172477064,0.174311927,0.176146789,
0.177981651,0.179816514,0.181651376,0.183486239,0.185321101,0.187155963,
0.188990826,0.190825688,0.19266055,0.194495413,0.196330275,0.198165138,
0.2,0.201834862,0.203669725,0.205504587,0.20733945,0.209174312,0.211009174,
0.212844037,0.214678899,0.216513761,0.218348624,0.220183486,0.222018349,
0.223853211,0.225688073,0.227522936,0.229357798,0.231192661,0.233027523,
0.234862385,0.236697248,0.23853211,0.240366972,0.242201835,0.244036697,
0.24587156,0.247706422,0.249541284,0.251376147,0.253211009,0.255045872,
0.256880734,0.258715596,0.260550459,0.262385321,0.264220183,0.266055046,
0.267889908,0.269724771,0.271559633,0.273394495,0.275229358,0.27706422,
0.278899083,0.280733945,0.282568807,0.28440367,0.286238532,0.288073394,
0.289908257,0.291743119,0.293577982,0.295412844,0.297247706,0.299082569,
0.300917431,0.302752294,0.304587156,0.306422018,0.308256881,0.310091743,
0.311926606,0.313761468,0.31559633,0.317431193,0.319266055,0.321100917,
0.32293578,0.324770642,0.326605505,0.328440367,0.330275229,0.332110092,
0.333944954,0.335779817,0.337614679,0.339449541,0.341284404,0.343119266,
0.344954128,0.346788991,0.348623853,0.350458716,0.352293578,0.35412844,
0.355963303,0.357798165,0.359633028,0.36146789,0.363302752,0.365137615,
0.366972477,0.368807339,0.370642202,0.372477064,0.374311927,0.376146789,
0.377981651,0.379816514,0.381651376,0.383486239,0.385321101,0.387155963,
0.388990826,0.390825688,0.39266055,0.394495413,0.396330275,0.398165138,
0.4,0.401834862,0.403669725,0.405504587,0.40733945,0.409174312,0.411009174,
0.412844037,0.414678899,0.416513761,0.418348624,0.420183486,0.422018349,
0.423853211,0.425688073,0.427522936,0.429357798,0.431192661,0.433027523,
0.434862385,0.436697248,0.43853211,0.440366972,0.442201835,0.444036697,
0.44587156,0.447706422,0.449541284,0.451376147,0.453211009,0.455045872,
0.456880734,0.458715596,0.460550459,0.462385321,0.464220183,0.466055046,
0.467889908,0.469724771,0.471559633,0.473394495,0.475229358,0.47706422,
0.478899083,0.480733945,0.482568807,0.48440367,0.486238532,0.488073394,
0.489908257,0.491743119,0.493577982,0.495412844,0.497247706,0.499082569,
0.500917431,0.502752294,0.504587156,0.506422018,0.508256881,0.510091743,
0.511926606,0.513761468,0.51559633,0.517431193,0.519266055,0.521100917,
0.52293578,0.524770642,0.526605505,0.528440367,0.530275229,0.532110092,
0.533944954,0.535779817,0.537614679,0.539449541,0.541284404,0.543119266,
0.544954128,0.546788991,0.548623853,0.550458716,0.552293578,0.55412844,
0.555963303,0.557798165,0.559633028,0.56146789,0.563302752,0.565137615,
0.566972477,0.568807339,0.570642202,0.572477064,0.574311927,0.576146789,
0.577981651,0.579816514,0.581651376,0.583486239,0.585321101,0.587155963,
0.588990826,0.590825688,0.59266055,0.594495413,0.596330275,0.598165138,
0.6,0.601834862,0.603669725,0.605504587,0.60733945,0.609174312,0.611009174,
0.612844037,0.614678899,0.616513761,0.618348624,0.620183486,0.622018349,
0.623853211,0.625688073,0.627522936,0.629357798,0.631192661,0.633027523,
0.634862385,0.636697248,0.63853211,0.640366972,0.642201835,0.644036697,
0.64587156,0.647706422,0.649541284,0.651376147,0.653211009,0.655045872,
0.656880734,0.658715596,0.660550459,0.662385321,0.664220183,0.666055046,
0.667889908,0.669724771,0.671559633,0.673394495,0.675229358,0.67706422,
0.678899083,0.680733945,0.682568807,0.68440367,0.686238532,0.688073394,
0.689908257,0.691743119,0.693577982,0.695412844,0.697247706,0.699082569,
0.700917431,0.702752294,0.704587156,0.706422018,0.708256881,0.710091743,
0.711926606,0.713761468,0.71559633,0.717431193,0.719266055,0.721100917,
0.72293578,0.724770642,0.726605505,0.728440367,0.730275229,0.732110092,
0.733944954,0.735779817,0.737614679,0.739449541,0.741284404,0.743119266,
0.744954128,0.746788991,0.748623853,0.750458716,0.752293578,0.75412844,
0.755963303,0.757798165,0.759633028,0.76146789,0.763302752,0.765137615,
0.766972477,0.768807339,0.770642202,0.772477064,0.774311927,0.776146789,
0.777981651,0.779816514,0.781651376,0.783486239,0.785321101,0.787155963,
0.788990826,0.790825688,0.79266055,0.794495413,0.796330275,0.798165138,
0.8,0.801834862,0.803669725,0.805504587,0.80733945,0.809174312,0.811009174,
0.812844037,0.814678899,0.816513761,0.818348624,0.820183486,0.822018349,
0.823853211,0.825688073,0.827522936,0.829357798,0.831192661,0.833027523,
0.834862385,0.836697248,0.83853211,0.840366972,0.842201835,0.844036697,
0.84587156,0.847706422,0.849541284,0.851376147,0.853211009,0.855045872,
0.856880734,0.858715596,0.860550459,0.862385321,0.864220183,0.866055046,
0.867889908,0.869724771,0.871559633,0.873394495,0.875229358,0.87706422,
0.878899083,0.880733945,0.882568807,0.88440367,0.886238532,0.888073394,
0.889908257,0.891743119,0.893577982,0.895412844,0.897247706,0.899082569,
0.900917431,0.902752294,0.904587156,0.906422018,0.908256881,0.910091743,
0.911926606,0.913761468,0.91559633,0.917431193,0.919266055,0.921100917,
0.92293578,0.924770642,0.926605505,0.928440367,0.930275229,0.932110092,
0.933944954,0.935779817,0.937614679,0.939449541,0.941284404,0.943119266,
0.944954128,0.946788991,0.948623853,0.950458716,0.952293578,0.95412844,
0.955963303,0.957798165,0.959633028,0.96146789,0.963302752,0.965137615,
0.966972477,0.968807339,0.970642202,0.972477064,0.974311927,0.976146789,
0.977981651,0.979816514,0.981651376,0.983486239,0.985321101,0.987155963,
0.988990826,0.990825688,0.99266055,0.994495413,0.996330275,0.998165138,
1.),(0.,0.36),.UNSPECIFIED.);
#6300=B_SPLINE_SURFACE_WITH_KNOTS('',5,1,((#294807,#294808),(#294809,#294810),
(#294811,#294812),(#294813,#294814),(#294815,#294816),(#294817,#294818),
(#294819,#294820),(#294821,#294822),(#294823,#294824),(#294825,#294826),
(#294827,#294828),(#294829,#294830),(#294831,#294832),(#294833,#294834),
(#294835,#294836),(#294837,#294838),(#294839,#294840),(#294841,#294842),
(#294843,#294844),(#294845,#294846),(#294847,#294848),(#294849,#294850),
(#294851,#294852),(#294853,#294854),(#294855,#294856),(#294857,#294858),
(#294859,#294860),(#294861,#294862),(#294863,#294864),(#294865,#294866),
(#294867,#294868),(#294869,#294870),(#294871,#294872),(#294873,#294874),
(#294875,#294876),(#294877,#294878),(#294879,#294880),(#294881,#294882),
(#294883,#294884),(#294885,#294886),(#294887,#294888),(#294889,#294890),
(#294891,#294892),(#294893,#294894),(#294895,#294896),(#294897,#294898),
(#294899,#294900),(#294901,#294902),(#294903,#294904),(#294905,#294906),
(#294907,#294908),(#294909,#294910),(#294911,#294912),(#294913,#294914),
(#294915,#294916),(#294917,#294918),(#294919,#294920),(#294921,#294922),
(#294923,#294924),(#294925,#294926),(#294927,#294928),(#294929,#294930),
(#294931,#294932),(#294933,#294934),(#294935,#294936),(#294937,#294938),
(#294939,#294940),(#294941,#294942),(#294943,#294944),(#294945,#294946),
(#294947,#294948),(#294949,#294950),(#294951,#294952),(#294953,#294954),
(#294955,#294956),(#294957,#294958),(#294959,#294960),(#294961,#294962),
(#294963,#294964),(#294965,#294966),(#294967,#294968),(#294969,#294970),
(#294971,#294972),(#294973,#294974),(#294975,#294976),(#294977,#294978),
(#294979,#294980),(#294981,#294982),(#294983,#294984),(#294985,#294986),
(#294987,#294988),(#294989,#294990),(#294991,#294992),(#294993,#294994),
(#294995,#294996),(#294997,#294998),(#294999,#295000),(#295001,#295002),
(#295003,#295004),(#295005,#295006),(#295007,#295008),(#295009,#295010),
(#295011,#295012),(#295013,#295014),(#295015,#295016),(#295017,#295018),
(#295019,#295020),(#295021,#295022),(#295023,#295024),(#295025,#295026),
(#295027,#295028),(#295029,#295030),(#295031,#295032),(#295033,#295034),
(#295035,#295036),(#295037,#295038),(#295039,#295040),(#295041,#295042),
(#295043,#295044),(#295045,#295046),(#295047,#295048),(#295049,#295050),
(#295051,#295052),(#295053,#295054),(#295055,#295056),(#295057,#295058),
(#295059,#295060),(#295061,#295062),(#295063,#295064),(#295065,#295066),
(#295067,#295068),(#295069,#295070),(#295071,#295072),(#295073,#295074),
(#295075,#295076),(#295077,#295078),(#295079,#295080),(#295081,#295082),
(#295083,#295084),(#295085,#295086),(#295087,#295088),(#295089,#295090),
(#295091,#295092),(#295093,#295094),(#295095,#295096),(#295097,#295098),
(#295099,#295100),(#295101,#295102),(#295103,#295104),(#295105,#295106),
(#295107,#295108),(#295109,#295110),(#295111,#295112),(#295113,#295114),
(#295115,#295116),(#295117,#295118),(#295119,#295120),(#295121,#295122),
(#295123,#295124),(#295125,#295126),(#295127,#295128),(#295129,#295130),
(#295131,#295132),(#295133,#295134),(#295135,#295136),(#295137,#295138),
(#295139,#295140),(#295141,#295142),(#295143,#295144),(#295145,#295146),
(#295147,#295148),(#295149,#295150),(#295151,#295152),(#295153,#295154),
(#295155,#295156),(#295157,#295158),(#295159,#295160),(#295161,#295162),
(#295163,#295164),(#295165,#295166),(#295167,#295168),(#295169,#295170),
(#295171,#295172),(#295173,#295174),(#295175,#295176),(#295177,#295178),
(#295179,#295180),(#295181,#295182),(#295183,#295184),(#295185,#295186),
(#295187,#295188),(#295189,#295190),(#295191,#295192),(#295193,#295194),
(#295195,#295196),(#295197,#295198),(#295199,#295200),(#295201,#295202),
(#295203,#295204),(#295205,#295206),(#295207,#295208),(#295209,#295210),
(#295211,#295212),(#295213,#295214),(#295215,#295216),(#295217,#295218),
(#295219,#295220),(#295221,#295222),(#295223,#295224),(#295225,#295226),
(#295227,#295228),(#295229,#295230),(#295231,#295232),(#295233,#295234),
(#295235,#295236),(#295237,#295238),(#295239,#295240),(#295241,#295242),
(#295243,#295244),(#295245,#295246),(#295247,#295248),(#295249,#295250),
(#295251,#295252),(#295253,#295254),(#295255,#295256),(#295257,#295258),
(#295259,#295260),(#295261,#295262),(#295263,#295264),(#295265,#295266),
(#295267,#295268),(#295269,#295270),(#295271,#295272),(#295273,#295274),
(#295275,#295276),(#295277,#295278),(#295279,#295280),(#295281,#295282),
(#295283,#295284),(#295285,#295286),(#295287,#295288),(#295289,#295290),
(#295291,#295292),(#295293,#295294),(#295295,#295296),(#295297,#295298),
(#295299,#295300),(#295301,#295302),(#295303,#295304),(#295305,#295306),
(#295307,#295308),(#295309,#295310),(#295311,#295312),(#295313,#295314),
(#295315,#295316),(#295317,#295318),(#295319,#295320),(#295321,#295322),
(#295323,#295324),(#295325,#295326),(#295327,#295328),(#295329,#295330),
(#295331,#295332),(#295333,#295334),(#295335,#295336),(#295337,#295338),
(#295339,#295340),(#295341,#295342),(#295343,#295344),(#295345,#295346),
(#295347,#295348),(#295349,#295350),(#295351,#295352),(#295353,#295354),
(#295355,#295356),(#295357,#295358),(#295359,#295360),(#295361,#295362),
(#295363,#295364),(#295365,#295366),(#295367,#295368),(#295369,#295370),
(#295371,#295372),(#295373,#295374),(#295375,#295376),(#295377,#295378),
(#295379,#295380),(#295381,#295382),(#295383,#295384),(#295385,#295386),
(#295387,#295388),(#295389,#295390),(#295391,#295392),(#295393,#295394),
(#295395,#295396),(#295397,#295398),(#295399,#295400),(#295401,#295402),
(#295403,#295404),(#295405,#295406),(#295407,#295408),(#295409,#295410),
(#295411,#295412),(#295413,#295414),(#295415,#295416),(#295417,#295418),
(#295419,#295420),(#295421,#295422),(#295423,#295424),(#295425,#295426),
(#295427,#295428),(#295429,#295430),(#295431,#295432),(#295433,#295434),
(#295435,#295436),(#295437,#295438),(#295439,#295440),(#295441,#295442),
(#295443,#295444),(#295445,#295446),(#295447,#295448),(#295449,#295450),
(#295451,#295452),(#295453,#295454),(#295455,#295456),(#295457,#295458),
(#295459,#295460),(#295461,#295462),(#295463,#295464),(#295465,#295466),
(#295467,#295468),(#295469,#295470),(#295471,#295472),(#295473,#295474),
(#295475,#295476),(#295477,#295478),(#295479,#295480),(#295481,#295482),
(#295483,#295484),(#295485,#295486),(#295487,#295488),(#295489,#295490),
(#295491,#295492),(#295493,#295494),(#295495,#295496),(#295497,#295498),
(#295499,#295500),(#295501,#295502),(#295503,#295504),(#295505,#295506),
(#295507,#295508),(#295509,#295510),(#295511,#295512),(#295513,#295514),
(#295515,#295516),(#295517,#295518),(#295519,#295520),(#295521,#295522),
(#295523,#295524),(#295525,#295526),(#295527,#295528),(#295529,#295530),
(#295531,#295532),(#295533,#295534),(#295535,#295536),(#295537,#295538),
(#295539,#295540),(#295541,#295542),(#295543,#295544),(#295545,#295546),
(#295547,#295548),(#295549,#295550),(#295551,#295552),(#295553,#295554),
(#295555,#295556),(#295557,#295558),(#295559,#295560),(#295561,#295562),
(#295563,#295564),(#295565,#295566),(#295567,#295568),(#295569,#295570),
(#295571,#295572),(#295573,#295574),(#295575,#295576),(#295577,#295578),
(#295579,#295580),(#295581,#295582),(#295583,#295584),(#295585,#295586),
(#295587,#295588),(#295589,#295590),(#295591,#295592),(#295593,#295594),
(#295595,#295596),(#295597,#295598),(#295599,#295600),(#295601,#295602),
(#295603,#295604),(#295605,#295606),(#295607,#295608),(#295609,#295610),
(#295611,#295612),(#295613,#295614),(#295615,#295616),(#295617,#295618),
(#295619,#295620),(#295621,#295622),(#295623,#295624),(#295625,#295626),
(#295627,#295628),(#295629,#295630),(#295631,#295632),(#295633,#295634),
(#295635,#295636),(#295637,#295638),(#295639,#295640),(#295641,#295642),
(#295643,#295644),(#295645,#295646),(#295647,#295648),(#295649,#295650),
(#295651,#295652),(#295653,#295654),(#295655,#295656),(#295657,#295658),
(#295659,#295660),(#295661,#295662),(#295663,#295664),(#295665,#295666),
(#295667,#295668),(#295669,#295670),(#295671,#295672),(#295673,#295674),
(#295675,#295676),(#295677,#295678),(#295679,#295680),(#295681,#295682),
(#295683,#295684),(#295685,#295686),(#295687,#295688),(#295689,#295690),
(#295691,#295692),(#295693,#295694),(#295695,#295696),(#295697,#295698),
(#295699,#295700),(#295701,#295702),(#295703,#295704),(#295705,#295706),
(#295707,#295708),(#295709,#295710),(#295711,#295712),(#295713,#295714),
(#295715,#295716),(#295717,#295718),(#295719,#295720),(#295721,#295722),
(#295723,#295724),(#295725,#295726),(#295727,#295728),(#295729,#295730),
(#295731,#295732),(#295733,#295734),(#295735,#295736),(#295737,#295738),
(#295739,#295740),(#295741,#295742),(#295743,#295744),(#295745,#295746),
(#295747,#295748),(#295749,#295750)),.UNSPECIFIED.,.F.,.F.,.F.,(6,1,1,1,
1,1,1,1,1,1,1,1,1,1,1,1,1,1,1,1,1,1,1,1,1,1,1,1,1,1,1,1,1,1,1,1,1,1,1,1,
1,1,1,1,1,1,1,1,1,1,1,1,1,1,1,1,1,1,1,1,1,1,1,1,1,1,1,1,1,1,1,1,1,1,1,1,
1,1,1,1,1,1,1,1,1,1,1,1,1,1,1,1,1,1,1,1,1,1,1,1,1,1,1,1,1,1,1,1,1,1,1,1,
1,1,1,1,1,1,1,1,1,1,1,1,1,1,1,1,1,1,1,1,1,1,1,1,1,1,1,1,1,1,1,1,1,1,1,1,
1,1,1,1,1,1,1,1,1,1,1,1,1,1,1,1,1,1,1,1,1,1,1,1,1,1,1,1,1,1,1,1,1,1,1,1,
1,1,1,1,1,1,1,1,1,1,1,1,1,1,1,1,1,1,1,1,1,1,1,1,1,1,1,1,1,1,1,1,1,1,1,1,
1,1,1,1,1,1,1,1,1,1,1,1,1,1,1,1,1,1,1,1,1,1,1,1,1,1,1,1,1,1,1,1,1,1,1,1,
1,1,1,1,1,1,1,1,1,1,1,1,1,1,1,1,1,1,1,1,1,1,1,1,1,1,1,1,1,1,1,1,1,1,1,1,
1,1,1,1,1,1,1,1,1,1,1,1,1,1,1,1,1,1,1,1,1,1,1,1,1,1,1,1,1,1,1,1,1,1,1,1,
1,1,1,1,1,1,1,1,1,1,1,1,1,1,1,1,1,1,1,1,1,1,1,1,1,1,1,1,1,1,1,1,1,1,1,1,
1,1,1,1,1,1,1,1,1,1,1,1,1,1,1,1,1,1,1,1,1,1,1,1,1,1,1,1,1,1,1,1,1,1,1,1,
1,1,1,1,1,1,1,1,1,1,1,1,1,1,1,1,1,1,1,1,1,1,1,1,1,1,1,1,1,1,1,1,1,1,1,1,
1,1,1,1,1,1,1,1,1,1,1,1,1,1,1,1,1,1,1,1,1,1,1,1,1,1,1,1,1,1,1,6),(2,2),
(-1.,-0.998165138,-0.996330275,-0.994495413,-0.99266055,-0.990825688,-0.988990826,
-0.987155963,-0.985321101,-0.983486239,-0.981651376,-0.979816514,-0.977981651,
-0.976146789,-0.974311927,-0.972477064,-0.970642202,-0.968807339,-0.966972477,
-0.965137615,-0.963302752,-0.96146789,-0.959633028,-0.957798165,-0.955963303,
-0.95412844,-0.952293578,-0.950458716,-0.948623853,-0.946788991,-0.944954128,
-0.943119266,-0.941284404,-0.939449541,-0.937614679,-0.935779817,-0.933944954,
-0.932110092,-0.930275229,-0.928440367,-0.926605505,-0.924770642,-0.92293578,
-0.921100917,-0.919266055,-0.917431193,-0.91559633,-0.913761468,-0.911926606,
-0.910091743,-0.908256881,-0.906422018,-0.904587156,-0.902752294,-0.900917431,
-0.899082569,-0.897247706,-0.895412844,-0.893577982,-0.891743119,-0.889908257,
-0.888073394,-0.886238532,-0.88440367,-0.882568807,-0.880733945,-0.878899083,
-0.87706422,-0.875229358,-0.873394495,-0.871559633,-0.869724771,-0.867889908,
-0.866055046,-0.864220183,-0.862385321,-0.860550459,-0.858715596,-0.856880734,
-0.855045872,-0.853211009,-0.851376147,-0.849541284,-0.847706422,-0.84587156,
-0.844036697,-0.842201835,-0.840366972,-0.83853211,-0.836697248,-0.834862385,
-0.833027523,-0.831192661,-0.829357798,-0.827522936,-0.825688073,-0.823853211,
-0.822018349,-0.820183486,-0.818348624,-0.816513761,-0.814678899,-0.812844037,
-0.811009174,-0.809174312,-0.80733945,-0.805504587,-0.803669725,-0.801834862,
-0.8,-0.798165138,-0.796330275,-0.794495413,-0.79266055,-0.790825688,-0.788990826,
-0.787155963,-0.785321101,-0.783486239,-0.781651376,-0.779816514,-0.777981651,
-0.776146789,-0.774311927,-0.772477064,-0.770642202,-0.768807339,-0.766972477,
-0.765137615,-0.763302752,-0.76146789,-0.759633028,-0.757798165,-0.755963303,
-0.75412844,-0.752293578,-0.750458716,-0.748623853,-0.746788991,-0.744954128,
-0.743119266,-0.741284404,-0.739449541,-0.737614679,-0.735779817,-0.733944954,
-0.732110092,-0.730275229,-0.728440367,-0.726605505,-0.724770642,-0.72293578,
-0.721100917,-0.719266055,-0.717431193,-0.71559633,-0.713761468,-0.711926606,
-0.710091743,-0.708256881,-0.706422018,-0.704587156,-0.702752294,-0.700917431,
-0.699082569,-0.697247706,-0.695412844,-0.693577982,-0.691743119,-0.689908257,
-0.688073394,-0.686238532,-0.68440367,-0.682568807,-0.680733945,-0.678899083,
-0.67706422,-0.675229358,-0.673394495,-0.671559633,-0.669724771,-0.667889908,
-0.666055046,-0.664220183,-0.662385321,-0.660550459,-0.658715596,-0.656880734,
-0.655045872,-0.653211009,-0.651376147,-0.649541284,-0.647706422,-0.64587156,
-0.644036697,-0.642201835,-0.640366972,-0.63853211,-0.636697248,-0.634862385,
-0.633027523,-0.631192661,-0.629357798,-0.627522936,-0.625688073,-0.623853211,
-0.622018349,-0.620183486,-0.618348624,-0.616513761,-0.614678899,-0.612844037,
-0.611009174,-0.609174312,-0.60733945,-0.605504587,-0.603669725,-0.601834862,
-0.6,-0.598165138,-0.596330275,-0.594495413,-0.59266055,-0.590825688,-0.588990826,
-0.587155963,-0.585321101,-0.583486239,-0.581651376,-0.579816514,-0.577981651,
-0.576146789,-0.574311927,-0.572477064,-0.570642202,-0.568807339,-0.566972477,
-0.565137615,-0.563302752,-0.56146789,-0.559633028,-0.557798165,-0.555963303,
-0.55412844,-0.552293578,-0.550458716,-0.548623853,-0.546788991,-0.544954128,
-0.543119266,-0.541284404,-0.539449541,-0.537614679,-0.535779817,-0.533944954,
-0.532110092,-0.530275229,-0.528440367,-0.526605505,-0.524770642,-0.52293578,
-0.521100917,-0.519266055,-0.517431193,-0.51559633,-0.513761468,-0.511926606,
-0.510091743,-0.508256881,-0.506422018,-0.504587156,-0.502752294,-0.500917431,
-0.499082569,-0.497247706,-0.495412844,-0.493577982,-0.491743119,-0.489908257,
-0.488073394,-0.486238532,-0.48440367,-0.482568807,-0.480733945,-0.478899083,
-0.47706422,-0.475229358,-0.473394495,-0.471559633,-0.469724771,-0.467889908,
-0.466055046,-0.464220183,-0.462385321,-0.460550459,-0.458715596,-0.456880734,
-0.455045872,-0.453211009,-0.451376147,-0.449541284,-0.447706422,-0.44587156,
-0.444036697,-0.442201835,-0.440366972,-0.43853211,-0.436697248,-0.434862385,
-0.433027523,-0.431192661,-0.429357798,-0.427522936,-0.425688073,-0.423853211,
-0.422018349,-0.420183486,-0.418348624,-0.416513761,-0.414678899,-0.412844037,
-0.411009174,-0.409174312,-0.40733945,-0.405504587,-0.403669725,-0.401834862,
-0.4,-0.398165138,-0.396330275,-0.394495413,-0.39266055,-0.390825688,-0.388990826,
-0.387155963,-0.385321101,-0.383486239,-0.381651376,-0.379816514,-0.377981651,
-0.376146789,-0.374311927,-0.372477064,-0.370642202,-0.368807339,-0.366972477,
-0.365137615,-0.363302752,-0.36146789,-0.359633028,-0.357798165,-0.355963303,
-0.35412844,-0.352293578,-0.350458716,-0.348623853,-0.346788991,-0.344954128,
-0.343119266,-0.341284404,-0.339449541,-0.337614679,-0.335779817,-0.333944954,
-0.332110092,-0.330275229,-0.328440367,-0.326605505,-0.324770642,-0.32293578,
-0.321100917,-0.319266055,-0.317431193,-0.31559633,-0.313761468,-0.311926606,
-0.310091743,-0.308256881,-0.306422018,-0.304587156,-0.302752294,-0.300917431,
-0.299082569,-0.297247706,-0.295412844,-0.293577982,-0.291743119,-0.289908257,
-0.288073394,-0.286238532,-0.28440367,-0.282568807,-0.280733945,-0.278899083,
-0.27706422,-0.275229358,-0.273394495,-0.271559633,-0.269724771,-0.267889908,
-0.266055046,-0.264220183,-0.262385321,-0.260550459,-0.258715596,-0.256880734,
-0.255045872,-0.253211009,-0.251376147,-0.249541284,-0.247706422,-0.24587156,
-0.244036697,-0.242201835,-0.240366972,-0.23853211,-0.236697248,-0.234862385,
-0.233027523,-0.231192661,-0.229357798,-0.227522936,-0.225688073,-0.223853211,
-0.222018349,-0.220183486,-0.218348624,-0.216513761,-0.214678899,-0.212844037,
-0.211009174,-0.209174312,-0.20733945,-0.205504587,-0.203669725,-0.201834862,
-0.2,-0.198165138,-0.196330275,-0.194495413,-0.19266055,-0.190825688,-0.188990826,
-0.187155963,-0.185321101,-0.183486239,-0.181651376,-0.179816514,-0.177981651,
-0.176146789,-0.174311927,-0.172477064,-0.170642202,-0.168807339,-0.166972477,
-0.165137615,-0.163302752,-0.16146789,-0.159633028,-0.157798165,-0.155963303,
-0.15412844,-0.152293578,-0.150458716,-0.148623853,-0.146788991,-0.144954128,
-0.143172103),(0.,0.36),.UNSPECIFIED.);
#6301=B_SPLINE_SURFACE_WITH_KNOTS('',5,1,((#297515,#297516),(#297517,#297518),
(#297519,#297520),(#297521,#297522),(#297523,#297524),(#297525,#297526),
(#297527,#297528),(#297529,#297530),(#297531,#297532),(#297533,#297534),
(#297535,#297536),(#297537,#297538),(#297539,#297540),(#297541,#297542),
(#297543,#297544),(#297545,#297546),(#297547,#297548),(#297549,#297550),
(#297551,#297552),(#297553,#297554),(#297555,#297556),(#297557,#297558),
(#297559,#297560),(#297561,#297562),(#297563,#297564),(#297565,#297566),
(#297567,#297568),(#297569,#297570),(#297571,#297572),(#297573,#297574),
(#297575,#297576),(#297577,#297578),(#297579,#297580),(#297581,#297582),
(#297583,#297584),(#297585,#297586),(#297587,#297588),(#297589,#297590),
(#297591,#297592),(#297593,#297594),(#297595,#297596),(#297597,#297598),
(#297599,#297600),(#297601,#297602),(#297603,#297604),(#297605,#297606),
(#297607,#297608),(#297609,#297610),(#297611,#297612),(#297613,#297614),
(#297615,#297616),(#297617,#297618),(#297619,#297620),(#297621,#297622),
(#297623,#297624),(#297625,#297626),(#297627,#297628),(#297629,#297630),
(#297631,#297632),(#297633,#297634),(#297635,#297636),(#297637,#297638),
(#297639,#297640),(#297641,#297642),(#297643,#297644),(#297645,#297646),
(#297647,#297648),(#297649,#297650),(#297651,#297652),(#297653,#297654),
(#297655,#297656),(#297657,#297658),(#297659,#297660),(#297661,#297662),
(#297663,#297664),(#297665,#297666),(#297667,#297668),(#297669,#297670),
(#297671,#297672),(#297673,#297674),(#297675,#297676),(#297677,#297678),
(#297679,#297680),(#297681,#297682),(#297683,#297684),(#297685,#297686),
(#297687,#297688),(#297689,#297690),(#297691,#297692),(#297693,#297694),
(#297695,#297696),(#297697,#297698),(#297699,#297700),(#297701,#297702),
(#297703,#297704),(#297705,#297706),(#297707,#297708),(#297709,#297710),
(#297711,#297712),(#297713,#297714),(#297715,#297716),(#297717,#297718),
(#297719,#297720),(#297721,#297722),(#297723,#297724),(#297725,#297726),
(#297727,#297728),(#297729,#297730),(#297731,#297732),(#297733,#297734),
(#297735,#297736),(#297737,#297738),(#297739,#297740),(#297741,#297742),
(#297743,#297744),(#297745,#297746),(#297747,#297748),(#297749,#297750),
(#297751,#297752),(#297753,#297754),(#297755,#297756),(#297757,#297758),
(#297759,#297760),(#297761,#297762),(#297763,#297764),(#297765,#297766),
(#297767,#297768),(#297769,#297770),(#297771,#297772),(#297773,#297774),
(#297775,#297776),(#297777,#297778),(#297779,#297780),(#297781,#297782),
(#297783,#297784),(#297785,#297786),(#297787,#297788),(#297789,#297790),
(#297791,#297792),(#297793,#297794),(#297795,#297796),(#297797,#297798),
(#297799,#297800),(#297801,#297802),(#297803,#297804),(#297805,#297806),
(#297807,#297808),(#297809,#297810),(#297811,#297812),(#297813,#297814),
(#297815,#297816),(#297817,#297818),(#297819,#297820),(#297821,#297822),
(#297823,#297824),(#297825,#297826),(#297827,#297828),(#297829,#297830),
(#297831,#297832),(#297833,#297834),(#297835,#297836),(#297837,#297838),
(#297839,#297840),(#297841,#297842),(#297843,#297844),(#297845,#297846),
(#297847,#297848),(#297849,#297850),(#297851,#297852),(#297853,#297854),
(#297855,#297856),(#297857,#297858),(#297859,#297860),(#297861,#297862),
(#297863,#297864),(#297865,#297866),(#297867,#297868),(#297869,#297870),
(#297871,#297872),(#297873,#297874),(#297875,#297876),(#297877,#297878),
(#297879,#297880),(#297881,#297882),(#297883,#297884),(#297885,#297886),
(#297887,#297888),(#297889,#297890),(#297891,#297892),(#297893,#297894),
(#297895,#297896),(#297897,#297898),(#297899,#297900),(#297901,#297902),
(#297903,#297904),(#297905,#297906),(#297907,#297908),(#297909,#297910),
(#297911,#297912),(#297913,#297914),(#297915,#297916),(#297917,#297918),
(#297919,#297920),(#297921,#297922),(#297923,#297924),(#297925,#297926),
(#297927,#297928),(#297929,#297930),(#297931,#297932),(#297933,#297934),
(#297935,#297936),(#297937,#297938),(#297939,#297940),(#297941,#297942),
(#297943,#297944),(#297945,#297946),(#297947,#297948),(#297949,#297950),
(#297951,#297952),(#297953,#297954),(#297955,#297956),(#297957,#297958),
(#297959,#297960),(#297961,#297962),(#297963,#297964),(#297965,#297966),
(#297967,#297968),(#297969,#297970),(#297971,#297972),(#297973,#297974),
(#297975,#297976),(#297977,#297978),(#297979,#297980),(#297981,#297982),
(#297983,#297984),(#297985,#297986),(#297987,#297988),(#297989,#297990),
(#297991,#297992),(#297993,#297994),(#297995,#297996),(#297997,#297998),
(#297999,#298000),(#298001,#298002),(#298003,#298004),(#298005,#298006),
(#298007,#298008),(#298009,#298010),(#298011,#298012),(#298013,#298014),
(#298015,#298016),(#298017,#298018),(#298019,#298020),(#298021,#298022),
(#298023,#298024),(#298025,#298026),(#298027,#298028),(#298029,#298030),
(#298031,#298032),(#298033,#298034),(#298035,#298036),(#298037,#298038),
(#298039,#298040),(#298041,#298042),(#298043,#298044),(#298045,#298046),
(#298047,#298048),(#298049,#298050),(#298051,#298052),(#298053,#298054),
(#298055,#298056),(#298057,#298058),(#298059,#298060),(#298061,#298062),
(#298063,#298064),(#298065,#298066),(#298067,#298068),(#298069,#298070),
(#298071,#298072),(#298073,#298074),(#298075,#298076),(#298077,#298078),
(#298079,#298080),(#298081,#298082),(#298083,#298084),(#298085,#298086),
(#298087,#298088),(#298089,#298090),(#298091,#298092),(#298093,#298094),
(#298095,#298096),(#298097,#298098),(#298099,#298100),(#298101,#298102),
(#298103,#298104),(#298105,#298106),(#298107,#298108),(#298109,#298110),
(#298111,#298112),(#298113,#298114),(#298115,#298116),(#298117,#298118),
(#298119,#298120),(#298121,#298122),(#298123,#298124),(#298125,#298126),
(#298127,#298128),(#298129,#298130),(#298131,#298132),(#298133,#298134),
(#298135,#298136),(#298137,#298138),(#298139,#298140),(#298141,#298142),
(#298143,#298144),(#298145,#298146),(#298147,#298148),(#298149,#298150),
(#298151,#298152),(#298153,#298154),(#298155,#298156),(#298157,#298158),
(#298159,#298160),(#298161,#298162),(#298163,#298164),(#298165,#298166),
(#298167,#298168),(#298169,#298170),(#298171,#298172),(#298173,#298174),
(#298175,#298176),(#298177,#298178),(#298179,#298180),(#298181,#298182),
(#298183,#298184),(#298185,#298186),(#298187,#298188),(#298189,#298190),
(#298191,#298192),(#298193,#298194),(#298195,#298196),(#298197,#298198),
(#298199,#298200),(#298201,#298202),(#298203,#298204),(#298205,#298206),
(#298207,#298208),(#298209,#298210),(#298211,#298212),(#298213,#298214),
(#298215,#298216),(#298217,#298218),(#298219,#298220),(#298221,#298222),
(#298223,#298224),(#298225,#298226),(#298227,#298228),(#298229,#298230),
(#298231,#298232),(#298233,#298234),(#298235,#298236),(#298237,#298238),
(#298239,#298240),(#298241,#298242),(#298243,#298244),(#298245,#298246),
(#298247,#298248),(#298249,#298250),(#298251,#298252),(#298253,#298254),
(#298255,#298256),(#298257,#298258),(#298259,#298260),(#298261,#298262),
(#298263,#298264),(#298265,#298266),(#298267,#298268),(#298269,#298270),
(#298271,#298272),(#298273,#298274),(#298275,#298276),(#298277,#298278),
(#298279,#298280),(#298281,#298282),(#298283,#298284),(#298285,#298286),
(#298287,#298288),(#298289,#298290),(#298291,#298292),(#298293,#298294),
(#298295,#298296),(#298297,#298298),(#298299,#298300),(#298301,#298302),
(#298303,#298304),(#298305,#298306),(#298307,#298308),(#298309,#298310),
(#298311,#298312),(#298313,#298314),(#298315,#298316),(#298317,#298318),
(#298319,#298320),(#298321,#298322),(#298323,#298324),(#298325,#298326),
(#298327,#298328),(#298329,#298330),(#298331,#298332),(#298333,#298334),
(#298335,#298336),(#298337,#298338),(#298339,#298340),(#298341,#298342),
(#298343,#298344),(#298345,#298346),(#298347,#298348),(#298349,#298350),
(#298351,#298352),(#298353,#298354),(#298355,#298356),(#298357,#298358),
(#298359,#298360),(#298361,#298362),(#298363,#298364),(#298365,#298366),
(#298367,#298368),(#298369,#298370),(#298371,#298372),(#298373,#298374),
(#298375,#298376),(#298377,#298378),(#298379,#298380),(#298381,#298382),
(#298383,#298384),(#298385,#298386),(#298387,#298388),(#298389,#298390),
(#298391,#298392),(#298393,#298394),(#298395,#298396),(#298397,#298398),
(#298399,#298400),(#298401,#298402),(#298403,#298404),(#298405,#298406),
(#298407,#298408),(#298409,#298410),(#298411,#298412),(#298413,#298414),
(#298415,#298416),(#298417,#298418),(#298419,#298420),(#298421,#298422),
(#298423,#298424),(#298425,#298426),(#298427,#298428),(#298429,#298430),
(#298431,#298432),(#298433,#298434),(#298435,#298436),(#298437,#298438),
(#298439,#298440),(#298441,#298442),(#298443,#298444),(#298445,#298446),
(#298447,#298448),(#298449,#298450),(#298451,#298452),(#298453,#298454),
(#298455,#298456),(#298457,#298458)),.UNSPECIFIED.,.F.,.F.,.F.,(6,1,1,1,
1,1,1,1,1,1,1,1,1,1,1,1,1,1,1,1,1,1,1,1,1,1,1,1,1,1,1,1,1,1,1,1,1,1,1,1,
1,1,1,1,1,1,1,1,1,1,1,1,1,1,1,1,1,1,1,1,1,1,1,1,1,1,1,1,1,1,1,1,1,1,1,1,
1,1,1,1,1,1,1,1,1,1,1,1,1,1,1,1,1,1,1,1,1,1,1,1,1,1,1,1,1,1,1,1,1,1,1,1,
1,1,1,1,1,1,1,1,1,1,1,1,1,1,1,1,1,1,1,1,1,1,1,1,1,1,1,1,1,1,1,1,1,1,1,1,
1,1,1,1,1,1,1,1,1,1,1,1,1,1,1,1,1,1,1,1,1,1,1,1,1,1,1,1,1,1,1,1,1,1,1,1,
1,1,1,1,1,1,1,1,1,1,1,1,1,1,1,1,1,1,1,1,1,1,1,1,1,1,1,1,1,1,1,1,1,1,1,1,
1,1,1,1,1,1,1,1,1,1,1,1,1,1,1,1,1,1,1,1,1,1,1,1,1,1,1,1,1,1,1,1,1,1,1,1,
1,1,1,1,1,1,1,1,1,1,1,1,1,1,1,1,1,1,1,1,1,1,1,1,1,1,1,1,1,1,1,1,1,1,1,1,
1,1,1,1,1,1,1,1,1,1,1,1,1,1,1,1,1,1,1,1,1,1,1,1,1,1,1,1,1,1,1,1,1,1,1,1,
1,1,1,1,1,1,1,1,1,1,1,1,1,1,1,1,1,1,1,1,1,1,1,1,1,1,1,1,1,1,1,1,1,1,1,1,
1,1,1,1,1,1,1,1,1,1,1,1,1,1,1,1,1,1,1,1,1,1,1,1,1,1,1,1,1,1,1,1,1,1,1,1,
1,1,1,1,1,1,1,1,1,1,1,1,1,1,1,1,1,1,1,1,1,1,1,1,1,1,1,1,1,1,1,1,1,1,1,1,
1,1,1,1,1,1,1,1,1,1,1,1,1,1,1,1,1,1,1,1,1,1,1,1,1,1,1,1,1,1,1,6),(2,2),
(-1.,-0.998165138,-0.996330275,-0.994495413,-0.99266055,-0.990825688,-0.988990826,
-0.987155963,-0.985321101,-0.983486239,-0.981651376,-0.979816514,-0.977981651,
-0.976146789,-0.974311927,-0.972477064,-0.970642202,-0.968807339,-0.966972477,
-0.965137615,-0.963302752,-0.96146789,-0.959633028,-0.957798165,-0.955963303,
-0.95412844,-0.952293578,-0.950458716,-0.948623853,-0.946788991,-0.944954128,
-0.943119266,-0.941284404,-0.939449541,-0.937614679,-0.935779817,-0.933944954,
-0.932110092,-0.930275229,-0.928440367,-0.926605505,-0.924770642,-0.92293578,
-0.921100917,-0.919266055,-0.917431193,-0.91559633,-0.913761468,-0.911926606,
-0.910091743,-0.908256881,-0.906422018,-0.904587156,-0.902752294,-0.900917431,
-0.899082569,-0.897247706,-0.895412844,-0.893577982,-0.891743119,-0.889908257,
-0.888073394,-0.886238532,-0.88440367,-0.882568807,-0.880733945,-0.878899083,
-0.87706422,-0.875229358,-0.873394495,-0.871559633,-0.869724771,-0.867889908,
-0.866055046,-0.864220183,-0.862385321,-0.860550459,-0.858715596,-0.856880734,
-0.855045872,-0.853211009,-0.851376147,-0.849541284,-0.847706422,-0.84587156,
-0.844036697,-0.842201835,-0.840366972,-0.83853211,-0.836697248,-0.834862385,
-0.833027523,-0.831192661,-0.829357798,-0.827522936,-0.825688073,-0.823853211,
-0.822018349,-0.820183486,-0.818348624,-0.816513761,-0.814678899,-0.812844037,
-0.811009174,-0.809174312,-0.80733945,-0.805504587,-0.803669725,-0.801834862,
-0.8,-0.798165138,-0.796330275,-0.794495413,-0.79266055,-0.790825688,-0.788990826,
-0.787155963,-0.785321101,-0.783486239,-0.781651376,-0.779816514,-0.777981651,
-0.776146789,-0.774311927,-0.772477064,-0.770642202,-0.768807339,-0.766972477,
-0.765137615,-0.763302752,-0.76146789,-0.759633028,-0.757798165,-0.755963303,
-0.75412844,-0.752293578,-0.750458716,-0.748623853,-0.746788991,-0.744954128,
-0.743119266,-0.741284404,-0.739449541,-0.737614679,-0.735779817,-0.733944954,
-0.732110092,-0.730275229,-0.728440367,-0.726605505,-0.724770642,-0.72293578,
-0.721100917,-0.719266055,-0.717431193,-0.71559633,-0.713761468,-0.711926606,
-0.710091743,-0.708256881,-0.706422018,-0.704587156,-0.702752294,-0.700917431,
-0.699082569,-0.697247706,-0.695412844,-0.693577982,-0.691743119,-0.689908257,
-0.688073394,-0.686238532,-0.68440367,-0.682568807,-0.680733945,-0.678899083,
-0.67706422,-0.675229358,-0.673394495,-0.671559633,-0.669724771,-0.667889908,
-0.666055046,-0.664220183,-0.662385321,-0.660550459,-0.658715596,-0.656880734,
-0.655045872,-0.653211009,-0.651376147,-0.649541284,-0.647706422,-0.64587156,
-0.644036697,-0.642201835,-0.640366972,-0.63853211,-0.636697248,-0.634862385,
-0.633027523,-0.631192661,-0.629357798,-0.627522936,-0.625688073,-0.623853211,
-0.622018349,-0.620183486,-0.618348624,-0.616513761,-0.614678899,-0.612844037,
-0.611009174,-0.609174312,-0.60733945,-0.605504587,-0.603669725,-0.601834862,
-0.6,-0.598165138,-0.596330275,-0.594495413,-0.59266055,-0.590825688,-0.588990826,
-0.587155963,-0.585321101,-0.583486239,-0.581651376,-0.579816514,-0.577981651,
-0.576146789,-0.574311927,-0.572477064,-0.570642202,-0.568807339,-0.566972477,
-0.565137615,-0.563302752,-0.56146789,-0.559633028,-0.557798165,-0.555963303,
-0.55412844,-0.552293578,-0.550458716,-0.548623853,-0.546788991,-0.544954128,
-0.543119266,-0.541284404,-0.539449541,-0.537614679,-0.535779817,-0.533944954,
-0.532110092,-0.530275229,-0.528440367,-0.526605505,-0.524770642,-0.52293578,
-0.521100917,-0.519266055,-0.517431193,-0.51559633,-0.513761468,-0.511926606,
-0.510091743,-0.508256881,-0.506422018,-0.504587156,-0.502752294,-0.500917431,
-0.499082569,-0.497247706,-0.495412844,-0.493577982,-0.491743119,-0.489908257,
-0.488073394,-0.486238532,-0.48440367,-0.482568807,-0.480733945,-0.478899083,
-0.47706422,-0.475229358,-0.473394495,-0.471559633,-0.469724771,-0.467889908,
-0.466055046,-0.464220183,-0.462385321,-0.460550459,-0.458715596,-0.456880734,
-0.455045872,-0.453211009,-0.451376147,-0.449541284,-0.447706422,-0.44587156,
-0.444036697,-0.442201835,-0.440366972,-0.43853211,-0.436697248,-0.434862385,
-0.433027523,-0.431192661,-0.429357798,-0.427522936,-0.425688073,-0.423853211,
-0.422018349,-0.420183486,-0.418348624,-0.416513761,-0.414678899,-0.412844037,
-0.411009174,-0.409174312,-0.40733945,-0.405504587,-0.403669725,-0.401834862,
-0.4,-0.398165138,-0.396330275,-0.394495413,-0.39266055,-0.390825688,-0.388990826,
-0.387155963,-0.385321101,-0.383486239,-0.381651376,-0.379816514,-0.377981651,
-0.376146789,-0.374311927,-0.372477064,-0.370642202,-0.368807339,-0.366972477,
-0.365137615,-0.363302752,-0.36146789,-0.359633028,-0.357798165,-0.355963303,
-0.35412844,-0.352293578,-0.350458716,-0.348623853,-0.346788991,-0.344954128,
-0.343119266,-0.341284404,-0.339449541,-0.337614679,-0.335779817,-0.333944954,
-0.332110092,-0.330275229,-0.328440367,-0.326605505,-0.324770642,-0.32293578,
-0.321100917,-0.319266055,-0.317431193,-0.31559633,-0.313761468,-0.311926606,
-0.310091743,-0.308256881,-0.306422018,-0.304587156,-0.302752294,-0.300917431,
-0.299082569,-0.297247706,-0.295412844,-0.293577982,-0.291743119,-0.289908257,
-0.288073394,-0.286238532,-0.28440367,-0.282568807,-0.280733945,-0.278899083,
-0.27706422,-0.275229358,-0.273394495,-0.271559633,-0.269724771,-0.267889908,
-0.266055046,-0.264220183,-0.262385321,-0.260550459,-0.258715596,-0.256880734,
-0.255045872,-0.253211009,-0.251376147,-0.249541284,-0.247706422,-0.24587156,
-0.244036697,-0.242201835,-0.240366972,-0.23853211,-0.236697248,-0.234862385,
-0.233027523,-0.231192661,-0.229357798,-0.227522936,-0.225688073,-0.223853211,
-0.222018349,-0.220183486,-0.218348624,-0.216513761,-0.214678899,-0.212844037,
-0.211009174,-0.209174312,-0.20733945,-0.205504587,-0.203669725,-0.201834862,
-0.2,-0.198165138,-0.196330275,-0.194495413,-0.19266055,-0.190825688,-0.188990826,
-0.187155963,-0.185321101,-0.183486239,-0.181651376,-0.179816514,-0.177981651,
-0.176146789,-0.174311927,-0.172477064,-0.170642202,-0.168807339,-0.166972477,
-0.165137615,-0.163302752,-0.16146789,-0.159633028,-0.157798165,-0.155963303,
-0.15412844,-0.152293578,-0.150458716,-0.148623853,-0.146788991,-0.144954128,
-0.143172103),(0.,0.36),.UNSPECIFIED.);
#6302=B_SPLINE_SURFACE_WITH_KNOTS('',5,1,((#298930,#298931),(#298932,#298933),
(#298934,#298935),(#298936,#298937),(#298938,#298939),(#298940,#298941),
(#298942,#298943),(#298944,#298945),(#298946,#298947),(#298948,#298949),
(#298950,#298951),(#298952,#298953),(#298954,#298955),(#298956,#298957),
(#298958,#298959),(#298960,#298961),(#298962,#298963),(#298964,#298965),
(#298966,#298967),(#298968,#298969),(#298970,#298971),(#298972,#298973),
(#298974,#298975),(#298976,#298977),(#298978,#298979),(#298980,#298981),
(#298982,#298983),(#298984,#298985),(#298986,#298987),(#298988,#298989),
(#298990,#298991),(#298992,#298993),(#298994,#298995),(#298996,#298997),
(#298998,#298999),(#299000,#299001),(#299002,#299003),(#299004,#299005),
(#299006,#299007),(#299008,#299009),(#299010,#299011),(#299012,#299013),
(#299014,#299015),(#299016,#299017),(#299018,#299019),(#299020,#299021),
(#299022,#299023),(#299024,#299025),(#299026,#299027),(#299028,#299029),
(#299030,#299031),(#299032,#299033),(#299034,#299035),(#299036,#299037),
(#299038,#299039),(#299040,#299041),(#299042,#299043),(#299044,#299045),
(#299046,#299047),(#299048,#299049),(#299050,#299051),(#299052,#299053),
(#299054,#299055),(#299056,#299057),(#299058,#299059),(#299060,#299061),
(#299062,#299063),(#299064,#299065),(#299066,#299067),(#299068,#299069),
(#299070,#299071),(#299072,#299073),(#299074,#299075),(#299076,#299077),
(#299078,#299079),(#299080,#299081),(#299082,#299083),(#299084,#299085),
(#299086,#299087),(#299088,#299089),(#299090,#299091),(#299092,#299093),
(#299094,#299095),(#299096,#299097),(#299098,#299099),(#299100,#299101),
(#299102,#299103),(#299104,#299105),(#299106,#299107),(#299108,#299109),
(#299110,#299111),(#299112,#299113),(#299114,#299115),(#299116,#299117),
(#299118,#299119),(#299120,#299121),(#299122,#299123),(#299124,#299125),
(#299126,#299127),(#299128,#299129),(#299130,#299131),(#299132,#299133),
(#299134,#299135),(#299136,#299137),(#299138,#299139),(#299140,#299141),
(#299142,#299143),(#299144,#299145),(#299146,#299147),(#299148,#299149),
(#299150,#299151),(#299152,#299153),(#299154,#299155),(#299156,#299157),
(#299158,#299159),(#299160,#299161),(#299162,#299163),(#299164,#299165),
(#299166,#299167),(#299168,#299169),(#299170,#299171),(#299172,#299173),
(#299174,#299175),(#299176,#299177),(#299178,#299179),(#299180,#299181),
(#299182,#299183),(#299184,#299185),(#299186,#299187),(#299188,#299189),
(#299190,#299191),(#299192,#299193),(#299194,#299195),(#299196,#299197),
(#299198,#299199),(#299200,#299201),(#299202,#299203),(#299204,#299205),
(#299206,#299207),(#299208,#299209),(#299210,#299211),(#299212,#299213),
(#299214,#299215),(#299216,#299217),(#299218,#299219),(#299220,#299221),
(#299222,#299223),(#299224,#299225),(#299226,#299227),(#299228,#299229),
(#299230,#299231),(#299232,#299233),(#299234,#299235),(#299236,#299237),
(#299238,#299239),(#299240,#299241),(#299242,#299243),(#299244,#299245),
(#299246,#299247),(#299248,#299249),(#299250,#299251),(#299252,#299253),
(#299254,#299255),(#299256,#299257),(#299258,#299259),(#299260,#299261),
(#299262,#299263),(#299264,#299265),(#299266,#299267),(#299268,#299269),
(#299270,#299271),(#299272,#299273),(#299274,#299275),(#299276,#299277),
(#299278,#299279),(#299280,#299281),(#299282,#299283),(#299284,#299285),
(#299286,#299287),(#299288,#299289),(#299290,#299291),(#299292,#299293),
(#299294,#299295),(#299296,#299297),(#299298,#299299),(#299300,#299301),
(#299302,#299303),(#299304,#299305),(#299306,#299307),(#299308,#299309),
(#299310,#299311),(#299312,#299313),(#299314,#299315),(#299316,#299317),
(#299318,#299319),(#299320,#299321),(#299322,#299323),(#299324,#299325),
(#299326,#299327),(#299328,#299329),(#299330,#299331),(#299332,#299333),
(#299334,#299335),(#299336,#299337),(#299338,#299339),(#299340,#299341),
(#299342,#299343),(#299344,#299345),(#299346,#299347),(#299348,#299349),
(#299350,#299351),(#299352,#299353),(#299354,#299355),(#299356,#299357),
(#299358,#299359),(#299360,#299361),(#299362,#299363),(#299364,#299365),
(#299366,#299367),(#299368,#299369),(#299370,#299371),(#299372,#299373),
(#299374,#299375),(#299376,#299377),(#299378,#299379),(#299380,#299381),
(#299382,#299383),(#299384,#299385),(#299386,#299387),(#299388,#299389),
(#299390,#299391),(#299392,#299393),(#299394,#299395),(#299396,#299397),
(#299398,#299399),(#299400,#299401),(#299402,#299403),(#299404,#299405),
(#299406,#299407),(#299408,#299409),(#299410,#299411),(#299412,#299413),
(#299414,#299415),(#299416,#299417),(#299418,#299419),(#299420,#299421),
(#299422,#299423),(#299424,#299425),(#299426,#299427),(#299428,#299429),
(#299430,#299431),(#299432,#299433),(#299434,#299435),(#299436,#299437),
(#299438,#299439),(#299440,#299441),(#299442,#299443),(#299444,#299445),
(#299446,#299447),(#299448,#299449),(#299450,#299451),(#299452,#299453),
(#299454,#299455),(#299456,#299457),(#299458,#299459),(#299460,#299461),
(#299462,#299463),(#299464,#299465),(#299466,#299467),(#299468,#299469),
(#299470,#299471),(#299472,#299473),(#299474,#299475),(#299476,#299477),
(#299478,#299479),(#299480,#299481),(#299482,#299483),(#299484,#299485),
(#299486,#299487),(#299488,#299489),(#299490,#299491),(#299492,#299493),
(#299494,#299495),(#299496,#299497),(#299498,#299499),(#299500,#299501),
(#299502,#299503),(#299504,#299505),(#299506,#299507),(#299508,#299509),
(#299510,#299511),(#299512,#299513),(#299514,#299515),(#299516,#299517),
(#299518,#299519),(#299520,#299521),(#299522,#299523),(#299524,#299525),
(#299526,#299527),(#299528,#299529),(#299530,#299531),(#299532,#299533),
(#299534,#299535),(#299536,#299537),(#299538,#299539),(#299540,#299541),
(#299542,#299543),(#299544,#299545),(#299546,#299547),(#299548,#299549),
(#299550,#299551),(#299552,#299553),(#299554,#299555),(#299556,#299557),
(#299558,#299559),(#299560,#299561),(#299562,#299563),(#299564,#299565),
(#299566,#299567),(#299568,#299569),(#299570,#299571),(#299572,#299573),
(#299574,#299575),(#299576,#299577),(#299578,#299579),(#299580,#299581),
(#299582,#299583),(#299584,#299585),(#299586,#299587),(#299588,#299589),
(#299590,#299591),(#299592,#299593),(#299594,#299595),(#299596,#299597),
(#299598,#299599),(#299600,#299601),(#299602,#299603),(#299604,#299605),
(#299606,#299607),(#299608,#299609),(#299610,#299611),(#299612,#299613),
(#299614,#299615),(#299616,#299617),(#299618,#299619),(#299620,#299621),
(#299622,#299623),(#299624,#299625),(#299626,#299627),(#299628,#299629),
(#299630,#299631),(#299632,#299633),(#299634,#299635),(#299636,#299637),
(#299638,#299639),(#299640,#299641),(#299642,#299643),(#299644,#299645),
(#299646,#299647),(#299648,#299649),(#299650,#299651),(#299652,#299653),
(#299654,#299655),(#299656,#299657),(#299658,#299659),(#299660,#299661),
(#299662,#299663),(#299664,#299665),(#299666,#299667),(#299668,#299669),
(#299670,#299671),(#299672,#299673),(#299674,#299675),(#299676,#299677),
(#299678,#299679),(#299680,#299681),(#299682,#299683),(#299684,#299685),
(#299686,#299687),(#299688,#299689),(#299690,#299691),(#299692,#299693),
(#299694,#299695),(#299696,#299697),(#299698,#299699),(#299700,#299701),
(#299702,#299703),(#299704,#299705),(#299706,#299707),(#299708,#299709),
(#299710,#299711),(#299712,#299713),(#299714,#299715),(#299716,#299717),
(#299718,#299719),(#299720,#299721),(#299722,#299723),(#299724,#299725),
(#299726,#299727),(#299728,#299729),(#299730,#299731),(#299732,#299733),
(#299734,#299735),(#299736,#299737),(#299738,#299739),(#299740,#299741),
(#299742,#299743),(#299744,#299745),(#299746,#299747),(#299748,#299749),
(#299750,#299751),(#299752,#299753),(#299754,#299755),(#299756,#299757),
(#299758,#299759),(#299760,#299761),(#299762,#299763),(#299764,#299765),
(#299766,#299767),(#299768,#299769),(#299770,#299771),(#299772,#299773),
(#299774,#299775),(#299776,#299777),(#299778,#299779),(#299780,#299781),
(#299782,#299783),(#299784,#299785),(#299786,#299787),(#299788,#299789),
(#299790,#299791),(#299792,#299793),(#299794,#299795),(#299796,#299797),
(#299798,#299799),(#299800,#299801),(#299802,#299803),(#299804,#299805),
(#299806,#299807),(#299808,#299809),(#299810,#299811),(#299812,#299813),
(#299814,#299815),(#299816,#299817),(#299818,#299819),(#299820,#299821),
(#299822,#299823),(#299824,#299825),(#299826,#299827),(#299828,#299829),
(#299830,#299831),(#299832,#299833),(#299834,#299835),(#299836,#299837),
(#299838,#299839),(#299840,#299841),(#299842,#299843),(#299844,#299845),
(#299846,#299847),(#299848,#299849),(#299850,#299851),(#299852,#299853),
(#299854,#299855),(#299856,#299857),(#299858,#299859),(#299860,#299861),
(#299862,#299863),(#299864,#299865),(#299866,#299867),(#299868,#299869),
(#299870,#299871),(#299872,#299873)),.UNSPECIFIED.,.F.,.F.,.F.,(6,1,1,1,
1,1,1,1,1,1,1,1,1,1,1,1,1,1,1,1,1,1,1,1,1,1,1,1,1,1,1,1,1,1,1,1,1,1,1,1,
1,1,1,1,1,1,1,1,1,1,1,1,1,1,1,1,1,1,1,1,1,1,1,1,1,1,1,1,1,1,1,1,1,1,1,1,
1,1,1,1,1,1,1,1,1,1,1,1,1,1,1,1,1,1,1,1,1,1,1,1,1,1,1,1,1,1,1,1,1,1,1,1,
1,1,1,1,1,1,1,1,1,1,1,1,1,1,1,1,1,1,1,1,1,1,1,1,1,1,1,1,1,1,1,1,1,1,1,1,
1,1,1,1,1,1,1,1,1,1,1,1,1,1,1,1,1,1,1,1,1,1,1,1,1,1,1,1,1,1,1,1,1,1,1,1,
1,1,1,1,1,1,1,1,1,1,1,1,1,1,1,1,1,1,1,1,1,1,1,1,1,1,1,1,1,1,1,1,1,1,1,1,
1,1,1,1,1,1,1,1,1,1,1,1,1,1,1,1,1,1,1,1,1,1,1,1,1,1,1,1,1,1,1,1,1,1,1,1,
1,1,1,1,1,1,1,1,1,1,1,1,1,1,1,1,1,1,1,1,1,1,1,1,1,1,1,1,1,1,1,1,1,1,1,1,
1,1,1,1,1,1,1,1,1,1,1,1,1,1,1,1,1,1,1,1,1,1,1,1,1,1,1,1,1,1,1,1,1,1,1,1,
1,1,1,1,1,1,1,1,1,1,1,1,1,1,1,1,1,1,1,1,1,1,1,1,1,1,1,1,1,1,1,1,1,1,1,1,
1,1,1,1,1,1,1,1,1,1,1,1,1,1,1,1,1,1,1,1,1,1,1,1,1,1,1,1,1,1,1,1,1,1,1,1,
1,1,1,1,1,1,1,1,1,1,1,1,1,1,1,1,1,1,1,1,1,1,1,1,1,1,1,1,1,1,1,1,1,1,1,1,
1,1,1,1,1,1,1,1,1,1,1,1,1,1,1,1,1,1,1,1,1,1,1,1,1,1,1,1,1,1,1,6),(2,2),
(0.143172104,0.144954128,0.146788991,0.148623853,0.150458716,0.152293578,
0.15412844,0.155963303,0.157798165,0.159633028,0.16146789,0.163302752,0.165137615,
0.166972477,0.168807339,0.170642202,0.172477064,0.174311927,0.176146789,
0.177981651,0.179816514,0.181651376,0.183486239,0.185321101,0.187155963,
0.188990826,0.190825688,0.19266055,0.194495413,0.196330275,0.198165138,
0.2,0.201834862,0.203669725,0.205504587,0.20733945,0.209174312,0.211009174,
0.212844037,0.214678899,0.216513761,0.218348624,0.220183486,0.222018349,
0.223853211,0.225688073,0.227522936,0.229357798,0.231192661,0.233027523,
0.234862385,0.236697248,0.23853211,0.240366972,0.242201835,0.244036697,
0.24587156,0.247706422,0.249541284,0.251376147,0.253211009,0.255045872,
0.256880734,0.258715596,0.260550459,0.262385321,0.264220183,0.266055046,
0.267889908,0.269724771,0.271559633,0.273394495,0.275229358,0.27706422,
0.278899083,0.280733945,0.282568807,0.28440367,0.286238532,0.288073394,
0.289908257,0.291743119,0.293577982,0.295412844,0.297247706,0.299082569,
0.300917431,0.302752294,0.304587156,0.306422018,0.308256881,0.310091743,
0.311926606,0.313761468,0.31559633,0.317431193,0.319266055,0.321100917,
0.32293578,0.324770642,0.326605505,0.328440367,0.330275229,0.332110092,
0.333944954,0.335779817,0.337614679,0.339449541,0.341284404,0.343119266,
0.344954128,0.346788991,0.348623853,0.350458716,0.352293578,0.35412844,
0.355963303,0.357798165,0.359633028,0.36146789,0.363302752,0.365137615,
0.366972477,0.368807339,0.370642202,0.372477064,0.374311927,0.376146789,
0.377981651,0.379816514,0.381651376,0.383486239,0.385321101,0.387155963,
0.388990826,0.390825688,0.39266055,0.394495413,0.396330275,0.398165138,
0.4,0.401834862,0.403669725,0.405504587,0.40733945,0.409174312,0.411009174,
0.412844037,0.414678899,0.416513761,0.418348624,0.420183486,0.422018349,
0.423853211,0.425688073,0.427522936,0.429357798,0.431192661,0.433027523,
0.434862385,0.436697248,0.43853211,0.440366972,0.442201835,0.444036697,
0.44587156,0.447706422,0.449541284,0.451376147,0.453211009,0.455045872,
0.456880734,0.458715596,0.460550459,0.462385321,0.464220183,0.466055046,
0.467889908,0.469724771,0.471559633,0.473394495,0.475229358,0.47706422,
0.478899083,0.480733945,0.482568807,0.48440367,0.486238532,0.488073394,
0.489908257,0.491743119,0.493577982,0.495412844,0.497247706,0.499082569,
0.500917431,0.502752294,0.504587156,0.506422018,0.508256881,0.510091743,
0.511926606,0.513761468,0.51559633,0.517431193,0.519266055,0.521100917,
0.52293578,0.524770642,0.526605505,0.528440367,0.530275229,0.532110092,
0.533944954,0.535779817,0.537614679,0.539449541,0.541284404,0.543119266,
0.544954128,0.546788991,0.548623853,0.550458716,0.552293578,0.55412844,
0.555963303,0.557798165,0.559633028,0.56146789,0.563302752,0.565137615,
0.566972477,0.568807339,0.570642202,0.572477064,0.574311927,0.576146789,
0.577981651,0.579816514,0.581651376,0.583486239,0.585321101,0.587155963,
0.588990826,0.590825688,0.59266055,0.594495413,0.596330275,0.598165138,
0.6,0.601834862,0.603669725,0.605504587,0.60733945,0.609174312,0.611009174,
0.612844037,0.614678899,0.616513761,0.618348624,0.620183486,0.622018349,
0.623853211,0.625688073,0.627522936,0.629357798,0.631192661,0.633027523,
0.634862385,0.636697248,0.63853211,0.640366972,0.642201835,0.644036697,
0.64587156,0.647706422,0.649541284,0.651376147,0.653211009,0.655045872,
0.656880734,0.658715596,0.660550459,0.662385321,0.664220183,0.666055046,
0.667889908,0.669724771,0.671559633,0.673394495,0.675229358,0.67706422,
0.678899083,0.680733945,0.682568807,0.68440367,0.686238532,0.688073394,
0.689908257,0.691743119,0.693577982,0.695412844,0.697247706,0.699082569,
0.700917431,0.702752294,0.704587156,0.706422018,0.708256881,0.710091743,
0.711926606,0.713761468,0.71559633,0.717431193,0.719266055,0.721100917,
0.72293578,0.724770642,0.726605505,0.728440367,0.730275229,0.732110092,
0.733944954,0.735779817,0.737614679,0.739449541,0.741284404,0.743119266,
0.744954128,0.746788991,0.748623853,0.750458716,0.752293578,0.75412844,
0.755963303,0.757798165,0.759633028,0.76146789,0.763302752,0.765137615,
0.766972477,0.768807339,0.770642202,0.772477064,0.774311927,0.776146789,
0.777981651,0.779816514,0.781651376,0.783486239,0.785321101,0.787155963,
0.788990826,0.790825688,0.79266055,0.794495413,0.796330275,0.798165138,
0.8,0.801834862,0.803669725,0.805504587,0.80733945,0.809174312,0.811009174,
0.812844037,0.814678899,0.816513761,0.818348624,0.820183486,0.822018349,
0.823853211,0.825688073,0.827522936,0.829357798,0.831192661,0.833027523,
0.834862385,0.836697248,0.83853211,0.840366972,0.842201835,0.844036697,
0.84587156,0.847706422,0.849541284,0.851376147,0.853211009,0.855045872,
0.856880734,0.858715596,0.860550459,0.862385321,0.864220183,0.866055046,
0.867889908,0.869724771,0.871559633,0.873394495,0.875229358,0.87706422,
0.878899083,0.880733945,0.882568807,0.88440367,0.886238532,0.888073394,
0.889908257,0.891743119,0.893577982,0.895412844,0.897247706,0.899082569,
0.900917431,0.902752294,0.904587156,0.906422018,0.908256881,0.910091743,
0.911926606,0.913761468,0.91559633,0.917431193,0.919266055,0.921100917,
0.92293578,0.924770642,0.926605505,0.928440367,0.930275229,0.932110092,
0.933944954,0.935779817,0.937614679,0.939449541,0.941284404,0.943119266,
0.944954128,0.946788991,0.948623853,0.950458716,0.952293578,0.95412844,
0.955963303,0.957798165,0.959633028,0.96146789,0.963302752,0.965137615,
0.966972477,0.968807339,0.970642202,0.972477064,0.974311927,0.976146789,
0.977981651,0.979816514,0.981651376,0.983486239,0.985321101,0.987155963,
0.988990826,0.990825688,0.99266055,0.994495413,0.996330275,0.998165138,
1.),(0.,0.36),.UNSPECIFIED.);
#6303=B_SPLINE_SURFACE_WITH_KNOTS('',5,1,((#301296,#301297,#301298),(#301299,
#301300,#301301),(#301302,#301303,#301304),(#301305,#301306,#301307),(#301308,
#301309,#301310),(#301311,#301312,#301313),(#301314,#301315,#301316),(#301317,
#301318,#301319),(#301320,#301321,#301322),(#301323,#301324,#301325),(#301326,
#301327,#301328),(#301329,#301330,#301331),(#301332,#301333,#301334),(#301335,
#301336,#301337),(#301338,#301339,#301340),(#301341,#301342,#301343),(#301344,
#301345,#301346),(#301347,#301348,#301349),(#301350,#301351,#301352),(#301353,
#301354,#301355),(#301356,#301357,#301358),(#301359,#301360,#301361),(#301362,
#301363,#301364),(#301365,#301366,#301367),(#301368,#301369,#301370),(#301371,
#301372,#301373),(#301374,#301375,#301376),(#301377,#301378,#301379),(#301380,
#301381,#301382),(#301383,#301384,#301385),(#301386,#301387,#301388),(#301389,
#301390,#301391),(#301392,#301393,#301394),(#301395,#301396,#301397),(#301398,
#301399,#301400),(#301401,#301402,#301403),(#301404,#301405,#301406),(#301407,
#301408,#301409),(#301410,#301411,#301412),(#301413,#301414,#301415),(#301416,
#301417,#301418),(#301419,#301420,#301421),(#301422,#301423,#301424),(#301425,
#301426,#301427),(#301428,#301429,#301430),(#301431,#301432,#301433),(#301434,
#301435,#301436),(#301437,#301438,#301439),(#301440,#301441,#301442),(#301443,
#301444,#301445),(#301446,#301447,#301448),(#301449,#301450,#301451),(#301452,
#301453,#301454),(#301455,#301456,#301457),(#301458,#301459,#301460),(#301461,
#301462,#301463),(#301464,#301465,#301466),(#301467,#301468,#301469),(#301470,
#301471,#301472),(#301473,#301474,#301475),(#301476,#301477,#301478),(#301479,
#301480,#301481),(#301482,#301483,#301484),(#301485,#301486,#301487),(#301488,
#301489,#301490),(#301491,#301492,#301493),(#301494,#301495,#301496),(#301497,
#301498,#301499),(#301500,#301501,#301502),(#301503,#301504,#301505),(#301506,
#301507,#301508),(#301509,#301510,#301511),(#301512,#301513,#301514),(#301515,
#301516,#301517),(#301518,#301519,#301520),(#301521,#301522,#301523),(#301524,
#301525,#301526),(#301527,#301528,#301529),(#301530,#301531,#301532),(#301533,
#301534,#301535),(#301536,#301537,#301538),(#301539,#301540,#301541),(#301542,
#301543,#301544),(#301545,#301546,#301547),(#301548,#301549,#301550),(#301551,
#301552,#301553),(#301554,#301555,#301556),(#301557,#301558,#301559),(#301560,
#301561,#301562),(#301563,#301564,#301565),(#301566,#301567,#301568),(#301569,
#301570,#301571),(#301572,#301573,#301574),(#301575,#301576,#301577),(#301578,
#301579,#301580),(#301581,#301582,#301583),(#301584,#301585,#301586),(#301587,
#301588,#301589),(#301590,#301591,#301592),(#301593,#301594,#301595),(#301596,
#301597,#301598),(#301599,#301600,#301601),(#301602,#301603,#301604),(#301605,
#301606,#301607),(#301608,#301609,#301610),(#301611,#301612,#301613),(#301614,
#301615,#301616),(#301617,#301618,#301619),(#301620,#301621,#301622),(#301623,
#301624,#301625),(#301626,#301627,#301628),(#301629,#301630,#301631),(#301632,
#301633,#301634),(#301635,#301636,#301637),(#301638,#301639,#301640),(#301641,
#301642,#301643),(#301644,#301645,#301646),(#301647,#301648,#301649),(#301650,
#301651,#301652),(#301653,#301654,#301655),(#301656,#301657,#301658),(#301659,
#301660,#301661),(#301662,#301663,#301664),(#301665,#301666,#301667),(#301668,
#301669,#301670),(#301671,#301672,#301673),(#301674,#301675,#301676),(#301677,
#301678,#301679),(#301680,#301681,#301682),(#301683,#301684,#301685),(#301686,
#301687,#301688),(#301689,#301690,#301691),(#301692,#301693,#301694),(#301695,
#301696,#301697),(#301698,#301699,#301700),(#301701,#301702,#301703),(#301704,
#301705,#301706),(#301707,#301708,#301709),(#301710,#301711,#301712),(#301713,
#301714,#301715),(#301716,#301717,#301718),(#301719,#301720,#301721),(#301722,
#301723,#301724),(#301725,#301726,#301727),(#301728,#301729,#301730),(#301731,
#301732,#301733),(#301734,#301735,#301736),(#301737,#301738,#301739),(#301740,
#301741,#301742),(#301743,#301744,#301745),(#301746,#301747,#301748),(#301749,
#301750,#301751),(#301752,#301753,#301754),(#301755,#301756,#301757),(#301758,
#301759,#301760),(#301761,#301762,#301763),(#301764,#301765,#301766),(#301767,
#301768,#301769),(#301770,#301771,#301772),(#301773,#301774,#301775),(#301776,
#301777,#301778),(#301779,#301780,#301781),(#301782,#301783,#301784),(#301785,
#301786,#301787),(#301788,#301789,#301790),(#301791,#301792,#301793),(#301794,
#301795,#301796),(#301797,#301798,#301799),(#301800,#301801,#301802),(#301803,
#301804,#301805),(#301806,#301807,#301808),(#301809,#301810,#301811),(#301812,
#301813,#301814),(#301815,#301816,#301817),(#301818,#301819,#301820),(#301821,
#301822,#301823),(#301824,#301825,#301826),(#301827,#301828,#301829),(#301830,
#301831,#301832),(#301833,#301834,#301835),(#301836,#301837,#301838),(#301839,
#301840,#301841),(#301842,#301843,#301844),(#301845,#301846,#301847),(#301848,
#301849,#301850),(#301851,#301852,#301853),(#301854,#301855,#301856),(#301857,
#301858,#301859),(#301860,#301861,#301862),(#301863,#301864,#301865),(#301866,
#301867,#301868),(#301869,#301870,#301871),(#301872,#301873,#301874),(#301875,
#301876,#301877),(#301878,#301879,#301880),(#301881,#301882,#301883),(#301884,
#301885,#301886),(#301887,#301888,#301889),(#301890,#301891,#301892),(#301893,
#301894,#301895),(#301896,#301897,#301898),(#301899,#301900,#301901),(#301902,
#301903,#301904),(#301905,#301906,#301907),(#301908,#301909,#301910),(#301911,
#301912,#301913),(#301914,#301915,#301916),(#301917,#301918,#301919),(#301920,
#301921,#301922),(#301923,#301924,#301925),(#301926,#301927,#301928),(#301929,
#301930,#301931),(#301932,#301933,#301934),(#301935,#301936,#301937),(#301938,
#301939,#301940),(#301941,#301942,#301943),(#301944,#301945,#301946),(#301947,
#301948,#301949),(#301950,#301951,#301952),(#301953,#301954,#301955),(#301956,
#301957,#301958),(#301959,#301960,#301961),(#301962,#301963,#301964),(#301965,
#301966,#301967),(#301968,#301969,#301970),(#301971,#301972,#301973),(#301974,
#301975,#301976),(#301977,#301978,#301979),(#301980,#301981,#301982),(#301983,
#301984,#301985),(#301986,#301987,#301988),(#301989,#301990,#301991),(#301992,
#301993,#301994),(#301995,#301996,#301997),(#301998,#301999,#302000),(#302001,
#302002,#302003),(#302004,#302005,#302006),(#302007,#302008,#302009),(#302010,
#302011,#302012),(#302013,#302014,#302015),(#302016,#302017,#302018),(#302019,
#302020,#302021),(#302022,#302023,#302024),(#302025,#302026,#302027),(#302028,
#302029,#302030),(#302031,#302032,#302033),(#302034,#302035,#302036),(#302037,
#302038,#302039),(#302040,#302041,#302042),(#302043,#302044,#302045),(#302046,
#302047,#302048),(#302049,#302050,#302051),(#302052,#302053,#302054),(#302055,
#302056,#302057),(#302058,#302059,#302060),(#302061,#302062,#302063),(#302064,
#302065,#302066),(#302067,#302068,#302069),(#302070,#302071,#302072),(#302073,
#302074,#302075),(#302076,#302077,#302078),(#302079,#302080,#302081),(#302082,
#302083,#302084),(#302085,#302086,#302087),(#302088,#302089,#302090),(#302091,
#302092,#302093),(#302094,#302095,#302096),(#302097,#302098,#302099),(#302100,
#302101,#302102),(#302103,#302104,#302105),(#302106,#302107,#302108),(#302109,
#302110,#302111),(#302112,#302113,#302114),(#302115,#302116,#302117),(#302118,
#302119,#302120),(#302121,#302122,#302123),(#302124,#302125,#302126),(#302127,
#302128,#302129),(#302130,#302131,#302132),(#302133,#302134,#302135),(#302136,
#302137,#302138),(#302139,#302140,#302141),(#302142,#302143,#302144),(#302145,
#302146,#302147),(#302148,#302149,#302150),(#302151,#302152,#302153),(#302154,
#302155,#302156),(#302157,#302158,#302159),(#302160,#302161,#302162),(#302163,
#302164,#302165),(#302166,#302167,#302168),(#302169,#302170,#302171),(#302172,
#302173,#302174),(#302175,#302176,#302177),(#302178,#302179,#302180),(#302181,
#302182,#302183),(#302184,#302185,#302186),(#302187,#302188,#302189),(#302190,
#302191,#302192),(#302193,#302194,#302195),(#302196,#302197,#302198),(#302199,
#302200,#302201),(#302202,#302203,#302204),(#302205,#302206,#302207),(#302208,
#302209,#302210),(#302211,#302212,#302213),(#302214,#302215,#302216),(#302217,
#302218,#302219),(#302220,#302221,#302222),(#302223,#302224,#302225),(#302226,
#302227,#302228),(#302229,#302230,#302231),(#302232,#302233,#302234),(#302235,
#302236,#302237),(#302238,#302239,#302240),(#302241,#302242,#302243),(#302244,
#302245,#302246),(#302247,#302248,#302249),(#302250,#302251,#302252),(#302253,
#302254,#302255),(#302256,#302257,#302258),(#302259,#302260,#302261),(#302262,
#302263,#302264),(#302265,#302266,#302267),(#302268,#302269,#302270),(#302271,
#302272,#302273),(#302274,#302275,#302276),(#302277,#302278,#302279),(#302280,
#302281,#302282),(#302283,#302284,#302285),(#302286,#302287,#302288),(#302289,
#302290,#302291),(#302292,#302293,#302294),(#302295,#302296,#302297),(#302298,
#302299,#302300),(#302301,#302302,#302303),(#302304,#302305,#302306),(#302307,
#302308,#302309),(#302310,#302311,#302312),(#302313,#302314,#302315),(#302316,
#302317,#302318),(#302319,#302320,#302321),(#302322,#302323,#302324),(#302325,
#302326,#302327),(#302328,#302329,#302330),(#302331,#302332,#302333),(#302334,
#302335,#302336),(#302337,#302338,#302339),(#302340,#302341,#302342),(#302343,
#302344,#302345),(#302346,#302347,#302348),(#302349,#302350,#302351),(#302352,
#302353,#302354),(#302355,#302356,#302357),(#302358,#302359,#302360),(#302361,
#302362,#302363),(#302364,#302365,#302366),(#302367,#302368,#302369),(#302370,
#302371,#302372),(#302373,#302374,#302375),(#302376,#302377,#302378),(#302379,
#302380,#302381),(#302382,#302383,#302384),(#302385,#302386,#302387),(#302388,
#302389,#302390),(#302391,#302392,#302393),(#302394,#302395,#302396),(#302397,
#302398,#302399),(#302400,#302401,#302402),(#302403,#302404,#302405),(#302406,
#302407,#302408),(#302409,#302410,#302411),(#302412,#302413,#302414),(#302415,
#302416,#302417),(#302418,#302419,#302420),(#302421,#302422,#302423),(#302424,
#302425,#302426),(#302427,#302428,#302429),(#302430,#302431,#302432),(#302433,
#302434,#302435),(#302436,#302437,#302438),(#302439,#302440,#302441),(#302442,
#302443,#302444),(#302445,#302446,#302447),(#302448,#302449,#302450),(#302451,
#302452,#302453),(#302454,#302455,#302456),(#302457,#302458,#302459),(#302460,
#302461,#302462),(#302463,#302464,#302465),(#302466,#302467,#302468),(#302469,
#302470,#302471),(#302472,#302473,#302474),(#302475,#302476,#302477),(#302478,
#302479,#302480),(#302481,#302482,#302483),(#302484,#302485,#302486),(#302487,
#302488,#302489),(#302490,#302491,#302492),(#302493,#302494,#302495),(#302496,
#302497,#302498),(#302499,#302500,#302501),(#302502,#302503,#302504),(#302505,
#302506,#302507),(#302508,#302509,#302510),(#302511,#302512,#302513),(#302514,
#302515,#302516),(#302517,#302518,#302519),(#302520,#302521,#302522),(#302523,
#302524,#302525),(#302526,#302527,#302528),(#302529,#302530,#302531),(#302532,
#302533,#302534),(#302535,#302536,#302537),(#302538,#302539,#302540),(#302541,
#302542,#302543),(#302544,#302545,#302546),(#302547,#302548,#302549),(#302550,
#302551,#302552),(#302553,#302554,#302555),(#302556,#302557,#302558),(#302559,
#302560,#302561),(#302562,#302563,#302564),(#302565,#302566,#302567),(#302568,
#302569,#302570),(#302571,#302572,#302573),(#302574,#302575,#302576),(#302577,
#302578,#302579),(#302580,#302581,#302582),(#302583,#302584,#302585),(#302586,
#302587,#302588),(#302589,#302590,#302591),(#302592,#302593,#302594),(#302595,
#302596,#302597),(#302598,#302599,#302600),(#302601,#302602,#302603),(#302604,
#302605,#302606),(#302607,#302608,#302609),(#302610,#302611,#302612),(#302613,
#302614,#302615),(#302616,#302617,#302618),(#302619,#302620,#302621),(#302622,
#302623,#302624),(#302625,#302626,#302627),(#302628,#302629,#302630),(#302631,
#302632,#302633),(#302634,#302635,#302636),(#302637,#302638,#302639),(#302640,
#302641,#302642),(#302643,#302644,#302645),(#302646,#302647,#302648),(#302649,
#302650,#302651),(#302652,#302653,#302654),(#302655,#302656,#302657),(#302658,
#302659,#302660),(#302661,#302662,#302663),(#302664,#302665,#302666),(#302667,
#302668,#302669),(#302670,#302671,#302672),(#302673,#302674,#302675),(#302676,
#302677,#302678),(#302679,#302680,#302681),(#302682,#302683,#302684),(#302685,
#302686,#302687),(#302688,#302689,#302690),(#302691,#302692,#302693),(#302694,
#302695,#302696),(#302697,#302698,#302699),(#302700,#302701,#302702),(#302703,
#302704,#302705),(#302706,#302707,#302708),(#302709,#302710,#302711),(#302712,
#302713,#302714),(#302715,#302716,#302717),(#302718,#302719,#302720),(#302721,
#302722,#302723),(#302724,#302725,#302726),(#302727,#302728,#302729),(#302730,
#302731,#302732),(#302733,#302734,#302735),(#302736,#302737,#302738),(#302739,
#302740,#302741),(#302742,#302743,#302744),(#302745,#302746,#302747),(#302748,
#302749,#302750),(#302751,#302752,#302753),(#302754,#302755,#302756),(#302757,
#302758,#302759),(#302760,#302761,#302762),(#302763,#302764,#302765),(#302766,
#302767,#302768),(#302769,#302770,#302771),(#302772,#302773,#302774),(#302775,
#302776,#302777),(#302778,#302779,#302780),(#302781,#302782,#302783),(#302784,
#302785,#302786),(#302787,#302788,#302789),(#302790,#302791,#302792),(#302793,
#302794,#302795),(#302796,#302797,#302798),(#302799,#302800,#302801),(#302802,
#302803,#302804),(#302805,#302806,#302807),(#302808,#302809,#302810),(#302811,
#302812,#302813),(#302814,#302815,#302816),(#302817,#302818,#302819),(#302820,
#302821,#302822),(#302823,#302824,#302825),(#302826,#302827,#302828),(#302829,
#302830,#302831),(#302832,#302833,#302834),(#302835,#302836,#302837),(#302838,
#302839,#302840),(#302841,#302842,#302843),(#302844,#302845,#302846),(#302847,
#302848,#302849),(#302850,#302851,#302852),(#302853,#302854,#302855),(#302856,
#302857,#302858),(#302859,#302860,#302861),(#302862,#302863,#302864),(#302865,
#302866,#302867),(#302868,#302869,#302870),(#302871,#302872,#302873),(#302874,
#302875,#302876),(#302877,#302878,#302879),(#302880,#302881,#302882),(#302883,
#302884,#302885),(#302886,#302887,#302888),(#302889,#302890,#302891),(#302892,
#302893,#302894),(#302895,#302896,#302897),(#302898,#302899,#302900),(#302901,
#302902,#302903),(#302904,#302905,#302906),(#302907,#302908,#302909),(#302910,
#302911,#302912),(#302913,#302914,#302915),(#302916,#302917,#302918),(#302919,
#302920,#302921),(#302922,#302923,#302924),(#302925,#302926,#302927),(#302928,
#302929,#302930),(#302931,#302932,#302933),(#302934,#302935,#302936),(#302937,
#302938,#302939),(#302940,#302941,#302942),(#302943,#302944,#302945)),
 .UNSPECIFIED.,.F.,.F.,.F.,(6,1,1,1,1,1,1,1,1,1,1,1,1,1,1,1,1,1,1,1,1,1,
1,1,1,1,1,1,1,1,1,1,1,1,1,1,1,1,1,1,1,1,1,1,1,1,1,1,1,1,1,1,1,1,1,1,1,1,
1,1,1,1,1,1,1,1,1,1,1,1,1,1,1,1,1,1,1,1,1,1,1,1,1,1,1,1,1,1,1,1,1,1,1,1,
1,1,1,1,1,1,1,1,1,1,1,1,1,1,1,1,1,1,1,1,1,1,1,1,1,1,1,1,1,1,1,1,1,1,1,1,
1,1,1,1,1,1,1,1,1,1,1,1,1,1,1,1,1,1,1,1,1,1,1,1,1,1,1,1,1,1,1,1,1,1,1,1,
1,1,1,1,1,1,1,1,1,1,1,1,1,1,1,1,1,1,1,1,1,1,1,1,1,1,1,1,1,1,1,1,1,1,1,1,
1,1,1,1,1,1,1,1,1,1,1,1,1,1,1,1,1,1,1,1,1,1,1,1,1,1,1,1,1,1,1,1,1,1,1,1,
1,1,1,1,1,1,1,1,1,1,1,1,1,1,1,1,1,1,1,1,1,1,1,1,1,1,1,1,1,1,1,1,1,1,1,1,
1,1,1,1,1,1,1,1,1,1,1,1,1,1,1,1,1,1,1,1,1,1,1,1,1,1,1,1,1,1,1,1,1,1,1,1,
1,1,1,1,1,1,1,1,1,1,1,1,1,1,1,1,1,1,1,1,1,1,1,1,1,1,1,1,1,1,1,1,1,1,1,1,
1,1,1,1,1,1,1,1,1,1,1,1,1,1,1,1,1,1,1,1,1,1,1,1,1,1,1,1,1,1,1,1,1,1,1,1,
1,1,1,1,1,1,1,1,1,1,1,1,1,1,1,1,1,1,1,1,1,1,1,1,1,1,1,1,1,1,1,1,1,1,1,1,
1,1,1,1,1,1,1,1,1,1,1,1,1,1,1,1,1,1,1,1,1,1,1,1,1,1,1,1,1,1,1,1,1,1,1,1,
1,1,1,1,1,1,1,1,1,1,1,1,1,1,1,1,1,1,1,1,1,1,1,1,1,1,1,1,1,1,1,1,1,1,1,1,
1,1,1,1,1,1,1,1,1,1,1,1,1,1,1,1,1,1,1,1,1,1,1,1,1,1,1,1,1,1,1,1,1,1,1,1,
1,1,1,1,1,1,1,1,1,1,1,1,1,1,1,1,1,1,1,6),(2,1,2),(-1.,-0.998165138,-0.996330275,
-0.994495413,-0.99266055,-0.990825688,-0.988990826,-0.987155963,-0.985321101,
-0.983486239,-0.981651376,-0.979816514,-0.977981651,-0.976146789,-0.974311927,
-0.972477064,-0.970642202,-0.968807339,-0.966972477,-0.965137615,-0.963302752,
-0.96146789,-0.959633028,-0.957798165,-0.955963303,-0.95412844,-0.952293578,
-0.950458716,-0.948623853,-0.946788991,-0.944954128,-0.943119266,-0.941284404,
-0.939449541,-0.937614679,-0.935779817,-0.933944954,-0.932110092,-0.930275229,
-0.928440367,-0.926605505,-0.924770642,-0.92293578,-0.921100917,-0.919266055,
-0.917431193,-0.91559633,-0.913761468,-0.911926606,-0.910091743,-0.908256881,
-0.906422018,-0.904587156,-0.902752294,-0.900917431,-0.899082569,-0.897247706,
-0.895412844,-0.893577982,-0.891743119,-0.889908257,-0.888073394,-0.886238532,
-0.88440367,-0.882568807,-0.880733945,-0.878899083,-0.87706422,-0.875229358,
-0.873394495,-0.871559633,-0.869724771,-0.867889908,-0.866055046,-0.864220183,
-0.862385321,-0.860550459,-0.858715596,-0.856880734,-0.855045872,-0.853211009,
-0.851376147,-0.849541284,-0.847706422,-0.84587156,-0.844036697,-0.842201835,
-0.840366972,-0.83853211,-0.836697248,-0.834862385,-0.833027523,-0.831192661,
-0.829357798,-0.827522936,-0.825688073,-0.823853211,-0.822018349,-0.820183486,
-0.818348624,-0.816513761,-0.814678899,-0.812844037,-0.811009174,-0.809174312,
-0.80733945,-0.805504587,-0.803669725,-0.801834862,-0.8,-0.798165138,-0.796330275,
-0.794495413,-0.79266055,-0.790825688,-0.788990826,-0.787155963,-0.785321101,
-0.783486239,-0.781651376,-0.779816514,-0.777981651,-0.776146789,-0.774311927,
-0.772477064,-0.770642202,-0.768807339,-0.766972477,-0.765137615,-0.763302752,
-0.76146789,-0.759633028,-0.757798165,-0.755963303,-0.75412844,-0.752293578,
-0.750458716,-0.748623853,-0.746788991,-0.744954128,-0.743119266,-0.741284404,
-0.739449541,-0.737614679,-0.735779817,-0.733944954,-0.732110092,-0.730275229,
-0.728440367,-0.726605505,-0.724770642,-0.72293578,-0.721100917,-0.719266055,
-0.717431193,-0.71559633,-0.713761468,-0.711926606,-0.710091743,-0.708256881,
-0.706422018,-0.704587156,-0.702752294,-0.700917431,-0.699082569,-0.697247706,
-0.695412844,-0.693577982,-0.691743119,-0.689908257,-0.688073394,-0.686238532,
-0.68440367,-0.682568807,-0.680733945,-0.678899083,-0.67706422,-0.675229358,
-0.673394495,-0.671559633,-0.669724771,-0.667889908,-0.666055046,-0.664220183,
-0.662385321,-0.660550459,-0.658715596,-0.656880734,-0.655045872,-0.653211009,
-0.651376147,-0.649541284,-0.647706422,-0.64587156,-0.644036697,-0.642201835,
-0.640366972,-0.63853211,-0.636697248,-0.634862385,-0.633027523,-0.631192661,
-0.629357798,-0.627522936,-0.625688073,-0.623853211,-0.622018349,-0.620183486,
-0.618348624,-0.616513761,-0.614678899,-0.612844037,-0.611009174,-0.609174312,
-0.60733945,-0.605504587,-0.603669725,-0.601834862,-0.6,-0.598165138,-0.596330275,
-0.594495413,-0.59266055,-0.590825688,-0.588990826,-0.587155963,-0.585321101,
-0.583486239,-0.581651376,-0.579816514,-0.577981651,-0.576146789,-0.574311927,
-0.572477064,-0.570642202,-0.568807339,-0.566972477,-0.565137615,-0.563302752,
-0.56146789,-0.559633028,-0.557798165,-0.555963303,-0.55412844,-0.552293578,
-0.550458716,-0.548623853,-0.546788991,-0.544954128,-0.543119266,-0.541284404,
-0.539449541,-0.537614679,-0.535779817,-0.533944954,-0.532110092,-0.530275229,
-0.528440367,-0.526605505,-0.524770642,-0.52293578,-0.521100917,-0.519266055,
-0.517431193,-0.51559633,-0.513761468,-0.511926606,-0.510091743,-0.508256881,
-0.506422018,-0.504587156,-0.502752294,-0.500917431,-0.499082569,-0.497247706,
-0.495412844,-0.493577982,-0.491743119,-0.489908257,-0.488073394,-0.486238532,
-0.48440367,-0.482568807,-0.480733945,-0.478899083,-0.47706422,-0.475229358,
-0.473394495,-0.471559633,-0.469724771,-0.467889908,-0.466055046,-0.464220183,
-0.462385321,-0.460550459,-0.458715596,-0.456880734,-0.455045872,-0.453211009,
-0.451376147,-0.449541284,-0.447706422,-0.44587156,-0.444036697,-0.442201835,
-0.440366972,-0.43853211,-0.436697248,-0.434862385,-0.433027523,-0.431192661,
-0.429357798,-0.427522936,-0.425688073,-0.423853211,-0.422018349,-0.420183486,
-0.418348624,-0.416513761,-0.414678899,-0.412844037,-0.411009174,-0.409174312,
-0.40733945,-0.405504587,-0.403669725,-0.401834862,-0.4,-0.398165138,-0.396330275,
-0.394495413,-0.39266055,-0.390825688,-0.388990826,-0.387155963,-0.385321101,
-0.383486239,-0.381651376,-0.379816514,-0.377981651,-0.376146789,-0.374311927,
-0.372477064,-0.370642202,-0.368807339,-0.366972477,-0.365137615,-0.363302752,
-0.36146789,-0.359633028,-0.357798165,-0.355963303,-0.35412844,-0.352293578,
-0.350458716,-0.348623853,-0.346788991,-0.344954128,-0.343119266,-0.341284404,
-0.339449541,-0.337614679,-0.335779817,-0.333944954,-0.332110092,-0.330275229,
-0.328440367,-0.326605505,-0.324770642,-0.32293578,-0.321100917,-0.319266055,
-0.317431193,-0.31559633,-0.313761468,-0.311926606,-0.310091743,-0.308256881,
-0.306422018,-0.304587156,-0.302752294,-0.300917431,-0.299082569,-0.297247706,
-0.295412844,-0.293577982,-0.291743119,-0.289908257,-0.288073394,-0.286238532,
-0.28440367,-0.282568807,-0.280733945,-0.278899083,-0.27706422,-0.275229358,
-0.273394495,-0.271559633,-0.269724771,-0.267889908,-0.266055046,-0.264220183,
-0.262385321,-0.260550459,-0.258715596,-0.256880734,-0.255045872,-0.253211009,
-0.251376147,-0.249541284,-0.247706422,-0.24587156,-0.244036697,-0.242201835,
-0.240366972,-0.23853211,-0.236697248,-0.234862385,-0.233027523,-0.231192661,
-0.229357798,-0.227522936,-0.225688073,-0.223853211,-0.222018349,-0.220183486,
-0.218348624,-0.216513761,-0.214678899,-0.212844037,-0.211009174,-0.209174312,
-0.20733945,-0.205504587,-0.203669725,-0.201834862,-0.2,-0.198165138,-0.196330275,
-0.194495413,-0.19266055,-0.190825688,-0.188990826,-0.187155963,-0.185321101,
-0.183486239,-0.181651376,-0.179816514,-0.177981651,-0.176146789,-0.174311927,
-0.172477064,-0.170642202,-0.168807339,-0.166972477,-0.165137615,-0.163302752,
-0.16146789,-0.159633028,-0.157798165,-0.155963303,-0.15412844,-0.152293578,
-0.150458716,-0.148623853,-0.146788991,-0.144954128,-0.143119266,-0.141284404,
-0.139449541,-0.137614679,-0.135779817,-0.133944954,-0.132110092,-0.130275229,
-0.128440367,-0.126605505,-0.124770642,-0.12293578,-0.121100917,-0.119266055,
-0.117431193,-0.11559633,-0.113761468,-0.111926606,-0.110091743,-0.108256881,
-0.106422018,-0.104587156,-0.102752294,-0.100917431,-0.099082569,-0.097247706,
-0.095412844,-0.093577982,-0.091743119,-0.089908257,-0.088073394,-0.086238532,
-0.08440367,-0.082568807,-0.080733945,-0.078899083,-0.07706422,-0.075229358,
-0.073394495,-0.071559633,-0.069724771,-0.067889908,-0.066055046,-0.064220183,
-0.062385321,-0.060550459,-0.058715596,-0.056880734,-0.055045872,-0.053211009,
-0.051376147,-0.049541284,-0.047706422,-0.04587156,-0.044036697,-0.042201835,
-0.040366972,-0.03853211,-0.036697248,-0.034862385,-0.033027523,-0.031192661,
-0.029357798,-0.027522936,-0.025688073,-0.023853211,-0.022018349,-0.020183486,
-0.018348624,-0.016513761,-0.014678899,-0.012844037,-0.011009174,-0.009174312,
-0.00733945,-0.005504587,-0.003669725,-0.001834862,0.000982105),(0.3,1.,
1.3),.UNSPECIFIED.);
#6304=B_SPLINE_SURFACE_WITH_KNOTS('',5,1,((#302968,#302969,#302970),(#302971,
#302972,#302973),(#302974,#302975,#302976),(#302977,#302978,#302979),(#302980,
#302981,#302982),(#302983,#302984,#302985),(#302986,#302987,#302988),(#302989,
#302990,#302991),(#302992,#302993,#302994),(#302995,#302996,#302997),(#302998,
#302999,#303000),(#303001,#303002,#303003),(#303004,#303005,#303006),(#303007,
#303008,#303009),(#303010,#303011,#303012),(#303013,#303014,#303015),(#303016,
#303017,#303018),(#303019,#303020,#303021),(#303022,#303023,#303024),(#303025,
#303026,#303027),(#303028,#303029,#303030),(#303031,#303032,#303033),(#303034,
#303035,#303036),(#303037,#303038,#303039),(#303040,#303041,#303042),(#303043,
#303044,#303045),(#303046,#303047,#303048),(#303049,#303050,#303051),(#303052,
#303053,#303054),(#303055,#303056,#303057),(#303058,#303059,#303060),(#303061,
#303062,#303063),(#303064,#303065,#303066),(#303067,#303068,#303069),(#303070,
#303071,#303072),(#303073,#303074,#303075),(#303076,#303077,#303078),(#303079,
#303080,#303081),(#303082,#303083,#303084),(#303085,#303086,#303087),(#303088,
#303089,#303090),(#303091,#303092,#303093),(#303094,#303095,#303096),(#303097,
#303098,#303099),(#303100,#303101,#303102),(#303103,#303104,#303105),(#303106,
#303107,#303108),(#303109,#303110,#303111),(#303112,#303113,#303114),(#303115,
#303116,#303117),(#303118,#303119,#303120),(#303121,#303122,#303123),(#303124,
#303125,#303126),(#303127,#303128,#303129),(#303130,#303131,#303132),(#303133,
#303134,#303135),(#303136,#303137,#303138),(#303139,#303140,#303141),(#303142,
#303143,#303144),(#303145,#303146,#303147),(#303148,#303149,#303150),(#303151,
#303152,#303153),(#303154,#303155,#303156),(#303157,#303158,#303159),(#303160,
#303161,#303162),(#303163,#303164,#303165),(#303166,#303167,#303168),(#303169,
#303170,#303171),(#303172,#303173,#303174),(#303175,#303176,#303177),(#303178,
#303179,#303180),(#303181,#303182,#303183),(#303184,#303185,#303186),(#303187,
#303188,#303189),(#303190,#303191,#303192),(#303193,#303194,#303195),(#303196,
#303197,#303198),(#303199,#303200,#303201),(#303202,#303203,#303204),(#303205,
#303206,#303207),(#303208,#303209,#303210),(#303211,#303212,#303213),(#303214,
#303215,#303216),(#303217,#303218,#303219),(#303220,#303221,#303222),(#303223,
#303224,#303225),(#303226,#303227,#303228),(#303229,#303230,#303231),(#303232,
#303233,#303234),(#303235,#303236,#303237),(#303238,#303239,#303240),(#303241,
#303242,#303243),(#303244,#303245,#303246),(#303247,#303248,#303249),(#303250,
#303251,#303252),(#303253,#303254,#303255),(#303256,#303257,#303258),(#303259,
#303260,#303261),(#303262,#303263,#303264),(#303265,#303266,#303267),(#303268,
#303269,#303270),(#303271,#303272,#303273),(#303274,#303275,#303276),(#303277,
#303278,#303279),(#303280,#303281,#303282),(#303283,#303284,#303285),(#303286,
#303287,#303288),(#303289,#303290,#303291),(#303292,#303293,#303294),(#303295,
#303296,#303297),(#303298,#303299,#303300),(#303301,#303302,#303303),(#303304,
#303305,#303306),(#303307,#303308,#303309),(#303310,#303311,#303312),(#303313,
#303314,#303315),(#303316,#303317,#303318),(#303319,#303320,#303321),(#303322,
#303323,#303324),(#303325,#303326,#303327),(#303328,#303329,#303330),(#303331,
#303332,#303333),(#303334,#303335,#303336),(#303337,#303338,#303339),(#303340,
#303341,#303342),(#303343,#303344,#303345),(#303346,#303347,#303348),(#303349,
#303350,#303351),(#303352,#303353,#303354),(#303355,#303356,#303357),(#303358,
#303359,#303360),(#303361,#303362,#303363),(#303364,#303365,#303366),(#303367,
#303368,#303369),(#303370,#303371,#303372),(#303373,#303374,#303375),(#303376,
#303377,#303378),(#303379,#303380,#303381),(#303382,#303383,#303384),(#303385,
#303386,#303387),(#303388,#303389,#303390),(#303391,#303392,#303393),(#303394,
#303395,#303396),(#303397,#303398,#303399),(#303400,#303401,#303402),(#303403,
#303404,#303405),(#303406,#303407,#303408),(#303409,#303410,#303411),(#303412,
#303413,#303414),(#303415,#303416,#303417),(#303418,#303419,#303420),(#303421,
#303422,#303423),(#303424,#303425,#303426),(#303427,#303428,#303429),(#303430,
#303431,#303432),(#303433,#303434,#303435),(#303436,#303437,#303438),(#303439,
#303440,#303441),(#303442,#303443,#303444),(#303445,#303446,#303447),(#303448,
#303449,#303450),(#303451,#303452,#303453),(#303454,#303455,#303456),(#303457,
#303458,#303459),(#303460,#303461,#303462),(#303463,#303464,#303465),(#303466,
#303467,#303468),(#303469,#303470,#303471),(#303472,#303473,#303474),(#303475,
#303476,#303477),(#303478,#303479,#303480),(#303481,#303482,#303483),(#303484,
#303485,#303486),(#303487,#303488,#303489),(#303490,#303491,#303492),(#303493,
#303494,#303495),(#303496,#303497,#303498),(#303499,#303500,#303501),(#303502,
#303503,#303504),(#303505,#303506,#303507),(#303508,#303509,#303510),(#303511,
#303512,#303513),(#303514,#303515,#303516),(#303517,#303518,#303519),(#303520,
#303521,#303522),(#303523,#303524,#303525),(#303526,#303527,#303528),(#303529,
#303530,#303531),(#303532,#303533,#303534),(#303535,#303536,#303537),(#303538,
#303539,#303540),(#303541,#303542,#303543),(#303544,#303545,#303546),(#303547,
#303548,#303549),(#303550,#303551,#303552),(#303553,#303554,#303555),(#303556,
#303557,#303558),(#303559,#303560,#303561),(#303562,#303563,#303564),(#303565,
#303566,#303567),(#303568,#303569,#303570),(#303571,#303572,#303573),(#303574,
#303575,#303576),(#303577,#303578,#303579),(#303580,#303581,#303582),(#303583,
#303584,#303585),(#303586,#303587,#303588),(#303589,#303590,#303591),(#303592,
#303593,#303594),(#303595,#303596,#303597),(#303598,#303599,#303600),(#303601,
#303602,#303603),(#303604,#303605,#303606),(#303607,#303608,#303609),(#303610,
#303611,#303612),(#303613,#303614,#303615),(#303616,#303617,#303618),(#303619,
#303620,#303621),(#303622,#303623,#303624),(#303625,#303626,#303627),(#303628,
#303629,#303630),(#303631,#303632,#303633),(#303634,#303635,#303636),(#303637,
#303638,#303639),(#303640,#303641,#303642),(#303643,#303644,#303645),(#303646,
#303647,#303648),(#303649,#303650,#303651),(#303652,#303653,#303654),(#303655,
#303656,#303657),(#303658,#303659,#303660),(#303661,#303662,#303663),(#303664,
#303665,#303666),(#303667,#303668,#303669),(#303670,#303671,#303672),(#303673,
#303674,#303675),(#303676,#303677,#303678),(#303679,#303680,#303681),(#303682,
#303683,#303684),(#303685,#303686,#303687),(#303688,#303689,#303690),(#303691,
#303692,#303693),(#303694,#303695,#303696),(#303697,#303698,#303699),(#303700,
#303701,#303702),(#303703,#303704,#303705),(#303706,#303707,#303708),(#303709,
#303710,#303711),(#303712,#303713,#303714),(#303715,#303716,#303717),(#303718,
#303719,#303720),(#303721,#303722,#303723),(#303724,#303725,#303726),(#303727,
#303728,#303729),(#303730,#303731,#303732),(#303733,#303734,#303735),(#303736,
#303737,#303738),(#303739,#303740,#303741),(#303742,#303743,#303744),(#303745,
#303746,#303747),(#303748,#303749,#303750),(#303751,#303752,#303753),(#303754,
#303755,#303756),(#303757,#303758,#303759),(#303760,#303761,#303762),(#303763,
#303764,#303765),(#303766,#303767,#303768),(#303769,#303770,#303771),(#303772,
#303773,#303774),(#303775,#303776,#303777),(#303778,#303779,#303780),(#303781,
#303782,#303783),(#303784,#303785,#303786),(#303787,#303788,#303789),(#303790,
#303791,#303792),(#303793,#303794,#303795),(#303796,#303797,#303798),(#303799,
#303800,#303801),(#303802,#303803,#303804),(#303805,#303806,#303807),(#303808,
#303809,#303810),(#303811,#303812,#303813),(#303814,#303815,#303816),(#303817,
#303818,#303819),(#303820,#303821,#303822),(#303823,#303824,#303825),(#303826,
#303827,#303828),(#303829,#303830,#303831),(#303832,#303833,#303834),(#303835,
#303836,#303837),(#303838,#303839,#303840),(#303841,#303842,#303843),(#303844,
#303845,#303846),(#303847,#303848,#303849),(#303850,#303851,#303852),(#303853,
#303854,#303855),(#303856,#303857,#303858),(#303859,#303860,#303861),(#303862,
#303863,#303864),(#303865,#303866,#303867),(#303868,#303869,#303870),(#303871,
#303872,#303873),(#303874,#303875,#303876),(#303877,#303878,#303879),(#303880,
#303881,#303882),(#303883,#303884,#303885),(#303886,#303887,#303888),(#303889,
#303890,#303891),(#303892,#303893,#303894),(#303895,#303896,#303897),(#303898,
#303899,#303900),(#303901,#303902,#303903),(#303904,#303905,#303906),(#303907,
#303908,#303909),(#303910,#303911,#303912),(#303913,#303914,#303915),(#303916,
#303917,#303918),(#303919,#303920,#303921),(#303922,#303923,#303924),(#303925,
#303926,#303927),(#303928,#303929,#303930),(#303931,#303932,#303933),(#303934,
#303935,#303936),(#303937,#303938,#303939),(#303940,#303941,#303942),(#303943,
#303944,#303945),(#303946,#303947,#303948),(#303949,#303950,#303951),(#303952,
#303953,#303954),(#303955,#303956,#303957),(#303958,#303959,#303960),(#303961,
#303962,#303963),(#303964,#303965,#303966),(#303967,#303968,#303969),(#303970,
#303971,#303972),(#303973,#303974,#303975),(#303976,#303977,#303978),(#303979,
#303980,#303981),(#303982,#303983,#303984),(#303985,#303986,#303987),(#303988,
#303989,#303990),(#303991,#303992,#303993),(#303994,#303995,#303996),(#303997,
#303998,#303999),(#304000,#304001,#304002),(#304003,#304004,#304005),(#304006,
#304007,#304008),(#304009,#304010,#304011),(#304012,#304013,#304014),(#304015,
#304016,#304017),(#304018,#304019,#304020),(#304021,#304022,#304023),(#304024,
#304025,#304026),(#304027,#304028,#304029),(#304030,#304031,#304032),(#304033,
#304034,#304035),(#304036,#304037,#304038),(#304039,#304040,#304041),(#304042,
#304043,#304044),(#304045,#304046,#304047),(#304048,#304049,#304050),(#304051,
#304052,#304053),(#304054,#304055,#304056),(#304057,#304058,#304059),(#304060,
#304061,#304062),(#304063,#304064,#304065),(#304066,#304067,#304068),(#304069,
#304070,#304071),(#304072,#304073,#304074),(#304075,#304076,#304077),(#304078,
#304079,#304080),(#304081,#304082,#304083),(#304084,#304085,#304086),(#304087,
#304088,#304089),(#304090,#304091,#304092),(#304093,#304094,#304095),(#304096,
#304097,#304098),(#304099,#304100,#304101),(#304102,#304103,#304104),(#304105,
#304106,#304107),(#304108,#304109,#304110),(#304111,#304112,#304113),(#304114,
#304115,#304116),(#304117,#304118,#304119),(#304120,#304121,#304122),(#304123,
#304124,#304125),(#304126,#304127,#304128),(#304129,#304130,#304131),(#304132,
#304133,#304134),(#304135,#304136,#304137),(#304138,#304139,#304140),(#304141,
#304142,#304143),(#304144,#304145,#304146),(#304147,#304148,#304149),(#304150,
#304151,#304152),(#304153,#304154,#304155),(#304156,#304157,#304158),(#304159,
#304160,#304161),(#304162,#304163,#304164),(#304165,#304166,#304167),(#304168,
#304169,#304170),(#304171,#304172,#304173),(#304174,#304175,#304176),(#304177,
#304178,#304179),(#304180,#304181,#304182),(#304183,#304184,#304185),(#304186,
#304187,#304188),(#304189,#304190,#304191),(#304192,#304193,#304194),(#304195,
#304196,#304197),(#304198,#304199,#304200),(#304201,#304202,#304203),(#304204,
#304205,#304206),(#304207,#304208,#304209),(#304210,#304211,#304212),(#304213,
#304214,#304215),(#304216,#304217,#304218),(#304219,#304220,#304221),(#304222,
#304223,#304224),(#304225,#304226,#304227),(#304228,#304229,#304230),(#304231,
#304232,#304233),(#304234,#304235,#304236),(#304237,#304238,#304239),(#304240,
#304241,#304242),(#304243,#304244,#304245),(#304246,#304247,#304248),(#304249,
#304250,#304251),(#304252,#304253,#304254),(#304255,#304256,#304257),(#304258,
#304259,#304260),(#304261,#304262,#304263),(#304264,#304265,#304266),(#304267,
#304268,#304269),(#304270,#304271,#304272),(#304273,#304274,#304275),(#304276,
#304277,#304278),(#304279,#304280,#304281),(#304282,#304283,#304284),(#304285,
#304286,#304287),(#304288,#304289,#304290),(#304291,#304292,#304293),(#304294,
#304295,#304296),(#304297,#304298,#304299),(#304300,#304301,#304302),(#304303,
#304304,#304305),(#304306,#304307,#304308),(#304309,#304310,#304311),(#304312,
#304313,#304314),(#304315,#304316,#304317),(#304318,#304319,#304320),(#304321,
#304322,#304323),(#304324,#304325,#304326),(#304327,#304328,#304329),(#304330,
#304331,#304332),(#304333,#304334,#304335),(#304336,#304337,#304338),(#304339,
#304340,#304341),(#304342,#304343,#304344),(#304345,#304346,#304347),(#304348,
#304349,#304350),(#304351,#304352,#304353),(#304354,#304355,#304356),(#304357,
#304358,#304359),(#304360,#304361,#304362),(#304363,#304364,#304365),(#304366,
#304367,#304368),(#304369,#304370,#304371),(#304372,#304373,#304374),(#304375,
#304376,#304377),(#304378,#304379,#304380),(#304381,#304382,#304383),(#304384,
#304385,#304386),(#304387,#304388,#304389),(#304390,#304391,#304392),(#304393,
#304394,#304395),(#304396,#304397,#304398),(#304399,#304400,#304401),(#304402,
#304403,#304404),(#304405,#304406,#304407),(#304408,#304409,#304410),(#304411,
#304412,#304413),(#304414,#304415,#304416),(#304417,#304418,#304419),(#304420,
#304421,#304422),(#304423,#304424,#304425),(#304426,#304427,#304428),(#304429,
#304430,#304431),(#304432,#304433,#304434),(#304435,#304436,#304437),(#304438,
#304439,#304440),(#304441,#304442,#304443),(#304444,#304445,#304446),(#304447,
#304448,#304449),(#304450,#304451,#304452),(#304453,#304454,#304455),(#304456,
#304457,#304458),(#304459,#304460,#304461),(#304462,#304463,#304464),(#304465,
#304466,#304467),(#304468,#304469,#304470),(#304471,#304472,#304473),(#304474,
#304475,#304476),(#304477,#304478,#304479),(#304480,#304481,#304482),(#304483,
#304484,#304485),(#304486,#304487,#304488),(#304489,#304490,#304491),(#304492,
#304493,#304494),(#304495,#304496,#304497),(#304498,#304499,#304500),(#304501,
#304502,#304503),(#304504,#304505,#304506),(#304507,#304508,#304509),(#304510,
#304511,#304512),(#304513,#304514,#304515),(#304516,#304517,#304518),(#304519,
#304520,#304521),(#304522,#304523,#304524),(#304525,#304526,#304527),(#304528,
#304529,#304530),(#304531,#304532,#304533),(#304534,#304535,#304536),(#304537,
#304538,#304539),(#304540,#304541,#304542),(#304543,#304544,#304545),(#304546,
#304547,#304548),(#304549,#304550,#304551),(#304552,#304553,#304554),(#304555,
#304556,#304557),(#304558,#304559,#304560),(#304561,#304562,#304563),(#304564,
#304565,#304566),(#304567,#304568,#304569),(#304570,#304571,#304572),(#304573,
#304574,#304575),(#304576,#304577,#304578),(#304579,#304580,#304581),(#304582,
#304583,#304584),(#304585,#304586,#304587),(#304588,#304589,#304590),(#304591,
#304592,#304593),(#304594,#304595,#304596),(#304597,#304598,#304599),(#304600,
#304601,#304602),(#304603,#304604,#304605),(#304606,#304607,#304608),(#304609,
#304610,#304611),(#304612,#304613,#304614),(#304615,#304616,#304617),(#304618,
#304619,#304620)),.UNSPECIFIED.,.F.,.F.,.F.,(6,1,1,1,1,1,1,1,1,1,1,1,1,
1,1,1,1,1,1,1,1,1,1,1,1,1,1,1,1,1,1,1,1,1,1,1,1,1,1,1,1,1,1,1,1,1,1,1,1,
1,1,1,1,1,1,1,1,1,1,1,1,1,1,1,1,1,1,1,1,1,1,1,1,1,1,1,1,1,1,1,1,1,1,1,1,
1,1,1,1,1,1,1,1,1,1,1,1,1,1,1,1,1,1,1,1,1,1,1,1,1,1,1,1,1,1,1,1,1,1,1,1,
1,1,1,1,1,1,1,1,1,1,1,1,1,1,1,1,1,1,1,1,1,1,1,1,1,1,1,1,1,1,1,1,1,1,1,1,
1,1,1,1,1,1,1,1,1,1,1,1,1,1,1,1,1,1,1,1,1,1,1,1,1,1,1,1,1,1,1,1,1,1,1,1,
1,1,1,1,1,1,1,1,1,1,1,1,1,1,1,1,1,1,1,1,1,1,1,1,1,1,1,1,1,1,1,1,1,1,1,1,
1,1,1,1,1,1,1,1,1,1,1,1,1,1,1,1,1,1,1,1,1,1,1,1,1,1,1,1,1,1,1,1,1,1,1,1,
1,1,1,1,1,1,1,1,1,1,1,1,1,1,1,1,1,1,1,1,1,1,1,1,1,1,1,1,1,1,1,1,1,1,1,1,
1,1,1,1,1,1,1,1,1,1,1,1,1,1,1,1,1,1,1,1,1,1,1,1,1,1,1,1,1,1,1,1,1,1,1,1,
1,1,1,1,1,1,1,1,1,1,1,1,1,1,1,1,1,1,1,1,1,1,1,1,1,1,1,1,1,1,1,1,1,1,1,1,
1,1,1,1,1,1,1,1,1,1,1,1,1,1,1,1,1,1,1,1,1,1,1,1,1,1,1,1,1,1,1,1,1,1,1,1,
1,1,1,1,1,1,1,1,1,1,1,1,1,1,1,1,1,1,1,1,1,1,1,1,1,1,1,1,1,1,1,1,1,1,1,1,
1,1,1,1,1,1,1,1,1,1,1,1,1,1,1,1,1,1,1,1,1,1,1,1,1,1,1,1,1,1,1,1,1,1,1,1,
1,1,1,1,1,1,1,1,1,1,1,1,1,1,1,1,1,1,1,1,1,1,1,1,1,1,1,1,1,1,1,1,1,1,1,1,
1,1,1,1,1,1,1,1,1,1,1,1,1,1,1,1,1,1,1,1,1,1,1,1,1,1,1,1,1,6),(2,1,2),(-0.001964151,
0.,0.001834862,0.003669725,0.005504587,0.00733945,0.009174312,0.011009174,
0.012844037,0.014678899,0.016513761,0.018348624,0.020183486,0.022018349,
0.023853211,0.025688073,0.027522936,0.029357798,0.031192661,0.033027523,
0.034862385,0.036697248,0.03853211,0.040366972,0.042201835,0.044036697,
0.04587156,0.047706422,0.049541284,0.051376147,0.053211009,0.055045872,
0.056880734,0.058715596,0.060550459,0.062385321,0.064220183,0.066055046,
0.067889908,0.069724771,0.071559633,0.073394495,0.075229358,0.07706422,
0.078899083,0.080733945,0.082568807,0.08440367,0.086238532,0.088073394,
0.089908257,0.091743119,0.093577982,0.095412844,0.097247706,0.099082569,
0.100917431,0.102752294,0.104587156,0.106422018,0.108256881,0.110091743,
0.111926606,0.113761468,0.11559633,0.117431193,0.119266055,0.121100917,
0.12293578,0.124770642,0.126605505,0.128440367,0.130275229,0.132110092,
0.133944954,0.135779817,0.137614679,0.139449541,0.141284404,0.143119266,
0.144954128,0.146788991,0.148623853,0.150458716,0.152293578,0.15412844,
0.155963303,0.157798165,0.159633028,0.16146789,0.163302752,0.165137615,
0.166972477,0.168807339,0.170642202,0.172477064,0.174311927,0.176146789,
0.177981651,0.179816514,0.181651376,0.183486239,0.185321101,0.187155963,
0.188990826,0.190825688,0.19266055,0.194495413,0.196330275,0.198165138,
0.2,0.201834862,0.203669725,0.205504587,0.20733945,0.209174312,0.211009174,
0.212844037,0.214678899,0.216513761,0.218348624,0.220183486,0.222018349,
0.223853211,0.225688073,0.227522936,0.229357798,0.231192661,0.233027523,
0.234862385,0.236697248,0.23853211,0.240366972,0.242201835,0.244036697,
0.24587156,0.247706422,0.249541284,0.251376147,0.253211009,0.255045872,
0.256880734,0.258715596,0.260550459,0.262385321,0.264220183,0.266055046,
0.267889908,0.269724771,0.271559633,0.273394495,0.275229358,0.27706422,
0.278899083,0.280733945,0.282568807,0.28440367,0.286238532,0.288073394,
0.289908257,0.291743119,0.293577982,0.295412844,0.297247706,0.299082569,
0.300917431,0.302752294,0.304587156,0.306422018,0.308256881,0.310091743,
0.311926606,0.313761468,0.31559633,0.317431193,0.319266055,0.321100917,
0.32293578,0.324770642,0.326605505,0.328440367,0.330275229,0.332110092,
0.333944954,0.335779817,0.337614679,0.339449541,0.341284404,0.343119266,
0.344954128,0.346788991,0.348623853,0.350458716,0.352293578,0.35412844,
0.355963303,0.357798165,0.359633028,0.36146789,0.363302752,0.365137615,
0.366972477,0.368807339,0.370642202,0.372477064,0.374311927,0.376146789,
0.377981651,0.379816514,0.381651376,0.383486239,0.385321101,0.387155963,
0.388990826,0.390825688,0.39266055,0.394495413,0.396330275,0.398165138,
0.4,0.401834862,0.403669725,0.405504587,0.40733945,0.409174312,0.411009174,
0.412844037,0.414678899,0.416513761,0.418348624,0.420183486,0.422018349,
0.423853211,0.425688073,0.427522936,0.429357798,0.431192661,0.433027523,
0.434862385,0.436697248,0.43853211,0.440366972,0.442201835,0.444036697,
0.44587156,0.447706422,0.449541284,0.451376147,0.453211009,0.455045872,
0.456880734,0.458715596,0.460550459,0.462385321,0.464220183,0.466055046,
0.467889908,0.469724771,0.471559633,0.473394495,0.475229358,0.47706422,
0.478899083,0.480733945,0.482568807,0.48440367,0.486238532,0.488073394,
0.489908257,0.491743119,0.493577982,0.495412844,0.497247706,0.499082569,
0.500917431,0.502752294,0.504587156,0.506422018,0.508256881,0.510091743,
0.511926606,0.513761468,0.51559633,0.517431193,0.519266055,0.521100917,
0.52293578,0.524770642,0.526605505,0.528440367,0.530275229,0.532110092,
0.533944954,0.535779817,0.537614679,0.539449541,0.541284404,0.543119266,
0.544954128,0.546788991,0.548623853,0.550458716,0.552293578,0.55412844,
0.555963303,0.557798165,0.559633028,0.56146789,0.563302752,0.565137615,
0.566972477,0.568807339,0.570642202,0.572477064,0.574311927,0.576146789,
0.577981651,0.579816514,0.581651376,0.583486239,0.585321101,0.587155963,
0.588990826,0.590825688,0.59266055,0.594495413,0.596330275,0.598165138,
0.6,0.601834862,0.603669725,0.605504587,0.60733945,0.609174312,0.611009174,
0.612844037,0.614678899,0.616513761,0.618348624,0.620183486,0.622018349,
0.623853211,0.625688073,0.627522936,0.629357798,0.631192661,0.633027523,
0.634862385,0.636697248,0.63853211,0.640366972,0.642201835,0.644036697,
0.64587156,0.647706422,0.649541284,0.651376147,0.653211009,0.655045872,
0.656880734,0.658715596,0.660550459,0.662385321,0.664220183,0.666055046,
0.667889908,0.669724771,0.671559633,0.673394495,0.675229358,0.67706422,
0.678899083,0.680733945,0.682568807,0.68440367,0.686238532,0.688073394,
0.689908257,0.691743119,0.693577982,0.695412844,0.697247706,0.699082569,
0.700917431,0.702752294,0.704587156,0.706422018,0.708256881,0.710091743,
0.711926606,0.713761468,0.71559633,0.717431193,0.719266055,0.721100917,
0.72293578,0.724770642,0.726605505,0.728440367,0.730275229,0.732110092,
0.733944954,0.735779817,0.737614679,0.739449541,0.741284404,0.743119266,
0.744954128,0.746788991,0.748623853,0.750458716,0.752293578,0.75412844,
0.755963303,0.757798165,0.759633028,0.76146789,0.763302752,0.765137615,
0.766972477,0.768807339,0.770642202,0.772477064,0.774311927,0.776146789,
0.777981651,0.779816514,0.781651376,0.783486239,0.785321101,0.787155963,
0.788990826,0.790825688,0.79266055,0.794495413,0.796330275,0.798165138,
0.8,0.801834862,0.803669725,0.805504587,0.80733945,0.809174312,0.811009174,
0.812844037,0.814678899,0.816513761,0.818348624,0.820183486,0.822018349,
0.823853211,0.825688073,0.827522936,0.829357798,0.831192661,0.833027523,
0.834862385,0.836697248,0.83853211,0.840366972,0.842201835,0.844036697,
0.84587156,0.847706422,0.849541284,0.851376147,0.853211009,0.855045872,
0.856880734,0.858715596,0.860550459,0.862385321,0.864220183,0.866055046,
0.867889908,0.869724771,0.871559633,0.873394495,0.875229358,0.87706422,
0.878899083,0.880733945,0.882568807,0.88440367,0.886238532,0.888073394,
0.889908257,0.891743119,0.893577982,0.895412844,0.897247706,0.899082569,
0.900917431,0.902752294,0.904587156,0.906422018,0.908256881,0.910091743,
0.911926606,0.913761468,0.91559633,0.917431193,0.919266055,0.921100917,
0.92293578,0.924770642,0.926605505,0.928440367,0.930275229,0.932110092,
0.933944954,0.935779817,0.937614679,0.939449541,0.941284404,0.943119266,
0.944954128,0.946788991,0.948623853,0.950458716,0.952293578,0.95412844,
0.955963303,0.957798165,0.959633028,0.96146789,0.963302752,0.965137615,
0.966972477,0.968807339,0.970642202,0.972477064,0.974311927,0.976146789,
0.977981651,0.979816514,0.981651376,0.983486239,0.985321101,0.987155963,
0.988990826,0.990825688,0.99266055,0.994495413,0.996330275,0.998165138,
1.000000000411),(0.3,1.,1.3),.UNSPECIFIED.);
#6305=B_SPLINE_SURFACE_WITH_KNOTS('',5,1,((#304635,#304636,#304637),(#304638,
#304639,#304640),(#304641,#304642,#304643),(#304644,#304645,#304646),(#304647,
#304648,#304649),(#304650,#304651,#304652),(#304653,#304654,#304655),(#304656,
#304657,#304658),(#304659,#304660,#304661),(#304662,#304663,#304664),(#304665,
#304666,#304667),(#304668,#304669,#304670),(#304671,#304672,#304673),(#304674,
#304675,#304676),(#304677,#304678,#304679),(#304680,#304681,#304682),(#304683,
#304684,#304685),(#304686,#304687,#304688),(#304689,#304690,#304691),(#304692,
#304693,#304694),(#304695,#304696,#304697),(#304698,#304699,#304700),(#304701,
#304702,#304703),(#304704,#304705,#304706),(#304707,#304708,#304709),(#304710,
#304711,#304712),(#304713,#304714,#304715),(#304716,#304717,#304718),(#304719,
#304720,#304721),(#304722,#304723,#304724),(#304725,#304726,#304727),(#304728,
#304729,#304730),(#304731,#304732,#304733),(#304734,#304735,#304736),(#304737,
#304738,#304739),(#304740,#304741,#304742),(#304743,#304744,#304745),(#304746,
#304747,#304748),(#304749,#304750,#304751),(#304752,#304753,#304754),(#304755,
#304756,#304757),(#304758,#304759,#304760),(#304761,#304762,#304763),(#304764,
#304765,#304766),(#304767,#304768,#304769),(#304770,#304771,#304772),(#304773,
#304774,#304775),(#304776,#304777,#304778),(#304779,#304780,#304781),(#304782,
#304783,#304784),(#304785,#304786,#304787),(#304788,#304789,#304790),(#304791,
#304792,#304793),(#304794,#304795,#304796),(#304797,#304798,#304799),(#304800,
#304801,#304802),(#304803,#304804,#304805),(#304806,#304807,#304808),(#304809,
#304810,#304811),(#304812,#304813,#304814),(#304815,#304816,#304817),(#304818,
#304819,#304820),(#304821,#304822,#304823),(#304824,#304825,#304826),(#304827,
#304828,#304829),(#304830,#304831,#304832),(#304833,#304834,#304835),(#304836,
#304837,#304838),(#304839,#304840,#304841),(#304842,#304843,#304844),(#304845,
#304846,#304847),(#304848,#304849,#304850),(#304851,#304852,#304853),(#304854,
#304855,#304856),(#304857,#304858,#304859),(#304860,#304861,#304862),(#304863,
#304864,#304865),(#304866,#304867,#304868),(#304869,#304870,#304871),(#304872,
#304873,#304874),(#304875,#304876,#304877),(#304878,#304879,#304880),(#304881,
#304882,#304883),(#304884,#304885,#304886),(#304887,#304888,#304889),(#304890,
#304891,#304892),(#304893,#304894,#304895),(#304896,#304897,#304898),(#304899,
#304900,#304901),(#304902,#304903,#304904),(#304905,#304906,#304907),(#304908,
#304909,#304910),(#304911,#304912,#304913),(#304914,#304915,#304916),(#304917,
#304918,#304919),(#304920,#304921,#304922),(#304923,#304924,#304925),(#304926,
#304927,#304928),(#304929,#304930,#304931),(#304932,#304933,#304934),(#304935,
#304936,#304937),(#304938,#304939,#304940),(#304941,#304942,#304943),(#304944,
#304945,#304946),(#304947,#304948,#304949),(#304950,#304951,#304952),(#304953,
#304954,#304955),(#304956,#304957,#304958),(#304959,#304960,#304961),(#304962,
#304963,#304964),(#304965,#304966,#304967),(#304968,#304969,#304970),(#304971,
#304972,#304973),(#304974,#304975,#304976),(#304977,#304978,#304979),(#304980,
#304981,#304982),(#304983,#304984,#304985),(#304986,#304987,#304988),(#304989,
#304990,#304991),(#304992,#304993,#304994),(#304995,#304996,#304997),(#304998,
#304999,#305000),(#305001,#305002,#305003),(#305004,#305005,#305006),(#305007,
#305008,#305009),(#305010,#305011,#305012),(#305013,#305014,#305015),(#305016,
#305017,#305018),(#305019,#305020,#305021),(#305022,#305023,#305024),(#305025,
#305026,#305027),(#305028,#305029,#305030),(#305031,#305032,#305033),(#305034,
#305035,#305036),(#305037,#305038,#305039),(#305040,#305041,#305042),(#305043,
#305044,#305045),(#305046,#305047,#305048),(#305049,#305050,#305051),(#305052,
#305053,#305054),(#305055,#305056,#305057),(#305058,#305059,#305060),(#305061,
#305062,#305063),(#305064,#305065,#305066),(#305067,#305068,#305069),(#305070,
#305071,#305072),(#305073,#305074,#305075),(#305076,#305077,#305078),(#305079,
#305080,#305081),(#305082,#305083,#305084),(#305085,#305086,#305087),(#305088,
#305089,#305090),(#305091,#305092,#305093),(#305094,#305095,#305096),(#305097,
#305098,#305099),(#305100,#305101,#305102),(#305103,#305104,#305105),(#305106,
#305107,#305108),(#305109,#305110,#305111),(#305112,#305113,#305114),(#305115,
#305116,#305117),(#305118,#305119,#305120),(#305121,#305122,#305123),(#305124,
#305125,#305126),(#305127,#305128,#305129),(#305130,#305131,#305132),(#305133,
#305134,#305135),(#305136,#305137,#305138),(#305139,#305140,#305141),(#305142,
#305143,#305144),(#305145,#305146,#305147),(#305148,#305149,#305150),(#305151,
#305152,#305153),(#305154,#305155,#305156),(#305157,#305158,#305159),(#305160,
#305161,#305162),(#305163,#305164,#305165),(#305166,#305167,#305168),(#305169,
#305170,#305171),(#305172,#305173,#305174),(#305175,#305176,#305177),(#305178,
#305179,#305180),(#305181,#305182,#305183),(#305184,#305185,#305186),(#305187,
#305188,#305189),(#305190,#305191,#305192),(#305193,#305194,#305195),(#305196,
#305197,#305198),(#305199,#305200,#305201),(#305202,#305203,#305204),(#305205,
#305206,#305207),(#305208,#305209,#305210),(#305211,#305212,#305213),(#305214,
#305215,#305216),(#305217,#305218,#305219),(#305220,#305221,#305222),(#305223,
#305224,#305225),(#305226,#305227,#305228),(#305229,#305230,#305231),(#305232,
#305233,#305234),(#305235,#305236,#305237),(#305238,#305239,#305240),(#305241,
#305242,#305243),(#305244,#305245,#305246),(#305247,#305248,#305249),(#305250,
#305251,#305252),(#305253,#305254,#305255),(#305256,#305257,#305258),(#305259,
#305260,#305261),(#305262,#305263,#305264),(#305265,#305266,#305267),(#305268,
#305269,#305270),(#305271,#305272,#305273),(#305274,#305275,#305276),(#305277,
#305278,#305279),(#305280,#305281,#305282),(#305283,#305284,#305285),(#305286,
#305287,#305288),(#305289,#305290,#305291),(#305292,#305293,#305294),(#305295,
#305296,#305297),(#305298,#305299,#305300),(#305301,#305302,#305303),(#305304,
#305305,#305306),(#305307,#305308,#305309),(#305310,#305311,#305312),(#305313,
#305314,#305315),(#305316,#305317,#305318),(#305319,#305320,#305321),(#305322,
#305323,#305324),(#305325,#305326,#305327),(#305328,#305329,#305330),(#305331,
#305332,#305333),(#305334,#305335,#305336),(#305337,#305338,#305339),(#305340,
#305341,#305342),(#305343,#305344,#305345),(#305346,#305347,#305348),(#305349,
#305350,#305351),(#305352,#305353,#305354),(#305355,#305356,#305357),(#305358,
#305359,#305360),(#305361,#305362,#305363),(#305364,#305365,#305366),(#305367,
#305368,#305369),(#305370,#305371,#305372),(#305373,#305374,#305375),(#305376,
#305377,#305378),(#305379,#305380,#305381),(#305382,#305383,#305384),(#305385,
#305386,#305387),(#305388,#305389,#305390),(#305391,#305392,#305393),(#305394,
#305395,#305396),(#305397,#305398,#305399),(#305400,#305401,#305402),(#305403,
#305404,#305405),(#305406,#305407,#305408),(#305409,#305410,#305411),(#305412,
#305413,#305414),(#305415,#305416,#305417),(#305418,#305419,#305420),(#305421,
#305422,#305423),(#305424,#305425,#305426),(#305427,#305428,#305429),(#305430,
#305431,#305432),(#305433,#305434,#305435),(#305436,#305437,#305438),(#305439,
#305440,#305441),(#305442,#305443,#305444),(#305445,#305446,#305447),(#305448,
#305449,#305450),(#305451,#305452,#305453),(#305454,#305455,#305456),(#305457,
#305458,#305459),(#305460,#305461,#305462),(#305463,#305464,#305465),(#305466,
#305467,#305468),(#305469,#305470,#305471),(#305472,#305473,#305474),(#305475,
#305476,#305477),(#305478,#305479,#305480),(#305481,#305482,#305483),(#305484,
#305485,#305486),(#305487,#305488,#305489),(#305490,#305491,#305492),(#305493,
#305494,#305495),(#305496,#305497,#305498),(#305499,#305500,#305501),(#305502,
#305503,#305504),(#305505,#305506,#305507),(#305508,#305509,#305510),(#305511,
#305512,#305513),(#305514,#305515,#305516),(#305517,#305518,#305519),(#305520,
#305521,#305522),(#305523,#305524,#305525),(#305526,#305527,#305528),(#305529,
#305530,#305531),(#305532,#305533,#305534),(#305535,#305536,#305537),(#305538,
#305539,#305540),(#305541,#305542,#305543),(#305544,#305545,#305546),(#305547,
#305548,#305549),(#305550,#305551,#305552),(#305553,#305554,#305555),(#305556,
#305557,#305558),(#305559,#305560,#305561),(#305562,#305563,#305564),(#305565,
#305566,#305567),(#305568,#305569,#305570),(#305571,#305572,#305573),(#305574,
#305575,#305576),(#305577,#305578,#305579),(#305580,#305581,#305582),(#305583,
#305584,#305585),(#305586,#305587,#305588),(#305589,#305590,#305591),(#305592,
#305593,#305594),(#305595,#305596,#305597),(#305598,#305599,#305600),(#305601,
#305602,#305603),(#305604,#305605,#305606),(#305607,#305608,#305609),(#305610,
#305611,#305612),(#305613,#305614,#305615),(#305616,#305617,#305618),(#305619,
#305620,#305621),(#305622,#305623,#305624),(#305625,#305626,#305627),(#305628,
#305629,#305630),(#305631,#305632,#305633),(#305634,#305635,#305636),(#305637,
#305638,#305639),(#305640,#305641,#305642),(#305643,#305644,#305645),(#305646,
#305647,#305648),(#305649,#305650,#305651),(#305652,#305653,#305654),(#305655,
#305656,#305657),(#305658,#305659,#305660),(#305661,#305662,#305663),(#305664,
#305665,#305666),(#305667,#305668,#305669),(#305670,#305671,#305672),(#305673,
#305674,#305675),(#305676,#305677,#305678),(#305679,#305680,#305681),(#305682,
#305683,#305684),(#305685,#305686,#305687),(#305688,#305689,#305690),(#305691,
#305692,#305693),(#305694,#305695,#305696),(#305697,#305698,#305699),(#305700,
#305701,#305702),(#305703,#305704,#305705),(#305706,#305707,#305708),(#305709,
#305710,#305711),(#305712,#305713,#305714),(#305715,#305716,#305717),(#305718,
#305719,#305720),(#305721,#305722,#305723),(#305724,#305725,#305726),(#305727,
#305728,#305729),(#305730,#305731,#305732),(#305733,#305734,#305735),(#305736,
#305737,#305738),(#305739,#305740,#305741),(#305742,#305743,#305744),(#305745,
#305746,#305747),(#305748,#305749,#305750),(#305751,#305752,#305753),(#305754,
#305755,#305756),(#305757,#305758,#305759),(#305760,#305761,#305762),(#305763,
#305764,#305765),(#305766,#305767,#305768),(#305769,#305770,#305771),(#305772,
#305773,#305774),(#305775,#305776,#305777),(#305778,#305779,#305780),(#305781,
#305782,#305783),(#305784,#305785,#305786),(#305787,#305788,#305789),(#305790,
#305791,#305792),(#305793,#305794,#305795),(#305796,#305797,#305798),(#305799,
#305800,#305801),(#305802,#305803,#305804),(#305805,#305806,#305807),(#305808,
#305809,#305810),(#305811,#305812,#305813),(#305814,#305815,#305816),(#305817,
#305818,#305819),(#305820,#305821,#305822),(#305823,#305824,#305825),(#305826,
#305827,#305828),(#305829,#305830,#305831),(#305832,#305833,#305834),(#305835,
#305836,#305837),(#305838,#305839,#305840),(#305841,#305842,#305843),(#305844,
#305845,#305846),(#305847,#305848,#305849),(#305850,#305851,#305852),(#305853,
#305854,#305855),(#305856,#305857,#305858),(#305859,#305860,#305861),(#305862,
#305863,#305864),(#305865,#305866,#305867),(#305868,#305869,#305870),(#305871,
#305872,#305873),(#305874,#305875,#305876),(#305877,#305878,#305879),(#305880,
#305881,#305882),(#305883,#305884,#305885),(#305886,#305887,#305888),(#305889,
#305890,#305891),(#305892,#305893,#305894),(#305895,#305896,#305897),(#305898,
#305899,#305900),(#305901,#305902,#305903),(#305904,#305905,#305906),(#305907,
#305908,#305909),(#305910,#305911,#305912),(#305913,#305914,#305915),(#305916,
#305917,#305918),(#305919,#305920,#305921),(#305922,#305923,#305924),(#305925,
#305926,#305927),(#305928,#305929,#305930),(#305931,#305932,#305933),(#305934,
#305935,#305936),(#305937,#305938,#305939),(#305940,#305941,#305942),(#305943,
#305944,#305945),(#305946,#305947,#305948),(#305949,#305950,#305951),(#305952,
#305953,#305954),(#305955,#305956,#305957),(#305958,#305959,#305960),(#305961,
#305962,#305963),(#305964,#305965,#305966),(#305967,#305968,#305969),(#305970,
#305971,#305972),(#305973,#305974,#305975),(#305976,#305977,#305978),(#305979,
#305980,#305981),(#305982,#305983,#305984),(#305985,#305986,#305987),(#305988,
#305989,#305990),(#305991,#305992,#305993),(#305994,#305995,#305996),(#305997,
#305998,#305999),(#306000,#306001,#306002),(#306003,#306004,#306005),(#306006,
#306007,#306008),(#306009,#306010,#306011),(#306012,#306013,#306014),(#306015,
#306016,#306017),(#306018,#306019,#306020),(#306021,#306022,#306023),(#306024,
#306025,#306026),(#306027,#306028,#306029),(#306030,#306031,#306032),(#306033,
#306034,#306035),(#306036,#306037,#306038),(#306039,#306040,#306041),(#306042,
#306043,#306044),(#306045,#306046,#306047),(#306048,#306049,#306050),(#306051,
#306052,#306053),(#306054,#306055,#306056),(#306057,#306058,#306059),(#306060,
#306061,#306062),(#306063,#306064,#306065),(#306066,#306067,#306068),(#306069,
#306070,#306071),(#306072,#306073,#306074),(#306075,#306076,#306077),(#306078,
#306079,#306080),(#306081,#306082,#306083),(#306084,#306085,#306086),(#306087,
#306088,#306089),(#306090,#306091,#306092),(#306093,#306094,#306095),(#306096,
#306097,#306098),(#306099,#306100,#306101),(#306102,#306103,#306104),(#306105,
#306106,#306107),(#306108,#306109,#306110),(#306111,#306112,#306113),(#306114,
#306115,#306116),(#306117,#306118,#306119),(#306120,#306121,#306122),(#306123,
#306124,#306125),(#306126,#306127,#306128),(#306129,#306130,#306131),(#306132,
#306133,#306134),(#306135,#306136,#306137),(#306138,#306139,#306140),(#306141,
#306142,#306143),(#306144,#306145,#306146),(#306147,#306148,#306149),(#306150,
#306151,#306152),(#306153,#306154,#306155),(#306156,#306157,#306158),(#306159,
#306160,#306161),(#306162,#306163,#306164),(#306165,#306166,#306167),(#306168,
#306169,#306170),(#306171,#306172,#306173),(#306174,#306175,#306176),(#306177,
#306178,#306179),(#306180,#306181,#306182),(#306183,#306184,#306185),(#306186,
#306187,#306188),(#306189,#306190,#306191),(#306192,#306193,#306194),(#306195,
#306196,#306197),(#306198,#306199,#306200),(#306201,#306202,#306203),(#306204,
#306205,#306206),(#306207,#306208,#306209),(#306210,#306211,#306212),(#306213,
#306214,#306215),(#306216,#306217,#306218),(#306219,#306220,#306221),(#306222,
#306223,#306224),(#306225,#306226,#306227),(#306228,#306229,#306230),(#306231,
#306232,#306233),(#306234,#306235,#306236),(#306237,#306238,#306239),(#306240,
#306241,#306242),(#306243,#306244,#306245),(#306246,#306247,#306248),(#306249,
#306250,#306251),(#306252,#306253,#306254),(#306255,#306256,#306257),(#306258,
#306259,#306260),(#306261,#306262,#306263),(#306264,#306265,#306266),(#306267,
#306268,#306269),(#306270,#306271,#306272),(#306273,#306274,#306275),(#306276,
#306277,#306278),(#306279,#306280,#306281),(#306282,#306283,#306284)),
 .UNSPECIFIED.,.F.,.F.,.F.,(6,1,1,1,1,1,1,1,1,1,1,1,1,1,1,1,1,1,1,1,1,1,
1,1,1,1,1,1,1,1,1,1,1,1,1,1,1,1,1,1,1,1,1,1,1,1,1,1,1,1,1,1,1,1,1,1,1,1,
1,1,1,1,1,1,1,1,1,1,1,1,1,1,1,1,1,1,1,1,1,1,1,1,1,1,1,1,1,1,1,1,1,1,1,1,
1,1,1,1,1,1,1,1,1,1,1,1,1,1,1,1,1,1,1,1,1,1,1,1,1,1,1,1,1,1,1,1,1,1,1,1,
1,1,1,1,1,1,1,1,1,1,1,1,1,1,1,1,1,1,1,1,1,1,1,1,1,1,1,1,1,1,1,1,1,1,1,1,
1,1,1,1,1,1,1,1,1,1,1,1,1,1,1,1,1,1,1,1,1,1,1,1,1,1,1,1,1,1,1,1,1,1,1,1,
1,1,1,1,1,1,1,1,1,1,1,1,1,1,1,1,1,1,1,1,1,1,1,1,1,1,1,1,1,1,1,1,1,1,1,1,
1,1,1,1,1,1,1,1,1,1,1,1,1,1,1,1,1,1,1,1,1,1,1,1,1,1,1,1,1,1,1,1,1,1,1,1,
1,1,1,1,1,1,1,1,1,1,1,1,1,1,1,1,1,1,1,1,1,1,1,1,1,1,1,1,1,1,1,1,1,1,1,1,
1,1,1,1,1,1,1,1,1,1,1,1,1,1,1,1,1,1,1,1,1,1,1,1,1,1,1,1,1,1,1,1,1,1,1,1,
1,1,1,1,1,1,1,1,1,1,1,1,1,1,1,1,1,1,1,1,1,1,1,1,1,1,1,1,1,1,1,1,1,1,1,1,
1,1,1,1,1,1,1,1,1,1,1,1,1,1,1,1,1,1,1,1,1,1,1,1,1,1,1,1,1,1,1,1,1,1,1,1,
1,1,1,1,1,1,1,1,1,1,1,1,1,1,1,1,1,1,1,1,1,1,1,1,1,1,1,1,1,1,1,1,1,1,1,1,
1,1,1,1,1,1,1,1,1,1,1,1,1,1,1,1,1,1,1,1,1,1,1,1,1,1,1,1,1,1,1,1,1,1,1,1,
1,1,1,1,1,1,1,1,1,1,1,1,1,1,1,1,1,1,1,1,1,1,1,1,1,1,1,1,1,1,1,1,1,1,1,1,
1,1,1,1,1,1,1,1,1,1,1,1,1,1,1,1,1,1,1,6),(2,1,2),(-1.,-0.998165138,-0.996330275,
-0.994495413,-0.99266055,-0.990825688,-0.988990826,-0.987155963,-0.985321101,
-0.983486239,-0.981651376,-0.979816514,-0.977981651,-0.976146789,-0.974311927,
-0.972477064,-0.970642202,-0.968807339,-0.966972477,-0.965137615,-0.963302752,
-0.96146789,-0.959633028,-0.957798165,-0.955963303,-0.95412844,-0.952293578,
-0.950458716,-0.948623853,-0.946788991,-0.944954128,-0.943119266,-0.941284404,
-0.939449541,-0.937614679,-0.935779817,-0.933944954,-0.932110092,-0.930275229,
-0.928440367,-0.926605505,-0.924770642,-0.92293578,-0.921100917,-0.919266055,
-0.917431193,-0.91559633,-0.913761468,-0.911926606,-0.910091743,-0.908256881,
-0.906422018,-0.904587156,-0.902752294,-0.900917431,-0.899082569,-0.897247706,
-0.895412844,-0.893577982,-0.891743119,-0.889908257,-0.888073394,-0.886238532,
-0.88440367,-0.882568807,-0.880733945,-0.878899083,-0.87706422,-0.875229358,
-0.873394495,-0.871559633,-0.869724771,-0.867889908,-0.866055046,-0.864220183,
-0.862385321,-0.860550459,-0.858715596,-0.856880734,-0.855045872,-0.853211009,
-0.851376147,-0.849541284,-0.847706422,-0.84587156,-0.844036697,-0.842201835,
-0.840366972,-0.83853211,-0.836697248,-0.834862385,-0.833027523,-0.831192661,
-0.829357798,-0.827522936,-0.825688073,-0.823853211,-0.822018349,-0.820183486,
-0.818348624,-0.816513761,-0.814678899,-0.812844037,-0.811009174,-0.809174312,
-0.80733945,-0.805504587,-0.803669725,-0.801834862,-0.8,-0.798165138,-0.796330275,
-0.794495413,-0.79266055,-0.790825688,-0.788990826,-0.787155963,-0.785321101,
-0.783486239,-0.781651376,-0.779816514,-0.777981651,-0.776146789,-0.774311927,
-0.772477064,-0.770642202,-0.768807339,-0.766972477,-0.765137615,-0.763302752,
-0.76146789,-0.759633028,-0.757798165,-0.755963303,-0.75412844,-0.752293578,
-0.750458716,-0.748623853,-0.746788991,-0.744954128,-0.743119266,-0.741284404,
-0.739449541,-0.737614679,-0.735779817,-0.733944954,-0.732110092,-0.730275229,
-0.728440367,-0.726605505,-0.724770642,-0.72293578,-0.721100917,-0.719266055,
-0.717431193,-0.71559633,-0.713761468,-0.711926606,-0.710091743,-0.708256881,
-0.706422018,-0.704587156,-0.702752294,-0.700917431,-0.699082569,-0.697247706,
-0.695412844,-0.693577982,-0.691743119,-0.689908257,-0.688073394,-0.686238532,
-0.68440367,-0.682568807,-0.680733945,-0.678899083,-0.67706422,-0.675229358,
-0.673394495,-0.671559633,-0.669724771,-0.667889908,-0.666055046,-0.664220183,
-0.662385321,-0.660550459,-0.658715596,-0.656880734,-0.655045872,-0.653211009,
-0.651376147,-0.649541284,-0.647706422,-0.64587156,-0.644036697,-0.642201835,
-0.640366972,-0.63853211,-0.636697248,-0.634862385,-0.633027523,-0.631192661,
-0.629357798,-0.627522936,-0.625688073,-0.623853211,-0.622018349,-0.620183486,
-0.618348624,-0.616513761,-0.614678899,-0.612844037,-0.611009174,-0.609174312,
-0.60733945,-0.605504587,-0.603669725,-0.601834862,-0.6,-0.598165138,-0.596330275,
-0.594495413,-0.59266055,-0.590825688,-0.588990826,-0.587155963,-0.585321101,
-0.583486239,-0.581651376,-0.579816514,-0.577981651,-0.576146789,-0.574311927,
-0.572477064,-0.570642202,-0.568807339,-0.566972477,-0.565137615,-0.563302752,
-0.56146789,-0.559633028,-0.557798165,-0.555963303,-0.55412844,-0.552293578,
-0.550458716,-0.548623853,-0.546788991,-0.544954128,-0.543119266,-0.541284404,
-0.539449541,-0.537614679,-0.535779817,-0.533944954,-0.532110092,-0.530275229,
-0.528440367,-0.526605505,-0.524770642,-0.52293578,-0.521100917,-0.519266055,
-0.517431193,-0.51559633,-0.513761468,-0.511926606,-0.510091743,-0.508256881,
-0.506422018,-0.504587156,-0.502752294,-0.500917431,-0.499082569,-0.497247706,
-0.495412844,-0.493577982,-0.491743119,-0.489908257,-0.488073394,-0.486238532,
-0.48440367,-0.482568807,-0.480733945,-0.478899083,-0.47706422,-0.475229358,
-0.473394495,-0.471559633,-0.469724771,-0.467889908,-0.466055046,-0.464220183,
-0.462385321,-0.460550459,-0.458715596,-0.456880734,-0.455045872,-0.453211009,
-0.451376147,-0.449541284,-0.447706422,-0.44587156,-0.444036697,-0.442201835,
-0.440366972,-0.43853211,-0.436697248,-0.434862385,-0.433027523,-0.431192661,
-0.429357798,-0.427522936,-0.425688073,-0.423853211,-0.422018349,-0.420183486,
-0.418348624,-0.416513761,-0.414678899,-0.412844037,-0.411009174,-0.409174312,
-0.40733945,-0.405504587,-0.403669725,-0.401834862,-0.4,-0.398165138,-0.396330275,
-0.394495413,-0.39266055,-0.390825688,-0.388990826,-0.387155963,-0.385321101,
-0.383486239,-0.381651376,-0.379816514,-0.377981651,-0.376146789,-0.374311927,
-0.372477064,-0.370642202,-0.368807339,-0.366972477,-0.365137615,-0.363302752,
-0.36146789,-0.359633028,-0.357798165,-0.355963303,-0.35412844,-0.352293578,
-0.350458716,-0.348623853,-0.346788991,-0.344954128,-0.343119266,-0.341284404,
-0.339449541,-0.337614679,-0.335779817,-0.333944954,-0.332110092,-0.330275229,
-0.328440367,-0.326605505,-0.324770642,-0.32293578,-0.321100917,-0.319266055,
-0.317431193,-0.31559633,-0.313761468,-0.311926606,-0.310091743,-0.308256881,
-0.306422018,-0.304587156,-0.302752294,-0.300917431,-0.299082569,-0.297247706,
-0.295412844,-0.293577982,-0.291743119,-0.289908257,-0.288073394,-0.286238532,
-0.28440367,-0.282568807,-0.280733945,-0.278899083,-0.27706422,-0.275229358,
-0.273394495,-0.271559633,-0.269724771,-0.267889908,-0.266055046,-0.264220183,
-0.262385321,-0.260550459,-0.258715596,-0.256880734,-0.255045872,-0.253211009,
-0.251376147,-0.249541284,-0.247706422,-0.24587156,-0.244036697,-0.242201835,
-0.240366972,-0.23853211,-0.236697248,-0.234862385,-0.233027523,-0.231192661,
-0.229357798,-0.227522936,-0.225688073,-0.223853211,-0.222018349,-0.220183486,
-0.218348624,-0.216513761,-0.214678899,-0.212844037,-0.211009174,-0.209174312,
-0.20733945,-0.205504587,-0.203669725,-0.201834862,-0.2,-0.198165138,-0.196330275,
-0.194495413,-0.19266055,-0.190825688,-0.188990826,-0.187155963,-0.185321101,
-0.183486239,-0.181651376,-0.179816514,-0.177981651,-0.176146789,-0.174311927,
-0.172477064,-0.170642202,-0.168807339,-0.166972477,-0.165137615,-0.163302752,
-0.16146789,-0.159633028,-0.157798165,-0.155963303,-0.15412844,-0.152293578,
-0.150458716,-0.148623853,-0.146788991,-0.144954128,-0.143119266,-0.141284404,
-0.139449541,-0.137614679,-0.135779817,-0.133944954,-0.132110092,-0.130275229,
-0.128440367,-0.126605505,-0.124770642,-0.12293578,-0.121100917,-0.119266055,
-0.117431193,-0.11559633,-0.113761468,-0.111926606,-0.110091743,-0.108256881,
-0.106422018,-0.104587156,-0.102752294,-0.100917431,-0.099082569,-0.097247706,
-0.095412844,-0.093577982,-0.091743119,-0.089908257,-0.088073394,-0.086238532,
-0.08440367,-0.082568807,-0.080733945,-0.078899083,-0.07706422,-0.075229358,
-0.073394495,-0.071559633,-0.069724771,-0.067889908,-0.066055046,-0.064220183,
-0.062385321,-0.060550459,-0.058715596,-0.056880734,-0.055045872,-0.053211009,
-0.051376147,-0.049541284,-0.047706422,-0.04587156,-0.044036697,-0.042201835,
-0.040366972,-0.03853211,-0.036697248,-0.034862385,-0.033027523,-0.031192661,
-0.029357798,-0.027522936,-0.025688073,-0.023853211,-0.022018349,-0.020183486,
-0.018348624,-0.016513761,-0.014678899,-0.012844037,-0.011009174,-0.009174312,
-0.00733945,-0.005504587,-0.003669725,-0.001834862,0.000982135),(0.3,1.,
1.3),.UNSPECIFIED.);
#6306=B_SPLINE_SURFACE_WITH_KNOTS('',5,1,((#306307,#306308,#306309),(#306310,
#306311,#306312),(#306313,#306314,#306315),(#306316,#306317,#306318),(#306319,
#306320,#306321),(#306322,#306323,#306324),(#306325,#306326,#306327),(#306328,
#306329,#306330),(#306331,#306332,#306333),(#306334,#306335,#306336),(#306337,
#306338,#306339),(#306340,#306341,#306342),(#306343,#306344,#306345),(#306346,
#306347,#306348),(#306349,#306350,#306351),(#306352,#306353,#306354),(#306355,
#306356,#306357),(#306358,#306359,#306360),(#306361,#306362,#306363),(#306364,
#306365,#306366),(#306367,#306368,#306369),(#306370,#306371,#306372),(#306373,
#306374,#306375),(#306376,#306377,#306378),(#306379,#306380,#306381),(#306382,
#306383,#306384),(#306385,#306386,#306387),(#306388,#306389,#306390),(#306391,
#306392,#306393),(#306394,#306395,#306396),(#306397,#306398,#306399),(#306400,
#306401,#306402),(#306403,#306404,#306405),(#306406,#306407,#306408),(#306409,
#306410,#306411),(#306412,#306413,#306414),(#306415,#306416,#306417),(#306418,
#306419,#306420),(#306421,#306422,#306423),(#306424,#306425,#306426),(#306427,
#306428,#306429),(#306430,#306431,#306432),(#306433,#306434,#306435),(#306436,
#306437,#306438),(#306439,#306440,#306441),(#306442,#306443,#306444),(#306445,
#306446,#306447),(#306448,#306449,#306450),(#306451,#306452,#306453),(#306454,
#306455,#306456),(#306457,#306458,#306459),(#306460,#306461,#306462),(#306463,
#306464,#306465),(#306466,#306467,#306468),(#306469,#306470,#306471),(#306472,
#306473,#306474),(#306475,#306476,#306477),(#306478,#306479,#306480),(#306481,
#306482,#306483),(#306484,#306485,#306486),(#306487,#306488,#306489),(#306490,
#306491,#306492),(#306493,#306494,#306495),(#306496,#306497,#306498),(#306499,
#306500,#306501),(#306502,#306503,#306504),(#306505,#306506,#306507),(#306508,
#306509,#306510),(#306511,#306512,#306513),(#306514,#306515,#306516),(#306517,
#306518,#306519),(#306520,#306521,#306522),(#306523,#306524,#306525),(#306526,
#306527,#306528),(#306529,#306530,#306531),(#306532,#306533,#306534),(#306535,
#306536,#306537),(#306538,#306539,#306540),(#306541,#306542,#306543),(#306544,
#306545,#306546),(#306547,#306548,#306549),(#306550,#306551,#306552),(#306553,
#306554,#306555),(#306556,#306557,#306558),(#306559,#306560,#306561),(#306562,
#306563,#306564),(#306565,#306566,#306567),(#306568,#306569,#306570),(#306571,
#306572,#306573),(#306574,#306575,#306576),(#306577,#306578,#306579),(#306580,
#306581,#306582),(#306583,#306584,#306585),(#306586,#306587,#306588),(#306589,
#306590,#306591),(#306592,#306593,#306594),(#306595,#306596,#306597),(#306598,
#306599,#306600),(#306601,#306602,#306603),(#306604,#306605,#306606),(#306607,
#306608,#306609),(#306610,#306611,#306612),(#306613,#306614,#306615),(#306616,
#306617,#306618),(#306619,#306620,#306621),(#306622,#306623,#306624),(#306625,
#306626,#306627),(#306628,#306629,#306630),(#306631,#306632,#306633),(#306634,
#306635,#306636),(#306637,#306638,#306639),(#306640,#306641,#306642),(#306643,
#306644,#306645),(#306646,#306647,#306648),(#306649,#306650,#306651),(#306652,
#306653,#306654),(#306655,#306656,#306657),(#306658,#306659,#306660),(#306661,
#306662,#306663),(#306664,#306665,#306666),(#306667,#306668,#306669),(#306670,
#306671,#306672),(#306673,#306674,#306675),(#306676,#306677,#306678),(#306679,
#306680,#306681),(#306682,#306683,#306684),(#306685,#306686,#306687),(#306688,
#306689,#306690),(#306691,#306692,#306693),(#306694,#306695,#306696),(#306697,
#306698,#306699),(#306700,#306701,#306702),(#306703,#306704,#306705),(#306706,
#306707,#306708),(#306709,#306710,#306711),(#306712,#306713,#306714),(#306715,
#306716,#306717),(#306718,#306719,#306720),(#306721,#306722,#306723),(#306724,
#306725,#306726),(#306727,#306728,#306729),(#306730,#306731,#306732),(#306733,
#306734,#306735),(#306736,#306737,#306738),(#306739,#306740,#306741),(#306742,
#306743,#306744),(#306745,#306746,#306747),(#306748,#306749,#306750),(#306751,
#306752,#306753),(#306754,#306755,#306756),(#306757,#306758,#306759),(#306760,
#306761,#306762),(#306763,#306764,#306765),(#306766,#306767,#306768),(#306769,
#306770,#306771),(#306772,#306773,#306774),(#306775,#306776,#306777),(#306778,
#306779,#306780),(#306781,#306782,#306783),(#306784,#306785,#306786),(#306787,
#306788,#306789),(#306790,#306791,#306792),(#306793,#306794,#306795),(#306796,
#306797,#306798),(#306799,#306800,#306801),(#306802,#306803,#306804),(#306805,
#306806,#306807),(#306808,#306809,#306810),(#306811,#306812,#306813),(#306814,
#306815,#306816),(#306817,#306818,#306819),(#306820,#306821,#306822),(#306823,
#306824,#306825),(#306826,#306827,#306828),(#306829,#306830,#306831),(#306832,
#306833,#306834),(#306835,#306836,#306837),(#306838,#306839,#306840),(#306841,
#306842,#306843),(#306844,#306845,#306846),(#306847,#306848,#306849),(#306850,
#306851,#306852),(#306853,#306854,#306855),(#306856,#306857,#306858),(#306859,
#306860,#306861),(#306862,#306863,#306864),(#306865,#306866,#306867),(#306868,
#306869,#306870),(#306871,#306872,#306873),(#306874,#306875,#306876),(#306877,
#306878,#306879),(#306880,#306881,#306882),(#306883,#306884,#306885),(#306886,
#306887,#306888),(#306889,#306890,#306891),(#306892,#306893,#306894),(#306895,
#306896,#306897),(#306898,#306899,#306900),(#306901,#306902,#306903),(#306904,
#306905,#306906),(#306907,#306908,#306909),(#306910,#306911,#306912),(#306913,
#306914,#306915),(#306916,#306917,#306918),(#306919,#306920,#306921),(#306922,
#306923,#306924),(#306925,#306926,#306927),(#306928,#306929,#306930),(#306931,
#306932,#306933),(#306934,#306935,#306936),(#306937,#306938,#306939),(#306940,
#306941,#306942),(#306943,#306944,#306945),(#306946,#306947,#306948),(#306949,
#306950,#306951),(#306952,#306953,#306954),(#306955,#306956,#306957),(#306958,
#306959,#306960),(#306961,#306962,#306963),(#306964,#306965,#306966),(#306967,
#306968,#306969),(#306970,#306971,#306972),(#306973,#306974,#306975),(#306976,
#306977,#306978),(#306979,#306980,#306981),(#306982,#306983,#306984),(#306985,
#306986,#306987),(#306988,#306989,#306990),(#306991,#306992,#306993),(#306994,
#306995,#306996),(#306997,#306998,#306999),(#307000,#307001,#307002),(#307003,
#307004,#307005),(#307006,#307007,#307008),(#307009,#307010,#307011),(#307012,
#307013,#307014),(#307015,#307016,#307017),(#307018,#307019,#307020),(#307021,
#307022,#307023),(#307024,#307025,#307026),(#307027,#307028,#307029),(#307030,
#307031,#307032),(#307033,#307034,#307035),(#307036,#307037,#307038),(#307039,
#307040,#307041),(#307042,#307043,#307044),(#307045,#307046,#307047),(#307048,
#307049,#307050),(#307051,#307052,#307053),(#307054,#307055,#307056),(#307057,
#307058,#307059),(#307060,#307061,#307062),(#307063,#307064,#307065),(#307066,
#307067,#307068),(#307069,#307070,#307071),(#307072,#307073,#307074),(#307075,
#307076,#307077),(#307078,#307079,#307080),(#307081,#307082,#307083),(#307084,
#307085,#307086),(#307087,#307088,#307089),(#307090,#307091,#307092),(#307093,
#307094,#307095),(#307096,#307097,#307098),(#307099,#307100,#307101),(#307102,
#307103,#307104),(#307105,#307106,#307107),(#307108,#307109,#307110),(#307111,
#307112,#307113),(#307114,#307115,#307116),(#307117,#307118,#307119),(#307120,
#307121,#307122),(#307123,#307124,#307125),(#307126,#307127,#307128),(#307129,
#307130,#307131),(#307132,#307133,#307134),(#307135,#307136,#307137),(#307138,
#307139,#307140),(#307141,#307142,#307143),(#307144,#307145,#307146),(#307147,
#307148,#307149),(#307150,#307151,#307152),(#307153,#307154,#307155),(#307156,
#307157,#307158),(#307159,#307160,#307161),(#307162,#307163,#307164),(#307165,
#307166,#307167),(#307168,#307169,#307170),(#307171,#307172,#307173),(#307174,
#307175,#307176),(#307177,#307178,#307179),(#307180,#307181,#307182),(#307183,
#307184,#307185),(#307186,#307187,#307188),(#307189,#307190,#307191),(#307192,
#307193,#307194),(#307195,#307196,#307197),(#307198,#307199,#307200),(#307201,
#307202,#307203),(#307204,#307205,#307206),(#307207,#307208,#307209),(#307210,
#307211,#307212),(#307213,#307214,#307215),(#307216,#307217,#307218),(#307219,
#307220,#307221),(#307222,#307223,#307224),(#307225,#307226,#307227),(#307228,
#307229,#307230),(#307231,#307232,#307233),(#307234,#307235,#307236),(#307237,
#307238,#307239),(#307240,#307241,#307242),(#307243,#307244,#307245),(#307246,
#307247,#307248),(#307249,#307250,#307251),(#307252,#307253,#307254),(#307255,
#307256,#307257),(#307258,#307259,#307260),(#307261,#307262,#307263),(#307264,
#307265,#307266),(#307267,#307268,#307269),(#307270,#307271,#307272),(#307273,
#307274,#307275),(#307276,#307277,#307278),(#307279,#307280,#307281),(#307282,
#307283,#307284),(#307285,#307286,#307287),(#307288,#307289,#307290),(#307291,
#307292,#307293),(#307294,#307295,#307296),(#307297,#307298,#307299),(#307300,
#307301,#307302),(#307303,#307304,#307305),(#307306,#307307,#307308),(#307309,
#307310,#307311),(#307312,#307313,#307314),(#307315,#307316,#307317),(#307318,
#307319,#307320),(#307321,#307322,#307323),(#307324,#307325,#307326),(#307327,
#307328,#307329),(#307330,#307331,#307332),(#307333,#307334,#307335),(#307336,
#307337,#307338),(#307339,#307340,#307341),(#307342,#307343,#307344),(#307345,
#307346,#307347),(#307348,#307349,#307350),(#307351,#307352,#307353),(#307354,
#307355,#307356),(#307357,#307358,#307359),(#307360,#307361,#307362),(#307363,
#307364,#307365),(#307366,#307367,#307368),(#307369,#307370,#307371),(#307372,
#307373,#307374),(#307375,#307376,#307377),(#307378,#307379,#307380),(#307381,
#307382,#307383),(#307384,#307385,#307386),(#307387,#307388,#307389),(#307390,
#307391,#307392),(#307393,#307394,#307395),(#307396,#307397,#307398),(#307399,
#307400,#307401),(#307402,#307403,#307404),(#307405,#307406,#307407),(#307408,
#307409,#307410),(#307411,#307412,#307413),(#307414,#307415,#307416),(#307417,
#307418,#307419),(#307420,#307421,#307422),(#307423,#307424,#307425),(#307426,
#307427,#307428),(#307429,#307430,#307431),(#307432,#307433,#307434),(#307435,
#307436,#307437),(#307438,#307439,#307440),(#307441,#307442,#307443),(#307444,
#307445,#307446),(#307447,#307448,#307449),(#307450,#307451,#307452),(#307453,
#307454,#307455),(#307456,#307457,#307458),(#307459,#307460,#307461),(#307462,
#307463,#307464),(#307465,#307466,#307467),(#307468,#307469,#307470),(#307471,
#307472,#307473),(#307474,#307475,#307476),(#307477,#307478,#307479),(#307480,
#307481,#307482),(#307483,#307484,#307485),(#307486,#307487,#307488),(#307489,
#307490,#307491),(#307492,#307493,#307494),(#307495,#307496,#307497),(#307498,
#307499,#307500),(#307501,#307502,#307503),(#307504,#307505,#307506),(#307507,
#307508,#307509),(#307510,#307511,#307512),(#307513,#307514,#307515),(#307516,
#307517,#307518),(#307519,#307520,#307521),(#307522,#307523,#307524),(#307525,
#307526,#307527),(#307528,#307529,#307530),(#307531,#307532,#307533),(#307534,
#307535,#307536),(#307537,#307538,#307539),(#307540,#307541,#307542),(#307543,
#307544,#307545),(#307546,#307547,#307548),(#307549,#307550,#307551),(#307552,
#307553,#307554),(#307555,#307556,#307557),(#307558,#307559,#307560),(#307561,
#307562,#307563),(#307564,#307565,#307566),(#307567,#307568,#307569),(#307570,
#307571,#307572),(#307573,#307574,#307575),(#307576,#307577,#307578),(#307579,
#307580,#307581),(#307582,#307583,#307584),(#307585,#307586,#307587),(#307588,
#307589,#307590),(#307591,#307592,#307593),(#307594,#307595,#307596),(#307597,
#307598,#307599),(#307600,#307601,#307602),(#307603,#307604,#307605),(#307606,
#307607,#307608),(#307609,#307610,#307611),(#307612,#307613,#307614),(#307615,
#307616,#307617),(#307618,#307619,#307620),(#307621,#307622,#307623),(#307624,
#307625,#307626),(#307627,#307628,#307629),(#307630,#307631,#307632),(#307633,
#307634,#307635),(#307636,#307637,#307638),(#307639,#307640,#307641),(#307642,
#307643,#307644),(#307645,#307646,#307647),(#307648,#307649,#307650),(#307651,
#307652,#307653),(#307654,#307655,#307656),(#307657,#307658,#307659),(#307660,
#307661,#307662),(#307663,#307664,#307665),(#307666,#307667,#307668),(#307669,
#307670,#307671),(#307672,#307673,#307674),(#307675,#307676,#307677),(#307678,
#307679,#307680),(#307681,#307682,#307683),(#307684,#307685,#307686),(#307687,
#307688,#307689),(#307690,#307691,#307692),(#307693,#307694,#307695),(#307696,
#307697,#307698),(#307699,#307700,#307701),(#307702,#307703,#307704),(#307705,
#307706,#307707),(#307708,#307709,#307710),(#307711,#307712,#307713),(#307714,
#307715,#307716),(#307717,#307718,#307719),(#307720,#307721,#307722),(#307723,
#307724,#307725),(#307726,#307727,#307728),(#307729,#307730,#307731),(#307732,
#307733,#307734),(#307735,#307736,#307737),(#307738,#307739,#307740),(#307741,
#307742,#307743),(#307744,#307745,#307746),(#307747,#307748,#307749),(#307750,
#307751,#307752),(#307753,#307754,#307755),(#307756,#307757,#307758),(#307759,
#307760,#307761),(#307762,#307763,#307764),(#307765,#307766,#307767),(#307768,
#307769,#307770),(#307771,#307772,#307773),(#307774,#307775,#307776),(#307777,
#307778,#307779),(#307780,#307781,#307782),(#307783,#307784,#307785),(#307786,
#307787,#307788),(#307789,#307790,#307791),(#307792,#307793,#307794),(#307795,
#307796,#307797),(#307798,#307799,#307800),(#307801,#307802,#307803),(#307804,
#307805,#307806),(#307807,#307808,#307809),(#307810,#307811,#307812),(#307813,
#307814,#307815),(#307816,#307817,#307818),(#307819,#307820,#307821),(#307822,
#307823,#307824),(#307825,#307826,#307827),(#307828,#307829,#307830),(#307831,
#307832,#307833),(#307834,#307835,#307836),(#307837,#307838,#307839),(#307840,
#307841,#307842),(#307843,#307844,#307845),(#307846,#307847,#307848),(#307849,
#307850,#307851),(#307852,#307853,#307854),(#307855,#307856,#307857),(#307858,
#307859,#307860),(#307861,#307862,#307863),(#307864,#307865,#307866),(#307867,
#307868,#307869),(#307870,#307871,#307872),(#307873,#307874,#307875),(#307876,
#307877,#307878),(#307879,#307880,#307881),(#307882,#307883,#307884),(#307885,
#307886,#307887),(#307888,#307889,#307890),(#307891,#307892,#307893),(#307894,
#307895,#307896),(#307897,#307898,#307899),(#307900,#307901,#307902),(#307903,
#307904,#307905),(#307906,#307907,#307908),(#307909,#307910,#307911),(#307912,
#307913,#307914),(#307915,#307916,#307917),(#307918,#307919,#307920),(#307921,
#307922,#307923),(#307924,#307925,#307926),(#307927,#307928,#307929),(#307930,
#307931,#307932),(#307933,#307934,#307935),(#307936,#307937,#307938),(#307939,
#307940,#307941),(#307942,#307943,#307944),(#307945,#307946,#307947),(#307948,
#307949,#307950),(#307951,#307952,#307953),(#307954,#307955,#307956),(#307957,
#307958,#307959)),.UNSPECIFIED.,.F.,.F.,.F.,(6,1,1,1,1,1,1,1,1,1,1,1,1,
1,1,1,1,1,1,1,1,1,1,1,1,1,1,1,1,1,1,1,1,1,1,1,1,1,1,1,1,1,1,1,1,1,1,1,1,
1,1,1,1,1,1,1,1,1,1,1,1,1,1,1,1,1,1,1,1,1,1,1,1,1,1,1,1,1,1,1,1,1,1,1,1,
1,1,1,1,1,1,1,1,1,1,1,1,1,1,1,1,1,1,1,1,1,1,1,1,1,1,1,1,1,1,1,1,1,1,1,1,
1,1,1,1,1,1,1,1,1,1,1,1,1,1,1,1,1,1,1,1,1,1,1,1,1,1,1,1,1,1,1,1,1,1,1,1,
1,1,1,1,1,1,1,1,1,1,1,1,1,1,1,1,1,1,1,1,1,1,1,1,1,1,1,1,1,1,1,1,1,1,1,1,
1,1,1,1,1,1,1,1,1,1,1,1,1,1,1,1,1,1,1,1,1,1,1,1,1,1,1,1,1,1,1,1,1,1,1,1,
1,1,1,1,1,1,1,1,1,1,1,1,1,1,1,1,1,1,1,1,1,1,1,1,1,1,1,1,1,1,1,1,1,1,1,1,
1,1,1,1,1,1,1,1,1,1,1,1,1,1,1,1,1,1,1,1,1,1,1,1,1,1,1,1,1,1,1,1,1,1,1,1,
1,1,1,1,1,1,1,1,1,1,1,1,1,1,1,1,1,1,1,1,1,1,1,1,1,1,1,1,1,1,1,1,1,1,1,1,
1,1,1,1,1,1,1,1,1,1,1,1,1,1,1,1,1,1,1,1,1,1,1,1,1,1,1,1,1,1,1,1,1,1,1,1,
1,1,1,1,1,1,1,1,1,1,1,1,1,1,1,1,1,1,1,1,1,1,1,1,1,1,1,1,1,1,1,1,1,1,1,1,
1,1,1,1,1,1,1,1,1,1,1,1,1,1,1,1,1,1,1,1,1,1,1,1,1,1,1,1,1,1,1,1,1,1,1,1,
1,1,1,1,1,1,1,1,1,1,1,1,1,1,1,1,1,1,1,1,1,1,1,1,1,1,1,1,1,1,1,1,1,1,1,1,
1,1,1,1,1,1,1,1,1,1,1,1,1,1,1,1,1,1,1,1,1,1,1,1,1,1,1,1,1,1,1,1,1,1,1,1,
1,1,1,1,1,1,1,1,1,1,1,1,1,1,1,1,1,1,1,1,1,1,1,1,1,1,1,1,1,6),(2,1,2),(-0.001964191,
0.,0.001834862,0.003669725,0.005504587,0.00733945,0.009174312,0.011009174,
0.012844037,0.014678899,0.016513761,0.018348624,0.020183486,0.022018349,
0.023853211,0.025688073,0.027522936,0.029357798,0.031192661,0.033027523,
0.034862385,0.036697248,0.03853211,0.040366972,0.042201835,0.044036697,
0.04587156,0.047706422,0.049541284,0.051376147,0.053211009,0.055045872,
0.056880734,0.058715596,0.060550459,0.062385321,0.064220183,0.066055046,
0.067889908,0.069724771,0.071559633,0.073394495,0.075229358,0.07706422,
0.078899083,0.080733945,0.082568807,0.08440367,0.086238532,0.088073394,
0.089908257,0.091743119,0.093577982,0.095412844,0.097247706,0.099082569,
0.100917431,0.102752294,0.104587156,0.106422018,0.108256881,0.110091743,
0.111926606,0.113761468,0.11559633,0.117431193,0.119266055,0.121100917,
0.12293578,0.124770642,0.126605505,0.128440367,0.130275229,0.132110092,
0.133944954,0.135779817,0.137614679,0.139449541,0.141284404,0.143119266,
0.144954128,0.146788991,0.148623853,0.150458716,0.152293578,0.15412844,
0.155963303,0.157798165,0.159633028,0.16146789,0.163302752,0.165137615,
0.166972477,0.168807339,0.170642202,0.172477064,0.174311927,0.176146789,
0.177981651,0.179816514,0.181651376,0.183486239,0.185321101,0.187155963,
0.188990826,0.190825688,0.19266055,0.194495413,0.196330275,0.198165138,
0.2,0.201834862,0.203669725,0.205504587,0.20733945,0.209174312,0.211009174,
0.212844037,0.214678899,0.216513761,0.218348624,0.220183486,0.222018349,
0.223853211,0.225688073,0.227522936,0.229357798,0.231192661,0.233027523,
0.234862385,0.236697248,0.23853211,0.240366972,0.242201835,0.244036697,
0.24587156,0.247706422,0.249541284,0.251376147,0.253211009,0.255045872,
0.256880734,0.258715596,0.260550459,0.262385321,0.264220183,0.266055046,
0.267889908,0.269724771,0.271559633,0.273394495,0.275229358,0.27706422,
0.278899083,0.280733945,0.282568807,0.28440367,0.286238532,0.288073394,
0.289908257,0.291743119,0.293577982,0.295412844,0.297247706,0.299082569,
0.300917431,0.302752294,0.304587156,0.306422018,0.308256881,0.310091743,
0.311926606,0.313761468,0.31559633,0.317431193,0.319266055,0.321100917,
0.32293578,0.324770642,0.326605505,0.328440367,0.330275229,0.332110092,
0.333944954,0.335779817,0.337614679,0.339449541,0.341284404,0.343119266,
0.344954128,0.346788991,0.348623853,0.350458716,0.352293578,0.35412844,
0.355963303,0.357798165,0.359633028,0.36146789,0.363302752,0.365137615,
0.366972477,0.368807339,0.370642202,0.372477064,0.374311927,0.376146789,
0.377981651,0.379816514,0.381651376,0.383486239,0.385321101,0.387155963,
0.388990826,0.390825688,0.39266055,0.394495413,0.396330275,0.398165138,
0.4,0.401834862,0.403669725,0.405504587,0.40733945,0.409174312,0.411009174,
0.412844037,0.414678899,0.416513761,0.418348624,0.420183486,0.422018349,
0.423853211,0.425688073,0.427522936,0.429357798,0.431192661,0.433027523,
0.434862385,0.436697248,0.43853211,0.440366972,0.442201835,0.444036697,
0.44587156,0.447706422,0.449541284,0.451376147,0.453211009,0.455045872,
0.456880734,0.458715596,0.460550459,0.462385321,0.464220183,0.466055046,
0.467889908,0.469724771,0.471559633,0.473394495,0.475229358,0.47706422,
0.478899083,0.480733945,0.482568807,0.48440367,0.486238532,0.488073394,
0.489908257,0.491743119,0.493577982,0.495412844,0.497247706,0.499082569,
0.500917431,0.502752294,0.504587156,0.506422018,0.508256881,0.510091743,
0.511926606,0.513761468,0.51559633,0.517431193,0.519266055,0.521100917,
0.52293578,0.524770642,0.526605505,0.528440367,0.530275229,0.532110092,
0.533944954,0.535779817,0.537614679,0.539449541,0.541284404,0.543119266,
0.544954128,0.546788991,0.548623853,0.550458716,0.552293578,0.55412844,
0.555963303,0.557798165,0.559633028,0.56146789,0.563302752,0.565137615,
0.566972477,0.568807339,0.570642202,0.572477064,0.574311927,0.576146789,
0.577981651,0.579816514,0.581651376,0.583486239,0.585321101,0.587155963,
0.588990826,0.590825688,0.59266055,0.594495413,0.596330275,0.598165138,
0.6,0.601834862,0.603669725,0.605504587,0.60733945,0.609174312,0.611009174,
0.612844037,0.614678899,0.616513761,0.618348624,0.620183486,0.622018349,
0.623853211,0.625688073,0.627522936,0.629357798,0.631192661,0.633027523,
0.634862385,0.636697248,0.63853211,0.640366972,0.642201835,0.644036697,
0.64587156,0.647706422,0.649541284,0.651376147,0.653211009,0.655045872,
0.656880734,0.658715596,0.660550459,0.662385321,0.664220183,0.666055046,
0.667889908,0.669724771,0.671559633,0.673394495,0.675229358,0.67706422,
0.678899083,0.680733945,0.682568807,0.68440367,0.686238532,0.688073394,
0.689908257,0.691743119,0.693577982,0.695412844,0.697247706,0.699082569,
0.700917431,0.702752294,0.704587156,0.706422018,0.708256881,0.710091743,
0.711926606,0.713761468,0.71559633,0.717431193,0.719266055,0.721100917,
0.72293578,0.724770642,0.726605505,0.728440367,0.730275229,0.732110092,
0.733944954,0.735779817,0.737614679,0.739449541,0.741284404,0.743119266,
0.744954128,0.746788991,0.748623853,0.750458716,0.752293578,0.75412844,
0.755963303,0.757798165,0.759633028,0.76146789,0.763302752,0.765137615,
0.766972477,0.768807339,0.770642202,0.772477064,0.774311927,0.776146789,
0.777981651,0.779816514,0.781651376,0.783486239,0.785321101,0.787155963,
0.788990826,0.790825688,0.79266055,0.794495413,0.796330275,0.798165138,
0.8,0.801834862,0.803669725,0.805504587,0.80733945,0.809174312,0.811009174,
0.812844037,0.814678899,0.816513761,0.818348624,0.820183486,0.822018349,
0.823853211,0.825688073,0.827522936,0.829357798,0.831192661,0.833027523,
0.834862385,0.836697248,0.83853211,0.840366972,0.842201835,0.844036697,
0.84587156,0.847706422,0.849541284,0.851376147,0.853211009,0.855045872,
0.856880734,0.858715596,0.860550459,0.862385321,0.864220183,0.866055046,
0.867889908,0.869724771,0.871559633,0.873394495,0.875229358,0.87706422,
0.878899083,0.880733945,0.882568807,0.88440367,0.886238532,0.888073394,
0.889908257,0.891743119,0.893577982,0.895412844,0.897247706,0.899082569,
0.900917431,0.902752294,0.904587156,0.906422018,0.908256881,0.910091743,
0.911926606,0.913761468,0.91559633,0.917431193,0.919266055,0.921100917,
0.92293578,0.924770642,0.926605505,0.928440367,0.930275229,0.932110092,
0.933944954,0.935779817,0.937614679,0.939449541,0.941284404,0.943119266,
0.944954128,0.946788991,0.948623853,0.950458716,0.952293578,0.95412844,
0.955963303,0.957798165,0.959633028,0.96146789,0.963302752,0.965137615,
0.966972477,0.968807339,0.970642202,0.972477064,0.974311927,0.976146789,
0.977981651,0.979816514,0.981651376,0.983486239,0.985321101,0.987155963,
0.988990826,0.990825688,0.99266055,0.994495413,0.996330275,0.998165138,
1.),(0.3,1.,1.3),.UNSPECIFIED.);
#6307=B_SPLINE_SURFACE_WITH_KNOTS('',5,1,((#307978,#307979,#307980),(#307981,
#307982,#307983),(#307984,#307985,#307986),(#307987,#307988,#307989),(#307990,
#307991,#307992),(#307993,#307994,#307995),(#307996,#307997,#307998),(#307999,
#308000,#308001),(#308002,#308003,#308004),(#308005,#308006,#308007),(#308008,
#308009,#308010),(#308011,#308012,#308013),(#308014,#308015,#308016),(#308017,
#308018,#308019),(#308020,#308021,#308022),(#308023,#308024,#308025),(#308026,
#308027,#308028),(#308029,#308030,#308031),(#308032,#308033,#308034),(#308035,
#308036,#308037),(#308038,#308039,#308040),(#308041,#308042,#308043),(#308044,
#308045,#308046),(#308047,#308048,#308049),(#308050,#308051,#308052),(#308053,
#308054,#308055),(#308056,#308057,#308058),(#308059,#308060,#308061),(#308062,
#308063,#308064),(#308065,#308066,#308067),(#308068,#308069,#308070),(#308071,
#308072,#308073),(#308074,#308075,#308076),(#308077,#308078,#308079),(#308080,
#308081,#308082),(#308083,#308084,#308085),(#308086,#308087,#308088),(#308089,
#308090,#308091),(#308092,#308093,#308094),(#308095,#308096,#308097),(#308098,
#308099,#308100),(#308101,#308102,#308103),(#308104,#308105,#308106),(#308107,
#308108,#308109),(#308110,#308111,#308112),(#308113,#308114,#308115),(#308116,
#308117,#308118),(#308119,#308120,#308121),(#308122,#308123,#308124),(#308125,
#308126,#308127),(#308128,#308129,#308130),(#308131,#308132,#308133),(#308134,
#308135,#308136),(#308137,#308138,#308139),(#308140,#308141,#308142),(#308143,
#308144,#308145),(#308146,#308147,#308148),(#308149,#308150,#308151),(#308152,
#308153,#308154),(#308155,#308156,#308157),(#308158,#308159,#308160),(#308161,
#308162,#308163),(#308164,#308165,#308166),(#308167,#308168,#308169),(#308170,
#308171,#308172),(#308173,#308174,#308175),(#308176,#308177,#308178),(#308179,
#308180,#308181),(#308182,#308183,#308184),(#308185,#308186,#308187),(#308188,
#308189,#308190),(#308191,#308192,#308193),(#308194,#308195,#308196),(#308197,
#308198,#308199),(#308200,#308201,#308202),(#308203,#308204,#308205),(#308206,
#308207,#308208),(#308209,#308210,#308211),(#308212,#308213,#308214),(#308215,
#308216,#308217),(#308218,#308219,#308220),(#308221,#308222,#308223),(#308224,
#308225,#308226),(#308227,#308228,#308229),(#308230,#308231,#308232),(#308233,
#308234,#308235),(#308236,#308237,#308238),(#308239,#308240,#308241),(#308242,
#308243,#308244),(#308245,#308246,#308247),(#308248,#308249,#308250),(#308251,
#308252,#308253),(#308254,#308255,#308256),(#308257,#308258,#308259),(#308260,
#308261,#308262),(#308263,#308264,#308265),(#308266,#308267,#308268),(#308269,
#308270,#308271),(#308272,#308273,#308274),(#308275,#308276,#308277),(#308278,
#308279,#308280),(#308281,#308282,#308283),(#308284,#308285,#308286),(#308287,
#308288,#308289),(#308290,#308291,#308292),(#308293,#308294,#308295),(#308296,
#308297,#308298),(#308299,#308300,#308301),(#308302,#308303,#308304),(#308305,
#308306,#308307),(#308308,#308309,#308310),(#308311,#308312,#308313),(#308314,
#308315,#308316),(#308317,#308318,#308319),(#308320,#308321,#308322),(#308323,
#308324,#308325),(#308326,#308327,#308328),(#308329,#308330,#308331),(#308332,
#308333,#308334),(#308335,#308336,#308337),(#308338,#308339,#308340),(#308341,
#308342,#308343),(#308344,#308345,#308346),(#308347,#308348,#308349),(#308350,
#308351,#308352),(#308353,#308354,#308355),(#308356,#308357,#308358),(#308359,
#308360,#308361),(#308362,#308363,#308364),(#308365,#308366,#308367),(#308368,
#308369,#308370),(#308371,#308372,#308373),(#308374,#308375,#308376),(#308377,
#308378,#308379),(#308380,#308381,#308382),(#308383,#308384,#308385),(#308386,
#308387,#308388),(#308389,#308390,#308391),(#308392,#308393,#308394),(#308395,
#308396,#308397),(#308398,#308399,#308400),(#308401,#308402,#308403),(#308404,
#308405,#308406),(#308407,#308408,#308409),(#308410,#308411,#308412),(#308413,
#308414,#308415),(#308416,#308417,#308418),(#308419,#308420,#308421),(#308422,
#308423,#308424),(#308425,#308426,#308427),(#308428,#308429,#308430),(#308431,
#308432,#308433),(#308434,#308435,#308436),(#308437,#308438,#308439),(#308440,
#308441,#308442),(#308443,#308444,#308445),(#308446,#308447,#308448),(#308449,
#308450,#308451),(#308452,#308453,#308454),(#308455,#308456,#308457),(#308458,
#308459,#308460),(#308461,#308462,#308463),(#308464,#308465,#308466),(#308467,
#308468,#308469),(#308470,#308471,#308472),(#308473,#308474,#308475),(#308476,
#308477,#308478),(#308479,#308480,#308481),(#308482,#308483,#308484),(#308485,
#308486,#308487),(#308488,#308489,#308490),(#308491,#308492,#308493),(#308494,
#308495,#308496),(#308497,#308498,#308499),(#308500,#308501,#308502),(#308503,
#308504,#308505),(#308506,#308507,#308508),(#308509,#308510,#308511),(#308512,
#308513,#308514),(#308515,#308516,#308517),(#308518,#308519,#308520),(#308521,
#308522,#308523),(#308524,#308525,#308526),(#308527,#308528,#308529),(#308530,
#308531,#308532),(#308533,#308534,#308535),(#308536,#308537,#308538),(#308539,
#308540,#308541),(#308542,#308543,#308544),(#308545,#308546,#308547),(#308548,
#308549,#308550),(#308551,#308552,#308553),(#308554,#308555,#308556),(#308557,
#308558,#308559),(#308560,#308561,#308562),(#308563,#308564,#308565),(#308566,
#308567,#308568),(#308569,#308570,#308571),(#308572,#308573,#308574),(#308575,
#308576,#308577),(#308578,#308579,#308580),(#308581,#308582,#308583),(#308584,
#308585,#308586),(#308587,#308588,#308589),(#308590,#308591,#308592),(#308593,
#308594,#308595),(#308596,#308597,#308598),(#308599,#308600,#308601),(#308602,
#308603,#308604),(#308605,#308606,#308607),(#308608,#308609,#308610),(#308611,
#308612,#308613),(#308614,#308615,#308616),(#308617,#308618,#308619),(#308620,
#308621,#308622),(#308623,#308624,#308625),(#308626,#308627,#308628),(#308629,
#308630,#308631),(#308632,#308633,#308634),(#308635,#308636,#308637),(#308638,
#308639,#308640),(#308641,#308642,#308643),(#308644,#308645,#308646),(#308647,
#308648,#308649),(#308650,#308651,#308652),(#308653,#308654,#308655),(#308656,
#308657,#308658),(#308659,#308660,#308661),(#308662,#308663,#308664),(#308665,
#308666,#308667),(#308668,#308669,#308670),(#308671,#308672,#308673),(#308674,
#308675,#308676),(#308677,#308678,#308679),(#308680,#308681,#308682),(#308683,
#308684,#308685),(#308686,#308687,#308688),(#308689,#308690,#308691),(#308692,
#308693,#308694),(#308695,#308696,#308697),(#308698,#308699,#308700),(#308701,
#308702,#308703),(#308704,#308705,#308706),(#308707,#308708,#308709),(#308710,
#308711,#308712),(#308713,#308714,#308715),(#308716,#308717,#308718),(#308719,
#308720,#308721),(#308722,#308723,#308724),(#308725,#308726,#308727),(#308728,
#308729,#308730),(#308731,#308732,#308733),(#308734,#308735,#308736),(#308737,
#308738,#308739),(#308740,#308741,#308742),(#308743,#308744,#308745),(#308746,
#308747,#308748),(#308749,#308750,#308751),(#308752,#308753,#308754),(#308755,
#308756,#308757),(#308758,#308759,#308760),(#308761,#308762,#308763),(#308764,
#308765,#308766),(#308767,#308768,#308769),(#308770,#308771,#308772),(#308773,
#308774,#308775),(#308776,#308777,#308778),(#308779,#308780,#308781),(#308782,
#308783,#308784),(#308785,#308786,#308787),(#308788,#308789,#308790),(#308791,
#308792,#308793),(#308794,#308795,#308796),(#308797,#308798,#308799),(#308800,
#308801,#308802),(#308803,#308804,#308805),(#308806,#308807,#308808),(#308809,
#308810,#308811),(#308812,#308813,#308814),(#308815,#308816,#308817),(#308818,
#308819,#308820),(#308821,#308822,#308823),(#308824,#308825,#308826),(#308827,
#308828,#308829),(#308830,#308831,#308832),(#308833,#308834,#308835),(#308836,
#308837,#308838),(#308839,#308840,#308841),(#308842,#308843,#308844),(#308845,
#308846,#308847),(#308848,#308849,#308850),(#308851,#308852,#308853),(#308854,
#308855,#308856),(#308857,#308858,#308859),(#308860,#308861,#308862),(#308863,
#308864,#308865),(#308866,#308867,#308868),(#308869,#308870,#308871),(#308872,
#308873,#308874),(#308875,#308876,#308877),(#308878,#308879,#308880),(#308881,
#308882,#308883),(#308884,#308885,#308886),(#308887,#308888,#308889),(#308890,
#308891,#308892),(#308893,#308894,#308895),(#308896,#308897,#308898),(#308899,
#308900,#308901),(#308902,#308903,#308904),(#308905,#308906,#308907),(#308908,
#308909,#308910),(#308911,#308912,#308913),(#308914,#308915,#308916),(#308917,
#308918,#308919),(#308920,#308921,#308922),(#308923,#308924,#308925),(#308926,
#308927,#308928),(#308929,#308930,#308931),(#308932,#308933,#308934),(#308935,
#308936,#308937),(#308938,#308939,#308940),(#308941,#308942,#308943),(#308944,
#308945,#308946),(#308947,#308948,#308949),(#308950,#308951,#308952),(#308953,
#308954,#308955),(#308956,#308957,#308958),(#308959,#308960,#308961),(#308962,
#308963,#308964),(#308965,#308966,#308967),(#308968,#308969,#308970),(#308971,
#308972,#308973),(#308974,#308975,#308976),(#308977,#308978,#308979),(#308980,
#308981,#308982),(#308983,#308984,#308985),(#308986,#308987,#308988),(#308989,
#308990,#308991),(#308992,#308993,#308994),(#308995,#308996,#308997),(#308998,
#308999,#309000),(#309001,#309002,#309003),(#309004,#309005,#309006),(#309007,
#309008,#309009),(#309010,#309011,#309012),(#309013,#309014,#309015),(#309016,
#309017,#309018),(#309019,#309020,#309021),(#309022,#309023,#309024),(#309025,
#309026,#309027),(#309028,#309029,#309030),(#309031,#309032,#309033),(#309034,
#309035,#309036),(#309037,#309038,#309039),(#309040,#309041,#309042),(#309043,
#309044,#309045),(#309046,#309047,#309048),(#309049,#309050,#309051),(#309052,
#309053,#309054),(#309055,#309056,#309057),(#309058,#309059,#309060),(#309061,
#309062,#309063),(#309064,#309065,#309066),(#309067,#309068,#309069),(#309070,
#309071,#309072),(#309073,#309074,#309075),(#309076,#309077,#309078),(#309079,
#309080,#309081),(#309082,#309083,#309084),(#309085,#309086,#309087),(#309088,
#309089,#309090),(#309091,#309092,#309093),(#309094,#309095,#309096),(#309097,
#309098,#309099),(#309100,#309101,#309102),(#309103,#309104,#309105),(#309106,
#309107,#309108),(#309109,#309110,#309111),(#309112,#309113,#309114),(#309115,
#309116,#309117),(#309118,#309119,#309120),(#309121,#309122,#309123),(#309124,
#309125,#309126),(#309127,#309128,#309129),(#309130,#309131,#309132),(#309133,
#309134,#309135),(#309136,#309137,#309138),(#309139,#309140,#309141),(#309142,
#309143,#309144),(#309145,#309146,#309147),(#309148,#309149,#309150),(#309151,
#309152,#309153),(#309154,#309155,#309156),(#309157,#309158,#309159),(#309160,
#309161,#309162),(#309163,#309164,#309165),(#309166,#309167,#309168),(#309169,
#309170,#309171),(#309172,#309173,#309174),(#309175,#309176,#309177),(#309178,
#309179,#309180),(#309181,#309182,#309183),(#309184,#309185,#309186),(#309187,
#309188,#309189),(#309190,#309191,#309192),(#309193,#309194,#309195),(#309196,
#309197,#309198),(#309199,#309200,#309201),(#309202,#309203,#309204),(#309205,
#309206,#309207),(#309208,#309209,#309210),(#309211,#309212,#309213),(#309214,
#309215,#309216),(#309217,#309218,#309219),(#309220,#309221,#309222),(#309223,
#309224,#309225),(#309226,#309227,#309228),(#309229,#309230,#309231),(#309232,
#309233,#309234),(#309235,#309236,#309237),(#309238,#309239,#309240),(#309241,
#309242,#309243),(#309244,#309245,#309246),(#309247,#309248,#309249),(#309250,
#309251,#309252),(#309253,#309254,#309255),(#309256,#309257,#309258),(#309259,
#309260,#309261),(#309262,#309263,#309264),(#309265,#309266,#309267),(#309268,
#309269,#309270),(#309271,#309272,#309273),(#309274,#309275,#309276),(#309277,
#309278,#309279),(#309280,#309281,#309282),(#309283,#309284,#309285),(#309286,
#309287,#309288),(#309289,#309290,#309291),(#309292,#309293,#309294),(#309295,
#309296,#309297),(#309298,#309299,#309300),(#309301,#309302,#309303),(#309304,
#309305,#309306),(#309307,#309308,#309309),(#309310,#309311,#309312),(#309313,
#309314,#309315),(#309316,#309317,#309318),(#309319,#309320,#309321),(#309322,
#309323,#309324),(#309325,#309326,#309327),(#309328,#309329,#309330),(#309331,
#309332,#309333),(#309334,#309335,#309336),(#309337,#309338,#309339),(#309340,
#309341,#309342),(#309343,#309344,#309345),(#309346,#309347,#309348),(#309349,
#309350,#309351),(#309352,#309353,#309354),(#309355,#309356,#309357),(#309358,
#309359,#309360),(#309361,#309362,#309363),(#309364,#309365,#309366),(#309367,
#309368,#309369),(#309370,#309371,#309372),(#309373,#309374,#309375),(#309376,
#309377,#309378),(#309379,#309380,#309381),(#309382,#309383,#309384),(#309385,
#309386,#309387),(#309388,#309389,#309390),(#309391,#309392,#309393),(#309394,
#309395,#309396),(#309397,#309398,#309399),(#309400,#309401,#309402),(#309403,
#309404,#309405),(#309406,#309407,#309408),(#309409,#309410,#309411),(#309412,
#309413,#309414),(#309415,#309416,#309417),(#309418,#309419,#309420),(#309421,
#309422,#309423),(#309424,#309425,#309426),(#309427,#309428,#309429),(#309430,
#309431,#309432),(#309433,#309434,#309435),(#309436,#309437,#309438),(#309439,
#309440,#309441),(#309442,#309443,#309444),(#309445,#309446,#309447),(#309448,
#309449,#309450),(#309451,#309452,#309453),(#309454,#309455,#309456),(#309457,
#309458,#309459),(#309460,#309461,#309462),(#309463,#309464,#309465),(#309466,
#309467,#309468),(#309469,#309470,#309471),(#309472,#309473,#309474),(#309475,
#309476,#309477),(#309478,#309479,#309480),(#309481,#309482,#309483),(#309484,
#309485,#309486),(#309487,#309488,#309489),(#309490,#309491,#309492),(#309493,
#309494,#309495),(#309496,#309497,#309498),(#309499,#309500,#309501),(#309502,
#309503,#309504),(#309505,#309506,#309507),(#309508,#309509,#309510),(#309511,
#309512,#309513),(#309514,#309515,#309516),(#309517,#309518,#309519),(#309520,
#309521,#309522),(#309523,#309524,#309525),(#309526,#309527,#309528),(#309529,
#309530,#309531),(#309532,#309533,#309534),(#309535,#309536,#309537),(#309538,
#309539,#309540),(#309541,#309542,#309543),(#309544,#309545,#309546),(#309547,
#309548,#309549),(#309550,#309551,#309552),(#309553,#309554,#309555),(#309556,
#309557,#309558),(#309559,#309560,#309561),(#309562,#309563,#309564),(#309565,
#309566,#309567),(#309568,#309569,#309570),(#309571,#309572,#309573),(#309574,
#309575,#309576),(#309577,#309578,#309579),(#309580,#309581,#309582),(#309583,
#309584,#309585),(#309586,#309587,#309588),(#309589,#309590,#309591),(#309592,
#309593,#309594),(#309595,#309596,#309597),(#309598,#309599,#309600),(#309601,
#309602,#309603),(#309604,#309605,#309606),(#309607,#309608,#309609),(#309610,
#309611,#309612),(#309613,#309614,#309615),(#309616,#309617,#309618),(#309619,
#309620,#309621),(#309622,#309623,#309624),(#309625,#309626,#309627)),
 .UNSPECIFIED.,.F.,.F.,.F.,(6,1,1,1,1,1,1,1,1,1,1,1,1,1,1,1,1,1,1,1,1,1,
1,1,1,1,1,1,1,1,1,1,1,1,1,1,1,1,1,1,1,1,1,1,1,1,1,1,1,1,1,1,1,1,1,1,1,1,
1,1,1,1,1,1,1,1,1,1,1,1,1,1,1,1,1,1,1,1,1,1,1,1,1,1,1,1,1,1,1,1,1,1,1,1,
1,1,1,1,1,1,1,1,1,1,1,1,1,1,1,1,1,1,1,1,1,1,1,1,1,1,1,1,1,1,1,1,1,1,1,1,
1,1,1,1,1,1,1,1,1,1,1,1,1,1,1,1,1,1,1,1,1,1,1,1,1,1,1,1,1,1,1,1,1,1,1,1,
1,1,1,1,1,1,1,1,1,1,1,1,1,1,1,1,1,1,1,1,1,1,1,1,1,1,1,1,1,1,1,1,1,1,1,1,
1,1,1,1,1,1,1,1,1,1,1,1,1,1,1,1,1,1,1,1,1,1,1,1,1,1,1,1,1,1,1,1,1,1,1,1,
1,1,1,1,1,1,1,1,1,1,1,1,1,1,1,1,1,1,1,1,1,1,1,1,1,1,1,1,1,1,1,1,1,1,1,1,
1,1,1,1,1,1,1,1,1,1,1,1,1,1,1,1,1,1,1,1,1,1,1,1,1,1,1,1,1,1,1,1,1,1,1,1,
1,1,1,1,1,1,1,1,1,1,1,1,1,1,1,1,1,1,1,1,1,1,1,1,1,1,1,1,1,1,1,1,1,1,1,1,
1,1,1,1,1,1,1,1,1,1,1,1,1,1,1,1,1,1,1,1,1,1,1,1,1,1,1,1,1,1,1,1,1,1,1,1,
1,1,1,1,1,1,1,1,1,1,1,1,1,1,1,1,1,1,1,1,1,1,1,1,1,1,1,1,1,1,1,1,1,1,1,1,
1,1,1,1,1,1,1,1,1,1,1,1,1,1,1,1,1,1,1,1,1,1,1,1,1,1,1,1,1,1,1,1,1,1,1,1,
1,1,1,1,1,1,1,1,1,1,1,1,1,1,1,1,1,1,1,1,1,1,1,1,1,1,1,1,1,1,1,1,1,1,1,1,
1,1,1,1,1,1,1,1,1,1,1,1,1,1,1,1,1,1,1,1,1,1,1,1,1,1,1,1,1,1,1,1,1,1,1,1,
1,1,1,1,1,1,1,1,1,1,1,1,1,1,1,1,1,1,1,6),(2,1,2),(-1.,-0.998165138,-0.996330275,
-0.994495413,-0.99266055,-0.990825688,-0.988990826,-0.987155963,-0.985321101,
-0.983486239,-0.981651376,-0.979816514,-0.977981651,-0.976146789,-0.974311927,
-0.972477064,-0.970642202,-0.968807339,-0.966972477,-0.965137615,-0.963302752,
-0.96146789,-0.959633028,-0.957798165,-0.955963303,-0.95412844,-0.952293578,
-0.950458716,-0.948623853,-0.946788991,-0.944954128,-0.943119266,-0.941284404,
-0.939449541,-0.937614679,-0.935779817,-0.933944954,-0.932110092,-0.930275229,
-0.928440367,-0.926605505,-0.924770642,-0.92293578,-0.921100917,-0.919266055,
-0.917431193,-0.91559633,-0.913761468,-0.911926606,-0.910091743,-0.908256881,
-0.906422018,-0.904587156,-0.902752294,-0.900917431,-0.899082569,-0.897247706,
-0.895412844,-0.893577982,-0.891743119,-0.889908257,-0.888073394,-0.886238532,
-0.88440367,-0.882568807,-0.880733945,-0.878899083,-0.87706422,-0.875229358,
-0.873394495,-0.871559633,-0.869724771,-0.867889908,-0.866055046,-0.864220183,
-0.862385321,-0.860550459,-0.858715596,-0.856880734,-0.855045872,-0.853211009,
-0.851376147,-0.849541284,-0.847706422,-0.84587156,-0.844036697,-0.842201835,
-0.840366972,-0.83853211,-0.836697248,-0.834862385,-0.833027523,-0.831192661,
-0.829357798,-0.827522936,-0.825688073,-0.823853211,-0.822018349,-0.820183486,
-0.818348624,-0.816513761,-0.814678899,-0.812844037,-0.811009174,-0.809174312,
-0.80733945,-0.805504587,-0.803669725,-0.801834862,-0.8,-0.798165138,-0.796330275,
-0.794495413,-0.79266055,-0.790825688,-0.788990826,-0.787155963,-0.785321101,
-0.783486239,-0.781651376,-0.779816514,-0.777981651,-0.776146789,-0.774311927,
-0.772477064,-0.770642202,-0.768807339,-0.766972477,-0.765137615,-0.763302752,
-0.76146789,-0.759633028,-0.757798165,-0.755963303,-0.75412844,-0.752293578,
-0.750458716,-0.748623853,-0.746788991,-0.744954128,-0.743119266,-0.741284404,
-0.739449541,-0.737614679,-0.735779817,-0.733944954,-0.732110092,-0.730275229,
-0.728440367,-0.726605505,-0.724770642,-0.72293578,-0.721100917,-0.719266055,
-0.717431193,-0.71559633,-0.713761468,-0.711926606,-0.710091743,-0.708256881,
-0.706422018,-0.704587156,-0.702752294,-0.700917431,-0.699082569,-0.697247706,
-0.695412844,-0.693577982,-0.691743119,-0.689908257,-0.688073394,-0.686238532,
-0.68440367,-0.682568807,-0.680733945,-0.678899083,-0.67706422,-0.675229358,
-0.673394495,-0.671559633,-0.669724771,-0.667889908,-0.666055046,-0.664220183,
-0.662385321,-0.660550459,-0.658715596,-0.656880734,-0.655045872,-0.653211009,
-0.651376147,-0.649541284,-0.647706422,-0.64587156,-0.644036697,-0.642201835,
-0.640366972,-0.63853211,-0.636697248,-0.634862385,-0.633027523,-0.631192661,
-0.629357798,-0.627522936,-0.625688073,-0.623853211,-0.622018349,-0.620183486,
-0.618348624,-0.616513761,-0.614678899,-0.612844037,-0.611009174,-0.609174312,
-0.60733945,-0.605504587,-0.603669725,-0.601834862,-0.6,-0.598165138,-0.596330275,
-0.594495413,-0.59266055,-0.590825688,-0.588990826,-0.587155963,-0.585321101,
-0.583486239,-0.581651376,-0.579816514,-0.577981651,-0.576146789,-0.574311927,
-0.572477064,-0.570642202,-0.568807339,-0.566972477,-0.565137615,-0.563302752,
-0.56146789,-0.559633028,-0.557798165,-0.555963303,-0.55412844,-0.552293578,
-0.550458716,-0.548623853,-0.546788991,-0.544954128,-0.543119266,-0.541284404,
-0.539449541,-0.537614679,-0.535779817,-0.533944954,-0.532110092,-0.530275229,
-0.528440367,-0.526605505,-0.524770642,-0.52293578,-0.521100917,-0.519266055,
-0.517431193,-0.51559633,-0.513761468,-0.511926606,-0.510091743,-0.508256881,
-0.506422018,-0.504587156,-0.502752294,-0.500917431,-0.499082569,-0.497247706,
-0.495412844,-0.493577982,-0.491743119,-0.489908257,-0.488073394,-0.486238532,
-0.48440367,-0.482568807,-0.480733945,-0.478899083,-0.47706422,-0.475229358,
-0.473394495,-0.471559633,-0.469724771,-0.467889908,-0.466055046,-0.464220183,
-0.462385321,-0.460550459,-0.458715596,-0.456880734,-0.455045872,-0.453211009,
-0.451376147,-0.449541284,-0.447706422,-0.44587156,-0.444036697,-0.442201835,
-0.440366972,-0.43853211,-0.436697248,-0.434862385,-0.433027523,-0.431192661,
-0.429357798,-0.427522936,-0.425688073,-0.423853211,-0.422018349,-0.420183486,
-0.418348624,-0.416513761,-0.414678899,-0.412844037,-0.411009174,-0.409174312,
-0.40733945,-0.405504587,-0.403669725,-0.401834862,-0.4,-0.398165138,-0.396330275,
-0.394495413,-0.39266055,-0.390825688,-0.388990826,-0.387155963,-0.385321101,
-0.383486239,-0.381651376,-0.379816514,-0.377981651,-0.376146789,-0.374311927,
-0.372477064,-0.370642202,-0.368807339,-0.366972477,-0.365137615,-0.363302752,
-0.36146789,-0.359633028,-0.357798165,-0.355963303,-0.35412844,-0.352293578,
-0.350458716,-0.348623853,-0.346788991,-0.344954128,-0.343119266,-0.341284404,
-0.339449541,-0.337614679,-0.335779817,-0.333944954,-0.332110092,-0.330275229,
-0.328440367,-0.326605505,-0.324770642,-0.32293578,-0.321100917,-0.319266055,
-0.317431193,-0.31559633,-0.313761468,-0.311926606,-0.310091743,-0.308256881,
-0.306422018,-0.304587156,-0.302752294,-0.300917431,-0.299082569,-0.297247706,
-0.295412844,-0.293577982,-0.291743119,-0.289908257,-0.288073394,-0.286238532,
-0.28440367,-0.282568807,-0.280733945,-0.278899083,-0.27706422,-0.275229358,
-0.273394495,-0.271559633,-0.269724771,-0.267889908,-0.266055046,-0.264220183,
-0.262385321,-0.260550459,-0.258715596,-0.256880734,-0.255045872,-0.253211009,
-0.251376147,-0.249541284,-0.247706422,-0.24587156,-0.244036697,-0.242201835,
-0.240366972,-0.23853211,-0.236697248,-0.234862385,-0.233027523,-0.231192661,
-0.229357798,-0.227522936,-0.225688073,-0.223853211,-0.222018349,-0.220183486,
-0.218348624,-0.216513761,-0.214678899,-0.212844037,-0.211009174,-0.209174312,
-0.20733945,-0.205504587,-0.203669725,-0.201834862,-0.2,-0.198165138,-0.196330275,
-0.194495413,-0.19266055,-0.190825688,-0.188990826,-0.187155963,-0.185321101,
-0.183486239,-0.181651376,-0.179816514,-0.177981651,-0.176146789,-0.174311927,
-0.172477064,-0.170642202,-0.168807339,-0.166972477,-0.165137615,-0.163302752,
-0.16146789,-0.159633028,-0.157798165,-0.155963303,-0.15412844,-0.152293578,
-0.150458716,-0.148623853,-0.146788991,-0.144954128,-0.143119266,-0.141284404,
-0.139449541,-0.137614679,-0.135779817,-0.133944954,-0.132110092,-0.130275229,
-0.128440367,-0.126605505,-0.124770642,-0.12293578,-0.121100917,-0.119266055,
-0.117431193,-0.11559633,-0.113761468,-0.111926606,-0.110091743,-0.108256881,
-0.106422018,-0.104587156,-0.102752294,-0.100917431,-0.099082569,-0.097247706,
-0.095412844,-0.093577982,-0.091743119,-0.089908257,-0.088073394,-0.086238532,
-0.08440367,-0.082568807,-0.080733945,-0.078899083,-0.07706422,-0.075229358,
-0.073394495,-0.071559633,-0.069724771,-0.067889908,-0.066055046,-0.064220183,
-0.062385321,-0.060550459,-0.058715596,-0.056880734,-0.055045872,-0.053211009,
-0.051376147,-0.049541284,-0.047706422,-0.04587156,-0.044036697,-0.042201835,
-0.040366972,-0.03853211,-0.036697248,-0.034862385,-0.033027523,-0.031192661,
-0.029357798,-0.027522936,-0.025688073,-0.023853211,-0.022018349,-0.020183486,
-0.018348624,-0.016513761,-0.014678899,-0.012844037,-0.011009174,-0.009174312,
-0.00733945,-0.005504587,-0.003669725,-0.001834862,0.000982108),(0.3,1.,
1.3),.UNSPECIFIED.);
#6308=B_SPLINE_SURFACE_WITH_KNOTS('',5,1,((#309650,#309651,#309652),(#309653,
#309654,#309655),(#309656,#309657,#309658),(#309659,#309660,#309661),(#309662,
#309663,#309664),(#309665,#309666,#309667),(#309668,#309669,#309670),(#309671,
#309672,#309673),(#309674,#309675,#309676),(#309677,#309678,#309679),(#309680,
#309681,#309682),(#309683,#309684,#309685),(#309686,#309687,#309688),(#309689,
#309690,#309691),(#309692,#309693,#309694),(#309695,#309696,#309697),(#309698,
#309699,#309700),(#309701,#309702,#309703),(#309704,#309705,#309706),(#309707,
#309708,#309709),(#309710,#309711,#309712),(#309713,#309714,#309715),(#309716,
#309717,#309718),(#309719,#309720,#309721),(#309722,#309723,#309724),(#309725,
#309726,#309727),(#309728,#309729,#309730),(#309731,#309732,#309733),(#309734,
#309735,#309736),(#309737,#309738,#309739),(#309740,#309741,#309742),(#309743,
#309744,#309745),(#309746,#309747,#309748),(#309749,#309750,#309751),(#309752,
#309753,#309754),(#309755,#309756,#309757),(#309758,#309759,#309760),(#309761,
#309762,#309763),(#309764,#309765,#309766),(#309767,#309768,#309769),(#309770,
#309771,#309772),(#309773,#309774,#309775),(#309776,#309777,#309778),(#309779,
#309780,#309781),(#309782,#309783,#309784),(#309785,#309786,#309787),(#309788,
#309789,#309790),(#309791,#309792,#309793),(#309794,#309795,#309796),(#309797,
#309798,#309799),(#309800,#309801,#309802),(#309803,#309804,#309805),(#309806,
#309807,#309808),(#309809,#309810,#309811),(#309812,#309813,#309814),(#309815,
#309816,#309817),(#309818,#309819,#309820),(#309821,#309822,#309823),(#309824,
#309825,#309826),(#309827,#309828,#309829),(#309830,#309831,#309832),(#309833,
#309834,#309835),(#309836,#309837,#309838),(#309839,#309840,#309841),(#309842,
#309843,#309844),(#309845,#309846,#309847),(#309848,#309849,#309850),(#309851,
#309852,#309853),(#309854,#309855,#309856),(#309857,#309858,#309859),(#309860,
#309861,#309862),(#309863,#309864,#309865),(#309866,#309867,#309868),(#309869,
#309870,#309871),(#309872,#309873,#309874),(#309875,#309876,#309877),(#309878,
#309879,#309880),(#309881,#309882,#309883),(#309884,#309885,#309886),(#309887,
#309888,#309889),(#309890,#309891,#309892),(#309893,#309894,#309895),(#309896,
#309897,#309898),(#309899,#309900,#309901),(#309902,#309903,#309904),(#309905,
#309906,#309907),(#309908,#309909,#309910),(#309911,#309912,#309913),(#309914,
#309915,#309916),(#309917,#309918,#309919),(#309920,#309921,#309922),(#309923,
#309924,#309925),(#309926,#309927,#309928),(#309929,#309930,#309931),(#309932,
#309933,#309934),(#309935,#309936,#309937),(#309938,#309939,#309940),(#309941,
#309942,#309943),(#309944,#309945,#309946),(#309947,#309948,#309949),(#309950,
#309951,#309952),(#309953,#309954,#309955),(#309956,#309957,#309958),(#309959,
#309960,#309961),(#309962,#309963,#309964),(#309965,#309966,#309967),(#309968,
#309969,#309970),(#309971,#309972,#309973),(#309974,#309975,#309976),(#309977,
#309978,#309979),(#309980,#309981,#309982),(#309983,#309984,#309985),(#309986,
#309987,#309988),(#309989,#309990,#309991),(#309992,#309993,#309994),(#309995,
#309996,#309997),(#309998,#309999,#310000),(#310001,#310002,#310003),(#310004,
#310005,#310006),(#310007,#310008,#310009),(#310010,#310011,#310012),(#310013,
#310014,#310015),(#310016,#310017,#310018),(#310019,#310020,#310021),(#310022,
#310023,#310024),(#310025,#310026,#310027),(#310028,#310029,#310030),(#310031,
#310032,#310033),(#310034,#310035,#310036),(#310037,#310038,#310039),(#310040,
#310041,#310042),(#310043,#310044,#310045),(#310046,#310047,#310048),(#310049,
#310050,#310051),(#310052,#310053,#310054),(#310055,#310056,#310057),(#310058,
#310059,#310060),(#310061,#310062,#310063),(#310064,#310065,#310066),(#310067,
#310068,#310069),(#310070,#310071,#310072),(#310073,#310074,#310075),(#310076,
#310077,#310078),(#310079,#310080,#310081),(#310082,#310083,#310084),(#310085,
#310086,#310087),(#310088,#310089,#310090),(#310091,#310092,#310093),(#310094,
#310095,#310096),(#310097,#310098,#310099),(#310100,#310101,#310102),(#310103,
#310104,#310105),(#310106,#310107,#310108),(#310109,#310110,#310111),(#310112,
#310113,#310114),(#310115,#310116,#310117),(#310118,#310119,#310120),(#310121,
#310122,#310123),(#310124,#310125,#310126),(#310127,#310128,#310129),(#310130,
#310131,#310132),(#310133,#310134,#310135),(#310136,#310137,#310138),(#310139,
#310140,#310141),(#310142,#310143,#310144),(#310145,#310146,#310147),(#310148,
#310149,#310150),(#310151,#310152,#310153),(#310154,#310155,#310156),(#310157,
#310158,#310159),(#310160,#310161,#310162),(#310163,#310164,#310165),(#310166,
#310167,#310168),(#310169,#310170,#310171),(#310172,#310173,#310174),(#310175,
#310176,#310177),(#310178,#310179,#310180),(#310181,#310182,#310183),(#310184,
#310185,#310186),(#310187,#310188,#310189),(#310190,#310191,#310192),(#310193,
#310194,#310195),(#310196,#310197,#310198),(#310199,#310200,#310201),(#310202,
#310203,#310204),(#310205,#310206,#310207),(#310208,#310209,#310210),(#310211,
#310212,#310213),(#310214,#310215,#310216),(#310217,#310218,#310219),(#310220,
#310221,#310222),(#310223,#310224,#310225),(#310226,#310227,#310228),(#310229,
#310230,#310231),(#310232,#310233,#310234),(#310235,#310236,#310237),(#310238,
#310239,#310240),(#310241,#310242,#310243),(#310244,#310245,#310246),(#310247,
#310248,#310249),(#310250,#310251,#310252),(#310253,#310254,#310255),(#310256,
#310257,#310258),(#310259,#310260,#310261),(#310262,#310263,#310264),(#310265,
#310266,#310267),(#310268,#310269,#310270),(#310271,#310272,#310273),(#310274,
#310275,#310276),(#310277,#310278,#310279),(#310280,#310281,#310282),(#310283,
#310284,#310285),(#310286,#310287,#310288),(#310289,#310290,#310291),(#310292,
#310293,#310294),(#310295,#310296,#310297),(#310298,#310299,#310300),(#310301,
#310302,#310303),(#310304,#310305,#310306),(#310307,#310308,#310309),(#310310,
#310311,#310312),(#310313,#310314,#310315),(#310316,#310317,#310318),(#310319,
#310320,#310321),(#310322,#310323,#310324),(#310325,#310326,#310327),(#310328,
#310329,#310330),(#310331,#310332,#310333),(#310334,#310335,#310336),(#310337,
#310338,#310339),(#310340,#310341,#310342),(#310343,#310344,#310345),(#310346,
#310347,#310348),(#310349,#310350,#310351),(#310352,#310353,#310354),(#310355,
#310356,#310357),(#310358,#310359,#310360),(#310361,#310362,#310363),(#310364,
#310365,#310366),(#310367,#310368,#310369),(#310370,#310371,#310372),(#310373,
#310374,#310375),(#310376,#310377,#310378),(#310379,#310380,#310381),(#310382,
#310383,#310384),(#310385,#310386,#310387),(#310388,#310389,#310390),(#310391,
#310392,#310393),(#310394,#310395,#310396),(#310397,#310398,#310399),(#310400,
#310401,#310402),(#310403,#310404,#310405),(#310406,#310407,#310408),(#310409,
#310410,#310411),(#310412,#310413,#310414),(#310415,#310416,#310417),(#310418,
#310419,#310420),(#310421,#310422,#310423),(#310424,#310425,#310426),(#310427,
#310428,#310429),(#310430,#310431,#310432),(#310433,#310434,#310435),(#310436,
#310437,#310438),(#310439,#310440,#310441),(#310442,#310443,#310444),(#310445,
#310446,#310447),(#310448,#310449,#310450),(#310451,#310452,#310453),(#310454,
#310455,#310456),(#310457,#310458,#310459),(#310460,#310461,#310462),(#310463,
#310464,#310465),(#310466,#310467,#310468),(#310469,#310470,#310471),(#310472,
#310473,#310474),(#310475,#310476,#310477),(#310478,#310479,#310480),(#310481,
#310482,#310483),(#310484,#310485,#310486),(#310487,#310488,#310489),(#310490,
#310491,#310492),(#310493,#310494,#310495),(#310496,#310497,#310498),(#310499,
#310500,#310501),(#310502,#310503,#310504),(#310505,#310506,#310507),(#310508,
#310509,#310510),(#310511,#310512,#310513),(#310514,#310515,#310516),(#310517,
#310518,#310519),(#310520,#310521,#310522),(#310523,#310524,#310525),(#310526,
#310527,#310528),(#310529,#310530,#310531),(#310532,#310533,#310534),(#310535,
#310536,#310537),(#310538,#310539,#310540),(#310541,#310542,#310543),(#310544,
#310545,#310546),(#310547,#310548,#310549),(#310550,#310551,#310552),(#310553,
#310554,#310555),(#310556,#310557,#310558),(#310559,#310560,#310561),(#310562,
#310563,#310564),(#310565,#310566,#310567),(#310568,#310569,#310570),(#310571,
#310572,#310573),(#310574,#310575,#310576),(#310577,#310578,#310579),(#310580,
#310581,#310582),(#310583,#310584,#310585),(#310586,#310587,#310588),(#310589,
#310590,#310591),(#310592,#310593,#310594),(#310595,#310596,#310597),(#310598,
#310599,#310600),(#310601,#310602,#310603),(#310604,#310605,#310606),(#310607,
#310608,#310609),(#310610,#310611,#310612),(#310613,#310614,#310615),(#310616,
#310617,#310618),(#310619,#310620,#310621),(#310622,#310623,#310624),(#310625,
#310626,#310627),(#310628,#310629,#310630),(#310631,#310632,#310633),(#310634,
#310635,#310636),(#310637,#310638,#310639),(#310640,#310641,#310642),(#310643,
#310644,#310645),(#310646,#310647,#310648),(#310649,#310650,#310651),(#310652,
#310653,#310654),(#310655,#310656,#310657),(#310658,#310659,#310660),(#310661,
#310662,#310663),(#310664,#310665,#310666),(#310667,#310668,#310669),(#310670,
#310671,#310672),(#310673,#310674,#310675),(#310676,#310677,#310678),(#310679,
#310680,#310681),(#310682,#310683,#310684),(#310685,#310686,#310687),(#310688,
#310689,#310690),(#310691,#310692,#310693),(#310694,#310695,#310696),(#310697,
#310698,#310699),(#310700,#310701,#310702),(#310703,#310704,#310705),(#310706,
#310707,#310708),(#310709,#310710,#310711),(#310712,#310713,#310714),(#310715,
#310716,#310717),(#310718,#310719,#310720),(#310721,#310722,#310723),(#310724,
#310725,#310726),(#310727,#310728,#310729),(#310730,#310731,#310732),(#310733,
#310734,#310735),(#310736,#310737,#310738),(#310739,#310740,#310741),(#310742,
#310743,#310744),(#310745,#310746,#310747),(#310748,#310749,#310750),(#310751,
#310752,#310753),(#310754,#310755,#310756),(#310757,#310758,#310759),(#310760,
#310761,#310762),(#310763,#310764,#310765),(#310766,#310767,#310768),(#310769,
#310770,#310771),(#310772,#310773,#310774),(#310775,#310776,#310777),(#310778,
#310779,#310780),(#310781,#310782,#310783),(#310784,#310785,#310786),(#310787,
#310788,#310789),(#310790,#310791,#310792),(#310793,#310794,#310795),(#310796,
#310797,#310798),(#310799,#310800,#310801),(#310802,#310803,#310804),(#310805,
#310806,#310807),(#310808,#310809,#310810),(#310811,#310812,#310813),(#310814,
#310815,#310816),(#310817,#310818,#310819),(#310820,#310821,#310822),(#310823,
#310824,#310825),(#310826,#310827,#310828),(#310829,#310830,#310831),(#310832,
#310833,#310834),(#310835,#310836,#310837),(#310838,#310839,#310840),(#310841,
#310842,#310843),(#310844,#310845,#310846),(#310847,#310848,#310849),(#310850,
#310851,#310852),(#310853,#310854,#310855),(#310856,#310857,#310858),(#310859,
#310860,#310861),(#310862,#310863,#310864),(#310865,#310866,#310867),(#310868,
#310869,#310870),(#310871,#310872,#310873),(#310874,#310875,#310876),(#310877,
#310878,#310879),(#310880,#310881,#310882),(#310883,#310884,#310885),(#310886,
#310887,#310888),(#310889,#310890,#310891),(#310892,#310893,#310894),(#310895,
#310896,#310897),(#310898,#310899,#310900),(#310901,#310902,#310903),(#310904,
#310905,#310906),(#310907,#310908,#310909),(#310910,#310911,#310912),(#310913,
#310914,#310915),(#310916,#310917,#310918),(#310919,#310920,#310921),(#310922,
#310923,#310924),(#310925,#310926,#310927),(#310928,#310929,#310930),(#310931,
#310932,#310933),(#310934,#310935,#310936),(#310937,#310938,#310939),(#310940,
#310941,#310942),(#310943,#310944,#310945),(#310946,#310947,#310948),(#310949,
#310950,#310951),(#310952,#310953,#310954),(#310955,#310956,#310957),(#310958,
#310959,#310960),(#310961,#310962,#310963),(#310964,#310965,#310966),(#310967,
#310968,#310969),(#310970,#310971,#310972),(#310973,#310974,#310975),(#310976,
#310977,#310978),(#310979,#310980,#310981),(#310982,#310983,#310984),(#310985,
#310986,#310987),(#310988,#310989,#310990),(#310991,#310992,#310993),(#310994,
#310995,#310996),(#310997,#310998,#310999),(#311000,#311001,#311002),(#311003,
#311004,#311005),(#311006,#311007,#311008),(#311009,#311010,#311011),(#311012,
#311013,#311014),(#311015,#311016,#311017),(#311018,#311019,#311020),(#311021,
#311022,#311023),(#311024,#311025,#311026),(#311027,#311028,#311029),(#311030,
#311031,#311032),(#311033,#311034,#311035),(#311036,#311037,#311038),(#311039,
#311040,#311041),(#311042,#311043,#311044),(#311045,#311046,#311047),(#311048,
#311049,#311050),(#311051,#311052,#311053),(#311054,#311055,#311056),(#311057,
#311058,#311059),(#311060,#311061,#311062),(#311063,#311064,#311065),(#311066,
#311067,#311068),(#311069,#311070,#311071),(#311072,#311073,#311074),(#311075,
#311076,#311077),(#311078,#311079,#311080),(#311081,#311082,#311083),(#311084,
#311085,#311086),(#311087,#311088,#311089),(#311090,#311091,#311092),(#311093,
#311094,#311095),(#311096,#311097,#311098),(#311099,#311100,#311101),(#311102,
#311103,#311104),(#311105,#311106,#311107),(#311108,#311109,#311110),(#311111,
#311112,#311113),(#311114,#311115,#311116),(#311117,#311118,#311119),(#311120,
#311121,#311122),(#311123,#311124,#311125),(#311126,#311127,#311128),(#311129,
#311130,#311131),(#311132,#311133,#311134),(#311135,#311136,#311137),(#311138,
#311139,#311140),(#311141,#311142,#311143),(#311144,#311145,#311146),(#311147,
#311148,#311149),(#311150,#311151,#311152),(#311153,#311154,#311155),(#311156,
#311157,#311158),(#311159,#311160,#311161),(#311162,#311163,#311164),(#311165,
#311166,#311167),(#311168,#311169,#311170),(#311171,#311172,#311173),(#311174,
#311175,#311176),(#311177,#311178,#311179),(#311180,#311181,#311182),(#311183,
#311184,#311185),(#311186,#311187,#311188),(#311189,#311190,#311191),(#311192,
#311193,#311194),(#311195,#311196,#311197),(#311198,#311199,#311200),(#311201,
#311202,#311203),(#311204,#311205,#311206),(#311207,#311208,#311209),(#311210,
#311211,#311212),(#311213,#311214,#311215),(#311216,#311217,#311218),(#311219,
#311220,#311221),(#311222,#311223,#311224),(#311225,#311226,#311227),(#311228,
#311229,#311230),(#311231,#311232,#311233),(#311234,#311235,#311236),(#311237,
#311238,#311239),(#311240,#311241,#311242),(#311243,#311244,#311245),(#311246,
#311247,#311248),(#311249,#311250,#311251),(#311252,#311253,#311254),(#311255,
#311256,#311257),(#311258,#311259,#311260),(#311261,#311262,#311263),(#311264,
#311265,#311266),(#311267,#311268,#311269),(#311270,#311271,#311272),(#311273,
#311274,#311275),(#311276,#311277,#311278),(#311279,#311280,#311281),(#311282,
#311283,#311284),(#311285,#311286,#311287),(#311288,#311289,#311290),(#311291,
#311292,#311293),(#311294,#311295,#311296),(#311297,#311298,#311299)),
 .UNSPECIFIED.,.F.,.F.,.F.,(6,1,1,1,1,1,1,1,1,1,1,1,1,1,1,1,1,1,1,1,1,1,
1,1,1,1,1,1,1,1,1,1,1,1,1,1,1,1,1,1,1,1,1,1,1,1,1,1,1,1,1,1,1,1,1,1,1,1,
1,1,1,1,1,1,1,1,1,1,1,1,1,1,1,1,1,1,1,1,1,1,1,1,1,1,1,1,1,1,1,1,1,1,1,1,
1,1,1,1,1,1,1,1,1,1,1,1,1,1,1,1,1,1,1,1,1,1,1,1,1,1,1,1,1,1,1,1,1,1,1,1,
1,1,1,1,1,1,1,1,1,1,1,1,1,1,1,1,1,1,1,1,1,1,1,1,1,1,1,1,1,1,1,1,1,1,1,1,
1,1,1,1,1,1,1,1,1,1,1,1,1,1,1,1,1,1,1,1,1,1,1,1,1,1,1,1,1,1,1,1,1,1,1,1,
1,1,1,1,1,1,1,1,1,1,1,1,1,1,1,1,1,1,1,1,1,1,1,1,1,1,1,1,1,1,1,1,1,1,1,1,
1,1,1,1,1,1,1,1,1,1,1,1,1,1,1,1,1,1,1,1,1,1,1,1,1,1,1,1,1,1,1,1,1,1,1,1,
1,1,1,1,1,1,1,1,1,1,1,1,1,1,1,1,1,1,1,1,1,1,1,1,1,1,1,1,1,1,1,1,1,1,1,1,
1,1,1,1,1,1,1,1,1,1,1,1,1,1,1,1,1,1,1,1,1,1,1,1,1,1,1,1,1,1,1,1,1,1,1,1,
1,1,1,1,1,1,1,1,1,1,1,1,1,1,1,1,1,1,1,1,1,1,1,1,1,1,1,1,1,1,1,1,1,1,1,1,
1,1,1,1,1,1,1,1,1,1,1,1,1,1,1,1,1,1,1,1,1,1,1,1,1,1,1,1,1,1,1,1,1,1,1,1,
1,1,1,1,1,1,1,1,1,1,1,1,1,1,1,1,1,1,1,1,1,1,1,1,1,1,1,1,1,1,1,1,1,1,1,1,
1,1,1,1,1,1,1,1,1,1,1,1,1,1,1,1,1,1,1,1,1,1,1,1,1,1,1,1,1,1,1,1,1,1,1,1,
1,1,1,1,1,1,1,1,1,1,1,1,1,1,1,1,1,1,1,1,1,1,1,1,1,1,1,1,1,1,1,1,1,1,1,1,
1,1,1,1,1,1,1,1,1,1,1,1,1,1,1,1,1,1,1,6),(2,1,2),(0.,0.001834862,0.003669725,
0.005504587,0.00733945,0.009174312,0.011009174,0.012844037,0.014678899,
0.016513761,0.018348624,0.020183486,0.022018349,0.023853211,0.025688073,
0.027522936,0.029357798,0.031192661,0.033027523,0.034862385,0.036697248,
0.03853211,0.040366972,0.042201835,0.044036697,0.04587156,0.047706422,0.049541284,
0.051376147,0.053211009,0.055045872,0.056880734,0.058715596,0.060550459,
0.062385321,0.064220183,0.066055046,0.067889908,0.069724771,0.071559633,
0.073394495,0.075229358,0.07706422,0.078899083,0.080733945,0.082568807,
0.08440367,0.086238532,0.088073394,0.089908257,0.091743119,0.093577982,
0.095412844,0.097247706,0.099082569,0.100917431,0.102752294,0.104587156,
0.106422018,0.108256881,0.110091743,0.111926606,0.113761468,0.11559633,
0.117431193,0.119266055,0.121100917,0.12293578,0.124770642,0.126605505,
0.128440367,0.130275229,0.132110092,0.133944954,0.135779817,0.137614679,
0.139449541,0.141284404,0.143119266,0.144954128,0.146788991,0.148623853,
0.150458716,0.152293578,0.15412844,0.155963303,0.157798165,0.159633028,
0.16146789,0.163302752,0.165137615,0.166972477,0.168807339,0.170642202,
0.172477064,0.174311927,0.176146789,0.177981651,0.179816514,0.181651376,
0.183486239,0.185321101,0.187155963,0.188990826,0.190825688,0.19266055,
0.194495413,0.196330275,0.198165138,0.2,0.201834862,0.203669725,0.205504587,
0.20733945,0.209174312,0.211009174,0.212844037,0.214678899,0.216513761,
0.218348624,0.220183486,0.222018349,0.223853211,0.225688073,0.227522936,
0.229357798,0.231192661,0.233027523,0.234862385,0.236697248,0.23853211,
0.240366972,0.242201835,0.244036697,0.24587156,0.247706422,0.249541284,
0.251376147,0.253211009,0.255045872,0.256880734,0.258715596,0.260550459,
0.262385321,0.264220183,0.266055046,0.267889908,0.269724771,0.271559633,
0.273394495,0.275229358,0.27706422,0.278899083,0.280733945,0.282568807,
0.28440367,0.286238532,0.288073394,0.289908257,0.291743119,0.293577982,
0.295412844,0.297247706,0.299082569,0.300917431,0.302752294,0.304587156,
0.306422018,0.308256881,0.310091743,0.311926606,0.313761468,0.31559633,
0.317431193,0.319266055,0.321100917,0.32293578,0.324770642,0.326605505,
0.328440367,0.330275229,0.332110092,0.333944954,0.335779817,0.337614679,
0.339449541,0.341284404,0.343119266,0.344954128,0.346788991,0.348623853,
0.350458716,0.352293578,0.35412844,0.355963303,0.357798165,0.359633028,
0.36146789,0.363302752,0.365137615,0.366972477,0.368807339,0.370642202,
0.372477064,0.374311927,0.376146789,0.377981651,0.379816514,0.381651376,
0.383486239,0.385321101,0.387155963,0.388990826,0.390825688,0.39266055,
0.394495413,0.396330275,0.398165138,0.4,0.401834862,0.403669725,0.405504587,
0.40733945,0.409174312,0.411009174,0.412844037,0.414678899,0.416513761,
0.418348624,0.420183486,0.422018349,0.423853211,0.425688073,0.427522936,
0.429357798,0.431192661,0.433027523,0.434862385,0.436697248,0.43853211,
0.440366972,0.442201835,0.444036697,0.44587156,0.447706422,0.449541284,
0.451376147,0.453211009,0.455045872,0.456880734,0.458715596,0.460550459,
0.462385321,0.464220183,0.466055046,0.467889908,0.469724771,0.471559633,
0.473394495,0.475229358,0.47706422,0.478899083,0.480733945,0.482568807,
0.48440367,0.486238532,0.488073394,0.489908257,0.491743119,0.493577982,
0.495412844,0.497247706,0.499082569,0.500917431,0.502752294,0.504587156,
0.506422018,0.508256881,0.510091743,0.511926606,0.513761468,0.51559633,
0.517431193,0.519266055,0.521100917,0.52293578,0.524770642,0.526605505,
0.528440367,0.530275229,0.532110092,0.533944954,0.535779817,0.537614679,
0.539449541,0.541284404,0.543119266,0.544954128,0.546788991,0.548623853,
0.550458716,0.552293578,0.55412844,0.555963303,0.557798165,0.559633028,
0.56146789,0.563302752,0.565137615,0.566972477,0.568807339,0.570642202,
0.572477064,0.574311927,0.576146789,0.577981651,0.579816514,0.581651376,
0.583486239,0.585321101,0.587155963,0.588990826,0.590825688,0.59266055,
0.594495413,0.596330275,0.598165138,0.6,0.601834862,0.603669725,0.605504587,
0.60733945,0.609174312,0.611009174,0.612844037,0.614678899,0.616513761,
0.618348624,0.620183486,0.622018349,0.623853211,0.625688073,0.627522936,
0.629357798,0.631192661,0.633027523,0.634862385,0.636697248,0.63853211,
0.640366972,0.642201835,0.644036697,0.64587156,0.647706422,0.649541284,
0.651376147,0.653211009,0.655045872,0.656880734,0.658715596,0.660550459,
0.662385321,0.664220183,0.666055046,0.667889908,0.669724771,0.671559633,
0.673394495,0.675229358,0.67706422,0.678899083,0.680733945,0.682568807,
0.68440367,0.686238532,0.688073394,0.689908257,0.691743119,0.693577982,
0.695412844,0.697247706,0.699082569,0.700917431,0.702752294,0.704587156,
0.706422018,0.708256881,0.710091743,0.711926606,0.713761468,0.71559633,
0.717431193,0.719266055,0.721100917,0.72293578,0.724770642,0.726605505,
0.728440367,0.730275229,0.732110092,0.733944954,0.735779817,0.737614679,
0.739449541,0.741284404,0.743119266,0.744954128,0.746788991,0.748623853,
0.750458716,0.752293578,0.75412844,0.755963303,0.757798165,0.759633028,
0.76146789,0.763302752,0.765137615,0.766972477,0.768807339,0.770642202,
0.772477064,0.774311927,0.776146789,0.777981651,0.779816514,0.781651376,
0.783486239,0.785321101,0.787155963,0.788990826,0.790825688,0.79266055,
0.794495413,0.796330275,0.798165138,0.8,0.801834862,0.803669725,0.805504587,
0.80733945,0.809174312,0.811009174,0.812844037,0.814678899,0.816513761,
0.818348624,0.820183486,0.822018349,0.823853211,0.825688073,0.827522936,
0.829357798,0.831192661,0.833027523,0.834862385,0.836697248,0.83853211,
0.840366972,0.842201835,0.844036697,0.84587156,0.847706422,0.849541284,
0.851376147,0.853211009,0.855045872,0.856880734,0.858715596,0.860550459,
0.862385321,0.864220183,0.866055046,0.867889908,0.869724771,0.871559633,
0.873394495,0.875229358,0.87706422,0.878899083,0.880733945,0.882568807,
0.88440367,0.886238532,0.888073394,0.889908257,0.891743119,0.893577982,
0.895412844,0.897247706,0.899082569,0.900917431,0.902752294,0.904587156,
0.906422018,0.908256881,0.910091743,0.911926606,0.913761468,0.91559633,
0.917431193,0.919266055,0.921100917,0.92293578,0.924770642,0.926605505,
0.928440367,0.930275229,0.932110092,0.933944954,0.935779817,0.937614679,
0.939449541,0.941284404,0.943119266,0.944954128,0.946788991,0.948623853,
0.950458716,0.952293578,0.95412844,0.955963303,0.957798165,0.959633028,
0.96146789,0.963302752,0.965137615,0.966972477,0.968807339,0.970642202,
0.972477064,0.974311927,0.976146789,0.977981651,0.979816514,0.981651376,
0.983486239,0.985321101,0.987155963,0.988990826,0.990825688,0.99266055,
0.994495413,0.996330275,0.998165138,1.),(0.3,1.,1.3),.UNSPECIFIED.);
#6309=B_SPLINE_SURFACE_WITH_KNOTS('',5,1,((#311318,#311319,#311320),(#311321,
#311322,#311323),(#311324,#311325,#311326),(#311327,#311328,#311329),(#311330,
#311331,#311332),(#311333,#311334,#311335),(#311336,#311337,#311338),(#311339,
#311340,#311341),(#311342,#311343,#311344),(#311345,#311346,#311347),(#311348,
#311349,#311350),(#311351,#311352,#311353),(#311354,#311355,#311356),(#311357,
#311358,#311359),(#311360,#311361,#311362),(#311363,#311364,#311365),(#311366,
#311367,#311368),(#311369,#311370,#311371),(#311372,#311373,#311374),(#311375,
#311376,#311377),(#311378,#311379,#311380),(#311381,#311382,#311383),(#311384,
#311385,#311386),(#311387,#311388,#311389),(#311390,#311391,#311392),(#311393,
#311394,#311395),(#311396,#311397,#311398),(#311399,#311400,#311401),(#311402,
#311403,#311404),(#311405,#311406,#311407),(#311408,#311409,#311410),(#311411,
#311412,#311413),(#311414,#311415,#311416),(#311417,#311418,#311419),(#311420,
#311421,#311422),(#311423,#311424,#311425),(#311426,#311427,#311428),(#311429,
#311430,#311431),(#311432,#311433,#311434),(#311435,#311436,#311437),(#311438,
#311439,#311440),(#311441,#311442,#311443),(#311444,#311445,#311446),(#311447,
#311448,#311449),(#311450,#311451,#311452),(#311453,#311454,#311455),(#311456,
#311457,#311458),(#311459,#311460,#311461),(#311462,#311463,#311464),(#311465,
#311466,#311467),(#311468,#311469,#311470),(#311471,#311472,#311473),(#311474,
#311475,#311476),(#311477,#311478,#311479),(#311480,#311481,#311482),(#311483,
#311484,#311485),(#311486,#311487,#311488),(#311489,#311490,#311491),(#311492,
#311493,#311494),(#311495,#311496,#311497),(#311498,#311499,#311500),(#311501,
#311502,#311503),(#311504,#311505,#311506),(#311507,#311508,#311509),(#311510,
#311511,#311512),(#311513,#311514,#311515),(#311516,#311517,#311518),(#311519,
#311520,#311521),(#311522,#311523,#311524),(#311525,#311526,#311527),(#311528,
#311529,#311530),(#311531,#311532,#311533),(#311534,#311535,#311536),(#311537,
#311538,#311539),(#311540,#311541,#311542),(#311543,#311544,#311545),(#311546,
#311547,#311548),(#311549,#311550,#311551),(#311552,#311553,#311554),(#311555,
#311556,#311557),(#311558,#311559,#311560),(#311561,#311562,#311563),(#311564,
#311565,#311566),(#311567,#311568,#311569),(#311570,#311571,#311572),(#311573,
#311574,#311575),(#311576,#311577,#311578),(#311579,#311580,#311581),(#311582,
#311583,#311584),(#311585,#311586,#311587),(#311588,#311589,#311590),(#311591,
#311592,#311593),(#311594,#311595,#311596),(#311597,#311598,#311599),(#311600,
#311601,#311602),(#311603,#311604,#311605),(#311606,#311607,#311608),(#311609,
#311610,#311611),(#311612,#311613,#311614),(#311615,#311616,#311617),(#311618,
#311619,#311620),(#311621,#311622,#311623),(#311624,#311625,#311626),(#311627,
#311628,#311629),(#311630,#311631,#311632),(#311633,#311634,#311635),(#311636,
#311637,#311638),(#311639,#311640,#311641),(#311642,#311643,#311644),(#311645,
#311646,#311647),(#311648,#311649,#311650),(#311651,#311652,#311653),(#311654,
#311655,#311656),(#311657,#311658,#311659),(#311660,#311661,#311662),(#311663,
#311664,#311665),(#311666,#311667,#311668),(#311669,#311670,#311671),(#311672,
#311673,#311674),(#311675,#311676,#311677),(#311678,#311679,#311680),(#311681,
#311682,#311683),(#311684,#311685,#311686),(#311687,#311688,#311689),(#311690,
#311691,#311692),(#311693,#311694,#311695),(#311696,#311697,#311698),(#311699,
#311700,#311701),(#311702,#311703,#311704),(#311705,#311706,#311707),(#311708,
#311709,#311710),(#311711,#311712,#311713),(#311714,#311715,#311716),(#311717,
#311718,#311719),(#311720,#311721,#311722),(#311723,#311724,#311725),(#311726,
#311727,#311728),(#311729,#311730,#311731),(#311732,#311733,#311734),(#311735,
#311736,#311737),(#311738,#311739,#311740),(#311741,#311742,#311743),(#311744,
#311745,#311746),(#311747,#311748,#311749),(#311750,#311751,#311752),(#311753,
#311754,#311755),(#311756,#311757,#311758),(#311759,#311760,#311761),(#311762,
#311763,#311764),(#311765,#311766,#311767),(#311768,#311769,#311770),(#311771,
#311772,#311773),(#311774,#311775,#311776),(#311777,#311778,#311779),(#311780,
#311781,#311782),(#311783,#311784,#311785),(#311786,#311787,#311788),(#311789,
#311790,#311791),(#311792,#311793,#311794),(#311795,#311796,#311797),(#311798,
#311799,#311800),(#311801,#311802,#311803),(#311804,#311805,#311806),(#311807,
#311808,#311809),(#311810,#311811,#311812),(#311813,#311814,#311815),(#311816,
#311817,#311818),(#311819,#311820,#311821),(#311822,#311823,#311824),(#311825,
#311826,#311827),(#311828,#311829,#311830),(#311831,#311832,#311833),(#311834,
#311835,#311836),(#311837,#311838,#311839),(#311840,#311841,#311842),(#311843,
#311844,#311845),(#311846,#311847,#311848),(#311849,#311850,#311851),(#311852,
#311853,#311854),(#311855,#311856,#311857),(#311858,#311859,#311860),(#311861,
#311862,#311863),(#311864,#311865,#311866),(#311867,#311868,#311869),(#311870,
#311871,#311872),(#311873,#311874,#311875),(#311876,#311877,#311878),(#311879,
#311880,#311881),(#311882,#311883,#311884),(#311885,#311886,#311887),(#311888,
#311889,#311890),(#311891,#311892,#311893),(#311894,#311895,#311896),(#311897,
#311898,#311899),(#311900,#311901,#311902),(#311903,#311904,#311905),(#311906,
#311907,#311908),(#311909,#311910,#311911),(#311912,#311913,#311914),(#311915,
#311916,#311917),(#311918,#311919,#311920),(#311921,#311922,#311923),(#311924,
#311925,#311926),(#311927,#311928,#311929),(#311930,#311931,#311932),(#311933,
#311934,#311935),(#311936,#311937,#311938),(#311939,#311940,#311941),(#311942,
#311943,#311944),(#311945,#311946,#311947),(#311948,#311949,#311950),(#311951,
#311952,#311953),(#311954,#311955,#311956),(#311957,#311958,#311959),(#311960,
#311961,#311962),(#311963,#311964,#311965),(#311966,#311967,#311968),(#311969,
#311970,#311971),(#311972,#311973,#311974),(#311975,#311976,#311977),(#311978,
#311979,#311980),(#311981,#311982,#311983),(#311984,#311985,#311986),(#311987,
#311988,#311989),(#311990,#311991,#311992),(#311993,#311994,#311995),(#311996,
#311997,#311998),(#311999,#312000,#312001),(#312002,#312003,#312004),(#312005,
#312006,#312007),(#312008,#312009,#312010),(#312011,#312012,#312013),(#312014,
#312015,#312016),(#312017,#312018,#312019),(#312020,#312021,#312022),(#312023,
#312024,#312025),(#312026,#312027,#312028),(#312029,#312030,#312031),(#312032,
#312033,#312034),(#312035,#312036,#312037),(#312038,#312039,#312040),(#312041,
#312042,#312043),(#312044,#312045,#312046),(#312047,#312048,#312049),(#312050,
#312051,#312052),(#312053,#312054,#312055),(#312056,#312057,#312058),(#312059,
#312060,#312061),(#312062,#312063,#312064),(#312065,#312066,#312067),(#312068,
#312069,#312070),(#312071,#312072,#312073),(#312074,#312075,#312076),(#312077,
#312078,#312079),(#312080,#312081,#312082),(#312083,#312084,#312085),(#312086,
#312087,#312088),(#312089,#312090,#312091),(#312092,#312093,#312094),(#312095,
#312096,#312097),(#312098,#312099,#312100),(#312101,#312102,#312103),(#312104,
#312105,#312106),(#312107,#312108,#312109),(#312110,#312111,#312112),(#312113,
#312114,#312115),(#312116,#312117,#312118),(#312119,#312120,#312121),(#312122,
#312123,#312124),(#312125,#312126,#312127),(#312128,#312129,#312130),(#312131,
#312132,#312133),(#312134,#312135,#312136),(#312137,#312138,#312139),(#312140,
#312141,#312142),(#312143,#312144,#312145),(#312146,#312147,#312148),(#312149,
#312150,#312151),(#312152,#312153,#312154),(#312155,#312156,#312157),(#312158,
#312159,#312160),(#312161,#312162,#312163),(#312164,#312165,#312166),(#312167,
#312168,#312169),(#312170,#312171,#312172),(#312173,#312174,#312175),(#312176,
#312177,#312178),(#312179,#312180,#312181),(#312182,#312183,#312184),(#312185,
#312186,#312187),(#312188,#312189,#312190),(#312191,#312192,#312193),(#312194,
#312195,#312196),(#312197,#312198,#312199),(#312200,#312201,#312202),(#312203,
#312204,#312205),(#312206,#312207,#312208),(#312209,#312210,#312211),(#312212,
#312213,#312214),(#312215,#312216,#312217),(#312218,#312219,#312220),(#312221,
#312222,#312223),(#312224,#312225,#312226),(#312227,#312228,#312229),(#312230,
#312231,#312232),(#312233,#312234,#312235),(#312236,#312237,#312238),(#312239,
#312240,#312241),(#312242,#312243,#312244),(#312245,#312246,#312247),(#312248,
#312249,#312250),(#312251,#312252,#312253),(#312254,#312255,#312256),(#312257,
#312258,#312259),(#312260,#312261,#312262),(#312263,#312264,#312265),(#312266,
#312267,#312268),(#312269,#312270,#312271),(#312272,#312273,#312274),(#312275,
#312276,#312277),(#312278,#312279,#312280),(#312281,#312282,#312283),(#312284,
#312285,#312286),(#312287,#312288,#312289),(#312290,#312291,#312292),(#312293,
#312294,#312295),(#312296,#312297,#312298),(#312299,#312300,#312301),(#312302,
#312303,#312304),(#312305,#312306,#312307),(#312308,#312309,#312310),(#312311,
#312312,#312313),(#312314,#312315,#312316),(#312317,#312318,#312319),(#312320,
#312321,#312322),(#312323,#312324,#312325),(#312326,#312327,#312328),(#312329,
#312330,#312331),(#312332,#312333,#312334),(#312335,#312336,#312337),(#312338,
#312339,#312340),(#312341,#312342,#312343),(#312344,#312345,#312346),(#312347,
#312348,#312349),(#312350,#312351,#312352),(#312353,#312354,#312355),(#312356,
#312357,#312358),(#312359,#312360,#312361),(#312362,#312363,#312364),(#312365,
#312366,#312367),(#312368,#312369,#312370),(#312371,#312372,#312373),(#312374,
#312375,#312376),(#312377,#312378,#312379),(#312380,#312381,#312382),(#312383,
#312384,#312385),(#312386,#312387,#312388),(#312389,#312390,#312391),(#312392,
#312393,#312394),(#312395,#312396,#312397),(#312398,#312399,#312400),(#312401,
#312402,#312403),(#312404,#312405,#312406),(#312407,#312408,#312409),(#312410,
#312411,#312412),(#312413,#312414,#312415),(#312416,#312417,#312418),(#312419,
#312420,#312421),(#312422,#312423,#312424),(#312425,#312426,#312427),(#312428,
#312429,#312430),(#312431,#312432,#312433),(#312434,#312435,#312436),(#312437,
#312438,#312439),(#312440,#312441,#312442),(#312443,#312444,#312445),(#312446,
#312447,#312448),(#312449,#312450,#312451),(#312452,#312453,#312454),(#312455,
#312456,#312457),(#312458,#312459,#312460),(#312461,#312462,#312463),(#312464,
#312465,#312466),(#312467,#312468,#312469),(#312470,#312471,#312472),(#312473,
#312474,#312475),(#312476,#312477,#312478),(#312479,#312480,#312481),(#312482,
#312483,#312484),(#312485,#312486,#312487),(#312488,#312489,#312490),(#312491,
#312492,#312493),(#312494,#312495,#312496),(#312497,#312498,#312499),(#312500,
#312501,#312502),(#312503,#312504,#312505),(#312506,#312507,#312508),(#312509,
#312510,#312511),(#312512,#312513,#312514),(#312515,#312516,#312517),(#312518,
#312519,#312520),(#312521,#312522,#312523),(#312524,#312525,#312526),(#312527,
#312528,#312529),(#312530,#312531,#312532),(#312533,#312534,#312535),(#312536,
#312537,#312538),(#312539,#312540,#312541),(#312542,#312543,#312544),(#312545,
#312546,#312547),(#312548,#312549,#312550),(#312551,#312552,#312553),(#312554,
#312555,#312556),(#312557,#312558,#312559),(#312560,#312561,#312562),(#312563,
#312564,#312565),(#312566,#312567,#312568),(#312569,#312570,#312571),(#312572,
#312573,#312574),(#312575,#312576,#312577),(#312578,#312579,#312580),(#312581,
#312582,#312583),(#312584,#312585,#312586),(#312587,#312588,#312589),(#312590,
#312591,#312592),(#312593,#312594,#312595),(#312596,#312597,#312598),(#312599,
#312600,#312601),(#312602,#312603,#312604),(#312605,#312606,#312607),(#312608,
#312609,#312610),(#312611,#312612,#312613),(#312614,#312615,#312616),(#312617,
#312618,#312619),(#312620,#312621,#312622),(#312623,#312624,#312625),(#312626,
#312627,#312628),(#312629,#312630,#312631),(#312632,#312633,#312634),(#312635,
#312636,#312637),(#312638,#312639,#312640),(#312641,#312642,#312643),(#312644,
#312645,#312646),(#312647,#312648,#312649),(#312650,#312651,#312652),(#312653,
#312654,#312655),(#312656,#312657,#312658),(#312659,#312660,#312661),(#312662,
#312663,#312664),(#312665,#312666,#312667),(#312668,#312669,#312670),(#312671,
#312672,#312673),(#312674,#312675,#312676),(#312677,#312678,#312679),(#312680,
#312681,#312682),(#312683,#312684,#312685),(#312686,#312687,#312688),(#312689,
#312690,#312691),(#312692,#312693,#312694),(#312695,#312696,#312697),(#312698,
#312699,#312700),(#312701,#312702,#312703),(#312704,#312705,#312706),(#312707,
#312708,#312709),(#312710,#312711,#312712),(#312713,#312714,#312715),(#312716,
#312717,#312718),(#312719,#312720,#312721),(#312722,#312723,#312724),(#312725,
#312726,#312727),(#312728,#312729,#312730),(#312731,#312732,#312733),(#312734,
#312735,#312736),(#312737,#312738,#312739),(#312740,#312741,#312742),(#312743,
#312744,#312745),(#312746,#312747,#312748),(#312749,#312750,#312751),(#312752,
#312753,#312754),(#312755,#312756,#312757),(#312758,#312759,#312760),(#312761,
#312762,#312763),(#312764,#312765,#312766),(#312767,#312768,#312769),(#312770,
#312771,#312772),(#312773,#312774,#312775),(#312776,#312777,#312778),(#312779,
#312780,#312781),(#312782,#312783,#312784),(#312785,#312786,#312787),(#312788,
#312789,#312790),(#312791,#312792,#312793),(#312794,#312795,#312796),(#312797,
#312798,#312799),(#312800,#312801,#312802),(#312803,#312804,#312805),(#312806,
#312807,#312808),(#312809,#312810,#312811),(#312812,#312813,#312814),(#312815,
#312816,#312817),(#312818,#312819,#312820),(#312821,#312822,#312823),(#312824,
#312825,#312826),(#312827,#312828,#312829),(#312830,#312831,#312832),(#312833,
#312834,#312835),(#312836,#312837,#312838),(#312839,#312840,#312841),(#312842,
#312843,#312844),(#312845,#312846,#312847),(#312848,#312849,#312850),(#312851,
#312852,#312853),(#312854,#312855,#312856),(#312857,#312858,#312859),(#312860,
#312861,#312862),(#312863,#312864,#312865),(#312866,#312867,#312868),(#312869,
#312870,#312871),(#312872,#312873,#312874),(#312875,#312876,#312877),(#312878,
#312879,#312880),(#312881,#312882,#312883),(#312884,#312885,#312886),(#312887,
#312888,#312889),(#312890,#312891,#312892),(#312893,#312894,#312895),(#312896,
#312897,#312898),(#312899,#312900,#312901),(#312902,#312903,#312904),(#312905,
#312906,#312907),(#312908,#312909,#312910),(#312911,#312912,#312913),(#312914,
#312915,#312916),(#312917,#312918,#312919),(#312920,#312921,#312922),(#312923,
#312924,#312925),(#312926,#312927,#312928),(#312929,#312930,#312931),(#312932,
#312933,#312934),(#312935,#312936,#312937),(#312938,#312939,#312940),(#312941,
#312942,#312943),(#312944,#312945,#312946),(#312947,#312948,#312949),(#312950,
#312951,#312952),(#312953,#312954,#312955),(#312956,#312957,#312958),(#312959,
#312960,#312961),(#312962,#312963,#312964),(#312965,#312966,#312967)),
 .UNSPECIFIED.,.F.,.F.,.F.,(6,1,1,1,1,1,1,1,1,1,1,1,1,1,1,1,1,1,1,1,1,1,
1,1,1,1,1,1,1,1,1,1,1,1,1,1,1,1,1,1,1,1,1,1,1,1,1,1,1,1,1,1,1,1,1,1,1,1,
1,1,1,1,1,1,1,1,1,1,1,1,1,1,1,1,1,1,1,1,1,1,1,1,1,1,1,1,1,1,1,1,1,1,1,1,
1,1,1,1,1,1,1,1,1,1,1,1,1,1,1,1,1,1,1,1,1,1,1,1,1,1,1,1,1,1,1,1,1,1,1,1,
1,1,1,1,1,1,1,1,1,1,1,1,1,1,1,1,1,1,1,1,1,1,1,1,1,1,1,1,1,1,1,1,1,1,1,1,
1,1,1,1,1,1,1,1,1,1,1,1,1,1,1,1,1,1,1,1,1,1,1,1,1,1,1,1,1,1,1,1,1,1,1,1,
1,1,1,1,1,1,1,1,1,1,1,1,1,1,1,1,1,1,1,1,1,1,1,1,1,1,1,1,1,1,1,1,1,1,1,1,
1,1,1,1,1,1,1,1,1,1,1,1,1,1,1,1,1,1,1,1,1,1,1,1,1,1,1,1,1,1,1,1,1,1,1,1,
1,1,1,1,1,1,1,1,1,1,1,1,1,1,1,1,1,1,1,1,1,1,1,1,1,1,1,1,1,1,1,1,1,1,1,1,
1,1,1,1,1,1,1,1,1,1,1,1,1,1,1,1,1,1,1,1,1,1,1,1,1,1,1,1,1,1,1,1,1,1,1,1,
1,1,1,1,1,1,1,1,1,1,1,1,1,1,1,1,1,1,1,1,1,1,1,1,1,1,1,1,1,1,1,1,1,1,1,1,
1,1,1,1,1,1,1,1,1,1,1,1,1,1,1,1,1,1,1,1,1,1,1,1,1,1,1,1,1,1,1,1,1,1,1,1,
1,1,1,1,1,1,1,1,1,1,1,1,1,1,1,1,1,1,1,1,1,1,1,1,1,1,1,1,1,1,1,1,1,1,1,1,
1,1,1,1,1,1,1,1,1,1,1,1,1,1,1,1,1,1,1,1,1,1,1,1,1,1,1,1,1,1,1,1,1,1,1,1,
1,1,1,1,1,1,1,1,1,1,1,1,1,1,1,1,1,1,1,1,1,1,1,1,1,1,1,1,1,1,1,1,1,1,1,1,
1,1,1,1,1,1,1,1,1,1,1,1,1,1,1,1,1,1,1,6),(2,1,2),(-1.,-0.998165138,-0.996330275,
-0.994495413,-0.99266055,-0.990825688,-0.988990826,-0.987155963,-0.985321101,
-0.983486239,-0.981651376,-0.979816514,-0.977981651,-0.976146789,-0.974311927,
-0.972477064,-0.970642202,-0.968807339,-0.966972477,-0.965137615,-0.963302752,
-0.96146789,-0.959633028,-0.957798165,-0.955963303,-0.95412844,-0.952293578,
-0.950458716,-0.948623853,-0.946788991,-0.944954128,-0.943119266,-0.941284404,
-0.939449541,-0.937614679,-0.935779817,-0.933944954,-0.932110092,-0.930275229,
-0.928440367,-0.926605505,-0.924770642,-0.92293578,-0.921100917,-0.919266055,
-0.917431193,-0.91559633,-0.913761468,-0.911926606,-0.910091743,-0.908256881,
-0.906422018,-0.904587156,-0.902752294,-0.900917431,-0.899082569,-0.897247706,
-0.895412844,-0.893577982,-0.891743119,-0.889908257,-0.888073394,-0.886238532,
-0.88440367,-0.882568807,-0.880733945,-0.878899083,-0.87706422,-0.875229358,
-0.873394495,-0.871559633,-0.869724771,-0.867889908,-0.866055046,-0.864220183,
-0.862385321,-0.860550459,-0.858715596,-0.856880734,-0.855045872,-0.853211009,
-0.851376147,-0.849541284,-0.847706422,-0.84587156,-0.844036697,-0.842201835,
-0.840366972,-0.83853211,-0.836697248,-0.834862385,-0.833027523,-0.831192661,
-0.829357798,-0.827522936,-0.825688073,-0.823853211,-0.822018349,-0.820183486,
-0.818348624,-0.816513761,-0.814678899,-0.812844037,-0.811009174,-0.809174312,
-0.80733945,-0.805504587,-0.803669725,-0.801834862,-0.8,-0.798165138,-0.796330275,
-0.794495413,-0.79266055,-0.790825688,-0.788990826,-0.787155963,-0.785321101,
-0.783486239,-0.781651376,-0.779816514,-0.777981651,-0.776146789,-0.774311927,
-0.772477064,-0.770642202,-0.768807339,-0.766972477,-0.765137615,-0.763302752,
-0.76146789,-0.759633028,-0.757798165,-0.755963303,-0.75412844,-0.752293578,
-0.750458716,-0.748623853,-0.746788991,-0.744954128,-0.743119266,-0.741284404,
-0.739449541,-0.737614679,-0.735779817,-0.733944954,-0.732110092,-0.730275229,
-0.728440367,-0.726605505,-0.724770642,-0.72293578,-0.721100917,-0.719266055,
-0.717431193,-0.71559633,-0.713761468,-0.711926606,-0.710091743,-0.708256881,
-0.706422018,-0.704587156,-0.702752294,-0.700917431,-0.699082569,-0.697247706,
-0.695412844,-0.693577982,-0.691743119,-0.689908257,-0.688073394,-0.686238532,
-0.68440367,-0.682568807,-0.680733945,-0.678899083,-0.67706422,-0.675229358,
-0.673394495,-0.671559633,-0.669724771,-0.667889908,-0.666055046,-0.664220183,
-0.662385321,-0.660550459,-0.658715596,-0.656880734,-0.655045872,-0.653211009,
-0.651376147,-0.649541284,-0.647706422,-0.64587156,-0.644036697,-0.642201835,
-0.640366972,-0.63853211,-0.636697248,-0.634862385,-0.633027523,-0.631192661,
-0.629357798,-0.627522936,-0.625688073,-0.623853211,-0.622018349,-0.620183486,
-0.618348624,-0.616513761,-0.614678899,-0.612844037,-0.611009174,-0.609174312,
-0.60733945,-0.605504587,-0.603669725,-0.601834862,-0.6,-0.598165138,-0.596330275,
-0.594495413,-0.59266055,-0.590825688,-0.588990826,-0.587155963,-0.585321101,
-0.583486239,-0.581651376,-0.579816514,-0.577981651,-0.576146789,-0.574311927,
-0.572477064,-0.570642202,-0.568807339,-0.566972477,-0.565137615,-0.563302752,
-0.56146789,-0.559633028,-0.557798165,-0.555963303,-0.55412844,-0.552293578,
-0.550458716,-0.548623853,-0.546788991,-0.544954128,-0.543119266,-0.541284404,
-0.539449541,-0.537614679,-0.535779817,-0.533944954,-0.532110092,-0.530275229,
-0.528440367,-0.526605505,-0.524770642,-0.52293578,-0.521100917,-0.519266055,
-0.517431193,-0.51559633,-0.513761468,-0.511926606,-0.510091743,-0.508256881,
-0.506422018,-0.504587156,-0.502752294,-0.500917431,-0.499082569,-0.497247706,
-0.495412844,-0.493577982,-0.491743119,-0.489908257,-0.488073394,-0.486238532,
-0.48440367,-0.482568807,-0.480733945,-0.478899083,-0.47706422,-0.475229358,
-0.473394495,-0.471559633,-0.469724771,-0.467889908,-0.466055046,-0.464220183,
-0.462385321,-0.460550459,-0.458715596,-0.456880734,-0.455045872,-0.453211009,
-0.451376147,-0.449541284,-0.447706422,-0.44587156,-0.444036697,-0.442201835,
-0.440366972,-0.43853211,-0.436697248,-0.434862385,-0.433027523,-0.431192661,
-0.429357798,-0.427522936,-0.425688073,-0.423853211,-0.422018349,-0.420183486,
-0.418348624,-0.416513761,-0.414678899,-0.412844037,-0.411009174,-0.409174312,
-0.40733945,-0.405504587,-0.403669725,-0.401834862,-0.4,-0.398165138,-0.396330275,
-0.394495413,-0.39266055,-0.390825688,-0.388990826,-0.387155963,-0.385321101,
-0.383486239,-0.381651376,-0.379816514,-0.377981651,-0.376146789,-0.374311927,
-0.372477064,-0.370642202,-0.368807339,-0.366972477,-0.365137615,-0.363302752,
-0.36146789,-0.359633028,-0.357798165,-0.355963303,-0.35412844,-0.352293578,
-0.350458716,-0.348623853,-0.346788991,-0.344954128,-0.343119266,-0.341284404,
-0.339449541,-0.337614679,-0.335779817,-0.333944954,-0.332110092,-0.330275229,
-0.328440367,-0.326605505,-0.324770642,-0.32293578,-0.321100917,-0.319266055,
-0.317431193,-0.31559633,-0.313761468,-0.311926606,-0.310091743,-0.308256881,
-0.306422018,-0.304587156,-0.302752294,-0.300917431,-0.299082569,-0.297247706,
-0.295412844,-0.293577982,-0.291743119,-0.289908257,-0.288073394,-0.286238532,
-0.28440367,-0.282568807,-0.280733945,-0.278899083,-0.27706422,-0.275229358,
-0.273394495,-0.271559633,-0.269724771,-0.267889908,-0.266055046,-0.264220183,
-0.262385321,-0.260550459,-0.258715596,-0.256880734,-0.255045872,-0.253211009,
-0.251376147,-0.249541284,-0.247706422,-0.24587156,-0.244036697,-0.242201835,
-0.240366972,-0.23853211,-0.236697248,-0.234862385,-0.233027523,-0.231192661,
-0.229357798,-0.227522936,-0.225688073,-0.223853211,-0.222018349,-0.220183486,
-0.218348624,-0.216513761,-0.214678899,-0.212844037,-0.211009174,-0.209174312,
-0.20733945,-0.205504587,-0.203669725,-0.201834862,-0.2,-0.198165138,-0.196330275,
-0.194495413,-0.19266055,-0.190825688,-0.188990826,-0.187155963,-0.185321101,
-0.183486239,-0.181651376,-0.179816514,-0.177981651,-0.176146789,-0.174311927,
-0.172477064,-0.170642202,-0.168807339,-0.166972477,-0.165137615,-0.163302752,
-0.16146789,-0.159633028,-0.157798165,-0.155963303,-0.15412844,-0.152293578,
-0.150458716,-0.148623853,-0.146788991,-0.144954128,-0.143119266,-0.141284404,
-0.139449541,-0.137614679,-0.135779817,-0.133944954,-0.132110092,-0.130275229,
-0.128440367,-0.126605505,-0.124770642,-0.12293578,-0.121100917,-0.119266055,
-0.117431193,-0.11559633,-0.113761468,-0.111926606,-0.110091743,-0.108256881,
-0.106422018,-0.104587156,-0.102752294,-0.100917431,-0.099082569,-0.097247706,
-0.095412844,-0.093577982,-0.091743119,-0.089908257,-0.088073394,-0.086238532,
-0.08440367,-0.082568807,-0.080733945,-0.078899083,-0.07706422,-0.075229358,
-0.073394495,-0.071559633,-0.069724771,-0.067889908,-0.066055046,-0.064220183,
-0.062385321,-0.060550459,-0.058715596,-0.056880734,-0.055045872,-0.053211009,
-0.051376147,-0.049541284,-0.047706422,-0.04587156,-0.044036697,-0.042201835,
-0.040366972,-0.03853211,-0.036697248,-0.034862385,-0.033027523,-0.031192661,
-0.029357798,-0.027522936,-0.025688073,-0.023853211,-0.022018349,-0.020183486,
-0.018348624,-0.016513761,-0.014678899,-0.012844037,-0.011009174,-0.009174312,
-0.00733945,-0.005504587,-0.003669725,-0.001834862,0.00098212),(0.3,1.,
1.3),.UNSPECIFIED.);
#6310=B_SPLINE_SURFACE_WITH_KNOTS('',5,1,((#312990,#312991,#312992),(#312993,
#312994,#312995),(#312996,#312997,#312998),(#312999,#313000,#313001),(#313002,
#313003,#313004),(#313005,#313006,#313007),(#313008,#313009,#313010),(#313011,
#313012,#313013),(#313014,#313015,#313016),(#313017,#313018,#313019),(#313020,
#313021,#313022),(#313023,#313024,#313025),(#313026,#313027,#313028),(#313029,
#313030,#313031),(#313032,#313033,#313034),(#313035,#313036,#313037),(#313038,
#313039,#313040),(#313041,#313042,#313043),(#313044,#313045,#313046),(#313047,
#313048,#313049),(#313050,#313051,#313052),(#313053,#313054,#313055),(#313056,
#313057,#313058),(#313059,#313060,#313061),(#313062,#313063,#313064),(#313065,
#313066,#313067),(#313068,#313069,#313070),(#313071,#313072,#313073),(#313074,
#313075,#313076),(#313077,#313078,#313079),(#313080,#313081,#313082),(#313083,
#313084,#313085),(#313086,#313087,#313088),(#313089,#313090,#313091),(#313092,
#313093,#313094),(#313095,#313096,#313097),(#313098,#313099,#313100),(#313101,
#313102,#313103),(#313104,#313105,#313106),(#313107,#313108,#313109),(#313110,
#313111,#313112),(#313113,#313114,#313115),(#313116,#313117,#313118),(#313119,
#313120,#313121),(#313122,#313123,#313124),(#313125,#313126,#313127),(#313128,
#313129,#313130),(#313131,#313132,#313133),(#313134,#313135,#313136),(#313137,
#313138,#313139),(#313140,#313141,#313142),(#313143,#313144,#313145),(#313146,
#313147,#313148),(#313149,#313150,#313151),(#313152,#313153,#313154),(#313155,
#313156,#313157),(#313158,#313159,#313160),(#313161,#313162,#313163),(#313164,
#313165,#313166),(#313167,#313168,#313169),(#313170,#313171,#313172),(#313173,
#313174,#313175),(#313176,#313177,#313178),(#313179,#313180,#313181),(#313182,
#313183,#313184),(#313185,#313186,#313187),(#313188,#313189,#313190),(#313191,
#313192,#313193),(#313194,#313195,#313196),(#313197,#313198,#313199),(#313200,
#313201,#313202),(#313203,#313204,#313205),(#313206,#313207,#313208),(#313209,
#313210,#313211),(#313212,#313213,#313214),(#313215,#313216,#313217),(#313218,
#313219,#313220),(#313221,#313222,#313223),(#313224,#313225,#313226),(#313227,
#313228,#313229),(#313230,#313231,#313232),(#313233,#313234,#313235),(#313236,
#313237,#313238),(#313239,#313240,#313241),(#313242,#313243,#313244),(#313245,
#313246,#313247),(#313248,#313249,#313250),(#313251,#313252,#313253),(#313254,
#313255,#313256),(#313257,#313258,#313259),(#313260,#313261,#313262),(#313263,
#313264,#313265),(#313266,#313267,#313268),(#313269,#313270,#313271),(#313272,
#313273,#313274),(#313275,#313276,#313277),(#313278,#313279,#313280),(#313281,
#313282,#313283),(#313284,#313285,#313286),(#313287,#313288,#313289),(#313290,
#313291,#313292),(#313293,#313294,#313295),(#313296,#313297,#313298),(#313299,
#313300,#313301),(#313302,#313303,#313304),(#313305,#313306,#313307),(#313308,
#313309,#313310),(#313311,#313312,#313313),(#313314,#313315,#313316),(#313317,
#313318,#313319),(#313320,#313321,#313322),(#313323,#313324,#313325),(#313326,
#313327,#313328),(#313329,#313330,#313331),(#313332,#313333,#313334),(#313335,
#313336,#313337),(#313338,#313339,#313340),(#313341,#313342,#313343),(#313344,
#313345,#313346),(#313347,#313348,#313349),(#313350,#313351,#313352),(#313353,
#313354,#313355),(#313356,#313357,#313358),(#313359,#313360,#313361),(#313362,
#313363,#313364),(#313365,#313366,#313367),(#313368,#313369,#313370),(#313371,
#313372,#313373),(#313374,#313375,#313376),(#313377,#313378,#313379),(#313380,
#313381,#313382),(#313383,#313384,#313385),(#313386,#313387,#313388),(#313389,
#313390,#313391),(#313392,#313393,#313394),(#313395,#313396,#313397),(#313398,
#313399,#313400),(#313401,#313402,#313403),(#313404,#313405,#313406),(#313407,
#313408,#313409),(#313410,#313411,#313412),(#313413,#313414,#313415),(#313416,
#313417,#313418),(#313419,#313420,#313421),(#313422,#313423,#313424),(#313425,
#313426,#313427),(#313428,#313429,#313430),(#313431,#313432,#313433),(#313434,
#313435,#313436),(#313437,#313438,#313439),(#313440,#313441,#313442),(#313443,
#313444,#313445),(#313446,#313447,#313448),(#313449,#313450,#313451),(#313452,
#313453,#313454),(#313455,#313456,#313457),(#313458,#313459,#313460),(#313461,
#313462,#313463),(#313464,#313465,#313466),(#313467,#313468,#313469),(#313470,
#313471,#313472),(#313473,#313474,#313475),(#313476,#313477,#313478),(#313479,
#313480,#313481),(#313482,#313483,#313484),(#313485,#313486,#313487),(#313488,
#313489,#313490),(#313491,#313492,#313493),(#313494,#313495,#313496),(#313497,
#313498,#313499),(#313500,#313501,#313502),(#313503,#313504,#313505),(#313506,
#313507,#313508),(#313509,#313510,#313511),(#313512,#313513,#313514),(#313515,
#313516,#313517),(#313518,#313519,#313520),(#313521,#313522,#313523),(#313524,
#313525,#313526),(#313527,#313528,#313529),(#313530,#313531,#313532),(#313533,
#313534,#313535),(#313536,#313537,#313538),(#313539,#313540,#313541),(#313542,
#313543,#313544),(#313545,#313546,#313547),(#313548,#313549,#313550),(#313551,
#313552,#313553),(#313554,#313555,#313556),(#313557,#313558,#313559),(#313560,
#313561,#313562),(#313563,#313564,#313565),(#313566,#313567,#313568),(#313569,
#313570,#313571),(#313572,#313573,#313574),(#313575,#313576,#313577),(#313578,
#313579,#313580),(#313581,#313582,#313583),(#313584,#313585,#313586),(#313587,
#313588,#313589),(#313590,#313591,#313592),(#313593,#313594,#313595),(#313596,
#313597,#313598),(#313599,#313600,#313601),(#313602,#313603,#313604),(#313605,
#313606,#313607),(#313608,#313609,#313610),(#313611,#313612,#313613),(#313614,
#313615,#313616),(#313617,#313618,#313619),(#313620,#313621,#313622),(#313623,
#313624,#313625),(#313626,#313627,#313628),(#313629,#313630,#313631),(#313632,
#313633,#313634),(#313635,#313636,#313637),(#313638,#313639,#313640),(#313641,
#313642,#313643),(#313644,#313645,#313646),(#313647,#313648,#313649),(#313650,
#313651,#313652),(#313653,#313654,#313655),(#313656,#313657,#313658),(#313659,
#313660,#313661),(#313662,#313663,#313664),(#313665,#313666,#313667),(#313668,
#313669,#313670),(#313671,#313672,#313673),(#313674,#313675,#313676),(#313677,
#313678,#313679),(#313680,#313681,#313682),(#313683,#313684,#313685),(#313686,
#313687,#313688),(#313689,#313690,#313691),(#313692,#313693,#313694),(#313695,
#313696,#313697),(#313698,#313699,#313700),(#313701,#313702,#313703),(#313704,
#313705,#313706),(#313707,#313708,#313709),(#313710,#313711,#313712),(#313713,
#313714,#313715),(#313716,#313717,#313718),(#313719,#313720,#313721),(#313722,
#313723,#313724),(#313725,#313726,#313727),(#313728,#313729,#313730),(#313731,
#313732,#313733),(#313734,#313735,#313736),(#313737,#313738,#313739),(#313740,
#313741,#313742),(#313743,#313744,#313745),(#313746,#313747,#313748),(#313749,
#313750,#313751),(#313752,#313753,#313754),(#313755,#313756,#313757),(#313758,
#313759,#313760),(#313761,#313762,#313763),(#313764,#313765,#313766),(#313767,
#313768,#313769),(#313770,#313771,#313772),(#313773,#313774,#313775),(#313776,
#313777,#313778),(#313779,#313780,#313781),(#313782,#313783,#313784),(#313785,
#313786,#313787),(#313788,#313789,#313790),(#313791,#313792,#313793),(#313794,
#313795,#313796),(#313797,#313798,#313799),(#313800,#313801,#313802),(#313803,
#313804,#313805),(#313806,#313807,#313808),(#313809,#313810,#313811),(#313812,
#313813,#313814),(#313815,#313816,#313817),(#313818,#313819,#313820),(#313821,
#313822,#313823),(#313824,#313825,#313826),(#313827,#313828,#313829),(#313830,
#313831,#313832),(#313833,#313834,#313835),(#313836,#313837,#313838),(#313839,
#313840,#313841),(#313842,#313843,#313844),(#313845,#313846,#313847),(#313848,
#313849,#313850),(#313851,#313852,#313853),(#313854,#313855,#313856),(#313857,
#313858,#313859),(#313860,#313861,#313862),(#313863,#313864,#313865),(#313866,
#313867,#313868),(#313869,#313870,#313871),(#313872,#313873,#313874),(#313875,
#313876,#313877),(#313878,#313879,#313880),(#313881,#313882,#313883),(#313884,
#313885,#313886),(#313887,#313888,#313889),(#313890,#313891,#313892),(#313893,
#313894,#313895),(#313896,#313897,#313898),(#313899,#313900,#313901),(#313902,
#313903,#313904),(#313905,#313906,#313907),(#313908,#313909,#313910),(#313911,
#313912,#313913),(#313914,#313915,#313916),(#313917,#313918,#313919),(#313920,
#313921,#313922),(#313923,#313924,#313925),(#313926,#313927,#313928),(#313929,
#313930,#313931),(#313932,#313933,#313934),(#313935,#313936,#313937),(#313938,
#313939,#313940),(#313941,#313942,#313943),(#313944,#313945,#313946),(#313947,
#313948,#313949),(#313950,#313951,#313952),(#313953,#313954,#313955),(#313956,
#313957,#313958),(#313959,#313960,#313961),(#313962,#313963,#313964),(#313965,
#313966,#313967),(#313968,#313969,#313970),(#313971,#313972,#313973),(#313974,
#313975,#313976),(#313977,#313978,#313979),(#313980,#313981,#313982),(#313983,
#313984,#313985),(#313986,#313987,#313988),(#313989,#313990,#313991),(#313992,
#313993,#313994),(#313995,#313996,#313997),(#313998,#313999,#314000),(#314001,
#314002,#314003),(#314004,#314005,#314006),(#314007,#314008,#314009),(#314010,
#314011,#314012),(#314013,#314014,#314015),(#314016,#314017,#314018),(#314019,
#314020,#314021),(#314022,#314023,#314024),(#314025,#314026,#314027),(#314028,
#314029,#314030),(#314031,#314032,#314033),(#314034,#314035,#314036),(#314037,
#314038,#314039),(#314040,#314041,#314042),(#314043,#314044,#314045),(#314046,
#314047,#314048),(#314049,#314050,#314051),(#314052,#314053,#314054),(#314055,
#314056,#314057),(#314058,#314059,#314060),(#314061,#314062,#314063),(#314064,
#314065,#314066),(#314067,#314068,#314069),(#314070,#314071,#314072),(#314073,
#314074,#314075),(#314076,#314077,#314078),(#314079,#314080,#314081),(#314082,
#314083,#314084),(#314085,#314086,#314087),(#314088,#314089,#314090),(#314091,
#314092,#314093),(#314094,#314095,#314096),(#314097,#314098,#314099),(#314100,
#314101,#314102),(#314103,#314104,#314105),(#314106,#314107,#314108),(#314109,
#314110,#314111),(#314112,#314113,#314114),(#314115,#314116,#314117),(#314118,
#314119,#314120),(#314121,#314122,#314123),(#314124,#314125,#314126),(#314127,
#314128,#314129),(#314130,#314131,#314132),(#314133,#314134,#314135),(#314136,
#314137,#314138),(#314139,#314140,#314141),(#314142,#314143,#314144),(#314145,
#314146,#314147),(#314148,#314149,#314150),(#314151,#314152,#314153),(#314154,
#314155,#314156),(#314157,#314158,#314159),(#314160,#314161,#314162),(#314163,
#314164,#314165),(#314166,#314167,#314168),(#314169,#314170,#314171),(#314172,
#314173,#314174),(#314175,#314176,#314177),(#314178,#314179,#314180),(#314181,
#314182,#314183),(#314184,#314185,#314186),(#314187,#314188,#314189),(#314190,
#314191,#314192),(#314193,#314194,#314195),(#314196,#314197,#314198),(#314199,
#314200,#314201),(#314202,#314203,#314204),(#314205,#314206,#314207),(#314208,
#314209,#314210),(#314211,#314212,#314213),(#314214,#314215,#314216),(#314217,
#314218,#314219),(#314220,#314221,#314222),(#314223,#314224,#314225),(#314226,
#314227,#314228),(#314229,#314230,#314231),(#314232,#314233,#314234),(#314235,
#314236,#314237),(#314238,#314239,#314240),(#314241,#314242,#314243),(#314244,
#314245,#314246),(#314247,#314248,#314249),(#314250,#314251,#314252),(#314253,
#314254,#314255),(#314256,#314257,#314258),(#314259,#314260,#314261),(#314262,
#314263,#314264),(#314265,#314266,#314267),(#314268,#314269,#314270),(#314271,
#314272,#314273),(#314274,#314275,#314276),(#314277,#314278,#314279),(#314280,
#314281,#314282),(#314283,#314284,#314285),(#314286,#314287,#314288),(#314289,
#314290,#314291),(#314292,#314293,#314294),(#314295,#314296,#314297),(#314298,
#314299,#314300),(#314301,#314302,#314303),(#314304,#314305,#314306),(#314307,
#314308,#314309),(#314310,#314311,#314312),(#314313,#314314,#314315),(#314316,
#314317,#314318),(#314319,#314320,#314321),(#314322,#314323,#314324),(#314325,
#314326,#314327),(#314328,#314329,#314330),(#314331,#314332,#314333),(#314334,
#314335,#314336),(#314337,#314338,#314339),(#314340,#314341,#314342),(#314343,
#314344,#314345),(#314346,#314347,#314348),(#314349,#314350,#314351),(#314352,
#314353,#314354),(#314355,#314356,#314357),(#314358,#314359,#314360),(#314361,
#314362,#314363),(#314364,#314365,#314366),(#314367,#314368,#314369),(#314370,
#314371,#314372),(#314373,#314374,#314375),(#314376,#314377,#314378),(#314379,
#314380,#314381),(#314382,#314383,#314384),(#314385,#314386,#314387),(#314388,
#314389,#314390),(#314391,#314392,#314393),(#314394,#314395,#314396),(#314397,
#314398,#314399),(#314400,#314401,#314402),(#314403,#314404,#314405),(#314406,
#314407,#314408),(#314409,#314410,#314411),(#314412,#314413,#314414),(#314415,
#314416,#314417),(#314418,#314419,#314420),(#314421,#314422,#314423),(#314424,
#314425,#314426),(#314427,#314428,#314429),(#314430,#314431,#314432),(#314433,
#314434,#314435),(#314436,#314437,#314438),(#314439,#314440,#314441),(#314442,
#314443,#314444),(#314445,#314446,#314447),(#314448,#314449,#314450),(#314451,
#314452,#314453),(#314454,#314455,#314456),(#314457,#314458,#314459),(#314460,
#314461,#314462),(#314463,#314464,#314465),(#314466,#314467,#314468),(#314469,
#314470,#314471),(#314472,#314473,#314474),(#314475,#314476,#314477),(#314478,
#314479,#314480),(#314481,#314482,#314483),(#314484,#314485,#314486),(#314487,
#314488,#314489),(#314490,#314491,#314492),(#314493,#314494,#314495),(#314496,
#314497,#314498),(#314499,#314500,#314501),(#314502,#314503,#314504),(#314505,
#314506,#314507),(#314508,#314509,#314510),(#314511,#314512,#314513),(#314514,
#314515,#314516),(#314517,#314518,#314519),(#314520,#314521,#314522),(#314523,
#314524,#314525),(#314526,#314527,#314528),(#314529,#314530,#314531),(#314532,
#314533,#314534),(#314535,#314536,#314537),(#314538,#314539,#314540),(#314541,
#314542,#314543),(#314544,#314545,#314546),(#314547,#314548,#314549),(#314550,
#314551,#314552),(#314553,#314554,#314555),(#314556,#314557,#314558),(#314559,
#314560,#314561),(#314562,#314563,#314564),(#314565,#314566,#314567),(#314568,
#314569,#314570),(#314571,#314572,#314573),(#314574,#314575,#314576),(#314577,
#314578,#314579),(#314580,#314581,#314582),(#314583,#314584,#314585),(#314586,
#314587,#314588),(#314589,#314590,#314591),(#314592,#314593,#314594),(#314595,
#314596,#314597),(#314598,#314599,#314600),(#314601,#314602,#314603),(#314604,
#314605,#314606),(#314607,#314608,#314609),(#314610,#314611,#314612),(#314613,
#314614,#314615),(#314616,#314617,#314618),(#314619,#314620,#314621),(#314622,
#314623,#314624),(#314625,#314626,#314627),(#314628,#314629,#314630),(#314631,
#314632,#314633),(#314634,#314635,#314636),(#314637,#314638,#314639),(#314640,
#314641,#314642)),.UNSPECIFIED.,.F.,.F.,.F.,(6,1,1,1,1,1,1,1,1,1,1,1,1,
1,1,1,1,1,1,1,1,1,1,1,1,1,1,1,1,1,1,1,1,1,1,1,1,1,1,1,1,1,1,1,1,1,1,1,1,
1,1,1,1,1,1,1,1,1,1,1,1,1,1,1,1,1,1,1,1,1,1,1,1,1,1,1,1,1,1,1,1,1,1,1,1,
1,1,1,1,1,1,1,1,1,1,1,1,1,1,1,1,1,1,1,1,1,1,1,1,1,1,1,1,1,1,1,1,1,1,1,1,
1,1,1,1,1,1,1,1,1,1,1,1,1,1,1,1,1,1,1,1,1,1,1,1,1,1,1,1,1,1,1,1,1,1,1,1,
1,1,1,1,1,1,1,1,1,1,1,1,1,1,1,1,1,1,1,1,1,1,1,1,1,1,1,1,1,1,1,1,1,1,1,1,
1,1,1,1,1,1,1,1,1,1,1,1,1,1,1,1,1,1,1,1,1,1,1,1,1,1,1,1,1,1,1,1,1,1,1,1,
1,1,1,1,1,1,1,1,1,1,1,1,1,1,1,1,1,1,1,1,1,1,1,1,1,1,1,1,1,1,1,1,1,1,1,1,
1,1,1,1,1,1,1,1,1,1,1,1,1,1,1,1,1,1,1,1,1,1,1,1,1,1,1,1,1,1,1,1,1,1,1,1,
1,1,1,1,1,1,1,1,1,1,1,1,1,1,1,1,1,1,1,1,1,1,1,1,1,1,1,1,1,1,1,1,1,1,1,1,
1,1,1,1,1,1,1,1,1,1,1,1,1,1,1,1,1,1,1,1,1,1,1,1,1,1,1,1,1,1,1,1,1,1,1,1,
1,1,1,1,1,1,1,1,1,1,1,1,1,1,1,1,1,1,1,1,1,1,1,1,1,1,1,1,1,1,1,1,1,1,1,1,
1,1,1,1,1,1,1,1,1,1,1,1,1,1,1,1,1,1,1,1,1,1,1,1,1,1,1,1,1,1,1,1,1,1,1,1,
1,1,1,1,1,1,1,1,1,1,1,1,1,1,1,1,1,1,1,1,1,1,1,1,1,1,1,1,1,1,1,1,1,1,1,1,
1,1,1,1,1,1,1,1,1,1,1,1,1,1,1,1,1,1,1,1,1,1,1,1,1,1,1,1,1,1,1,1,1,1,1,1,
1,1,1,1,1,1,1,1,1,1,1,1,1,1,1,1,1,1,1,1,1,1,1,1,1,1,1,1,1,6),(2,1,2),(-0.001964204,
0.,0.001834862,0.003669725,0.005504587,0.00733945,0.009174312,0.011009174,
0.012844037,0.014678899,0.016513761,0.018348624,0.020183486,0.022018349,
0.023853211,0.025688073,0.027522936,0.029357798,0.031192661,0.033027523,
0.034862385,0.036697248,0.03853211,0.040366972,0.042201835,0.044036697,
0.04587156,0.047706422,0.049541284,0.051376147,0.053211009,0.055045872,
0.056880734,0.058715596,0.060550459,0.062385321,0.064220183,0.066055046,
0.067889908,0.069724771,0.071559633,0.073394495,0.075229358,0.07706422,
0.078899083,0.080733945,0.082568807,0.08440367,0.086238532,0.088073394,
0.089908257,0.091743119,0.093577982,0.095412844,0.097247706,0.099082569,
0.100917431,0.102752294,0.104587156,0.106422018,0.108256881,0.110091743,
0.111926606,0.113761468,0.11559633,0.117431193,0.119266055,0.121100917,
0.12293578,0.124770642,0.126605505,0.128440367,0.130275229,0.132110092,
0.133944954,0.135779817,0.137614679,0.139449541,0.141284404,0.143119266,
0.144954128,0.146788991,0.148623853,0.150458716,0.152293578,0.15412844,
0.155963303,0.157798165,0.159633028,0.16146789,0.163302752,0.165137615,
0.166972477,0.168807339,0.170642202,0.172477064,0.174311927,0.176146789,
0.177981651,0.179816514,0.181651376,0.183486239,0.185321101,0.187155963,
0.188990826,0.190825688,0.19266055,0.194495413,0.196330275,0.198165138,
0.2,0.201834862,0.203669725,0.205504587,0.20733945,0.209174312,0.211009174,
0.212844037,0.214678899,0.216513761,0.218348624,0.220183486,0.222018349,
0.223853211,0.225688073,0.227522936,0.229357798,0.231192661,0.233027523,
0.234862385,0.236697248,0.23853211,0.240366972,0.242201835,0.244036697,
0.24587156,0.247706422,0.249541284,0.251376147,0.253211009,0.255045872,
0.256880734,0.258715596,0.260550459,0.262385321,0.264220183,0.266055046,
0.267889908,0.269724771,0.271559633,0.273394495,0.275229358,0.27706422,
0.278899083,0.280733945,0.282568807,0.28440367,0.286238532,0.288073394,
0.289908257,0.291743119,0.293577982,0.295412844,0.297247706,0.299082569,
0.300917431,0.302752294,0.304587156,0.306422018,0.308256881,0.310091743,
0.311926606,0.313761468,0.31559633,0.317431193,0.319266055,0.321100917,
0.32293578,0.324770642,0.326605505,0.328440367,0.330275229,0.332110092,
0.333944954,0.335779817,0.337614679,0.339449541,0.341284404,0.343119266,
0.344954128,0.346788991,0.348623853,0.350458716,0.352293578,0.35412844,
0.355963303,0.357798165,0.359633028,0.36146789,0.363302752,0.365137615,
0.366972477,0.368807339,0.370642202,0.372477064,0.374311927,0.376146789,
0.377981651,0.379816514,0.381651376,0.383486239,0.385321101,0.387155963,
0.388990826,0.390825688,0.39266055,0.394495413,0.396330275,0.398165138,
0.4,0.401834862,0.403669725,0.405504587,0.40733945,0.409174312,0.411009174,
0.412844037,0.414678899,0.416513761,0.418348624,0.420183486,0.422018349,
0.423853211,0.425688073,0.427522936,0.429357798,0.431192661,0.433027523,
0.434862385,0.436697248,0.43853211,0.440366972,0.442201835,0.444036697,
0.44587156,0.447706422,0.449541284,0.451376147,0.453211009,0.455045872,
0.456880734,0.458715596,0.460550459,0.462385321,0.464220183,0.466055046,
0.467889908,0.469724771,0.471559633,0.473394495,0.475229358,0.47706422,
0.478899083,0.480733945,0.482568807,0.48440367,0.486238532,0.488073394,
0.489908257,0.491743119,0.493577982,0.495412844,0.497247706,0.499082569,
0.500917431,0.502752294,0.504587156,0.506422018,0.508256881,0.510091743,
0.511926606,0.513761468,0.51559633,0.517431193,0.519266055,0.521100917,
0.52293578,0.524770642,0.526605505,0.528440367,0.530275229,0.532110092,
0.533944954,0.535779817,0.537614679,0.539449541,0.541284404,0.543119266,
0.544954128,0.546788991,0.548623853,0.550458716,0.552293578,0.55412844,
0.555963303,0.557798165,0.559633028,0.56146789,0.563302752,0.565137615,
0.566972477,0.568807339,0.570642202,0.572477064,0.574311927,0.576146789,
0.577981651,0.579816514,0.581651376,0.583486239,0.585321101,0.587155963,
0.588990826,0.590825688,0.59266055,0.594495413,0.596330275,0.598165138,
0.6,0.601834862,0.603669725,0.605504587,0.60733945,0.609174312,0.611009174,
0.612844037,0.614678899,0.616513761,0.618348624,0.620183486,0.622018349,
0.623853211,0.625688073,0.627522936,0.629357798,0.631192661,0.633027523,
0.634862385,0.636697248,0.63853211,0.640366972,0.642201835,0.644036697,
0.64587156,0.647706422,0.649541284,0.651376147,0.653211009,0.655045872,
0.656880734,0.658715596,0.660550459,0.662385321,0.664220183,0.666055046,
0.667889908,0.669724771,0.671559633,0.673394495,0.675229358,0.67706422,
0.678899083,0.680733945,0.682568807,0.68440367,0.686238532,0.688073394,
0.689908257,0.691743119,0.693577982,0.695412844,0.697247706,0.699082569,
0.700917431,0.702752294,0.704587156,0.706422018,0.708256881,0.710091743,
0.711926606,0.713761468,0.71559633,0.717431193,0.719266055,0.721100917,
0.72293578,0.724770642,0.726605505,0.728440367,0.730275229,0.732110092,
0.733944954,0.735779817,0.737614679,0.739449541,0.741284404,0.743119266,
0.744954128,0.746788991,0.748623853,0.750458716,0.752293578,0.75412844,
0.755963303,0.757798165,0.759633028,0.76146789,0.763302752,0.765137615,
0.766972477,0.768807339,0.770642202,0.772477064,0.774311927,0.776146789,
0.777981651,0.779816514,0.781651376,0.783486239,0.785321101,0.787155963,
0.788990826,0.790825688,0.79266055,0.794495413,0.796330275,0.798165138,
0.8,0.801834862,0.803669725,0.805504587,0.80733945,0.809174312,0.811009174,
0.812844037,0.814678899,0.816513761,0.818348624,0.820183486,0.822018349,
0.823853211,0.825688073,0.827522936,0.829357798,0.831192661,0.833027523,
0.834862385,0.836697248,0.83853211,0.840366972,0.842201835,0.844036697,
0.84587156,0.847706422,0.849541284,0.851376147,0.853211009,0.855045872,
0.856880734,0.858715596,0.860550459,0.862385321,0.864220183,0.866055046,
0.867889908,0.869724771,0.871559633,0.873394495,0.875229358,0.87706422,
0.878899083,0.880733945,0.882568807,0.88440367,0.886238532,0.888073394,
0.889908257,0.891743119,0.893577982,0.895412844,0.897247706,0.899082569,
0.900917431,0.902752294,0.904587156,0.906422018,0.908256881,0.910091743,
0.911926606,0.913761468,0.91559633,0.917431193,0.919266055,0.921100917,
0.92293578,0.924770642,0.926605505,0.928440367,0.930275229,0.932110092,
0.933944954,0.935779817,0.937614679,0.939449541,0.941284404,0.943119266,
0.944954128,0.946788991,0.948623853,0.950458716,0.952293578,0.95412844,
0.955963303,0.957798165,0.959633028,0.96146789,0.963302752,0.965137615,
0.966972477,0.968807339,0.970642202,0.972477064,0.974311927,0.976146789,
0.977981651,0.979816514,0.981651376,0.983486239,0.985321101,0.987155963,
0.988990826,0.990825688,0.99266055,0.994495413,0.996330275,0.998165138,
1.),(0.3,1.,1.3),.UNSPECIFIED.);
#6311=B_SPLINE_SURFACE_WITH_KNOTS('',5,1,((#314665,#314666,#314667),(#314668,
#314669,#314670),(#314671,#314672,#314673),(#314674,#314675,#314676),(#314677,
#314678,#314679),(#314680,#314681,#314682),(#314683,#314684,#314685),(#314686,
#314687,#314688),(#314689,#314690,#314691),(#314692,#314693,#314694),(#314695,
#314696,#314697),(#314698,#314699,#314700),(#314701,#314702,#314703),(#314704,
#314705,#314706),(#314707,#314708,#314709),(#314710,#314711,#314712),(#314713,
#314714,#314715),(#314716,#314717,#314718),(#314719,#314720,#314721),(#314722,
#314723,#314724),(#314725,#314726,#314727),(#314728,#314729,#314730),(#314731,
#314732,#314733),(#314734,#314735,#314736),(#314737,#314738,#314739),(#314740,
#314741,#314742),(#314743,#314744,#314745),(#314746,#314747,#314748),(#314749,
#314750,#314751),(#314752,#314753,#314754),(#314755,#314756,#314757),(#314758,
#314759,#314760),(#314761,#314762,#314763),(#314764,#314765,#314766),(#314767,
#314768,#314769),(#314770,#314771,#314772),(#314773,#314774,#314775),(#314776,
#314777,#314778),(#314779,#314780,#314781),(#314782,#314783,#314784),(#314785,
#314786,#314787),(#314788,#314789,#314790),(#314791,#314792,#314793),(#314794,
#314795,#314796),(#314797,#314798,#314799),(#314800,#314801,#314802),(#314803,
#314804,#314805),(#314806,#314807,#314808),(#314809,#314810,#314811),(#314812,
#314813,#314814),(#314815,#314816,#314817),(#314818,#314819,#314820),(#314821,
#314822,#314823),(#314824,#314825,#314826),(#314827,#314828,#314829),(#314830,
#314831,#314832),(#314833,#314834,#314835),(#314836,#314837,#314838),(#314839,
#314840,#314841),(#314842,#314843,#314844),(#314845,#314846,#314847),(#314848,
#314849,#314850),(#314851,#314852,#314853),(#314854,#314855,#314856),(#314857,
#314858,#314859),(#314860,#314861,#314862),(#314863,#314864,#314865),(#314866,
#314867,#314868),(#314869,#314870,#314871),(#314872,#314873,#314874),(#314875,
#314876,#314877),(#314878,#314879,#314880),(#314881,#314882,#314883),(#314884,
#314885,#314886),(#314887,#314888,#314889),(#314890,#314891,#314892),(#314893,
#314894,#314895),(#314896,#314897,#314898),(#314899,#314900,#314901),(#314902,
#314903,#314904),(#314905,#314906,#314907),(#314908,#314909,#314910),(#314911,
#314912,#314913),(#314914,#314915,#314916),(#314917,#314918,#314919),(#314920,
#314921,#314922),(#314923,#314924,#314925),(#314926,#314927,#314928),(#314929,
#314930,#314931),(#314932,#314933,#314934),(#314935,#314936,#314937),(#314938,
#314939,#314940),(#314941,#314942,#314943),(#314944,#314945,#314946),(#314947,
#314948,#314949),(#314950,#314951,#314952),(#314953,#314954,#314955),(#314956,
#314957,#314958),(#314959,#314960,#314961),(#314962,#314963,#314964),(#314965,
#314966,#314967),(#314968,#314969,#314970),(#314971,#314972,#314973),(#314974,
#314975,#314976),(#314977,#314978,#314979),(#314980,#314981,#314982),(#314983,
#314984,#314985),(#314986,#314987,#314988),(#314989,#314990,#314991),(#314992,
#314993,#314994),(#314995,#314996,#314997),(#314998,#314999,#315000),(#315001,
#315002,#315003),(#315004,#315005,#315006),(#315007,#315008,#315009),(#315010,
#315011,#315012),(#315013,#315014,#315015),(#315016,#315017,#315018),(#315019,
#315020,#315021),(#315022,#315023,#315024),(#315025,#315026,#315027),(#315028,
#315029,#315030),(#315031,#315032,#315033),(#315034,#315035,#315036),(#315037,
#315038,#315039),(#315040,#315041,#315042),(#315043,#315044,#315045),(#315046,
#315047,#315048),(#315049,#315050,#315051),(#315052,#315053,#315054),(#315055,
#315056,#315057),(#315058,#315059,#315060),(#315061,#315062,#315063),(#315064,
#315065,#315066),(#315067,#315068,#315069),(#315070,#315071,#315072),(#315073,
#315074,#315075),(#315076,#315077,#315078),(#315079,#315080,#315081),(#315082,
#315083,#315084),(#315085,#315086,#315087),(#315088,#315089,#315090),(#315091,
#315092,#315093),(#315094,#315095,#315096),(#315097,#315098,#315099),(#315100,
#315101,#315102),(#315103,#315104,#315105),(#315106,#315107,#315108),(#315109,
#315110,#315111),(#315112,#315113,#315114),(#315115,#315116,#315117),(#315118,
#315119,#315120),(#315121,#315122,#315123),(#315124,#315125,#315126),(#315127,
#315128,#315129),(#315130,#315131,#315132),(#315133,#315134,#315135),(#315136,
#315137,#315138),(#315139,#315140,#315141),(#315142,#315143,#315144),(#315145,
#315146,#315147),(#315148,#315149,#315150),(#315151,#315152,#315153),(#315154,
#315155,#315156),(#315157,#315158,#315159),(#315160,#315161,#315162),(#315163,
#315164,#315165),(#315166,#315167,#315168),(#315169,#315170,#315171),(#315172,
#315173,#315174),(#315175,#315176,#315177),(#315178,#315179,#315180),(#315181,
#315182,#315183),(#315184,#315185,#315186),(#315187,#315188,#315189),(#315190,
#315191,#315192),(#315193,#315194,#315195),(#315196,#315197,#315198),(#315199,
#315200,#315201),(#315202,#315203,#315204),(#315205,#315206,#315207),(#315208,
#315209,#315210),(#315211,#315212,#315213),(#315214,#315215,#315216),(#315217,
#315218,#315219),(#315220,#315221,#315222),(#315223,#315224,#315225),(#315226,
#315227,#315228),(#315229,#315230,#315231),(#315232,#315233,#315234),(#315235,
#315236,#315237),(#315238,#315239,#315240),(#315241,#315242,#315243),(#315244,
#315245,#315246),(#315247,#315248,#315249),(#315250,#315251,#315252),(#315253,
#315254,#315255),(#315256,#315257,#315258),(#315259,#315260,#315261),(#315262,
#315263,#315264),(#315265,#315266,#315267),(#315268,#315269,#315270),(#315271,
#315272,#315273),(#315274,#315275,#315276),(#315277,#315278,#315279),(#315280,
#315281,#315282),(#315283,#315284,#315285),(#315286,#315287,#315288),(#315289,
#315290,#315291),(#315292,#315293,#315294),(#315295,#315296,#315297),(#315298,
#315299,#315300),(#315301,#315302,#315303),(#315304,#315305,#315306),(#315307,
#315308,#315309),(#315310,#315311,#315312),(#315313,#315314,#315315),(#315316,
#315317,#315318),(#315319,#315320,#315321),(#315322,#315323,#315324),(#315325,
#315326,#315327),(#315328,#315329,#315330),(#315331,#315332,#315333),(#315334,
#315335,#315336),(#315337,#315338,#315339),(#315340,#315341,#315342),(#315343,
#315344,#315345),(#315346,#315347,#315348),(#315349,#315350,#315351),(#315352,
#315353,#315354),(#315355,#315356,#315357),(#315358,#315359,#315360),(#315361,
#315362,#315363),(#315364,#315365,#315366),(#315367,#315368,#315369),(#315370,
#315371,#315372),(#315373,#315374,#315375),(#315376,#315377,#315378),(#315379,
#315380,#315381),(#315382,#315383,#315384),(#315385,#315386,#315387),(#315388,
#315389,#315390),(#315391,#315392,#315393),(#315394,#315395,#315396),(#315397,
#315398,#315399),(#315400,#315401,#315402),(#315403,#315404,#315405),(#315406,
#315407,#315408),(#315409,#315410,#315411),(#315412,#315413,#315414),(#315415,
#315416,#315417),(#315418,#315419,#315420),(#315421,#315422,#315423),(#315424,
#315425,#315426),(#315427,#315428,#315429),(#315430,#315431,#315432),(#315433,
#315434,#315435),(#315436,#315437,#315438),(#315439,#315440,#315441),(#315442,
#315443,#315444),(#315445,#315446,#315447),(#315448,#315449,#315450),(#315451,
#315452,#315453),(#315454,#315455,#315456),(#315457,#315458,#315459),(#315460,
#315461,#315462),(#315463,#315464,#315465),(#315466,#315467,#315468),(#315469,
#315470,#315471),(#315472,#315473,#315474),(#315475,#315476,#315477),(#315478,
#315479,#315480),(#315481,#315482,#315483),(#315484,#315485,#315486),(#315487,
#315488,#315489),(#315490,#315491,#315492),(#315493,#315494,#315495),(#315496,
#315497,#315498),(#315499,#315500,#315501),(#315502,#315503,#315504),(#315505,
#315506,#315507),(#315508,#315509,#315510),(#315511,#315512,#315513),(#315514,
#315515,#315516),(#315517,#315518,#315519),(#315520,#315521,#315522),(#315523,
#315524,#315525),(#315526,#315527,#315528),(#315529,#315530,#315531),(#315532,
#315533,#315534),(#315535,#315536,#315537),(#315538,#315539,#315540),(#315541,
#315542,#315543),(#315544,#315545,#315546),(#315547,#315548,#315549),(#315550,
#315551,#315552),(#315553,#315554,#315555),(#315556,#315557,#315558),(#315559,
#315560,#315561),(#315562,#315563,#315564),(#315565,#315566,#315567),(#315568,
#315569,#315570),(#315571,#315572,#315573),(#315574,#315575,#315576),(#315577,
#315578,#315579),(#315580,#315581,#315582),(#315583,#315584,#315585),(#315586,
#315587,#315588),(#315589,#315590,#315591),(#315592,#315593,#315594),(#315595,
#315596,#315597),(#315598,#315599,#315600),(#315601,#315602,#315603),(#315604,
#315605,#315606),(#315607,#315608,#315609),(#315610,#315611,#315612),(#315613,
#315614,#315615),(#315616,#315617,#315618),(#315619,#315620,#315621),(#315622,
#315623,#315624),(#315625,#315626,#315627),(#315628,#315629,#315630),(#315631,
#315632,#315633),(#315634,#315635,#315636),(#315637,#315638,#315639),(#315640,
#315641,#315642),(#315643,#315644,#315645),(#315646,#315647,#315648),(#315649,
#315650,#315651),(#315652,#315653,#315654),(#315655,#315656,#315657),(#315658,
#315659,#315660),(#315661,#315662,#315663),(#315664,#315665,#315666),(#315667,
#315668,#315669),(#315670,#315671,#315672),(#315673,#315674,#315675),(#315676,
#315677,#315678),(#315679,#315680,#315681),(#315682,#315683,#315684),(#315685,
#315686,#315687),(#315688,#315689,#315690),(#315691,#315692,#315693),(#315694,
#315695,#315696),(#315697,#315698,#315699),(#315700,#315701,#315702),(#315703,
#315704,#315705),(#315706,#315707,#315708),(#315709,#315710,#315711),(#315712,
#315713,#315714),(#315715,#315716,#315717),(#315718,#315719,#315720),(#315721,
#315722,#315723),(#315724,#315725,#315726),(#315727,#315728,#315729),(#315730,
#315731,#315732),(#315733,#315734,#315735),(#315736,#315737,#315738),(#315739,
#315740,#315741),(#315742,#315743,#315744),(#315745,#315746,#315747),(#315748,
#315749,#315750),(#315751,#315752,#315753),(#315754,#315755,#315756),(#315757,
#315758,#315759),(#315760,#315761,#315762),(#315763,#315764,#315765),(#315766,
#315767,#315768),(#315769,#315770,#315771),(#315772,#315773,#315774),(#315775,
#315776,#315777),(#315778,#315779,#315780),(#315781,#315782,#315783),(#315784,
#315785,#315786),(#315787,#315788,#315789),(#315790,#315791,#315792),(#315793,
#315794,#315795),(#315796,#315797,#315798),(#315799,#315800,#315801),(#315802,
#315803,#315804),(#315805,#315806,#315807),(#315808,#315809,#315810),(#315811,
#315812,#315813),(#315814,#315815,#315816),(#315817,#315818,#315819),(#315820,
#315821,#315822),(#315823,#315824,#315825),(#315826,#315827,#315828),(#315829,
#315830,#315831),(#315832,#315833,#315834),(#315835,#315836,#315837),(#315838,
#315839,#315840),(#315841,#315842,#315843),(#315844,#315845,#315846),(#315847,
#315848,#315849),(#315850,#315851,#315852),(#315853,#315854,#315855),(#315856,
#315857,#315858),(#315859,#315860,#315861),(#315862,#315863,#315864),(#315865,
#315866,#315867),(#315868,#315869,#315870),(#315871,#315872,#315873),(#315874,
#315875,#315876),(#315877,#315878,#315879),(#315880,#315881,#315882),(#315883,
#315884,#315885),(#315886,#315887,#315888),(#315889,#315890,#315891),(#315892,
#315893,#315894),(#315895,#315896,#315897),(#315898,#315899,#315900),(#315901,
#315902,#315903),(#315904,#315905,#315906),(#315907,#315908,#315909),(#315910,
#315911,#315912),(#315913,#315914,#315915),(#315916,#315917,#315918),(#315919,
#315920,#315921),(#315922,#315923,#315924),(#315925,#315926,#315927),(#315928,
#315929,#315930),(#315931,#315932,#315933),(#315934,#315935,#315936),(#315937,
#315938,#315939),(#315940,#315941,#315942),(#315943,#315944,#315945),(#315946,
#315947,#315948),(#315949,#315950,#315951),(#315952,#315953,#315954),(#315955,
#315956,#315957),(#315958,#315959,#315960),(#315961,#315962,#315963),(#315964,
#315965,#315966),(#315967,#315968,#315969),(#315970,#315971,#315972),(#315973,
#315974,#315975),(#315976,#315977,#315978),(#315979,#315980,#315981),(#315982,
#315983,#315984),(#315985,#315986,#315987),(#315988,#315989,#315990),(#315991,
#315992,#315993),(#315994,#315995,#315996),(#315997,#315998,#315999),(#316000,
#316001,#316002),(#316003,#316004,#316005),(#316006,#316007,#316008),(#316009,
#316010,#316011),(#316012,#316013,#316014),(#316015,#316016,#316017),(#316018,
#316019,#316020),(#316021,#316022,#316023),(#316024,#316025,#316026),(#316027,
#316028,#316029),(#316030,#316031,#316032),(#316033,#316034,#316035),(#316036,
#316037,#316038),(#316039,#316040,#316041),(#316042,#316043,#316044),(#316045,
#316046,#316047),(#316048,#316049,#316050),(#316051,#316052,#316053),(#316054,
#316055,#316056),(#316057,#316058,#316059),(#316060,#316061,#316062),(#316063,
#316064,#316065),(#316066,#316067,#316068),(#316069,#316070,#316071),(#316072,
#316073,#316074),(#316075,#316076,#316077),(#316078,#316079,#316080),(#316081,
#316082,#316083),(#316084,#316085,#316086),(#316087,#316088,#316089),(#316090,
#316091,#316092),(#316093,#316094,#316095),(#316096,#316097,#316098),(#316099,
#316100,#316101),(#316102,#316103,#316104),(#316105,#316106,#316107),(#316108,
#316109,#316110),(#316111,#316112,#316113),(#316114,#316115,#316116),(#316117,
#316118,#316119),(#316120,#316121,#316122),(#316123,#316124,#316125),(#316126,
#316127,#316128),(#316129,#316130,#316131),(#316132,#316133,#316134),(#316135,
#316136,#316137),(#316138,#316139,#316140),(#316141,#316142,#316143),(#316144,
#316145,#316146),(#316147,#316148,#316149),(#316150,#316151,#316152),(#316153,
#316154,#316155),(#316156,#316157,#316158),(#316159,#316160,#316161),(#316162,
#316163,#316164),(#316165,#316166,#316167),(#316168,#316169,#316170),(#316171,
#316172,#316173),(#316174,#316175,#316176),(#316177,#316178,#316179),(#316180,
#316181,#316182),(#316183,#316184,#316185),(#316186,#316187,#316188),(#316189,
#316190,#316191),(#316192,#316193,#316194),(#316195,#316196,#316197),(#316198,
#316199,#316200),(#316201,#316202,#316203),(#316204,#316205,#316206),(#316207,
#316208,#316209),(#316210,#316211,#316212),(#316213,#316214,#316215),(#316216,
#316217,#316218),(#316219,#316220,#316221),(#316222,#316223,#316224),(#316225,
#316226,#316227),(#316228,#316229,#316230),(#316231,#316232,#316233),(#316234,
#316235,#316236),(#316237,#316238,#316239),(#316240,#316241,#316242),(#316243,
#316244,#316245),(#316246,#316247,#316248),(#316249,#316250,#316251),(#316252,
#316253,#316254),(#316255,#316256,#316257),(#316258,#316259,#316260),(#316261,
#316262,#316263),(#316264,#316265,#316266),(#316267,#316268,#316269),(#316270,
#316271,#316272),(#316273,#316274,#316275),(#316276,#316277,#316278),(#316279,
#316280,#316281),(#316282,#316283,#316284),(#316285,#316286,#316287),(#316288,
#316289,#316290),(#316291,#316292,#316293),(#316294,#316295,#316296),(#316297,
#316298,#316299),(#316300,#316301,#316302),(#316303,#316304,#316305),(#316306,
#316307,#316308),(#316309,#316310,#316311),(#316312,#316313,#316314)),
 .UNSPECIFIED.,.F.,.F.,.F.,(6,1,1,1,1,1,1,1,1,1,1,1,1,1,1,1,1,1,1,1,1,1,
1,1,1,1,1,1,1,1,1,1,1,1,1,1,1,1,1,1,1,1,1,1,1,1,1,1,1,1,1,1,1,1,1,1,1,1,
1,1,1,1,1,1,1,1,1,1,1,1,1,1,1,1,1,1,1,1,1,1,1,1,1,1,1,1,1,1,1,1,1,1,1,1,
1,1,1,1,1,1,1,1,1,1,1,1,1,1,1,1,1,1,1,1,1,1,1,1,1,1,1,1,1,1,1,1,1,1,1,1,
1,1,1,1,1,1,1,1,1,1,1,1,1,1,1,1,1,1,1,1,1,1,1,1,1,1,1,1,1,1,1,1,1,1,1,1,
1,1,1,1,1,1,1,1,1,1,1,1,1,1,1,1,1,1,1,1,1,1,1,1,1,1,1,1,1,1,1,1,1,1,1,1,
1,1,1,1,1,1,1,1,1,1,1,1,1,1,1,1,1,1,1,1,1,1,1,1,1,1,1,1,1,1,1,1,1,1,1,1,
1,1,1,1,1,1,1,1,1,1,1,1,1,1,1,1,1,1,1,1,1,1,1,1,1,1,1,1,1,1,1,1,1,1,1,1,
1,1,1,1,1,1,1,1,1,1,1,1,1,1,1,1,1,1,1,1,1,1,1,1,1,1,1,1,1,1,1,1,1,1,1,1,
1,1,1,1,1,1,1,1,1,1,1,1,1,1,1,1,1,1,1,1,1,1,1,1,1,1,1,1,1,1,1,1,1,1,1,1,
1,1,1,1,1,1,1,1,1,1,1,1,1,1,1,1,1,1,1,1,1,1,1,1,1,1,1,1,1,1,1,1,1,1,1,1,
1,1,1,1,1,1,1,1,1,1,1,1,1,1,1,1,1,1,1,1,1,1,1,1,1,1,1,1,1,1,1,1,1,1,1,1,
1,1,1,1,1,1,1,1,1,1,1,1,1,1,1,1,1,1,1,1,1,1,1,1,1,1,1,1,1,1,1,1,1,1,1,1,
1,1,1,1,1,1,1,1,1,1,1,1,1,1,1,1,1,1,1,1,1,1,1,1,1,1,1,1,1,1,1,1,1,1,1,1,
1,1,1,1,1,1,1,1,1,1,1,1,1,1,1,1,1,1,1,1,1,1,1,1,1,1,1,1,1,1,1,1,1,1,1,1,
1,1,1,1,1,1,1,1,1,1,1,1,1,1,1,1,1,1,1,6),(2,1,2),(-1.,-0.998165138,-0.996330275,
-0.994495413,-0.99266055,-0.990825688,-0.988990826,-0.987155963,-0.985321101,
-0.983486239,-0.981651376,-0.979816514,-0.977981651,-0.976146789,-0.974311927,
-0.972477064,-0.970642202,-0.968807339,-0.966972477,-0.965137615,-0.963302752,
-0.96146789,-0.959633028,-0.957798165,-0.955963303,-0.95412844,-0.952293578,
-0.950458716,-0.948623853,-0.946788991,-0.944954128,-0.943119266,-0.941284404,
-0.939449541,-0.937614679,-0.935779817,-0.933944954,-0.932110092,-0.930275229,
-0.928440367,-0.926605505,-0.924770642,-0.92293578,-0.921100917,-0.919266055,
-0.917431193,-0.91559633,-0.913761468,-0.911926606,-0.910091743,-0.908256881,
-0.906422018,-0.904587156,-0.902752294,-0.900917431,-0.899082569,-0.897247706,
-0.895412844,-0.893577982,-0.891743119,-0.889908257,-0.888073394,-0.886238532,
-0.88440367,-0.882568807,-0.880733945,-0.878899083,-0.87706422,-0.875229358,
-0.873394495,-0.871559633,-0.869724771,-0.867889908,-0.866055046,-0.864220183,
-0.862385321,-0.860550459,-0.858715596,-0.856880734,-0.855045872,-0.853211009,
-0.851376147,-0.849541284,-0.847706422,-0.84587156,-0.844036697,-0.842201835,
-0.840366972,-0.83853211,-0.836697248,-0.834862385,-0.833027523,-0.831192661,
-0.829357798,-0.827522936,-0.825688073,-0.823853211,-0.822018349,-0.820183486,
-0.818348624,-0.816513761,-0.814678899,-0.812844037,-0.811009174,-0.809174312,
-0.80733945,-0.805504587,-0.803669725,-0.801834862,-0.8,-0.798165138,-0.796330275,
-0.794495413,-0.79266055,-0.790825688,-0.788990826,-0.787155963,-0.785321101,
-0.783486239,-0.781651376,-0.779816514,-0.777981651,-0.776146789,-0.774311927,
-0.772477064,-0.770642202,-0.768807339,-0.766972477,-0.765137615,-0.763302752,
-0.76146789,-0.759633028,-0.757798165,-0.755963303,-0.75412844,-0.752293578,
-0.750458716,-0.748623853,-0.746788991,-0.744954128,-0.743119266,-0.741284404,
-0.739449541,-0.737614679,-0.735779817,-0.733944954,-0.732110092,-0.730275229,
-0.728440367,-0.726605505,-0.724770642,-0.72293578,-0.721100917,-0.719266055,
-0.717431193,-0.71559633,-0.713761468,-0.711926606,-0.710091743,-0.708256881,
-0.706422018,-0.704587156,-0.702752294,-0.700917431,-0.699082569,-0.697247706,
-0.695412844,-0.693577982,-0.691743119,-0.689908257,-0.688073394,-0.686238532,
-0.68440367,-0.682568807,-0.680733945,-0.678899083,-0.67706422,-0.675229358,
-0.673394495,-0.671559633,-0.669724771,-0.667889908,-0.666055046,-0.664220183,
-0.662385321,-0.660550459,-0.658715596,-0.656880734,-0.655045872,-0.653211009,
-0.651376147,-0.649541284,-0.647706422,-0.64587156,-0.644036697,-0.642201835,
-0.640366972,-0.63853211,-0.636697248,-0.634862385,-0.633027523,-0.631192661,
-0.629357798,-0.627522936,-0.625688073,-0.623853211,-0.622018349,-0.620183486,
-0.618348624,-0.616513761,-0.614678899,-0.612844037,-0.611009174,-0.609174312,
-0.60733945,-0.605504587,-0.603669725,-0.601834862,-0.6,-0.598165138,-0.596330275,
-0.594495413,-0.59266055,-0.590825688,-0.588990826,-0.587155963,-0.585321101,
-0.583486239,-0.581651376,-0.579816514,-0.577981651,-0.576146789,-0.574311927,
-0.572477064,-0.570642202,-0.568807339,-0.566972477,-0.565137615,-0.563302752,
-0.56146789,-0.559633028,-0.557798165,-0.555963303,-0.55412844,-0.552293578,
-0.550458716,-0.548623853,-0.546788991,-0.544954128,-0.543119266,-0.541284404,
-0.539449541,-0.537614679,-0.535779817,-0.533944954,-0.532110092,-0.530275229,
-0.528440367,-0.526605505,-0.524770642,-0.52293578,-0.521100917,-0.519266055,
-0.517431193,-0.51559633,-0.513761468,-0.511926606,-0.510091743,-0.508256881,
-0.506422018,-0.504587156,-0.502752294,-0.500917431,-0.499082569,-0.497247706,
-0.495412844,-0.493577982,-0.491743119,-0.489908257,-0.488073394,-0.486238532,
-0.48440367,-0.482568807,-0.480733945,-0.478899083,-0.47706422,-0.475229358,
-0.473394495,-0.471559633,-0.469724771,-0.467889908,-0.466055046,-0.464220183,
-0.462385321,-0.460550459,-0.458715596,-0.456880734,-0.455045872,-0.453211009,
-0.451376147,-0.449541284,-0.447706422,-0.44587156,-0.444036697,-0.442201835,
-0.440366972,-0.43853211,-0.436697248,-0.434862385,-0.433027523,-0.431192661,
-0.429357798,-0.427522936,-0.425688073,-0.423853211,-0.422018349,-0.420183486,
-0.418348624,-0.416513761,-0.414678899,-0.412844037,-0.411009174,-0.409174312,
-0.40733945,-0.405504587,-0.403669725,-0.401834862,-0.4,-0.398165138,-0.396330275,
-0.394495413,-0.39266055,-0.390825688,-0.388990826,-0.387155963,-0.385321101,
-0.383486239,-0.381651376,-0.379816514,-0.377981651,-0.376146789,-0.374311927,
-0.372477064,-0.370642202,-0.368807339,-0.366972477,-0.365137615,-0.363302752,
-0.36146789,-0.359633028,-0.357798165,-0.355963303,-0.35412844,-0.352293578,
-0.350458716,-0.348623853,-0.346788991,-0.344954128,-0.343119266,-0.341284404,
-0.339449541,-0.337614679,-0.335779817,-0.333944954,-0.332110092,-0.330275229,
-0.328440367,-0.326605505,-0.324770642,-0.32293578,-0.321100917,-0.319266055,
-0.317431193,-0.31559633,-0.313761468,-0.311926606,-0.310091743,-0.308256881,
-0.306422018,-0.304587156,-0.302752294,-0.300917431,-0.299082569,-0.297247706,
-0.295412844,-0.293577982,-0.291743119,-0.289908257,-0.288073394,-0.286238532,
-0.28440367,-0.282568807,-0.280733945,-0.278899083,-0.27706422,-0.275229358,
-0.273394495,-0.271559633,-0.269724771,-0.267889908,-0.266055046,-0.264220183,
-0.262385321,-0.260550459,-0.258715596,-0.256880734,-0.255045872,-0.253211009,
-0.251376147,-0.249541284,-0.247706422,-0.24587156,-0.244036697,-0.242201835,
-0.240366972,-0.23853211,-0.236697248,-0.234862385,-0.233027523,-0.231192661,
-0.229357798,-0.227522936,-0.225688073,-0.223853211,-0.222018349,-0.220183486,
-0.218348624,-0.216513761,-0.214678899,-0.212844037,-0.211009174,-0.209174312,
-0.20733945,-0.205504587,-0.203669725,-0.201834862,-0.2,-0.198165138,-0.196330275,
-0.194495413,-0.19266055,-0.190825688,-0.188990826,-0.187155963,-0.185321101,
-0.183486239,-0.181651376,-0.179816514,-0.177981651,-0.176146789,-0.174311927,
-0.172477064,-0.170642202,-0.168807339,-0.166972477,-0.165137615,-0.163302752,
-0.16146789,-0.159633028,-0.157798165,-0.155963303,-0.15412844,-0.152293578,
-0.150458716,-0.148623853,-0.146788991,-0.144954128,-0.143119266,-0.141284404,
-0.139449541,-0.137614679,-0.135779817,-0.133944954,-0.132110092,-0.130275229,
-0.128440367,-0.126605505,-0.124770642,-0.12293578,-0.121100917,-0.119266055,
-0.117431193,-0.11559633,-0.113761468,-0.111926606,-0.110091743,-0.108256881,
-0.106422018,-0.104587156,-0.102752294,-0.100917431,-0.099082569,-0.097247706,
-0.095412844,-0.093577982,-0.091743119,-0.089908257,-0.088073394,-0.086238532,
-0.08440367,-0.082568807,-0.080733945,-0.078899083,-0.07706422,-0.075229358,
-0.073394495,-0.071559633,-0.069724771,-0.067889908,-0.066055046,-0.064220183,
-0.062385321,-0.060550459,-0.058715596,-0.056880734,-0.055045872,-0.053211009,
-0.051376147,-0.049541284,-0.047706422,-0.04587156,-0.044036697,-0.042201835,
-0.040366972,-0.03853211,-0.036697248,-0.034862385,-0.033027523,-0.031192661,
-0.029357798,-0.027522936,-0.025688073,-0.023853211,-0.022018349,-0.020183486,
-0.018348624,-0.016513761,-0.014678899,-0.012844037,-0.011009174,-0.009174312,
-0.00733945,-0.005504587,-0.003669725,-0.001834862,0.000982124),(0.3,1.,
1.3),.UNSPECIFIED.);
#6312=B_SPLINE_SURFACE_WITH_KNOTS('',5,1,((#316337,#316338,#316339),(#316340,
#316341,#316342),(#316343,#316344,#316345),(#316346,#316347,#316348),(#316349,
#316350,#316351),(#316352,#316353,#316354),(#316355,#316356,#316357),(#316358,
#316359,#316360),(#316361,#316362,#316363),(#316364,#316365,#316366),(#316367,
#316368,#316369),(#316370,#316371,#316372),(#316373,#316374,#316375),(#316376,
#316377,#316378),(#316379,#316380,#316381),(#316382,#316383,#316384),(#316385,
#316386,#316387),(#316388,#316389,#316390),(#316391,#316392,#316393),(#316394,
#316395,#316396),(#316397,#316398,#316399),(#316400,#316401,#316402),(#316403,
#316404,#316405),(#316406,#316407,#316408),(#316409,#316410,#316411),(#316412,
#316413,#316414),(#316415,#316416,#316417),(#316418,#316419,#316420),(#316421,
#316422,#316423),(#316424,#316425,#316426),(#316427,#316428,#316429),(#316430,
#316431,#316432),(#316433,#316434,#316435),(#316436,#316437,#316438),(#316439,
#316440,#316441),(#316442,#316443,#316444),(#316445,#316446,#316447),(#316448,
#316449,#316450),(#316451,#316452,#316453),(#316454,#316455,#316456),(#316457,
#316458,#316459),(#316460,#316461,#316462),(#316463,#316464,#316465),(#316466,
#316467,#316468),(#316469,#316470,#316471),(#316472,#316473,#316474),(#316475,
#316476,#316477),(#316478,#316479,#316480),(#316481,#316482,#316483),(#316484,
#316485,#316486),(#316487,#316488,#316489),(#316490,#316491,#316492),(#316493,
#316494,#316495),(#316496,#316497,#316498),(#316499,#316500,#316501),(#316502,
#316503,#316504),(#316505,#316506,#316507),(#316508,#316509,#316510),(#316511,
#316512,#316513),(#316514,#316515,#316516),(#316517,#316518,#316519),(#316520,
#316521,#316522),(#316523,#316524,#316525),(#316526,#316527,#316528),(#316529,
#316530,#316531),(#316532,#316533,#316534),(#316535,#316536,#316537),(#316538,
#316539,#316540),(#316541,#316542,#316543),(#316544,#316545,#316546),(#316547,
#316548,#316549),(#316550,#316551,#316552),(#316553,#316554,#316555),(#316556,
#316557,#316558),(#316559,#316560,#316561),(#316562,#316563,#316564),(#316565,
#316566,#316567),(#316568,#316569,#316570),(#316571,#316572,#316573),(#316574,
#316575,#316576),(#316577,#316578,#316579),(#316580,#316581,#316582),(#316583,
#316584,#316585),(#316586,#316587,#316588),(#316589,#316590,#316591),(#316592,
#316593,#316594),(#316595,#316596,#316597),(#316598,#316599,#316600),(#316601,
#316602,#316603),(#316604,#316605,#316606),(#316607,#316608,#316609),(#316610,
#316611,#316612),(#316613,#316614,#316615),(#316616,#316617,#316618),(#316619,
#316620,#316621),(#316622,#316623,#316624),(#316625,#316626,#316627),(#316628,
#316629,#316630),(#316631,#316632,#316633),(#316634,#316635,#316636),(#316637,
#316638,#316639),(#316640,#316641,#316642),(#316643,#316644,#316645),(#316646,
#316647,#316648),(#316649,#316650,#316651),(#316652,#316653,#316654),(#316655,
#316656,#316657),(#316658,#316659,#316660),(#316661,#316662,#316663),(#316664,
#316665,#316666),(#316667,#316668,#316669),(#316670,#316671,#316672),(#316673,
#316674,#316675),(#316676,#316677,#316678),(#316679,#316680,#316681),(#316682,
#316683,#316684),(#316685,#316686,#316687),(#316688,#316689,#316690),(#316691,
#316692,#316693),(#316694,#316695,#316696),(#316697,#316698,#316699),(#316700,
#316701,#316702),(#316703,#316704,#316705),(#316706,#316707,#316708),(#316709,
#316710,#316711),(#316712,#316713,#316714),(#316715,#316716,#316717),(#316718,
#316719,#316720),(#316721,#316722,#316723),(#316724,#316725,#316726),(#316727,
#316728,#316729),(#316730,#316731,#316732),(#316733,#316734,#316735),(#316736,
#316737,#316738),(#316739,#316740,#316741),(#316742,#316743,#316744),(#316745,
#316746,#316747),(#316748,#316749,#316750),(#316751,#316752,#316753),(#316754,
#316755,#316756),(#316757,#316758,#316759),(#316760,#316761,#316762),(#316763,
#316764,#316765),(#316766,#316767,#316768),(#316769,#316770,#316771),(#316772,
#316773,#316774),(#316775,#316776,#316777),(#316778,#316779,#316780),(#316781,
#316782,#316783),(#316784,#316785,#316786),(#316787,#316788,#316789),(#316790,
#316791,#316792),(#316793,#316794,#316795),(#316796,#316797,#316798),(#316799,
#316800,#316801),(#316802,#316803,#316804),(#316805,#316806,#316807),(#316808,
#316809,#316810),(#316811,#316812,#316813),(#316814,#316815,#316816),(#316817,
#316818,#316819),(#316820,#316821,#316822),(#316823,#316824,#316825),(#316826,
#316827,#316828),(#316829,#316830,#316831),(#316832,#316833,#316834),(#316835,
#316836,#316837),(#316838,#316839,#316840),(#316841,#316842,#316843),(#316844,
#316845,#316846),(#316847,#316848,#316849),(#316850,#316851,#316852),(#316853,
#316854,#316855),(#316856,#316857,#316858),(#316859,#316860,#316861),(#316862,
#316863,#316864),(#316865,#316866,#316867),(#316868,#316869,#316870),(#316871,
#316872,#316873),(#316874,#316875,#316876),(#316877,#316878,#316879),(#316880,
#316881,#316882),(#316883,#316884,#316885),(#316886,#316887,#316888),(#316889,
#316890,#316891),(#316892,#316893,#316894),(#316895,#316896,#316897),(#316898,
#316899,#316900),(#316901,#316902,#316903),(#316904,#316905,#316906),(#316907,
#316908,#316909),(#316910,#316911,#316912),(#316913,#316914,#316915),(#316916,
#316917,#316918),(#316919,#316920,#316921),(#316922,#316923,#316924),(#316925,
#316926,#316927),(#316928,#316929,#316930),(#316931,#316932,#316933),(#316934,
#316935,#316936),(#316937,#316938,#316939),(#316940,#316941,#316942),(#316943,
#316944,#316945),(#316946,#316947,#316948),(#316949,#316950,#316951),(#316952,
#316953,#316954),(#316955,#316956,#316957),(#316958,#316959,#316960),(#316961,
#316962,#316963),(#316964,#316965,#316966),(#316967,#316968,#316969),(#316970,
#316971,#316972),(#316973,#316974,#316975),(#316976,#316977,#316978),(#316979,
#316980,#316981),(#316982,#316983,#316984),(#316985,#316986,#316987),(#316988,
#316989,#316990),(#316991,#316992,#316993),(#316994,#316995,#316996),(#316997,
#316998,#316999),(#317000,#317001,#317002),(#317003,#317004,#317005),(#317006,
#317007,#317008),(#317009,#317010,#317011),(#317012,#317013,#317014),(#317015,
#317016,#317017),(#317018,#317019,#317020),(#317021,#317022,#317023),(#317024,
#317025,#317026),(#317027,#317028,#317029),(#317030,#317031,#317032),(#317033,
#317034,#317035),(#317036,#317037,#317038),(#317039,#317040,#317041),(#317042,
#317043,#317044),(#317045,#317046,#317047),(#317048,#317049,#317050),(#317051,
#317052,#317053),(#317054,#317055,#317056),(#317057,#317058,#317059),(#317060,
#317061,#317062),(#317063,#317064,#317065),(#317066,#317067,#317068),(#317069,
#317070,#317071),(#317072,#317073,#317074),(#317075,#317076,#317077),(#317078,
#317079,#317080),(#317081,#317082,#317083),(#317084,#317085,#317086),(#317087,
#317088,#317089),(#317090,#317091,#317092),(#317093,#317094,#317095),(#317096,
#317097,#317098),(#317099,#317100,#317101),(#317102,#317103,#317104),(#317105,
#317106,#317107),(#317108,#317109,#317110),(#317111,#317112,#317113),(#317114,
#317115,#317116),(#317117,#317118,#317119),(#317120,#317121,#317122),(#317123,
#317124,#317125),(#317126,#317127,#317128),(#317129,#317130,#317131),(#317132,
#317133,#317134),(#317135,#317136,#317137),(#317138,#317139,#317140),(#317141,
#317142,#317143),(#317144,#317145,#317146),(#317147,#317148,#317149),(#317150,
#317151,#317152),(#317153,#317154,#317155),(#317156,#317157,#317158),(#317159,
#317160,#317161),(#317162,#317163,#317164),(#317165,#317166,#317167),(#317168,
#317169,#317170),(#317171,#317172,#317173),(#317174,#317175,#317176),(#317177,
#317178,#317179),(#317180,#317181,#317182),(#317183,#317184,#317185),(#317186,
#317187,#317188),(#317189,#317190,#317191),(#317192,#317193,#317194),(#317195,
#317196,#317197),(#317198,#317199,#317200),(#317201,#317202,#317203),(#317204,
#317205,#317206),(#317207,#317208,#317209),(#317210,#317211,#317212),(#317213,
#317214,#317215),(#317216,#317217,#317218),(#317219,#317220,#317221),(#317222,
#317223,#317224),(#317225,#317226,#317227),(#317228,#317229,#317230),(#317231,
#317232,#317233),(#317234,#317235,#317236),(#317237,#317238,#317239),(#317240,
#317241,#317242),(#317243,#317244,#317245),(#317246,#317247,#317248),(#317249,
#317250,#317251),(#317252,#317253,#317254),(#317255,#317256,#317257),(#317258,
#317259,#317260),(#317261,#317262,#317263),(#317264,#317265,#317266),(#317267,
#317268,#317269),(#317270,#317271,#317272),(#317273,#317274,#317275),(#317276,
#317277,#317278),(#317279,#317280,#317281),(#317282,#317283,#317284),(#317285,
#317286,#317287),(#317288,#317289,#317290),(#317291,#317292,#317293),(#317294,
#317295,#317296),(#317297,#317298,#317299),(#317300,#317301,#317302),(#317303,
#317304,#317305),(#317306,#317307,#317308),(#317309,#317310,#317311),(#317312,
#317313,#317314),(#317315,#317316,#317317),(#317318,#317319,#317320),(#317321,
#317322,#317323),(#317324,#317325,#317326),(#317327,#317328,#317329),(#317330,
#317331,#317332),(#317333,#317334,#317335),(#317336,#317337,#317338),(#317339,
#317340,#317341),(#317342,#317343,#317344),(#317345,#317346,#317347),(#317348,
#317349,#317350),(#317351,#317352,#317353),(#317354,#317355,#317356),(#317357,
#317358,#317359),(#317360,#317361,#317362),(#317363,#317364,#317365),(#317366,
#317367,#317368),(#317369,#317370,#317371),(#317372,#317373,#317374),(#317375,
#317376,#317377),(#317378,#317379,#317380),(#317381,#317382,#317383),(#317384,
#317385,#317386),(#317387,#317388,#317389),(#317390,#317391,#317392),(#317393,
#317394,#317395),(#317396,#317397,#317398),(#317399,#317400,#317401),(#317402,
#317403,#317404),(#317405,#317406,#317407),(#317408,#317409,#317410),(#317411,
#317412,#317413),(#317414,#317415,#317416),(#317417,#317418,#317419),(#317420,
#317421,#317422),(#317423,#317424,#317425),(#317426,#317427,#317428),(#317429,
#317430,#317431),(#317432,#317433,#317434),(#317435,#317436,#317437),(#317438,
#317439,#317440),(#317441,#317442,#317443),(#317444,#317445,#317446),(#317447,
#317448,#317449),(#317450,#317451,#317452),(#317453,#317454,#317455),(#317456,
#317457,#317458),(#317459,#317460,#317461),(#317462,#317463,#317464),(#317465,
#317466,#317467),(#317468,#317469,#317470),(#317471,#317472,#317473),(#317474,
#317475,#317476),(#317477,#317478,#317479),(#317480,#317481,#317482),(#317483,
#317484,#317485),(#317486,#317487,#317488),(#317489,#317490,#317491),(#317492,
#317493,#317494),(#317495,#317496,#317497),(#317498,#317499,#317500),(#317501,
#317502,#317503),(#317504,#317505,#317506),(#317507,#317508,#317509),(#317510,
#317511,#317512),(#317513,#317514,#317515),(#317516,#317517,#317518),(#317519,
#317520,#317521),(#317522,#317523,#317524),(#317525,#317526,#317527),(#317528,
#317529,#317530),(#317531,#317532,#317533),(#317534,#317535,#317536),(#317537,
#317538,#317539),(#317540,#317541,#317542),(#317543,#317544,#317545),(#317546,
#317547,#317548),(#317549,#317550,#317551),(#317552,#317553,#317554),(#317555,
#317556,#317557),(#317558,#317559,#317560),(#317561,#317562,#317563),(#317564,
#317565,#317566),(#317567,#317568,#317569),(#317570,#317571,#317572),(#317573,
#317574,#317575),(#317576,#317577,#317578),(#317579,#317580,#317581),(#317582,
#317583,#317584),(#317585,#317586,#317587),(#317588,#317589,#317590),(#317591,
#317592,#317593),(#317594,#317595,#317596),(#317597,#317598,#317599),(#317600,
#317601,#317602),(#317603,#317604,#317605),(#317606,#317607,#317608),(#317609,
#317610,#317611),(#317612,#317613,#317614),(#317615,#317616,#317617),(#317618,
#317619,#317620),(#317621,#317622,#317623),(#317624,#317625,#317626),(#317627,
#317628,#317629),(#317630,#317631,#317632),(#317633,#317634,#317635),(#317636,
#317637,#317638),(#317639,#317640,#317641),(#317642,#317643,#317644),(#317645,
#317646,#317647),(#317648,#317649,#317650),(#317651,#317652,#317653),(#317654,
#317655,#317656),(#317657,#317658,#317659),(#317660,#317661,#317662),(#317663,
#317664,#317665),(#317666,#317667,#317668),(#317669,#317670,#317671),(#317672,
#317673,#317674),(#317675,#317676,#317677),(#317678,#317679,#317680),(#317681,
#317682,#317683),(#317684,#317685,#317686),(#317687,#317688,#317689),(#317690,
#317691,#317692),(#317693,#317694,#317695),(#317696,#317697,#317698),(#317699,
#317700,#317701),(#317702,#317703,#317704),(#317705,#317706,#317707),(#317708,
#317709,#317710),(#317711,#317712,#317713),(#317714,#317715,#317716),(#317717,
#317718,#317719),(#317720,#317721,#317722),(#317723,#317724,#317725),(#317726,
#317727,#317728),(#317729,#317730,#317731),(#317732,#317733,#317734),(#317735,
#317736,#317737),(#317738,#317739,#317740),(#317741,#317742,#317743),(#317744,
#317745,#317746),(#317747,#317748,#317749),(#317750,#317751,#317752),(#317753,
#317754,#317755),(#317756,#317757,#317758),(#317759,#317760,#317761),(#317762,
#317763,#317764),(#317765,#317766,#317767),(#317768,#317769,#317770),(#317771,
#317772,#317773),(#317774,#317775,#317776),(#317777,#317778,#317779),(#317780,
#317781,#317782),(#317783,#317784,#317785),(#317786,#317787,#317788),(#317789,
#317790,#317791),(#317792,#317793,#317794),(#317795,#317796,#317797),(#317798,
#317799,#317800),(#317801,#317802,#317803),(#317804,#317805,#317806),(#317807,
#317808,#317809),(#317810,#317811,#317812),(#317813,#317814,#317815),(#317816,
#317817,#317818),(#317819,#317820,#317821),(#317822,#317823,#317824),(#317825,
#317826,#317827),(#317828,#317829,#317830),(#317831,#317832,#317833),(#317834,
#317835,#317836),(#317837,#317838,#317839),(#317840,#317841,#317842),(#317843,
#317844,#317845),(#317846,#317847,#317848),(#317849,#317850,#317851),(#317852,
#317853,#317854),(#317855,#317856,#317857),(#317858,#317859,#317860),(#317861,
#317862,#317863),(#317864,#317865,#317866),(#317867,#317868,#317869),(#317870,
#317871,#317872),(#317873,#317874,#317875),(#317876,#317877,#317878),(#317879,
#317880,#317881),(#317882,#317883,#317884),(#317885,#317886,#317887),(#317888,
#317889,#317890),(#317891,#317892,#317893),(#317894,#317895,#317896),(#317897,
#317898,#317899),(#317900,#317901,#317902),(#317903,#317904,#317905),(#317906,
#317907,#317908),(#317909,#317910,#317911),(#317912,#317913,#317914),(#317915,
#317916,#317917),(#317918,#317919,#317920),(#317921,#317922,#317923),(#317924,
#317925,#317926),(#317927,#317928,#317929),(#317930,#317931,#317932),(#317933,
#317934,#317935),(#317936,#317937,#317938),(#317939,#317940,#317941),(#317942,
#317943,#317944),(#317945,#317946,#317947),(#317948,#317949,#317950),(#317951,
#317952,#317953),(#317954,#317955,#317956),(#317957,#317958,#317959),(#317960,
#317961,#317962),(#317963,#317964,#317965),(#317966,#317967,#317968),(#317969,
#317970,#317971),(#317972,#317973,#317974),(#317975,#317976,#317977),(#317978,
#317979,#317980),(#317981,#317982,#317983),(#317984,#317985,#317986),(#317987,
#317988,#317989)),.UNSPECIFIED.,.F.,.F.,.F.,(6,1,1,1,1,1,1,1,1,1,1,1,1,
1,1,1,1,1,1,1,1,1,1,1,1,1,1,1,1,1,1,1,1,1,1,1,1,1,1,1,1,1,1,1,1,1,1,1,1,
1,1,1,1,1,1,1,1,1,1,1,1,1,1,1,1,1,1,1,1,1,1,1,1,1,1,1,1,1,1,1,1,1,1,1,1,
1,1,1,1,1,1,1,1,1,1,1,1,1,1,1,1,1,1,1,1,1,1,1,1,1,1,1,1,1,1,1,1,1,1,1,1,
1,1,1,1,1,1,1,1,1,1,1,1,1,1,1,1,1,1,1,1,1,1,1,1,1,1,1,1,1,1,1,1,1,1,1,1,
1,1,1,1,1,1,1,1,1,1,1,1,1,1,1,1,1,1,1,1,1,1,1,1,1,1,1,1,1,1,1,1,1,1,1,1,
1,1,1,1,1,1,1,1,1,1,1,1,1,1,1,1,1,1,1,1,1,1,1,1,1,1,1,1,1,1,1,1,1,1,1,1,
1,1,1,1,1,1,1,1,1,1,1,1,1,1,1,1,1,1,1,1,1,1,1,1,1,1,1,1,1,1,1,1,1,1,1,1,
1,1,1,1,1,1,1,1,1,1,1,1,1,1,1,1,1,1,1,1,1,1,1,1,1,1,1,1,1,1,1,1,1,1,1,1,
1,1,1,1,1,1,1,1,1,1,1,1,1,1,1,1,1,1,1,1,1,1,1,1,1,1,1,1,1,1,1,1,1,1,1,1,
1,1,1,1,1,1,1,1,1,1,1,1,1,1,1,1,1,1,1,1,1,1,1,1,1,1,1,1,1,1,1,1,1,1,1,1,
1,1,1,1,1,1,1,1,1,1,1,1,1,1,1,1,1,1,1,1,1,1,1,1,1,1,1,1,1,1,1,1,1,1,1,1,
1,1,1,1,1,1,1,1,1,1,1,1,1,1,1,1,1,1,1,1,1,1,1,1,1,1,1,1,1,1,1,1,1,1,1,1,
1,1,1,1,1,1,1,1,1,1,1,1,1,1,1,1,1,1,1,1,1,1,1,1,1,1,1,1,1,1,1,1,1,1,1,1,
1,1,1,1,1,1,1,1,1,1,1,1,1,1,1,1,1,1,1,1,1,1,1,1,1,1,1,1,1,1,1,1,1,1,1,1,
1,1,1,1,1,1,1,1,1,1,1,1,1,1,1,1,1,1,1,1,1,1,1,1,1,1,1,1,1,6),(2,1,2),(-0.001964191,
0.,0.001834862,0.003669725,0.005504587,0.00733945,0.009174312,0.011009174,
0.012844037,0.014678899,0.016513761,0.018348624,0.020183486,0.022018349,
0.023853211,0.025688073,0.027522936,0.029357798,0.031192661,0.033027523,
0.034862385,0.036697248,0.03853211,0.040366972,0.042201835,0.044036697,
0.04587156,0.047706422,0.049541284,0.051376147,0.053211009,0.055045872,
0.056880734,0.058715596,0.060550459,0.062385321,0.064220183,0.066055046,
0.067889908,0.069724771,0.071559633,0.073394495,0.075229358,0.07706422,
0.078899083,0.080733945,0.082568807,0.08440367,0.086238532,0.088073394,
0.089908257,0.091743119,0.093577982,0.095412844,0.097247706,0.099082569,
0.100917431,0.102752294,0.104587156,0.106422018,0.108256881,0.110091743,
0.111926606,0.113761468,0.11559633,0.117431193,0.119266055,0.121100917,
0.12293578,0.124770642,0.126605505,0.128440367,0.130275229,0.132110092,
0.133944954,0.135779817,0.137614679,0.139449541,0.141284404,0.143119266,
0.144954128,0.146788991,0.148623853,0.150458716,0.152293578,0.15412844,
0.155963303,0.157798165,0.159633028,0.16146789,0.163302752,0.165137615,
0.166972477,0.168807339,0.170642202,0.172477064,0.174311927,0.176146789,
0.177981651,0.179816514,0.181651376,0.183486239,0.185321101,0.187155963,
0.188990826,0.190825688,0.19266055,0.194495413,0.196330275,0.198165138,
0.2,0.201834862,0.203669725,0.205504587,0.20733945,0.209174312,0.211009174,
0.212844037,0.214678899,0.216513761,0.218348624,0.220183486,0.222018349,
0.223853211,0.225688073,0.227522936,0.229357798,0.231192661,0.233027523,
0.234862385,0.236697248,0.23853211,0.240366972,0.242201835,0.244036697,
0.24587156,0.247706422,0.249541284,0.251376147,0.253211009,0.255045872,
0.256880734,0.258715596,0.260550459,0.262385321,0.264220183,0.266055046,
0.267889908,0.269724771,0.271559633,0.273394495,0.275229358,0.27706422,
0.278899083,0.280733945,0.282568807,0.28440367,0.286238532,0.288073394,
0.289908257,0.291743119,0.293577982,0.295412844,0.297247706,0.299082569,
0.300917431,0.302752294,0.304587156,0.306422018,0.308256881,0.310091743,
0.311926606,0.313761468,0.31559633,0.317431193,0.319266055,0.321100917,
0.32293578,0.324770642,0.326605505,0.328440367,0.330275229,0.332110092,
0.333944954,0.335779817,0.337614679,0.339449541,0.341284404,0.343119266,
0.344954128,0.346788991,0.348623853,0.350458716,0.352293578,0.35412844,
0.355963303,0.357798165,0.359633028,0.36146789,0.363302752,0.365137615,
0.366972477,0.368807339,0.370642202,0.372477064,0.374311927,0.376146789,
0.377981651,0.379816514,0.381651376,0.383486239,0.385321101,0.387155963,
0.388990826,0.390825688,0.39266055,0.394495413,0.396330275,0.398165138,
0.4,0.401834862,0.403669725,0.405504587,0.40733945,0.409174312,0.411009174,
0.412844037,0.414678899,0.416513761,0.418348624,0.420183486,0.422018349,
0.423853211,0.425688073,0.427522936,0.429357798,0.431192661,0.433027523,
0.434862385,0.436697248,0.43853211,0.440366972,0.442201835,0.444036697,
0.44587156,0.447706422,0.449541284,0.451376147,0.453211009,0.455045872,
0.456880734,0.458715596,0.460550459,0.462385321,0.464220183,0.466055046,
0.467889908,0.469724771,0.471559633,0.473394495,0.475229358,0.47706422,
0.478899083,0.480733945,0.482568807,0.48440367,0.486238532,0.488073394,
0.489908257,0.491743119,0.493577982,0.495412844,0.497247706,0.499082569,
0.500917431,0.502752294,0.504587156,0.506422018,0.508256881,0.510091743,
0.511926606,0.513761468,0.51559633,0.517431193,0.519266055,0.521100917,
0.52293578,0.524770642,0.526605505,0.528440367,0.530275229,0.532110092,
0.533944954,0.535779817,0.537614679,0.539449541,0.541284404,0.543119266,
0.544954128,0.546788991,0.548623853,0.550458716,0.552293578,0.55412844,
0.555963303,0.557798165,0.559633028,0.56146789,0.563302752,0.565137615,
0.566972477,0.568807339,0.570642202,0.572477064,0.574311927,0.576146789,
0.577981651,0.579816514,0.581651376,0.583486239,0.585321101,0.587155963,
0.588990826,0.590825688,0.59266055,0.594495413,0.596330275,0.598165138,
0.6,0.601834862,0.603669725,0.605504587,0.60733945,0.609174312,0.611009174,
0.612844037,0.614678899,0.616513761,0.618348624,0.620183486,0.622018349,
0.623853211,0.625688073,0.627522936,0.629357798,0.631192661,0.633027523,
0.634862385,0.636697248,0.63853211,0.640366972,0.642201835,0.644036697,
0.64587156,0.647706422,0.649541284,0.651376147,0.653211009,0.655045872,
0.656880734,0.658715596,0.660550459,0.662385321,0.664220183,0.666055046,
0.667889908,0.669724771,0.671559633,0.673394495,0.675229358,0.67706422,
0.678899083,0.680733945,0.682568807,0.68440367,0.686238532,0.688073394,
0.689908257,0.691743119,0.693577982,0.695412844,0.697247706,0.699082569,
0.700917431,0.702752294,0.704587156,0.706422018,0.708256881,0.710091743,
0.711926606,0.713761468,0.71559633,0.717431193,0.719266055,0.721100917,
0.72293578,0.724770642,0.726605505,0.728440367,0.730275229,0.732110092,
0.733944954,0.735779817,0.737614679,0.739449541,0.741284404,0.743119266,
0.744954128,0.746788991,0.748623853,0.750458716,0.752293578,0.75412844,
0.755963303,0.757798165,0.759633028,0.76146789,0.763302752,0.765137615,
0.766972477,0.768807339,0.770642202,0.772477064,0.774311927,0.776146789,
0.777981651,0.779816514,0.781651376,0.783486239,0.785321101,0.787155963,
0.788990826,0.790825688,0.79266055,0.794495413,0.796330275,0.798165138,
0.8,0.801834862,0.803669725,0.805504587,0.80733945,0.809174312,0.811009174,
0.812844037,0.814678899,0.816513761,0.818348624,0.820183486,0.822018349,
0.823853211,0.825688073,0.827522936,0.829357798,0.831192661,0.833027523,
0.834862385,0.836697248,0.83853211,0.840366972,0.842201835,0.844036697,
0.84587156,0.847706422,0.849541284,0.851376147,0.853211009,0.855045872,
0.856880734,0.858715596,0.860550459,0.862385321,0.864220183,0.866055046,
0.867889908,0.869724771,0.871559633,0.873394495,0.875229358,0.87706422,
0.878899083,0.880733945,0.882568807,0.88440367,0.886238532,0.888073394,
0.889908257,0.891743119,0.893577982,0.895412844,0.897247706,0.899082569,
0.900917431,0.902752294,0.904587156,0.906422018,0.908256881,0.910091743,
0.911926606,0.913761468,0.91559633,0.917431193,0.919266055,0.921100917,
0.92293578,0.924770642,0.926605505,0.928440367,0.930275229,0.932110092,
0.933944954,0.935779817,0.937614679,0.939449541,0.941284404,0.943119266,
0.944954128,0.946788991,0.948623853,0.950458716,0.952293578,0.95412844,
0.955963303,0.957798165,0.959633028,0.96146789,0.963302752,0.965137615,
0.966972477,0.968807339,0.970642202,0.972477064,0.974311927,0.976146789,
0.977981651,0.979816514,0.981651376,0.983486239,0.985321101,0.987155963,
0.988990826,0.990825688,0.99266055,0.994495413,0.996330275,0.998165138,
1.),(0.3,1.,1.3),.UNSPECIFIED.);
#6313=B_SPLINE_SURFACE_WITH_KNOTS('',5,1,((#318012,#318013,#318014),(#318015,
#318016,#318017),(#318018,#318019,#318020),(#318021,#318022,#318023),(#318024,
#318025,#318026),(#318027,#318028,#318029),(#318030,#318031,#318032),(#318033,
#318034,#318035),(#318036,#318037,#318038),(#318039,#318040,#318041),(#318042,
#318043,#318044),(#318045,#318046,#318047),(#318048,#318049,#318050),(#318051,
#318052,#318053),(#318054,#318055,#318056),(#318057,#318058,#318059),(#318060,
#318061,#318062),(#318063,#318064,#318065),(#318066,#318067,#318068),(#318069,
#318070,#318071),(#318072,#318073,#318074),(#318075,#318076,#318077),(#318078,
#318079,#318080),(#318081,#318082,#318083),(#318084,#318085,#318086),(#318087,
#318088,#318089),(#318090,#318091,#318092),(#318093,#318094,#318095),(#318096,
#318097,#318098),(#318099,#318100,#318101),(#318102,#318103,#318104),(#318105,
#318106,#318107),(#318108,#318109,#318110),(#318111,#318112,#318113),(#318114,
#318115,#318116),(#318117,#318118,#318119),(#318120,#318121,#318122),(#318123,
#318124,#318125),(#318126,#318127,#318128),(#318129,#318130,#318131),(#318132,
#318133,#318134),(#318135,#318136,#318137),(#318138,#318139,#318140),(#318141,
#318142,#318143),(#318144,#318145,#318146),(#318147,#318148,#318149),(#318150,
#318151,#318152),(#318153,#318154,#318155),(#318156,#318157,#318158),(#318159,
#318160,#318161),(#318162,#318163,#318164),(#318165,#318166,#318167),(#318168,
#318169,#318170),(#318171,#318172,#318173),(#318174,#318175,#318176),(#318177,
#318178,#318179),(#318180,#318181,#318182),(#318183,#318184,#318185),(#318186,
#318187,#318188),(#318189,#318190,#318191),(#318192,#318193,#318194),(#318195,
#318196,#318197),(#318198,#318199,#318200),(#318201,#318202,#318203),(#318204,
#318205,#318206),(#318207,#318208,#318209),(#318210,#318211,#318212),(#318213,
#318214,#318215),(#318216,#318217,#318218),(#318219,#318220,#318221),(#318222,
#318223,#318224),(#318225,#318226,#318227),(#318228,#318229,#318230),(#318231,
#318232,#318233),(#318234,#318235,#318236),(#318237,#318238,#318239),(#318240,
#318241,#318242),(#318243,#318244,#318245),(#318246,#318247,#318248),(#318249,
#318250,#318251),(#318252,#318253,#318254),(#318255,#318256,#318257),(#318258,
#318259,#318260),(#318261,#318262,#318263),(#318264,#318265,#318266),(#318267,
#318268,#318269),(#318270,#318271,#318272),(#318273,#318274,#318275),(#318276,
#318277,#318278),(#318279,#318280,#318281),(#318282,#318283,#318284),(#318285,
#318286,#318287),(#318288,#318289,#318290),(#318291,#318292,#318293),(#318294,
#318295,#318296),(#318297,#318298,#318299),(#318300,#318301,#318302),(#318303,
#318304,#318305),(#318306,#318307,#318308),(#318309,#318310,#318311),(#318312,
#318313,#318314),(#318315,#318316,#318317),(#318318,#318319,#318320),(#318321,
#318322,#318323),(#318324,#318325,#318326),(#318327,#318328,#318329),(#318330,
#318331,#318332),(#318333,#318334,#318335),(#318336,#318337,#318338),(#318339,
#318340,#318341),(#318342,#318343,#318344),(#318345,#318346,#318347),(#318348,
#318349,#318350),(#318351,#318352,#318353),(#318354,#318355,#318356),(#318357,
#318358,#318359),(#318360,#318361,#318362),(#318363,#318364,#318365),(#318366,
#318367,#318368),(#318369,#318370,#318371),(#318372,#318373,#318374),(#318375,
#318376,#318377),(#318378,#318379,#318380),(#318381,#318382,#318383),(#318384,
#318385,#318386),(#318387,#318388,#318389),(#318390,#318391,#318392),(#318393,
#318394,#318395),(#318396,#318397,#318398),(#318399,#318400,#318401),(#318402,
#318403,#318404),(#318405,#318406,#318407),(#318408,#318409,#318410),(#318411,
#318412,#318413),(#318414,#318415,#318416),(#318417,#318418,#318419),(#318420,
#318421,#318422),(#318423,#318424,#318425),(#318426,#318427,#318428),(#318429,
#318430,#318431),(#318432,#318433,#318434),(#318435,#318436,#318437),(#318438,
#318439,#318440),(#318441,#318442,#318443),(#318444,#318445,#318446),(#318447,
#318448,#318449),(#318450,#318451,#318452),(#318453,#318454,#318455),(#318456,
#318457,#318458),(#318459,#318460,#318461),(#318462,#318463,#318464),(#318465,
#318466,#318467),(#318468,#318469,#318470),(#318471,#318472,#318473),(#318474,
#318475,#318476),(#318477,#318478,#318479),(#318480,#318481,#318482),(#318483,
#318484,#318485),(#318486,#318487,#318488),(#318489,#318490,#318491),(#318492,
#318493,#318494),(#318495,#318496,#318497),(#318498,#318499,#318500),(#318501,
#318502,#318503),(#318504,#318505,#318506),(#318507,#318508,#318509),(#318510,
#318511,#318512),(#318513,#318514,#318515),(#318516,#318517,#318518),(#318519,
#318520,#318521),(#318522,#318523,#318524),(#318525,#318526,#318527),(#318528,
#318529,#318530),(#318531,#318532,#318533),(#318534,#318535,#318536),(#318537,
#318538,#318539),(#318540,#318541,#318542),(#318543,#318544,#318545),(#318546,
#318547,#318548),(#318549,#318550,#318551),(#318552,#318553,#318554),(#318555,
#318556,#318557),(#318558,#318559,#318560),(#318561,#318562,#318563),(#318564,
#318565,#318566),(#318567,#318568,#318569),(#318570,#318571,#318572),(#318573,
#318574,#318575),(#318576,#318577,#318578),(#318579,#318580,#318581),(#318582,
#318583,#318584),(#318585,#318586,#318587),(#318588,#318589,#318590),(#318591,
#318592,#318593),(#318594,#318595,#318596),(#318597,#318598,#318599),(#318600,
#318601,#318602),(#318603,#318604,#318605),(#318606,#318607,#318608),(#318609,
#318610,#318611),(#318612,#318613,#318614),(#318615,#318616,#318617),(#318618,
#318619,#318620),(#318621,#318622,#318623),(#318624,#318625,#318626),(#318627,
#318628,#318629),(#318630,#318631,#318632),(#318633,#318634,#318635),(#318636,
#318637,#318638),(#318639,#318640,#318641),(#318642,#318643,#318644),(#318645,
#318646,#318647),(#318648,#318649,#318650),(#318651,#318652,#318653),(#318654,
#318655,#318656),(#318657,#318658,#318659),(#318660,#318661,#318662),(#318663,
#318664,#318665),(#318666,#318667,#318668),(#318669,#318670,#318671),(#318672,
#318673,#318674),(#318675,#318676,#318677),(#318678,#318679,#318680),(#318681,
#318682,#318683),(#318684,#318685,#318686),(#318687,#318688,#318689),(#318690,
#318691,#318692),(#318693,#318694,#318695),(#318696,#318697,#318698),(#318699,
#318700,#318701),(#318702,#318703,#318704),(#318705,#318706,#318707),(#318708,
#318709,#318710),(#318711,#318712,#318713),(#318714,#318715,#318716),(#318717,
#318718,#318719),(#318720,#318721,#318722),(#318723,#318724,#318725),(#318726,
#318727,#318728),(#318729,#318730,#318731),(#318732,#318733,#318734),(#318735,
#318736,#318737),(#318738,#318739,#318740),(#318741,#318742,#318743),(#318744,
#318745,#318746),(#318747,#318748,#318749),(#318750,#318751,#318752),(#318753,
#318754,#318755),(#318756,#318757,#318758),(#318759,#318760,#318761),(#318762,
#318763,#318764),(#318765,#318766,#318767),(#318768,#318769,#318770),(#318771,
#318772,#318773),(#318774,#318775,#318776),(#318777,#318778,#318779),(#318780,
#318781,#318782),(#318783,#318784,#318785),(#318786,#318787,#318788),(#318789,
#318790,#318791),(#318792,#318793,#318794),(#318795,#318796,#318797),(#318798,
#318799,#318800),(#318801,#318802,#318803),(#318804,#318805,#318806),(#318807,
#318808,#318809),(#318810,#318811,#318812),(#318813,#318814,#318815),(#318816,
#318817,#318818),(#318819,#318820,#318821),(#318822,#318823,#318824),(#318825,
#318826,#318827),(#318828,#318829,#318830),(#318831,#318832,#318833),(#318834,
#318835,#318836),(#318837,#318838,#318839),(#318840,#318841,#318842),(#318843,
#318844,#318845),(#318846,#318847,#318848),(#318849,#318850,#318851),(#318852,
#318853,#318854),(#318855,#318856,#318857),(#318858,#318859,#318860),(#318861,
#318862,#318863),(#318864,#318865,#318866),(#318867,#318868,#318869),(#318870,
#318871,#318872),(#318873,#318874,#318875),(#318876,#318877,#318878),(#318879,
#318880,#318881),(#318882,#318883,#318884),(#318885,#318886,#318887),(#318888,
#318889,#318890),(#318891,#318892,#318893),(#318894,#318895,#318896),(#318897,
#318898,#318899),(#318900,#318901,#318902),(#318903,#318904,#318905),(#318906,
#318907,#318908),(#318909,#318910,#318911),(#318912,#318913,#318914),(#318915,
#318916,#318917),(#318918,#318919,#318920),(#318921,#318922,#318923),(#318924,
#318925,#318926),(#318927,#318928,#318929),(#318930,#318931,#318932),(#318933,
#318934,#318935),(#318936,#318937,#318938),(#318939,#318940,#318941),(#318942,
#318943,#318944),(#318945,#318946,#318947),(#318948,#318949,#318950),(#318951,
#318952,#318953),(#318954,#318955,#318956),(#318957,#318958,#318959),(#318960,
#318961,#318962),(#318963,#318964,#318965),(#318966,#318967,#318968),(#318969,
#318970,#318971),(#318972,#318973,#318974),(#318975,#318976,#318977),(#318978,
#318979,#318980),(#318981,#318982,#318983),(#318984,#318985,#318986),(#318987,
#318988,#318989),(#318990,#318991,#318992),(#318993,#318994,#318995),(#318996,
#318997,#318998),(#318999,#319000,#319001),(#319002,#319003,#319004),(#319005,
#319006,#319007),(#319008,#319009,#319010),(#319011,#319012,#319013),(#319014,
#319015,#319016),(#319017,#319018,#319019),(#319020,#319021,#319022),(#319023,
#319024,#319025),(#319026,#319027,#319028),(#319029,#319030,#319031),(#319032,
#319033,#319034),(#319035,#319036,#319037),(#319038,#319039,#319040),(#319041,
#319042,#319043),(#319044,#319045,#319046),(#319047,#319048,#319049),(#319050,
#319051,#319052),(#319053,#319054,#319055),(#319056,#319057,#319058),(#319059,
#319060,#319061),(#319062,#319063,#319064),(#319065,#319066,#319067),(#319068,
#319069,#319070),(#319071,#319072,#319073),(#319074,#319075,#319076),(#319077,
#319078,#319079),(#319080,#319081,#319082),(#319083,#319084,#319085),(#319086,
#319087,#319088),(#319089,#319090,#319091),(#319092,#319093,#319094),(#319095,
#319096,#319097),(#319098,#319099,#319100),(#319101,#319102,#319103),(#319104,
#319105,#319106),(#319107,#319108,#319109),(#319110,#319111,#319112),(#319113,
#319114,#319115),(#319116,#319117,#319118),(#319119,#319120,#319121),(#319122,
#319123,#319124),(#319125,#319126,#319127),(#319128,#319129,#319130),(#319131,
#319132,#319133),(#319134,#319135,#319136),(#319137,#319138,#319139),(#319140,
#319141,#319142),(#319143,#319144,#319145),(#319146,#319147,#319148),(#319149,
#319150,#319151),(#319152,#319153,#319154),(#319155,#319156,#319157),(#319158,
#319159,#319160),(#319161,#319162,#319163),(#319164,#319165,#319166),(#319167,
#319168,#319169),(#319170,#319171,#319172),(#319173,#319174,#319175),(#319176,
#319177,#319178),(#319179,#319180,#319181),(#319182,#319183,#319184),(#319185,
#319186,#319187),(#319188,#319189,#319190),(#319191,#319192,#319193),(#319194,
#319195,#319196),(#319197,#319198,#319199),(#319200,#319201,#319202),(#319203,
#319204,#319205),(#319206,#319207,#319208),(#319209,#319210,#319211),(#319212,
#319213,#319214),(#319215,#319216,#319217),(#319218,#319219,#319220),(#319221,
#319222,#319223),(#319224,#319225,#319226),(#319227,#319228,#319229),(#319230,
#319231,#319232),(#319233,#319234,#319235),(#319236,#319237,#319238),(#319239,
#319240,#319241),(#319242,#319243,#319244),(#319245,#319246,#319247),(#319248,
#319249,#319250),(#319251,#319252,#319253),(#319254,#319255,#319256),(#319257,
#319258,#319259),(#319260,#319261,#319262),(#319263,#319264,#319265),(#319266,
#319267,#319268),(#319269,#319270,#319271),(#319272,#319273,#319274),(#319275,
#319276,#319277),(#319278,#319279,#319280),(#319281,#319282,#319283),(#319284,
#319285,#319286),(#319287,#319288,#319289),(#319290,#319291,#319292),(#319293,
#319294,#319295),(#319296,#319297,#319298),(#319299,#319300,#319301),(#319302,
#319303,#319304),(#319305,#319306,#319307),(#319308,#319309,#319310),(#319311,
#319312,#319313),(#319314,#319315,#319316),(#319317,#319318,#319319),(#319320,
#319321,#319322),(#319323,#319324,#319325),(#319326,#319327,#319328),(#319329,
#319330,#319331),(#319332,#319333,#319334),(#319335,#319336,#319337),(#319338,
#319339,#319340),(#319341,#319342,#319343),(#319344,#319345,#319346),(#319347,
#319348,#319349),(#319350,#319351,#319352),(#319353,#319354,#319355),(#319356,
#319357,#319358),(#319359,#319360,#319361),(#319362,#319363,#319364),(#319365,
#319366,#319367),(#319368,#319369,#319370),(#319371,#319372,#319373),(#319374,
#319375,#319376),(#319377,#319378,#319379),(#319380,#319381,#319382),(#319383,
#319384,#319385),(#319386,#319387,#319388),(#319389,#319390,#319391),(#319392,
#319393,#319394),(#319395,#319396,#319397),(#319398,#319399,#319400),(#319401,
#319402,#319403),(#319404,#319405,#319406),(#319407,#319408,#319409),(#319410,
#319411,#319412),(#319413,#319414,#319415),(#319416,#319417,#319418),(#319419,
#319420,#319421),(#319422,#319423,#319424),(#319425,#319426,#319427),(#319428,
#319429,#319430),(#319431,#319432,#319433),(#319434,#319435,#319436),(#319437,
#319438,#319439),(#319440,#319441,#319442),(#319443,#319444,#319445),(#319446,
#319447,#319448),(#319449,#319450,#319451),(#319452,#319453,#319454),(#319455,
#319456,#319457),(#319458,#319459,#319460),(#319461,#319462,#319463),(#319464,
#319465,#319466),(#319467,#319468,#319469),(#319470,#319471,#319472),(#319473,
#319474,#319475),(#319476,#319477,#319478),(#319479,#319480,#319481),(#319482,
#319483,#319484),(#319485,#319486,#319487),(#319488,#319489,#319490),(#319491,
#319492,#319493),(#319494,#319495,#319496),(#319497,#319498,#319499),(#319500,
#319501,#319502),(#319503,#319504,#319505),(#319506,#319507,#319508),(#319509,
#319510,#319511),(#319512,#319513,#319514),(#319515,#319516,#319517),(#319518,
#319519,#319520),(#319521,#319522,#319523),(#319524,#319525,#319526),(#319527,
#319528,#319529),(#319530,#319531,#319532),(#319533,#319534,#319535),(#319536,
#319537,#319538),(#319539,#319540,#319541),(#319542,#319543,#319544),(#319545,
#319546,#319547),(#319548,#319549,#319550),(#319551,#319552,#319553),(#319554,
#319555,#319556),(#319557,#319558,#319559),(#319560,#319561,#319562),(#319563,
#319564,#319565),(#319566,#319567,#319568),(#319569,#319570,#319571),(#319572,
#319573,#319574),(#319575,#319576,#319577),(#319578,#319579,#319580),(#319581,
#319582,#319583),(#319584,#319585,#319586),(#319587,#319588,#319589),(#319590,
#319591,#319592),(#319593,#319594,#319595),(#319596,#319597,#319598),(#319599,
#319600,#319601),(#319602,#319603,#319604),(#319605,#319606,#319607),(#319608,
#319609,#319610),(#319611,#319612,#319613),(#319614,#319615,#319616),(#319617,
#319618,#319619),(#319620,#319621,#319622),(#319623,#319624,#319625),(#319626,
#319627,#319628),(#319629,#319630,#319631),(#319632,#319633,#319634),(#319635,
#319636,#319637),(#319638,#319639,#319640),(#319641,#319642,#319643),(#319644,
#319645,#319646),(#319647,#319648,#319649),(#319650,#319651,#319652),(#319653,
#319654,#319655),(#319656,#319657,#319658),(#319659,#319660,#319661)),
 .UNSPECIFIED.,.F.,.F.,.F.,(6,1,1,1,1,1,1,1,1,1,1,1,1,1,1,1,1,1,1,1,1,1,
1,1,1,1,1,1,1,1,1,1,1,1,1,1,1,1,1,1,1,1,1,1,1,1,1,1,1,1,1,1,1,1,1,1,1,1,
1,1,1,1,1,1,1,1,1,1,1,1,1,1,1,1,1,1,1,1,1,1,1,1,1,1,1,1,1,1,1,1,1,1,1,1,
1,1,1,1,1,1,1,1,1,1,1,1,1,1,1,1,1,1,1,1,1,1,1,1,1,1,1,1,1,1,1,1,1,1,1,1,
1,1,1,1,1,1,1,1,1,1,1,1,1,1,1,1,1,1,1,1,1,1,1,1,1,1,1,1,1,1,1,1,1,1,1,1,
1,1,1,1,1,1,1,1,1,1,1,1,1,1,1,1,1,1,1,1,1,1,1,1,1,1,1,1,1,1,1,1,1,1,1,1,
1,1,1,1,1,1,1,1,1,1,1,1,1,1,1,1,1,1,1,1,1,1,1,1,1,1,1,1,1,1,1,1,1,1,1,1,
1,1,1,1,1,1,1,1,1,1,1,1,1,1,1,1,1,1,1,1,1,1,1,1,1,1,1,1,1,1,1,1,1,1,1,1,
1,1,1,1,1,1,1,1,1,1,1,1,1,1,1,1,1,1,1,1,1,1,1,1,1,1,1,1,1,1,1,1,1,1,1,1,
1,1,1,1,1,1,1,1,1,1,1,1,1,1,1,1,1,1,1,1,1,1,1,1,1,1,1,1,1,1,1,1,1,1,1,1,
1,1,1,1,1,1,1,1,1,1,1,1,1,1,1,1,1,1,1,1,1,1,1,1,1,1,1,1,1,1,1,1,1,1,1,1,
1,1,1,1,1,1,1,1,1,1,1,1,1,1,1,1,1,1,1,1,1,1,1,1,1,1,1,1,1,1,1,1,1,1,1,1,
1,1,1,1,1,1,1,1,1,1,1,1,1,1,1,1,1,1,1,1,1,1,1,1,1,1,1,1,1,1,1,1,1,1,1,1,
1,1,1,1,1,1,1,1,1,1,1,1,1,1,1,1,1,1,1,1,1,1,1,1,1,1,1,1,1,1,1,1,1,1,1,1,
1,1,1,1,1,1,1,1,1,1,1,1,1,1,1,1,1,1,1,1,1,1,1,1,1,1,1,1,1,1,1,1,1,1,1,1,
1,1,1,1,1,1,1,1,1,1,1,1,1,1,1,1,1,1,1,6),(2,1,2),(-1.,-0.998165138,-0.996330275,
-0.994495413,-0.99266055,-0.990825688,-0.988990826,-0.987155963,-0.985321101,
-0.983486239,-0.981651376,-0.979816514,-0.977981651,-0.976146789,-0.974311927,
-0.972477064,-0.970642202,-0.968807339,-0.966972477,-0.965137615,-0.963302752,
-0.96146789,-0.959633028,-0.957798165,-0.955963303,-0.95412844,-0.952293578,
-0.950458716,-0.948623853,-0.946788991,-0.944954128,-0.943119266,-0.941284404,
-0.939449541,-0.937614679,-0.935779817,-0.933944954,-0.932110092,-0.930275229,
-0.928440367,-0.926605505,-0.924770642,-0.92293578,-0.921100917,-0.919266055,
-0.917431193,-0.91559633,-0.913761468,-0.911926606,-0.910091743,-0.908256881,
-0.906422018,-0.904587156,-0.902752294,-0.900917431,-0.899082569,-0.897247706,
-0.895412844,-0.893577982,-0.891743119,-0.889908257,-0.888073394,-0.886238532,
-0.88440367,-0.882568807,-0.880733945,-0.878899083,-0.87706422,-0.875229358,
-0.873394495,-0.871559633,-0.869724771,-0.867889908,-0.866055046,-0.864220183,
-0.862385321,-0.860550459,-0.858715596,-0.856880734,-0.855045872,-0.853211009,
-0.851376147,-0.849541284,-0.847706422,-0.84587156,-0.844036697,-0.842201835,
-0.840366972,-0.83853211,-0.836697248,-0.834862385,-0.833027523,-0.831192661,
-0.829357798,-0.827522936,-0.825688073,-0.823853211,-0.822018349,-0.820183486,
-0.818348624,-0.816513761,-0.814678899,-0.812844037,-0.811009174,-0.809174312,
-0.80733945,-0.805504587,-0.803669725,-0.801834862,-0.8,-0.798165138,-0.796330275,
-0.794495413,-0.79266055,-0.790825688,-0.788990826,-0.787155963,-0.785321101,
-0.783486239,-0.781651376,-0.779816514,-0.777981651,-0.776146789,-0.774311927,
-0.772477064,-0.770642202,-0.768807339,-0.766972477,-0.765137615,-0.763302752,
-0.76146789,-0.759633028,-0.757798165,-0.755963303,-0.75412844,-0.752293578,
-0.750458716,-0.748623853,-0.746788991,-0.744954128,-0.743119266,-0.741284404,
-0.739449541,-0.737614679,-0.735779817,-0.733944954,-0.732110092,-0.730275229,
-0.728440367,-0.726605505,-0.724770642,-0.72293578,-0.721100917,-0.719266055,
-0.717431193,-0.71559633,-0.713761468,-0.711926606,-0.710091743,-0.708256881,
-0.706422018,-0.704587156,-0.702752294,-0.700917431,-0.699082569,-0.697247706,
-0.695412844,-0.693577982,-0.691743119,-0.689908257,-0.688073394,-0.686238532,
-0.68440367,-0.682568807,-0.680733945,-0.678899083,-0.67706422,-0.675229358,
-0.673394495,-0.671559633,-0.669724771,-0.667889908,-0.666055046,-0.664220183,
-0.662385321,-0.660550459,-0.658715596,-0.656880734,-0.655045872,-0.653211009,
-0.651376147,-0.649541284,-0.647706422,-0.64587156,-0.644036697,-0.642201835,
-0.640366972,-0.63853211,-0.636697248,-0.634862385,-0.633027523,-0.631192661,
-0.629357798,-0.627522936,-0.625688073,-0.623853211,-0.622018349,-0.620183486,
-0.618348624,-0.616513761,-0.614678899,-0.612844037,-0.611009174,-0.609174312,
-0.60733945,-0.605504587,-0.603669725,-0.601834862,-0.6,-0.598165138,-0.596330275,
-0.594495413,-0.59266055,-0.590825688,-0.588990826,-0.587155963,-0.585321101,
-0.583486239,-0.581651376,-0.579816514,-0.577981651,-0.576146789,-0.574311927,
-0.572477064,-0.570642202,-0.568807339,-0.566972477,-0.565137615,-0.563302752,
-0.56146789,-0.559633028,-0.557798165,-0.555963303,-0.55412844,-0.552293578,
-0.550458716,-0.548623853,-0.546788991,-0.544954128,-0.543119266,-0.541284404,
-0.539449541,-0.537614679,-0.535779817,-0.533944954,-0.532110092,-0.530275229,
-0.528440367,-0.526605505,-0.524770642,-0.52293578,-0.521100917,-0.519266055,
-0.517431193,-0.51559633,-0.513761468,-0.511926606,-0.510091743,-0.508256881,
-0.506422018,-0.504587156,-0.502752294,-0.500917431,-0.499082569,-0.497247706,
-0.495412844,-0.493577982,-0.491743119,-0.489908257,-0.488073394,-0.486238532,
-0.48440367,-0.482568807,-0.480733945,-0.478899083,-0.47706422,-0.475229358,
-0.473394495,-0.471559633,-0.469724771,-0.467889908,-0.466055046,-0.464220183,
-0.462385321,-0.460550459,-0.458715596,-0.456880734,-0.455045872,-0.453211009,
-0.451376147,-0.449541284,-0.447706422,-0.44587156,-0.444036697,-0.442201835,
-0.440366972,-0.43853211,-0.436697248,-0.434862385,-0.433027523,-0.431192661,
-0.429357798,-0.427522936,-0.425688073,-0.423853211,-0.422018349,-0.420183486,
-0.418348624,-0.416513761,-0.414678899,-0.412844037,-0.411009174,-0.409174312,
-0.40733945,-0.405504587,-0.403669725,-0.401834862,-0.4,-0.398165138,-0.396330275,
-0.394495413,-0.39266055,-0.390825688,-0.388990826,-0.387155963,-0.385321101,
-0.383486239,-0.381651376,-0.379816514,-0.377981651,-0.376146789,-0.374311927,
-0.372477064,-0.370642202,-0.368807339,-0.366972477,-0.365137615,-0.363302752,
-0.36146789,-0.359633028,-0.357798165,-0.355963303,-0.35412844,-0.352293578,
-0.350458716,-0.348623853,-0.346788991,-0.344954128,-0.343119266,-0.341284404,
-0.339449541,-0.337614679,-0.335779817,-0.333944954,-0.332110092,-0.330275229,
-0.328440367,-0.326605505,-0.324770642,-0.32293578,-0.321100917,-0.319266055,
-0.317431193,-0.31559633,-0.313761468,-0.311926606,-0.310091743,-0.308256881,
-0.306422018,-0.304587156,-0.302752294,-0.300917431,-0.299082569,-0.297247706,
-0.295412844,-0.293577982,-0.291743119,-0.289908257,-0.288073394,-0.286238532,
-0.28440367,-0.282568807,-0.280733945,-0.278899083,-0.27706422,-0.275229358,
-0.273394495,-0.271559633,-0.269724771,-0.267889908,-0.266055046,-0.264220183,
-0.262385321,-0.260550459,-0.258715596,-0.256880734,-0.255045872,-0.253211009,
-0.251376147,-0.249541284,-0.247706422,-0.24587156,-0.244036697,-0.242201835,
-0.240366972,-0.23853211,-0.236697248,-0.234862385,-0.233027523,-0.231192661,
-0.229357798,-0.227522936,-0.225688073,-0.223853211,-0.222018349,-0.220183486,
-0.218348624,-0.216513761,-0.214678899,-0.212844037,-0.211009174,-0.209174312,
-0.20733945,-0.205504587,-0.203669725,-0.201834862,-0.2,-0.198165138,-0.196330275,
-0.194495413,-0.19266055,-0.190825688,-0.188990826,-0.187155963,-0.185321101,
-0.183486239,-0.181651376,-0.179816514,-0.177981651,-0.176146789,-0.174311927,
-0.172477064,-0.170642202,-0.168807339,-0.166972477,-0.165137615,-0.163302752,
-0.16146789,-0.159633028,-0.157798165,-0.155963303,-0.15412844,-0.152293578,
-0.150458716,-0.148623853,-0.146788991,-0.144954128,-0.143119266,-0.141284404,
-0.139449541,-0.137614679,-0.135779817,-0.133944954,-0.132110092,-0.130275229,
-0.128440367,-0.126605505,-0.124770642,-0.12293578,-0.121100917,-0.119266055,
-0.117431193,-0.11559633,-0.113761468,-0.111926606,-0.110091743,-0.108256881,
-0.106422018,-0.104587156,-0.102752294,-0.100917431,-0.099082569,-0.097247706,
-0.095412844,-0.093577982,-0.091743119,-0.089908257,-0.088073394,-0.086238532,
-0.08440367,-0.082568807,-0.080733945,-0.078899083,-0.07706422,-0.075229358,
-0.073394495,-0.071559633,-0.069724771,-0.067889908,-0.066055046,-0.064220183,
-0.062385321,-0.060550459,-0.058715596,-0.056880734,-0.055045872,-0.053211009,
-0.051376147,-0.049541284,-0.047706422,-0.04587156,-0.044036697,-0.042201835,
-0.040366972,-0.03853211,-0.036697248,-0.034862385,-0.033027523,-0.031192661,
-0.029357798,-0.027522936,-0.025688073,-0.023853211,-0.022018349,-0.020183486,
-0.018348624,-0.016513761,-0.014678899,-0.012844037,-0.011009174,-0.009174312,
-0.00733945,-0.005504587,-0.003669725,-0.001834862,0.000982134),(0.3,1.,
1.3),.UNSPECIFIED.);
#6314=B_SPLINE_SURFACE_WITH_KNOTS('',5,1,((#319684,#319685,#319686),(#319687,
#319688,#319689),(#319690,#319691,#319692),(#319693,#319694,#319695),(#319696,
#319697,#319698),(#319699,#319700,#319701),(#319702,#319703,#319704),(#319705,
#319706,#319707),(#319708,#319709,#319710),(#319711,#319712,#319713),(#319714,
#319715,#319716),(#319717,#319718,#319719),(#319720,#319721,#319722),(#319723,
#319724,#319725),(#319726,#319727,#319728),(#319729,#319730,#319731),(#319732,
#319733,#319734),(#319735,#319736,#319737),(#319738,#319739,#319740),(#319741,
#319742,#319743),(#319744,#319745,#319746),(#319747,#319748,#319749),(#319750,
#319751,#319752),(#319753,#319754,#319755),(#319756,#319757,#319758),(#319759,
#319760,#319761),(#319762,#319763,#319764),(#319765,#319766,#319767),(#319768,
#319769,#319770),(#319771,#319772,#319773),(#319774,#319775,#319776),(#319777,
#319778,#319779),(#319780,#319781,#319782),(#319783,#319784,#319785),(#319786,
#319787,#319788),(#319789,#319790,#319791),(#319792,#319793,#319794),(#319795,
#319796,#319797),(#319798,#319799,#319800),(#319801,#319802,#319803),(#319804,
#319805,#319806),(#319807,#319808,#319809),(#319810,#319811,#319812),(#319813,
#319814,#319815),(#319816,#319817,#319818),(#319819,#319820,#319821),(#319822,
#319823,#319824),(#319825,#319826,#319827),(#319828,#319829,#319830),(#319831,
#319832,#319833),(#319834,#319835,#319836),(#319837,#319838,#319839),(#319840,
#319841,#319842),(#319843,#319844,#319845),(#319846,#319847,#319848),(#319849,
#319850,#319851),(#319852,#319853,#319854),(#319855,#319856,#319857),(#319858,
#319859,#319860),(#319861,#319862,#319863),(#319864,#319865,#319866),(#319867,
#319868,#319869),(#319870,#319871,#319872),(#319873,#319874,#319875),(#319876,
#319877,#319878),(#319879,#319880,#319881),(#319882,#319883,#319884),(#319885,
#319886,#319887),(#319888,#319889,#319890),(#319891,#319892,#319893),(#319894,
#319895,#319896),(#319897,#319898,#319899),(#319900,#319901,#319902),(#319903,
#319904,#319905),(#319906,#319907,#319908),(#319909,#319910,#319911),(#319912,
#319913,#319914),(#319915,#319916,#319917),(#319918,#319919,#319920),(#319921,
#319922,#319923),(#319924,#319925,#319926),(#319927,#319928,#319929),(#319930,
#319931,#319932),(#319933,#319934,#319935),(#319936,#319937,#319938),(#319939,
#319940,#319941),(#319942,#319943,#319944),(#319945,#319946,#319947),(#319948,
#319949,#319950),(#319951,#319952,#319953),(#319954,#319955,#319956),(#319957,
#319958,#319959),(#319960,#319961,#319962),(#319963,#319964,#319965),(#319966,
#319967,#319968),(#319969,#319970,#319971),(#319972,#319973,#319974),(#319975,
#319976,#319977),(#319978,#319979,#319980),(#319981,#319982,#319983),(#319984,
#319985,#319986),(#319987,#319988,#319989),(#319990,#319991,#319992),(#319993,
#319994,#319995),(#319996,#319997,#319998),(#319999,#320000,#320001),(#320002,
#320003,#320004),(#320005,#320006,#320007),(#320008,#320009,#320010),(#320011,
#320012,#320013),(#320014,#320015,#320016),(#320017,#320018,#320019),(#320020,
#320021,#320022),(#320023,#320024,#320025),(#320026,#320027,#320028),(#320029,
#320030,#320031),(#320032,#320033,#320034),(#320035,#320036,#320037),(#320038,
#320039,#320040),(#320041,#320042,#320043),(#320044,#320045,#320046),(#320047,
#320048,#320049),(#320050,#320051,#320052),(#320053,#320054,#320055),(#320056,
#320057,#320058),(#320059,#320060,#320061),(#320062,#320063,#320064),(#320065,
#320066,#320067),(#320068,#320069,#320070),(#320071,#320072,#320073),(#320074,
#320075,#320076),(#320077,#320078,#320079),(#320080,#320081,#320082),(#320083,
#320084,#320085),(#320086,#320087,#320088),(#320089,#320090,#320091),(#320092,
#320093,#320094),(#320095,#320096,#320097),(#320098,#320099,#320100),(#320101,
#320102,#320103),(#320104,#320105,#320106),(#320107,#320108,#320109),(#320110,
#320111,#320112),(#320113,#320114,#320115),(#320116,#320117,#320118),(#320119,
#320120,#320121),(#320122,#320123,#320124),(#320125,#320126,#320127),(#320128,
#320129,#320130),(#320131,#320132,#320133),(#320134,#320135,#320136),(#320137,
#320138,#320139),(#320140,#320141,#320142),(#320143,#320144,#320145),(#320146,
#320147,#320148),(#320149,#320150,#320151),(#320152,#320153,#320154),(#320155,
#320156,#320157),(#320158,#320159,#320160),(#320161,#320162,#320163),(#320164,
#320165,#320166),(#320167,#320168,#320169),(#320170,#320171,#320172),(#320173,
#320174,#320175),(#320176,#320177,#320178),(#320179,#320180,#320181),(#320182,
#320183,#320184),(#320185,#320186,#320187),(#320188,#320189,#320190),(#320191,
#320192,#320193),(#320194,#320195,#320196),(#320197,#320198,#320199),(#320200,
#320201,#320202),(#320203,#320204,#320205),(#320206,#320207,#320208),(#320209,
#320210,#320211),(#320212,#320213,#320214),(#320215,#320216,#320217),(#320218,
#320219,#320220),(#320221,#320222,#320223),(#320224,#320225,#320226),(#320227,
#320228,#320229),(#320230,#320231,#320232),(#320233,#320234,#320235),(#320236,
#320237,#320238),(#320239,#320240,#320241),(#320242,#320243,#320244),(#320245,
#320246,#320247),(#320248,#320249,#320250),(#320251,#320252,#320253),(#320254,
#320255,#320256),(#320257,#320258,#320259),(#320260,#320261,#320262),(#320263,
#320264,#320265),(#320266,#320267,#320268),(#320269,#320270,#320271),(#320272,
#320273,#320274),(#320275,#320276,#320277),(#320278,#320279,#320280),(#320281,
#320282,#320283),(#320284,#320285,#320286),(#320287,#320288,#320289),(#320290,
#320291,#320292),(#320293,#320294,#320295),(#320296,#320297,#320298),(#320299,
#320300,#320301),(#320302,#320303,#320304),(#320305,#320306,#320307),(#320308,
#320309,#320310),(#320311,#320312,#320313),(#320314,#320315,#320316),(#320317,
#320318,#320319),(#320320,#320321,#320322),(#320323,#320324,#320325),(#320326,
#320327,#320328),(#320329,#320330,#320331),(#320332,#320333,#320334),(#320335,
#320336,#320337),(#320338,#320339,#320340),(#320341,#320342,#320343),(#320344,
#320345,#320346),(#320347,#320348,#320349),(#320350,#320351,#320352),(#320353,
#320354,#320355),(#320356,#320357,#320358),(#320359,#320360,#320361),(#320362,
#320363,#320364),(#320365,#320366,#320367),(#320368,#320369,#320370),(#320371,
#320372,#320373),(#320374,#320375,#320376),(#320377,#320378,#320379),(#320380,
#320381,#320382),(#320383,#320384,#320385),(#320386,#320387,#320388),(#320389,
#320390,#320391),(#320392,#320393,#320394),(#320395,#320396,#320397),(#320398,
#320399,#320400),(#320401,#320402,#320403),(#320404,#320405,#320406),(#320407,
#320408,#320409),(#320410,#320411,#320412),(#320413,#320414,#320415),(#320416,
#320417,#320418),(#320419,#320420,#320421),(#320422,#320423,#320424),(#320425,
#320426,#320427),(#320428,#320429,#320430),(#320431,#320432,#320433),(#320434,
#320435,#320436),(#320437,#320438,#320439),(#320440,#320441,#320442),(#320443,
#320444,#320445),(#320446,#320447,#320448),(#320449,#320450,#320451),(#320452,
#320453,#320454),(#320455,#320456,#320457),(#320458,#320459,#320460),(#320461,
#320462,#320463),(#320464,#320465,#320466),(#320467,#320468,#320469),(#320470,
#320471,#320472),(#320473,#320474,#320475),(#320476,#320477,#320478),(#320479,
#320480,#320481),(#320482,#320483,#320484),(#320485,#320486,#320487),(#320488,
#320489,#320490),(#320491,#320492,#320493),(#320494,#320495,#320496),(#320497,
#320498,#320499),(#320500,#320501,#320502),(#320503,#320504,#320505),(#320506,
#320507,#320508),(#320509,#320510,#320511),(#320512,#320513,#320514),(#320515,
#320516,#320517),(#320518,#320519,#320520),(#320521,#320522,#320523),(#320524,
#320525,#320526),(#320527,#320528,#320529),(#320530,#320531,#320532),(#320533,
#320534,#320535),(#320536,#320537,#320538),(#320539,#320540,#320541),(#320542,
#320543,#320544),(#320545,#320546,#320547),(#320548,#320549,#320550),(#320551,
#320552,#320553),(#320554,#320555,#320556),(#320557,#320558,#320559),(#320560,
#320561,#320562),(#320563,#320564,#320565),(#320566,#320567,#320568),(#320569,
#320570,#320571),(#320572,#320573,#320574),(#320575,#320576,#320577),(#320578,
#320579,#320580),(#320581,#320582,#320583),(#320584,#320585,#320586),(#320587,
#320588,#320589),(#320590,#320591,#320592),(#320593,#320594,#320595),(#320596,
#320597,#320598),(#320599,#320600,#320601),(#320602,#320603,#320604),(#320605,
#320606,#320607),(#320608,#320609,#320610),(#320611,#320612,#320613),(#320614,
#320615,#320616),(#320617,#320618,#320619),(#320620,#320621,#320622),(#320623,
#320624,#320625),(#320626,#320627,#320628),(#320629,#320630,#320631),(#320632,
#320633,#320634),(#320635,#320636,#320637),(#320638,#320639,#320640),(#320641,
#320642,#320643),(#320644,#320645,#320646),(#320647,#320648,#320649),(#320650,
#320651,#320652),(#320653,#320654,#320655),(#320656,#320657,#320658),(#320659,
#320660,#320661),(#320662,#320663,#320664),(#320665,#320666,#320667),(#320668,
#320669,#320670),(#320671,#320672,#320673),(#320674,#320675,#320676),(#320677,
#320678,#320679),(#320680,#320681,#320682),(#320683,#320684,#320685),(#320686,
#320687,#320688),(#320689,#320690,#320691),(#320692,#320693,#320694),(#320695,
#320696,#320697),(#320698,#320699,#320700),(#320701,#320702,#320703),(#320704,
#320705,#320706),(#320707,#320708,#320709),(#320710,#320711,#320712),(#320713,
#320714,#320715),(#320716,#320717,#320718),(#320719,#320720,#320721),(#320722,
#320723,#320724),(#320725,#320726,#320727),(#320728,#320729,#320730),(#320731,
#320732,#320733),(#320734,#320735,#320736),(#320737,#320738,#320739),(#320740,
#320741,#320742),(#320743,#320744,#320745),(#320746,#320747,#320748),(#320749,
#320750,#320751),(#320752,#320753,#320754),(#320755,#320756,#320757),(#320758,
#320759,#320760),(#320761,#320762,#320763),(#320764,#320765,#320766),(#320767,
#320768,#320769),(#320770,#320771,#320772),(#320773,#320774,#320775),(#320776,
#320777,#320778),(#320779,#320780,#320781),(#320782,#320783,#320784),(#320785,
#320786,#320787),(#320788,#320789,#320790),(#320791,#320792,#320793),(#320794,
#320795,#320796),(#320797,#320798,#320799),(#320800,#320801,#320802),(#320803,
#320804,#320805),(#320806,#320807,#320808),(#320809,#320810,#320811),(#320812,
#320813,#320814),(#320815,#320816,#320817),(#320818,#320819,#320820),(#320821,
#320822,#320823),(#320824,#320825,#320826),(#320827,#320828,#320829),(#320830,
#320831,#320832),(#320833,#320834,#320835),(#320836,#320837,#320838),(#320839,
#320840,#320841),(#320842,#320843,#320844),(#320845,#320846,#320847),(#320848,
#320849,#320850),(#320851,#320852,#320853),(#320854,#320855,#320856),(#320857,
#320858,#320859),(#320860,#320861,#320862),(#320863,#320864,#320865),(#320866,
#320867,#320868),(#320869,#320870,#320871),(#320872,#320873,#320874),(#320875,
#320876,#320877),(#320878,#320879,#320880),(#320881,#320882,#320883),(#320884,
#320885,#320886),(#320887,#320888,#320889),(#320890,#320891,#320892),(#320893,
#320894,#320895),(#320896,#320897,#320898),(#320899,#320900,#320901),(#320902,
#320903,#320904),(#320905,#320906,#320907),(#320908,#320909,#320910),(#320911,
#320912,#320913),(#320914,#320915,#320916),(#320917,#320918,#320919),(#320920,
#320921,#320922),(#320923,#320924,#320925),(#320926,#320927,#320928),(#320929,
#320930,#320931),(#320932,#320933,#320934),(#320935,#320936,#320937),(#320938,
#320939,#320940),(#320941,#320942,#320943),(#320944,#320945,#320946),(#320947,
#320948,#320949),(#320950,#320951,#320952),(#320953,#320954,#320955),(#320956,
#320957,#320958),(#320959,#320960,#320961),(#320962,#320963,#320964),(#320965,
#320966,#320967),(#320968,#320969,#320970),(#320971,#320972,#320973),(#320974,
#320975,#320976),(#320977,#320978,#320979),(#320980,#320981,#320982),(#320983,
#320984,#320985),(#320986,#320987,#320988),(#320989,#320990,#320991),(#320992,
#320993,#320994),(#320995,#320996,#320997),(#320998,#320999,#321000),(#321001,
#321002,#321003),(#321004,#321005,#321006),(#321007,#321008,#321009),(#321010,
#321011,#321012),(#321013,#321014,#321015),(#321016,#321017,#321018),(#321019,
#321020,#321021),(#321022,#321023,#321024),(#321025,#321026,#321027),(#321028,
#321029,#321030),(#321031,#321032,#321033),(#321034,#321035,#321036),(#321037,
#321038,#321039),(#321040,#321041,#321042),(#321043,#321044,#321045),(#321046,
#321047,#321048),(#321049,#321050,#321051),(#321052,#321053,#321054),(#321055,
#321056,#321057),(#321058,#321059,#321060),(#321061,#321062,#321063),(#321064,
#321065,#321066),(#321067,#321068,#321069),(#321070,#321071,#321072),(#321073,
#321074,#321075),(#321076,#321077,#321078),(#321079,#321080,#321081),(#321082,
#321083,#321084),(#321085,#321086,#321087),(#321088,#321089,#321090),(#321091,
#321092,#321093),(#321094,#321095,#321096),(#321097,#321098,#321099),(#321100,
#321101,#321102),(#321103,#321104,#321105),(#321106,#321107,#321108),(#321109,
#321110,#321111),(#321112,#321113,#321114),(#321115,#321116,#321117),(#321118,
#321119,#321120),(#321121,#321122,#321123),(#321124,#321125,#321126),(#321127,
#321128,#321129),(#321130,#321131,#321132),(#321133,#321134,#321135),(#321136,
#321137,#321138),(#321139,#321140,#321141),(#321142,#321143,#321144),(#321145,
#321146,#321147),(#321148,#321149,#321150),(#321151,#321152,#321153),(#321154,
#321155,#321156),(#321157,#321158,#321159),(#321160,#321161,#321162),(#321163,
#321164,#321165),(#321166,#321167,#321168),(#321169,#321170,#321171),(#321172,
#321173,#321174),(#321175,#321176,#321177),(#321178,#321179,#321180),(#321181,
#321182,#321183),(#321184,#321185,#321186),(#321187,#321188,#321189),(#321190,
#321191,#321192),(#321193,#321194,#321195),(#321196,#321197,#321198),(#321199,
#321200,#321201),(#321202,#321203,#321204),(#321205,#321206,#321207),(#321208,
#321209,#321210),(#321211,#321212,#321213),(#321214,#321215,#321216),(#321217,
#321218,#321219),(#321220,#321221,#321222),(#321223,#321224,#321225),(#321226,
#321227,#321228),(#321229,#321230,#321231),(#321232,#321233,#321234),(#321235,
#321236,#321237),(#321238,#321239,#321240),(#321241,#321242,#321243),(#321244,
#321245,#321246),(#321247,#321248,#321249),(#321250,#321251,#321252),(#321253,
#321254,#321255),(#321256,#321257,#321258),(#321259,#321260,#321261),(#321262,
#321263,#321264),(#321265,#321266,#321267),(#321268,#321269,#321270),(#321271,
#321272,#321273),(#321274,#321275,#321276),(#321277,#321278,#321279),(#321280,
#321281,#321282),(#321283,#321284,#321285),(#321286,#321287,#321288),(#321289,
#321290,#321291),(#321292,#321293,#321294),(#321295,#321296,#321297),(#321298,
#321299,#321300),(#321301,#321302,#321303),(#321304,#321305,#321306),(#321307,
#321308,#321309),(#321310,#321311,#321312),(#321313,#321314,#321315),(#321316,
#321317,#321318),(#321319,#321320,#321321),(#321322,#321323,#321324),(#321325,
#321326,#321327),(#321328,#321329,#321330),(#321331,#321332,#321333),(#321334,
#321335,#321336)),.UNSPECIFIED.,.F.,.F.,.F.,(6,1,1,1,1,1,1,1,1,1,1,1,1,
1,1,1,1,1,1,1,1,1,1,1,1,1,1,1,1,1,1,1,1,1,1,1,1,1,1,1,1,1,1,1,1,1,1,1,1,
1,1,1,1,1,1,1,1,1,1,1,1,1,1,1,1,1,1,1,1,1,1,1,1,1,1,1,1,1,1,1,1,1,1,1,1,
1,1,1,1,1,1,1,1,1,1,1,1,1,1,1,1,1,1,1,1,1,1,1,1,1,1,1,1,1,1,1,1,1,1,1,1,
1,1,1,1,1,1,1,1,1,1,1,1,1,1,1,1,1,1,1,1,1,1,1,1,1,1,1,1,1,1,1,1,1,1,1,1,
1,1,1,1,1,1,1,1,1,1,1,1,1,1,1,1,1,1,1,1,1,1,1,1,1,1,1,1,1,1,1,1,1,1,1,1,
1,1,1,1,1,1,1,1,1,1,1,1,1,1,1,1,1,1,1,1,1,1,1,1,1,1,1,1,1,1,1,1,1,1,1,1,
1,1,1,1,1,1,1,1,1,1,1,1,1,1,1,1,1,1,1,1,1,1,1,1,1,1,1,1,1,1,1,1,1,1,1,1,
1,1,1,1,1,1,1,1,1,1,1,1,1,1,1,1,1,1,1,1,1,1,1,1,1,1,1,1,1,1,1,1,1,1,1,1,
1,1,1,1,1,1,1,1,1,1,1,1,1,1,1,1,1,1,1,1,1,1,1,1,1,1,1,1,1,1,1,1,1,1,1,1,
1,1,1,1,1,1,1,1,1,1,1,1,1,1,1,1,1,1,1,1,1,1,1,1,1,1,1,1,1,1,1,1,1,1,1,1,
1,1,1,1,1,1,1,1,1,1,1,1,1,1,1,1,1,1,1,1,1,1,1,1,1,1,1,1,1,1,1,1,1,1,1,1,
1,1,1,1,1,1,1,1,1,1,1,1,1,1,1,1,1,1,1,1,1,1,1,1,1,1,1,1,1,1,1,1,1,1,1,1,
1,1,1,1,1,1,1,1,1,1,1,1,1,1,1,1,1,1,1,1,1,1,1,1,1,1,1,1,1,1,1,1,1,1,1,1,
1,1,1,1,1,1,1,1,1,1,1,1,1,1,1,1,1,1,1,1,1,1,1,1,1,1,1,1,1,1,1,1,1,1,1,1,
1,1,1,1,1,1,1,1,1,1,1,1,1,1,1,1,1,1,1,1,1,1,1,1,1,1,1,1,1,6),(2,1,2),(-0.00196418,
0.,0.001834862,0.003669725,0.005504587,0.00733945,0.009174312,0.011009174,
0.012844037,0.014678899,0.016513761,0.018348624,0.020183486,0.022018349,
0.023853211,0.025688073,0.027522936,0.029357798,0.031192661,0.033027523,
0.034862385,0.036697248,0.03853211,0.040366972,0.042201835,0.044036697,
0.04587156,0.047706422,0.049541284,0.051376147,0.053211009,0.055045872,
0.056880734,0.058715596,0.060550459,0.062385321,0.064220183,0.066055046,
0.067889908,0.069724771,0.071559633,0.073394495,0.075229358,0.07706422,
0.078899083,0.080733945,0.082568807,0.08440367,0.086238532,0.088073394,
0.089908257,0.091743119,0.093577982,0.095412844,0.097247706,0.099082569,
0.100917431,0.102752294,0.104587156,0.106422018,0.108256881,0.110091743,
0.111926606,0.113761468,0.11559633,0.117431193,0.119266055,0.121100917,
0.12293578,0.124770642,0.126605505,0.128440367,0.130275229,0.132110092,
0.133944954,0.135779817,0.137614679,0.139449541,0.141284404,0.143119266,
0.144954128,0.146788991,0.148623853,0.150458716,0.152293578,0.15412844,
0.155963303,0.157798165,0.159633028,0.16146789,0.163302752,0.165137615,
0.166972477,0.168807339,0.170642202,0.172477064,0.174311927,0.176146789,
0.177981651,0.179816514,0.181651376,0.183486239,0.185321101,0.187155963,
0.188990826,0.190825688,0.19266055,0.194495413,0.196330275,0.198165138,
0.2,0.201834862,0.203669725,0.205504587,0.20733945,0.209174312,0.211009174,
0.212844037,0.214678899,0.216513761,0.218348624,0.220183486,0.222018349,
0.223853211,0.225688073,0.227522936,0.229357798,0.231192661,0.233027523,
0.234862385,0.236697248,0.23853211,0.240366972,0.242201835,0.244036697,
0.24587156,0.247706422,0.249541284,0.251376147,0.253211009,0.255045872,
0.256880734,0.258715596,0.260550459,0.262385321,0.264220183,0.266055046,
0.267889908,0.269724771,0.271559633,0.273394495,0.275229358,0.27706422,
0.278899083,0.280733945,0.282568807,0.28440367,0.286238532,0.288073394,
0.289908257,0.291743119,0.293577982,0.295412844,0.297247706,0.299082569,
0.300917431,0.302752294,0.304587156,0.306422018,0.308256881,0.310091743,
0.311926606,0.313761468,0.31559633,0.317431193,0.319266055,0.321100917,
0.32293578,0.324770642,0.326605505,0.328440367,0.330275229,0.332110092,
0.333944954,0.335779817,0.337614679,0.339449541,0.341284404,0.343119266,
0.344954128,0.346788991,0.348623853,0.350458716,0.352293578,0.35412844,
0.355963303,0.357798165,0.359633028,0.36146789,0.363302752,0.365137615,
0.366972477,0.368807339,0.370642202,0.372477064,0.374311927,0.376146789,
0.377981651,0.379816514,0.381651376,0.383486239,0.385321101,0.387155963,
0.388990826,0.390825688,0.39266055,0.394495413,0.396330275,0.398165138,
0.4,0.401834862,0.403669725,0.405504587,0.40733945,0.409174312,0.411009174,
0.412844037,0.414678899,0.416513761,0.418348624,0.420183486,0.422018349,
0.423853211,0.425688073,0.427522936,0.429357798,0.431192661,0.433027523,
0.434862385,0.436697248,0.43853211,0.440366972,0.442201835,0.444036697,
0.44587156,0.447706422,0.449541284,0.451376147,0.453211009,0.455045872,
0.456880734,0.458715596,0.460550459,0.462385321,0.464220183,0.466055046,
0.467889908,0.469724771,0.471559633,0.473394495,0.475229358,0.47706422,
0.478899083,0.480733945,0.482568807,0.48440367,0.486238532,0.488073394,
0.489908257,0.491743119,0.493577982,0.495412844,0.497247706,0.499082569,
0.500917431,0.502752294,0.504587156,0.506422018,0.508256881,0.510091743,
0.511926606,0.513761468,0.51559633,0.517431193,0.519266055,0.521100917,
0.52293578,0.524770642,0.526605505,0.528440367,0.530275229,0.532110092,
0.533944954,0.535779817,0.537614679,0.539449541,0.541284404,0.543119266,
0.544954128,0.546788991,0.548623853,0.550458716,0.552293578,0.55412844,
0.555963303,0.557798165,0.559633028,0.56146789,0.563302752,0.565137615,
0.566972477,0.568807339,0.570642202,0.572477064,0.574311927,0.576146789,
0.577981651,0.579816514,0.581651376,0.583486239,0.585321101,0.587155963,
0.588990826,0.590825688,0.59266055,0.594495413,0.596330275,0.598165138,
0.6,0.601834862,0.603669725,0.605504587,0.60733945,0.609174312,0.611009174,
0.612844037,0.614678899,0.616513761,0.618348624,0.620183486,0.622018349,
0.623853211,0.625688073,0.627522936,0.629357798,0.631192661,0.633027523,
0.634862385,0.636697248,0.63853211,0.640366972,0.642201835,0.644036697,
0.64587156,0.647706422,0.649541284,0.651376147,0.653211009,0.655045872,
0.656880734,0.658715596,0.660550459,0.662385321,0.664220183,0.666055046,
0.667889908,0.669724771,0.671559633,0.673394495,0.675229358,0.67706422,
0.678899083,0.680733945,0.682568807,0.68440367,0.686238532,0.688073394,
0.689908257,0.691743119,0.693577982,0.695412844,0.697247706,0.699082569,
0.700917431,0.702752294,0.704587156,0.706422018,0.708256881,0.710091743,
0.711926606,0.713761468,0.71559633,0.717431193,0.719266055,0.721100917,
0.72293578,0.724770642,0.726605505,0.728440367,0.730275229,0.732110092,
0.733944954,0.735779817,0.737614679,0.739449541,0.741284404,0.743119266,
0.744954128,0.746788991,0.748623853,0.750458716,0.752293578,0.75412844,
0.755963303,0.757798165,0.759633028,0.76146789,0.763302752,0.765137615,
0.766972477,0.768807339,0.770642202,0.772477064,0.774311927,0.776146789,
0.777981651,0.779816514,0.781651376,0.783486239,0.785321101,0.787155963,
0.788990826,0.790825688,0.79266055,0.794495413,0.796330275,0.798165138,
0.8,0.801834862,0.803669725,0.805504587,0.80733945,0.809174312,0.811009174,
0.812844037,0.814678899,0.816513761,0.818348624,0.820183486,0.822018349,
0.823853211,0.825688073,0.827522936,0.829357798,0.831192661,0.833027523,
0.834862385,0.836697248,0.83853211,0.840366972,0.842201835,0.844036697,
0.84587156,0.847706422,0.849541284,0.851376147,0.853211009,0.855045872,
0.856880734,0.858715596,0.860550459,0.862385321,0.864220183,0.866055046,
0.867889908,0.869724771,0.871559633,0.873394495,0.875229358,0.87706422,
0.878899083,0.880733945,0.882568807,0.88440367,0.886238532,0.888073394,
0.889908257,0.891743119,0.893577982,0.895412844,0.897247706,0.899082569,
0.900917431,0.902752294,0.904587156,0.906422018,0.908256881,0.910091743,
0.911926606,0.913761468,0.91559633,0.917431193,0.919266055,0.921100917,
0.92293578,0.924770642,0.926605505,0.928440367,0.930275229,0.932110092,
0.933944954,0.935779817,0.937614679,0.939449541,0.941284404,0.943119266,
0.944954128,0.946788991,0.948623853,0.950458716,0.952293578,0.95412844,
0.955963303,0.957798165,0.959633028,0.96146789,0.963302752,0.965137615,
0.966972477,0.968807339,0.970642202,0.972477064,0.974311927,0.976146789,
0.977981651,0.979816514,0.981651376,0.983486239,0.985321101,0.987155963,
0.988990826,0.990825688,0.99266055,0.994495413,0.996330275,0.998165138,
1.),(0.3,1.,1.3),.UNSPECIFIED.);
#6315=B_SPLINE_SURFACE_WITH_KNOTS('',5,1,((#321359,#321360,#321361),(#321362,
#321363,#321364),(#321365,#321366,#321367),(#321368,#321369,#321370),(#321371,
#321372,#321373),(#321374,#321375,#321376),(#321377,#321378,#321379),(#321380,
#321381,#321382),(#321383,#321384,#321385),(#321386,#321387,#321388),(#321389,
#321390,#321391),(#321392,#321393,#321394),(#321395,#321396,#321397),(#321398,
#321399,#321400),(#321401,#321402,#321403),(#321404,#321405,#321406),(#321407,
#321408,#321409),(#321410,#321411,#321412),(#321413,#321414,#321415),(#321416,
#321417,#321418),(#321419,#321420,#321421),(#321422,#321423,#321424),(#321425,
#321426,#321427),(#321428,#321429,#321430),(#321431,#321432,#321433),(#321434,
#321435,#321436),(#321437,#321438,#321439),(#321440,#321441,#321442),(#321443,
#321444,#321445),(#321446,#321447,#321448),(#321449,#321450,#321451),(#321452,
#321453,#321454),(#321455,#321456,#321457),(#321458,#321459,#321460),(#321461,
#321462,#321463),(#321464,#321465,#321466),(#321467,#321468,#321469),(#321470,
#321471,#321472),(#321473,#321474,#321475),(#321476,#321477,#321478),(#321479,
#321480,#321481),(#321482,#321483,#321484),(#321485,#321486,#321487),(#321488,
#321489,#321490),(#321491,#321492,#321493),(#321494,#321495,#321496),(#321497,
#321498,#321499),(#321500,#321501,#321502),(#321503,#321504,#321505),(#321506,
#321507,#321508),(#321509,#321510,#321511),(#321512,#321513,#321514),(#321515,
#321516,#321517),(#321518,#321519,#321520),(#321521,#321522,#321523),(#321524,
#321525,#321526),(#321527,#321528,#321529),(#321530,#321531,#321532),(#321533,
#321534,#321535),(#321536,#321537,#321538),(#321539,#321540,#321541),(#321542,
#321543,#321544),(#321545,#321546,#321547),(#321548,#321549,#321550),(#321551,
#321552,#321553),(#321554,#321555,#321556),(#321557,#321558,#321559),(#321560,
#321561,#321562),(#321563,#321564,#321565),(#321566,#321567,#321568),(#321569,
#321570,#321571),(#321572,#321573,#321574),(#321575,#321576,#321577),(#321578,
#321579,#321580),(#321581,#321582,#321583),(#321584,#321585,#321586),(#321587,
#321588,#321589),(#321590,#321591,#321592),(#321593,#321594,#321595),(#321596,
#321597,#321598),(#321599,#321600,#321601),(#321602,#321603,#321604),(#321605,
#321606,#321607),(#321608,#321609,#321610),(#321611,#321612,#321613),(#321614,
#321615,#321616),(#321617,#321618,#321619),(#321620,#321621,#321622),(#321623,
#321624,#321625),(#321626,#321627,#321628),(#321629,#321630,#321631),(#321632,
#321633,#321634),(#321635,#321636,#321637),(#321638,#321639,#321640),(#321641,
#321642,#321643),(#321644,#321645,#321646),(#321647,#321648,#321649),(#321650,
#321651,#321652),(#321653,#321654,#321655),(#321656,#321657,#321658),(#321659,
#321660,#321661),(#321662,#321663,#321664),(#321665,#321666,#321667),(#321668,
#321669,#321670),(#321671,#321672,#321673),(#321674,#321675,#321676),(#321677,
#321678,#321679),(#321680,#321681,#321682),(#321683,#321684,#321685),(#321686,
#321687,#321688),(#321689,#321690,#321691),(#321692,#321693,#321694),(#321695,
#321696,#321697),(#321698,#321699,#321700),(#321701,#321702,#321703),(#321704,
#321705,#321706),(#321707,#321708,#321709),(#321710,#321711,#321712),(#321713,
#321714,#321715),(#321716,#321717,#321718),(#321719,#321720,#321721),(#321722,
#321723,#321724),(#321725,#321726,#321727),(#321728,#321729,#321730),(#321731,
#321732,#321733),(#321734,#321735,#321736),(#321737,#321738,#321739),(#321740,
#321741,#321742),(#321743,#321744,#321745),(#321746,#321747,#321748),(#321749,
#321750,#321751),(#321752,#321753,#321754),(#321755,#321756,#321757),(#321758,
#321759,#321760),(#321761,#321762,#321763),(#321764,#321765,#321766),(#321767,
#321768,#321769),(#321770,#321771,#321772),(#321773,#321774,#321775),(#321776,
#321777,#321778),(#321779,#321780,#321781),(#321782,#321783,#321784),(#321785,
#321786,#321787),(#321788,#321789,#321790),(#321791,#321792,#321793),(#321794,
#321795,#321796),(#321797,#321798,#321799),(#321800,#321801,#321802),(#321803,
#321804,#321805),(#321806,#321807,#321808),(#321809,#321810,#321811),(#321812,
#321813,#321814),(#321815,#321816,#321817),(#321818,#321819,#321820),(#321821,
#321822,#321823),(#321824,#321825,#321826),(#321827,#321828,#321829),(#321830,
#321831,#321832),(#321833,#321834,#321835),(#321836,#321837,#321838),(#321839,
#321840,#321841),(#321842,#321843,#321844),(#321845,#321846,#321847),(#321848,
#321849,#321850),(#321851,#321852,#321853),(#321854,#321855,#321856),(#321857,
#321858,#321859),(#321860,#321861,#321862),(#321863,#321864,#321865),(#321866,
#321867,#321868),(#321869,#321870,#321871),(#321872,#321873,#321874),(#321875,
#321876,#321877),(#321878,#321879,#321880),(#321881,#321882,#321883),(#321884,
#321885,#321886),(#321887,#321888,#321889),(#321890,#321891,#321892),(#321893,
#321894,#321895),(#321896,#321897,#321898),(#321899,#321900,#321901),(#321902,
#321903,#321904),(#321905,#321906,#321907),(#321908,#321909,#321910),(#321911,
#321912,#321913),(#321914,#321915,#321916),(#321917,#321918,#321919),(#321920,
#321921,#321922),(#321923,#321924,#321925),(#321926,#321927,#321928),(#321929,
#321930,#321931),(#321932,#321933,#321934),(#321935,#321936,#321937),(#321938,
#321939,#321940),(#321941,#321942,#321943),(#321944,#321945,#321946),(#321947,
#321948,#321949),(#321950,#321951,#321952),(#321953,#321954,#321955),(#321956,
#321957,#321958),(#321959,#321960,#321961),(#321962,#321963,#321964),(#321965,
#321966,#321967),(#321968,#321969,#321970),(#321971,#321972,#321973),(#321974,
#321975,#321976),(#321977,#321978,#321979),(#321980,#321981,#321982),(#321983,
#321984,#321985),(#321986,#321987,#321988),(#321989,#321990,#321991),(#321992,
#321993,#321994),(#321995,#321996,#321997),(#321998,#321999,#322000),(#322001,
#322002,#322003),(#322004,#322005,#322006),(#322007,#322008,#322009),(#322010,
#322011,#322012),(#322013,#322014,#322015),(#322016,#322017,#322018),(#322019,
#322020,#322021),(#322022,#322023,#322024),(#322025,#322026,#322027),(#322028,
#322029,#322030),(#322031,#322032,#322033),(#322034,#322035,#322036),(#322037,
#322038,#322039),(#322040,#322041,#322042),(#322043,#322044,#322045),(#322046,
#322047,#322048),(#322049,#322050,#322051),(#322052,#322053,#322054),(#322055,
#322056,#322057),(#322058,#322059,#322060),(#322061,#322062,#322063),(#322064,
#322065,#322066),(#322067,#322068,#322069),(#322070,#322071,#322072),(#322073,
#322074,#322075),(#322076,#322077,#322078),(#322079,#322080,#322081),(#322082,
#322083,#322084),(#322085,#322086,#322087),(#322088,#322089,#322090),(#322091,
#322092,#322093),(#322094,#322095,#322096),(#322097,#322098,#322099),(#322100,
#322101,#322102),(#322103,#322104,#322105),(#322106,#322107,#322108),(#322109,
#322110,#322111),(#322112,#322113,#322114),(#322115,#322116,#322117),(#322118,
#322119,#322120),(#322121,#322122,#322123),(#322124,#322125,#322126),(#322127,
#322128,#322129),(#322130,#322131,#322132),(#322133,#322134,#322135),(#322136,
#322137,#322138),(#322139,#322140,#322141),(#322142,#322143,#322144),(#322145,
#322146,#322147),(#322148,#322149,#322150),(#322151,#322152,#322153),(#322154,
#322155,#322156),(#322157,#322158,#322159),(#322160,#322161,#322162),(#322163,
#322164,#322165),(#322166,#322167,#322168),(#322169,#322170,#322171),(#322172,
#322173,#322174),(#322175,#322176,#322177),(#322178,#322179,#322180),(#322181,
#322182,#322183),(#322184,#322185,#322186),(#322187,#322188,#322189),(#322190,
#322191,#322192),(#322193,#322194,#322195),(#322196,#322197,#322198),(#322199,
#322200,#322201),(#322202,#322203,#322204),(#322205,#322206,#322207),(#322208,
#322209,#322210),(#322211,#322212,#322213),(#322214,#322215,#322216),(#322217,
#322218,#322219),(#322220,#322221,#322222),(#322223,#322224,#322225),(#322226,
#322227,#322228),(#322229,#322230,#322231),(#322232,#322233,#322234),(#322235,
#322236,#322237),(#322238,#322239,#322240),(#322241,#322242,#322243),(#322244,
#322245,#322246),(#322247,#322248,#322249),(#322250,#322251,#322252),(#322253,
#322254,#322255),(#322256,#322257,#322258),(#322259,#322260,#322261),(#322262,
#322263,#322264),(#322265,#322266,#322267),(#322268,#322269,#322270),(#322271,
#322272,#322273),(#322274,#322275,#322276),(#322277,#322278,#322279),(#322280,
#322281,#322282),(#322283,#322284,#322285),(#322286,#322287,#322288),(#322289,
#322290,#322291),(#322292,#322293,#322294),(#322295,#322296,#322297),(#322298,
#322299,#322300),(#322301,#322302,#322303),(#322304,#322305,#322306),(#322307,
#322308,#322309),(#322310,#322311,#322312),(#322313,#322314,#322315),(#322316,
#322317,#322318),(#322319,#322320,#322321),(#322322,#322323,#322324),(#322325,
#322326,#322327),(#322328,#322329,#322330),(#322331,#322332,#322333),(#322334,
#322335,#322336),(#322337,#322338,#322339),(#322340,#322341,#322342),(#322343,
#322344,#322345),(#322346,#322347,#322348),(#322349,#322350,#322351),(#322352,
#322353,#322354),(#322355,#322356,#322357),(#322358,#322359,#322360),(#322361,
#322362,#322363),(#322364,#322365,#322366),(#322367,#322368,#322369),(#322370,
#322371,#322372),(#322373,#322374,#322375),(#322376,#322377,#322378),(#322379,
#322380,#322381),(#322382,#322383,#322384),(#322385,#322386,#322387),(#322388,
#322389,#322390),(#322391,#322392,#322393),(#322394,#322395,#322396),(#322397,
#322398,#322399),(#322400,#322401,#322402),(#322403,#322404,#322405),(#322406,
#322407,#322408),(#322409,#322410,#322411),(#322412,#322413,#322414),(#322415,
#322416,#322417),(#322418,#322419,#322420),(#322421,#322422,#322423),(#322424,
#322425,#322426),(#322427,#322428,#322429),(#322430,#322431,#322432),(#322433,
#322434,#322435),(#322436,#322437,#322438),(#322439,#322440,#322441),(#322442,
#322443,#322444),(#322445,#322446,#322447),(#322448,#322449,#322450),(#322451,
#322452,#322453),(#322454,#322455,#322456),(#322457,#322458,#322459),(#322460,
#322461,#322462),(#322463,#322464,#322465),(#322466,#322467,#322468),(#322469,
#322470,#322471),(#322472,#322473,#322474),(#322475,#322476,#322477),(#322478,
#322479,#322480),(#322481,#322482,#322483),(#322484,#322485,#322486),(#322487,
#322488,#322489),(#322490,#322491,#322492),(#322493,#322494,#322495),(#322496,
#322497,#322498),(#322499,#322500,#322501),(#322502,#322503,#322504),(#322505,
#322506,#322507),(#322508,#322509,#322510),(#322511,#322512,#322513),(#322514,
#322515,#322516),(#322517,#322518,#322519),(#322520,#322521,#322522),(#322523,
#322524,#322525),(#322526,#322527,#322528),(#322529,#322530,#322531),(#322532,
#322533,#322534),(#322535,#322536,#322537),(#322538,#322539,#322540),(#322541,
#322542,#322543),(#322544,#322545,#322546),(#322547,#322548,#322549),(#322550,
#322551,#322552),(#322553,#322554,#322555),(#322556,#322557,#322558),(#322559,
#322560,#322561),(#322562,#322563,#322564),(#322565,#322566,#322567),(#322568,
#322569,#322570),(#322571,#322572,#322573),(#322574,#322575,#322576),(#322577,
#322578,#322579),(#322580,#322581,#322582),(#322583,#322584,#322585),(#322586,
#322587,#322588),(#322589,#322590,#322591),(#322592,#322593,#322594),(#322595,
#322596,#322597),(#322598,#322599,#322600),(#322601,#322602,#322603),(#322604,
#322605,#322606),(#322607,#322608,#322609),(#322610,#322611,#322612),(#322613,
#322614,#322615),(#322616,#322617,#322618),(#322619,#322620,#322621),(#322622,
#322623,#322624),(#322625,#322626,#322627),(#322628,#322629,#322630),(#322631,
#322632,#322633),(#322634,#322635,#322636),(#322637,#322638,#322639),(#322640,
#322641,#322642),(#322643,#322644,#322645),(#322646,#322647,#322648),(#322649,
#322650,#322651),(#322652,#322653,#322654),(#322655,#322656,#322657),(#322658,
#322659,#322660),(#322661,#322662,#322663),(#322664,#322665,#322666),(#322667,
#322668,#322669),(#322670,#322671,#322672),(#322673,#322674,#322675),(#322676,
#322677,#322678),(#322679,#322680,#322681),(#322682,#322683,#322684),(#322685,
#322686,#322687),(#322688,#322689,#322690),(#322691,#322692,#322693),(#322694,
#322695,#322696),(#322697,#322698,#322699),(#322700,#322701,#322702),(#322703,
#322704,#322705),(#322706,#322707,#322708),(#322709,#322710,#322711),(#322712,
#322713,#322714),(#322715,#322716,#322717),(#322718,#322719,#322720),(#322721,
#322722,#322723),(#322724,#322725,#322726),(#322727,#322728,#322729),(#322730,
#322731,#322732),(#322733,#322734,#322735),(#322736,#322737,#322738),(#322739,
#322740,#322741),(#322742,#322743,#322744),(#322745,#322746,#322747),(#322748,
#322749,#322750),(#322751,#322752,#322753),(#322754,#322755,#322756),(#322757,
#322758,#322759),(#322760,#322761,#322762),(#322763,#322764,#322765),(#322766,
#322767,#322768),(#322769,#322770,#322771),(#322772,#322773,#322774),(#322775,
#322776,#322777),(#322778,#322779,#322780),(#322781,#322782,#322783),(#322784,
#322785,#322786),(#322787,#322788,#322789),(#322790,#322791,#322792),(#322793,
#322794,#322795),(#322796,#322797,#322798),(#322799,#322800,#322801),(#322802,
#322803,#322804),(#322805,#322806,#322807),(#322808,#322809,#322810),(#322811,
#322812,#322813),(#322814,#322815,#322816),(#322817,#322818,#322819),(#322820,
#322821,#322822),(#322823,#322824,#322825),(#322826,#322827,#322828),(#322829,
#322830,#322831),(#322832,#322833,#322834),(#322835,#322836,#322837),(#322838,
#322839,#322840),(#322841,#322842,#322843),(#322844,#322845,#322846),(#322847,
#322848,#322849),(#322850,#322851,#322852),(#322853,#322854,#322855),(#322856,
#322857,#322858),(#322859,#322860,#322861),(#322862,#322863,#322864),(#322865,
#322866,#322867),(#322868,#322869,#322870),(#322871,#322872,#322873),(#322874,
#322875,#322876),(#322877,#322878,#322879),(#322880,#322881,#322882),(#322883,
#322884,#322885),(#322886,#322887,#322888),(#322889,#322890,#322891),(#322892,
#322893,#322894),(#322895,#322896,#322897),(#322898,#322899,#322900),(#322901,
#322902,#322903),(#322904,#322905,#322906),(#322907,#322908,#322909),(#322910,
#322911,#322912),(#322913,#322914,#322915),(#322916,#322917,#322918),(#322919,
#322920,#322921),(#322922,#322923,#322924),(#322925,#322926,#322927),(#322928,
#322929,#322930),(#322931,#322932,#322933),(#322934,#322935,#322936),(#322937,
#322938,#322939),(#322940,#322941,#322942),(#322943,#322944,#322945),(#322946,
#322947,#322948),(#322949,#322950,#322951),(#322952,#322953,#322954),(#322955,
#322956,#322957),(#322958,#322959,#322960),(#322961,#322962,#322963),(#322964,
#322965,#322966),(#322967,#322968,#322969),(#322970,#322971,#322972),(#322973,
#322974,#322975),(#322976,#322977,#322978),(#322979,#322980,#322981),(#322982,
#322983,#322984),(#322985,#322986,#322987),(#322988,#322989,#322990),(#322991,
#322992,#322993),(#322994,#322995,#322996),(#322997,#322998,#322999),(#323000,
#323001,#323002),(#323003,#323004,#323005),(#323006,#323007,#323008)),
 .UNSPECIFIED.,.F.,.F.,.F.,(6,1,1,1,1,1,1,1,1,1,1,1,1,1,1,1,1,1,1,1,1,1,
1,1,1,1,1,1,1,1,1,1,1,1,1,1,1,1,1,1,1,1,1,1,1,1,1,1,1,1,1,1,1,1,1,1,1,1,
1,1,1,1,1,1,1,1,1,1,1,1,1,1,1,1,1,1,1,1,1,1,1,1,1,1,1,1,1,1,1,1,1,1,1,1,
1,1,1,1,1,1,1,1,1,1,1,1,1,1,1,1,1,1,1,1,1,1,1,1,1,1,1,1,1,1,1,1,1,1,1,1,
1,1,1,1,1,1,1,1,1,1,1,1,1,1,1,1,1,1,1,1,1,1,1,1,1,1,1,1,1,1,1,1,1,1,1,1,
1,1,1,1,1,1,1,1,1,1,1,1,1,1,1,1,1,1,1,1,1,1,1,1,1,1,1,1,1,1,1,1,1,1,1,1,
1,1,1,1,1,1,1,1,1,1,1,1,1,1,1,1,1,1,1,1,1,1,1,1,1,1,1,1,1,1,1,1,1,1,1,1,
1,1,1,1,1,1,1,1,1,1,1,1,1,1,1,1,1,1,1,1,1,1,1,1,1,1,1,1,1,1,1,1,1,1,1,1,
1,1,1,1,1,1,1,1,1,1,1,1,1,1,1,1,1,1,1,1,1,1,1,1,1,1,1,1,1,1,1,1,1,1,1,1,
1,1,1,1,1,1,1,1,1,1,1,1,1,1,1,1,1,1,1,1,1,1,1,1,1,1,1,1,1,1,1,1,1,1,1,1,
1,1,1,1,1,1,1,1,1,1,1,1,1,1,1,1,1,1,1,1,1,1,1,1,1,1,1,1,1,1,1,1,1,1,1,1,
1,1,1,1,1,1,1,1,1,1,1,1,1,1,1,1,1,1,1,1,1,1,1,1,1,1,1,1,1,1,1,1,1,1,1,1,
1,1,1,1,1,1,1,1,1,1,1,1,1,1,1,1,1,1,1,1,1,1,1,1,1,1,1,1,1,1,1,1,1,1,1,1,
1,1,1,1,1,1,1,1,1,1,1,1,1,1,1,1,1,1,1,1,1,1,1,1,1,1,1,1,1,1,1,1,1,1,1,1,
1,1,1,1,1,1,1,1,1,1,1,1,1,1,1,1,1,1,1,1,1,1,1,1,1,1,1,1,1,1,1,1,1,1,1,1,
1,1,1,1,1,1,1,1,1,1,1,1,1,1,1,1,1,1,1,6),(2,1,2),(-1.,-0.998165138,-0.996330275,
-0.994495413,-0.99266055,-0.990825688,-0.988990826,-0.987155963,-0.985321101,
-0.983486239,-0.981651376,-0.979816514,-0.977981651,-0.976146789,-0.974311927,
-0.972477064,-0.970642202,-0.968807339,-0.966972477,-0.965137615,-0.963302752,
-0.96146789,-0.959633028,-0.957798165,-0.955963303,-0.95412844,-0.952293578,
-0.950458716,-0.948623853,-0.946788991,-0.944954128,-0.943119266,-0.941284404,
-0.939449541,-0.937614679,-0.935779817,-0.933944954,-0.932110092,-0.930275229,
-0.928440367,-0.926605505,-0.924770642,-0.92293578,-0.921100917,-0.919266055,
-0.917431193,-0.91559633,-0.913761468,-0.911926606,-0.910091743,-0.908256881,
-0.906422018,-0.904587156,-0.902752294,-0.900917431,-0.899082569,-0.897247706,
-0.895412844,-0.893577982,-0.891743119,-0.889908257,-0.888073394,-0.886238532,
-0.88440367,-0.882568807,-0.880733945,-0.878899083,-0.87706422,-0.875229358,
-0.873394495,-0.871559633,-0.869724771,-0.867889908,-0.866055046,-0.864220183,
-0.862385321,-0.860550459,-0.858715596,-0.856880734,-0.855045872,-0.853211009,
-0.851376147,-0.849541284,-0.847706422,-0.84587156,-0.844036697,-0.842201835,
-0.840366972,-0.83853211,-0.836697248,-0.834862385,-0.833027523,-0.831192661,
-0.829357798,-0.827522936,-0.825688073,-0.823853211,-0.822018349,-0.820183486,
-0.818348624,-0.816513761,-0.814678899,-0.812844037,-0.811009174,-0.809174312,
-0.80733945,-0.805504587,-0.803669725,-0.801834862,-0.8,-0.798165138,-0.796330275,
-0.794495413,-0.79266055,-0.790825688,-0.788990826,-0.787155963,-0.785321101,
-0.783486239,-0.781651376,-0.779816514,-0.777981651,-0.776146789,-0.774311927,
-0.772477064,-0.770642202,-0.768807339,-0.766972477,-0.765137615,-0.763302752,
-0.76146789,-0.759633028,-0.757798165,-0.755963303,-0.75412844,-0.752293578,
-0.750458716,-0.748623853,-0.746788991,-0.744954128,-0.743119266,-0.741284404,
-0.739449541,-0.737614679,-0.735779817,-0.733944954,-0.732110092,-0.730275229,
-0.728440367,-0.726605505,-0.724770642,-0.72293578,-0.721100917,-0.719266055,
-0.717431193,-0.71559633,-0.713761468,-0.711926606,-0.710091743,-0.708256881,
-0.706422018,-0.704587156,-0.702752294,-0.700917431,-0.699082569,-0.697247706,
-0.695412844,-0.693577982,-0.691743119,-0.689908257,-0.688073394,-0.686238532,
-0.68440367,-0.682568807,-0.680733945,-0.678899083,-0.67706422,-0.675229358,
-0.673394495,-0.671559633,-0.669724771,-0.667889908,-0.666055046,-0.664220183,
-0.662385321,-0.660550459,-0.658715596,-0.656880734,-0.655045872,-0.653211009,
-0.651376147,-0.649541284,-0.647706422,-0.64587156,-0.644036697,-0.642201835,
-0.640366972,-0.63853211,-0.636697248,-0.634862385,-0.633027523,-0.631192661,
-0.629357798,-0.627522936,-0.625688073,-0.623853211,-0.622018349,-0.620183486,
-0.618348624,-0.616513761,-0.614678899,-0.612844037,-0.611009174,-0.609174312,
-0.60733945,-0.605504587,-0.603669725,-0.601834862,-0.6,-0.598165138,-0.596330275,
-0.594495413,-0.59266055,-0.590825688,-0.588990826,-0.587155963,-0.585321101,
-0.583486239,-0.581651376,-0.579816514,-0.577981651,-0.576146789,-0.574311927,
-0.572477064,-0.570642202,-0.568807339,-0.566972477,-0.565137615,-0.563302752,
-0.56146789,-0.559633028,-0.557798165,-0.555963303,-0.55412844,-0.552293578,
-0.550458716,-0.548623853,-0.546788991,-0.544954128,-0.543119266,-0.541284404,
-0.539449541,-0.537614679,-0.535779817,-0.533944954,-0.532110092,-0.530275229,
-0.528440367,-0.526605505,-0.524770642,-0.52293578,-0.521100917,-0.519266055,
-0.517431193,-0.51559633,-0.513761468,-0.511926606,-0.510091743,-0.508256881,
-0.506422018,-0.504587156,-0.502752294,-0.500917431,-0.499082569,-0.497247706,
-0.495412844,-0.493577982,-0.491743119,-0.489908257,-0.488073394,-0.486238532,
-0.48440367,-0.482568807,-0.480733945,-0.478899083,-0.47706422,-0.475229358,
-0.473394495,-0.471559633,-0.469724771,-0.467889908,-0.466055046,-0.464220183,
-0.462385321,-0.460550459,-0.458715596,-0.456880734,-0.455045872,-0.453211009,
-0.451376147,-0.449541284,-0.447706422,-0.44587156,-0.444036697,-0.442201835,
-0.440366972,-0.43853211,-0.436697248,-0.434862385,-0.433027523,-0.431192661,
-0.429357798,-0.427522936,-0.425688073,-0.423853211,-0.422018349,-0.420183486,
-0.418348624,-0.416513761,-0.414678899,-0.412844037,-0.411009174,-0.409174312,
-0.40733945,-0.405504587,-0.403669725,-0.401834862,-0.4,-0.398165138,-0.396330275,
-0.394495413,-0.39266055,-0.390825688,-0.388990826,-0.387155963,-0.385321101,
-0.383486239,-0.381651376,-0.379816514,-0.377981651,-0.376146789,-0.374311927,
-0.372477064,-0.370642202,-0.368807339,-0.366972477,-0.365137615,-0.363302752,
-0.36146789,-0.359633028,-0.357798165,-0.355963303,-0.35412844,-0.352293578,
-0.350458716,-0.348623853,-0.346788991,-0.344954128,-0.343119266,-0.341284404,
-0.339449541,-0.337614679,-0.335779817,-0.333944954,-0.332110092,-0.330275229,
-0.328440367,-0.326605505,-0.324770642,-0.32293578,-0.321100917,-0.319266055,
-0.317431193,-0.31559633,-0.313761468,-0.311926606,-0.310091743,-0.308256881,
-0.306422018,-0.304587156,-0.302752294,-0.300917431,-0.299082569,-0.297247706,
-0.295412844,-0.293577982,-0.291743119,-0.289908257,-0.288073394,-0.286238532,
-0.28440367,-0.282568807,-0.280733945,-0.278899083,-0.27706422,-0.275229358,
-0.273394495,-0.271559633,-0.269724771,-0.267889908,-0.266055046,-0.264220183,
-0.262385321,-0.260550459,-0.258715596,-0.256880734,-0.255045872,-0.253211009,
-0.251376147,-0.249541284,-0.247706422,-0.24587156,-0.244036697,-0.242201835,
-0.240366972,-0.23853211,-0.236697248,-0.234862385,-0.233027523,-0.231192661,
-0.229357798,-0.227522936,-0.225688073,-0.223853211,-0.222018349,-0.220183486,
-0.218348624,-0.216513761,-0.214678899,-0.212844037,-0.211009174,-0.209174312,
-0.20733945,-0.205504587,-0.203669725,-0.201834862,-0.2,-0.198165138,-0.196330275,
-0.194495413,-0.19266055,-0.190825688,-0.188990826,-0.187155963,-0.185321101,
-0.183486239,-0.181651376,-0.179816514,-0.177981651,-0.176146789,-0.174311927,
-0.172477064,-0.170642202,-0.168807339,-0.166972477,-0.165137615,-0.163302752,
-0.16146789,-0.159633028,-0.157798165,-0.155963303,-0.15412844,-0.152293578,
-0.150458716,-0.148623853,-0.146788991,-0.144954128,-0.143119266,-0.141284404,
-0.139449541,-0.137614679,-0.135779817,-0.133944954,-0.132110092,-0.130275229,
-0.128440367,-0.126605505,-0.124770642,-0.12293578,-0.121100917,-0.119266055,
-0.117431193,-0.11559633,-0.113761468,-0.111926606,-0.110091743,-0.108256881,
-0.106422018,-0.104587156,-0.102752294,-0.100917431,-0.099082569,-0.097247706,
-0.095412844,-0.093577982,-0.091743119,-0.089908257,-0.088073394,-0.086238532,
-0.08440367,-0.082568807,-0.080733945,-0.078899083,-0.07706422,-0.075229358,
-0.073394495,-0.071559633,-0.069724771,-0.067889908,-0.066055046,-0.064220183,
-0.062385321,-0.060550459,-0.058715596,-0.056880734,-0.055045872,-0.053211009,
-0.051376147,-0.049541284,-0.047706422,-0.04587156,-0.044036697,-0.042201835,
-0.040366972,-0.03853211,-0.036697248,-0.034862385,-0.033027523,-0.031192661,
-0.029357798,-0.027522936,-0.025688073,-0.023853211,-0.022018349,-0.020183486,
-0.018348624,-0.016513761,-0.014678899,-0.012844037,-0.011009174,-0.009174312,
-0.00733945,-0.005504587,-0.003669725,-0.001834862,0.000982105),(0.3,1.,
1.3),.UNSPECIFIED.);
#6316=B_SPLINE_SURFACE_WITH_KNOTS('',5,1,((#323031,#323032,#323033),(#323034,
#323035,#323036),(#323037,#323038,#323039),(#323040,#323041,#323042),(#323043,
#323044,#323045),(#323046,#323047,#323048),(#323049,#323050,#323051),(#323052,
#323053,#323054),(#323055,#323056,#323057),(#323058,#323059,#323060),(#323061,
#323062,#323063),(#323064,#323065,#323066),(#323067,#323068,#323069),(#323070,
#323071,#323072),(#323073,#323074,#323075),(#323076,#323077,#323078),(#323079,
#323080,#323081),(#323082,#323083,#323084),(#323085,#323086,#323087),(#323088,
#323089,#323090),(#323091,#323092,#323093),(#323094,#323095,#323096),(#323097,
#323098,#323099),(#323100,#323101,#323102),(#323103,#323104,#323105),(#323106,
#323107,#323108),(#323109,#323110,#323111),(#323112,#323113,#323114),(#323115,
#323116,#323117),(#323118,#323119,#323120),(#323121,#323122,#323123),(#323124,
#323125,#323126),(#323127,#323128,#323129),(#323130,#323131,#323132),(#323133,
#323134,#323135),(#323136,#323137,#323138),(#323139,#323140,#323141),(#323142,
#323143,#323144),(#323145,#323146,#323147),(#323148,#323149,#323150),(#323151,
#323152,#323153),(#323154,#323155,#323156),(#323157,#323158,#323159),(#323160,
#323161,#323162),(#323163,#323164,#323165),(#323166,#323167,#323168),(#323169,
#323170,#323171),(#323172,#323173,#323174),(#323175,#323176,#323177),(#323178,
#323179,#323180),(#323181,#323182,#323183),(#323184,#323185,#323186),(#323187,
#323188,#323189),(#323190,#323191,#323192),(#323193,#323194,#323195),(#323196,
#323197,#323198),(#323199,#323200,#323201),(#323202,#323203,#323204),(#323205,
#323206,#323207),(#323208,#323209,#323210),(#323211,#323212,#323213),(#323214,
#323215,#323216),(#323217,#323218,#323219),(#323220,#323221,#323222),(#323223,
#323224,#323225),(#323226,#323227,#323228),(#323229,#323230,#323231),(#323232,
#323233,#323234),(#323235,#323236,#323237),(#323238,#323239,#323240),(#323241,
#323242,#323243),(#323244,#323245,#323246),(#323247,#323248,#323249),(#323250,
#323251,#323252),(#323253,#323254,#323255),(#323256,#323257,#323258),(#323259,
#323260,#323261),(#323262,#323263,#323264),(#323265,#323266,#323267),(#323268,
#323269,#323270),(#323271,#323272,#323273),(#323274,#323275,#323276),(#323277,
#323278,#323279),(#323280,#323281,#323282),(#323283,#323284,#323285),(#323286,
#323287,#323288),(#323289,#323290,#323291),(#323292,#323293,#323294),(#323295,
#323296,#323297),(#323298,#323299,#323300),(#323301,#323302,#323303),(#323304,
#323305,#323306),(#323307,#323308,#323309),(#323310,#323311,#323312),(#323313,
#323314,#323315),(#323316,#323317,#323318),(#323319,#323320,#323321),(#323322,
#323323,#323324),(#323325,#323326,#323327),(#323328,#323329,#323330),(#323331,
#323332,#323333),(#323334,#323335,#323336),(#323337,#323338,#323339),(#323340,
#323341,#323342),(#323343,#323344,#323345),(#323346,#323347,#323348),(#323349,
#323350,#323351),(#323352,#323353,#323354),(#323355,#323356,#323357),(#323358,
#323359,#323360),(#323361,#323362,#323363),(#323364,#323365,#323366),(#323367,
#323368,#323369),(#323370,#323371,#323372),(#323373,#323374,#323375),(#323376,
#323377,#323378),(#323379,#323380,#323381),(#323382,#323383,#323384),(#323385,
#323386,#323387),(#323388,#323389,#323390),(#323391,#323392,#323393),(#323394,
#323395,#323396),(#323397,#323398,#323399),(#323400,#323401,#323402),(#323403,
#323404,#323405),(#323406,#323407,#323408),(#323409,#323410,#323411),(#323412,
#323413,#323414),(#323415,#323416,#323417),(#323418,#323419,#323420),(#323421,
#323422,#323423),(#323424,#323425,#323426),(#323427,#323428,#323429),(#323430,
#323431,#323432),(#323433,#323434,#323435),(#323436,#323437,#323438),(#323439,
#323440,#323441),(#323442,#323443,#323444),(#323445,#323446,#323447),(#323448,
#323449,#323450),(#323451,#323452,#323453),(#323454,#323455,#323456),(#323457,
#323458,#323459),(#323460,#323461,#323462),(#323463,#323464,#323465),(#323466,
#323467,#323468),(#323469,#323470,#323471),(#323472,#323473,#323474),(#323475,
#323476,#323477),(#323478,#323479,#323480),(#323481,#323482,#323483),(#323484,
#323485,#323486),(#323487,#323488,#323489),(#323490,#323491,#323492),(#323493,
#323494,#323495),(#323496,#323497,#323498),(#323499,#323500,#323501),(#323502,
#323503,#323504),(#323505,#323506,#323507),(#323508,#323509,#323510),(#323511,
#323512,#323513),(#323514,#323515,#323516),(#323517,#323518,#323519),(#323520,
#323521,#323522),(#323523,#323524,#323525),(#323526,#323527,#323528),(#323529,
#323530,#323531),(#323532,#323533,#323534),(#323535,#323536,#323537),(#323538,
#323539,#323540),(#323541,#323542,#323543),(#323544,#323545,#323546),(#323547,
#323548,#323549),(#323550,#323551,#323552),(#323553,#323554,#323555),(#323556,
#323557,#323558),(#323559,#323560,#323561),(#323562,#323563,#323564),(#323565,
#323566,#323567),(#323568,#323569,#323570),(#323571,#323572,#323573),(#323574,
#323575,#323576),(#323577,#323578,#323579),(#323580,#323581,#323582),(#323583,
#323584,#323585),(#323586,#323587,#323588),(#323589,#323590,#323591),(#323592,
#323593,#323594),(#323595,#323596,#323597),(#323598,#323599,#323600),(#323601,
#323602,#323603),(#323604,#323605,#323606),(#323607,#323608,#323609),(#323610,
#323611,#323612),(#323613,#323614,#323615),(#323616,#323617,#323618),(#323619,
#323620,#323621),(#323622,#323623,#323624),(#323625,#323626,#323627),(#323628,
#323629,#323630),(#323631,#323632,#323633),(#323634,#323635,#323636),(#323637,
#323638,#323639),(#323640,#323641,#323642),(#323643,#323644,#323645),(#323646,
#323647,#323648),(#323649,#323650,#323651),(#323652,#323653,#323654),(#323655,
#323656,#323657),(#323658,#323659,#323660),(#323661,#323662,#323663),(#323664,
#323665,#323666),(#323667,#323668,#323669),(#323670,#323671,#323672),(#323673,
#323674,#323675),(#323676,#323677,#323678),(#323679,#323680,#323681),(#323682,
#323683,#323684),(#323685,#323686,#323687),(#323688,#323689,#323690),(#323691,
#323692,#323693),(#323694,#323695,#323696),(#323697,#323698,#323699),(#323700,
#323701,#323702),(#323703,#323704,#323705),(#323706,#323707,#323708),(#323709,
#323710,#323711),(#323712,#323713,#323714),(#323715,#323716,#323717),(#323718,
#323719,#323720),(#323721,#323722,#323723),(#323724,#323725,#323726),(#323727,
#323728,#323729),(#323730,#323731,#323732),(#323733,#323734,#323735),(#323736,
#323737,#323738),(#323739,#323740,#323741),(#323742,#323743,#323744),(#323745,
#323746,#323747),(#323748,#323749,#323750),(#323751,#323752,#323753),(#323754,
#323755,#323756),(#323757,#323758,#323759),(#323760,#323761,#323762),(#323763,
#323764,#323765),(#323766,#323767,#323768),(#323769,#323770,#323771),(#323772,
#323773,#323774),(#323775,#323776,#323777),(#323778,#323779,#323780),(#323781,
#323782,#323783),(#323784,#323785,#323786),(#323787,#323788,#323789),(#323790,
#323791,#323792),(#323793,#323794,#323795),(#323796,#323797,#323798),(#323799,
#323800,#323801),(#323802,#323803,#323804),(#323805,#323806,#323807),(#323808,
#323809,#323810),(#323811,#323812,#323813),(#323814,#323815,#323816),(#323817,
#323818,#323819),(#323820,#323821,#323822),(#323823,#323824,#323825),(#323826,
#323827,#323828),(#323829,#323830,#323831),(#323832,#323833,#323834),(#323835,
#323836,#323837),(#323838,#323839,#323840),(#323841,#323842,#323843),(#323844,
#323845,#323846),(#323847,#323848,#323849),(#323850,#323851,#323852),(#323853,
#323854,#323855),(#323856,#323857,#323858),(#323859,#323860,#323861),(#323862,
#323863,#323864),(#323865,#323866,#323867),(#323868,#323869,#323870),(#323871,
#323872,#323873),(#323874,#323875,#323876),(#323877,#323878,#323879),(#323880,
#323881,#323882),(#323883,#323884,#323885),(#323886,#323887,#323888),(#323889,
#323890,#323891),(#323892,#323893,#323894),(#323895,#323896,#323897),(#323898,
#323899,#323900),(#323901,#323902,#323903),(#323904,#323905,#323906),(#323907,
#323908,#323909),(#323910,#323911,#323912),(#323913,#323914,#323915),(#323916,
#323917,#323918),(#323919,#323920,#323921),(#323922,#323923,#323924),(#323925,
#323926,#323927),(#323928,#323929,#323930),(#323931,#323932,#323933),(#323934,
#323935,#323936),(#323937,#323938,#323939),(#323940,#323941,#323942),(#323943,
#323944,#323945),(#323946,#323947,#323948),(#323949,#323950,#323951),(#323952,
#323953,#323954),(#323955,#323956,#323957),(#323958,#323959,#323960),(#323961,
#323962,#323963),(#323964,#323965,#323966),(#323967,#323968,#323969),(#323970,
#323971,#323972),(#323973,#323974,#323975),(#323976,#323977,#323978),(#323979,
#323980,#323981),(#323982,#323983,#323984),(#323985,#323986,#323987),(#323988,
#323989,#323990),(#323991,#323992,#323993),(#323994,#323995,#323996),(#323997,
#323998,#323999),(#324000,#324001,#324002),(#324003,#324004,#324005),(#324006,
#324007,#324008),(#324009,#324010,#324011),(#324012,#324013,#324014),(#324015,
#324016,#324017),(#324018,#324019,#324020),(#324021,#324022,#324023),(#324024,
#324025,#324026),(#324027,#324028,#324029),(#324030,#324031,#324032),(#324033,
#324034,#324035),(#324036,#324037,#324038),(#324039,#324040,#324041),(#324042,
#324043,#324044),(#324045,#324046,#324047),(#324048,#324049,#324050),(#324051,
#324052,#324053),(#324054,#324055,#324056),(#324057,#324058,#324059),(#324060,
#324061,#324062),(#324063,#324064,#324065),(#324066,#324067,#324068),(#324069,
#324070,#324071),(#324072,#324073,#324074),(#324075,#324076,#324077),(#324078,
#324079,#324080),(#324081,#324082,#324083),(#324084,#324085,#324086),(#324087,
#324088,#324089),(#324090,#324091,#324092),(#324093,#324094,#324095),(#324096,
#324097,#324098),(#324099,#324100,#324101),(#324102,#324103,#324104),(#324105,
#324106,#324107),(#324108,#324109,#324110),(#324111,#324112,#324113),(#324114,
#324115,#324116),(#324117,#324118,#324119),(#324120,#324121,#324122),(#324123,
#324124,#324125),(#324126,#324127,#324128),(#324129,#324130,#324131),(#324132,
#324133,#324134),(#324135,#324136,#324137),(#324138,#324139,#324140),(#324141,
#324142,#324143),(#324144,#324145,#324146),(#324147,#324148,#324149),(#324150,
#324151,#324152),(#324153,#324154,#324155),(#324156,#324157,#324158),(#324159,
#324160,#324161),(#324162,#324163,#324164),(#324165,#324166,#324167),(#324168,
#324169,#324170),(#324171,#324172,#324173),(#324174,#324175,#324176),(#324177,
#324178,#324179),(#324180,#324181,#324182),(#324183,#324184,#324185),(#324186,
#324187,#324188),(#324189,#324190,#324191),(#324192,#324193,#324194),(#324195,
#324196,#324197),(#324198,#324199,#324200),(#324201,#324202,#324203),(#324204,
#324205,#324206),(#324207,#324208,#324209),(#324210,#324211,#324212),(#324213,
#324214,#324215),(#324216,#324217,#324218),(#324219,#324220,#324221),(#324222,
#324223,#324224),(#324225,#324226,#324227),(#324228,#324229,#324230),(#324231,
#324232,#324233),(#324234,#324235,#324236),(#324237,#324238,#324239),(#324240,
#324241,#324242),(#324243,#324244,#324245),(#324246,#324247,#324248),(#324249,
#324250,#324251),(#324252,#324253,#324254),(#324255,#324256,#324257),(#324258,
#324259,#324260),(#324261,#324262,#324263),(#324264,#324265,#324266),(#324267,
#324268,#324269),(#324270,#324271,#324272),(#324273,#324274,#324275),(#324276,
#324277,#324278),(#324279,#324280,#324281),(#324282,#324283,#324284),(#324285,
#324286,#324287),(#324288,#324289,#324290),(#324291,#324292,#324293),(#324294,
#324295,#324296),(#324297,#324298,#324299),(#324300,#324301,#324302),(#324303,
#324304,#324305),(#324306,#324307,#324308),(#324309,#324310,#324311),(#324312,
#324313,#324314),(#324315,#324316,#324317),(#324318,#324319,#324320),(#324321,
#324322,#324323),(#324324,#324325,#324326),(#324327,#324328,#324329),(#324330,
#324331,#324332),(#324333,#324334,#324335),(#324336,#324337,#324338),(#324339,
#324340,#324341),(#324342,#324343,#324344),(#324345,#324346,#324347),(#324348,
#324349,#324350),(#324351,#324352,#324353),(#324354,#324355,#324356),(#324357,
#324358,#324359),(#324360,#324361,#324362),(#324363,#324364,#324365),(#324366,
#324367,#324368),(#324369,#324370,#324371),(#324372,#324373,#324374),(#324375,
#324376,#324377),(#324378,#324379,#324380),(#324381,#324382,#324383),(#324384,
#324385,#324386),(#324387,#324388,#324389),(#324390,#324391,#324392),(#324393,
#324394,#324395),(#324396,#324397,#324398),(#324399,#324400,#324401),(#324402,
#324403,#324404),(#324405,#324406,#324407),(#324408,#324409,#324410),(#324411,
#324412,#324413),(#324414,#324415,#324416),(#324417,#324418,#324419),(#324420,
#324421,#324422),(#324423,#324424,#324425),(#324426,#324427,#324428),(#324429,
#324430,#324431),(#324432,#324433,#324434),(#324435,#324436,#324437),(#324438,
#324439,#324440),(#324441,#324442,#324443),(#324444,#324445,#324446),(#324447,
#324448,#324449),(#324450,#324451,#324452),(#324453,#324454,#324455),(#324456,
#324457,#324458),(#324459,#324460,#324461),(#324462,#324463,#324464),(#324465,
#324466,#324467),(#324468,#324469,#324470),(#324471,#324472,#324473),(#324474,
#324475,#324476),(#324477,#324478,#324479),(#324480,#324481,#324482),(#324483,
#324484,#324485),(#324486,#324487,#324488),(#324489,#324490,#324491),(#324492,
#324493,#324494),(#324495,#324496,#324497),(#324498,#324499,#324500),(#324501,
#324502,#324503),(#324504,#324505,#324506),(#324507,#324508,#324509),(#324510,
#324511,#324512),(#324513,#324514,#324515),(#324516,#324517,#324518),(#324519,
#324520,#324521),(#324522,#324523,#324524),(#324525,#324526,#324527),(#324528,
#324529,#324530),(#324531,#324532,#324533),(#324534,#324535,#324536),(#324537,
#324538,#324539),(#324540,#324541,#324542),(#324543,#324544,#324545),(#324546,
#324547,#324548),(#324549,#324550,#324551),(#324552,#324553,#324554),(#324555,
#324556,#324557),(#324558,#324559,#324560),(#324561,#324562,#324563),(#324564,
#324565,#324566),(#324567,#324568,#324569),(#324570,#324571,#324572),(#324573,
#324574,#324575),(#324576,#324577,#324578),(#324579,#324580,#324581),(#324582,
#324583,#324584),(#324585,#324586,#324587),(#324588,#324589,#324590),(#324591,
#324592,#324593),(#324594,#324595,#324596),(#324597,#324598,#324599),(#324600,
#324601,#324602),(#324603,#324604,#324605),(#324606,#324607,#324608),(#324609,
#324610,#324611),(#324612,#324613,#324614),(#324615,#324616,#324617),(#324618,
#324619,#324620),(#324621,#324622,#324623),(#324624,#324625,#324626),(#324627,
#324628,#324629),(#324630,#324631,#324632),(#324633,#324634,#324635),(#324636,
#324637,#324638),(#324639,#324640,#324641),(#324642,#324643,#324644),(#324645,
#324646,#324647),(#324648,#324649,#324650),(#324651,#324652,#324653),(#324654,
#324655,#324656),(#324657,#324658,#324659),(#324660,#324661,#324662),(#324663,
#324664,#324665),(#324666,#324667,#324668),(#324669,#324670,#324671),(#324672,
#324673,#324674),(#324675,#324676,#324677),(#324678,#324679,#324680),(#324681,
#324682,#324683)),.UNSPECIFIED.,.F.,.F.,.F.,(6,1,1,1,1,1,1,1,1,1,1,1,1,
1,1,1,1,1,1,1,1,1,1,1,1,1,1,1,1,1,1,1,1,1,1,1,1,1,1,1,1,1,1,1,1,1,1,1,1,
1,1,1,1,1,1,1,1,1,1,1,1,1,1,1,1,1,1,1,1,1,1,1,1,1,1,1,1,1,1,1,1,1,1,1,1,
1,1,1,1,1,1,1,1,1,1,1,1,1,1,1,1,1,1,1,1,1,1,1,1,1,1,1,1,1,1,1,1,1,1,1,1,
1,1,1,1,1,1,1,1,1,1,1,1,1,1,1,1,1,1,1,1,1,1,1,1,1,1,1,1,1,1,1,1,1,1,1,1,
1,1,1,1,1,1,1,1,1,1,1,1,1,1,1,1,1,1,1,1,1,1,1,1,1,1,1,1,1,1,1,1,1,1,1,1,
1,1,1,1,1,1,1,1,1,1,1,1,1,1,1,1,1,1,1,1,1,1,1,1,1,1,1,1,1,1,1,1,1,1,1,1,
1,1,1,1,1,1,1,1,1,1,1,1,1,1,1,1,1,1,1,1,1,1,1,1,1,1,1,1,1,1,1,1,1,1,1,1,
1,1,1,1,1,1,1,1,1,1,1,1,1,1,1,1,1,1,1,1,1,1,1,1,1,1,1,1,1,1,1,1,1,1,1,1,
1,1,1,1,1,1,1,1,1,1,1,1,1,1,1,1,1,1,1,1,1,1,1,1,1,1,1,1,1,1,1,1,1,1,1,1,
1,1,1,1,1,1,1,1,1,1,1,1,1,1,1,1,1,1,1,1,1,1,1,1,1,1,1,1,1,1,1,1,1,1,1,1,
1,1,1,1,1,1,1,1,1,1,1,1,1,1,1,1,1,1,1,1,1,1,1,1,1,1,1,1,1,1,1,1,1,1,1,1,
1,1,1,1,1,1,1,1,1,1,1,1,1,1,1,1,1,1,1,1,1,1,1,1,1,1,1,1,1,1,1,1,1,1,1,1,
1,1,1,1,1,1,1,1,1,1,1,1,1,1,1,1,1,1,1,1,1,1,1,1,1,1,1,1,1,1,1,1,1,1,1,1,
1,1,1,1,1,1,1,1,1,1,1,1,1,1,1,1,1,1,1,1,1,1,1,1,1,1,1,1,1,1,1,1,1,1,1,1,
1,1,1,1,1,1,1,1,1,1,1,1,1,1,1,1,1,1,1,1,1,1,1,1,1,1,1,1,1,6),(2,1,2),(-0.001964187,
0.,0.001834862,0.003669725,0.005504587,0.00733945,0.009174312,0.011009174,
0.012844037,0.014678899,0.016513761,0.018348624,0.020183486,0.022018349,
0.023853211,0.025688073,0.027522936,0.029357798,0.031192661,0.033027523,
0.034862385,0.036697248,0.03853211,0.040366972,0.042201835,0.044036697,
0.04587156,0.047706422,0.049541284,0.051376147,0.053211009,0.055045872,
0.056880734,0.058715596,0.060550459,0.062385321,0.064220183,0.066055046,
0.067889908,0.069724771,0.071559633,0.073394495,0.075229358,0.07706422,
0.078899083,0.080733945,0.082568807,0.08440367,0.086238532,0.088073394,
0.089908257,0.091743119,0.093577982,0.095412844,0.097247706,0.099082569,
0.100917431,0.102752294,0.104587156,0.106422018,0.108256881,0.110091743,
0.111926606,0.113761468,0.11559633,0.117431193,0.119266055,0.121100917,
0.12293578,0.124770642,0.126605505,0.128440367,0.130275229,0.132110092,
0.133944954,0.135779817,0.137614679,0.139449541,0.141284404,0.143119266,
0.144954128,0.146788991,0.148623853,0.150458716,0.152293578,0.15412844,
0.155963303,0.157798165,0.159633028,0.16146789,0.163302752,0.165137615,
0.166972477,0.168807339,0.170642202,0.172477064,0.174311927,0.176146789,
0.177981651,0.179816514,0.181651376,0.183486239,0.185321101,0.187155963,
0.188990826,0.190825688,0.19266055,0.194495413,0.196330275,0.198165138,
0.2,0.201834862,0.203669725,0.205504587,0.20733945,0.209174312,0.211009174,
0.212844037,0.214678899,0.216513761,0.218348624,0.220183486,0.222018349,
0.223853211,0.225688073,0.227522936,0.229357798,0.231192661,0.233027523,
0.234862385,0.236697248,0.23853211,0.240366972,0.242201835,0.244036697,
0.24587156,0.247706422,0.249541284,0.251376147,0.253211009,0.255045872,
0.256880734,0.258715596,0.260550459,0.262385321,0.264220183,0.266055046,
0.267889908,0.269724771,0.271559633,0.273394495,0.275229358,0.27706422,
0.278899083,0.280733945,0.282568807,0.28440367,0.286238532,0.288073394,
0.289908257,0.291743119,0.293577982,0.295412844,0.297247706,0.299082569,
0.300917431,0.302752294,0.304587156,0.306422018,0.308256881,0.310091743,
0.311926606,0.313761468,0.31559633,0.317431193,0.319266055,0.321100917,
0.32293578,0.324770642,0.326605505,0.328440367,0.330275229,0.332110092,
0.333944954,0.335779817,0.337614679,0.339449541,0.341284404,0.343119266,
0.344954128,0.346788991,0.348623853,0.350458716,0.352293578,0.35412844,
0.355963303,0.357798165,0.359633028,0.36146789,0.363302752,0.365137615,
0.366972477,0.368807339,0.370642202,0.372477064,0.374311927,0.376146789,
0.377981651,0.379816514,0.381651376,0.383486239,0.385321101,0.387155963,
0.388990826,0.390825688,0.39266055,0.394495413,0.396330275,0.398165138,
0.4,0.401834862,0.403669725,0.405504587,0.40733945,0.409174312,0.411009174,
0.412844037,0.414678899,0.416513761,0.418348624,0.420183486,0.422018349,
0.423853211,0.425688073,0.427522936,0.429357798,0.431192661,0.433027523,
0.434862385,0.436697248,0.43853211,0.440366972,0.442201835,0.444036697,
0.44587156,0.447706422,0.449541284,0.451376147,0.453211009,0.455045872,
0.456880734,0.458715596,0.460550459,0.462385321,0.464220183,0.466055046,
0.467889908,0.469724771,0.471559633,0.473394495,0.475229358,0.47706422,
0.478899083,0.480733945,0.482568807,0.48440367,0.486238532,0.488073394,
0.489908257,0.491743119,0.493577982,0.495412844,0.497247706,0.499082569,
0.500917431,0.502752294,0.504587156,0.506422018,0.508256881,0.510091743,
0.511926606,0.513761468,0.51559633,0.517431193,0.519266055,0.521100917,
0.52293578,0.524770642,0.526605505,0.528440367,0.530275229,0.532110092,
0.533944954,0.535779817,0.537614679,0.539449541,0.541284404,0.543119266,
0.544954128,0.546788991,0.548623853,0.550458716,0.552293578,0.55412844,
0.555963303,0.557798165,0.559633028,0.56146789,0.563302752,0.565137615,
0.566972477,0.568807339,0.570642202,0.572477064,0.574311927,0.576146789,
0.577981651,0.579816514,0.581651376,0.583486239,0.585321101,0.587155963,
0.588990826,0.590825688,0.59266055,0.594495413,0.596330275,0.598165138,
0.6,0.601834862,0.603669725,0.605504587,0.60733945,0.609174312,0.611009174,
0.612844037,0.614678899,0.616513761,0.618348624,0.620183486,0.622018349,
0.623853211,0.625688073,0.627522936,0.629357798,0.631192661,0.633027523,
0.634862385,0.636697248,0.63853211,0.640366972,0.642201835,0.644036697,
0.64587156,0.647706422,0.649541284,0.651376147,0.653211009,0.655045872,
0.656880734,0.658715596,0.660550459,0.662385321,0.664220183,0.666055046,
0.667889908,0.669724771,0.671559633,0.673394495,0.675229358,0.67706422,
0.678899083,0.680733945,0.682568807,0.68440367,0.686238532,0.688073394,
0.689908257,0.691743119,0.693577982,0.695412844,0.697247706,0.699082569,
0.700917431,0.702752294,0.704587156,0.706422018,0.708256881,0.710091743,
0.711926606,0.713761468,0.71559633,0.717431193,0.719266055,0.721100917,
0.72293578,0.724770642,0.726605505,0.728440367,0.730275229,0.732110092,
0.733944954,0.735779817,0.737614679,0.739449541,0.741284404,0.743119266,
0.744954128,0.746788991,0.748623853,0.750458716,0.752293578,0.75412844,
0.755963303,0.757798165,0.759633028,0.76146789,0.763302752,0.765137615,
0.766972477,0.768807339,0.770642202,0.772477064,0.774311927,0.776146789,
0.777981651,0.779816514,0.781651376,0.783486239,0.785321101,0.787155963,
0.788990826,0.790825688,0.79266055,0.794495413,0.796330275,0.798165138,
0.8,0.801834862,0.803669725,0.805504587,0.80733945,0.809174312,0.811009174,
0.812844037,0.814678899,0.816513761,0.818348624,0.820183486,0.822018349,
0.823853211,0.825688073,0.827522936,0.829357798,0.831192661,0.833027523,
0.834862385,0.836697248,0.83853211,0.840366972,0.842201835,0.844036697,
0.84587156,0.847706422,0.849541284,0.851376147,0.853211009,0.855045872,
0.856880734,0.858715596,0.860550459,0.862385321,0.864220183,0.866055046,
0.867889908,0.869724771,0.871559633,0.873394495,0.875229358,0.87706422,
0.878899083,0.880733945,0.882568807,0.88440367,0.886238532,0.888073394,
0.889908257,0.891743119,0.893577982,0.895412844,0.897247706,0.899082569,
0.900917431,0.902752294,0.904587156,0.906422018,0.908256881,0.910091743,
0.911926606,0.913761468,0.91559633,0.917431193,0.919266055,0.921100917,
0.92293578,0.924770642,0.926605505,0.928440367,0.930275229,0.932110092,
0.933944954,0.935779817,0.937614679,0.939449541,0.941284404,0.943119266,
0.944954128,0.946788991,0.948623853,0.950458716,0.952293578,0.95412844,
0.955963303,0.957798165,0.959633028,0.96146789,0.963302752,0.965137615,
0.966972477,0.968807339,0.970642202,0.972477064,0.974311927,0.976146789,
0.977981651,0.979816514,0.981651376,0.983486239,0.985321101,0.987155963,
0.988990826,0.990825688,0.99266055,0.994495413,0.996330275,0.998165138,
1.),(0.3,1.,1.3),.UNSPECIFIED.);
#6317=B_SPLINE_SURFACE_WITH_KNOTS('',5,1,((#324706,#324707,#324708),(#324709,
#324710,#324711),(#324712,#324713,#324714),(#324715,#324716,#324717),(#324718,
#324719,#324720),(#324721,#324722,#324723),(#324724,#324725,#324726),(#324727,
#324728,#324729),(#324730,#324731,#324732),(#324733,#324734,#324735),(#324736,
#324737,#324738),(#324739,#324740,#324741),(#324742,#324743,#324744),(#324745,
#324746,#324747),(#324748,#324749,#324750),(#324751,#324752,#324753),(#324754,
#324755,#324756),(#324757,#324758,#324759),(#324760,#324761,#324762),(#324763,
#324764,#324765),(#324766,#324767,#324768),(#324769,#324770,#324771),(#324772,
#324773,#324774),(#324775,#324776,#324777),(#324778,#324779,#324780),(#324781,
#324782,#324783),(#324784,#324785,#324786),(#324787,#324788,#324789),(#324790,
#324791,#324792),(#324793,#324794,#324795),(#324796,#324797,#324798),(#324799,
#324800,#324801),(#324802,#324803,#324804),(#324805,#324806,#324807),(#324808,
#324809,#324810),(#324811,#324812,#324813),(#324814,#324815,#324816),(#324817,
#324818,#324819),(#324820,#324821,#324822),(#324823,#324824,#324825),(#324826,
#324827,#324828),(#324829,#324830,#324831),(#324832,#324833,#324834),(#324835,
#324836,#324837),(#324838,#324839,#324840),(#324841,#324842,#324843),(#324844,
#324845,#324846),(#324847,#324848,#324849),(#324850,#324851,#324852),(#324853,
#324854,#324855),(#324856,#324857,#324858),(#324859,#324860,#324861),(#324862,
#324863,#324864),(#324865,#324866,#324867),(#324868,#324869,#324870),(#324871,
#324872,#324873),(#324874,#324875,#324876),(#324877,#324878,#324879),(#324880,
#324881,#324882),(#324883,#324884,#324885),(#324886,#324887,#324888),(#324889,
#324890,#324891),(#324892,#324893,#324894),(#324895,#324896,#324897),(#324898,
#324899,#324900),(#324901,#324902,#324903),(#324904,#324905,#324906),(#324907,
#324908,#324909),(#324910,#324911,#324912),(#324913,#324914,#324915),(#324916,
#324917,#324918),(#324919,#324920,#324921),(#324922,#324923,#324924),(#324925,
#324926,#324927),(#324928,#324929,#324930),(#324931,#324932,#324933),(#324934,
#324935,#324936),(#324937,#324938,#324939),(#324940,#324941,#324942),(#324943,
#324944,#324945),(#324946,#324947,#324948),(#324949,#324950,#324951),(#324952,
#324953,#324954),(#324955,#324956,#324957),(#324958,#324959,#324960),(#324961,
#324962,#324963),(#324964,#324965,#324966),(#324967,#324968,#324969),(#324970,
#324971,#324972),(#324973,#324974,#324975),(#324976,#324977,#324978),(#324979,
#324980,#324981),(#324982,#324983,#324984),(#324985,#324986,#324987),(#324988,
#324989,#324990),(#324991,#324992,#324993),(#324994,#324995,#324996),(#324997,
#324998,#324999),(#325000,#325001,#325002),(#325003,#325004,#325005),(#325006,
#325007,#325008),(#325009,#325010,#325011),(#325012,#325013,#325014),(#325015,
#325016,#325017),(#325018,#325019,#325020),(#325021,#325022,#325023),(#325024,
#325025,#325026),(#325027,#325028,#325029),(#325030,#325031,#325032),(#325033,
#325034,#325035),(#325036,#325037,#325038),(#325039,#325040,#325041),(#325042,
#325043,#325044),(#325045,#325046,#325047),(#325048,#325049,#325050),(#325051,
#325052,#325053),(#325054,#325055,#325056),(#325057,#325058,#325059),(#325060,
#325061,#325062),(#325063,#325064,#325065),(#325066,#325067,#325068),(#325069,
#325070,#325071),(#325072,#325073,#325074),(#325075,#325076,#325077),(#325078,
#325079,#325080),(#325081,#325082,#325083),(#325084,#325085,#325086),(#325087,
#325088,#325089),(#325090,#325091,#325092),(#325093,#325094,#325095),(#325096,
#325097,#325098),(#325099,#325100,#325101),(#325102,#325103,#325104),(#325105,
#325106,#325107),(#325108,#325109,#325110),(#325111,#325112,#325113),(#325114,
#325115,#325116),(#325117,#325118,#325119),(#325120,#325121,#325122),(#325123,
#325124,#325125),(#325126,#325127,#325128),(#325129,#325130,#325131),(#325132,
#325133,#325134),(#325135,#325136,#325137),(#325138,#325139,#325140),(#325141,
#325142,#325143),(#325144,#325145,#325146),(#325147,#325148,#325149),(#325150,
#325151,#325152),(#325153,#325154,#325155),(#325156,#325157,#325158),(#325159,
#325160,#325161),(#325162,#325163,#325164),(#325165,#325166,#325167),(#325168,
#325169,#325170),(#325171,#325172,#325173),(#325174,#325175,#325176),(#325177,
#325178,#325179),(#325180,#325181,#325182),(#325183,#325184,#325185),(#325186,
#325187,#325188),(#325189,#325190,#325191),(#325192,#325193,#325194),(#325195,
#325196,#325197),(#325198,#325199,#325200),(#325201,#325202,#325203),(#325204,
#325205,#325206),(#325207,#325208,#325209),(#325210,#325211,#325212),(#325213,
#325214,#325215),(#325216,#325217,#325218),(#325219,#325220,#325221),(#325222,
#325223,#325224),(#325225,#325226,#325227),(#325228,#325229,#325230),(#325231,
#325232,#325233),(#325234,#325235,#325236),(#325237,#325238,#325239),(#325240,
#325241,#325242),(#325243,#325244,#325245),(#325246,#325247,#325248),(#325249,
#325250,#325251),(#325252,#325253,#325254),(#325255,#325256,#325257),(#325258,
#325259,#325260),(#325261,#325262,#325263),(#325264,#325265,#325266),(#325267,
#325268,#325269),(#325270,#325271,#325272),(#325273,#325274,#325275),(#325276,
#325277,#325278),(#325279,#325280,#325281),(#325282,#325283,#325284),(#325285,
#325286,#325287),(#325288,#325289,#325290),(#325291,#325292,#325293),(#325294,
#325295,#325296),(#325297,#325298,#325299),(#325300,#325301,#325302),(#325303,
#325304,#325305),(#325306,#325307,#325308),(#325309,#325310,#325311),(#325312,
#325313,#325314),(#325315,#325316,#325317),(#325318,#325319,#325320),(#325321,
#325322,#325323),(#325324,#325325,#325326),(#325327,#325328,#325329),(#325330,
#325331,#325332),(#325333,#325334,#325335),(#325336,#325337,#325338),(#325339,
#325340,#325341),(#325342,#325343,#325344),(#325345,#325346,#325347),(#325348,
#325349,#325350),(#325351,#325352,#325353),(#325354,#325355,#325356),(#325357,
#325358,#325359),(#325360,#325361,#325362),(#325363,#325364,#325365),(#325366,
#325367,#325368),(#325369,#325370,#325371),(#325372,#325373,#325374),(#325375,
#325376,#325377),(#325378,#325379,#325380),(#325381,#325382,#325383),(#325384,
#325385,#325386),(#325387,#325388,#325389),(#325390,#325391,#325392),(#325393,
#325394,#325395),(#325396,#325397,#325398),(#325399,#325400,#325401),(#325402,
#325403,#325404),(#325405,#325406,#325407),(#325408,#325409,#325410),(#325411,
#325412,#325413),(#325414,#325415,#325416),(#325417,#325418,#325419),(#325420,
#325421,#325422),(#325423,#325424,#325425),(#325426,#325427,#325428),(#325429,
#325430,#325431),(#325432,#325433,#325434),(#325435,#325436,#325437),(#325438,
#325439,#325440),(#325441,#325442,#325443),(#325444,#325445,#325446),(#325447,
#325448,#325449),(#325450,#325451,#325452),(#325453,#325454,#325455),(#325456,
#325457,#325458),(#325459,#325460,#325461),(#325462,#325463,#325464),(#325465,
#325466,#325467),(#325468,#325469,#325470),(#325471,#325472,#325473),(#325474,
#325475,#325476),(#325477,#325478,#325479),(#325480,#325481,#325482),(#325483,
#325484,#325485),(#325486,#325487,#325488),(#325489,#325490,#325491),(#325492,
#325493,#325494),(#325495,#325496,#325497),(#325498,#325499,#325500),(#325501,
#325502,#325503),(#325504,#325505,#325506),(#325507,#325508,#325509),(#325510,
#325511,#325512),(#325513,#325514,#325515),(#325516,#325517,#325518),(#325519,
#325520,#325521),(#325522,#325523,#325524),(#325525,#325526,#325527),(#325528,
#325529,#325530),(#325531,#325532,#325533),(#325534,#325535,#325536),(#325537,
#325538,#325539),(#325540,#325541,#325542),(#325543,#325544,#325545),(#325546,
#325547,#325548),(#325549,#325550,#325551),(#325552,#325553,#325554),(#325555,
#325556,#325557),(#325558,#325559,#325560),(#325561,#325562,#325563),(#325564,
#325565,#325566),(#325567,#325568,#325569),(#325570,#325571,#325572),(#325573,
#325574,#325575),(#325576,#325577,#325578),(#325579,#325580,#325581),(#325582,
#325583,#325584),(#325585,#325586,#325587),(#325588,#325589,#325590),(#325591,
#325592,#325593),(#325594,#325595,#325596),(#325597,#325598,#325599),(#325600,
#325601,#325602),(#325603,#325604,#325605),(#325606,#325607,#325608),(#325609,
#325610,#325611),(#325612,#325613,#325614),(#325615,#325616,#325617),(#325618,
#325619,#325620),(#325621,#325622,#325623),(#325624,#325625,#325626),(#325627,
#325628,#325629),(#325630,#325631,#325632),(#325633,#325634,#325635),(#325636,
#325637,#325638),(#325639,#325640,#325641),(#325642,#325643,#325644),(#325645,
#325646,#325647),(#325648,#325649,#325650),(#325651,#325652,#325653),(#325654,
#325655,#325656),(#325657,#325658,#325659),(#325660,#325661,#325662),(#325663,
#325664,#325665),(#325666,#325667,#325668),(#325669,#325670,#325671),(#325672,
#325673,#325674),(#325675,#325676,#325677),(#325678,#325679,#325680),(#325681,
#325682,#325683),(#325684,#325685,#325686),(#325687,#325688,#325689),(#325690,
#325691,#325692),(#325693,#325694,#325695),(#325696,#325697,#325698),(#325699,
#325700,#325701),(#325702,#325703,#325704),(#325705,#325706,#325707),(#325708,
#325709,#325710),(#325711,#325712,#325713),(#325714,#325715,#325716),(#325717,
#325718,#325719),(#325720,#325721,#325722),(#325723,#325724,#325725),(#325726,
#325727,#325728),(#325729,#325730,#325731),(#325732,#325733,#325734),(#325735,
#325736,#325737),(#325738,#325739,#325740),(#325741,#325742,#325743),(#325744,
#325745,#325746),(#325747,#325748,#325749),(#325750,#325751,#325752),(#325753,
#325754,#325755),(#325756,#325757,#325758),(#325759,#325760,#325761),(#325762,
#325763,#325764),(#325765,#325766,#325767),(#325768,#325769,#325770),(#325771,
#325772,#325773),(#325774,#325775,#325776),(#325777,#325778,#325779),(#325780,
#325781,#325782),(#325783,#325784,#325785),(#325786,#325787,#325788),(#325789,
#325790,#325791),(#325792,#325793,#325794),(#325795,#325796,#325797),(#325798,
#325799,#325800),(#325801,#325802,#325803),(#325804,#325805,#325806),(#325807,
#325808,#325809),(#325810,#325811,#325812),(#325813,#325814,#325815),(#325816,
#325817,#325818),(#325819,#325820,#325821),(#325822,#325823,#325824),(#325825,
#325826,#325827),(#325828,#325829,#325830),(#325831,#325832,#325833),(#325834,
#325835,#325836),(#325837,#325838,#325839),(#325840,#325841,#325842),(#325843,
#325844,#325845),(#325846,#325847,#325848),(#325849,#325850,#325851),(#325852,
#325853,#325854),(#325855,#325856,#325857),(#325858,#325859,#325860),(#325861,
#325862,#325863),(#325864,#325865,#325866),(#325867,#325868,#325869),(#325870,
#325871,#325872),(#325873,#325874,#325875),(#325876,#325877,#325878),(#325879,
#325880,#325881),(#325882,#325883,#325884),(#325885,#325886,#325887),(#325888,
#325889,#325890),(#325891,#325892,#325893),(#325894,#325895,#325896),(#325897,
#325898,#325899),(#325900,#325901,#325902),(#325903,#325904,#325905),(#325906,
#325907,#325908),(#325909,#325910,#325911),(#325912,#325913,#325914),(#325915,
#325916,#325917),(#325918,#325919,#325920),(#325921,#325922,#325923),(#325924,
#325925,#325926),(#325927,#325928,#325929),(#325930,#325931,#325932),(#325933,
#325934,#325935),(#325936,#325937,#325938),(#325939,#325940,#325941),(#325942,
#325943,#325944),(#325945,#325946,#325947),(#325948,#325949,#325950),(#325951,
#325952,#325953),(#325954,#325955,#325956),(#325957,#325958,#325959),(#325960,
#325961,#325962),(#325963,#325964,#325965),(#325966,#325967,#325968),(#325969,
#325970,#325971),(#325972,#325973,#325974),(#325975,#325976,#325977),(#325978,
#325979,#325980),(#325981,#325982,#325983),(#325984,#325985,#325986),(#325987,
#325988,#325989),(#325990,#325991,#325992),(#325993,#325994,#325995),(#325996,
#325997,#325998),(#325999,#326000,#326001),(#326002,#326003,#326004),(#326005,
#326006,#326007),(#326008,#326009,#326010),(#326011,#326012,#326013),(#326014,
#326015,#326016),(#326017,#326018,#326019),(#326020,#326021,#326022),(#326023,
#326024,#326025),(#326026,#326027,#326028),(#326029,#326030,#326031),(#326032,
#326033,#326034),(#326035,#326036,#326037),(#326038,#326039,#326040),(#326041,
#326042,#326043),(#326044,#326045,#326046),(#326047,#326048,#326049),(#326050,
#326051,#326052),(#326053,#326054,#326055),(#326056,#326057,#326058),(#326059,
#326060,#326061),(#326062,#326063,#326064),(#326065,#326066,#326067),(#326068,
#326069,#326070),(#326071,#326072,#326073),(#326074,#326075,#326076),(#326077,
#326078,#326079),(#326080,#326081,#326082),(#326083,#326084,#326085),(#326086,
#326087,#326088),(#326089,#326090,#326091),(#326092,#326093,#326094),(#326095,
#326096,#326097),(#326098,#326099,#326100),(#326101,#326102,#326103),(#326104,
#326105,#326106),(#326107,#326108,#326109),(#326110,#326111,#326112),(#326113,
#326114,#326115),(#326116,#326117,#326118),(#326119,#326120,#326121),(#326122,
#326123,#326124),(#326125,#326126,#326127),(#326128,#326129,#326130),(#326131,
#326132,#326133),(#326134,#326135,#326136),(#326137,#326138,#326139),(#326140,
#326141,#326142),(#326143,#326144,#326145),(#326146,#326147,#326148),(#326149,
#326150,#326151),(#326152,#326153,#326154),(#326155,#326156,#326157),(#326158,
#326159,#326160),(#326161,#326162,#326163),(#326164,#326165,#326166),(#326167,
#326168,#326169),(#326170,#326171,#326172),(#326173,#326174,#326175),(#326176,
#326177,#326178),(#326179,#326180,#326181),(#326182,#326183,#326184),(#326185,
#326186,#326187),(#326188,#326189,#326190),(#326191,#326192,#326193),(#326194,
#326195,#326196),(#326197,#326198,#326199),(#326200,#326201,#326202),(#326203,
#326204,#326205),(#326206,#326207,#326208),(#326209,#326210,#326211),(#326212,
#326213,#326214),(#326215,#326216,#326217),(#326218,#326219,#326220),(#326221,
#326222,#326223),(#326224,#326225,#326226),(#326227,#326228,#326229),(#326230,
#326231,#326232),(#326233,#326234,#326235),(#326236,#326237,#326238),(#326239,
#326240,#326241),(#326242,#326243,#326244),(#326245,#326246,#326247),(#326248,
#326249,#326250),(#326251,#326252,#326253),(#326254,#326255,#326256),(#326257,
#326258,#326259),(#326260,#326261,#326262),(#326263,#326264,#326265),(#326266,
#326267,#326268),(#326269,#326270,#326271),(#326272,#326273,#326274),(#326275,
#326276,#326277),(#326278,#326279,#326280),(#326281,#326282,#326283),(#326284,
#326285,#326286),(#326287,#326288,#326289),(#326290,#326291,#326292),(#326293,
#326294,#326295),(#326296,#326297,#326298),(#326299,#326300,#326301),(#326302,
#326303,#326304),(#326305,#326306,#326307),(#326308,#326309,#326310),(#326311,
#326312,#326313),(#326314,#326315,#326316),(#326317,#326318,#326319),(#326320,
#326321,#326322),(#326323,#326324,#326325),(#326326,#326327,#326328),(#326329,
#326330,#326331),(#326332,#326333,#326334),(#326335,#326336,#326337),(#326338,
#326339,#326340),(#326341,#326342,#326343),(#326344,#326345,#326346),(#326347,
#326348,#326349),(#326350,#326351,#326352),(#326353,#326354,#326355)),
 .UNSPECIFIED.,.F.,.F.,.F.,(6,1,1,1,1,1,1,1,1,1,1,1,1,1,1,1,1,1,1,1,1,1,
1,1,1,1,1,1,1,1,1,1,1,1,1,1,1,1,1,1,1,1,1,1,1,1,1,1,1,1,1,1,1,1,1,1,1,1,
1,1,1,1,1,1,1,1,1,1,1,1,1,1,1,1,1,1,1,1,1,1,1,1,1,1,1,1,1,1,1,1,1,1,1,1,
1,1,1,1,1,1,1,1,1,1,1,1,1,1,1,1,1,1,1,1,1,1,1,1,1,1,1,1,1,1,1,1,1,1,1,1,
1,1,1,1,1,1,1,1,1,1,1,1,1,1,1,1,1,1,1,1,1,1,1,1,1,1,1,1,1,1,1,1,1,1,1,1,
1,1,1,1,1,1,1,1,1,1,1,1,1,1,1,1,1,1,1,1,1,1,1,1,1,1,1,1,1,1,1,1,1,1,1,1,
1,1,1,1,1,1,1,1,1,1,1,1,1,1,1,1,1,1,1,1,1,1,1,1,1,1,1,1,1,1,1,1,1,1,1,1,
1,1,1,1,1,1,1,1,1,1,1,1,1,1,1,1,1,1,1,1,1,1,1,1,1,1,1,1,1,1,1,1,1,1,1,1,
1,1,1,1,1,1,1,1,1,1,1,1,1,1,1,1,1,1,1,1,1,1,1,1,1,1,1,1,1,1,1,1,1,1,1,1,
1,1,1,1,1,1,1,1,1,1,1,1,1,1,1,1,1,1,1,1,1,1,1,1,1,1,1,1,1,1,1,1,1,1,1,1,
1,1,1,1,1,1,1,1,1,1,1,1,1,1,1,1,1,1,1,1,1,1,1,1,1,1,1,1,1,1,1,1,1,1,1,1,
1,1,1,1,1,1,1,1,1,1,1,1,1,1,1,1,1,1,1,1,1,1,1,1,1,1,1,1,1,1,1,1,1,1,1,1,
1,1,1,1,1,1,1,1,1,1,1,1,1,1,1,1,1,1,1,1,1,1,1,1,1,1,1,1,1,1,1,1,1,1,1,1,
1,1,1,1,1,1,1,1,1,1,1,1,1,1,1,1,1,1,1,1,1,1,1,1,1,1,1,1,1,1,1,1,1,1,1,1,
1,1,1,1,1,1,1,1,1,1,1,1,1,1,1,1,1,1,1,1,1,1,1,1,1,1,1,1,1,1,1,1,1,1,1,1,
1,1,1,1,1,1,1,1,1,1,1,1,1,1,1,1,1,1,1,6),(2,1,2),(-1.,-0.998165138,-0.996330275,
-0.994495413,-0.99266055,-0.990825688,-0.988990826,-0.987155963,-0.985321101,
-0.983486239,-0.981651376,-0.979816514,-0.977981651,-0.976146789,-0.974311927,
-0.972477064,-0.970642202,-0.968807339,-0.966972477,-0.965137615,-0.963302752,
-0.96146789,-0.959633028,-0.957798165,-0.955963303,-0.95412844,-0.952293578,
-0.950458716,-0.948623853,-0.946788991,-0.944954128,-0.943119266,-0.941284404,
-0.939449541,-0.937614679,-0.935779817,-0.933944954,-0.932110092,-0.930275229,
-0.928440367,-0.926605505,-0.924770642,-0.92293578,-0.921100917,-0.919266055,
-0.917431193,-0.91559633,-0.913761468,-0.911926606,-0.910091743,-0.908256881,
-0.906422018,-0.904587156,-0.902752294,-0.900917431,-0.899082569,-0.897247706,
-0.895412844,-0.893577982,-0.891743119,-0.889908257,-0.888073394,-0.886238532,
-0.88440367,-0.882568807,-0.880733945,-0.878899083,-0.87706422,-0.875229358,
-0.873394495,-0.871559633,-0.869724771,-0.867889908,-0.866055046,-0.864220183,
-0.862385321,-0.860550459,-0.858715596,-0.856880734,-0.855045872,-0.853211009,
-0.851376147,-0.849541284,-0.847706422,-0.84587156,-0.844036697,-0.842201835,
-0.840366972,-0.83853211,-0.836697248,-0.834862385,-0.833027523,-0.831192661,
-0.829357798,-0.827522936,-0.825688073,-0.823853211,-0.822018349,-0.820183486,
-0.818348624,-0.816513761,-0.814678899,-0.812844037,-0.811009174,-0.809174312,
-0.80733945,-0.805504587,-0.803669725,-0.801834862,-0.8,-0.798165138,-0.796330275,
-0.794495413,-0.79266055,-0.790825688,-0.788990826,-0.787155963,-0.785321101,
-0.783486239,-0.781651376,-0.779816514,-0.777981651,-0.776146789,-0.774311927,
-0.772477064,-0.770642202,-0.768807339,-0.766972477,-0.765137615,-0.763302752,
-0.76146789,-0.759633028,-0.757798165,-0.755963303,-0.75412844,-0.752293578,
-0.750458716,-0.748623853,-0.746788991,-0.744954128,-0.743119266,-0.741284404,
-0.739449541,-0.737614679,-0.735779817,-0.733944954,-0.732110092,-0.730275229,
-0.728440367,-0.726605505,-0.724770642,-0.72293578,-0.721100917,-0.719266055,
-0.717431193,-0.71559633,-0.713761468,-0.711926606,-0.710091743,-0.708256881,
-0.706422018,-0.704587156,-0.702752294,-0.700917431,-0.699082569,-0.697247706,
-0.695412844,-0.693577982,-0.691743119,-0.689908257,-0.688073394,-0.686238532,
-0.68440367,-0.682568807,-0.680733945,-0.678899083,-0.67706422,-0.675229358,
-0.673394495,-0.671559633,-0.669724771,-0.667889908,-0.666055046,-0.664220183,
-0.662385321,-0.660550459,-0.658715596,-0.656880734,-0.655045872,-0.653211009,
-0.651376147,-0.649541284,-0.647706422,-0.64587156,-0.644036697,-0.642201835,
-0.640366972,-0.63853211,-0.636697248,-0.634862385,-0.633027523,-0.631192661,
-0.629357798,-0.627522936,-0.625688073,-0.623853211,-0.622018349,-0.620183486,
-0.618348624,-0.616513761,-0.614678899,-0.612844037,-0.611009174,-0.609174312,
-0.60733945,-0.605504587,-0.603669725,-0.601834862,-0.6,-0.598165138,-0.596330275,
-0.594495413,-0.59266055,-0.590825688,-0.588990826,-0.587155963,-0.585321101,
-0.583486239,-0.581651376,-0.579816514,-0.577981651,-0.576146789,-0.574311927,
-0.572477064,-0.570642202,-0.568807339,-0.566972477,-0.565137615,-0.563302752,
-0.56146789,-0.559633028,-0.557798165,-0.555963303,-0.55412844,-0.552293578,
-0.550458716,-0.548623853,-0.546788991,-0.544954128,-0.543119266,-0.541284404,
-0.539449541,-0.537614679,-0.535779817,-0.533944954,-0.532110092,-0.530275229,
-0.528440367,-0.526605505,-0.524770642,-0.52293578,-0.521100917,-0.519266055,
-0.517431193,-0.51559633,-0.513761468,-0.511926606,-0.510091743,-0.508256881,
-0.506422018,-0.504587156,-0.502752294,-0.500917431,-0.499082569,-0.497247706,
-0.495412844,-0.493577982,-0.491743119,-0.489908257,-0.488073394,-0.486238532,
-0.48440367,-0.482568807,-0.480733945,-0.478899083,-0.47706422,-0.475229358,
-0.473394495,-0.471559633,-0.469724771,-0.467889908,-0.466055046,-0.464220183,
-0.462385321,-0.460550459,-0.458715596,-0.456880734,-0.455045872,-0.453211009,
-0.451376147,-0.449541284,-0.447706422,-0.44587156,-0.444036697,-0.442201835,
-0.440366972,-0.43853211,-0.436697248,-0.434862385,-0.433027523,-0.431192661,
-0.429357798,-0.427522936,-0.425688073,-0.423853211,-0.422018349,-0.420183486,
-0.418348624,-0.416513761,-0.414678899,-0.412844037,-0.411009174,-0.409174312,
-0.40733945,-0.405504587,-0.403669725,-0.401834862,-0.4,-0.398165138,-0.396330275,
-0.394495413,-0.39266055,-0.390825688,-0.388990826,-0.387155963,-0.385321101,
-0.383486239,-0.381651376,-0.379816514,-0.377981651,-0.376146789,-0.374311927,
-0.372477064,-0.370642202,-0.368807339,-0.366972477,-0.365137615,-0.363302752,
-0.36146789,-0.359633028,-0.357798165,-0.355963303,-0.35412844,-0.352293578,
-0.350458716,-0.348623853,-0.346788991,-0.344954128,-0.343119266,-0.341284404,
-0.339449541,-0.337614679,-0.335779817,-0.333944954,-0.332110092,-0.330275229,
-0.328440367,-0.326605505,-0.324770642,-0.32293578,-0.321100917,-0.319266055,
-0.317431193,-0.31559633,-0.313761468,-0.311926606,-0.310091743,-0.308256881,
-0.306422018,-0.304587156,-0.302752294,-0.300917431,-0.299082569,-0.297247706,
-0.295412844,-0.293577982,-0.291743119,-0.289908257,-0.288073394,-0.286238532,
-0.28440367,-0.282568807,-0.280733945,-0.278899083,-0.27706422,-0.275229358,
-0.273394495,-0.271559633,-0.269724771,-0.267889908,-0.266055046,-0.264220183,
-0.262385321,-0.260550459,-0.258715596,-0.256880734,-0.255045872,-0.253211009,
-0.251376147,-0.249541284,-0.247706422,-0.24587156,-0.244036697,-0.242201835,
-0.240366972,-0.23853211,-0.236697248,-0.234862385,-0.233027523,-0.231192661,
-0.229357798,-0.227522936,-0.225688073,-0.223853211,-0.222018349,-0.220183486,
-0.218348624,-0.216513761,-0.214678899,-0.212844037,-0.211009174,-0.209174312,
-0.20733945,-0.205504587,-0.203669725,-0.201834862,-0.2,-0.198165138,-0.196330275,
-0.194495413,-0.19266055,-0.190825688,-0.188990826,-0.187155963,-0.185321101,
-0.183486239,-0.181651376,-0.179816514,-0.177981651,-0.176146789,-0.174311927,
-0.172477064,-0.170642202,-0.168807339,-0.166972477,-0.165137615,-0.163302752,
-0.16146789,-0.159633028,-0.157798165,-0.155963303,-0.15412844,-0.152293578,
-0.150458716,-0.148623853,-0.146788991,-0.144954128,-0.143119266,-0.141284404,
-0.139449541,-0.137614679,-0.135779817,-0.133944954,-0.132110092,-0.130275229,
-0.128440367,-0.126605505,-0.124770642,-0.12293578,-0.121100917,-0.119266055,
-0.117431193,-0.11559633,-0.113761468,-0.111926606,-0.110091743,-0.108256881,
-0.106422018,-0.104587156,-0.102752294,-0.100917431,-0.099082569,-0.097247706,
-0.095412844,-0.093577982,-0.091743119,-0.089908257,-0.088073394,-0.086238532,
-0.08440367,-0.082568807,-0.080733945,-0.078899083,-0.07706422,-0.075229358,
-0.073394495,-0.071559633,-0.069724771,-0.067889908,-0.066055046,-0.064220183,
-0.062385321,-0.060550459,-0.058715596,-0.056880734,-0.055045872,-0.053211009,
-0.051376147,-0.049541284,-0.047706422,-0.04587156,-0.044036697,-0.042201835,
-0.040366972,-0.03853211,-0.036697248,-0.034862385,-0.033027523,-0.031192661,
-0.029357798,-0.027522936,-0.025688073,-0.023853211,-0.022018349,-0.020183486,
-0.018348624,-0.016513761,-0.014678899,-0.012844037,-0.011009174,-0.009174312,
-0.00733945,-0.005504587,-0.003669725,-0.001834862,0.000982147),(0.3,1.,
1.3),.UNSPECIFIED.);
#6318=B_SPLINE_SURFACE_WITH_KNOTS('',5,1,((#326378,#326379,#326380),(#326381,
#326382,#326383),(#326384,#326385,#326386),(#326387,#326388,#326389),(#326390,
#326391,#326392),(#326393,#326394,#326395),(#326396,#326397,#326398),(#326399,
#326400,#326401),(#326402,#326403,#326404),(#326405,#326406,#326407),(#326408,
#326409,#326410),(#326411,#326412,#326413),(#326414,#326415,#326416),(#326417,
#326418,#326419),(#326420,#326421,#326422),(#326423,#326424,#326425),(#326426,
#326427,#326428),(#326429,#326430,#326431),(#326432,#326433,#326434),(#326435,
#326436,#326437),(#326438,#326439,#326440),(#326441,#326442,#326443),(#326444,
#326445,#326446),(#326447,#326448,#326449),(#326450,#326451,#326452),(#326453,
#326454,#326455),(#326456,#326457,#326458),(#326459,#326460,#326461),(#326462,
#326463,#326464),(#326465,#326466,#326467),(#326468,#326469,#326470),(#326471,
#326472,#326473),(#326474,#326475,#326476),(#326477,#326478,#326479),(#326480,
#326481,#326482),(#326483,#326484,#326485),(#326486,#326487,#326488),(#326489,
#326490,#326491),(#326492,#326493,#326494),(#326495,#326496,#326497),(#326498,
#326499,#326500),(#326501,#326502,#326503),(#326504,#326505,#326506),(#326507,
#326508,#326509),(#326510,#326511,#326512),(#326513,#326514,#326515),(#326516,
#326517,#326518),(#326519,#326520,#326521),(#326522,#326523,#326524),(#326525,
#326526,#326527),(#326528,#326529,#326530),(#326531,#326532,#326533),(#326534,
#326535,#326536),(#326537,#326538,#326539),(#326540,#326541,#326542),(#326543,
#326544,#326545),(#326546,#326547,#326548),(#326549,#326550,#326551),(#326552,
#326553,#326554),(#326555,#326556,#326557),(#326558,#326559,#326560),(#326561,
#326562,#326563),(#326564,#326565,#326566),(#326567,#326568,#326569),(#326570,
#326571,#326572),(#326573,#326574,#326575),(#326576,#326577,#326578),(#326579,
#326580,#326581),(#326582,#326583,#326584),(#326585,#326586,#326587),(#326588,
#326589,#326590),(#326591,#326592,#326593),(#326594,#326595,#326596),(#326597,
#326598,#326599),(#326600,#326601,#326602),(#326603,#326604,#326605),(#326606,
#326607,#326608),(#326609,#326610,#326611),(#326612,#326613,#326614),(#326615,
#326616,#326617),(#326618,#326619,#326620),(#326621,#326622,#326623),(#326624,
#326625,#326626),(#326627,#326628,#326629),(#326630,#326631,#326632),(#326633,
#326634,#326635),(#326636,#326637,#326638),(#326639,#326640,#326641),(#326642,
#326643,#326644),(#326645,#326646,#326647),(#326648,#326649,#326650),(#326651,
#326652,#326653),(#326654,#326655,#326656),(#326657,#326658,#326659),(#326660,
#326661,#326662),(#326663,#326664,#326665),(#326666,#326667,#326668),(#326669,
#326670,#326671),(#326672,#326673,#326674),(#326675,#326676,#326677),(#326678,
#326679,#326680),(#326681,#326682,#326683),(#326684,#326685,#326686),(#326687,
#326688,#326689),(#326690,#326691,#326692),(#326693,#326694,#326695),(#326696,
#326697,#326698),(#326699,#326700,#326701),(#326702,#326703,#326704),(#326705,
#326706,#326707),(#326708,#326709,#326710),(#326711,#326712,#326713),(#326714,
#326715,#326716),(#326717,#326718,#326719),(#326720,#326721,#326722),(#326723,
#326724,#326725),(#326726,#326727,#326728),(#326729,#326730,#326731),(#326732,
#326733,#326734),(#326735,#326736,#326737),(#326738,#326739,#326740),(#326741,
#326742,#326743),(#326744,#326745,#326746),(#326747,#326748,#326749),(#326750,
#326751,#326752),(#326753,#326754,#326755),(#326756,#326757,#326758),(#326759,
#326760,#326761),(#326762,#326763,#326764),(#326765,#326766,#326767),(#326768,
#326769,#326770),(#326771,#326772,#326773),(#326774,#326775,#326776),(#326777,
#326778,#326779),(#326780,#326781,#326782),(#326783,#326784,#326785),(#326786,
#326787,#326788),(#326789,#326790,#326791),(#326792,#326793,#326794),(#326795,
#326796,#326797),(#326798,#326799,#326800),(#326801,#326802,#326803),(#326804,
#326805,#326806),(#326807,#326808,#326809),(#326810,#326811,#326812),(#326813,
#326814,#326815),(#326816,#326817,#326818),(#326819,#326820,#326821),(#326822,
#326823,#326824),(#326825,#326826,#326827),(#326828,#326829,#326830),(#326831,
#326832,#326833),(#326834,#326835,#326836),(#326837,#326838,#326839),(#326840,
#326841,#326842),(#326843,#326844,#326845),(#326846,#326847,#326848),(#326849,
#326850,#326851),(#326852,#326853,#326854),(#326855,#326856,#326857),(#326858,
#326859,#326860),(#326861,#326862,#326863),(#326864,#326865,#326866),(#326867,
#326868,#326869),(#326870,#326871,#326872),(#326873,#326874,#326875),(#326876,
#326877,#326878),(#326879,#326880,#326881),(#326882,#326883,#326884),(#326885,
#326886,#326887),(#326888,#326889,#326890),(#326891,#326892,#326893),(#326894,
#326895,#326896),(#326897,#326898,#326899),(#326900,#326901,#326902),(#326903,
#326904,#326905),(#326906,#326907,#326908),(#326909,#326910,#326911),(#326912,
#326913,#326914),(#326915,#326916,#326917),(#326918,#326919,#326920),(#326921,
#326922,#326923),(#326924,#326925,#326926),(#326927,#326928,#326929),(#326930,
#326931,#326932),(#326933,#326934,#326935),(#326936,#326937,#326938),(#326939,
#326940,#326941),(#326942,#326943,#326944),(#326945,#326946,#326947),(#326948,
#326949,#326950),(#326951,#326952,#326953),(#326954,#326955,#326956),(#326957,
#326958,#326959),(#326960,#326961,#326962),(#326963,#326964,#326965),(#326966,
#326967,#326968),(#326969,#326970,#326971),(#326972,#326973,#326974),(#326975,
#326976,#326977),(#326978,#326979,#326980),(#326981,#326982,#326983),(#326984,
#326985,#326986),(#326987,#326988,#326989),(#326990,#326991,#326992),(#326993,
#326994,#326995),(#326996,#326997,#326998),(#326999,#327000,#327001),(#327002,
#327003,#327004),(#327005,#327006,#327007),(#327008,#327009,#327010),(#327011,
#327012,#327013),(#327014,#327015,#327016),(#327017,#327018,#327019),(#327020,
#327021,#327022),(#327023,#327024,#327025),(#327026,#327027,#327028),(#327029,
#327030,#327031),(#327032,#327033,#327034),(#327035,#327036,#327037),(#327038,
#327039,#327040),(#327041,#327042,#327043),(#327044,#327045,#327046),(#327047,
#327048,#327049),(#327050,#327051,#327052),(#327053,#327054,#327055),(#327056,
#327057,#327058),(#327059,#327060,#327061),(#327062,#327063,#327064),(#327065,
#327066,#327067),(#327068,#327069,#327070),(#327071,#327072,#327073),(#327074,
#327075,#327076),(#327077,#327078,#327079),(#327080,#327081,#327082),(#327083,
#327084,#327085),(#327086,#327087,#327088),(#327089,#327090,#327091),(#327092,
#327093,#327094),(#327095,#327096,#327097),(#327098,#327099,#327100),(#327101,
#327102,#327103),(#327104,#327105,#327106),(#327107,#327108,#327109),(#327110,
#327111,#327112),(#327113,#327114,#327115),(#327116,#327117,#327118),(#327119,
#327120,#327121),(#327122,#327123,#327124),(#327125,#327126,#327127),(#327128,
#327129,#327130),(#327131,#327132,#327133),(#327134,#327135,#327136),(#327137,
#327138,#327139),(#327140,#327141,#327142),(#327143,#327144,#327145),(#327146,
#327147,#327148),(#327149,#327150,#327151),(#327152,#327153,#327154),(#327155,
#327156,#327157),(#327158,#327159,#327160),(#327161,#327162,#327163),(#327164,
#327165,#327166),(#327167,#327168,#327169),(#327170,#327171,#327172),(#327173,
#327174,#327175),(#327176,#327177,#327178),(#327179,#327180,#327181),(#327182,
#327183,#327184),(#327185,#327186,#327187),(#327188,#327189,#327190),(#327191,
#327192,#327193),(#327194,#327195,#327196),(#327197,#327198,#327199),(#327200,
#327201,#327202),(#327203,#327204,#327205),(#327206,#327207,#327208),(#327209,
#327210,#327211),(#327212,#327213,#327214),(#327215,#327216,#327217),(#327218,
#327219,#327220),(#327221,#327222,#327223),(#327224,#327225,#327226),(#327227,
#327228,#327229),(#327230,#327231,#327232),(#327233,#327234,#327235),(#327236,
#327237,#327238),(#327239,#327240,#327241),(#327242,#327243,#327244),(#327245,
#327246,#327247),(#327248,#327249,#327250),(#327251,#327252,#327253),(#327254,
#327255,#327256),(#327257,#327258,#327259),(#327260,#327261,#327262),(#327263,
#327264,#327265),(#327266,#327267,#327268),(#327269,#327270,#327271),(#327272,
#327273,#327274),(#327275,#327276,#327277),(#327278,#327279,#327280),(#327281,
#327282,#327283),(#327284,#327285,#327286),(#327287,#327288,#327289),(#327290,
#327291,#327292),(#327293,#327294,#327295),(#327296,#327297,#327298),(#327299,
#327300,#327301),(#327302,#327303,#327304),(#327305,#327306,#327307),(#327308,
#327309,#327310),(#327311,#327312,#327313),(#327314,#327315,#327316),(#327317,
#327318,#327319),(#327320,#327321,#327322),(#327323,#327324,#327325),(#327326,
#327327,#327328),(#327329,#327330,#327331),(#327332,#327333,#327334),(#327335,
#327336,#327337),(#327338,#327339,#327340),(#327341,#327342,#327343),(#327344,
#327345,#327346),(#327347,#327348,#327349),(#327350,#327351,#327352),(#327353,
#327354,#327355),(#327356,#327357,#327358),(#327359,#327360,#327361),(#327362,
#327363,#327364),(#327365,#327366,#327367),(#327368,#327369,#327370),(#327371,
#327372,#327373),(#327374,#327375,#327376),(#327377,#327378,#327379),(#327380,
#327381,#327382),(#327383,#327384,#327385),(#327386,#327387,#327388),(#327389,
#327390,#327391),(#327392,#327393,#327394),(#327395,#327396,#327397),(#327398,
#327399,#327400),(#327401,#327402,#327403),(#327404,#327405,#327406),(#327407,
#327408,#327409),(#327410,#327411,#327412),(#327413,#327414,#327415),(#327416,
#327417,#327418),(#327419,#327420,#327421),(#327422,#327423,#327424),(#327425,
#327426,#327427),(#327428,#327429,#327430),(#327431,#327432,#327433),(#327434,
#327435,#327436),(#327437,#327438,#327439),(#327440,#327441,#327442),(#327443,
#327444,#327445),(#327446,#327447,#327448),(#327449,#327450,#327451),(#327452,
#327453,#327454),(#327455,#327456,#327457),(#327458,#327459,#327460),(#327461,
#327462,#327463),(#327464,#327465,#327466),(#327467,#327468,#327469),(#327470,
#327471,#327472),(#327473,#327474,#327475),(#327476,#327477,#327478),(#327479,
#327480,#327481),(#327482,#327483,#327484),(#327485,#327486,#327487),(#327488,
#327489,#327490),(#327491,#327492,#327493),(#327494,#327495,#327496),(#327497,
#327498,#327499),(#327500,#327501,#327502),(#327503,#327504,#327505),(#327506,
#327507,#327508),(#327509,#327510,#327511),(#327512,#327513,#327514),(#327515,
#327516,#327517),(#327518,#327519,#327520),(#327521,#327522,#327523),(#327524,
#327525,#327526),(#327527,#327528,#327529),(#327530,#327531,#327532),(#327533,
#327534,#327535),(#327536,#327537,#327538),(#327539,#327540,#327541),(#327542,
#327543,#327544),(#327545,#327546,#327547),(#327548,#327549,#327550),(#327551,
#327552,#327553),(#327554,#327555,#327556),(#327557,#327558,#327559),(#327560,
#327561,#327562),(#327563,#327564,#327565),(#327566,#327567,#327568),(#327569,
#327570,#327571),(#327572,#327573,#327574),(#327575,#327576,#327577),(#327578,
#327579,#327580),(#327581,#327582,#327583),(#327584,#327585,#327586),(#327587,
#327588,#327589),(#327590,#327591,#327592),(#327593,#327594,#327595),(#327596,
#327597,#327598),(#327599,#327600,#327601),(#327602,#327603,#327604),(#327605,
#327606,#327607),(#327608,#327609,#327610),(#327611,#327612,#327613),(#327614,
#327615,#327616),(#327617,#327618,#327619),(#327620,#327621,#327622),(#327623,
#327624,#327625),(#327626,#327627,#327628),(#327629,#327630,#327631),(#327632,
#327633,#327634),(#327635,#327636,#327637),(#327638,#327639,#327640),(#327641,
#327642,#327643),(#327644,#327645,#327646),(#327647,#327648,#327649),(#327650,
#327651,#327652),(#327653,#327654,#327655),(#327656,#327657,#327658),(#327659,
#327660,#327661),(#327662,#327663,#327664),(#327665,#327666,#327667),(#327668,
#327669,#327670),(#327671,#327672,#327673),(#327674,#327675,#327676),(#327677,
#327678,#327679),(#327680,#327681,#327682),(#327683,#327684,#327685),(#327686,
#327687,#327688),(#327689,#327690,#327691),(#327692,#327693,#327694),(#327695,
#327696,#327697),(#327698,#327699,#327700),(#327701,#327702,#327703),(#327704,
#327705,#327706),(#327707,#327708,#327709),(#327710,#327711,#327712),(#327713,
#327714,#327715),(#327716,#327717,#327718),(#327719,#327720,#327721),(#327722,
#327723,#327724),(#327725,#327726,#327727),(#327728,#327729,#327730),(#327731,
#327732,#327733),(#327734,#327735,#327736),(#327737,#327738,#327739),(#327740,
#327741,#327742),(#327743,#327744,#327745),(#327746,#327747,#327748),(#327749,
#327750,#327751),(#327752,#327753,#327754),(#327755,#327756,#327757),(#327758,
#327759,#327760),(#327761,#327762,#327763),(#327764,#327765,#327766),(#327767,
#327768,#327769),(#327770,#327771,#327772),(#327773,#327774,#327775),(#327776,
#327777,#327778),(#327779,#327780,#327781),(#327782,#327783,#327784),(#327785,
#327786,#327787),(#327788,#327789,#327790),(#327791,#327792,#327793),(#327794,
#327795,#327796),(#327797,#327798,#327799),(#327800,#327801,#327802),(#327803,
#327804,#327805),(#327806,#327807,#327808),(#327809,#327810,#327811),(#327812,
#327813,#327814),(#327815,#327816,#327817),(#327818,#327819,#327820),(#327821,
#327822,#327823),(#327824,#327825,#327826),(#327827,#327828,#327829),(#327830,
#327831,#327832),(#327833,#327834,#327835),(#327836,#327837,#327838),(#327839,
#327840,#327841),(#327842,#327843,#327844),(#327845,#327846,#327847),(#327848,
#327849,#327850),(#327851,#327852,#327853),(#327854,#327855,#327856),(#327857,
#327858,#327859),(#327860,#327861,#327862),(#327863,#327864,#327865),(#327866,
#327867,#327868),(#327869,#327870,#327871),(#327872,#327873,#327874),(#327875,
#327876,#327877),(#327878,#327879,#327880),(#327881,#327882,#327883),(#327884,
#327885,#327886),(#327887,#327888,#327889),(#327890,#327891,#327892),(#327893,
#327894,#327895),(#327896,#327897,#327898),(#327899,#327900,#327901),(#327902,
#327903,#327904),(#327905,#327906,#327907),(#327908,#327909,#327910),(#327911,
#327912,#327913),(#327914,#327915,#327916),(#327917,#327918,#327919),(#327920,
#327921,#327922),(#327923,#327924,#327925),(#327926,#327927,#327928),(#327929,
#327930,#327931),(#327932,#327933,#327934),(#327935,#327936,#327937),(#327938,
#327939,#327940),(#327941,#327942,#327943),(#327944,#327945,#327946),(#327947,
#327948,#327949),(#327950,#327951,#327952),(#327953,#327954,#327955),(#327956,
#327957,#327958),(#327959,#327960,#327961),(#327962,#327963,#327964),(#327965,
#327966,#327967),(#327968,#327969,#327970),(#327971,#327972,#327973),(#327974,
#327975,#327976),(#327977,#327978,#327979),(#327980,#327981,#327982),(#327983,
#327984,#327985),(#327986,#327987,#327988),(#327989,#327990,#327991),(#327992,
#327993,#327994),(#327995,#327996,#327997),(#327998,#327999,#328000),(#328001,
#328002,#328003),(#328004,#328005,#328006),(#328007,#328008,#328009),(#328010,
#328011,#328012),(#328013,#328014,#328015),(#328016,#328017,#328018),(#328019,
#328020,#328021),(#328022,#328023,#328024),(#328025,#328026,#328027),(#328028,
#328029,#328030)),.UNSPECIFIED.,.F.,.F.,.F.,(6,1,1,1,1,1,1,1,1,1,1,1,1,
1,1,1,1,1,1,1,1,1,1,1,1,1,1,1,1,1,1,1,1,1,1,1,1,1,1,1,1,1,1,1,1,1,1,1,1,
1,1,1,1,1,1,1,1,1,1,1,1,1,1,1,1,1,1,1,1,1,1,1,1,1,1,1,1,1,1,1,1,1,1,1,1,
1,1,1,1,1,1,1,1,1,1,1,1,1,1,1,1,1,1,1,1,1,1,1,1,1,1,1,1,1,1,1,1,1,1,1,1,
1,1,1,1,1,1,1,1,1,1,1,1,1,1,1,1,1,1,1,1,1,1,1,1,1,1,1,1,1,1,1,1,1,1,1,1,
1,1,1,1,1,1,1,1,1,1,1,1,1,1,1,1,1,1,1,1,1,1,1,1,1,1,1,1,1,1,1,1,1,1,1,1,
1,1,1,1,1,1,1,1,1,1,1,1,1,1,1,1,1,1,1,1,1,1,1,1,1,1,1,1,1,1,1,1,1,1,1,1,
1,1,1,1,1,1,1,1,1,1,1,1,1,1,1,1,1,1,1,1,1,1,1,1,1,1,1,1,1,1,1,1,1,1,1,1,
1,1,1,1,1,1,1,1,1,1,1,1,1,1,1,1,1,1,1,1,1,1,1,1,1,1,1,1,1,1,1,1,1,1,1,1,
1,1,1,1,1,1,1,1,1,1,1,1,1,1,1,1,1,1,1,1,1,1,1,1,1,1,1,1,1,1,1,1,1,1,1,1,
1,1,1,1,1,1,1,1,1,1,1,1,1,1,1,1,1,1,1,1,1,1,1,1,1,1,1,1,1,1,1,1,1,1,1,1,
1,1,1,1,1,1,1,1,1,1,1,1,1,1,1,1,1,1,1,1,1,1,1,1,1,1,1,1,1,1,1,1,1,1,1,1,
1,1,1,1,1,1,1,1,1,1,1,1,1,1,1,1,1,1,1,1,1,1,1,1,1,1,1,1,1,1,1,1,1,1,1,1,
1,1,1,1,1,1,1,1,1,1,1,1,1,1,1,1,1,1,1,1,1,1,1,1,1,1,1,1,1,1,1,1,1,1,1,1,
1,1,1,1,1,1,1,1,1,1,1,1,1,1,1,1,1,1,1,1,1,1,1,1,1,1,1,1,1,1,1,1,1,1,1,1,
1,1,1,1,1,1,1,1,1,1,1,1,1,1,1,1,1,1,1,1,1,1,1,1,1,1,1,1,1,6),(2,1,2),(-0.001964192,
0.,0.001834862,0.003669725,0.005504587,0.00733945,0.009174312,0.011009174,
0.012844037,0.014678899,0.016513761,0.018348624,0.020183486,0.022018349,
0.023853211,0.025688073,0.027522936,0.029357798,0.031192661,0.033027523,
0.034862385,0.036697248,0.03853211,0.040366972,0.042201835,0.044036697,
0.04587156,0.047706422,0.049541284,0.051376147,0.053211009,0.055045872,
0.056880734,0.058715596,0.060550459,0.062385321,0.064220183,0.066055046,
0.067889908,0.069724771,0.071559633,0.073394495,0.075229358,0.07706422,
0.078899083,0.080733945,0.082568807,0.08440367,0.086238532,0.088073394,
0.089908257,0.091743119,0.093577982,0.095412844,0.097247706,0.099082569,
0.100917431,0.102752294,0.104587156,0.106422018,0.108256881,0.110091743,
0.111926606,0.113761468,0.11559633,0.117431193,0.119266055,0.121100917,
0.12293578,0.124770642,0.126605505,0.128440367,0.130275229,0.132110092,
0.133944954,0.135779817,0.137614679,0.139449541,0.141284404,0.143119266,
0.144954128,0.146788991,0.148623853,0.150458716,0.152293578,0.15412844,
0.155963303,0.157798165,0.159633028,0.16146789,0.163302752,0.165137615,
0.166972477,0.168807339,0.170642202,0.172477064,0.174311927,0.176146789,
0.177981651,0.179816514,0.181651376,0.183486239,0.185321101,0.187155963,
0.188990826,0.190825688,0.19266055,0.194495413,0.196330275,0.198165138,
0.2,0.201834862,0.203669725,0.205504587,0.20733945,0.209174312,0.211009174,
0.212844037,0.214678899,0.216513761,0.218348624,0.220183486,0.222018349,
0.223853211,0.225688073,0.227522936,0.229357798,0.231192661,0.233027523,
0.234862385,0.236697248,0.23853211,0.240366972,0.242201835,0.244036697,
0.24587156,0.247706422,0.249541284,0.251376147,0.253211009,0.255045872,
0.256880734,0.258715596,0.260550459,0.262385321,0.264220183,0.266055046,
0.267889908,0.269724771,0.271559633,0.273394495,0.275229358,0.27706422,
0.278899083,0.280733945,0.282568807,0.28440367,0.286238532,0.288073394,
0.289908257,0.291743119,0.293577982,0.295412844,0.297247706,0.299082569,
0.300917431,0.302752294,0.304587156,0.306422018,0.308256881,0.310091743,
0.311926606,0.313761468,0.31559633,0.317431193,0.319266055,0.321100917,
0.32293578,0.324770642,0.326605505,0.328440367,0.330275229,0.332110092,
0.333944954,0.335779817,0.337614679,0.339449541,0.341284404,0.343119266,
0.344954128,0.346788991,0.348623853,0.350458716,0.352293578,0.35412844,
0.355963303,0.357798165,0.359633028,0.36146789,0.363302752,0.365137615,
0.366972477,0.368807339,0.370642202,0.372477064,0.374311927,0.376146789,
0.377981651,0.379816514,0.381651376,0.383486239,0.385321101,0.387155963,
0.388990826,0.390825688,0.39266055,0.394495413,0.396330275,0.398165138,
0.4,0.401834862,0.403669725,0.405504587,0.40733945,0.409174312,0.411009174,
0.412844037,0.414678899,0.416513761,0.418348624,0.420183486,0.422018349,
0.423853211,0.425688073,0.427522936,0.429357798,0.431192661,0.433027523,
0.434862385,0.436697248,0.43853211,0.440366972,0.442201835,0.444036697,
0.44587156,0.447706422,0.449541284,0.451376147,0.453211009,0.455045872,
0.456880734,0.458715596,0.460550459,0.462385321,0.464220183,0.466055046,
0.467889908,0.469724771,0.471559633,0.473394495,0.475229358,0.47706422,
0.478899083,0.480733945,0.482568807,0.48440367,0.486238532,0.488073394,
0.489908257,0.491743119,0.493577982,0.495412844,0.497247706,0.499082569,
0.500917431,0.502752294,0.504587156,0.506422018,0.508256881,0.510091743,
0.511926606,0.513761468,0.51559633,0.517431193,0.519266055,0.521100917,
0.52293578,0.524770642,0.526605505,0.528440367,0.530275229,0.532110092,
0.533944954,0.535779817,0.537614679,0.539449541,0.541284404,0.543119266,
0.544954128,0.546788991,0.548623853,0.550458716,0.552293578,0.55412844,
0.555963303,0.557798165,0.559633028,0.56146789,0.563302752,0.565137615,
0.566972477,0.568807339,0.570642202,0.572477064,0.574311927,0.576146789,
0.577981651,0.579816514,0.581651376,0.583486239,0.585321101,0.587155963,
0.588990826,0.590825688,0.59266055,0.594495413,0.596330275,0.598165138,
0.6,0.601834862,0.603669725,0.605504587,0.60733945,0.609174312,0.611009174,
0.612844037,0.614678899,0.616513761,0.618348624,0.620183486,0.622018349,
0.623853211,0.625688073,0.627522936,0.629357798,0.631192661,0.633027523,
0.634862385,0.636697248,0.63853211,0.640366972,0.642201835,0.644036697,
0.64587156,0.647706422,0.649541284,0.651376147,0.653211009,0.655045872,
0.656880734,0.658715596,0.660550459,0.662385321,0.664220183,0.666055046,
0.667889908,0.669724771,0.671559633,0.673394495,0.675229358,0.67706422,
0.678899083,0.680733945,0.682568807,0.68440367,0.686238532,0.688073394,
0.689908257,0.691743119,0.693577982,0.695412844,0.697247706,0.699082569,
0.700917431,0.702752294,0.704587156,0.706422018,0.708256881,0.710091743,
0.711926606,0.713761468,0.71559633,0.717431193,0.719266055,0.721100917,
0.72293578,0.724770642,0.726605505,0.728440367,0.730275229,0.732110092,
0.733944954,0.735779817,0.737614679,0.739449541,0.741284404,0.743119266,
0.744954128,0.746788991,0.748623853,0.750458716,0.752293578,0.75412844,
0.755963303,0.757798165,0.759633028,0.76146789,0.763302752,0.765137615,
0.766972477,0.768807339,0.770642202,0.772477064,0.774311927,0.776146789,
0.777981651,0.779816514,0.781651376,0.783486239,0.785321101,0.787155963,
0.788990826,0.790825688,0.79266055,0.794495413,0.796330275,0.798165138,
0.8,0.801834862,0.803669725,0.805504587,0.80733945,0.809174312,0.811009174,
0.812844037,0.814678899,0.816513761,0.818348624,0.820183486,0.822018349,
0.823853211,0.825688073,0.827522936,0.829357798,0.831192661,0.833027523,
0.834862385,0.836697248,0.83853211,0.840366972,0.842201835,0.844036697,
0.84587156,0.847706422,0.849541284,0.851376147,0.853211009,0.855045872,
0.856880734,0.858715596,0.860550459,0.862385321,0.864220183,0.866055046,
0.867889908,0.869724771,0.871559633,0.873394495,0.875229358,0.87706422,
0.878899083,0.880733945,0.882568807,0.88440367,0.886238532,0.888073394,
0.889908257,0.891743119,0.893577982,0.895412844,0.897247706,0.899082569,
0.900917431,0.902752294,0.904587156,0.906422018,0.908256881,0.910091743,
0.911926606,0.913761468,0.91559633,0.917431193,0.919266055,0.921100917,
0.92293578,0.924770642,0.926605505,0.928440367,0.930275229,0.932110092,
0.933944954,0.935779817,0.937614679,0.939449541,0.941284404,0.943119266,
0.944954128,0.946788991,0.948623853,0.950458716,0.952293578,0.95412844,
0.955963303,0.957798165,0.959633028,0.96146789,0.963302752,0.965137615,
0.966972477,0.968807339,0.970642202,0.972477064,0.974311927,0.976146789,
0.977981651,0.979816514,0.981651376,0.983486239,0.985321101,0.987155963,
0.988990826,0.990825688,0.99266055,0.994495413,0.996330275,0.998165138,
1.),(0.3,1.,1.3),.UNSPECIFIED.);
#6319=B_SPLINE_SURFACE_WITH_KNOTS('',5,1,((#328049,#328050,#328051),(#328052,
#328053,#328054),(#328055,#328056,#328057),(#328058,#328059,#328060),(#328061,
#328062,#328063),(#328064,#328065,#328066),(#328067,#328068,#328069),(#328070,
#328071,#328072),(#328073,#328074,#328075),(#328076,#328077,#328078),(#328079,
#328080,#328081),(#328082,#328083,#328084),(#328085,#328086,#328087),(#328088,
#328089,#328090),(#328091,#328092,#328093),(#328094,#328095,#328096),(#328097,
#328098,#328099),(#328100,#328101,#328102),(#328103,#328104,#328105),(#328106,
#328107,#328108),(#328109,#328110,#328111),(#328112,#328113,#328114),(#328115,
#328116,#328117),(#328118,#328119,#328120),(#328121,#328122,#328123),(#328124,
#328125,#328126),(#328127,#328128,#328129),(#328130,#328131,#328132),(#328133,
#328134,#328135),(#328136,#328137,#328138),(#328139,#328140,#328141),(#328142,
#328143,#328144),(#328145,#328146,#328147),(#328148,#328149,#328150),(#328151,
#328152,#328153),(#328154,#328155,#328156),(#328157,#328158,#328159),(#328160,
#328161,#328162),(#328163,#328164,#328165),(#328166,#328167,#328168),(#328169,
#328170,#328171),(#328172,#328173,#328174),(#328175,#328176,#328177),(#328178,
#328179,#328180),(#328181,#328182,#328183),(#328184,#328185,#328186),(#328187,
#328188,#328189),(#328190,#328191,#328192),(#328193,#328194,#328195),(#328196,
#328197,#328198),(#328199,#328200,#328201),(#328202,#328203,#328204),(#328205,
#328206,#328207),(#328208,#328209,#328210),(#328211,#328212,#328213),(#328214,
#328215,#328216),(#328217,#328218,#328219),(#328220,#328221,#328222),(#328223,
#328224,#328225),(#328226,#328227,#328228),(#328229,#328230,#328231),(#328232,
#328233,#328234),(#328235,#328236,#328237),(#328238,#328239,#328240),(#328241,
#328242,#328243),(#328244,#328245,#328246),(#328247,#328248,#328249),(#328250,
#328251,#328252),(#328253,#328254,#328255),(#328256,#328257,#328258),(#328259,
#328260,#328261),(#328262,#328263,#328264),(#328265,#328266,#328267),(#328268,
#328269,#328270),(#328271,#328272,#328273),(#328274,#328275,#328276),(#328277,
#328278,#328279),(#328280,#328281,#328282),(#328283,#328284,#328285),(#328286,
#328287,#328288),(#328289,#328290,#328291),(#328292,#328293,#328294),(#328295,
#328296,#328297),(#328298,#328299,#328300),(#328301,#328302,#328303),(#328304,
#328305,#328306),(#328307,#328308,#328309),(#328310,#328311,#328312),(#328313,
#328314,#328315),(#328316,#328317,#328318),(#328319,#328320,#328321),(#328322,
#328323,#328324),(#328325,#328326,#328327),(#328328,#328329,#328330),(#328331,
#328332,#328333),(#328334,#328335,#328336),(#328337,#328338,#328339),(#328340,
#328341,#328342),(#328343,#328344,#328345),(#328346,#328347,#328348),(#328349,
#328350,#328351),(#328352,#328353,#328354),(#328355,#328356,#328357),(#328358,
#328359,#328360),(#328361,#328362,#328363),(#328364,#328365,#328366),(#328367,
#328368,#328369),(#328370,#328371,#328372),(#328373,#328374,#328375),(#328376,
#328377,#328378),(#328379,#328380,#328381),(#328382,#328383,#328384),(#328385,
#328386,#328387),(#328388,#328389,#328390),(#328391,#328392,#328393),(#328394,
#328395,#328396),(#328397,#328398,#328399),(#328400,#328401,#328402),(#328403,
#328404,#328405),(#328406,#328407,#328408),(#328409,#328410,#328411),(#328412,
#328413,#328414),(#328415,#328416,#328417),(#328418,#328419,#328420),(#328421,
#328422,#328423),(#328424,#328425,#328426),(#328427,#328428,#328429),(#328430,
#328431,#328432),(#328433,#328434,#328435),(#328436,#328437,#328438),(#328439,
#328440,#328441),(#328442,#328443,#328444),(#328445,#328446,#328447),(#328448,
#328449,#328450),(#328451,#328452,#328453),(#328454,#328455,#328456),(#328457,
#328458,#328459),(#328460,#328461,#328462),(#328463,#328464,#328465),(#328466,
#328467,#328468),(#328469,#328470,#328471),(#328472,#328473,#328474),(#328475,
#328476,#328477),(#328478,#328479,#328480),(#328481,#328482,#328483),(#328484,
#328485,#328486),(#328487,#328488,#328489),(#328490,#328491,#328492),(#328493,
#328494,#328495),(#328496,#328497,#328498),(#328499,#328500,#328501),(#328502,
#328503,#328504),(#328505,#328506,#328507),(#328508,#328509,#328510),(#328511,
#328512,#328513),(#328514,#328515,#328516),(#328517,#328518,#328519),(#328520,
#328521,#328522),(#328523,#328524,#328525),(#328526,#328527,#328528),(#328529,
#328530,#328531),(#328532,#328533,#328534),(#328535,#328536,#328537),(#328538,
#328539,#328540),(#328541,#328542,#328543),(#328544,#328545,#328546),(#328547,
#328548,#328549),(#328550,#328551,#328552),(#328553,#328554,#328555),(#328556,
#328557,#328558),(#328559,#328560,#328561),(#328562,#328563,#328564),(#328565,
#328566,#328567),(#328568,#328569,#328570),(#328571,#328572,#328573),(#328574,
#328575,#328576),(#328577,#328578,#328579),(#328580,#328581,#328582),(#328583,
#328584,#328585),(#328586,#328587,#328588),(#328589,#328590,#328591),(#328592,
#328593,#328594),(#328595,#328596,#328597),(#328598,#328599,#328600),(#328601,
#328602,#328603),(#328604,#328605,#328606),(#328607,#328608,#328609),(#328610,
#328611,#328612),(#328613,#328614,#328615),(#328616,#328617,#328618),(#328619,
#328620,#328621),(#328622,#328623,#328624),(#328625,#328626,#328627),(#328628,
#328629,#328630),(#328631,#328632,#328633),(#328634,#328635,#328636),(#328637,
#328638,#328639),(#328640,#328641,#328642),(#328643,#328644,#328645),(#328646,
#328647,#328648),(#328649,#328650,#328651),(#328652,#328653,#328654),(#328655,
#328656,#328657),(#328658,#328659,#328660),(#328661,#328662,#328663),(#328664,
#328665,#328666),(#328667,#328668,#328669),(#328670,#328671,#328672),(#328673,
#328674,#328675),(#328676,#328677,#328678),(#328679,#328680,#328681),(#328682,
#328683,#328684),(#328685,#328686,#328687),(#328688,#328689,#328690),(#328691,
#328692,#328693),(#328694,#328695,#328696),(#328697,#328698,#328699),(#328700,
#328701,#328702),(#328703,#328704,#328705),(#328706,#328707,#328708),(#328709,
#328710,#328711),(#328712,#328713,#328714),(#328715,#328716,#328717),(#328718,
#328719,#328720),(#328721,#328722,#328723),(#328724,#328725,#328726),(#328727,
#328728,#328729),(#328730,#328731,#328732),(#328733,#328734,#328735),(#328736,
#328737,#328738),(#328739,#328740,#328741),(#328742,#328743,#328744),(#328745,
#328746,#328747),(#328748,#328749,#328750),(#328751,#328752,#328753),(#328754,
#328755,#328756),(#328757,#328758,#328759),(#328760,#328761,#328762),(#328763,
#328764,#328765),(#328766,#328767,#328768),(#328769,#328770,#328771),(#328772,
#328773,#328774),(#328775,#328776,#328777),(#328778,#328779,#328780),(#328781,
#328782,#328783),(#328784,#328785,#328786),(#328787,#328788,#328789),(#328790,
#328791,#328792),(#328793,#328794,#328795),(#328796,#328797,#328798),(#328799,
#328800,#328801),(#328802,#328803,#328804),(#328805,#328806,#328807),(#328808,
#328809,#328810),(#328811,#328812,#328813),(#328814,#328815,#328816),(#328817,
#328818,#328819),(#328820,#328821,#328822),(#328823,#328824,#328825),(#328826,
#328827,#328828),(#328829,#328830,#328831),(#328832,#328833,#328834),(#328835,
#328836,#328837),(#328838,#328839,#328840),(#328841,#328842,#328843),(#328844,
#328845,#328846),(#328847,#328848,#328849),(#328850,#328851,#328852),(#328853,
#328854,#328855),(#328856,#328857,#328858),(#328859,#328860,#328861),(#328862,
#328863,#328864),(#328865,#328866,#328867),(#328868,#328869,#328870),(#328871,
#328872,#328873),(#328874,#328875,#328876),(#328877,#328878,#328879),(#328880,
#328881,#328882),(#328883,#328884,#328885),(#328886,#328887,#328888),(#328889,
#328890,#328891),(#328892,#328893,#328894),(#328895,#328896,#328897),(#328898,
#328899,#328900),(#328901,#328902,#328903),(#328904,#328905,#328906),(#328907,
#328908,#328909),(#328910,#328911,#328912),(#328913,#328914,#328915),(#328916,
#328917,#328918),(#328919,#328920,#328921),(#328922,#328923,#328924),(#328925,
#328926,#328927),(#328928,#328929,#328930),(#328931,#328932,#328933),(#328934,
#328935,#328936),(#328937,#328938,#328939),(#328940,#328941,#328942),(#328943,
#328944,#328945),(#328946,#328947,#328948),(#328949,#328950,#328951),(#328952,
#328953,#328954),(#328955,#328956,#328957),(#328958,#328959,#328960),(#328961,
#328962,#328963),(#328964,#328965,#328966),(#328967,#328968,#328969),(#328970,
#328971,#328972),(#328973,#328974,#328975),(#328976,#328977,#328978),(#328979,
#328980,#328981),(#328982,#328983,#328984),(#328985,#328986,#328987),(#328988,
#328989,#328990),(#328991,#328992,#328993),(#328994,#328995,#328996),(#328997,
#328998,#328999),(#329000,#329001,#329002),(#329003,#329004,#329005),(#329006,
#329007,#329008),(#329009,#329010,#329011),(#329012,#329013,#329014),(#329015,
#329016,#329017),(#329018,#329019,#329020),(#329021,#329022,#329023),(#329024,
#329025,#329026),(#329027,#329028,#329029),(#329030,#329031,#329032),(#329033,
#329034,#329035),(#329036,#329037,#329038),(#329039,#329040,#329041),(#329042,
#329043,#329044),(#329045,#329046,#329047),(#329048,#329049,#329050),(#329051,
#329052,#329053),(#329054,#329055,#329056),(#329057,#329058,#329059),(#329060,
#329061,#329062),(#329063,#329064,#329065),(#329066,#329067,#329068),(#329069,
#329070,#329071),(#329072,#329073,#329074),(#329075,#329076,#329077),(#329078,
#329079,#329080),(#329081,#329082,#329083),(#329084,#329085,#329086),(#329087,
#329088,#329089),(#329090,#329091,#329092),(#329093,#329094,#329095),(#329096,
#329097,#329098),(#329099,#329100,#329101),(#329102,#329103,#329104),(#329105,
#329106,#329107),(#329108,#329109,#329110),(#329111,#329112,#329113),(#329114,
#329115,#329116),(#329117,#329118,#329119),(#329120,#329121,#329122),(#329123,
#329124,#329125),(#329126,#329127,#329128),(#329129,#329130,#329131),(#329132,
#329133,#329134),(#329135,#329136,#329137),(#329138,#329139,#329140),(#329141,
#329142,#329143),(#329144,#329145,#329146),(#329147,#329148,#329149),(#329150,
#329151,#329152),(#329153,#329154,#329155),(#329156,#329157,#329158),(#329159,
#329160,#329161),(#329162,#329163,#329164),(#329165,#329166,#329167),(#329168,
#329169,#329170),(#329171,#329172,#329173),(#329174,#329175,#329176),(#329177,
#329178,#329179),(#329180,#329181,#329182),(#329183,#329184,#329185),(#329186,
#329187,#329188),(#329189,#329190,#329191),(#329192,#329193,#329194),(#329195,
#329196,#329197),(#329198,#329199,#329200),(#329201,#329202,#329203),(#329204,
#329205,#329206),(#329207,#329208,#329209),(#329210,#329211,#329212),(#329213,
#329214,#329215),(#329216,#329217,#329218),(#329219,#329220,#329221),(#329222,
#329223,#329224),(#329225,#329226,#329227),(#329228,#329229,#329230),(#329231,
#329232,#329233),(#329234,#329235,#329236),(#329237,#329238,#329239),(#329240,
#329241,#329242),(#329243,#329244,#329245),(#329246,#329247,#329248),(#329249,
#329250,#329251),(#329252,#329253,#329254),(#329255,#329256,#329257),(#329258,
#329259,#329260),(#329261,#329262,#329263),(#329264,#329265,#329266),(#329267,
#329268,#329269),(#329270,#329271,#329272),(#329273,#329274,#329275),(#329276,
#329277,#329278),(#329279,#329280,#329281),(#329282,#329283,#329284),(#329285,
#329286,#329287),(#329288,#329289,#329290),(#329291,#329292,#329293),(#329294,
#329295,#329296),(#329297,#329298,#329299),(#329300,#329301,#329302),(#329303,
#329304,#329305),(#329306,#329307,#329308),(#329309,#329310,#329311),(#329312,
#329313,#329314),(#329315,#329316,#329317),(#329318,#329319,#329320),(#329321,
#329322,#329323),(#329324,#329325,#329326),(#329327,#329328,#329329),(#329330,
#329331,#329332),(#329333,#329334,#329335),(#329336,#329337,#329338),(#329339,
#329340,#329341),(#329342,#329343,#329344),(#329345,#329346,#329347),(#329348,
#329349,#329350),(#329351,#329352,#329353),(#329354,#329355,#329356),(#329357,
#329358,#329359),(#329360,#329361,#329362),(#329363,#329364,#329365),(#329366,
#329367,#329368),(#329369,#329370,#329371),(#329372,#329373,#329374),(#329375,
#329376,#329377),(#329378,#329379,#329380),(#329381,#329382,#329383),(#329384,
#329385,#329386),(#329387,#329388,#329389),(#329390,#329391,#329392),(#329393,
#329394,#329395),(#329396,#329397,#329398),(#329399,#329400,#329401),(#329402,
#329403,#329404),(#329405,#329406,#329407),(#329408,#329409,#329410),(#329411,
#329412,#329413),(#329414,#329415,#329416),(#329417,#329418,#329419),(#329420,
#329421,#329422),(#329423,#329424,#329425),(#329426,#329427,#329428),(#329429,
#329430,#329431),(#329432,#329433,#329434),(#329435,#329436,#329437),(#329438,
#329439,#329440),(#329441,#329442,#329443),(#329444,#329445,#329446),(#329447,
#329448,#329449),(#329450,#329451,#329452),(#329453,#329454,#329455),(#329456,
#329457,#329458),(#329459,#329460,#329461),(#329462,#329463,#329464),(#329465,
#329466,#329467),(#329468,#329469,#329470),(#329471,#329472,#329473),(#329474,
#329475,#329476),(#329477,#329478,#329479),(#329480,#329481,#329482),(#329483,
#329484,#329485),(#329486,#329487,#329488),(#329489,#329490,#329491),(#329492,
#329493,#329494),(#329495,#329496,#329497),(#329498,#329499,#329500),(#329501,
#329502,#329503),(#329504,#329505,#329506),(#329507,#329508,#329509),(#329510,
#329511,#329512),(#329513,#329514,#329515),(#329516,#329517,#329518),(#329519,
#329520,#329521),(#329522,#329523,#329524),(#329525,#329526,#329527),(#329528,
#329529,#329530),(#329531,#329532,#329533),(#329534,#329535,#329536),(#329537,
#329538,#329539),(#329540,#329541,#329542),(#329543,#329544,#329545),(#329546,
#329547,#329548),(#329549,#329550,#329551),(#329552,#329553,#329554),(#329555,
#329556,#329557),(#329558,#329559,#329560),(#329561,#329562,#329563),(#329564,
#329565,#329566),(#329567,#329568,#329569),(#329570,#329571,#329572),(#329573,
#329574,#329575),(#329576,#329577,#329578),(#329579,#329580,#329581),(#329582,
#329583,#329584),(#329585,#329586,#329587),(#329588,#329589,#329590),(#329591,
#329592,#329593),(#329594,#329595,#329596),(#329597,#329598,#329599),(#329600,
#329601,#329602),(#329603,#329604,#329605),(#329606,#329607,#329608),(#329609,
#329610,#329611),(#329612,#329613,#329614),(#329615,#329616,#329617),(#329618,
#329619,#329620),(#329621,#329622,#329623),(#329624,#329625,#329626),(#329627,
#329628,#329629),(#329630,#329631,#329632),(#329633,#329634,#329635),(#329636,
#329637,#329638),(#329639,#329640,#329641),(#329642,#329643,#329644),(#329645,
#329646,#329647),(#329648,#329649,#329650),(#329651,#329652,#329653),(#329654,
#329655,#329656),(#329657,#329658,#329659),(#329660,#329661,#329662),(#329663,
#329664,#329665),(#329666,#329667,#329668),(#329669,#329670,#329671),(#329672,
#329673,#329674),(#329675,#329676,#329677),(#329678,#329679,#329680),(#329681,
#329682,#329683),(#329684,#329685,#329686),(#329687,#329688,#329689),(#329690,
#329691,#329692),(#329693,#329694,#329695),(#329696,#329697,#329698)),
 .UNSPECIFIED.,.F.,.F.,.F.,(6,1,1,1,1,1,1,1,1,1,1,1,1,1,1,1,1,1,1,1,1,1,
1,1,1,1,1,1,1,1,1,1,1,1,1,1,1,1,1,1,1,1,1,1,1,1,1,1,1,1,1,1,1,1,1,1,1,1,
1,1,1,1,1,1,1,1,1,1,1,1,1,1,1,1,1,1,1,1,1,1,1,1,1,1,1,1,1,1,1,1,1,1,1,1,
1,1,1,1,1,1,1,1,1,1,1,1,1,1,1,1,1,1,1,1,1,1,1,1,1,1,1,1,1,1,1,1,1,1,1,1,
1,1,1,1,1,1,1,1,1,1,1,1,1,1,1,1,1,1,1,1,1,1,1,1,1,1,1,1,1,1,1,1,1,1,1,1,
1,1,1,1,1,1,1,1,1,1,1,1,1,1,1,1,1,1,1,1,1,1,1,1,1,1,1,1,1,1,1,1,1,1,1,1,
1,1,1,1,1,1,1,1,1,1,1,1,1,1,1,1,1,1,1,1,1,1,1,1,1,1,1,1,1,1,1,1,1,1,1,1,
1,1,1,1,1,1,1,1,1,1,1,1,1,1,1,1,1,1,1,1,1,1,1,1,1,1,1,1,1,1,1,1,1,1,1,1,
1,1,1,1,1,1,1,1,1,1,1,1,1,1,1,1,1,1,1,1,1,1,1,1,1,1,1,1,1,1,1,1,1,1,1,1,
1,1,1,1,1,1,1,1,1,1,1,1,1,1,1,1,1,1,1,1,1,1,1,1,1,1,1,1,1,1,1,1,1,1,1,1,
1,1,1,1,1,1,1,1,1,1,1,1,1,1,1,1,1,1,1,1,1,1,1,1,1,1,1,1,1,1,1,1,1,1,1,1,
1,1,1,1,1,1,1,1,1,1,1,1,1,1,1,1,1,1,1,1,1,1,1,1,1,1,1,1,1,1,1,1,1,1,1,1,
1,1,1,1,1,1,1,1,1,1,1,1,1,1,1,1,1,1,1,1,1,1,1,1,1,1,1,1,1,1,1,1,1,1,1,1,
1,1,1,1,1,1,1,1,1,1,1,1,1,1,1,1,1,1,1,1,1,1,1,1,1,1,1,1,1,1,1,1,1,1,1,1,
1,1,1,1,1,1,1,1,1,1,1,1,1,1,1,1,1,1,1,1,1,1,1,1,1,1,1,1,1,1,1,1,1,1,1,1,
1,1,1,1,1,1,1,1,1,1,1,1,1,1,1,1,1,1,1,6),(2,1,2),(-1.,-0.998165138,-0.996330275,
-0.994495413,-0.99266055,-0.990825688,-0.988990826,-0.987155963,-0.985321101,
-0.983486239,-0.981651376,-0.979816514,-0.977981651,-0.976146789,-0.974311927,
-0.972477064,-0.970642202,-0.968807339,-0.966972477,-0.965137615,-0.963302752,
-0.96146789,-0.959633028,-0.957798165,-0.955963303,-0.95412844,-0.952293578,
-0.950458716,-0.948623853,-0.946788991,-0.944954128,-0.943119266,-0.941284404,
-0.939449541,-0.937614679,-0.935779817,-0.933944954,-0.932110092,-0.930275229,
-0.928440367,-0.926605505,-0.924770642,-0.92293578,-0.921100917,-0.919266055,
-0.917431193,-0.91559633,-0.913761468,-0.911926606,-0.910091743,-0.908256881,
-0.906422018,-0.904587156,-0.902752294,-0.900917431,-0.899082569,-0.897247706,
-0.895412844,-0.893577982,-0.891743119,-0.889908257,-0.888073394,-0.886238532,
-0.88440367,-0.882568807,-0.880733945,-0.878899083,-0.87706422,-0.875229358,
-0.873394495,-0.871559633,-0.869724771,-0.867889908,-0.866055046,-0.864220183,
-0.862385321,-0.860550459,-0.858715596,-0.856880734,-0.855045872,-0.853211009,
-0.851376147,-0.849541284,-0.847706422,-0.84587156,-0.844036697,-0.842201835,
-0.840366972,-0.83853211,-0.836697248,-0.834862385,-0.833027523,-0.831192661,
-0.829357798,-0.827522936,-0.825688073,-0.823853211,-0.822018349,-0.820183486,
-0.818348624,-0.816513761,-0.814678899,-0.812844037,-0.811009174,-0.809174312,
-0.80733945,-0.805504587,-0.803669725,-0.801834862,-0.8,-0.798165138,-0.796330275,
-0.794495413,-0.79266055,-0.790825688,-0.788990826,-0.787155963,-0.785321101,
-0.783486239,-0.781651376,-0.779816514,-0.777981651,-0.776146789,-0.774311927,
-0.772477064,-0.770642202,-0.768807339,-0.766972477,-0.765137615,-0.763302752,
-0.76146789,-0.759633028,-0.757798165,-0.755963303,-0.75412844,-0.752293578,
-0.750458716,-0.748623853,-0.746788991,-0.744954128,-0.743119266,-0.741284404,
-0.739449541,-0.737614679,-0.735779817,-0.733944954,-0.732110092,-0.730275229,
-0.728440367,-0.726605505,-0.724770642,-0.72293578,-0.721100917,-0.719266055,
-0.717431193,-0.71559633,-0.713761468,-0.711926606,-0.710091743,-0.708256881,
-0.706422018,-0.704587156,-0.702752294,-0.700917431,-0.699082569,-0.697247706,
-0.695412844,-0.693577982,-0.691743119,-0.689908257,-0.688073394,-0.686238532,
-0.68440367,-0.682568807,-0.680733945,-0.678899083,-0.67706422,-0.675229358,
-0.673394495,-0.671559633,-0.669724771,-0.667889908,-0.666055046,-0.664220183,
-0.662385321,-0.660550459,-0.658715596,-0.656880734,-0.655045872,-0.653211009,
-0.651376147,-0.649541284,-0.647706422,-0.64587156,-0.644036697,-0.642201835,
-0.640366972,-0.63853211,-0.636697248,-0.634862385,-0.633027523,-0.631192661,
-0.629357798,-0.627522936,-0.625688073,-0.623853211,-0.622018349,-0.620183486,
-0.618348624,-0.616513761,-0.614678899,-0.612844037,-0.611009174,-0.609174312,
-0.60733945,-0.605504587,-0.603669725,-0.601834862,-0.6,-0.598165138,-0.596330275,
-0.594495413,-0.59266055,-0.590825688,-0.588990826,-0.587155963,-0.585321101,
-0.583486239,-0.581651376,-0.579816514,-0.577981651,-0.576146789,-0.574311927,
-0.572477064,-0.570642202,-0.568807339,-0.566972477,-0.565137615,-0.563302752,
-0.56146789,-0.559633028,-0.557798165,-0.555963303,-0.55412844,-0.552293578,
-0.550458716,-0.548623853,-0.546788991,-0.544954128,-0.543119266,-0.541284404,
-0.539449541,-0.537614679,-0.535779817,-0.533944954,-0.532110092,-0.530275229,
-0.528440367,-0.526605505,-0.524770642,-0.52293578,-0.521100917,-0.519266055,
-0.517431193,-0.51559633,-0.513761468,-0.511926606,-0.510091743,-0.508256881,
-0.506422018,-0.504587156,-0.502752294,-0.500917431,-0.499082569,-0.497247706,
-0.495412844,-0.493577982,-0.491743119,-0.489908257,-0.488073394,-0.486238532,
-0.48440367,-0.482568807,-0.480733945,-0.478899083,-0.47706422,-0.475229358,
-0.473394495,-0.471559633,-0.469724771,-0.467889908,-0.466055046,-0.464220183,
-0.462385321,-0.460550459,-0.458715596,-0.456880734,-0.455045872,-0.453211009,
-0.451376147,-0.449541284,-0.447706422,-0.44587156,-0.444036697,-0.442201835,
-0.440366972,-0.43853211,-0.436697248,-0.434862385,-0.433027523,-0.431192661,
-0.429357798,-0.427522936,-0.425688073,-0.423853211,-0.422018349,-0.420183486,
-0.418348624,-0.416513761,-0.414678899,-0.412844037,-0.411009174,-0.409174312,
-0.40733945,-0.405504587,-0.403669725,-0.401834862,-0.4,-0.398165138,-0.396330275,
-0.394495413,-0.39266055,-0.390825688,-0.388990826,-0.387155963,-0.385321101,
-0.383486239,-0.381651376,-0.379816514,-0.377981651,-0.376146789,-0.374311927,
-0.372477064,-0.370642202,-0.368807339,-0.366972477,-0.365137615,-0.363302752,
-0.36146789,-0.359633028,-0.357798165,-0.355963303,-0.35412844,-0.352293578,
-0.350458716,-0.348623853,-0.346788991,-0.344954128,-0.343119266,-0.341284404,
-0.339449541,-0.337614679,-0.335779817,-0.333944954,-0.332110092,-0.330275229,
-0.328440367,-0.326605505,-0.324770642,-0.32293578,-0.321100917,-0.319266055,
-0.317431193,-0.31559633,-0.313761468,-0.311926606,-0.310091743,-0.308256881,
-0.306422018,-0.304587156,-0.302752294,-0.300917431,-0.299082569,-0.297247706,
-0.295412844,-0.293577982,-0.291743119,-0.289908257,-0.288073394,-0.286238532,
-0.28440367,-0.282568807,-0.280733945,-0.278899083,-0.27706422,-0.275229358,
-0.273394495,-0.271559633,-0.269724771,-0.267889908,-0.266055046,-0.264220183,
-0.262385321,-0.260550459,-0.258715596,-0.256880734,-0.255045872,-0.253211009,
-0.251376147,-0.249541284,-0.247706422,-0.24587156,-0.244036697,-0.242201835,
-0.240366972,-0.23853211,-0.236697248,-0.234862385,-0.233027523,-0.231192661,
-0.229357798,-0.227522936,-0.225688073,-0.223853211,-0.222018349,-0.220183486,
-0.218348624,-0.216513761,-0.214678899,-0.212844037,-0.211009174,-0.209174312,
-0.20733945,-0.205504587,-0.203669725,-0.201834862,-0.2,-0.198165138,-0.196330275,
-0.194495413,-0.19266055,-0.190825688,-0.188990826,-0.187155963,-0.185321101,
-0.183486239,-0.181651376,-0.179816514,-0.177981651,-0.176146789,-0.174311927,
-0.172477064,-0.170642202,-0.168807339,-0.166972477,-0.165137615,-0.163302752,
-0.16146789,-0.159633028,-0.157798165,-0.155963303,-0.15412844,-0.152293578,
-0.150458716,-0.148623853,-0.146788991,-0.144954128,-0.143119266,-0.141284404,
-0.139449541,-0.137614679,-0.135779817,-0.133944954,-0.132110092,-0.130275229,
-0.128440367,-0.126605505,-0.124770642,-0.12293578,-0.121100917,-0.119266055,
-0.117431193,-0.11559633,-0.113761468,-0.111926606,-0.110091743,-0.108256881,
-0.106422018,-0.104587156,-0.102752294,-0.100917431,-0.099082569,-0.097247706,
-0.095412844,-0.093577982,-0.091743119,-0.089908257,-0.088073394,-0.086238532,
-0.08440367,-0.082568807,-0.080733945,-0.078899083,-0.07706422,-0.075229358,
-0.073394495,-0.071559633,-0.069724771,-0.067889908,-0.066055046,-0.064220183,
-0.062385321,-0.060550459,-0.058715596,-0.056880734,-0.055045872,-0.053211009,
-0.051376147,-0.049541284,-0.047706422,-0.04587156,-0.044036697,-0.042201835,
-0.040366972,-0.03853211,-0.036697248,-0.034862385,-0.033027523,-0.031192661,
-0.029357798,-0.027522936,-0.025688073,-0.023853211,-0.022018349,-0.020183486,
-0.018348624,-0.016513761,-0.014678899,-0.012844037,-0.011009174,-0.009174312,
-0.00733945,-0.005504587,-0.003669725,-0.001834862,0.000982137),(0.3,1.,
1.3),.UNSPECIFIED.);
#6320=B_SPLINE_SURFACE_WITH_KNOTS('',5,1,((#329997,#329998,#329999),(#330000,
#330001,#330002),(#330003,#330004,#330005),(#330006,#330007,#330008),(#330009,
#330010,#330011),(#330012,#330013,#330014),(#330015,#330016,#330017),(#330018,
#330019,#330020),(#330021,#330022,#330023),(#330024,#330025,#330026),(#330027,
#330028,#330029),(#330030,#330031,#330032),(#330033,#330034,#330035),(#330036,
#330037,#330038),(#330039,#330040,#330041),(#330042,#330043,#330044),(#330045,
#330046,#330047),(#330048,#330049,#330050),(#330051,#330052,#330053),(#330054,
#330055,#330056),(#330057,#330058,#330059),(#330060,#330061,#330062),(#330063,
#330064,#330065),(#330066,#330067,#330068),(#330069,#330070,#330071),(#330072,
#330073,#330074),(#330075,#330076,#330077),(#330078,#330079,#330080),(#330081,
#330082,#330083),(#330084,#330085,#330086),(#330087,#330088,#330089),(#330090,
#330091,#330092),(#330093,#330094,#330095),(#330096,#330097,#330098),(#330099,
#330100,#330101),(#330102,#330103,#330104),(#330105,#330106,#330107),(#330108,
#330109,#330110),(#330111,#330112,#330113),(#330114,#330115,#330116),(#330117,
#330118,#330119),(#330120,#330121,#330122),(#330123,#330124,#330125),(#330126,
#330127,#330128),(#330129,#330130,#330131),(#330132,#330133,#330134),(#330135,
#330136,#330137),(#330138,#330139,#330140),(#330141,#330142,#330143),(#330144,
#330145,#330146),(#330147,#330148,#330149),(#330150,#330151,#330152),(#330153,
#330154,#330155),(#330156,#330157,#330158),(#330159,#330160,#330161),(#330162,
#330163,#330164),(#330165,#330166,#330167),(#330168,#330169,#330170),(#330171,
#330172,#330173),(#330174,#330175,#330176),(#330177,#330178,#330179),(#330180,
#330181,#330182),(#330183,#330184,#330185),(#330186,#330187,#330188),(#330189,
#330190,#330191),(#330192,#330193,#330194),(#330195,#330196,#330197),(#330198,
#330199,#330200),(#330201,#330202,#330203),(#330204,#330205,#330206),(#330207,
#330208,#330209),(#330210,#330211,#330212),(#330213,#330214,#330215),(#330216,
#330217,#330218),(#330219,#330220,#330221),(#330222,#330223,#330224),(#330225,
#330226,#330227),(#330228,#330229,#330230),(#330231,#330232,#330233),(#330234,
#330235,#330236),(#330237,#330238,#330239),(#330240,#330241,#330242),(#330243,
#330244,#330245),(#330246,#330247,#330248),(#330249,#330250,#330251),(#330252,
#330253,#330254),(#330255,#330256,#330257),(#330258,#330259,#330260),(#330261,
#330262,#330263),(#330264,#330265,#330266),(#330267,#330268,#330269),(#330270,
#330271,#330272),(#330273,#330274,#330275),(#330276,#330277,#330278),(#330279,
#330280,#330281),(#330282,#330283,#330284),(#330285,#330286,#330287),(#330288,
#330289,#330290),(#330291,#330292,#330293),(#330294,#330295,#330296),(#330297,
#330298,#330299),(#330300,#330301,#330302),(#330303,#330304,#330305),(#330306,
#330307,#330308),(#330309,#330310,#330311),(#330312,#330313,#330314),(#330315,
#330316,#330317),(#330318,#330319,#330320),(#330321,#330322,#330323),(#330324,
#330325,#330326),(#330327,#330328,#330329),(#330330,#330331,#330332),(#330333,
#330334,#330335),(#330336,#330337,#330338),(#330339,#330340,#330341),(#330342,
#330343,#330344),(#330345,#330346,#330347),(#330348,#330349,#330350),(#330351,
#330352,#330353),(#330354,#330355,#330356),(#330357,#330358,#330359),(#330360,
#330361,#330362),(#330363,#330364,#330365),(#330366,#330367,#330368),(#330369,
#330370,#330371),(#330372,#330373,#330374),(#330375,#330376,#330377),(#330378,
#330379,#330380),(#330381,#330382,#330383),(#330384,#330385,#330386),(#330387,
#330388,#330389),(#330390,#330391,#330392),(#330393,#330394,#330395),(#330396,
#330397,#330398),(#330399,#330400,#330401),(#330402,#330403,#330404),(#330405,
#330406,#330407),(#330408,#330409,#330410),(#330411,#330412,#330413),(#330414,
#330415,#330416),(#330417,#330418,#330419),(#330420,#330421,#330422),(#330423,
#330424,#330425),(#330426,#330427,#330428),(#330429,#330430,#330431),(#330432,
#330433,#330434),(#330435,#330436,#330437),(#330438,#330439,#330440),(#330441,
#330442,#330443),(#330444,#330445,#330446),(#330447,#330448,#330449),(#330450,
#330451,#330452),(#330453,#330454,#330455),(#330456,#330457,#330458),(#330459,
#330460,#330461),(#330462,#330463,#330464),(#330465,#330466,#330467),(#330468,
#330469,#330470),(#330471,#330472,#330473),(#330474,#330475,#330476),(#330477,
#330478,#330479),(#330480,#330481,#330482),(#330483,#330484,#330485),(#330486,
#330487,#330488),(#330489,#330490,#330491),(#330492,#330493,#330494),(#330495,
#330496,#330497),(#330498,#330499,#330500),(#330501,#330502,#330503),(#330504,
#330505,#330506),(#330507,#330508,#330509),(#330510,#330511,#330512),(#330513,
#330514,#330515),(#330516,#330517,#330518),(#330519,#330520,#330521),(#330522,
#330523,#330524),(#330525,#330526,#330527),(#330528,#330529,#330530),(#330531,
#330532,#330533),(#330534,#330535,#330536),(#330537,#330538,#330539),(#330540,
#330541,#330542),(#330543,#330544,#330545),(#330546,#330547,#330548),(#330549,
#330550,#330551),(#330552,#330553,#330554),(#330555,#330556,#330557),(#330558,
#330559,#330560),(#330561,#330562,#330563),(#330564,#330565,#330566),(#330567,
#330568,#330569),(#330570,#330571,#330572),(#330573,#330574,#330575),(#330576,
#330577,#330578),(#330579,#330580,#330581),(#330582,#330583,#330584),(#330585,
#330586,#330587),(#330588,#330589,#330590),(#330591,#330592,#330593),(#330594,
#330595,#330596),(#330597,#330598,#330599),(#330600,#330601,#330602),(#330603,
#330604,#330605),(#330606,#330607,#330608),(#330609,#330610,#330611),(#330612,
#330613,#330614),(#330615,#330616,#330617),(#330618,#330619,#330620),(#330621,
#330622,#330623),(#330624,#330625,#330626),(#330627,#330628,#330629),(#330630,
#330631,#330632),(#330633,#330634,#330635),(#330636,#330637,#330638),(#330639,
#330640,#330641),(#330642,#330643,#330644),(#330645,#330646,#330647),(#330648,
#330649,#330650),(#330651,#330652,#330653),(#330654,#330655,#330656),(#330657,
#330658,#330659),(#330660,#330661,#330662),(#330663,#330664,#330665),(#330666,
#330667,#330668),(#330669,#330670,#330671),(#330672,#330673,#330674),(#330675,
#330676,#330677),(#330678,#330679,#330680),(#330681,#330682,#330683),(#330684,
#330685,#330686),(#330687,#330688,#330689),(#330690,#330691,#330692),(#330693,
#330694,#330695),(#330696,#330697,#330698),(#330699,#330700,#330701),(#330702,
#330703,#330704),(#330705,#330706,#330707),(#330708,#330709,#330710),(#330711,
#330712,#330713),(#330714,#330715,#330716),(#330717,#330718,#330719),(#330720,
#330721,#330722),(#330723,#330724,#330725),(#330726,#330727,#330728),(#330729,
#330730,#330731),(#330732,#330733,#330734),(#330735,#330736,#330737),(#330738,
#330739,#330740),(#330741,#330742,#330743),(#330744,#330745,#330746),(#330747,
#330748,#330749),(#330750,#330751,#330752),(#330753,#330754,#330755),(#330756,
#330757,#330758),(#330759,#330760,#330761),(#330762,#330763,#330764),(#330765,
#330766,#330767),(#330768,#330769,#330770),(#330771,#330772,#330773),(#330774,
#330775,#330776),(#330777,#330778,#330779),(#330780,#330781,#330782),(#330783,
#330784,#330785),(#330786,#330787,#330788),(#330789,#330790,#330791),(#330792,
#330793,#330794),(#330795,#330796,#330797),(#330798,#330799,#330800),(#330801,
#330802,#330803),(#330804,#330805,#330806),(#330807,#330808,#330809),(#330810,
#330811,#330812),(#330813,#330814,#330815),(#330816,#330817,#330818),(#330819,
#330820,#330821),(#330822,#330823,#330824),(#330825,#330826,#330827),(#330828,
#330829,#330830),(#330831,#330832,#330833),(#330834,#330835,#330836),(#330837,
#330838,#330839),(#330840,#330841,#330842),(#330843,#330844,#330845),(#330846,
#330847,#330848),(#330849,#330850,#330851),(#330852,#330853,#330854),(#330855,
#330856,#330857),(#330858,#330859,#330860),(#330861,#330862,#330863),(#330864,
#330865,#330866),(#330867,#330868,#330869),(#330870,#330871,#330872),(#330873,
#330874,#330875),(#330876,#330877,#330878),(#330879,#330880,#330881),(#330882,
#330883,#330884),(#330885,#330886,#330887),(#330888,#330889,#330890),(#330891,
#330892,#330893),(#330894,#330895,#330896),(#330897,#330898,#330899),(#330900,
#330901,#330902),(#330903,#330904,#330905),(#330906,#330907,#330908),(#330909,
#330910,#330911),(#330912,#330913,#330914),(#330915,#330916,#330917),(#330918,
#330919,#330920),(#330921,#330922,#330923),(#330924,#330925,#330926),(#330927,
#330928,#330929),(#330930,#330931,#330932),(#330933,#330934,#330935),(#330936,
#330937,#330938),(#330939,#330940,#330941),(#330942,#330943,#330944),(#330945,
#330946,#330947),(#330948,#330949,#330950),(#330951,#330952,#330953),(#330954,
#330955,#330956),(#330957,#330958,#330959),(#330960,#330961,#330962),(#330963,
#330964,#330965),(#330966,#330967,#330968),(#330969,#330970,#330971),(#330972,
#330973,#330974),(#330975,#330976,#330977),(#330978,#330979,#330980),(#330981,
#330982,#330983),(#330984,#330985,#330986),(#330987,#330988,#330989),(#330990,
#330991,#330992),(#330993,#330994,#330995),(#330996,#330997,#330998),(#330999,
#331000,#331001),(#331002,#331003,#331004),(#331005,#331006,#331007),(#331008,
#331009,#331010),(#331011,#331012,#331013),(#331014,#331015,#331016),(#331017,
#331018,#331019),(#331020,#331021,#331022),(#331023,#331024,#331025),(#331026,
#331027,#331028),(#331029,#331030,#331031),(#331032,#331033,#331034),(#331035,
#331036,#331037),(#331038,#331039,#331040),(#331041,#331042,#331043),(#331044,
#331045,#331046),(#331047,#331048,#331049),(#331050,#331051,#331052),(#331053,
#331054,#331055),(#331056,#331057,#331058),(#331059,#331060,#331061),(#331062,
#331063,#331064),(#331065,#331066,#331067),(#331068,#331069,#331070),(#331071,
#331072,#331073),(#331074,#331075,#331076),(#331077,#331078,#331079),(#331080,
#331081,#331082),(#331083,#331084,#331085),(#331086,#331087,#331088),(#331089,
#331090,#331091),(#331092,#331093,#331094),(#331095,#331096,#331097),(#331098,
#331099,#331100),(#331101,#331102,#331103),(#331104,#331105,#331106),(#331107,
#331108,#331109),(#331110,#331111,#331112),(#331113,#331114,#331115),(#331116,
#331117,#331118),(#331119,#331120,#331121),(#331122,#331123,#331124),(#331125,
#331126,#331127),(#331128,#331129,#331130),(#331131,#331132,#331133),(#331134,
#331135,#331136),(#331137,#331138,#331139),(#331140,#331141,#331142),(#331143,
#331144,#331145),(#331146,#331147,#331148),(#331149,#331150,#331151),(#331152,
#331153,#331154),(#331155,#331156,#331157),(#331158,#331159,#331160),(#331161,
#331162,#331163),(#331164,#331165,#331166),(#331167,#331168,#331169),(#331170,
#331171,#331172),(#331173,#331174,#331175),(#331176,#331177,#331178),(#331179,
#331180,#331181),(#331182,#331183,#331184),(#331185,#331186,#331187),(#331188,
#331189,#331190),(#331191,#331192,#331193),(#331194,#331195,#331196),(#331197,
#331198,#331199),(#331200,#331201,#331202),(#331203,#331204,#331205),(#331206,
#331207,#331208),(#331209,#331210,#331211),(#331212,#331213,#331214),(#331215,
#331216,#331217),(#331218,#331219,#331220),(#331221,#331222,#331223),(#331224,
#331225,#331226),(#331227,#331228,#331229),(#331230,#331231,#331232),(#331233,
#331234,#331235),(#331236,#331237,#331238),(#331239,#331240,#331241),(#331242,
#331243,#331244),(#331245,#331246,#331247),(#331248,#331249,#331250),(#331251,
#331252,#331253),(#331254,#331255,#331256),(#331257,#331258,#331259),(#331260,
#331261,#331262),(#331263,#331264,#331265),(#331266,#331267,#331268),(#331269,
#331270,#331271),(#331272,#331273,#331274),(#331275,#331276,#331277),(#331278,
#331279,#331280),(#331281,#331282,#331283),(#331284,#331285,#331286),(#331287,
#331288,#331289),(#331290,#331291,#331292),(#331293,#331294,#331295),(#331296,
#331297,#331298),(#331299,#331300,#331301),(#331302,#331303,#331304),(#331305,
#331306,#331307),(#331308,#331309,#331310),(#331311,#331312,#331313),(#331314,
#331315,#331316),(#331317,#331318,#331319),(#331320,#331321,#331322),(#331323,
#331324,#331325),(#331326,#331327,#331328),(#331329,#331330,#331331),(#331332,
#331333,#331334),(#331335,#331336,#331337),(#331338,#331339,#331340),(#331341,
#331342,#331343),(#331344,#331345,#331346),(#331347,#331348,#331349),(#331350,
#331351,#331352),(#331353,#331354,#331355),(#331356,#331357,#331358),(#331359,
#331360,#331361),(#331362,#331363,#331364),(#331365,#331366,#331367),(#331368,
#331369,#331370),(#331371,#331372,#331373),(#331374,#331375,#331376),(#331377,
#331378,#331379),(#331380,#331381,#331382),(#331383,#331384,#331385),(#331386,
#331387,#331388),(#331389,#331390,#331391),(#331392,#331393,#331394),(#331395,
#331396,#331397),(#331398,#331399,#331400),(#331401,#331402,#331403),(#331404,
#331405,#331406),(#331407,#331408,#331409),(#331410,#331411,#331412),(#331413,
#331414,#331415),(#331416,#331417,#331418),(#331419,#331420,#331421),(#331422,
#331423,#331424),(#331425,#331426,#331427),(#331428,#331429,#331430),(#331431,
#331432,#331433),(#331434,#331435,#331436),(#331437,#331438,#331439),(#331440,
#331441,#331442),(#331443,#331444,#331445),(#331446,#331447,#331448),(#331449,
#331450,#331451),(#331452,#331453,#331454),(#331455,#331456,#331457),(#331458,
#331459,#331460),(#331461,#331462,#331463),(#331464,#331465,#331466),(#331467,
#331468,#331469),(#331470,#331471,#331472),(#331473,#331474,#331475),(#331476,
#331477,#331478),(#331479,#331480,#331481),(#331482,#331483,#331484),(#331485,
#331486,#331487),(#331488,#331489,#331490),(#331491,#331492,#331493),(#331494,
#331495,#331496),(#331497,#331498,#331499),(#331500,#331501,#331502),(#331503,
#331504,#331505),(#331506,#331507,#331508),(#331509,#331510,#331511),(#331512,
#331513,#331514),(#331515,#331516,#331517),(#331518,#331519,#331520),(#331521,
#331522,#331523),(#331524,#331525,#331526),(#331527,#331528,#331529),(#331530,
#331531,#331532),(#331533,#331534,#331535),(#331536,#331537,#331538),(#331539,
#331540,#331541),(#331542,#331543,#331544),(#331545,#331546,#331547),(#331548,
#331549,#331550),(#331551,#331552,#331553),(#331554,#331555,#331556),(#331557,
#331558,#331559),(#331560,#331561,#331562),(#331563,#331564,#331565),(#331566,
#331567,#331568),(#331569,#331570,#331571),(#331572,#331573,#331574),(#331575,
#331576,#331577),(#331578,#331579,#331580),(#331581,#331582,#331583),(#331584,
#331585,#331586),(#331587,#331588,#331589),(#331590,#331591,#331592),(#331593,
#331594,#331595),(#331596,#331597,#331598),(#331599,#331600,#331601),(#331602,
#331603,#331604),(#331605,#331606,#331607),(#331608,#331609,#331610),(#331611,
#331612,#331613),(#331614,#331615,#331616),(#331617,#331618,#331619),(#331620,
#331621,#331622),(#331623,#331624,#331625),(#331626,#331627,#331628),(#331629,
#331630,#331631),(#331632,#331633,#331634),(#331635,#331636,#331637),(#331638,
#331639,#331640),(#331641,#331642,#331643),(#331644,#331645,#331646),(#331647,
#331648,#331649)),.UNSPECIFIED.,.F.,.F.,.F.,(6,1,1,1,1,1,1,1,1,1,1,1,1,
1,1,1,1,1,1,1,1,1,1,1,1,1,1,1,1,1,1,1,1,1,1,1,1,1,1,1,1,1,1,1,1,1,1,1,1,
1,1,1,1,1,1,1,1,1,1,1,1,1,1,1,1,1,1,1,1,1,1,1,1,1,1,1,1,1,1,1,1,1,1,1,1,
1,1,1,1,1,1,1,1,1,1,1,1,1,1,1,1,1,1,1,1,1,1,1,1,1,1,1,1,1,1,1,1,1,1,1,1,
1,1,1,1,1,1,1,1,1,1,1,1,1,1,1,1,1,1,1,1,1,1,1,1,1,1,1,1,1,1,1,1,1,1,1,1,
1,1,1,1,1,1,1,1,1,1,1,1,1,1,1,1,1,1,1,1,1,1,1,1,1,1,1,1,1,1,1,1,1,1,1,1,
1,1,1,1,1,1,1,1,1,1,1,1,1,1,1,1,1,1,1,1,1,1,1,1,1,1,1,1,1,1,1,1,1,1,1,1,
1,1,1,1,1,1,1,1,1,1,1,1,1,1,1,1,1,1,1,1,1,1,1,1,1,1,1,1,1,1,1,1,1,1,1,1,
1,1,1,1,1,1,1,1,1,1,1,1,1,1,1,1,1,1,1,1,1,1,1,1,1,1,1,1,1,1,1,1,1,1,1,1,
1,1,1,1,1,1,1,1,1,1,1,1,1,1,1,1,1,1,1,1,1,1,1,1,1,1,1,1,1,1,1,1,1,1,1,1,
1,1,1,1,1,1,1,1,1,1,1,1,1,1,1,1,1,1,1,1,1,1,1,1,1,1,1,1,1,1,1,1,1,1,1,1,
1,1,1,1,1,1,1,1,1,1,1,1,1,1,1,1,1,1,1,1,1,1,1,1,1,1,1,1,1,1,1,1,1,1,1,1,
1,1,1,1,1,1,1,1,1,1,1,1,1,1,1,1,1,1,1,1,1,1,1,1,1,1,1,1,1,1,1,1,1,1,1,1,
1,1,1,1,1,1,1,1,1,1,1,1,1,1,1,1,1,1,1,1,1,1,1,1,1,1,1,1,1,1,1,1,1,1,1,1,
1,1,1,1,1,1,1,1,1,1,1,1,1,1,1,1,1,1,1,1,1,1,1,1,1,1,1,1,1,1,1,1,1,1,1,1,
1,1,1,1,1,1,1,1,1,1,1,1,1,1,1,1,1,1,1,1,1,1,1,1,1,1,1,1,1,6),(2,1,2),(-0.001964159,
0.,0.001834862,0.003669725,0.005504587,0.00733945,0.009174312,0.011009174,
0.012844037,0.014678899,0.016513761,0.018348624,0.020183486,0.022018349,
0.023853211,0.025688073,0.027522936,0.029357798,0.031192661,0.033027523,
0.034862385,0.036697248,0.03853211,0.040366972,0.042201835,0.044036697,
0.04587156,0.047706422,0.049541284,0.051376147,0.053211009,0.055045872,
0.056880734,0.058715596,0.060550459,0.062385321,0.064220183,0.066055046,
0.067889908,0.069724771,0.071559633,0.073394495,0.075229358,0.07706422,
0.078899083,0.080733945,0.082568807,0.08440367,0.086238532,0.088073394,
0.089908257,0.091743119,0.093577982,0.095412844,0.097247706,0.099082569,
0.100917431,0.102752294,0.104587156,0.106422018,0.108256881,0.110091743,
0.111926606,0.113761468,0.11559633,0.117431193,0.119266055,0.121100917,
0.12293578,0.124770642,0.126605505,0.128440367,0.130275229,0.132110092,
0.133944954,0.135779817,0.137614679,0.139449541,0.141284404,0.143119266,
0.144954128,0.146788991,0.148623853,0.150458716,0.152293578,0.15412844,
0.155963303,0.157798165,0.159633028,0.16146789,0.163302752,0.165137615,
0.166972477,0.168807339,0.170642202,0.172477064,0.174311927,0.176146789,
0.177981651,0.179816514,0.181651376,0.183486239,0.185321101,0.187155963,
0.188990826,0.190825688,0.19266055,0.194495413,0.196330275,0.198165138,
0.2,0.201834862,0.203669725,0.205504587,0.20733945,0.209174312,0.211009174,
0.212844037,0.214678899,0.216513761,0.218348624,0.220183486,0.222018349,
0.223853211,0.225688073,0.227522936,0.229357798,0.231192661,0.233027523,
0.234862385,0.236697248,0.23853211,0.240366972,0.242201835,0.244036697,
0.24587156,0.247706422,0.249541284,0.251376147,0.253211009,0.255045872,
0.256880734,0.258715596,0.260550459,0.262385321,0.264220183,0.266055046,
0.267889908,0.269724771,0.271559633,0.273394495,0.275229358,0.27706422,
0.278899083,0.280733945,0.282568807,0.28440367,0.286238532,0.288073394,
0.289908257,0.291743119,0.293577982,0.295412844,0.297247706,0.299082569,
0.300917431,0.302752294,0.304587156,0.306422018,0.308256881,0.310091743,
0.311926606,0.313761468,0.31559633,0.317431193,0.319266055,0.321100917,
0.32293578,0.324770642,0.326605505,0.328440367,0.330275229,0.332110092,
0.333944954,0.335779817,0.337614679,0.339449541,0.341284404,0.343119266,
0.344954128,0.346788991,0.348623853,0.350458716,0.352293578,0.35412844,
0.355963303,0.357798165,0.359633028,0.36146789,0.363302752,0.365137615,
0.366972477,0.368807339,0.370642202,0.372477064,0.374311927,0.376146789,
0.377981651,0.379816514,0.381651376,0.383486239,0.385321101,0.387155963,
0.388990826,0.390825688,0.39266055,0.394495413,0.396330275,0.398165138,
0.4,0.401834862,0.403669725,0.405504587,0.40733945,0.409174312,0.411009174,
0.412844037,0.414678899,0.416513761,0.418348624,0.420183486,0.422018349,
0.423853211,0.425688073,0.427522936,0.429357798,0.431192661,0.433027523,
0.434862385,0.436697248,0.43853211,0.440366972,0.442201835,0.444036697,
0.44587156,0.447706422,0.449541284,0.451376147,0.453211009,0.455045872,
0.456880734,0.458715596,0.460550459,0.462385321,0.464220183,0.466055046,
0.467889908,0.469724771,0.471559633,0.473394495,0.475229358,0.47706422,
0.478899083,0.480733945,0.482568807,0.48440367,0.486238532,0.488073394,
0.489908257,0.491743119,0.493577982,0.495412844,0.497247706,0.499082569,
0.500917431,0.502752294,0.504587156,0.506422018,0.508256881,0.510091743,
0.511926606,0.513761468,0.51559633,0.517431193,0.519266055,0.521100917,
0.52293578,0.524770642,0.526605505,0.528440367,0.530275229,0.532110092,
0.533944954,0.535779817,0.537614679,0.539449541,0.541284404,0.543119266,
0.544954128,0.546788991,0.548623853,0.550458716,0.552293578,0.55412844,
0.555963303,0.557798165,0.559633028,0.56146789,0.563302752,0.565137615,
0.566972477,0.568807339,0.570642202,0.572477064,0.574311927,0.576146789,
0.577981651,0.579816514,0.581651376,0.583486239,0.585321101,0.587155963,
0.588990826,0.590825688,0.59266055,0.594495413,0.596330275,0.598165138,
0.6,0.601834862,0.603669725,0.605504587,0.60733945,0.609174312,0.611009174,
0.612844037,0.614678899,0.616513761,0.618348624,0.620183486,0.622018349,
0.623853211,0.625688073,0.627522936,0.629357798,0.631192661,0.633027523,
0.634862385,0.636697248,0.63853211,0.640366972,0.642201835,0.644036697,
0.64587156,0.647706422,0.649541284,0.651376147,0.653211009,0.655045872,
0.656880734,0.658715596,0.660550459,0.662385321,0.664220183,0.666055046,
0.667889908,0.669724771,0.671559633,0.673394495,0.675229358,0.67706422,
0.678899083,0.680733945,0.682568807,0.68440367,0.686238532,0.688073394,
0.689908257,0.691743119,0.693577982,0.695412844,0.697247706,0.699082569,
0.700917431,0.702752294,0.704587156,0.706422018,0.708256881,0.710091743,
0.711926606,0.713761468,0.71559633,0.717431193,0.719266055,0.721100917,
0.72293578,0.724770642,0.726605505,0.728440367,0.730275229,0.732110092,
0.733944954,0.735779817,0.737614679,0.739449541,0.741284404,0.743119266,
0.744954128,0.746788991,0.748623853,0.750458716,0.752293578,0.75412844,
0.755963303,0.757798165,0.759633028,0.76146789,0.763302752,0.765137615,
0.766972477,0.768807339,0.770642202,0.772477064,0.774311927,0.776146789,
0.777981651,0.779816514,0.781651376,0.783486239,0.785321101,0.787155963,
0.788990826,0.790825688,0.79266055,0.794495413,0.796330275,0.798165138,
0.8,0.801834862,0.803669725,0.805504587,0.80733945,0.809174312,0.811009174,
0.812844037,0.814678899,0.816513761,0.818348624,0.820183486,0.822018349,
0.823853211,0.825688073,0.827522936,0.829357798,0.831192661,0.833027523,
0.834862385,0.836697248,0.83853211,0.840366972,0.842201835,0.844036697,
0.84587156,0.847706422,0.849541284,0.851376147,0.853211009,0.855045872,
0.856880734,0.858715596,0.860550459,0.862385321,0.864220183,0.866055046,
0.867889908,0.869724771,0.871559633,0.873394495,0.875229358,0.87706422,
0.878899083,0.880733945,0.882568807,0.88440367,0.886238532,0.888073394,
0.889908257,0.891743119,0.893577982,0.895412844,0.897247706,0.899082569,
0.900917431,0.902752294,0.904587156,0.906422018,0.908256881,0.910091743,
0.911926606,0.913761468,0.91559633,0.917431193,0.919266055,0.921100917,
0.92293578,0.924770642,0.926605505,0.928440367,0.930275229,0.932110092,
0.933944954,0.935779817,0.937614679,0.939449541,0.941284404,0.943119266,
0.944954128,0.946788991,0.948623853,0.950458716,0.952293578,0.95412844,
0.955963303,0.957798165,0.959633028,0.96146789,0.963302752,0.965137615,
0.966972477,0.968807339,0.970642202,0.972477064,0.974311927,0.976146789,
0.977981651,0.979816514,0.981651376,0.983486239,0.985321101,0.987155963,
0.988990826,0.990825688,0.99266055,0.994495413,0.996330275,0.998165138,
1.000000000385),(0.3,1.,1.3),.UNSPECIFIED.);
#6321=B_SPLINE_SURFACE_WITH_KNOTS('',5,1,((#331654,#331655,#331656),(#331657,
#331658,#331659),(#331660,#331661,#331662),(#331663,#331664,#331665),(#331666,
#331667,#331668),(#331669,#331670,#331671),(#331672,#331673,#331674),(#331675,
#331676,#331677),(#331678,#331679,#331680),(#331681,#331682,#331683),(#331684,
#331685,#331686),(#331687,#331688,#331689),(#331690,#331691,#331692),(#331693,
#331694,#331695),(#331696,#331697,#331698),(#331699,#331700,#331701),(#331702,
#331703,#331704),(#331705,#331706,#331707),(#331708,#331709,#331710),(#331711,
#331712,#331713),(#331714,#331715,#331716),(#331717,#331718,#331719),(#331720,
#331721,#331722),(#331723,#331724,#331725),(#331726,#331727,#331728),(#331729,
#331730,#331731),(#331732,#331733,#331734),(#331735,#331736,#331737),(#331738,
#331739,#331740),(#331741,#331742,#331743),(#331744,#331745,#331746),(#331747,
#331748,#331749),(#331750,#331751,#331752),(#331753,#331754,#331755),(#331756,
#331757,#331758),(#331759,#331760,#331761),(#331762,#331763,#331764),(#331765,
#331766,#331767),(#331768,#331769,#331770),(#331771,#331772,#331773),(#331774,
#331775,#331776),(#331777,#331778,#331779),(#331780,#331781,#331782),(#331783,
#331784,#331785),(#331786,#331787,#331788),(#331789,#331790,#331791),(#331792,
#331793,#331794),(#331795,#331796,#331797),(#331798,#331799,#331800),(#331801,
#331802,#331803),(#331804,#331805,#331806),(#331807,#331808,#331809),(#331810,
#331811,#331812),(#331813,#331814,#331815),(#331816,#331817,#331818),(#331819,
#331820,#331821),(#331822,#331823,#331824),(#331825,#331826,#331827),(#331828,
#331829,#331830),(#331831,#331832,#331833),(#331834,#331835,#331836),(#331837,
#331838,#331839),(#331840,#331841,#331842),(#331843,#331844,#331845),(#331846,
#331847,#331848),(#331849,#331850,#331851),(#331852,#331853,#331854),(#331855,
#331856,#331857),(#331858,#331859,#331860),(#331861,#331862,#331863),(#331864,
#331865,#331866),(#331867,#331868,#331869),(#331870,#331871,#331872),(#331873,
#331874,#331875),(#331876,#331877,#331878),(#331879,#331880,#331881),(#331882,
#331883,#331884),(#331885,#331886,#331887),(#331888,#331889,#331890),(#331891,
#331892,#331893),(#331894,#331895,#331896),(#331897,#331898,#331899),(#331900,
#331901,#331902),(#331903,#331904,#331905),(#331906,#331907,#331908),(#331909,
#331910,#331911),(#331912,#331913,#331914),(#331915,#331916,#331917),(#331918,
#331919,#331920),(#331921,#331922,#331923),(#331924,#331925,#331926),(#331927,
#331928,#331929),(#331930,#331931,#331932),(#331933,#331934,#331935),(#331936,
#331937,#331938),(#331939,#331940,#331941),(#331942,#331943,#331944),(#331945,
#331946,#331947),(#331948,#331949,#331950),(#331951,#331952,#331953),(#331954,
#331955,#331956),(#331957,#331958,#331959),(#331960,#331961,#331962),(#331963,
#331964,#331965),(#331966,#331967,#331968),(#331969,#331970,#331971),(#331972,
#331973,#331974),(#331975,#331976,#331977),(#331978,#331979,#331980),(#331981,
#331982,#331983),(#331984,#331985,#331986),(#331987,#331988,#331989),(#331990,
#331991,#331992),(#331993,#331994,#331995),(#331996,#331997,#331998),(#331999,
#332000,#332001),(#332002,#332003,#332004),(#332005,#332006,#332007),(#332008,
#332009,#332010),(#332011,#332012,#332013),(#332014,#332015,#332016),(#332017,
#332018,#332019),(#332020,#332021,#332022),(#332023,#332024,#332025),(#332026,
#332027,#332028),(#332029,#332030,#332031),(#332032,#332033,#332034),(#332035,
#332036,#332037),(#332038,#332039,#332040),(#332041,#332042,#332043),(#332044,
#332045,#332046),(#332047,#332048,#332049),(#332050,#332051,#332052),(#332053,
#332054,#332055),(#332056,#332057,#332058),(#332059,#332060,#332061),(#332062,
#332063,#332064),(#332065,#332066,#332067),(#332068,#332069,#332070),(#332071,
#332072,#332073),(#332074,#332075,#332076),(#332077,#332078,#332079),(#332080,
#332081,#332082),(#332083,#332084,#332085),(#332086,#332087,#332088),(#332089,
#332090,#332091),(#332092,#332093,#332094),(#332095,#332096,#332097),(#332098,
#332099,#332100),(#332101,#332102,#332103),(#332104,#332105,#332106),(#332107,
#332108,#332109),(#332110,#332111,#332112),(#332113,#332114,#332115),(#332116,
#332117,#332118),(#332119,#332120,#332121),(#332122,#332123,#332124),(#332125,
#332126,#332127),(#332128,#332129,#332130),(#332131,#332132,#332133),(#332134,
#332135,#332136),(#332137,#332138,#332139),(#332140,#332141,#332142),(#332143,
#332144,#332145),(#332146,#332147,#332148),(#332149,#332150,#332151),(#332152,
#332153,#332154),(#332155,#332156,#332157),(#332158,#332159,#332160),(#332161,
#332162,#332163),(#332164,#332165,#332166),(#332167,#332168,#332169),(#332170,
#332171,#332172),(#332173,#332174,#332175),(#332176,#332177,#332178),(#332179,
#332180,#332181),(#332182,#332183,#332184),(#332185,#332186,#332187),(#332188,
#332189,#332190),(#332191,#332192,#332193),(#332194,#332195,#332196),(#332197,
#332198,#332199),(#332200,#332201,#332202),(#332203,#332204,#332205),(#332206,
#332207,#332208),(#332209,#332210,#332211),(#332212,#332213,#332214),(#332215,
#332216,#332217),(#332218,#332219,#332220),(#332221,#332222,#332223),(#332224,
#332225,#332226),(#332227,#332228,#332229),(#332230,#332231,#332232),(#332233,
#332234,#332235),(#332236,#332237,#332238),(#332239,#332240,#332241),(#332242,
#332243,#332244),(#332245,#332246,#332247),(#332248,#332249,#332250),(#332251,
#332252,#332253),(#332254,#332255,#332256),(#332257,#332258,#332259),(#332260,
#332261,#332262),(#332263,#332264,#332265),(#332266,#332267,#332268),(#332269,
#332270,#332271),(#332272,#332273,#332274),(#332275,#332276,#332277),(#332278,
#332279,#332280),(#332281,#332282,#332283),(#332284,#332285,#332286),(#332287,
#332288,#332289),(#332290,#332291,#332292),(#332293,#332294,#332295),(#332296,
#332297,#332298),(#332299,#332300,#332301),(#332302,#332303,#332304),(#332305,
#332306,#332307),(#332308,#332309,#332310),(#332311,#332312,#332313),(#332314,
#332315,#332316),(#332317,#332318,#332319),(#332320,#332321,#332322),(#332323,
#332324,#332325),(#332326,#332327,#332328),(#332329,#332330,#332331),(#332332,
#332333,#332334),(#332335,#332336,#332337),(#332338,#332339,#332340),(#332341,
#332342,#332343),(#332344,#332345,#332346),(#332347,#332348,#332349),(#332350,
#332351,#332352),(#332353,#332354,#332355),(#332356,#332357,#332358),(#332359,
#332360,#332361),(#332362,#332363,#332364),(#332365,#332366,#332367),(#332368,
#332369,#332370),(#332371,#332372,#332373),(#332374,#332375,#332376),(#332377,
#332378,#332379),(#332380,#332381,#332382),(#332383,#332384,#332385),(#332386,
#332387,#332388),(#332389,#332390,#332391),(#332392,#332393,#332394),(#332395,
#332396,#332397),(#332398,#332399,#332400),(#332401,#332402,#332403),(#332404,
#332405,#332406),(#332407,#332408,#332409),(#332410,#332411,#332412),(#332413,
#332414,#332415),(#332416,#332417,#332418),(#332419,#332420,#332421),(#332422,
#332423,#332424),(#332425,#332426,#332427),(#332428,#332429,#332430),(#332431,
#332432,#332433),(#332434,#332435,#332436),(#332437,#332438,#332439),(#332440,
#332441,#332442),(#332443,#332444,#332445),(#332446,#332447,#332448),(#332449,
#332450,#332451),(#332452,#332453,#332454),(#332455,#332456,#332457),(#332458,
#332459,#332460),(#332461,#332462,#332463),(#332464,#332465,#332466),(#332467,
#332468,#332469),(#332470,#332471,#332472),(#332473,#332474,#332475),(#332476,
#332477,#332478),(#332479,#332480,#332481),(#332482,#332483,#332484),(#332485,
#332486,#332487),(#332488,#332489,#332490),(#332491,#332492,#332493),(#332494,
#332495,#332496),(#332497,#332498,#332499),(#332500,#332501,#332502),(#332503,
#332504,#332505),(#332506,#332507,#332508),(#332509,#332510,#332511),(#332512,
#332513,#332514),(#332515,#332516,#332517),(#332518,#332519,#332520),(#332521,
#332522,#332523),(#332524,#332525,#332526),(#332527,#332528,#332529),(#332530,
#332531,#332532),(#332533,#332534,#332535),(#332536,#332537,#332538),(#332539,
#332540,#332541),(#332542,#332543,#332544),(#332545,#332546,#332547),(#332548,
#332549,#332550),(#332551,#332552,#332553),(#332554,#332555,#332556),(#332557,
#332558,#332559),(#332560,#332561,#332562),(#332563,#332564,#332565),(#332566,
#332567,#332568),(#332569,#332570,#332571),(#332572,#332573,#332574),(#332575,
#332576,#332577),(#332578,#332579,#332580),(#332581,#332582,#332583),(#332584,
#332585,#332586),(#332587,#332588,#332589),(#332590,#332591,#332592),(#332593,
#332594,#332595),(#332596,#332597,#332598),(#332599,#332600,#332601),(#332602,
#332603,#332604),(#332605,#332606,#332607),(#332608,#332609,#332610),(#332611,
#332612,#332613),(#332614,#332615,#332616),(#332617,#332618,#332619),(#332620,
#332621,#332622),(#332623,#332624,#332625),(#332626,#332627,#332628),(#332629,
#332630,#332631),(#332632,#332633,#332634),(#332635,#332636,#332637),(#332638,
#332639,#332640),(#332641,#332642,#332643),(#332644,#332645,#332646),(#332647,
#332648,#332649),(#332650,#332651,#332652),(#332653,#332654,#332655),(#332656,
#332657,#332658),(#332659,#332660,#332661),(#332662,#332663,#332664),(#332665,
#332666,#332667),(#332668,#332669,#332670),(#332671,#332672,#332673),(#332674,
#332675,#332676),(#332677,#332678,#332679),(#332680,#332681,#332682),(#332683,
#332684,#332685),(#332686,#332687,#332688),(#332689,#332690,#332691),(#332692,
#332693,#332694),(#332695,#332696,#332697),(#332698,#332699,#332700),(#332701,
#332702,#332703),(#332704,#332705,#332706),(#332707,#332708,#332709),(#332710,
#332711,#332712),(#332713,#332714,#332715),(#332716,#332717,#332718),(#332719,
#332720,#332721),(#332722,#332723,#332724),(#332725,#332726,#332727),(#332728,
#332729,#332730),(#332731,#332732,#332733),(#332734,#332735,#332736),(#332737,
#332738,#332739),(#332740,#332741,#332742),(#332743,#332744,#332745),(#332746,
#332747,#332748),(#332749,#332750,#332751),(#332752,#332753,#332754),(#332755,
#332756,#332757),(#332758,#332759,#332760),(#332761,#332762,#332763),(#332764,
#332765,#332766),(#332767,#332768,#332769),(#332770,#332771,#332772),(#332773,
#332774,#332775),(#332776,#332777,#332778),(#332779,#332780,#332781),(#332782,
#332783,#332784),(#332785,#332786,#332787),(#332788,#332789,#332790),(#332791,
#332792,#332793),(#332794,#332795,#332796),(#332797,#332798,#332799),(#332800,
#332801,#332802),(#332803,#332804,#332805),(#332806,#332807,#332808),(#332809,
#332810,#332811),(#332812,#332813,#332814),(#332815,#332816,#332817),(#332818,
#332819,#332820),(#332821,#332822,#332823),(#332824,#332825,#332826),(#332827,
#332828,#332829),(#332830,#332831,#332832),(#332833,#332834,#332835),(#332836,
#332837,#332838),(#332839,#332840,#332841),(#332842,#332843,#332844),(#332845,
#332846,#332847),(#332848,#332849,#332850),(#332851,#332852,#332853),(#332854,
#332855,#332856),(#332857,#332858,#332859),(#332860,#332861,#332862),(#332863,
#332864,#332865),(#332866,#332867,#332868),(#332869,#332870,#332871),(#332872,
#332873,#332874),(#332875,#332876,#332877),(#332878,#332879,#332880),(#332881,
#332882,#332883),(#332884,#332885,#332886),(#332887,#332888,#332889),(#332890,
#332891,#332892),(#332893,#332894,#332895),(#332896,#332897,#332898),(#332899,
#332900,#332901),(#332902,#332903,#332904),(#332905,#332906,#332907),(#332908,
#332909,#332910),(#332911,#332912,#332913),(#332914,#332915,#332916),(#332917,
#332918,#332919),(#332920,#332921,#332922),(#332923,#332924,#332925),(#332926,
#332927,#332928),(#332929,#332930,#332931),(#332932,#332933,#332934),(#332935,
#332936,#332937),(#332938,#332939,#332940),(#332941,#332942,#332943),(#332944,
#332945,#332946),(#332947,#332948,#332949),(#332950,#332951,#332952),(#332953,
#332954,#332955),(#332956,#332957,#332958),(#332959,#332960,#332961),(#332962,
#332963,#332964),(#332965,#332966,#332967),(#332968,#332969,#332970),(#332971,
#332972,#332973),(#332974,#332975,#332976),(#332977,#332978,#332979),(#332980,
#332981,#332982),(#332983,#332984,#332985),(#332986,#332987,#332988),(#332989,
#332990,#332991),(#332992,#332993,#332994),(#332995,#332996,#332997),(#332998,
#332999,#333000),(#333001,#333002,#333003),(#333004,#333005,#333006),(#333007,
#333008,#333009),(#333010,#333011,#333012),(#333013,#333014,#333015),(#333016,
#333017,#333018),(#333019,#333020,#333021),(#333022,#333023,#333024),(#333025,
#333026,#333027),(#333028,#333029,#333030),(#333031,#333032,#333033),(#333034,
#333035,#333036),(#333037,#333038,#333039),(#333040,#333041,#333042),(#333043,
#333044,#333045),(#333046,#333047,#333048),(#333049,#333050,#333051),(#333052,
#333053,#333054),(#333055,#333056,#333057),(#333058,#333059,#333060),(#333061,
#333062,#333063),(#333064,#333065,#333066),(#333067,#333068,#333069),(#333070,
#333071,#333072),(#333073,#333074,#333075),(#333076,#333077,#333078),(#333079,
#333080,#333081),(#333082,#333083,#333084),(#333085,#333086,#333087),(#333088,
#333089,#333090),(#333091,#333092,#333093),(#333094,#333095,#333096),(#333097,
#333098,#333099),(#333100,#333101,#333102),(#333103,#333104,#333105),(#333106,
#333107,#333108),(#333109,#333110,#333111),(#333112,#333113,#333114),(#333115,
#333116,#333117),(#333118,#333119,#333120),(#333121,#333122,#333123),(#333124,
#333125,#333126),(#333127,#333128,#333129),(#333130,#333131,#333132),(#333133,
#333134,#333135),(#333136,#333137,#333138),(#333139,#333140,#333141),(#333142,
#333143,#333144),(#333145,#333146,#333147),(#333148,#333149,#333150),(#333151,
#333152,#333153),(#333154,#333155,#333156),(#333157,#333158,#333159),(#333160,
#333161,#333162),(#333163,#333164,#333165),(#333166,#333167,#333168),(#333169,
#333170,#333171),(#333172,#333173,#333174),(#333175,#333176,#333177),(#333178,
#333179,#333180),(#333181,#333182,#333183),(#333184,#333185,#333186),(#333187,
#333188,#333189),(#333190,#333191,#333192),(#333193,#333194,#333195),(#333196,
#333197,#333198),(#333199,#333200,#333201),(#333202,#333203,#333204),(#333205,
#333206,#333207),(#333208,#333209,#333210),(#333211,#333212,#333213),(#333214,
#333215,#333216),(#333217,#333218,#333219),(#333220,#333221,#333222),(#333223,
#333224,#333225),(#333226,#333227,#333228),(#333229,#333230,#333231),(#333232,
#333233,#333234),(#333235,#333236,#333237),(#333238,#333239,#333240),(#333241,
#333242,#333243),(#333244,#333245,#333246),(#333247,#333248,#333249),(#333250,
#333251,#333252),(#333253,#333254,#333255),(#333256,#333257,#333258),(#333259,
#333260,#333261),(#333262,#333263,#333264),(#333265,#333266,#333267),(#333268,
#333269,#333270),(#333271,#333272,#333273),(#333274,#333275,#333276),(#333277,
#333278,#333279),(#333280,#333281,#333282),(#333283,#333284,#333285),(#333286,
#333287,#333288),(#333289,#333290,#333291),(#333292,#333293,#333294),(#333295,
#333296,#333297),(#333298,#333299,#333300),(#333301,#333302,#333303)),
 .UNSPECIFIED.,.F.,.F.,.F.,(6,1,1,1,1,1,1,1,1,1,1,1,1,1,1,1,1,1,1,1,1,1,
1,1,1,1,1,1,1,1,1,1,1,1,1,1,1,1,1,1,1,1,1,1,1,1,1,1,1,1,1,1,1,1,1,1,1,1,
1,1,1,1,1,1,1,1,1,1,1,1,1,1,1,1,1,1,1,1,1,1,1,1,1,1,1,1,1,1,1,1,1,1,1,1,
1,1,1,1,1,1,1,1,1,1,1,1,1,1,1,1,1,1,1,1,1,1,1,1,1,1,1,1,1,1,1,1,1,1,1,1,
1,1,1,1,1,1,1,1,1,1,1,1,1,1,1,1,1,1,1,1,1,1,1,1,1,1,1,1,1,1,1,1,1,1,1,1,
1,1,1,1,1,1,1,1,1,1,1,1,1,1,1,1,1,1,1,1,1,1,1,1,1,1,1,1,1,1,1,1,1,1,1,1,
1,1,1,1,1,1,1,1,1,1,1,1,1,1,1,1,1,1,1,1,1,1,1,1,1,1,1,1,1,1,1,1,1,1,1,1,
1,1,1,1,1,1,1,1,1,1,1,1,1,1,1,1,1,1,1,1,1,1,1,1,1,1,1,1,1,1,1,1,1,1,1,1,
1,1,1,1,1,1,1,1,1,1,1,1,1,1,1,1,1,1,1,1,1,1,1,1,1,1,1,1,1,1,1,1,1,1,1,1,
1,1,1,1,1,1,1,1,1,1,1,1,1,1,1,1,1,1,1,1,1,1,1,1,1,1,1,1,1,1,1,1,1,1,1,1,
1,1,1,1,1,1,1,1,1,1,1,1,1,1,1,1,1,1,1,1,1,1,1,1,1,1,1,1,1,1,1,1,1,1,1,1,
1,1,1,1,1,1,1,1,1,1,1,1,1,1,1,1,1,1,1,1,1,1,1,1,1,1,1,1,1,1,1,1,1,1,1,1,
1,1,1,1,1,1,1,1,1,1,1,1,1,1,1,1,1,1,1,1,1,1,1,1,1,1,1,1,1,1,1,1,1,1,1,1,
1,1,1,1,1,1,1,1,1,1,1,1,1,1,1,1,1,1,1,1,1,1,1,1,1,1,1,1,1,1,1,1,1,1,1,1,
1,1,1,1,1,1,1,1,1,1,1,1,1,1,1,1,1,1,1,1,1,1,1,1,1,1,1,1,1,1,1,1,1,1,1,1,
1,1,1,1,1,1,1,1,1,1,1,1,1,1,1,1,1,1,1,6),(2,1,2),(-1.,-0.998165138,-0.996330275,
-0.994495413,-0.99266055,-0.990825688,-0.988990826,-0.987155963,-0.985321101,
-0.983486239,-0.981651376,-0.979816514,-0.977981651,-0.976146789,-0.974311927,
-0.972477064,-0.970642202,-0.968807339,-0.966972477,-0.965137615,-0.963302752,
-0.96146789,-0.959633028,-0.957798165,-0.955963303,-0.95412844,-0.952293578,
-0.950458716,-0.948623853,-0.946788991,-0.944954128,-0.943119266,-0.941284404,
-0.939449541,-0.937614679,-0.935779817,-0.933944954,-0.932110092,-0.930275229,
-0.928440367,-0.926605505,-0.924770642,-0.92293578,-0.921100917,-0.919266055,
-0.917431193,-0.91559633,-0.913761468,-0.911926606,-0.910091743,-0.908256881,
-0.906422018,-0.904587156,-0.902752294,-0.900917431,-0.899082569,-0.897247706,
-0.895412844,-0.893577982,-0.891743119,-0.889908257,-0.888073394,-0.886238532,
-0.88440367,-0.882568807,-0.880733945,-0.878899083,-0.87706422,-0.875229358,
-0.873394495,-0.871559633,-0.869724771,-0.867889908,-0.866055046,-0.864220183,
-0.862385321,-0.860550459,-0.858715596,-0.856880734,-0.855045872,-0.853211009,
-0.851376147,-0.849541284,-0.847706422,-0.84587156,-0.844036697,-0.842201835,
-0.840366972,-0.83853211,-0.836697248,-0.834862385,-0.833027523,-0.831192661,
-0.829357798,-0.827522936,-0.825688073,-0.823853211,-0.822018349,-0.820183486,
-0.818348624,-0.816513761,-0.814678899,-0.812844037,-0.811009174,-0.809174312,
-0.80733945,-0.805504587,-0.803669725,-0.801834862,-0.8,-0.798165138,-0.796330275,
-0.794495413,-0.79266055,-0.790825688,-0.788990826,-0.787155963,-0.785321101,
-0.783486239,-0.781651376,-0.779816514,-0.777981651,-0.776146789,-0.774311927,
-0.772477064,-0.770642202,-0.768807339,-0.766972477,-0.765137615,-0.763302752,
-0.76146789,-0.759633028,-0.757798165,-0.755963303,-0.75412844,-0.752293578,
-0.750458716,-0.748623853,-0.746788991,-0.744954128,-0.743119266,-0.741284404,
-0.739449541,-0.737614679,-0.735779817,-0.733944954,-0.732110092,-0.730275229,
-0.728440367,-0.726605505,-0.724770642,-0.72293578,-0.721100917,-0.719266055,
-0.717431193,-0.71559633,-0.713761468,-0.711926606,-0.710091743,-0.708256881,
-0.706422018,-0.704587156,-0.702752294,-0.700917431,-0.699082569,-0.697247706,
-0.695412844,-0.693577982,-0.691743119,-0.689908257,-0.688073394,-0.686238532,
-0.68440367,-0.682568807,-0.680733945,-0.678899083,-0.67706422,-0.675229358,
-0.673394495,-0.671559633,-0.669724771,-0.667889908,-0.666055046,-0.664220183,
-0.662385321,-0.660550459,-0.658715596,-0.656880734,-0.655045872,-0.653211009,
-0.651376147,-0.649541284,-0.647706422,-0.64587156,-0.644036697,-0.642201835,
-0.640366972,-0.63853211,-0.636697248,-0.634862385,-0.633027523,-0.631192661,
-0.629357798,-0.627522936,-0.625688073,-0.623853211,-0.622018349,-0.620183486,
-0.618348624,-0.616513761,-0.614678899,-0.612844037,-0.611009174,-0.609174312,
-0.60733945,-0.605504587,-0.603669725,-0.601834862,-0.6,-0.598165138,-0.596330275,
-0.594495413,-0.59266055,-0.590825688,-0.588990826,-0.587155963,-0.585321101,
-0.583486239,-0.581651376,-0.579816514,-0.577981651,-0.576146789,-0.574311927,
-0.572477064,-0.570642202,-0.568807339,-0.566972477,-0.565137615,-0.563302752,
-0.56146789,-0.559633028,-0.557798165,-0.555963303,-0.55412844,-0.552293578,
-0.550458716,-0.548623853,-0.546788991,-0.544954128,-0.543119266,-0.541284404,
-0.539449541,-0.537614679,-0.535779817,-0.533944954,-0.532110092,-0.530275229,
-0.528440367,-0.526605505,-0.524770642,-0.52293578,-0.521100917,-0.519266055,
-0.517431193,-0.51559633,-0.513761468,-0.511926606,-0.510091743,-0.508256881,
-0.506422018,-0.504587156,-0.502752294,-0.500917431,-0.499082569,-0.497247706,
-0.495412844,-0.493577982,-0.491743119,-0.489908257,-0.488073394,-0.486238532,
-0.48440367,-0.482568807,-0.480733945,-0.478899083,-0.47706422,-0.475229358,
-0.473394495,-0.471559633,-0.469724771,-0.467889908,-0.466055046,-0.464220183,
-0.462385321,-0.460550459,-0.458715596,-0.456880734,-0.455045872,-0.453211009,
-0.451376147,-0.449541284,-0.447706422,-0.44587156,-0.444036697,-0.442201835,
-0.440366972,-0.43853211,-0.436697248,-0.434862385,-0.433027523,-0.431192661,
-0.429357798,-0.427522936,-0.425688073,-0.423853211,-0.422018349,-0.420183486,
-0.418348624,-0.416513761,-0.414678899,-0.412844037,-0.411009174,-0.409174312,
-0.40733945,-0.405504587,-0.403669725,-0.401834862,-0.4,-0.398165138,-0.396330275,
-0.394495413,-0.39266055,-0.390825688,-0.388990826,-0.387155963,-0.385321101,
-0.383486239,-0.381651376,-0.379816514,-0.377981651,-0.376146789,-0.374311927,
-0.372477064,-0.370642202,-0.368807339,-0.366972477,-0.365137615,-0.363302752,
-0.36146789,-0.359633028,-0.357798165,-0.355963303,-0.35412844,-0.352293578,
-0.350458716,-0.348623853,-0.346788991,-0.344954128,-0.343119266,-0.341284404,
-0.339449541,-0.337614679,-0.335779817,-0.333944954,-0.332110092,-0.330275229,
-0.328440367,-0.326605505,-0.324770642,-0.32293578,-0.321100917,-0.319266055,
-0.317431193,-0.31559633,-0.313761468,-0.311926606,-0.310091743,-0.308256881,
-0.306422018,-0.304587156,-0.302752294,-0.300917431,-0.299082569,-0.297247706,
-0.295412844,-0.293577982,-0.291743119,-0.289908257,-0.288073394,-0.286238532,
-0.28440367,-0.282568807,-0.280733945,-0.278899083,-0.27706422,-0.275229358,
-0.273394495,-0.271559633,-0.269724771,-0.267889908,-0.266055046,-0.264220183,
-0.262385321,-0.260550459,-0.258715596,-0.256880734,-0.255045872,-0.253211009,
-0.251376147,-0.249541284,-0.247706422,-0.24587156,-0.244036697,-0.242201835,
-0.240366972,-0.23853211,-0.236697248,-0.234862385,-0.233027523,-0.231192661,
-0.229357798,-0.227522936,-0.225688073,-0.223853211,-0.222018349,-0.220183486,
-0.218348624,-0.216513761,-0.214678899,-0.212844037,-0.211009174,-0.209174312,
-0.20733945,-0.205504587,-0.203669725,-0.201834862,-0.2,-0.198165138,-0.196330275,
-0.194495413,-0.19266055,-0.190825688,-0.188990826,-0.187155963,-0.185321101,
-0.183486239,-0.181651376,-0.179816514,-0.177981651,-0.176146789,-0.174311927,
-0.172477064,-0.170642202,-0.168807339,-0.166972477,-0.165137615,-0.163302752,
-0.16146789,-0.159633028,-0.157798165,-0.155963303,-0.15412844,-0.152293578,
-0.150458716,-0.148623853,-0.146788991,-0.144954128,-0.143119266,-0.141284404,
-0.139449541,-0.137614679,-0.135779817,-0.133944954,-0.132110092,-0.130275229,
-0.128440367,-0.126605505,-0.124770642,-0.12293578,-0.121100917,-0.119266055,
-0.117431193,-0.11559633,-0.113761468,-0.111926606,-0.110091743,-0.108256881,
-0.106422018,-0.104587156,-0.102752294,-0.100917431,-0.099082569,-0.097247706,
-0.095412844,-0.093577982,-0.091743119,-0.089908257,-0.088073394,-0.086238532,
-0.08440367,-0.082568807,-0.080733945,-0.078899083,-0.07706422,-0.075229358,
-0.073394495,-0.071559633,-0.069724771,-0.067889908,-0.066055046,-0.064220183,
-0.062385321,-0.060550459,-0.058715596,-0.056880734,-0.055045872,-0.053211009,
-0.051376147,-0.049541284,-0.047706422,-0.04587156,-0.044036697,-0.042201835,
-0.040366972,-0.03853211,-0.036697248,-0.034862385,-0.033027523,-0.031192661,
-0.029357798,-0.027522936,-0.025688073,-0.023853211,-0.022018349,-0.020183486,
-0.018348624,-0.016513761,-0.014678899,-0.012844037,-0.011009174,-0.009174312,
-0.00733945,-0.005504587,-0.003669725,-0.001834862,0.000982147),(0.3,1.,
1.3),.UNSPECIFIED.);
#6322=B_SPLINE_SURFACE_WITH_KNOTS('',5,1,((#333307,#333308,#333309),(#333310,
#333311,#333312),(#333313,#333314,#333315),(#333316,#333317,#333318),(#333319,
#333320,#333321),(#333322,#333323,#333324),(#333325,#333326,#333327),(#333328,
#333329,#333330),(#333331,#333332,#333333),(#333334,#333335,#333336),(#333337,
#333338,#333339),(#333340,#333341,#333342),(#333343,#333344,#333345),(#333346,
#333347,#333348),(#333349,#333350,#333351),(#333352,#333353,#333354),(#333355,
#333356,#333357),(#333358,#333359,#333360),(#333361,#333362,#333363),(#333364,
#333365,#333366),(#333367,#333368,#333369),(#333370,#333371,#333372),(#333373,
#333374,#333375),(#333376,#333377,#333378),(#333379,#333380,#333381),(#333382,
#333383,#333384),(#333385,#333386,#333387),(#333388,#333389,#333390),(#333391,
#333392,#333393),(#333394,#333395,#333396),(#333397,#333398,#333399),(#333400,
#333401,#333402),(#333403,#333404,#333405),(#333406,#333407,#333408),(#333409,
#333410,#333411),(#333412,#333413,#333414),(#333415,#333416,#333417),(#333418,
#333419,#333420),(#333421,#333422,#333423),(#333424,#333425,#333426),(#333427,
#333428,#333429),(#333430,#333431,#333432),(#333433,#333434,#333435),(#333436,
#333437,#333438),(#333439,#333440,#333441),(#333442,#333443,#333444),(#333445,
#333446,#333447),(#333448,#333449,#333450),(#333451,#333452,#333453),(#333454,
#333455,#333456),(#333457,#333458,#333459),(#333460,#333461,#333462),(#333463,
#333464,#333465),(#333466,#333467,#333468),(#333469,#333470,#333471),(#333472,
#333473,#333474),(#333475,#333476,#333477),(#333478,#333479,#333480),(#333481,
#333482,#333483),(#333484,#333485,#333486),(#333487,#333488,#333489),(#333490,
#333491,#333492),(#333493,#333494,#333495),(#333496,#333497,#333498),(#333499,
#333500,#333501),(#333502,#333503,#333504),(#333505,#333506,#333507),(#333508,
#333509,#333510),(#333511,#333512,#333513),(#333514,#333515,#333516),(#333517,
#333518,#333519),(#333520,#333521,#333522),(#333523,#333524,#333525),(#333526,
#333527,#333528),(#333529,#333530,#333531),(#333532,#333533,#333534),(#333535,
#333536,#333537),(#333538,#333539,#333540),(#333541,#333542,#333543),(#333544,
#333545,#333546),(#333547,#333548,#333549),(#333550,#333551,#333552),(#333553,
#333554,#333555),(#333556,#333557,#333558),(#333559,#333560,#333561),(#333562,
#333563,#333564),(#333565,#333566,#333567),(#333568,#333569,#333570),(#333571,
#333572,#333573),(#333574,#333575,#333576),(#333577,#333578,#333579),(#333580,
#333581,#333582),(#333583,#333584,#333585),(#333586,#333587,#333588),(#333589,
#333590,#333591),(#333592,#333593,#333594),(#333595,#333596,#333597),(#333598,
#333599,#333600),(#333601,#333602,#333603),(#333604,#333605,#333606),(#333607,
#333608,#333609),(#333610,#333611,#333612),(#333613,#333614,#333615),(#333616,
#333617,#333618),(#333619,#333620,#333621),(#333622,#333623,#333624),(#333625,
#333626,#333627),(#333628,#333629,#333630),(#333631,#333632,#333633),(#333634,
#333635,#333636),(#333637,#333638,#333639),(#333640,#333641,#333642),(#333643,
#333644,#333645),(#333646,#333647,#333648),(#333649,#333650,#333651),(#333652,
#333653,#333654),(#333655,#333656,#333657),(#333658,#333659,#333660),(#333661,
#333662,#333663),(#333664,#333665,#333666),(#333667,#333668,#333669),(#333670,
#333671,#333672),(#333673,#333674,#333675),(#333676,#333677,#333678),(#333679,
#333680,#333681),(#333682,#333683,#333684),(#333685,#333686,#333687),(#333688,
#333689,#333690),(#333691,#333692,#333693),(#333694,#333695,#333696),(#333697,
#333698,#333699),(#333700,#333701,#333702),(#333703,#333704,#333705),(#333706,
#333707,#333708),(#333709,#333710,#333711),(#333712,#333713,#333714),(#333715,
#333716,#333717),(#333718,#333719,#333720),(#333721,#333722,#333723),(#333724,
#333725,#333726),(#333727,#333728,#333729),(#333730,#333731,#333732),(#333733,
#333734,#333735),(#333736,#333737,#333738),(#333739,#333740,#333741),(#333742,
#333743,#333744),(#333745,#333746,#333747),(#333748,#333749,#333750),(#333751,
#333752,#333753),(#333754,#333755,#333756),(#333757,#333758,#333759),(#333760,
#333761,#333762),(#333763,#333764,#333765),(#333766,#333767,#333768),(#333769,
#333770,#333771),(#333772,#333773,#333774),(#333775,#333776,#333777),(#333778,
#333779,#333780),(#333781,#333782,#333783),(#333784,#333785,#333786),(#333787,
#333788,#333789),(#333790,#333791,#333792),(#333793,#333794,#333795),(#333796,
#333797,#333798),(#333799,#333800,#333801),(#333802,#333803,#333804),(#333805,
#333806,#333807),(#333808,#333809,#333810),(#333811,#333812,#333813),(#333814,
#333815,#333816),(#333817,#333818,#333819),(#333820,#333821,#333822),(#333823,
#333824,#333825),(#333826,#333827,#333828),(#333829,#333830,#333831),(#333832,
#333833,#333834),(#333835,#333836,#333837),(#333838,#333839,#333840),(#333841,
#333842,#333843),(#333844,#333845,#333846),(#333847,#333848,#333849),(#333850,
#333851,#333852),(#333853,#333854,#333855),(#333856,#333857,#333858),(#333859,
#333860,#333861),(#333862,#333863,#333864),(#333865,#333866,#333867),(#333868,
#333869,#333870),(#333871,#333872,#333873),(#333874,#333875,#333876),(#333877,
#333878,#333879),(#333880,#333881,#333882),(#333883,#333884,#333885),(#333886,
#333887,#333888),(#333889,#333890,#333891),(#333892,#333893,#333894),(#333895,
#333896,#333897),(#333898,#333899,#333900),(#333901,#333902,#333903),(#333904,
#333905,#333906),(#333907,#333908,#333909),(#333910,#333911,#333912),(#333913,
#333914,#333915),(#333916,#333917,#333918),(#333919,#333920,#333921),(#333922,
#333923,#333924),(#333925,#333926,#333927),(#333928,#333929,#333930),(#333931,
#333932,#333933),(#333934,#333935,#333936),(#333937,#333938,#333939),(#333940,
#333941,#333942),(#333943,#333944,#333945),(#333946,#333947,#333948),(#333949,
#333950,#333951),(#333952,#333953,#333954),(#333955,#333956,#333957),(#333958,
#333959,#333960),(#333961,#333962,#333963),(#333964,#333965,#333966),(#333967,
#333968,#333969),(#333970,#333971,#333972),(#333973,#333974,#333975),(#333976,
#333977,#333978),(#333979,#333980,#333981),(#333982,#333983,#333984),(#333985,
#333986,#333987),(#333988,#333989,#333990),(#333991,#333992,#333993),(#333994,
#333995,#333996),(#333997,#333998,#333999),(#334000,#334001,#334002),(#334003,
#334004,#334005),(#334006,#334007,#334008),(#334009,#334010,#334011),(#334012,
#334013,#334014),(#334015,#334016,#334017),(#334018,#334019,#334020),(#334021,
#334022,#334023),(#334024,#334025,#334026),(#334027,#334028,#334029),(#334030,
#334031,#334032),(#334033,#334034,#334035),(#334036,#334037,#334038),(#334039,
#334040,#334041),(#334042,#334043,#334044),(#334045,#334046,#334047),(#334048,
#334049,#334050),(#334051,#334052,#334053),(#334054,#334055,#334056),(#334057,
#334058,#334059),(#334060,#334061,#334062),(#334063,#334064,#334065),(#334066,
#334067,#334068),(#334069,#334070,#334071),(#334072,#334073,#334074),(#334075,
#334076,#334077),(#334078,#334079,#334080),(#334081,#334082,#334083),(#334084,
#334085,#334086),(#334087,#334088,#334089),(#334090,#334091,#334092),(#334093,
#334094,#334095),(#334096,#334097,#334098),(#334099,#334100,#334101),(#334102,
#334103,#334104),(#334105,#334106,#334107),(#334108,#334109,#334110),(#334111,
#334112,#334113),(#334114,#334115,#334116),(#334117,#334118,#334119),(#334120,
#334121,#334122),(#334123,#334124,#334125),(#334126,#334127,#334128),(#334129,
#334130,#334131),(#334132,#334133,#334134),(#334135,#334136,#334137),(#334138,
#334139,#334140),(#334141,#334142,#334143),(#334144,#334145,#334146),(#334147,
#334148,#334149),(#334150,#334151,#334152),(#334153,#334154,#334155),(#334156,
#334157,#334158),(#334159,#334160,#334161),(#334162,#334163,#334164),(#334165,
#334166,#334167),(#334168,#334169,#334170),(#334171,#334172,#334173),(#334174,
#334175,#334176),(#334177,#334178,#334179),(#334180,#334181,#334182),(#334183,
#334184,#334185),(#334186,#334187,#334188),(#334189,#334190,#334191),(#334192,
#334193,#334194),(#334195,#334196,#334197),(#334198,#334199,#334200),(#334201,
#334202,#334203),(#334204,#334205,#334206),(#334207,#334208,#334209),(#334210,
#334211,#334212),(#334213,#334214,#334215),(#334216,#334217,#334218),(#334219,
#334220,#334221),(#334222,#334223,#334224),(#334225,#334226,#334227),(#334228,
#334229,#334230),(#334231,#334232,#334233),(#334234,#334235,#334236),(#334237,
#334238,#334239),(#334240,#334241,#334242),(#334243,#334244,#334245),(#334246,
#334247,#334248),(#334249,#334250,#334251),(#334252,#334253,#334254),(#334255,
#334256,#334257),(#334258,#334259,#334260),(#334261,#334262,#334263),(#334264,
#334265,#334266),(#334267,#334268,#334269),(#334270,#334271,#334272),(#334273,
#334274,#334275),(#334276,#334277,#334278),(#334279,#334280,#334281),(#334282,
#334283,#334284),(#334285,#334286,#334287),(#334288,#334289,#334290),(#334291,
#334292,#334293),(#334294,#334295,#334296),(#334297,#334298,#334299),(#334300,
#334301,#334302),(#334303,#334304,#334305),(#334306,#334307,#334308),(#334309,
#334310,#334311),(#334312,#334313,#334314),(#334315,#334316,#334317),(#334318,
#334319,#334320),(#334321,#334322,#334323),(#334324,#334325,#334326),(#334327,
#334328,#334329),(#334330,#334331,#334332),(#334333,#334334,#334335),(#334336,
#334337,#334338),(#334339,#334340,#334341),(#334342,#334343,#334344),(#334345,
#334346,#334347),(#334348,#334349,#334350),(#334351,#334352,#334353),(#334354,
#334355,#334356),(#334357,#334358,#334359),(#334360,#334361,#334362),(#334363,
#334364,#334365),(#334366,#334367,#334368),(#334369,#334370,#334371),(#334372,
#334373,#334374),(#334375,#334376,#334377),(#334378,#334379,#334380),(#334381,
#334382,#334383),(#334384,#334385,#334386),(#334387,#334388,#334389),(#334390,
#334391,#334392),(#334393,#334394,#334395),(#334396,#334397,#334398),(#334399,
#334400,#334401),(#334402,#334403,#334404),(#334405,#334406,#334407),(#334408,
#334409,#334410),(#334411,#334412,#334413),(#334414,#334415,#334416),(#334417,
#334418,#334419),(#334420,#334421,#334422),(#334423,#334424,#334425),(#334426,
#334427,#334428),(#334429,#334430,#334431),(#334432,#334433,#334434),(#334435,
#334436,#334437),(#334438,#334439,#334440),(#334441,#334442,#334443),(#334444,
#334445,#334446),(#334447,#334448,#334449),(#334450,#334451,#334452),(#334453,
#334454,#334455),(#334456,#334457,#334458),(#334459,#334460,#334461),(#334462,
#334463,#334464),(#334465,#334466,#334467),(#334468,#334469,#334470),(#334471,
#334472,#334473),(#334474,#334475,#334476),(#334477,#334478,#334479),(#334480,
#334481,#334482),(#334483,#334484,#334485),(#334486,#334487,#334488),(#334489,
#334490,#334491),(#334492,#334493,#334494),(#334495,#334496,#334497),(#334498,
#334499,#334500),(#334501,#334502,#334503),(#334504,#334505,#334506),(#334507,
#334508,#334509),(#334510,#334511,#334512),(#334513,#334514,#334515),(#334516,
#334517,#334518),(#334519,#334520,#334521),(#334522,#334523,#334524),(#334525,
#334526,#334527),(#334528,#334529,#334530),(#334531,#334532,#334533),(#334534,
#334535,#334536),(#334537,#334538,#334539),(#334540,#334541,#334542),(#334543,
#334544,#334545),(#334546,#334547,#334548),(#334549,#334550,#334551),(#334552,
#334553,#334554),(#334555,#334556,#334557),(#334558,#334559,#334560),(#334561,
#334562,#334563),(#334564,#334565,#334566),(#334567,#334568,#334569),(#334570,
#334571,#334572),(#334573,#334574,#334575),(#334576,#334577,#334578),(#334579,
#334580,#334581),(#334582,#334583,#334584),(#334585,#334586,#334587),(#334588,
#334589,#334590),(#334591,#334592,#334593),(#334594,#334595,#334596),(#334597,
#334598,#334599),(#334600,#334601,#334602),(#334603,#334604,#334605),(#334606,
#334607,#334608),(#334609,#334610,#334611),(#334612,#334613,#334614),(#334615,
#334616,#334617),(#334618,#334619,#334620),(#334621,#334622,#334623),(#334624,
#334625,#334626),(#334627,#334628,#334629),(#334630,#334631,#334632),(#334633,
#334634,#334635),(#334636,#334637,#334638),(#334639,#334640,#334641),(#334642,
#334643,#334644),(#334645,#334646,#334647),(#334648,#334649,#334650),(#334651,
#334652,#334653),(#334654,#334655,#334656),(#334657,#334658,#334659),(#334660,
#334661,#334662),(#334663,#334664,#334665),(#334666,#334667,#334668),(#334669,
#334670,#334671),(#334672,#334673,#334674),(#334675,#334676,#334677),(#334678,
#334679,#334680),(#334681,#334682,#334683),(#334684,#334685,#334686),(#334687,
#334688,#334689),(#334690,#334691,#334692),(#334693,#334694,#334695),(#334696,
#334697,#334698),(#334699,#334700,#334701),(#334702,#334703,#334704),(#334705,
#334706,#334707),(#334708,#334709,#334710),(#334711,#334712,#334713),(#334714,
#334715,#334716),(#334717,#334718,#334719),(#334720,#334721,#334722),(#334723,
#334724,#334725),(#334726,#334727,#334728),(#334729,#334730,#334731),(#334732,
#334733,#334734),(#334735,#334736,#334737),(#334738,#334739,#334740),(#334741,
#334742,#334743),(#334744,#334745,#334746),(#334747,#334748,#334749),(#334750,
#334751,#334752),(#334753,#334754,#334755),(#334756,#334757,#334758),(#334759,
#334760,#334761),(#334762,#334763,#334764),(#334765,#334766,#334767),(#334768,
#334769,#334770),(#334771,#334772,#334773),(#334774,#334775,#334776),(#334777,
#334778,#334779),(#334780,#334781,#334782),(#334783,#334784,#334785),(#334786,
#334787,#334788),(#334789,#334790,#334791),(#334792,#334793,#334794),(#334795,
#334796,#334797),(#334798,#334799,#334800),(#334801,#334802,#334803),(#334804,
#334805,#334806),(#334807,#334808,#334809),(#334810,#334811,#334812),(#334813,
#334814,#334815),(#334816,#334817,#334818),(#334819,#334820,#334821),(#334822,
#334823,#334824),(#334825,#334826,#334827),(#334828,#334829,#334830),(#334831,
#334832,#334833),(#334834,#334835,#334836),(#334837,#334838,#334839),(#334840,
#334841,#334842),(#334843,#334844,#334845),(#334846,#334847,#334848),(#334849,
#334850,#334851),(#334852,#334853,#334854),(#334855,#334856,#334857),(#334858,
#334859,#334860),(#334861,#334862,#334863),(#334864,#334865,#334866),(#334867,
#334868,#334869),(#334870,#334871,#334872),(#334873,#334874,#334875),(#334876,
#334877,#334878),(#334879,#334880,#334881),(#334882,#334883,#334884),(#334885,
#334886,#334887),(#334888,#334889,#334890),(#334891,#334892,#334893),(#334894,
#334895,#334896),(#334897,#334898,#334899),(#334900,#334901,#334902),(#334903,
#334904,#334905),(#334906,#334907,#334908),(#334909,#334910,#334911),(#334912,
#334913,#334914),(#334915,#334916,#334917),(#334918,#334919,#334920),(#334921,
#334922,#334923),(#334924,#334925,#334926),(#334927,#334928,#334929),(#334930,
#334931,#334932),(#334933,#334934,#334935),(#334936,#334937,#334938),(#334939,
#334940,#334941),(#334942,#334943,#334944),(#334945,#334946,#334947),(#334948,
#334949,#334950),(#334951,#334952,#334953),(#334954,#334955,#334956),(#334957,
#334958,#334959)),.UNSPECIFIED.,.F.,.F.,.F.,(6,1,1,1,1,1,1,1,1,1,1,1,1,
1,1,1,1,1,1,1,1,1,1,1,1,1,1,1,1,1,1,1,1,1,1,1,1,1,1,1,1,1,1,1,1,1,1,1,1,
1,1,1,1,1,1,1,1,1,1,1,1,1,1,1,1,1,1,1,1,1,1,1,1,1,1,1,1,1,1,1,1,1,1,1,1,
1,1,1,1,1,1,1,1,1,1,1,1,1,1,1,1,1,1,1,1,1,1,1,1,1,1,1,1,1,1,1,1,1,1,1,1,
1,1,1,1,1,1,1,1,1,1,1,1,1,1,1,1,1,1,1,1,1,1,1,1,1,1,1,1,1,1,1,1,1,1,1,1,
1,1,1,1,1,1,1,1,1,1,1,1,1,1,1,1,1,1,1,1,1,1,1,1,1,1,1,1,1,1,1,1,1,1,1,1,
1,1,1,1,1,1,1,1,1,1,1,1,1,1,1,1,1,1,1,1,1,1,1,1,1,1,1,1,1,1,1,1,1,1,1,1,
1,1,1,1,1,1,1,1,1,1,1,1,1,1,1,1,1,1,1,1,1,1,1,1,1,1,1,1,1,1,1,1,1,1,1,1,
1,1,1,1,1,1,1,1,1,1,1,1,1,1,1,1,1,1,1,1,1,1,1,1,1,1,1,1,1,1,1,1,1,1,1,1,
1,1,1,1,1,1,1,1,1,1,1,1,1,1,1,1,1,1,1,1,1,1,1,1,1,1,1,1,1,1,1,1,1,1,1,1,
1,1,1,1,1,1,1,1,1,1,1,1,1,1,1,1,1,1,1,1,1,1,1,1,1,1,1,1,1,1,1,1,1,1,1,1,
1,1,1,1,1,1,1,1,1,1,1,1,1,1,1,1,1,1,1,1,1,1,1,1,1,1,1,1,1,1,1,1,1,1,1,1,
1,1,1,1,1,1,1,1,1,1,1,1,1,1,1,1,1,1,1,1,1,1,1,1,1,1,1,1,1,1,1,1,1,1,1,1,
1,1,1,1,1,1,1,1,1,1,1,1,1,1,1,1,1,1,1,1,1,1,1,1,1,1,1,1,1,1,1,1,1,1,1,1,
1,1,1,1,1,1,1,1,1,1,1,1,1,1,1,1,1,1,1,1,1,1,1,1,1,1,1,1,1,1,1,1,1,1,1,1,
1,1,1,1,1,1,1,1,1,1,1,1,1,1,1,1,1,1,1,1,1,1,1,1,1,1,1,1,1,6),(2,1,2),(-0.001964137,
0.,0.001834862,0.003669725,0.005504587,0.00733945,0.009174312,0.011009174,
0.012844037,0.014678899,0.016513761,0.018348624,0.020183486,0.022018349,
0.023853211,0.025688073,0.027522936,0.029357798,0.031192661,0.033027523,
0.034862385,0.036697248,0.03853211,0.040366972,0.042201835,0.044036697,
0.04587156,0.047706422,0.049541284,0.051376147,0.053211009,0.055045872,
0.056880734,0.058715596,0.060550459,0.062385321,0.064220183,0.066055046,
0.067889908,0.069724771,0.071559633,0.073394495,0.075229358,0.07706422,
0.078899083,0.080733945,0.082568807,0.08440367,0.086238532,0.088073394,
0.089908257,0.091743119,0.093577982,0.095412844,0.097247706,0.099082569,
0.100917431,0.102752294,0.104587156,0.106422018,0.108256881,0.110091743,
0.111926606,0.113761468,0.11559633,0.117431193,0.119266055,0.121100917,
0.12293578,0.124770642,0.126605505,0.128440367,0.130275229,0.132110092,
0.133944954,0.135779817,0.137614679,0.139449541,0.141284404,0.143119266,
0.144954128,0.146788991,0.148623853,0.150458716,0.152293578,0.15412844,
0.155963303,0.157798165,0.159633028,0.16146789,0.163302752,0.165137615,
0.166972477,0.168807339,0.170642202,0.172477064,0.174311927,0.176146789,
0.177981651,0.179816514,0.181651376,0.183486239,0.185321101,0.187155963,
0.188990826,0.190825688,0.19266055,0.194495413,0.196330275,0.198165138,
0.2,0.201834862,0.203669725,0.205504587,0.20733945,0.209174312,0.211009174,
0.212844037,0.214678899,0.216513761,0.218348624,0.220183486,0.222018349,
0.223853211,0.225688073,0.227522936,0.229357798,0.231192661,0.233027523,
0.234862385,0.236697248,0.23853211,0.240366972,0.242201835,0.244036697,
0.24587156,0.247706422,0.249541284,0.251376147,0.253211009,0.255045872,
0.256880734,0.258715596,0.260550459,0.262385321,0.264220183,0.266055046,
0.267889908,0.269724771,0.271559633,0.273394495,0.275229358,0.27706422,
0.278899083,0.280733945,0.282568807,0.28440367,0.286238532,0.288073394,
0.289908257,0.291743119,0.293577982,0.295412844,0.297247706,0.299082569,
0.300917431,0.302752294,0.304587156,0.306422018,0.308256881,0.310091743,
0.311926606,0.313761468,0.31559633,0.317431193,0.319266055,0.321100917,
0.32293578,0.324770642,0.326605505,0.328440367,0.330275229,0.332110092,
0.333944954,0.335779817,0.337614679,0.339449541,0.341284404,0.343119266,
0.344954128,0.346788991,0.348623853,0.350458716,0.352293578,0.35412844,
0.355963303,0.357798165,0.359633028,0.36146789,0.363302752,0.365137615,
0.366972477,0.368807339,0.370642202,0.372477064,0.374311927,0.376146789,
0.377981651,0.379816514,0.381651376,0.383486239,0.385321101,0.387155963,
0.388990826,0.390825688,0.39266055,0.394495413,0.396330275,0.398165138,
0.4,0.401834862,0.403669725,0.405504587,0.40733945,0.409174312,0.411009174,
0.412844037,0.414678899,0.416513761,0.418348624,0.420183486,0.422018349,
0.423853211,0.425688073,0.427522936,0.429357798,0.431192661,0.433027523,
0.434862385,0.436697248,0.43853211,0.440366972,0.442201835,0.444036697,
0.44587156,0.447706422,0.449541284,0.451376147,0.453211009,0.455045872,
0.456880734,0.458715596,0.460550459,0.462385321,0.464220183,0.466055046,
0.467889908,0.469724771,0.471559633,0.473394495,0.475229358,0.47706422,
0.478899083,0.480733945,0.482568807,0.48440367,0.486238532,0.488073394,
0.489908257,0.491743119,0.493577982,0.495412844,0.497247706,0.499082569,
0.500917431,0.502752294,0.504587156,0.506422018,0.508256881,0.510091743,
0.511926606,0.513761468,0.51559633,0.517431193,0.519266055,0.521100917,
0.52293578,0.524770642,0.526605505,0.528440367,0.530275229,0.532110092,
0.533944954,0.535779817,0.537614679,0.539449541,0.541284404,0.543119266,
0.544954128,0.546788991,0.548623853,0.550458716,0.552293578,0.55412844,
0.555963303,0.557798165,0.559633028,0.56146789,0.563302752,0.565137615,
0.566972477,0.568807339,0.570642202,0.572477064,0.574311927,0.576146789,
0.577981651,0.579816514,0.581651376,0.583486239,0.585321101,0.587155963,
0.588990826,0.590825688,0.59266055,0.594495413,0.596330275,0.598165138,
0.6,0.601834862,0.603669725,0.605504587,0.60733945,0.609174312,0.611009174,
0.612844037,0.614678899,0.616513761,0.618348624,0.620183486,0.622018349,
0.623853211,0.625688073,0.627522936,0.629357798,0.631192661,0.633027523,
0.634862385,0.636697248,0.63853211,0.640366972,0.642201835,0.644036697,
0.64587156,0.647706422,0.649541284,0.651376147,0.653211009,0.655045872,
0.656880734,0.658715596,0.660550459,0.662385321,0.664220183,0.666055046,
0.667889908,0.669724771,0.671559633,0.673394495,0.675229358,0.67706422,
0.678899083,0.680733945,0.682568807,0.68440367,0.686238532,0.688073394,
0.689908257,0.691743119,0.693577982,0.695412844,0.697247706,0.699082569,
0.700917431,0.702752294,0.704587156,0.706422018,0.708256881,0.710091743,
0.711926606,0.713761468,0.71559633,0.717431193,0.719266055,0.721100917,
0.72293578,0.724770642,0.726605505,0.728440367,0.730275229,0.732110092,
0.733944954,0.735779817,0.737614679,0.739449541,0.741284404,0.743119266,
0.744954128,0.746788991,0.748623853,0.750458716,0.752293578,0.75412844,
0.755963303,0.757798165,0.759633028,0.76146789,0.763302752,0.765137615,
0.766972477,0.768807339,0.770642202,0.772477064,0.774311927,0.776146789,
0.777981651,0.779816514,0.781651376,0.783486239,0.785321101,0.787155963,
0.788990826,0.790825688,0.79266055,0.794495413,0.796330275,0.798165138,
0.8,0.801834862,0.803669725,0.805504587,0.80733945,0.809174312,0.811009174,
0.812844037,0.814678899,0.816513761,0.818348624,0.820183486,0.822018349,
0.823853211,0.825688073,0.827522936,0.829357798,0.831192661,0.833027523,
0.834862385,0.836697248,0.83853211,0.840366972,0.842201835,0.844036697,
0.84587156,0.847706422,0.849541284,0.851376147,0.853211009,0.855045872,
0.856880734,0.858715596,0.860550459,0.862385321,0.864220183,0.866055046,
0.867889908,0.869724771,0.871559633,0.873394495,0.875229358,0.87706422,
0.878899083,0.880733945,0.882568807,0.88440367,0.886238532,0.888073394,
0.889908257,0.891743119,0.893577982,0.895412844,0.897247706,0.899082569,
0.900917431,0.902752294,0.904587156,0.906422018,0.908256881,0.910091743,
0.911926606,0.913761468,0.91559633,0.917431193,0.919266055,0.921100917,
0.92293578,0.924770642,0.926605505,0.928440367,0.930275229,0.932110092,
0.933944954,0.935779817,0.937614679,0.939449541,0.941284404,0.943119266,
0.944954128,0.946788991,0.948623853,0.950458716,0.952293578,0.95412844,
0.955963303,0.957798165,0.959633028,0.96146789,0.963302752,0.965137615,
0.966972477,0.968807339,0.970642202,0.972477064,0.974311927,0.976146789,
0.977981651,0.979816514,0.981651376,0.983486239,0.985321101,0.987155963,
0.988990826,0.990825688,0.99266055,0.994495413,0.996330275,0.998165138,
1.),(0.3,1.,1.3),.UNSPECIFIED.);
#6323=B_SPLINE_SURFACE_WITH_KNOTS('',5,1,((#334970,#334971,#334972),(#334973,
#334974,#334975),(#334976,#334977,#334978),(#334979,#334980,#334981),(#334982,
#334983,#334984),(#334985,#334986,#334987),(#334988,#334989,#334990),(#334991,
#334992,#334993),(#334994,#334995,#334996),(#334997,#334998,#334999),(#335000,
#335001,#335002),(#335003,#335004,#335005),(#335006,#335007,#335008),(#335009,
#335010,#335011),(#335012,#335013,#335014),(#335015,#335016,#335017),(#335018,
#335019,#335020),(#335021,#335022,#335023),(#335024,#335025,#335026),(#335027,
#335028,#335029),(#335030,#335031,#335032),(#335033,#335034,#335035),(#335036,
#335037,#335038),(#335039,#335040,#335041),(#335042,#335043,#335044),(#335045,
#335046,#335047),(#335048,#335049,#335050),(#335051,#335052,#335053),(#335054,
#335055,#335056),(#335057,#335058,#335059),(#335060,#335061,#335062),(#335063,
#335064,#335065),(#335066,#335067,#335068),(#335069,#335070,#335071),(#335072,
#335073,#335074),(#335075,#335076,#335077),(#335078,#335079,#335080),(#335081,
#335082,#335083),(#335084,#335085,#335086),(#335087,#335088,#335089),(#335090,
#335091,#335092),(#335093,#335094,#335095),(#335096,#335097,#335098),(#335099,
#335100,#335101),(#335102,#335103,#335104),(#335105,#335106,#335107),(#335108,
#335109,#335110),(#335111,#335112,#335113),(#335114,#335115,#335116),(#335117,
#335118,#335119),(#335120,#335121,#335122),(#335123,#335124,#335125),(#335126,
#335127,#335128),(#335129,#335130,#335131),(#335132,#335133,#335134),(#335135,
#335136,#335137),(#335138,#335139,#335140),(#335141,#335142,#335143),(#335144,
#335145,#335146),(#335147,#335148,#335149),(#335150,#335151,#335152),(#335153,
#335154,#335155),(#335156,#335157,#335158),(#335159,#335160,#335161),(#335162,
#335163,#335164),(#335165,#335166,#335167),(#335168,#335169,#335170),(#335171,
#335172,#335173),(#335174,#335175,#335176),(#335177,#335178,#335179),(#335180,
#335181,#335182),(#335183,#335184,#335185),(#335186,#335187,#335188),(#335189,
#335190,#335191),(#335192,#335193,#335194),(#335195,#335196,#335197),(#335198,
#335199,#335200),(#335201,#335202,#335203),(#335204,#335205,#335206),(#335207,
#335208,#335209),(#335210,#335211,#335212),(#335213,#335214,#335215),(#335216,
#335217,#335218),(#335219,#335220,#335221),(#335222,#335223,#335224),(#335225,
#335226,#335227),(#335228,#335229,#335230),(#335231,#335232,#335233),(#335234,
#335235,#335236),(#335237,#335238,#335239),(#335240,#335241,#335242),(#335243,
#335244,#335245),(#335246,#335247,#335248),(#335249,#335250,#335251),(#335252,
#335253,#335254),(#335255,#335256,#335257),(#335258,#335259,#335260),(#335261,
#335262,#335263),(#335264,#335265,#335266),(#335267,#335268,#335269),(#335270,
#335271,#335272),(#335273,#335274,#335275),(#335276,#335277,#335278),(#335279,
#335280,#335281),(#335282,#335283,#335284),(#335285,#335286,#335287),(#335288,
#335289,#335290),(#335291,#335292,#335293),(#335294,#335295,#335296),(#335297,
#335298,#335299),(#335300,#335301,#335302),(#335303,#335304,#335305),(#335306,
#335307,#335308),(#335309,#335310,#335311),(#335312,#335313,#335314),(#335315,
#335316,#335317),(#335318,#335319,#335320),(#335321,#335322,#335323),(#335324,
#335325,#335326),(#335327,#335328,#335329),(#335330,#335331,#335332),(#335333,
#335334,#335335),(#335336,#335337,#335338),(#335339,#335340,#335341),(#335342,
#335343,#335344),(#335345,#335346,#335347),(#335348,#335349,#335350),(#335351,
#335352,#335353),(#335354,#335355,#335356),(#335357,#335358,#335359),(#335360,
#335361,#335362),(#335363,#335364,#335365),(#335366,#335367,#335368),(#335369,
#335370,#335371),(#335372,#335373,#335374),(#335375,#335376,#335377),(#335378,
#335379,#335380),(#335381,#335382,#335383),(#335384,#335385,#335386),(#335387,
#335388,#335389),(#335390,#335391,#335392),(#335393,#335394,#335395),(#335396,
#335397,#335398),(#335399,#335400,#335401),(#335402,#335403,#335404),(#335405,
#335406,#335407),(#335408,#335409,#335410),(#335411,#335412,#335413),(#335414,
#335415,#335416),(#335417,#335418,#335419),(#335420,#335421,#335422),(#335423,
#335424,#335425),(#335426,#335427,#335428),(#335429,#335430,#335431),(#335432,
#335433,#335434),(#335435,#335436,#335437),(#335438,#335439,#335440),(#335441,
#335442,#335443),(#335444,#335445,#335446),(#335447,#335448,#335449),(#335450,
#335451,#335452),(#335453,#335454,#335455),(#335456,#335457,#335458),(#335459,
#335460,#335461),(#335462,#335463,#335464),(#335465,#335466,#335467),(#335468,
#335469,#335470),(#335471,#335472,#335473),(#335474,#335475,#335476),(#335477,
#335478,#335479),(#335480,#335481,#335482),(#335483,#335484,#335485),(#335486,
#335487,#335488),(#335489,#335490,#335491),(#335492,#335493,#335494),(#335495,
#335496,#335497),(#335498,#335499,#335500),(#335501,#335502,#335503),(#335504,
#335505,#335506),(#335507,#335508,#335509),(#335510,#335511,#335512),(#335513,
#335514,#335515),(#335516,#335517,#335518),(#335519,#335520,#335521),(#335522,
#335523,#335524),(#335525,#335526,#335527),(#335528,#335529,#335530),(#335531,
#335532,#335533),(#335534,#335535,#335536),(#335537,#335538,#335539),(#335540,
#335541,#335542),(#335543,#335544,#335545),(#335546,#335547,#335548),(#335549,
#335550,#335551),(#335552,#335553,#335554),(#335555,#335556,#335557),(#335558,
#335559,#335560),(#335561,#335562,#335563),(#335564,#335565,#335566),(#335567,
#335568,#335569),(#335570,#335571,#335572),(#335573,#335574,#335575),(#335576,
#335577,#335578),(#335579,#335580,#335581),(#335582,#335583,#335584),(#335585,
#335586,#335587),(#335588,#335589,#335590),(#335591,#335592,#335593),(#335594,
#335595,#335596),(#335597,#335598,#335599),(#335600,#335601,#335602),(#335603,
#335604,#335605),(#335606,#335607,#335608),(#335609,#335610,#335611),(#335612,
#335613,#335614),(#335615,#335616,#335617),(#335618,#335619,#335620),(#335621,
#335622,#335623),(#335624,#335625,#335626),(#335627,#335628,#335629),(#335630,
#335631,#335632),(#335633,#335634,#335635),(#335636,#335637,#335638),(#335639,
#335640,#335641),(#335642,#335643,#335644),(#335645,#335646,#335647),(#335648,
#335649,#335650),(#335651,#335652,#335653),(#335654,#335655,#335656),(#335657,
#335658,#335659),(#335660,#335661,#335662),(#335663,#335664,#335665),(#335666,
#335667,#335668),(#335669,#335670,#335671),(#335672,#335673,#335674),(#335675,
#335676,#335677),(#335678,#335679,#335680),(#335681,#335682,#335683),(#335684,
#335685,#335686),(#335687,#335688,#335689),(#335690,#335691,#335692),(#335693,
#335694,#335695),(#335696,#335697,#335698),(#335699,#335700,#335701),(#335702,
#335703,#335704),(#335705,#335706,#335707),(#335708,#335709,#335710),(#335711,
#335712,#335713),(#335714,#335715,#335716),(#335717,#335718,#335719),(#335720,
#335721,#335722),(#335723,#335724,#335725),(#335726,#335727,#335728),(#335729,
#335730,#335731),(#335732,#335733,#335734),(#335735,#335736,#335737),(#335738,
#335739,#335740),(#335741,#335742,#335743),(#335744,#335745,#335746),(#335747,
#335748,#335749),(#335750,#335751,#335752),(#335753,#335754,#335755),(#335756,
#335757,#335758),(#335759,#335760,#335761),(#335762,#335763,#335764),(#335765,
#335766,#335767),(#335768,#335769,#335770),(#335771,#335772,#335773),(#335774,
#335775,#335776),(#335777,#335778,#335779),(#335780,#335781,#335782),(#335783,
#335784,#335785),(#335786,#335787,#335788),(#335789,#335790,#335791),(#335792,
#335793,#335794),(#335795,#335796,#335797),(#335798,#335799,#335800),(#335801,
#335802,#335803),(#335804,#335805,#335806),(#335807,#335808,#335809),(#335810,
#335811,#335812),(#335813,#335814,#335815),(#335816,#335817,#335818),(#335819,
#335820,#335821),(#335822,#335823,#335824),(#335825,#335826,#335827),(#335828,
#335829,#335830),(#335831,#335832,#335833),(#335834,#335835,#335836),(#335837,
#335838,#335839),(#335840,#335841,#335842),(#335843,#335844,#335845),(#335846,
#335847,#335848),(#335849,#335850,#335851),(#335852,#335853,#335854),(#335855,
#335856,#335857),(#335858,#335859,#335860),(#335861,#335862,#335863),(#335864,
#335865,#335866),(#335867,#335868,#335869),(#335870,#335871,#335872),(#335873,
#335874,#335875),(#335876,#335877,#335878),(#335879,#335880,#335881),(#335882,
#335883,#335884),(#335885,#335886,#335887),(#335888,#335889,#335890),(#335891,
#335892,#335893),(#335894,#335895,#335896),(#335897,#335898,#335899),(#335900,
#335901,#335902),(#335903,#335904,#335905),(#335906,#335907,#335908),(#335909,
#335910,#335911),(#335912,#335913,#335914),(#335915,#335916,#335917),(#335918,
#335919,#335920),(#335921,#335922,#335923),(#335924,#335925,#335926),(#335927,
#335928,#335929),(#335930,#335931,#335932),(#335933,#335934,#335935),(#335936,
#335937,#335938),(#335939,#335940,#335941),(#335942,#335943,#335944),(#335945,
#335946,#335947),(#335948,#335949,#335950),(#335951,#335952,#335953),(#335954,
#335955,#335956),(#335957,#335958,#335959),(#335960,#335961,#335962),(#335963,
#335964,#335965),(#335966,#335967,#335968),(#335969,#335970,#335971),(#335972,
#335973,#335974),(#335975,#335976,#335977),(#335978,#335979,#335980),(#335981,
#335982,#335983),(#335984,#335985,#335986),(#335987,#335988,#335989),(#335990,
#335991,#335992),(#335993,#335994,#335995),(#335996,#335997,#335998),(#335999,
#336000,#336001),(#336002,#336003,#336004),(#336005,#336006,#336007),(#336008,
#336009,#336010),(#336011,#336012,#336013),(#336014,#336015,#336016),(#336017,
#336018,#336019),(#336020,#336021,#336022),(#336023,#336024,#336025),(#336026,
#336027,#336028),(#336029,#336030,#336031),(#336032,#336033,#336034),(#336035,
#336036,#336037),(#336038,#336039,#336040),(#336041,#336042,#336043),(#336044,
#336045,#336046),(#336047,#336048,#336049),(#336050,#336051,#336052),(#336053,
#336054,#336055),(#336056,#336057,#336058),(#336059,#336060,#336061),(#336062,
#336063,#336064),(#336065,#336066,#336067),(#336068,#336069,#336070),(#336071,
#336072,#336073),(#336074,#336075,#336076),(#336077,#336078,#336079),(#336080,
#336081,#336082),(#336083,#336084,#336085),(#336086,#336087,#336088),(#336089,
#336090,#336091),(#336092,#336093,#336094),(#336095,#336096,#336097),(#336098,
#336099,#336100),(#336101,#336102,#336103),(#336104,#336105,#336106),(#336107,
#336108,#336109),(#336110,#336111,#336112),(#336113,#336114,#336115),(#336116,
#336117,#336118),(#336119,#336120,#336121),(#336122,#336123,#336124),(#336125,
#336126,#336127),(#336128,#336129,#336130),(#336131,#336132,#336133),(#336134,
#336135,#336136),(#336137,#336138,#336139),(#336140,#336141,#336142),(#336143,
#336144,#336145),(#336146,#336147,#336148),(#336149,#336150,#336151),(#336152,
#336153,#336154),(#336155,#336156,#336157),(#336158,#336159,#336160),(#336161,
#336162,#336163),(#336164,#336165,#336166),(#336167,#336168,#336169),(#336170,
#336171,#336172),(#336173,#336174,#336175),(#336176,#336177,#336178),(#336179,
#336180,#336181),(#336182,#336183,#336184),(#336185,#336186,#336187),(#336188,
#336189,#336190),(#336191,#336192,#336193),(#336194,#336195,#336196),(#336197,
#336198,#336199),(#336200,#336201,#336202),(#336203,#336204,#336205),(#336206,
#336207,#336208),(#336209,#336210,#336211),(#336212,#336213,#336214),(#336215,
#336216,#336217),(#336218,#336219,#336220),(#336221,#336222,#336223),(#336224,
#336225,#336226),(#336227,#336228,#336229),(#336230,#336231,#336232),(#336233,
#336234,#336235),(#336236,#336237,#336238),(#336239,#336240,#336241),(#336242,
#336243,#336244),(#336245,#336246,#336247),(#336248,#336249,#336250),(#336251,
#336252,#336253),(#336254,#336255,#336256),(#336257,#336258,#336259),(#336260,
#336261,#336262),(#336263,#336264,#336265),(#336266,#336267,#336268),(#336269,
#336270,#336271),(#336272,#336273,#336274),(#336275,#336276,#336277),(#336278,
#336279,#336280),(#336281,#336282,#336283),(#336284,#336285,#336286),(#336287,
#336288,#336289),(#336290,#336291,#336292),(#336293,#336294,#336295),(#336296,
#336297,#336298),(#336299,#336300,#336301),(#336302,#336303,#336304),(#336305,
#336306,#336307),(#336308,#336309,#336310),(#336311,#336312,#336313),(#336314,
#336315,#336316),(#336317,#336318,#336319),(#336320,#336321,#336322),(#336323,
#336324,#336325),(#336326,#336327,#336328),(#336329,#336330,#336331),(#336332,
#336333,#336334),(#336335,#336336,#336337),(#336338,#336339,#336340),(#336341,
#336342,#336343),(#336344,#336345,#336346),(#336347,#336348,#336349),(#336350,
#336351,#336352),(#336353,#336354,#336355),(#336356,#336357,#336358),(#336359,
#336360,#336361),(#336362,#336363,#336364),(#336365,#336366,#336367),(#336368,
#336369,#336370),(#336371,#336372,#336373),(#336374,#336375,#336376),(#336377,
#336378,#336379),(#336380,#336381,#336382),(#336383,#336384,#336385),(#336386,
#336387,#336388),(#336389,#336390,#336391),(#336392,#336393,#336394),(#336395,
#336396,#336397),(#336398,#336399,#336400),(#336401,#336402,#336403),(#336404,
#336405,#336406),(#336407,#336408,#336409),(#336410,#336411,#336412),(#336413,
#336414,#336415),(#336416,#336417,#336418),(#336419,#336420,#336421),(#336422,
#336423,#336424),(#336425,#336426,#336427),(#336428,#336429,#336430),(#336431,
#336432,#336433),(#336434,#336435,#336436),(#336437,#336438,#336439),(#336440,
#336441,#336442),(#336443,#336444,#336445),(#336446,#336447,#336448),(#336449,
#336450,#336451),(#336452,#336453,#336454),(#336455,#336456,#336457),(#336458,
#336459,#336460),(#336461,#336462,#336463),(#336464,#336465,#336466),(#336467,
#336468,#336469),(#336470,#336471,#336472),(#336473,#336474,#336475),(#336476,
#336477,#336478),(#336479,#336480,#336481),(#336482,#336483,#336484),(#336485,
#336486,#336487),(#336488,#336489,#336490),(#336491,#336492,#336493),(#336494,
#336495,#336496),(#336497,#336498,#336499),(#336500,#336501,#336502),(#336503,
#336504,#336505),(#336506,#336507,#336508),(#336509,#336510,#336511),(#336512,
#336513,#336514),(#336515,#336516,#336517),(#336518,#336519,#336520),(#336521,
#336522,#336523),(#336524,#336525,#336526),(#336527,#336528,#336529),(#336530,
#336531,#336532),(#336533,#336534,#336535),(#336536,#336537,#336538),(#336539,
#336540,#336541),(#336542,#336543,#336544),(#336545,#336546,#336547),(#336548,
#336549,#336550),(#336551,#336552,#336553),(#336554,#336555,#336556),(#336557,
#336558,#336559),(#336560,#336561,#336562),(#336563,#336564,#336565),(#336566,
#336567,#336568),(#336569,#336570,#336571),(#336572,#336573,#336574),(#336575,
#336576,#336577),(#336578,#336579,#336580),(#336581,#336582,#336583),(#336584,
#336585,#336586),(#336587,#336588,#336589),(#336590,#336591,#336592),(#336593,
#336594,#336595),(#336596,#336597,#336598),(#336599,#336600,#336601),(#336602,
#336603,#336604),(#336605,#336606,#336607),(#336608,#336609,#336610),(#336611,
#336612,#336613),(#336614,#336615,#336616),(#336617,#336618,#336619)),
 .UNSPECIFIED.,.F.,.F.,.F.,(6,1,1,1,1,1,1,1,1,1,1,1,1,1,1,1,1,1,1,1,1,1,
1,1,1,1,1,1,1,1,1,1,1,1,1,1,1,1,1,1,1,1,1,1,1,1,1,1,1,1,1,1,1,1,1,1,1,1,
1,1,1,1,1,1,1,1,1,1,1,1,1,1,1,1,1,1,1,1,1,1,1,1,1,1,1,1,1,1,1,1,1,1,1,1,
1,1,1,1,1,1,1,1,1,1,1,1,1,1,1,1,1,1,1,1,1,1,1,1,1,1,1,1,1,1,1,1,1,1,1,1,
1,1,1,1,1,1,1,1,1,1,1,1,1,1,1,1,1,1,1,1,1,1,1,1,1,1,1,1,1,1,1,1,1,1,1,1,
1,1,1,1,1,1,1,1,1,1,1,1,1,1,1,1,1,1,1,1,1,1,1,1,1,1,1,1,1,1,1,1,1,1,1,1,
1,1,1,1,1,1,1,1,1,1,1,1,1,1,1,1,1,1,1,1,1,1,1,1,1,1,1,1,1,1,1,1,1,1,1,1,
1,1,1,1,1,1,1,1,1,1,1,1,1,1,1,1,1,1,1,1,1,1,1,1,1,1,1,1,1,1,1,1,1,1,1,1,
1,1,1,1,1,1,1,1,1,1,1,1,1,1,1,1,1,1,1,1,1,1,1,1,1,1,1,1,1,1,1,1,1,1,1,1,
1,1,1,1,1,1,1,1,1,1,1,1,1,1,1,1,1,1,1,1,1,1,1,1,1,1,1,1,1,1,1,1,1,1,1,1,
1,1,1,1,1,1,1,1,1,1,1,1,1,1,1,1,1,1,1,1,1,1,1,1,1,1,1,1,1,1,1,1,1,1,1,1,
1,1,1,1,1,1,1,1,1,1,1,1,1,1,1,1,1,1,1,1,1,1,1,1,1,1,1,1,1,1,1,1,1,1,1,1,
1,1,1,1,1,1,1,1,1,1,1,1,1,1,1,1,1,1,1,1,1,1,1,1,1,1,1,1,1,1,1,1,1,1,1,1,
1,1,1,1,1,1,1,1,1,1,1,1,1,1,1,1,1,1,1,1,1,1,1,1,1,1,1,1,1,1,1,1,1,1,1,1,
1,1,1,1,1,1,1,1,1,1,1,1,1,1,1,1,1,1,1,1,1,1,1,1,1,1,1,1,1,1,1,1,1,1,1,1,
1,1,1,1,1,1,1,1,1,1,1,1,1,1,1,1,1,1,1,6),(2,1,2),(-1.,-0.998165138,-0.996330275,
-0.994495413,-0.99266055,-0.990825688,-0.988990826,-0.987155963,-0.985321101,
-0.983486239,-0.981651376,-0.979816514,-0.977981651,-0.976146789,-0.974311927,
-0.972477064,-0.970642202,-0.968807339,-0.966972477,-0.965137615,-0.963302752,
-0.96146789,-0.959633028,-0.957798165,-0.955963303,-0.95412844,-0.952293578,
-0.950458716,-0.948623853,-0.946788991,-0.944954128,-0.943119266,-0.941284404,
-0.939449541,-0.937614679,-0.935779817,-0.933944954,-0.932110092,-0.930275229,
-0.928440367,-0.926605505,-0.924770642,-0.92293578,-0.921100917,-0.919266055,
-0.917431193,-0.91559633,-0.913761468,-0.911926606,-0.910091743,-0.908256881,
-0.906422018,-0.904587156,-0.902752294,-0.900917431,-0.899082569,-0.897247706,
-0.895412844,-0.893577982,-0.891743119,-0.889908257,-0.888073394,-0.886238532,
-0.88440367,-0.882568807,-0.880733945,-0.878899083,-0.87706422,-0.875229358,
-0.873394495,-0.871559633,-0.869724771,-0.867889908,-0.866055046,-0.864220183,
-0.862385321,-0.860550459,-0.858715596,-0.856880734,-0.855045872,-0.853211009,
-0.851376147,-0.849541284,-0.847706422,-0.84587156,-0.844036697,-0.842201835,
-0.840366972,-0.83853211,-0.836697248,-0.834862385,-0.833027523,-0.831192661,
-0.829357798,-0.827522936,-0.825688073,-0.823853211,-0.822018349,-0.820183486,
-0.818348624,-0.816513761,-0.814678899,-0.812844037,-0.811009174,-0.809174312,
-0.80733945,-0.805504587,-0.803669725,-0.801834862,-0.8,-0.798165138,-0.796330275,
-0.794495413,-0.79266055,-0.790825688,-0.788990826,-0.787155963,-0.785321101,
-0.783486239,-0.781651376,-0.779816514,-0.777981651,-0.776146789,-0.774311927,
-0.772477064,-0.770642202,-0.768807339,-0.766972477,-0.765137615,-0.763302752,
-0.76146789,-0.759633028,-0.757798165,-0.755963303,-0.75412844,-0.752293578,
-0.750458716,-0.748623853,-0.746788991,-0.744954128,-0.743119266,-0.741284404,
-0.739449541,-0.737614679,-0.735779817,-0.733944954,-0.732110092,-0.730275229,
-0.728440367,-0.726605505,-0.724770642,-0.72293578,-0.721100917,-0.719266055,
-0.717431193,-0.71559633,-0.713761468,-0.711926606,-0.710091743,-0.708256881,
-0.706422018,-0.704587156,-0.702752294,-0.700917431,-0.699082569,-0.697247706,
-0.695412844,-0.693577982,-0.691743119,-0.689908257,-0.688073394,-0.686238532,
-0.68440367,-0.682568807,-0.680733945,-0.678899083,-0.67706422,-0.675229358,
-0.673394495,-0.671559633,-0.669724771,-0.667889908,-0.666055046,-0.664220183,
-0.662385321,-0.660550459,-0.658715596,-0.656880734,-0.655045872,-0.653211009,
-0.651376147,-0.649541284,-0.647706422,-0.64587156,-0.644036697,-0.642201835,
-0.640366972,-0.63853211,-0.636697248,-0.634862385,-0.633027523,-0.631192661,
-0.629357798,-0.627522936,-0.625688073,-0.623853211,-0.622018349,-0.620183486,
-0.618348624,-0.616513761,-0.614678899,-0.612844037,-0.611009174,-0.609174312,
-0.60733945,-0.605504587,-0.603669725,-0.601834862,-0.6,-0.598165138,-0.596330275,
-0.594495413,-0.59266055,-0.590825688,-0.588990826,-0.587155963,-0.585321101,
-0.583486239,-0.581651376,-0.579816514,-0.577981651,-0.576146789,-0.574311927,
-0.572477064,-0.570642202,-0.568807339,-0.566972477,-0.565137615,-0.563302752,
-0.56146789,-0.559633028,-0.557798165,-0.555963303,-0.55412844,-0.552293578,
-0.550458716,-0.548623853,-0.546788991,-0.544954128,-0.543119266,-0.541284404,
-0.539449541,-0.537614679,-0.535779817,-0.533944954,-0.532110092,-0.530275229,
-0.528440367,-0.526605505,-0.524770642,-0.52293578,-0.521100917,-0.519266055,
-0.517431193,-0.51559633,-0.513761468,-0.511926606,-0.510091743,-0.508256881,
-0.506422018,-0.504587156,-0.502752294,-0.500917431,-0.499082569,-0.497247706,
-0.495412844,-0.493577982,-0.491743119,-0.489908257,-0.488073394,-0.486238532,
-0.48440367,-0.482568807,-0.480733945,-0.478899083,-0.47706422,-0.475229358,
-0.473394495,-0.471559633,-0.469724771,-0.467889908,-0.466055046,-0.464220183,
-0.462385321,-0.460550459,-0.458715596,-0.456880734,-0.455045872,-0.453211009,
-0.451376147,-0.449541284,-0.447706422,-0.44587156,-0.444036697,-0.442201835,
-0.440366972,-0.43853211,-0.436697248,-0.434862385,-0.433027523,-0.431192661,
-0.429357798,-0.427522936,-0.425688073,-0.423853211,-0.422018349,-0.420183486,
-0.418348624,-0.416513761,-0.414678899,-0.412844037,-0.411009174,-0.409174312,
-0.40733945,-0.405504587,-0.403669725,-0.401834862,-0.4,-0.398165138,-0.396330275,
-0.394495413,-0.39266055,-0.390825688,-0.388990826,-0.387155963,-0.385321101,
-0.383486239,-0.381651376,-0.379816514,-0.377981651,-0.376146789,-0.374311927,
-0.372477064,-0.370642202,-0.368807339,-0.366972477,-0.365137615,-0.363302752,
-0.36146789,-0.359633028,-0.357798165,-0.355963303,-0.35412844,-0.352293578,
-0.350458716,-0.348623853,-0.346788991,-0.344954128,-0.343119266,-0.341284404,
-0.339449541,-0.337614679,-0.335779817,-0.333944954,-0.332110092,-0.330275229,
-0.328440367,-0.326605505,-0.324770642,-0.32293578,-0.321100917,-0.319266055,
-0.317431193,-0.31559633,-0.313761468,-0.311926606,-0.310091743,-0.308256881,
-0.306422018,-0.304587156,-0.302752294,-0.300917431,-0.299082569,-0.297247706,
-0.295412844,-0.293577982,-0.291743119,-0.289908257,-0.288073394,-0.286238532,
-0.28440367,-0.282568807,-0.280733945,-0.278899083,-0.27706422,-0.275229358,
-0.273394495,-0.271559633,-0.269724771,-0.267889908,-0.266055046,-0.264220183,
-0.262385321,-0.260550459,-0.258715596,-0.256880734,-0.255045872,-0.253211009,
-0.251376147,-0.249541284,-0.247706422,-0.24587156,-0.244036697,-0.242201835,
-0.240366972,-0.23853211,-0.236697248,-0.234862385,-0.233027523,-0.231192661,
-0.229357798,-0.227522936,-0.225688073,-0.223853211,-0.222018349,-0.220183486,
-0.218348624,-0.216513761,-0.214678899,-0.212844037,-0.211009174,-0.209174312,
-0.20733945,-0.205504587,-0.203669725,-0.201834862,-0.2,-0.198165138,-0.196330275,
-0.194495413,-0.19266055,-0.190825688,-0.188990826,-0.187155963,-0.185321101,
-0.183486239,-0.181651376,-0.179816514,-0.177981651,-0.176146789,-0.174311927,
-0.172477064,-0.170642202,-0.168807339,-0.166972477,-0.165137615,-0.163302752,
-0.16146789,-0.159633028,-0.157798165,-0.155963303,-0.15412844,-0.152293578,
-0.150458716,-0.148623853,-0.146788991,-0.144954128,-0.143119266,-0.141284404,
-0.139449541,-0.137614679,-0.135779817,-0.133944954,-0.132110092,-0.130275229,
-0.128440367,-0.126605505,-0.124770642,-0.12293578,-0.121100917,-0.119266055,
-0.117431193,-0.11559633,-0.113761468,-0.111926606,-0.110091743,-0.108256881,
-0.106422018,-0.104587156,-0.102752294,-0.100917431,-0.099082569,-0.097247706,
-0.095412844,-0.093577982,-0.091743119,-0.089908257,-0.088073394,-0.086238532,
-0.08440367,-0.082568807,-0.080733945,-0.078899083,-0.07706422,-0.075229358,
-0.073394495,-0.071559633,-0.069724771,-0.067889908,-0.066055046,-0.064220183,
-0.062385321,-0.060550459,-0.058715596,-0.056880734,-0.055045872,-0.053211009,
-0.051376147,-0.049541284,-0.047706422,-0.04587156,-0.044036697,-0.042201835,
-0.040366972,-0.03853211,-0.036697248,-0.034862385,-0.033027523,-0.031192661,
-0.029357798,-0.027522936,-0.025688073,-0.023853211,-0.022018349,-0.020183486,
-0.018348624,-0.016513761,-0.014678899,-0.012844037,-0.011009174,-0.009174312,
-0.00733945,-0.005504587,-0.003669725,-0.001834862,0.000982116),(0.3,1.,
1.3),.UNSPECIFIED.);
#6324=B_SPLINE_SURFACE_WITH_KNOTS('',5,1,((#336623,#336624,#336625),(#336626,
#336627,#336628),(#336629,#336630,#336631),(#336632,#336633,#336634),(#336635,
#336636,#336637),(#336638,#336639,#336640),(#336641,#336642,#336643),(#336644,
#336645,#336646),(#336647,#336648,#336649),(#336650,#336651,#336652),(#336653,
#336654,#336655),(#336656,#336657,#336658),(#336659,#336660,#336661),(#336662,
#336663,#336664),(#336665,#336666,#336667),(#336668,#336669,#336670),(#336671,
#336672,#336673),(#336674,#336675,#336676),(#336677,#336678,#336679),(#336680,
#336681,#336682),(#336683,#336684,#336685),(#336686,#336687,#336688),(#336689,
#336690,#336691),(#336692,#336693,#336694),(#336695,#336696,#336697),(#336698,
#336699,#336700),(#336701,#336702,#336703),(#336704,#336705,#336706),(#336707,
#336708,#336709),(#336710,#336711,#336712),(#336713,#336714,#336715),(#336716,
#336717,#336718),(#336719,#336720,#336721),(#336722,#336723,#336724),(#336725,
#336726,#336727),(#336728,#336729,#336730),(#336731,#336732,#336733),(#336734,
#336735,#336736),(#336737,#336738,#336739),(#336740,#336741,#336742),(#336743,
#336744,#336745),(#336746,#336747,#336748),(#336749,#336750,#336751),(#336752,
#336753,#336754),(#336755,#336756,#336757),(#336758,#336759,#336760),(#336761,
#336762,#336763),(#336764,#336765,#336766),(#336767,#336768,#336769),(#336770,
#336771,#336772),(#336773,#336774,#336775),(#336776,#336777,#336778),(#336779,
#336780,#336781),(#336782,#336783,#336784),(#336785,#336786,#336787),(#336788,
#336789,#336790),(#336791,#336792,#336793),(#336794,#336795,#336796),(#336797,
#336798,#336799),(#336800,#336801,#336802),(#336803,#336804,#336805),(#336806,
#336807,#336808),(#336809,#336810,#336811),(#336812,#336813,#336814),(#336815,
#336816,#336817),(#336818,#336819,#336820),(#336821,#336822,#336823),(#336824,
#336825,#336826),(#336827,#336828,#336829),(#336830,#336831,#336832),(#336833,
#336834,#336835),(#336836,#336837,#336838),(#336839,#336840,#336841),(#336842,
#336843,#336844),(#336845,#336846,#336847),(#336848,#336849,#336850),(#336851,
#336852,#336853),(#336854,#336855,#336856),(#336857,#336858,#336859),(#336860,
#336861,#336862),(#336863,#336864,#336865),(#336866,#336867,#336868),(#336869,
#336870,#336871),(#336872,#336873,#336874),(#336875,#336876,#336877),(#336878,
#336879,#336880),(#336881,#336882,#336883),(#336884,#336885,#336886),(#336887,
#336888,#336889),(#336890,#336891,#336892),(#336893,#336894,#336895),(#336896,
#336897,#336898),(#336899,#336900,#336901),(#336902,#336903,#336904),(#336905,
#336906,#336907),(#336908,#336909,#336910),(#336911,#336912,#336913),(#336914,
#336915,#336916),(#336917,#336918,#336919),(#336920,#336921,#336922),(#336923,
#336924,#336925),(#336926,#336927,#336928),(#336929,#336930,#336931),(#336932,
#336933,#336934),(#336935,#336936,#336937),(#336938,#336939,#336940),(#336941,
#336942,#336943),(#336944,#336945,#336946),(#336947,#336948,#336949),(#336950,
#336951,#336952),(#336953,#336954,#336955),(#336956,#336957,#336958),(#336959,
#336960,#336961),(#336962,#336963,#336964),(#336965,#336966,#336967),(#336968,
#336969,#336970),(#336971,#336972,#336973),(#336974,#336975,#336976),(#336977,
#336978,#336979),(#336980,#336981,#336982),(#336983,#336984,#336985),(#336986,
#336987,#336988),(#336989,#336990,#336991),(#336992,#336993,#336994),(#336995,
#336996,#336997),(#336998,#336999,#337000),(#337001,#337002,#337003),(#337004,
#337005,#337006),(#337007,#337008,#337009),(#337010,#337011,#337012),(#337013,
#337014,#337015),(#337016,#337017,#337018),(#337019,#337020,#337021),(#337022,
#337023,#337024),(#337025,#337026,#337027),(#337028,#337029,#337030),(#337031,
#337032,#337033),(#337034,#337035,#337036),(#337037,#337038,#337039),(#337040,
#337041,#337042),(#337043,#337044,#337045),(#337046,#337047,#337048),(#337049,
#337050,#337051),(#337052,#337053,#337054),(#337055,#337056,#337057),(#337058,
#337059,#337060),(#337061,#337062,#337063),(#337064,#337065,#337066),(#337067,
#337068,#337069),(#337070,#337071,#337072),(#337073,#337074,#337075),(#337076,
#337077,#337078),(#337079,#337080,#337081),(#337082,#337083,#337084),(#337085,
#337086,#337087),(#337088,#337089,#337090),(#337091,#337092,#337093),(#337094,
#337095,#337096),(#337097,#337098,#337099),(#337100,#337101,#337102),(#337103,
#337104,#337105),(#337106,#337107,#337108),(#337109,#337110,#337111),(#337112,
#337113,#337114),(#337115,#337116,#337117),(#337118,#337119,#337120),(#337121,
#337122,#337123),(#337124,#337125,#337126),(#337127,#337128,#337129),(#337130,
#337131,#337132),(#337133,#337134,#337135),(#337136,#337137,#337138),(#337139,
#337140,#337141),(#337142,#337143,#337144),(#337145,#337146,#337147),(#337148,
#337149,#337150),(#337151,#337152,#337153),(#337154,#337155,#337156),(#337157,
#337158,#337159),(#337160,#337161,#337162),(#337163,#337164,#337165),(#337166,
#337167,#337168),(#337169,#337170,#337171),(#337172,#337173,#337174),(#337175,
#337176,#337177),(#337178,#337179,#337180),(#337181,#337182,#337183),(#337184,
#337185,#337186),(#337187,#337188,#337189),(#337190,#337191,#337192),(#337193,
#337194,#337195),(#337196,#337197,#337198),(#337199,#337200,#337201),(#337202,
#337203,#337204),(#337205,#337206,#337207),(#337208,#337209,#337210),(#337211,
#337212,#337213),(#337214,#337215,#337216),(#337217,#337218,#337219),(#337220,
#337221,#337222),(#337223,#337224,#337225),(#337226,#337227,#337228),(#337229,
#337230,#337231),(#337232,#337233,#337234),(#337235,#337236,#337237),(#337238,
#337239,#337240),(#337241,#337242,#337243),(#337244,#337245,#337246),(#337247,
#337248,#337249),(#337250,#337251,#337252),(#337253,#337254,#337255),(#337256,
#337257,#337258),(#337259,#337260,#337261),(#337262,#337263,#337264),(#337265,
#337266,#337267),(#337268,#337269,#337270),(#337271,#337272,#337273),(#337274,
#337275,#337276),(#337277,#337278,#337279),(#337280,#337281,#337282),(#337283,
#337284,#337285),(#337286,#337287,#337288),(#337289,#337290,#337291),(#337292,
#337293,#337294),(#337295,#337296,#337297),(#337298,#337299,#337300),(#337301,
#337302,#337303),(#337304,#337305,#337306),(#337307,#337308,#337309),(#337310,
#337311,#337312),(#337313,#337314,#337315),(#337316,#337317,#337318),(#337319,
#337320,#337321),(#337322,#337323,#337324),(#337325,#337326,#337327),(#337328,
#337329,#337330),(#337331,#337332,#337333),(#337334,#337335,#337336),(#337337,
#337338,#337339),(#337340,#337341,#337342),(#337343,#337344,#337345),(#337346,
#337347,#337348),(#337349,#337350,#337351),(#337352,#337353,#337354),(#337355,
#337356,#337357),(#337358,#337359,#337360),(#337361,#337362,#337363),(#337364,
#337365,#337366),(#337367,#337368,#337369),(#337370,#337371,#337372),(#337373,
#337374,#337375),(#337376,#337377,#337378),(#337379,#337380,#337381),(#337382,
#337383,#337384),(#337385,#337386,#337387),(#337388,#337389,#337390),(#337391,
#337392,#337393),(#337394,#337395,#337396),(#337397,#337398,#337399),(#337400,
#337401,#337402),(#337403,#337404,#337405),(#337406,#337407,#337408),(#337409,
#337410,#337411),(#337412,#337413,#337414),(#337415,#337416,#337417),(#337418,
#337419,#337420),(#337421,#337422,#337423),(#337424,#337425,#337426),(#337427,
#337428,#337429),(#337430,#337431,#337432),(#337433,#337434,#337435),(#337436,
#337437,#337438),(#337439,#337440,#337441),(#337442,#337443,#337444),(#337445,
#337446,#337447),(#337448,#337449,#337450),(#337451,#337452,#337453),(#337454,
#337455,#337456),(#337457,#337458,#337459),(#337460,#337461,#337462),(#337463,
#337464,#337465),(#337466,#337467,#337468),(#337469,#337470,#337471),(#337472,
#337473,#337474),(#337475,#337476,#337477),(#337478,#337479,#337480),(#337481,
#337482,#337483),(#337484,#337485,#337486),(#337487,#337488,#337489),(#337490,
#337491,#337492),(#337493,#337494,#337495),(#337496,#337497,#337498),(#337499,
#337500,#337501),(#337502,#337503,#337504),(#337505,#337506,#337507),(#337508,
#337509,#337510),(#337511,#337512,#337513),(#337514,#337515,#337516),(#337517,
#337518,#337519),(#337520,#337521,#337522),(#337523,#337524,#337525),(#337526,
#337527,#337528),(#337529,#337530,#337531),(#337532,#337533,#337534),(#337535,
#337536,#337537),(#337538,#337539,#337540),(#337541,#337542,#337543),(#337544,
#337545,#337546),(#337547,#337548,#337549),(#337550,#337551,#337552),(#337553,
#337554,#337555),(#337556,#337557,#337558),(#337559,#337560,#337561),(#337562,
#337563,#337564),(#337565,#337566,#337567),(#337568,#337569,#337570),(#337571,
#337572,#337573),(#337574,#337575,#337576),(#337577,#337578,#337579),(#337580,
#337581,#337582),(#337583,#337584,#337585),(#337586,#337587,#337588),(#337589,
#337590,#337591),(#337592,#337593,#337594),(#337595,#337596,#337597),(#337598,
#337599,#337600),(#337601,#337602,#337603),(#337604,#337605,#337606),(#337607,
#337608,#337609),(#337610,#337611,#337612),(#337613,#337614,#337615),(#337616,
#337617,#337618),(#337619,#337620,#337621),(#337622,#337623,#337624),(#337625,
#337626,#337627),(#337628,#337629,#337630),(#337631,#337632,#337633),(#337634,
#337635,#337636),(#337637,#337638,#337639),(#337640,#337641,#337642),(#337643,
#337644,#337645),(#337646,#337647,#337648),(#337649,#337650,#337651),(#337652,
#337653,#337654),(#337655,#337656,#337657),(#337658,#337659,#337660),(#337661,
#337662,#337663),(#337664,#337665,#337666),(#337667,#337668,#337669),(#337670,
#337671,#337672),(#337673,#337674,#337675),(#337676,#337677,#337678),(#337679,
#337680,#337681),(#337682,#337683,#337684),(#337685,#337686,#337687),(#337688,
#337689,#337690),(#337691,#337692,#337693),(#337694,#337695,#337696),(#337697,
#337698,#337699),(#337700,#337701,#337702),(#337703,#337704,#337705),(#337706,
#337707,#337708),(#337709,#337710,#337711),(#337712,#337713,#337714),(#337715,
#337716,#337717),(#337718,#337719,#337720),(#337721,#337722,#337723),(#337724,
#337725,#337726),(#337727,#337728,#337729),(#337730,#337731,#337732),(#337733,
#337734,#337735),(#337736,#337737,#337738),(#337739,#337740,#337741),(#337742,
#337743,#337744),(#337745,#337746,#337747),(#337748,#337749,#337750),(#337751,
#337752,#337753),(#337754,#337755,#337756),(#337757,#337758,#337759),(#337760,
#337761,#337762),(#337763,#337764,#337765),(#337766,#337767,#337768),(#337769,
#337770,#337771),(#337772,#337773,#337774),(#337775,#337776,#337777),(#337778,
#337779,#337780),(#337781,#337782,#337783),(#337784,#337785,#337786),(#337787,
#337788,#337789),(#337790,#337791,#337792),(#337793,#337794,#337795),(#337796,
#337797,#337798),(#337799,#337800,#337801),(#337802,#337803,#337804),(#337805,
#337806,#337807),(#337808,#337809,#337810),(#337811,#337812,#337813),(#337814,
#337815,#337816),(#337817,#337818,#337819),(#337820,#337821,#337822),(#337823,
#337824,#337825),(#337826,#337827,#337828),(#337829,#337830,#337831),(#337832,
#337833,#337834),(#337835,#337836,#337837),(#337838,#337839,#337840),(#337841,
#337842,#337843),(#337844,#337845,#337846),(#337847,#337848,#337849),(#337850,
#337851,#337852),(#337853,#337854,#337855),(#337856,#337857,#337858),(#337859,
#337860,#337861),(#337862,#337863,#337864),(#337865,#337866,#337867),(#337868,
#337869,#337870),(#337871,#337872,#337873),(#337874,#337875,#337876),(#337877,
#337878,#337879),(#337880,#337881,#337882),(#337883,#337884,#337885),(#337886,
#337887,#337888),(#337889,#337890,#337891),(#337892,#337893,#337894),(#337895,
#337896,#337897),(#337898,#337899,#337900),(#337901,#337902,#337903),(#337904,
#337905,#337906),(#337907,#337908,#337909),(#337910,#337911,#337912),(#337913,
#337914,#337915),(#337916,#337917,#337918),(#337919,#337920,#337921),(#337922,
#337923,#337924),(#337925,#337926,#337927),(#337928,#337929,#337930),(#337931,
#337932,#337933),(#337934,#337935,#337936),(#337937,#337938,#337939),(#337940,
#337941,#337942),(#337943,#337944,#337945),(#337946,#337947,#337948),(#337949,
#337950,#337951),(#337952,#337953,#337954),(#337955,#337956,#337957),(#337958,
#337959,#337960),(#337961,#337962,#337963),(#337964,#337965,#337966),(#337967,
#337968,#337969),(#337970,#337971,#337972),(#337973,#337974,#337975),(#337976,
#337977,#337978),(#337979,#337980,#337981),(#337982,#337983,#337984),(#337985,
#337986,#337987),(#337988,#337989,#337990),(#337991,#337992,#337993),(#337994,
#337995,#337996),(#337997,#337998,#337999),(#338000,#338001,#338002),(#338003,
#338004,#338005),(#338006,#338007,#338008),(#338009,#338010,#338011),(#338012,
#338013,#338014),(#338015,#338016,#338017),(#338018,#338019,#338020),(#338021,
#338022,#338023),(#338024,#338025,#338026),(#338027,#338028,#338029),(#338030,
#338031,#338032),(#338033,#338034,#338035),(#338036,#338037,#338038),(#338039,
#338040,#338041),(#338042,#338043,#338044),(#338045,#338046,#338047),(#338048,
#338049,#338050),(#338051,#338052,#338053),(#338054,#338055,#338056),(#338057,
#338058,#338059),(#338060,#338061,#338062),(#338063,#338064,#338065),(#338066,
#338067,#338068),(#338069,#338070,#338071),(#338072,#338073,#338074),(#338075,
#338076,#338077),(#338078,#338079,#338080),(#338081,#338082,#338083),(#338084,
#338085,#338086),(#338087,#338088,#338089),(#338090,#338091,#338092),(#338093,
#338094,#338095),(#338096,#338097,#338098),(#338099,#338100,#338101),(#338102,
#338103,#338104),(#338105,#338106,#338107),(#338108,#338109,#338110),(#338111,
#338112,#338113),(#338114,#338115,#338116),(#338117,#338118,#338119),(#338120,
#338121,#338122),(#338123,#338124,#338125),(#338126,#338127,#338128),(#338129,
#338130,#338131),(#338132,#338133,#338134),(#338135,#338136,#338137),(#338138,
#338139,#338140),(#338141,#338142,#338143),(#338144,#338145,#338146),(#338147,
#338148,#338149),(#338150,#338151,#338152),(#338153,#338154,#338155),(#338156,
#338157,#338158),(#338159,#338160,#338161),(#338162,#338163,#338164),(#338165,
#338166,#338167),(#338168,#338169,#338170),(#338171,#338172,#338173),(#338174,
#338175,#338176),(#338177,#338178,#338179),(#338180,#338181,#338182),(#338183,
#338184,#338185),(#338186,#338187,#338188),(#338189,#338190,#338191),(#338192,
#338193,#338194),(#338195,#338196,#338197),(#338198,#338199,#338200),(#338201,
#338202,#338203),(#338204,#338205,#338206),(#338207,#338208,#338209),(#338210,
#338211,#338212),(#338213,#338214,#338215),(#338216,#338217,#338218),(#338219,
#338220,#338221),(#338222,#338223,#338224),(#338225,#338226,#338227),(#338228,
#338229,#338230),(#338231,#338232,#338233),(#338234,#338235,#338236),(#338237,
#338238,#338239),(#338240,#338241,#338242),(#338243,#338244,#338245),(#338246,
#338247,#338248),(#338249,#338250,#338251),(#338252,#338253,#338254),(#338255,
#338256,#338257),(#338258,#338259,#338260),(#338261,#338262,#338263),(#338264,
#338265,#338266),(#338267,#338268,#338269),(#338270,#338271,#338272),(#338273,
#338274,#338275)),.UNSPECIFIED.,.F.,.F.,.F.,(6,1,1,1,1,1,1,1,1,1,1,1,1,
1,1,1,1,1,1,1,1,1,1,1,1,1,1,1,1,1,1,1,1,1,1,1,1,1,1,1,1,1,1,1,1,1,1,1,1,
1,1,1,1,1,1,1,1,1,1,1,1,1,1,1,1,1,1,1,1,1,1,1,1,1,1,1,1,1,1,1,1,1,1,1,1,
1,1,1,1,1,1,1,1,1,1,1,1,1,1,1,1,1,1,1,1,1,1,1,1,1,1,1,1,1,1,1,1,1,1,1,1,
1,1,1,1,1,1,1,1,1,1,1,1,1,1,1,1,1,1,1,1,1,1,1,1,1,1,1,1,1,1,1,1,1,1,1,1,
1,1,1,1,1,1,1,1,1,1,1,1,1,1,1,1,1,1,1,1,1,1,1,1,1,1,1,1,1,1,1,1,1,1,1,1,
1,1,1,1,1,1,1,1,1,1,1,1,1,1,1,1,1,1,1,1,1,1,1,1,1,1,1,1,1,1,1,1,1,1,1,1,
1,1,1,1,1,1,1,1,1,1,1,1,1,1,1,1,1,1,1,1,1,1,1,1,1,1,1,1,1,1,1,1,1,1,1,1,
1,1,1,1,1,1,1,1,1,1,1,1,1,1,1,1,1,1,1,1,1,1,1,1,1,1,1,1,1,1,1,1,1,1,1,1,
1,1,1,1,1,1,1,1,1,1,1,1,1,1,1,1,1,1,1,1,1,1,1,1,1,1,1,1,1,1,1,1,1,1,1,1,
1,1,1,1,1,1,1,1,1,1,1,1,1,1,1,1,1,1,1,1,1,1,1,1,1,1,1,1,1,1,1,1,1,1,1,1,
1,1,1,1,1,1,1,1,1,1,1,1,1,1,1,1,1,1,1,1,1,1,1,1,1,1,1,1,1,1,1,1,1,1,1,1,
1,1,1,1,1,1,1,1,1,1,1,1,1,1,1,1,1,1,1,1,1,1,1,1,1,1,1,1,1,1,1,1,1,1,1,1,
1,1,1,1,1,1,1,1,1,1,1,1,1,1,1,1,1,1,1,1,1,1,1,1,1,1,1,1,1,1,1,1,1,1,1,1,
1,1,1,1,1,1,1,1,1,1,1,1,1,1,1,1,1,1,1,1,1,1,1,1,1,1,1,1,1,1,1,1,1,1,1,1,
1,1,1,1,1,1,1,1,1,1,1,1,1,1,1,1,1,1,1,1,1,1,1,1,1,1,1,1,1,6),(2,1,2),(-0.001964156,
0.,0.001834862,0.003669725,0.005504587,0.00733945,0.009174312,0.011009174,
0.012844037,0.014678899,0.016513761,0.018348624,0.020183486,0.022018349,
0.023853211,0.025688073,0.027522936,0.029357798,0.031192661,0.033027523,
0.034862385,0.036697248,0.03853211,0.040366972,0.042201835,0.044036697,
0.04587156,0.047706422,0.049541284,0.051376147,0.053211009,0.055045872,
0.056880734,0.058715596,0.060550459,0.062385321,0.064220183,0.066055046,
0.067889908,0.069724771,0.071559633,0.073394495,0.075229358,0.07706422,
0.078899083,0.080733945,0.082568807,0.08440367,0.086238532,0.088073394,
0.089908257,0.091743119,0.093577982,0.095412844,0.097247706,0.099082569,
0.100917431,0.102752294,0.104587156,0.106422018,0.108256881,0.110091743,
0.111926606,0.113761468,0.11559633,0.117431193,0.119266055,0.121100917,
0.12293578,0.124770642,0.126605505,0.128440367,0.130275229,0.132110092,
0.133944954,0.135779817,0.137614679,0.139449541,0.141284404,0.143119266,
0.144954128,0.146788991,0.148623853,0.150458716,0.152293578,0.15412844,
0.155963303,0.157798165,0.159633028,0.16146789,0.163302752,0.165137615,
0.166972477,0.168807339,0.170642202,0.172477064,0.174311927,0.176146789,
0.177981651,0.179816514,0.181651376,0.183486239,0.185321101,0.187155963,
0.188990826,0.190825688,0.19266055,0.194495413,0.196330275,0.198165138,
0.2,0.201834862,0.203669725,0.205504587,0.20733945,0.209174312,0.211009174,
0.212844037,0.214678899,0.216513761,0.218348624,0.220183486,0.222018349,
0.223853211,0.225688073,0.227522936,0.229357798,0.231192661,0.233027523,
0.234862385,0.236697248,0.23853211,0.240366972,0.242201835,0.244036697,
0.24587156,0.247706422,0.249541284,0.251376147,0.253211009,0.255045872,
0.256880734,0.258715596,0.260550459,0.262385321,0.264220183,0.266055046,
0.267889908,0.269724771,0.271559633,0.273394495,0.275229358,0.27706422,
0.278899083,0.280733945,0.282568807,0.28440367,0.286238532,0.288073394,
0.289908257,0.291743119,0.293577982,0.295412844,0.297247706,0.299082569,
0.300917431,0.302752294,0.304587156,0.306422018,0.308256881,0.310091743,
0.311926606,0.313761468,0.31559633,0.317431193,0.319266055,0.321100917,
0.32293578,0.324770642,0.326605505,0.328440367,0.330275229,0.332110092,
0.333944954,0.335779817,0.337614679,0.339449541,0.341284404,0.343119266,
0.344954128,0.346788991,0.348623853,0.350458716,0.352293578,0.35412844,
0.355963303,0.357798165,0.359633028,0.36146789,0.363302752,0.365137615,
0.366972477,0.368807339,0.370642202,0.372477064,0.374311927,0.376146789,
0.377981651,0.379816514,0.381651376,0.383486239,0.385321101,0.387155963,
0.388990826,0.390825688,0.39266055,0.394495413,0.396330275,0.398165138,
0.4,0.401834862,0.403669725,0.405504587,0.40733945,0.409174312,0.411009174,
0.412844037,0.414678899,0.416513761,0.418348624,0.420183486,0.422018349,
0.423853211,0.425688073,0.427522936,0.429357798,0.431192661,0.433027523,
0.434862385,0.436697248,0.43853211,0.440366972,0.442201835,0.444036697,
0.44587156,0.447706422,0.449541284,0.451376147,0.453211009,0.455045872,
0.456880734,0.458715596,0.460550459,0.462385321,0.464220183,0.466055046,
0.467889908,0.469724771,0.471559633,0.473394495,0.475229358,0.47706422,
0.478899083,0.480733945,0.482568807,0.48440367,0.486238532,0.488073394,
0.489908257,0.491743119,0.493577982,0.495412844,0.497247706,0.499082569,
0.500917431,0.502752294,0.504587156,0.506422018,0.508256881,0.510091743,
0.511926606,0.513761468,0.51559633,0.517431193,0.519266055,0.521100917,
0.52293578,0.524770642,0.526605505,0.528440367,0.530275229,0.532110092,
0.533944954,0.535779817,0.537614679,0.539449541,0.541284404,0.543119266,
0.544954128,0.546788991,0.548623853,0.550458716,0.552293578,0.55412844,
0.555963303,0.557798165,0.559633028,0.56146789,0.563302752,0.565137615,
0.566972477,0.568807339,0.570642202,0.572477064,0.574311927,0.576146789,
0.577981651,0.579816514,0.581651376,0.583486239,0.585321101,0.587155963,
0.588990826,0.590825688,0.59266055,0.594495413,0.596330275,0.598165138,
0.6,0.601834862,0.603669725,0.605504587,0.60733945,0.609174312,0.611009174,
0.612844037,0.614678899,0.616513761,0.618348624,0.620183486,0.622018349,
0.623853211,0.625688073,0.627522936,0.629357798,0.631192661,0.633027523,
0.634862385,0.636697248,0.63853211,0.640366972,0.642201835,0.644036697,
0.64587156,0.647706422,0.649541284,0.651376147,0.653211009,0.655045872,
0.656880734,0.658715596,0.660550459,0.662385321,0.664220183,0.666055046,
0.667889908,0.669724771,0.671559633,0.673394495,0.675229358,0.67706422,
0.678899083,0.680733945,0.682568807,0.68440367,0.686238532,0.688073394,
0.689908257,0.691743119,0.693577982,0.695412844,0.697247706,0.699082569,
0.700917431,0.702752294,0.704587156,0.706422018,0.708256881,0.710091743,
0.711926606,0.713761468,0.71559633,0.717431193,0.719266055,0.721100917,
0.72293578,0.724770642,0.726605505,0.728440367,0.730275229,0.732110092,
0.733944954,0.735779817,0.737614679,0.739449541,0.741284404,0.743119266,
0.744954128,0.746788991,0.748623853,0.750458716,0.752293578,0.75412844,
0.755963303,0.757798165,0.759633028,0.76146789,0.763302752,0.765137615,
0.766972477,0.768807339,0.770642202,0.772477064,0.774311927,0.776146789,
0.777981651,0.779816514,0.781651376,0.783486239,0.785321101,0.787155963,
0.788990826,0.790825688,0.79266055,0.794495413,0.796330275,0.798165138,
0.8,0.801834862,0.803669725,0.805504587,0.80733945,0.809174312,0.811009174,
0.812844037,0.814678899,0.816513761,0.818348624,0.820183486,0.822018349,
0.823853211,0.825688073,0.827522936,0.829357798,0.831192661,0.833027523,
0.834862385,0.836697248,0.83853211,0.840366972,0.842201835,0.844036697,
0.84587156,0.847706422,0.849541284,0.851376147,0.853211009,0.855045872,
0.856880734,0.858715596,0.860550459,0.862385321,0.864220183,0.866055046,
0.867889908,0.869724771,0.871559633,0.873394495,0.875229358,0.87706422,
0.878899083,0.880733945,0.882568807,0.88440367,0.886238532,0.888073394,
0.889908257,0.891743119,0.893577982,0.895412844,0.897247706,0.899082569,
0.900917431,0.902752294,0.904587156,0.906422018,0.908256881,0.910091743,
0.911926606,0.913761468,0.91559633,0.917431193,0.919266055,0.921100917,
0.92293578,0.924770642,0.926605505,0.928440367,0.930275229,0.932110092,
0.933944954,0.935779817,0.937614679,0.939449541,0.941284404,0.943119266,
0.944954128,0.946788991,0.948623853,0.950458716,0.952293578,0.95412844,
0.955963303,0.957798165,0.959633028,0.96146789,0.963302752,0.965137615,
0.966972477,0.968807339,0.970642202,0.972477064,0.974311927,0.976146789,
0.977981651,0.979816514,0.981651376,0.983486239,0.985321101,0.987155963,
0.988990826,0.990825688,0.99266055,0.994495413,0.996330275,0.998165138,
1.000000000264),(0.3,1.,1.3),.UNSPECIFIED.);
#6325=B_SPLINE_SURFACE_WITH_KNOTS('',5,1,((#338282,#338283,#338284),(#338285,
#338286,#338287),(#338288,#338289,#338290),(#338291,#338292,#338293),(#338294,
#338295,#338296),(#338297,#338298,#338299),(#338300,#338301,#338302),(#338303,
#338304,#338305),(#338306,#338307,#338308),(#338309,#338310,#338311),(#338312,
#338313,#338314),(#338315,#338316,#338317),(#338318,#338319,#338320),(#338321,
#338322,#338323),(#338324,#338325,#338326),(#338327,#338328,#338329),(#338330,
#338331,#338332),(#338333,#338334,#338335),(#338336,#338337,#338338),(#338339,
#338340,#338341),(#338342,#338343,#338344),(#338345,#338346,#338347),(#338348,
#338349,#338350),(#338351,#338352,#338353),(#338354,#338355,#338356),(#338357,
#338358,#338359),(#338360,#338361,#338362),(#338363,#338364,#338365),(#338366,
#338367,#338368),(#338369,#338370,#338371),(#338372,#338373,#338374),(#338375,
#338376,#338377),(#338378,#338379,#338380),(#338381,#338382,#338383),(#338384,
#338385,#338386),(#338387,#338388,#338389),(#338390,#338391,#338392),(#338393,
#338394,#338395),(#338396,#338397,#338398),(#338399,#338400,#338401),(#338402,
#338403,#338404),(#338405,#338406,#338407),(#338408,#338409,#338410),(#338411,
#338412,#338413),(#338414,#338415,#338416),(#338417,#338418,#338419),(#338420,
#338421,#338422),(#338423,#338424,#338425),(#338426,#338427,#338428),(#338429,
#338430,#338431),(#338432,#338433,#338434),(#338435,#338436,#338437),(#338438,
#338439,#338440),(#338441,#338442,#338443),(#338444,#338445,#338446),(#338447,
#338448,#338449),(#338450,#338451,#338452),(#338453,#338454,#338455),(#338456,
#338457,#338458),(#338459,#338460,#338461),(#338462,#338463,#338464),(#338465,
#338466,#338467),(#338468,#338469,#338470),(#338471,#338472,#338473),(#338474,
#338475,#338476),(#338477,#338478,#338479),(#338480,#338481,#338482),(#338483,
#338484,#338485),(#338486,#338487,#338488),(#338489,#338490,#338491),(#338492,
#338493,#338494),(#338495,#338496,#338497),(#338498,#338499,#338500),(#338501,
#338502,#338503),(#338504,#338505,#338506),(#338507,#338508,#338509),(#338510,
#338511,#338512),(#338513,#338514,#338515),(#338516,#338517,#338518),(#338519,
#338520,#338521),(#338522,#338523,#338524),(#338525,#338526,#338527),(#338528,
#338529,#338530),(#338531,#338532,#338533),(#338534,#338535,#338536),(#338537,
#338538,#338539),(#338540,#338541,#338542),(#338543,#338544,#338545),(#338546,
#338547,#338548),(#338549,#338550,#338551),(#338552,#338553,#338554),(#338555,
#338556,#338557),(#338558,#338559,#338560),(#338561,#338562,#338563),(#338564,
#338565,#338566),(#338567,#338568,#338569),(#338570,#338571,#338572),(#338573,
#338574,#338575),(#338576,#338577,#338578),(#338579,#338580,#338581),(#338582,
#338583,#338584),(#338585,#338586,#338587),(#338588,#338589,#338590),(#338591,
#338592,#338593),(#338594,#338595,#338596),(#338597,#338598,#338599),(#338600,
#338601,#338602),(#338603,#338604,#338605),(#338606,#338607,#338608),(#338609,
#338610,#338611),(#338612,#338613,#338614),(#338615,#338616,#338617),(#338618,
#338619,#338620),(#338621,#338622,#338623),(#338624,#338625,#338626),(#338627,
#338628,#338629),(#338630,#338631,#338632),(#338633,#338634,#338635),(#338636,
#338637,#338638),(#338639,#338640,#338641),(#338642,#338643,#338644),(#338645,
#338646,#338647),(#338648,#338649,#338650),(#338651,#338652,#338653),(#338654,
#338655,#338656),(#338657,#338658,#338659),(#338660,#338661,#338662),(#338663,
#338664,#338665),(#338666,#338667,#338668),(#338669,#338670,#338671),(#338672,
#338673,#338674),(#338675,#338676,#338677),(#338678,#338679,#338680),(#338681,
#338682,#338683),(#338684,#338685,#338686),(#338687,#338688,#338689),(#338690,
#338691,#338692),(#338693,#338694,#338695),(#338696,#338697,#338698),(#338699,
#338700,#338701),(#338702,#338703,#338704),(#338705,#338706,#338707),(#338708,
#338709,#338710),(#338711,#338712,#338713),(#338714,#338715,#338716),(#338717,
#338718,#338719),(#338720,#338721,#338722),(#338723,#338724,#338725),(#338726,
#338727,#338728),(#338729,#338730,#338731),(#338732,#338733,#338734),(#338735,
#338736,#338737),(#338738,#338739,#338740),(#338741,#338742,#338743),(#338744,
#338745,#338746),(#338747,#338748,#338749),(#338750,#338751,#338752),(#338753,
#338754,#338755),(#338756,#338757,#338758),(#338759,#338760,#338761),(#338762,
#338763,#338764),(#338765,#338766,#338767),(#338768,#338769,#338770),(#338771,
#338772,#338773),(#338774,#338775,#338776),(#338777,#338778,#338779),(#338780,
#338781,#338782),(#338783,#338784,#338785),(#338786,#338787,#338788),(#338789,
#338790,#338791),(#338792,#338793,#338794),(#338795,#338796,#338797),(#338798,
#338799,#338800),(#338801,#338802,#338803),(#338804,#338805,#338806),(#338807,
#338808,#338809),(#338810,#338811,#338812),(#338813,#338814,#338815),(#338816,
#338817,#338818),(#338819,#338820,#338821),(#338822,#338823,#338824),(#338825,
#338826,#338827),(#338828,#338829,#338830),(#338831,#338832,#338833),(#338834,
#338835,#338836),(#338837,#338838,#338839),(#338840,#338841,#338842),(#338843,
#338844,#338845),(#338846,#338847,#338848),(#338849,#338850,#338851),(#338852,
#338853,#338854),(#338855,#338856,#338857),(#338858,#338859,#338860),(#338861,
#338862,#338863),(#338864,#338865,#338866),(#338867,#338868,#338869),(#338870,
#338871,#338872),(#338873,#338874,#338875),(#338876,#338877,#338878),(#338879,
#338880,#338881),(#338882,#338883,#338884),(#338885,#338886,#338887),(#338888,
#338889,#338890),(#338891,#338892,#338893),(#338894,#338895,#338896),(#338897,
#338898,#338899),(#338900,#338901,#338902),(#338903,#338904,#338905),(#338906,
#338907,#338908),(#338909,#338910,#338911),(#338912,#338913,#338914),(#338915,
#338916,#338917),(#338918,#338919,#338920),(#338921,#338922,#338923),(#338924,
#338925,#338926),(#338927,#338928,#338929),(#338930,#338931,#338932),(#338933,
#338934,#338935),(#338936,#338937,#338938),(#338939,#338940,#338941),(#338942,
#338943,#338944),(#338945,#338946,#338947),(#338948,#338949,#338950),(#338951,
#338952,#338953),(#338954,#338955,#338956),(#338957,#338958,#338959),(#338960,
#338961,#338962),(#338963,#338964,#338965),(#338966,#338967,#338968),(#338969,
#338970,#338971),(#338972,#338973,#338974),(#338975,#338976,#338977),(#338978,
#338979,#338980),(#338981,#338982,#338983),(#338984,#338985,#338986),(#338987,
#338988,#338989),(#338990,#338991,#338992),(#338993,#338994,#338995),(#338996,
#338997,#338998),(#338999,#339000,#339001),(#339002,#339003,#339004),(#339005,
#339006,#339007),(#339008,#339009,#339010),(#339011,#339012,#339013),(#339014,
#339015,#339016),(#339017,#339018,#339019),(#339020,#339021,#339022),(#339023,
#339024,#339025),(#339026,#339027,#339028),(#339029,#339030,#339031),(#339032,
#339033,#339034),(#339035,#339036,#339037),(#339038,#339039,#339040),(#339041,
#339042,#339043),(#339044,#339045,#339046),(#339047,#339048,#339049),(#339050,
#339051,#339052),(#339053,#339054,#339055),(#339056,#339057,#339058),(#339059,
#339060,#339061),(#339062,#339063,#339064),(#339065,#339066,#339067),(#339068,
#339069,#339070),(#339071,#339072,#339073),(#339074,#339075,#339076),(#339077,
#339078,#339079),(#339080,#339081,#339082),(#339083,#339084,#339085),(#339086,
#339087,#339088),(#339089,#339090,#339091),(#339092,#339093,#339094),(#339095,
#339096,#339097),(#339098,#339099,#339100),(#339101,#339102,#339103),(#339104,
#339105,#339106),(#339107,#339108,#339109),(#339110,#339111,#339112),(#339113,
#339114,#339115),(#339116,#339117,#339118),(#339119,#339120,#339121),(#339122,
#339123,#339124),(#339125,#339126,#339127),(#339128,#339129,#339130),(#339131,
#339132,#339133),(#339134,#339135,#339136),(#339137,#339138,#339139),(#339140,
#339141,#339142),(#339143,#339144,#339145),(#339146,#339147,#339148),(#339149,
#339150,#339151),(#339152,#339153,#339154),(#339155,#339156,#339157),(#339158,
#339159,#339160),(#339161,#339162,#339163),(#339164,#339165,#339166),(#339167,
#339168,#339169),(#339170,#339171,#339172),(#339173,#339174,#339175),(#339176,
#339177,#339178),(#339179,#339180,#339181),(#339182,#339183,#339184),(#339185,
#339186,#339187),(#339188,#339189,#339190),(#339191,#339192,#339193),(#339194,
#339195,#339196),(#339197,#339198,#339199),(#339200,#339201,#339202),(#339203,
#339204,#339205),(#339206,#339207,#339208),(#339209,#339210,#339211),(#339212,
#339213,#339214),(#339215,#339216,#339217),(#339218,#339219,#339220),(#339221,
#339222,#339223),(#339224,#339225,#339226),(#339227,#339228,#339229),(#339230,
#339231,#339232),(#339233,#339234,#339235),(#339236,#339237,#339238),(#339239,
#339240,#339241),(#339242,#339243,#339244),(#339245,#339246,#339247),(#339248,
#339249,#339250),(#339251,#339252,#339253),(#339254,#339255,#339256),(#339257,
#339258,#339259),(#339260,#339261,#339262),(#339263,#339264,#339265),(#339266,
#339267,#339268),(#339269,#339270,#339271),(#339272,#339273,#339274),(#339275,
#339276,#339277),(#339278,#339279,#339280),(#339281,#339282,#339283),(#339284,
#339285,#339286),(#339287,#339288,#339289),(#339290,#339291,#339292),(#339293,
#339294,#339295),(#339296,#339297,#339298),(#339299,#339300,#339301),(#339302,
#339303,#339304),(#339305,#339306,#339307),(#339308,#339309,#339310),(#339311,
#339312,#339313),(#339314,#339315,#339316),(#339317,#339318,#339319),(#339320,
#339321,#339322),(#339323,#339324,#339325),(#339326,#339327,#339328),(#339329,
#339330,#339331),(#339332,#339333,#339334),(#339335,#339336,#339337),(#339338,
#339339,#339340),(#339341,#339342,#339343),(#339344,#339345,#339346),(#339347,
#339348,#339349),(#339350,#339351,#339352),(#339353,#339354,#339355),(#339356,
#339357,#339358),(#339359,#339360,#339361),(#339362,#339363,#339364),(#339365,
#339366,#339367),(#339368,#339369,#339370),(#339371,#339372,#339373),(#339374,
#339375,#339376),(#339377,#339378,#339379),(#339380,#339381,#339382),(#339383,
#339384,#339385),(#339386,#339387,#339388),(#339389,#339390,#339391),(#339392,
#339393,#339394),(#339395,#339396,#339397),(#339398,#339399,#339400),(#339401,
#339402,#339403),(#339404,#339405,#339406),(#339407,#339408,#339409),(#339410,
#339411,#339412),(#339413,#339414,#339415),(#339416,#339417,#339418),(#339419,
#339420,#339421),(#339422,#339423,#339424),(#339425,#339426,#339427),(#339428,
#339429,#339430),(#339431,#339432,#339433),(#339434,#339435,#339436),(#339437,
#339438,#339439),(#339440,#339441,#339442),(#339443,#339444,#339445),(#339446,
#339447,#339448),(#339449,#339450,#339451),(#339452,#339453,#339454),(#339455,
#339456,#339457),(#339458,#339459,#339460),(#339461,#339462,#339463),(#339464,
#339465,#339466),(#339467,#339468,#339469),(#339470,#339471,#339472),(#339473,
#339474,#339475),(#339476,#339477,#339478),(#339479,#339480,#339481),(#339482,
#339483,#339484),(#339485,#339486,#339487),(#339488,#339489,#339490),(#339491,
#339492,#339493),(#339494,#339495,#339496),(#339497,#339498,#339499),(#339500,
#339501,#339502),(#339503,#339504,#339505),(#339506,#339507,#339508),(#339509,
#339510,#339511),(#339512,#339513,#339514),(#339515,#339516,#339517),(#339518,
#339519,#339520),(#339521,#339522,#339523),(#339524,#339525,#339526),(#339527,
#339528,#339529),(#339530,#339531,#339532),(#339533,#339534,#339535),(#339536,
#339537,#339538),(#339539,#339540,#339541),(#339542,#339543,#339544),(#339545,
#339546,#339547),(#339548,#339549,#339550),(#339551,#339552,#339553),(#339554,
#339555,#339556),(#339557,#339558,#339559),(#339560,#339561,#339562),(#339563,
#339564,#339565),(#339566,#339567,#339568),(#339569,#339570,#339571),(#339572,
#339573,#339574),(#339575,#339576,#339577),(#339578,#339579,#339580),(#339581,
#339582,#339583),(#339584,#339585,#339586),(#339587,#339588,#339589),(#339590,
#339591,#339592),(#339593,#339594,#339595),(#339596,#339597,#339598),(#339599,
#339600,#339601),(#339602,#339603,#339604),(#339605,#339606,#339607),(#339608,
#339609,#339610),(#339611,#339612,#339613),(#339614,#339615,#339616),(#339617,
#339618,#339619),(#339620,#339621,#339622),(#339623,#339624,#339625),(#339626,
#339627,#339628),(#339629,#339630,#339631),(#339632,#339633,#339634),(#339635,
#339636,#339637),(#339638,#339639,#339640),(#339641,#339642,#339643),(#339644,
#339645,#339646),(#339647,#339648,#339649),(#339650,#339651,#339652),(#339653,
#339654,#339655),(#339656,#339657,#339658),(#339659,#339660,#339661),(#339662,
#339663,#339664),(#339665,#339666,#339667),(#339668,#339669,#339670),(#339671,
#339672,#339673),(#339674,#339675,#339676),(#339677,#339678,#339679),(#339680,
#339681,#339682),(#339683,#339684,#339685),(#339686,#339687,#339688),(#339689,
#339690,#339691),(#339692,#339693,#339694),(#339695,#339696,#339697),(#339698,
#339699,#339700),(#339701,#339702,#339703),(#339704,#339705,#339706),(#339707,
#339708,#339709),(#339710,#339711,#339712),(#339713,#339714,#339715),(#339716,
#339717,#339718),(#339719,#339720,#339721),(#339722,#339723,#339724),(#339725,
#339726,#339727),(#339728,#339729,#339730),(#339731,#339732,#339733),(#339734,
#339735,#339736),(#339737,#339738,#339739),(#339740,#339741,#339742),(#339743,
#339744,#339745),(#339746,#339747,#339748),(#339749,#339750,#339751),(#339752,
#339753,#339754),(#339755,#339756,#339757),(#339758,#339759,#339760),(#339761,
#339762,#339763),(#339764,#339765,#339766),(#339767,#339768,#339769),(#339770,
#339771,#339772),(#339773,#339774,#339775),(#339776,#339777,#339778),(#339779,
#339780,#339781),(#339782,#339783,#339784),(#339785,#339786,#339787),(#339788,
#339789,#339790),(#339791,#339792,#339793),(#339794,#339795,#339796),(#339797,
#339798,#339799),(#339800,#339801,#339802),(#339803,#339804,#339805),(#339806,
#339807,#339808),(#339809,#339810,#339811),(#339812,#339813,#339814),(#339815,
#339816,#339817),(#339818,#339819,#339820),(#339821,#339822,#339823),(#339824,
#339825,#339826),(#339827,#339828,#339829),(#339830,#339831,#339832),(#339833,
#339834,#339835),(#339836,#339837,#339838),(#339839,#339840,#339841),(#339842,
#339843,#339844),(#339845,#339846,#339847),(#339848,#339849,#339850),(#339851,
#339852,#339853),(#339854,#339855,#339856),(#339857,#339858,#339859),(#339860,
#339861,#339862),(#339863,#339864,#339865),(#339866,#339867,#339868),(#339869,
#339870,#339871),(#339872,#339873,#339874),(#339875,#339876,#339877),(#339878,
#339879,#339880),(#339881,#339882,#339883),(#339884,#339885,#339886),(#339887,
#339888,#339889),(#339890,#339891,#339892),(#339893,#339894,#339895),(#339896,
#339897,#339898),(#339899,#339900,#339901),(#339902,#339903,#339904),(#339905,
#339906,#339907),(#339908,#339909,#339910),(#339911,#339912,#339913),(#339914,
#339915,#339916),(#339917,#339918,#339919),(#339920,#339921,#339922),(#339923,
#339924,#339925),(#339926,#339927,#339928),(#339929,#339930,#339931)),
 .UNSPECIFIED.,.F.,.F.,.F.,(6,1,1,1,1,1,1,1,1,1,1,1,1,1,1,1,1,1,1,1,1,1,
1,1,1,1,1,1,1,1,1,1,1,1,1,1,1,1,1,1,1,1,1,1,1,1,1,1,1,1,1,1,1,1,1,1,1,1,
1,1,1,1,1,1,1,1,1,1,1,1,1,1,1,1,1,1,1,1,1,1,1,1,1,1,1,1,1,1,1,1,1,1,1,1,
1,1,1,1,1,1,1,1,1,1,1,1,1,1,1,1,1,1,1,1,1,1,1,1,1,1,1,1,1,1,1,1,1,1,1,1,
1,1,1,1,1,1,1,1,1,1,1,1,1,1,1,1,1,1,1,1,1,1,1,1,1,1,1,1,1,1,1,1,1,1,1,1,
1,1,1,1,1,1,1,1,1,1,1,1,1,1,1,1,1,1,1,1,1,1,1,1,1,1,1,1,1,1,1,1,1,1,1,1,
1,1,1,1,1,1,1,1,1,1,1,1,1,1,1,1,1,1,1,1,1,1,1,1,1,1,1,1,1,1,1,1,1,1,1,1,
1,1,1,1,1,1,1,1,1,1,1,1,1,1,1,1,1,1,1,1,1,1,1,1,1,1,1,1,1,1,1,1,1,1,1,1,
1,1,1,1,1,1,1,1,1,1,1,1,1,1,1,1,1,1,1,1,1,1,1,1,1,1,1,1,1,1,1,1,1,1,1,1,
1,1,1,1,1,1,1,1,1,1,1,1,1,1,1,1,1,1,1,1,1,1,1,1,1,1,1,1,1,1,1,1,1,1,1,1,
1,1,1,1,1,1,1,1,1,1,1,1,1,1,1,1,1,1,1,1,1,1,1,1,1,1,1,1,1,1,1,1,1,1,1,1,
1,1,1,1,1,1,1,1,1,1,1,1,1,1,1,1,1,1,1,1,1,1,1,1,1,1,1,1,1,1,1,1,1,1,1,1,
1,1,1,1,1,1,1,1,1,1,1,1,1,1,1,1,1,1,1,1,1,1,1,1,1,1,1,1,1,1,1,1,1,1,1,1,
1,1,1,1,1,1,1,1,1,1,1,1,1,1,1,1,1,1,1,1,1,1,1,1,1,1,1,1,1,1,1,1,1,1,1,1,
1,1,1,1,1,1,1,1,1,1,1,1,1,1,1,1,1,1,1,1,1,1,1,1,1,1,1,1,1,1,1,1,1,1,1,1,
1,1,1,1,1,1,1,1,1,1,1,1,1,1,1,1,1,1,1,6),(2,1,2),(-1.,-0.998165138,-0.996330275,
-0.994495413,-0.99266055,-0.990825688,-0.988990826,-0.987155963,-0.985321101,
-0.983486239,-0.981651376,-0.979816514,-0.977981651,-0.976146789,-0.974311927,
-0.972477064,-0.970642202,-0.968807339,-0.966972477,-0.965137615,-0.963302752,
-0.96146789,-0.959633028,-0.957798165,-0.955963303,-0.95412844,-0.952293578,
-0.950458716,-0.948623853,-0.946788991,-0.944954128,-0.943119266,-0.941284404,
-0.939449541,-0.937614679,-0.935779817,-0.933944954,-0.932110092,-0.930275229,
-0.928440367,-0.926605505,-0.924770642,-0.92293578,-0.921100917,-0.919266055,
-0.917431193,-0.91559633,-0.913761468,-0.911926606,-0.910091743,-0.908256881,
-0.906422018,-0.904587156,-0.902752294,-0.900917431,-0.899082569,-0.897247706,
-0.895412844,-0.893577982,-0.891743119,-0.889908257,-0.888073394,-0.886238532,
-0.88440367,-0.882568807,-0.880733945,-0.878899083,-0.87706422,-0.875229358,
-0.873394495,-0.871559633,-0.869724771,-0.867889908,-0.866055046,-0.864220183,
-0.862385321,-0.860550459,-0.858715596,-0.856880734,-0.855045872,-0.853211009,
-0.851376147,-0.849541284,-0.847706422,-0.84587156,-0.844036697,-0.842201835,
-0.840366972,-0.83853211,-0.836697248,-0.834862385,-0.833027523,-0.831192661,
-0.829357798,-0.827522936,-0.825688073,-0.823853211,-0.822018349,-0.820183486,
-0.818348624,-0.816513761,-0.814678899,-0.812844037,-0.811009174,-0.809174312,
-0.80733945,-0.805504587,-0.803669725,-0.801834862,-0.8,-0.798165138,-0.796330275,
-0.794495413,-0.79266055,-0.790825688,-0.788990826,-0.787155963,-0.785321101,
-0.783486239,-0.781651376,-0.779816514,-0.777981651,-0.776146789,-0.774311927,
-0.772477064,-0.770642202,-0.768807339,-0.766972477,-0.765137615,-0.763302752,
-0.76146789,-0.759633028,-0.757798165,-0.755963303,-0.75412844,-0.752293578,
-0.750458716,-0.748623853,-0.746788991,-0.744954128,-0.743119266,-0.741284404,
-0.739449541,-0.737614679,-0.735779817,-0.733944954,-0.732110092,-0.730275229,
-0.728440367,-0.726605505,-0.724770642,-0.72293578,-0.721100917,-0.719266055,
-0.717431193,-0.71559633,-0.713761468,-0.711926606,-0.710091743,-0.708256881,
-0.706422018,-0.704587156,-0.702752294,-0.700917431,-0.699082569,-0.697247706,
-0.695412844,-0.693577982,-0.691743119,-0.689908257,-0.688073394,-0.686238532,
-0.68440367,-0.682568807,-0.680733945,-0.678899083,-0.67706422,-0.675229358,
-0.673394495,-0.671559633,-0.669724771,-0.667889908,-0.666055046,-0.664220183,
-0.662385321,-0.660550459,-0.658715596,-0.656880734,-0.655045872,-0.653211009,
-0.651376147,-0.649541284,-0.647706422,-0.64587156,-0.644036697,-0.642201835,
-0.640366972,-0.63853211,-0.636697248,-0.634862385,-0.633027523,-0.631192661,
-0.629357798,-0.627522936,-0.625688073,-0.623853211,-0.622018349,-0.620183486,
-0.618348624,-0.616513761,-0.614678899,-0.612844037,-0.611009174,-0.609174312,
-0.60733945,-0.605504587,-0.603669725,-0.601834862,-0.6,-0.598165138,-0.596330275,
-0.594495413,-0.59266055,-0.590825688,-0.588990826,-0.587155963,-0.585321101,
-0.583486239,-0.581651376,-0.579816514,-0.577981651,-0.576146789,-0.574311927,
-0.572477064,-0.570642202,-0.568807339,-0.566972477,-0.565137615,-0.563302752,
-0.56146789,-0.559633028,-0.557798165,-0.555963303,-0.55412844,-0.552293578,
-0.550458716,-0.548623853,-0.546788991,-0.544954128,-0.543119266,-0.541284404,
-0.539449541,-0.537614679,-0.535779817,-0.533944954,-0.532110092,-0.530275229,
-0.528440367,-0.526605505,-0.524770642,-0.52293578,-0.521100917,-0.519266055,
-0.517431193,-0.51559633,-0.513761468,-0.511926606,-0.510091743,-0.508256881,
-0.506422018,-0.504587156,-0.502752294,-0.500917431,-0.499082569,-0.497247706,
-0.495412844,-0.493577982,-0.491743119,-0.489908257,-0.488073394,-0.486238532,
-0.48440367,-0.482568807,-0.480733945,-0.478899083,-0.47706422,-0.475229358,
-0.473394495,-0.471559633,-0.469724771,-0.467889908,-0.466055046,-0.464220183,
-0.462385321,-0.460550459,-0.458715596,-0.456880734,-0.455045872,-0.453211009,
-0.451376147,-0.449541284,-0.447706422,-0.44587156,-0.444036697,-0.442201835,
-0.440366972,-0.43853211,-0.436697248,-0.434862385,-0.433027523,-0.431192661,
-0.429357798,-0.427522936,-0.425688073,-0.423853211,-0.422018349,-0.420183486,
-0.418348624,-0.416513761,-0.414678899,-0.412844037,-0.411009174,-0.409174312,
-0.40733945,-0.405504587,-0.403669725,-0.401834862,-0.4,-0.398165138,-0.396330275,
-0.394495413,-0.39266055,-0.390825688,-0.388990826,-0.387155963,-0.385321101,
-0.383486239,-0.381651376,-0.379816514,-0.377981651,-0.376146789,-0.374311927,
-0.372477064,-0.370642202,-0.368807339,-0.366972477,-0.365137615,-0.363302752,
-0.36146789,-0.359633028,-0.357798165,-0.355963303,-0.35412844,-0.352293578,
-0.350458716,-0.348623853,-0.346788991,-0.344954128,-0.343119266,-0.341284404,
-0.339449541,-0.337614679,-0.335779817,-0.333944954,-0.332110092,-0.330275229,
-0.328440367,-0.326605505,-0.324770642,-0.32293578,-0.321100917,-0.319266055,
-0.317431193,-0.31559633,-0.313761468,-0.311926606,-0.310091743,-0.308256881,
-0.306422018,-0.304587156,-0.302752294,-0.300917431,-0.299082569,-0.297247706,
-0.295412844,-0.293577982,-0.291743119,-0.289908257,-0.288073394,-0.286238532,
-0.28440367,-0.282568807,-0.280733945,-0.278899083,-0.27706422,-0.275229358,
-0.273394495,-0.271559633,-0.269724771,-0.267889908,-0.266055046,-0.264220183,
-0.262385321,-0.260550459,-0.258715596,-0.256880734,-0.255045872,-0.253211009,
-0.251376147,-0.249541284,-0.247706422,-0.24587156,-0.244036697,-0.242201835,
-0.240366972,-0.23853211,-0.236697248,-0.234862385,-0.233027523,-0.231192661,
-0.229357798,-0.227522936,-0.225688073,-0.223853211,-0.222018349,-0.220183486,
-0.218348624,-0.216513761,-0.214678899,-0.212844037,-0.211009174,-0.209174312,
-0.20733945,-0.205504587,-0.203669725,-0.201834862,-0.2,-0.198165138,-0.196330275,
-0.194495413,-0.19266055,-0.190825688,-0.188990826,-0.187155963,-0.185321101,
-0.183486239,-0.181651376,-0.179816514,-0.177981651,-0.176146789,-0.174311927,
-0.172477064,-0.170642202,-0.168807339,-0.166972477,-0.165137615,-0.163302752,
-0.16146789,-0.159633028,-0.157798165,-0.155963303,-0.15412844,-0.152293578,
-0.150458716,-0.148623853,-0.146788991,-0.144954128,-0.143119266,-0.141284404,
-0.139449541,-0.137614679,-0.135779817,-0.133944954,-0.132110092,-0.130275229,
-0.128440367,-0.126605505,-0.124770642,-0.12293578,-0.121100917,-0.119266055,
-0.117431193,-0.11559633,-0.113761468,-0.111926606,-0.110091743,-0.108256881,
-0.106422018,-0.104587156,-0.102752294,-0.100917431,-0.099082569,-0.097247706,
-0.095412844,-0.093577982,-0.091743119,-0.089908257,-0.088073394,-0.086238532,
-0.08440367,-0.082568807,-0.080733945,-0.078899083,-0.07706422,-0.075229358,
-0.073394495,-0.071559633,-0.069724771,-0.067889908,-0.066055046,-0.064220183,
-0.062385321,-0.060550459,-0.058715596,-0.056880734,-0.055045872,-0.053211009,
-0.051376147,-0.049541284,-0.047706422,-0.04587156,-0.044036697,-0.042201835,
-0.040366972,-0.03853211,-0.036697248,-0.034862385,-0.033027523,-0.031192661,
-0.029357798,-0.027522936,-0.025688073,-0.023853211,-0.022018349,-0.020183486,
-0.018348624,-0.016513761,-0.014678899,-0.012844037,-0.011009174,-0.009174312,
-0.00733945,-0.005504587,-0.003669725,-0.001834862,0.000982159),(0.3,1.,
1.3),.UNSPECIFIED.);
#6326=B_SPLINE_SURFACE_WITH_KNOTS('',5,1,((#339935,#339936,#339937),(#339938,
#339939,#339940),(#339941,#339942,#339943),(#339944,#339945,#339946),(#339947,
#339948,#339949),(#339950,#339951,#339952),(#339953,#339954,#339955),(#339956,
#339957,#339958),(#339959,#339960,#339961),(#339962,#339963,#339964),(#339965,
#339966,#339967),(#339968,#339969,#339970),(#339971,#339972,#339973),(#339974,
#339975,#339976),(#339977,#339978,#339979),(#339980,#339981,#339982),(#339983,
#339984,#339985),(#339986,#339987,#339988),(#339989,#339990,#339991),(#339992,
#339993,#339994),(#339995,#339996,#339997),(#339998,#339999,#340000),(#340001,
#340002,#340003),(#340004,#340005,#340006),(#340007,#340008,#340009),(#340010,
#340011,#340012),(#340013,#340014,#340015),(#340016,#340017,#340018),(#340019,
#340020,#340021),(#340022,#340023,#340024),(#340025,#340026,#340027),(#340028,
#340029,#340030),(#340031,#340032,#340033),(#340034,#340035,#340036),(#340037,
#340038,#340039),(#340040,#340041,#340042),(#340043,#340044,#340045),(#340046,
#340047,#340048),(#340049,#340050,#340051),(#340052,#340053,#340054),(#340055,
#340056,#340057),(#340058,#340059,#340060),(#340061,#340062,#340063),(#340064,
#340065,#340066),(#340067,#340068,#340069),(#340070,#340071,#340072),(#340073,
#340074,#340075),(#340076,#340077,#340078),(#340079,#340080,#340081),(#340082,
#340083,#340084),(#340085,#340086,#340087),(#340088,#340089,#340090),(#340091,
#340092,#340093),(#340094,#340095,#340096),(#340097,#340098,#340099),(#340100,
#340101,#340102),(#340103,#340104,#340105),(#340106,#340107,#340108),(#340109,
#340110,#340111),(#340112,#340113,#340114),(#340115,#340116,#340117),(#340118,
#340119,#340120),(#340121,#340122,#340123),(#340124,#340125,#340126),(#340127,
#340128,#340129),(#340130,#340131,#340132),(#340133,#340134,#340135),(#340136,
#340137,#340138),(#340139,#340140,#340141),(#340142,#340143,#340144),(#340145,
#340146,#340147),(#340148,#340149,#340150),(#340151,#340152,#340153),(#340154,
#340155,#340156),(#340157,#340158,#340159),(#340160,#340161,#340162),(#340163,
#340164,#340165),(#340166,#340167,#340168),(#340169,#340170,#340171),(#340172,
#340173,#340174),(#340175,#340176,#340177),(#340178,#340179,#340180),(#340181,
#340182,#340183),(#340184,#340185,#340186),(#340187,#340188,#340189),(#340190,
#340191,#340192),(#340193,#340194,#340195),(#340196,#340197,#340198),(#340199,
#340200,#340201),(#340202,#340203,#340204),(#340205,#340206,#340207),(#340208,
#340209,#340210),(#340211,#340212,#340213),(#340214,#340215,#340216),(#340217,
#340218,#340219),(#340220,#340221,#340222),(#340223,#340224,#340225),(#340226,
#340227,#340228),(#340229,#340230,#340231),(#340232,#340233,#340234),(#340235,
#340236,#340237),(#340238,#340239,#340240),(#340241,#340242,#340243),(#340244,
#340245,#340246),(#340247,#340248,#340249),(#340250,#340251,#340252),(#340253,
#340254,#340255),(#340256,#340257,#340258),(#340259,#340260,#340261),(#340262,
#340263,#340264),(#340265,#340266,#340267),(#340268,#340269,#340270),(#340271,
#340272,#340273),(#340274,#340275,#340276),(#340277,#340278,#340279),(#340280,
#340281,#340282),(#340283,#340284,#340285),(#340286,#340287,#340288),(#340289,
#340290,#340291),(#340292,#340293,#340294),(#340295,#340296,#340297),(#340298,
#340299,#340300),(#340301,#340302,#340303),(#340304,#340305,#340306),(#340307,
#340308,#340309),(#340310,#340311,#340312),(#340313,#340314,#340315),(#340316,
#340317,#340318),(#340319,#340320,#340321),(#340322,#340323,#340324),(#340325,
#340326,#340327),(#340328,#340329,#340330),(#340331,#340332,#340333),(#340334,
#340335,#340336),(#340337,#340338,#340339),(#340340,#340341,#340342),(#340343,
#340344,#340345),(#340346,#340347,#340348),(#340349,#340350,#340351),(#340352,
#340353,#340354),(#340355,#340356,#340357),(#340358,#340359,#340360),(#340361,
#340362,#340363),(#340364,#340365,#340366),(#340367,#340368,#340369),(#340370,
#340371,#340372),(#340373,#340374,#340375),(#340376,#340377,#340378),(#340379,
#340380,#340381),(#340382,#340383,#340384),(#340385,#340386,#340387),(#340388,
#340389,#340390),(#340391,#340392,#340393),(#340394,#340395,#340396),(#340397,
#340398,#340399),(#340400,#340401,#340402),(#340403,#340404,#340405),(#340406,
#340407,#340408),(#340409,#340410,#340411),(#340412,#340413,#340414),(#340415,
#340416,#340417),(#340418,#340419,#340420),(#340421,#340422,#340423),(#340424,
#340425,#340426),(#340427,#340428,#340429),(#340430,#340431,#340432),(#340433,
#340434,#340435),(#340436,#340437,#340438),(#340439,#340440,#340441),(#340442,
#340443,#340444),(#340445,#340446,#340447),(#340448,#340449,#340450),(#340451,
#340452,#340453),(#340454,#340455,#340456),(#340457,#340458,#340459),(#340460,
#340461,#340462),(#340463,#340464,#340465),(#340466,#340467,#340468),(#340469,
#340470,#340471),(#340472,#340473,#340474),(#340475,#340476,#340477),(#340478,
#340479,#340480),(#340481,#340482,#340483),(#340484,#340485,#340486),(#340487,
#340488,#340489),(#340490,#340491,#340492),(#340493,#340494,#340495),(#340496,
#340497,#340498),(#340499,#340500,#340501),(#340502,#340503,#340504),(#340505,
#340506,#340507),(#340508,#340509,#340510),(#340511,#340512,#340513),(#340514,
#340515,#340516),(#340517,#340518,#340519),(#340520,#340521,#340522),(#340523,
#340524,#340525),(#340526,#340527,#340528),(#340529,#340530,#340531),(#340532,
#340533,#340534),(#340535,#340536,#340537),(#340538,#340539,#340540),(#340541,
#340542,#340543),(#340544,#340545,#340546),(#340547,#340548,#340549),(#340550,
#340551,#340552),(#340553,#340554,#340555),(#340556,#340557,#340558),(#340559,
#340560,#340561),(#340562,#340563,#340564),(#340565,#340566,#340567),(#340568,
#340569,#340570),(#340571,#340572,#340573),(#340574,#340575,#340576),(#340577,
#340578,#340579),(#340580,#340581,#340582),(#340583,#340584,#340585),(#340586,
#340587,#340588),(#340589,#340590,#340591),(#340592,#340593,#340594),(#340595,
#340596,#340597),(#340598,#340599,#340600),(#340601,#340602,#340603),(#340604,
#340605,#340606),(#340607,#340608,#340609),(#340610,#340611,#340612),(#340613,
#340614,#340615),(#340616,#340617,#340618),(#340619,#340620,#340621),(#340622,
#340623,#340624),(#340625,#340626,#340627),(#340628,#340629,#340630),(#340631,
#340632,#340633),(#340634,#340635,#340636),(#340637,#340638,#340639),(#340640,
#340641,#340642),(#340643,#340644,#340645),(#340646,#340647,#340648),(#340649,
#340650,#340651),(#340652,#340653,#340654),(#340655,#340656,#340657),(#340658,
#340659,#340660),(#340661,#340662,#340663),(#340664,#340665,#340666),(#340667,
#340668,#340669),(#340670,#340671,#340672),(#340673,#340674,#340675),(#340676,
#340677,#340678),(#340679,#340680,#340681),(#340682,#340683,#340684),(#340685,
#340686,#340687),(#340688,#340689,#340690),(#340691,#340692,#340693),(#340694,
#340695,#340696),(#340697,#340698,#340699),(#340700,#340701,#340702),(#340703,
#340704,#340705),(#340706,#340707,#340708),(#340709,#340710,#340711),(#340712,
#340713,#340714),(#340715,#340716,#340717),(#340718,#340719,#340720),(#340721,
#340722,#340723),(#340724,#340725,#340726),(#340727,#340728,#340729),(#340730,
#340731,#340732),(#340733,#340734,#340735),(#340736,#340737,#340738),(#340739,
#340740,#340741),(#340742,#340743,#340744),(#340745,#340746,#340747),(#340748,
#340749,#340750),(#340751,#340752,#340753),(#340754,#340755,#340756),(#340757,
#340758,#340759),(#340760,#340761,#340762),(#340763,#340764,#340765),(#340766,
#340767,#340768),(#340769,#340770,#340771),(#340772,#340773,#340774),(#340775,
#340776,#340777),(#340778,#340779,#340780),(#340781,#340782,#340783),(#340784,
#340785,#340786),(#340787,#340788,#340789),(#340790,#340791,#340792),(#340793,
#340794,#340795),(#340796,#340797,#340798),(#340799,#340800,#340801),(#340802,
#340803,#340804),(#340805,#340806,#340807),(#340808,#340809,#340810),(#340811,
#340812,#340813),(#340814,#340815,#340816),(#340817,#340818,#340819),(#340820,
#340821,#340822),(#340823,#340824,#340825),(#340826,#340827,#340828),(#340829,
#340830,#340831),(#340832,#340833,#340834),(#340835,#340836,#340837),(#340838,
#340839,#340840),(#340841,#340842,#340843),(#340844,#340845,#340846),(#340847,
#340848,#340849),(#340850,#340851,#340852),(#340853,#340854,#340855),(#340856,
#340857,#340858),(#340859,#340860,#340861),(#340862,#340863,#340864),(#340865,
#340866,#340867),(#340868,#340869,#340870),(#340871,#340872,#340873),(#340874,
#340875,#340876),(#340877,#340878,#340879),(#340880,#340881,#340882),(#340883,
#340884,#340885),(#340886,#340887,#340888),(#340889,#340890,#340891),(#340892,
#340893,#340894),(#340895,#340896,#340897),(#340898,#340899,#340900),(#340901,
#340902,#340903),(#340904,#340905,#340906),(#340907,#340908,#340909),(#340910,
#340911,#340912),(#340913,#340914,#340915),(#340916,#340917,#340918),(#340919,
#340920,#340921),(#340922,#340923,#340924),(#340925,#340926,#340927),(#340928,
#340929,#340930),(#340931,#340932,#340933),(#340934,#340935,#340936),(#340937,
#340938,#340939),(#340940,#340941,#340942),(#340943,#340944,#340945),(#340946,
#340947,#340948),(#340949,#340950,#340951),(#340952,#340953,#340954),(#340955,
#340956,#340957),(#340958,#340959,#340960),(#340961,#340962,#340963),(#340964,
#340965,#340966),(#340967,#340968,#340969),(#340970,#340971,#340972),(#340973,
#340974,#340975),(#340976,#340977,#340978),(#340979,#340980,#340981),(#340982,
#340983,#340984),(#340985,#340986,#340987),(#340988,#340989,#340990),(#340991,
#340992,#340993),(#340994,#340995,#340996),(#340997,#340998,#340999),(#341000,
#341001,#341002),(#341003,#341004,#341005),(#341006,#341007,#341008),(#341009,
#341010,#341011),(#341012,#341013,#341014),(#341015,#341016,#341017),(#341018,
#341019,#341020),(#341021,#341022,#341023),(#341024,#341025,#341026),(#341027,
#341028,#341029),(#341030,#341031,#341032),(#341033,#341034,#341035),(#341036,
#341037,#341038),(#341039,#341040,#341041),(#341042,#341043,#341044),(#341045,
#341046,#341047),(#341048,#341049,#341050),(#341051,#341052,#341053),(#341054,
#341055,#341056),(#341057,#341058,#341059),(#341060,#341061,#341062),(#341063,
#341064,#341065),(#341066,#341067,#341068),(#341069,#341070,#341071),(#341072,
#341073,#341074),(#341075,#341076,#341077),(#341078,#341079,#341080),(#341081,
#341082,#341083),(#341084,#341085,#341086),(#341087,#341088,#341089),(#341090,
#341091,#341092),(#341093,#341094,#341095),(#341096,#341097,#341098),(#341099,
#341100,#341101),(#341102,#341103,#341104),(#341105,#341106,#341107),(#341108,
#341109,#341110),(#341111,#341112,#341113),(#341114,#341115,#341116),(#341117,
#341118,#341119),(#341120,#341121,#341122),(#341123,#341124,#341125),(#341126,
#341127,#341128),(#341129,#341130,#341131),(#341132,#341133,#341134),(#341135,
#341136,#341137),(#341138,#341139,#341140),(#341141,#341142,#341143),(#341144,
#341145,#341146),(#341147,#341148,#341149),(#341150,#341151,#341152),(#341153,
#341154,#341155),(#341156,#341157,#341158),(#341159,#341160,#341161),(#341162,
#341163,#341164),(#341165,#341166,#341167),(#341168,#341169,#341170),(#341171,
#341172,#341173),(#341174,#341175,#341176),(#341177,#341178,#341179),(#341180,
#341181,#341182),(#341183,#341184,#341185),(#341186,#341187,#341188),(#341189,
#341190,#341191),(#341192,#341193,#341194),(#341195,#341196,#341197),(#341198,
#341199,#341200),(#341201,#341202,#341203),(#341204,#341205,#341206),(#341207,
#341208,#341209),(#341210,#341211,#341212),(#341213,#341214,#341215),(#341216,
#341217,#341218),(#341219,#341220,#341221),(#341222,#341223,#341224),(#341225,
#341226,#341227),(#341228,#341229,#341230),(#341231,#341232,#341233),(#341234,
#341235,#341236),(#341237,#341238,#341239),(#341240,#341241,#341242),(#341243,
#341244,#341245),(#341246,#341247,#341248),(#341249,#341250,#341251),(#341252,
#341253,#341254),(#341255,#341256,#341257),(#341258,#341259,#341260),(#341261,
#341262,#341263),(#341264,#341265,#341266),(#341267,#341268,#341269),(#341270,
#341271,#341272),(#341273,#341274,#341275),(#341276,#341277,#341278),(#341279,
#341280,#341281),(#341282,#341283,#341284),(#341285,#341286,#341287),(#341288,
#341289,#341290),(#341291,#341292,#341293),(#341294,#341295,#341296),(#341297,
#341298,#341299),(#341300,#341301,#341302),(#341303,#341304,#341305),(#341306,
#341307,#341308),(#341309,#341310,#341311),(#341312,#341313,#341314),(#341315,
#341316,#341317),(#341318,#341319,#341320),(#341321,#341322,#341323),(#341324,
#341325,#341326),(#341327,#341328,#341329),(#341330,#341331,#341332),(#341333,
#341334,#341335),(#341336,#341337,#341338),(#341339,#341340,#341341),(#341342,
#341343,#341344),(#341345,#341346,#341347),(#341348,#341349,#341350),(#341351,
#341352,#341353),(#341354,#341355,#341356),(#341357,#341358,#341359),(#341360,
#341361,#341362),(#341363,#341364,#341365),(#341366,#341367,#341368),(#341369,
#341370,#341371),(#341372,#341373,#341374),(#341375,#341376,#341377),(#341378,
#341379,#341380),(#341381,#341382,#341383),(#341384,#341385,#341386),(#341387,
#341388,#341389),(#341390,#341391,#341392),(#341393,#341394,#341395),(#341396,
#341397,#341398),(#341399,#341400,#341401),(#341402,#341403,#341404),(#341405,
#341406,#341407),(#341408,#341409,#341410),(#341411,#341412,#341413),(#341414,
#341415,#341416),(#341417,#341418,#341419),(#341420,#341421,#341422),(#341423,
#341424,#341425),(#341426,#341427,#341428),(#341429,#341430,#341431),(#341432,
#341433,#341434),(#341435,#341436,#341437),(#341438,#341439,#341440),(#341441,
#341442,#341443),(#341444,#341445,#341446),(#341447,#341448,#341449),(#341450,
#341451,#341452),(#341453,#341454,#341455),(#341456,#341457,#341458),(#341459,
#341460,#341461),(#341462,#341463,#341464),(#341465,#341466,#341467),(#341468,
#341469,#341470),(#341471,#341472,#341473),(#341474,#341475,#341476),(#341477,
#341478,#341479),(#341480,#341481,#341482),(#341483,#341484,#341485),(#341486,
#341487,#341488),(#341489,#341490,#341491),(#341492,#341493,#341494),(#341495,
#341496,#341497),(#341498,#341499,#341500),(#341501,#341502,#341503),(#341504,
#341505,#341506),(#341507,#341508,#341509),(#341510,#341511,#341512),(#341513,
#341514,#341515),(#341516,#341517,#341518),(#341519,#341520,#341521),(#341522,
#341523,#341524),(#341525,#341526,#341527),(#341528,#341529,#341530),(#341531,
#341532,#341533),(#341534,#341535,#341536),(#341537,#341538,#341539),(#341540,
#341541,#341542),(#341543,#341544,#341545),(#341546,#341547,#341548),(#341549,
#341550,#341551),(#341552,#341553,#341554),(#341555,#341556,#341557),(#341558,
#341559,#341560),(#341561,#341562,#341563),(#341564,#341565,#341566),(#341567,
#341568,#341569),(#341570,#341571,#341572),(#341573,#341574,#341575),(#341576,
#341577,#341578),(#341579,#341580,#341581),(#341582,#341583,#341584),(#341585,
#341586,#341587)),.UNSPECIFIED.,.F.,.F.,.F.,(6,1,1,1,1,1,1,1,1,1,1,1,1,
1,1,1,1,1,1,1,1,1,1,1,1,1,1,1,1,1,1,1,1,1,1,1,1,1,1,1,1,1,1,1,1,1,1,1,1,
1,1,1,1,1,1,1,1,1,1,1,1,1,1,1,1,1,1,1,1,1,1,1,1,1,1,1,1,1,1,1,1,1,1,1,1,
1,1,1,1,1,1,1,1,1,1,1,1,1,1,1,1,1,1,1,1,1,1,1,1,1,1,1,1,1,1,1,1,1,1,1,1,
1,1,1,1,1,1,1,1,1,1,1,1,1,1,1,1,1,1,1,1,1,1,1,1,1,1,1,1,1,1,1,1,1,1,1,1,
1,1,1,1,1,1,1,1,1,1,1,1,1,1,1,1,1,1,1,1,1,1,1,1,1,1,1,1,1,1,1,1,1,1,1,1,
1,1,1,1,1,1,1,1,1,1,1,1,1,1,1,1,1,1,1,1,1,1,1,1,1,1,1,1,1,1,1,1,1,1,1,1,
1,1,1,1,1,1,1,1,1,1,1,1,1,1,1,1,1,1,1,1,1,1,1,1,1,1,1,1,1,1,1,1,1,1,1,1,
1,1,1,1,1,1,1,1,1,1,1,1,1,1,1,1,1,1,1,1,1,1,1,1,1,1,1,1,1,1,1,1,1,1,1,1,
1,1,1,1,1,1,1,1,1,1,1,1,1,1,1,1,1,1,1,1,1,1,1,1,1,1,1,1,1,1,1,1,1,1,1,1,
1,1,1,1,1,1,1,1,1,1,1,1,1,1,1,1,1,1,1,1,1,1,1,1,1,1,1,1,1,1,1,1,1,1,1,1,
1,1,1,1,1,1,1,1,1,1,1,1,1,1,1,1,1,1,1,1,1,1,1,1,1,1,1,1,1,1,1,1,1,1,1,1,
1,1,1,1,1,1,1,1,1,1,1,1,1,1,1,1,1,1,1,1,1,1,1,1,1,1,1,1,1,1,1,1,1,1,1,1,
1,1,1,1,1,1,1,1,1,1,1,1,1,1,1,1,1,1,1,1,1,1,1,1,1,1,1,1,1,1,1,1,1,1,1,1,
1,1,1,1,1,1,1,1,1,1,1,1,1,1,1,1,1,1,1,1,1,1,1,1,1,1,1,1,1,1,1,1,1,1,1,1,
1,1,1,1,1,1,1,1,1,1,1,1,1,1,1,1,1,1,1,1,1,1,1,1,1,1,1,1,1,6),(2,1,2),(-0.001964156,
0.,0.001834862,0.003669725,0.005504587,0.00733945,0.009174312,0.011009174,
0.012844037,0.014678899,0.016513761,0.018348624,0.020183486,0.022018349,
0.023853211,0.025688073,0.027522936,0.029357798,0.031192661,0.033027523,
0.034862385,0.036697248,0.03853211,0.040366972,0.042201835,0.044036697,
0.04587156,0.047706422,0.049541284,0.051376147,0.053211009,0.055045872,
0.056880734,0.058715596,0.060550459,0.062385321,0.064220183,0.066055046,
0.067889908,0.069724771,0.071559633,0.073394495,0.075229358,0.07706422,
0.078899083,0.080733945,0.082568807,0.08440367,0.086238532,0.088073394,
0.089908257,0.091743119,0.093577982,0.095412844,0.097247706,0.099082569,
0.100917431,0.102752294,0.104587156,0.106422018,0.108256881,0.110091743,
0.111926606,0.113761468,0.11559633,0.117431193,0.119266055,0.121100917,
0.12293578,0.124770642,0.126605505,0.128440367,0.130275229,0.132110092,
0.133944954,0.135779817,0.137614679,0.139449541,0.141284404,0.143119266,
0.144954128,0.146788991,0.148623853,0.150458716,0.152293578,0.15412844,
0.155963303,0.157798165,0.159633028,0.16146789,0.163302752,0.165137615,
0.166972477,0.168807339,0.170642202,0.172477064,0.174311927,0.176146789,
0.177981651,0.179816514,0.181651376,0.183486239,0.185321101,0.187155963,
0.188990826,0.190825688,0.19266055,0.194495413,0.196330275,0.198165138,
0.2,0.201834862,0.203669725,0.205504587,0.20733945,0.209174312,0.211009174,
0.212844037,0.214678899,0.216513761,0.218348624,0.220183486,0.222018349,
0.223853211,0.225688073,0.227522936,0.229357798,0.231192661,0.233027523,
0.234862385,0.236697248,0.23853211,0.240366972,0.242201835,0.244036697,
0.24587156,0.247706422,0.249541284,0.251376147,0.253211009,0.255045872,
0.256880734,0.258715596,0.260550459,0.262385321,0.264220183,0.266055046,
0.267889908,0.269724771,0.271559633,0.273394495,0.275229358,0.27706422,
0.278899083,0.280733945,0.282568807,0.28440367,0.286238532,0.288073394,
0.289908257,0.291743119,0.293577982,0.295412844,0.297247706,0.299082569,
0.300917431,0.302752294,0.304587156,0.306422018,0.308256881,0.310091743,
0.311926606,0.313761468,0.31559633,0.317431193,0.319266055,0.321100917,
0.32293578,0.324770642,0.326605505,0.328440367,0.330275229,0.332110092,
0.333944954,0.335779817,0.337614679,0.339449541,0.341284404,0.343119266,
0.344954128,0.346788991,0.348623853,0.350458716,0.352293578,0.35412844,
0.355963303,0.357798165,0.359633028,0.36146789,0.363302752,0.365137615,
0.366972477,0.368807339,0.370642202,0.372477064,0.374311927,0.376146789,
0.377981651,0.379816514,0.381651376,0.383486239,0.385321101,0.387155963,
0.388990826,0.390825688,0.39266055,0.394495413,0.396330275,0.398165138,
0.4,0.401834862,0.403669725,0.405504587,0.40733945,0.409174312,0.411009174,
0.412844037,0.414678899,0.416513761,0.418348624,0.420183486,0.422018349,
0.423853211,0.425688073,0.427522936,0.429357798,0.431192661,0.433027523,
0.434862385,0.436697248,0.43853211,0.440366972,0.442201835,0.444036697,
0.44587156,0.447706422,0.449541284,0.451376147,0.453211009,0.455045872,
0.456880734,0.458715596,0.460550459,0.462385321,0.464220183,0.466055046,
0.467889908,0.469724771,0.471559633,0.473394495,0.475229358,0.47706422,
0.478899083,0.480733945,0.482568807,0.48440367,0.486238532,0.488073394,
0.489908257,0.491743119,0.493577982,0.495412844,0.497247706,0.499082569,
0.500917431,0.502752294,0.504587156,0.506422018,0.508256881,0.510091743,
0.511926606,0.513761468,0.51559633,0.517431193,0.519266055,0.521100917,
0.52293578,0.524770642,0.526605505,0.528440367,0.530275229,0.532110092,
0.533944954,0.535779817,0.537614679,0.539449541,0.541284404,0.543119266,
0.544954128,0.546788991,0.548623853,0.550458716,0.552293578,0.55412844,
0.555963303,0.557798165,0.559633028,0.56146789,0.563302752,0.565137615,
0.566972477,0.568807339,0.570642202,0.572477064,0.574311927,0.576146789,
0.577981651,0.579816514,0.581651376,0.583486239,0.585321101,0.587155963,
0.588990826,0.590825688,0.59266055,0.594495413,0.596330275,0.598165138,
0.6,0.601834862,0.603669725,0.605504587,0.60733945,0.609174312,0.611009174,
0.612844037,0.614678899,0.616513761,0.618348624,0.620183486,0.622018349,
0.623853211,0.625688073,0.627522936,0.629357798,0.631192661,0.633027523,
0.634862385,0.636697248,0.63853211,0.640366972,0.642201835,0.644036697,
0.64587156,0.647706422,0.649541284,0.651376147,0.653211009,0.655045872,
0.656880734,0.658715596,0.660550459,0.662385321,0.664220183,0.666055046,
0.667889908,0.669724771,0.671559633,0.673394495,0.675229358,0.67706422,
0.678899083,0.680733945,0.682568807,0.68440367,0.686238532,0.688073394,
0.689908257,0.691743119,0.693577982,0.695412844,0.697247706,0.699082569,
0.700917431,0.702752294,0.704587156,0.706422018,0.708256881,0.710091743,
0.711926606,0.713761468,0.71559633,0.717431193,0.719266055,0.721100917,
0.72293578,0.724770642,0.726605505,0.728440367,0.730275229,0.732110092,
0.733944954,0.735779817,0.737614679,0.739449541,0.741284404,0.743119266,
0.744954128,0.746788991,0.748623853,0.750458716,0.752293578,0.75412844,
0.755963303,0.757798165,0.759633028,0.76146789,0.763302752,0.765137615,
0.766972477,0.768807339,0.770642202,0.772477064,0.774311927,0.776146789,
0.777981651,0.779816514,0.781651376,0.783486239,0.785321101,0.787155963,
0.788990826,0.790825688,0.79266055,0.794495413,0.796330275,0.798165138,
0.8,0.801834862,0.803669725,0.805504587,0.80733945,0.809174312,0.811009174,
0.812844037,0.814678899,0.816513761,0.818348624,0.820183486,0.822018349,
0.823853211,0.825688073,0.827522936,0.829357798,0.831192661,0.833027523,
0.834862385,0.836697248,0.83853211,0.840366972,0.842201835,0.844036697,
0.84587156,0.847706422,0.849541284,0.851376147,0.853211009,0.855045872,
0.856880734,0.858715596,0.860550459,0.862385321,0.864220183,0.866055046,
0.867889908,0.869724771,0.871559633,0.873394495,0.875229358,0.87706422,
0.878899083,0.880733945,0.882568807,0.88440367,0.886238532,0.888073394,
0.889908257,0.891743119,0.893577982,0.895412844,0.897247706,0.899082569,
0.900917431,0.902752294,0.904587156,0.906422018,0.908256881,0.910091743,
0.911926606,0.913761468,0.91559633,0.917431193,0.919266055,0.921100917,
0.92293578,0.924770642,0.926605505,0.928440367,0.930275229,0.932110092,
0.933944954,0.935779817,0.937614679,0.939449541,0.941284404,0.943119266,
0.944954128,0.946788991,0.948623853,0.950458716,0.952293578,0.95412844,
0.955963303,0.957798165,0.959633028,0.96146789,0.963302752,0.965137615,
0.966972477,0.968807339,0.970642202,0.972477064,0.974311927,0.976146789,
0.977981651,0.979816514,0.981651376,0.983486239,0.985321101,0.987155963,
0.988990826,0.990825688,0.99266055,0.994495413,0.996330275,0.998165138,
1.000000000441),(0.3,1.,1.3),.UNSPECIFIED.);
#6327=B_SPLINE_SURFACE_WITH_KNOTS('',5,1,((#341592,#341593,#341594),(#341595,
#341596,#341597),(#341598,#341599,#341600),(#341601,#341602,#341603),(#341604,
#341605,#341606),(#341607,#341608,#341609),(#341610,#341611,#341612),(#341613,
#341614,#341615),(#341616,#341617,#341618),(#341619,#341620,#341621),(#341622,
#341623,#341624),(#341625,#341626,#341627),(#341628,#341629,#341630),(#341631,
#341632,#341633),(#341634,#341635,#341636),(#341637,#341638,#341639),(#341640,
#341641,#341642),(#341643,#341644,#341645),(#341646,#341647,#341648),(#341649,
#341650,#341651),(#341652,#341653,#341654),(#341655,#341656,#341657),(#341658,
#341659,#341660),(#341661,#341662,#341663),(#341664,#341665,#341666),(#341667,
#341668,#341669),(#341670,#341671,#341672),(#341673,#341674,#341675),(#341676,
#341677,#341678),(#341679,#341680,#341681),(#341682,#341683,#341684),(#341685,
#341686,#341687),(#341688,#341689,#341690),(#341691,#341692,#341693),(#341694,
#341695,#341696),(#341697,#341698,#341699),(#341700,#341701,#341702),(#341703,
#341704,#341705),(#341706,#341707,#341708),(#341709,#341710,#341711),(#341712,
#341713,#341714),(#341715,#341716,#341717),(#341718,#341719,#341720),(#341721,
#341722,#341723),(#341724,#341725,#341726),(#341727,#341728,#341729),(#341730,
#341731,#341732),(#341733,#341734,#341735),(#341736,#341737,#341738),(#341739,
#341740,#341741),(#341742,#341743,#341744),(#341745,#341746,#341747),(#341748,
#341749,#341750),(#341751,#341752,#341753),(#341754,#341755,#341756),(#341757,
#341758,#341759),(#341760,#341761,#341762),(#341763,#341764,#341765),(#341766,
#341767,#341768),(#341769,#341770,#341771),(#341772,#341773,#341774),(#341775,
#341776,#341777),(#341778,#341779,#341780),(#341781,#341782,#341783),(#341784,
#341785,#341786),(#341787,#341788,#341789),(#341790,#341791,#341792),(#341793,
#341794,#341795),(#341796,#341797,#341798),(#341799,#341800,#341801),(#341802,
#341803,#341804),(#341805,#341806,#341807),(#341808,#341809,#341810),(#341811,
#341812,#341813),(#341814,#341815,#341816),(#341817,#341818,#341819),(#341820,
#341821,#341822),(#341823,#341824,#341825),(#341826,#341827,#341828),(#341829,
#341830,#341831),(#341832,#341833,#341834),(#341835,#341836,#341837),(#341838,
#341839,#341840),(#341841,#341842,#341843),(#341844,#341845,#341846),(#341847,
#341848,#341849),(#341850,#341851,#341852),(#341853,#341854,#341855),(#341856,
#341857,#341858),(#341859,#341860,#341861),(#341862,#341863,#341864),(#341865,
#341866,#341867),(#341868,#341869,#341870),(#341871,#341872,#341873),(#341874,
#341875,#341876),(#341877,#341878,#341879),(#341880,#341881,#341882),(#341883,
#341884,#341885),(#341886,#341887,#341888),(#341889,#341890,#341891),(#341892,
#341893,#341894),(#341895,#341896,#341897),(#341898,#341899,#341900),(#341901,
#341902,#341903),(#341904,#341905,#341906),(#341907,#341908,#341909),(#341910,
#341911,#341912),(#341913,#341914,#341915),(#341916,#341917,#341918),(#341919,
#341920,#341921),(#341922,#341923,#341924),(#341925,#341926,#341927),(#341928,
#341929,#341930),(#341931,#341932,#341933),(#341934,#341935,#341936),(#341937,
#341938,#341939),(#341940,#341941,#341942),(#341943,#341944,#341945),(#341946,
#341947,#341948),(#341949,#341950,#341951),(#341952,#341953,#341954),(#341955,
#341956,#341957),(#341958,#341959,#341960),(#341961,#341962,#341963),(#341964,
#341965,#341966),(#341967,#341968,#341969),(#341970,#341971,#341972),(#341973,
#341974,#341975),(#341976,#341977,#341978),(#341979,#341980,#341981),(#341982,
#341983,#341984),(#341985,#341986,#341987),(#341988,#341989,#341990),(#341991,
#341992,#341993),(#341994,#341995,#341996),(#341997,#341998,#341999),(#342000,
#342001,#342002),(#342003,#342004,#342005),(#342006,#342007,#342008),(#342009,
#342010,#342011),(#342012,#342013,#342014),(#342015,#342016,#342017),(#342018,
#342019,#342020),(#342021,#342022,#342023),(#342024,#342025,#342026),(#342027,
#342028,#342029),(#342030,#342031,#342032),(#342033,#342034,#342035),(#342036,
#342037,#342038),(#342039,#342040,#342041),(#342042,#342043,#342044),(#342045,
#342046,#342047),(#342048,#342049,#342050),(#342051,#342052,#342053),(#342054,
#342055,#342056),(#342057,#342058,#342059),(#342060,#342061,#342062),(#342063,
#342064,#342065),(#342066,#342067,#342068),(#342069,#342070,#342071),(#342072,
#342073,#342074),(#342075,#342076,#342077),(#342078,#342079,#342080),(#342081,
#342082,#342083),(#342084,#342085,#342086),(#342087,#342088,#342089),(#342090,
#342091,#342092),(#342093,#342094,#342095),(#342096,#342097,#342098),(#342099,
#342100,#342101),(#342102,#342103,#342104),(#342105,#342106,#342107),(#342108,
#342109,#342110),(#342111,#342112,#342113),(#342114,#342115,#342116),(#342117,
#342118,#342119),(#342120,#342121,#342122),(#342123,#342124,#342125),(#342126,
#342127,#342128),(#342129,#342130,#342131),(#342132,#342133,#342134),(#342135,
#342136,#342137),(#342138,#342139,#342140),(#342141,#342142,#342143),(#342144,
#342145,#342146),(#342147,#342148,#342149),(#342150,#342151,#342152),(#342153,
#342154,#342155),(#342156,#342157,#342158),(#342159,#342160,#342161),(#342162,
#342163,#342164),(#342165,#342166,#342167),(#342168,#342169,#342170),(#342171,
#342172,#342173),(#342174,#342175,#342176),(#342177,#342178,#342179),(#342180,
#342181,#342182),(#342183,#342184,#342185),(#342186,#342187,#342188),(#342189,
#342190,#342191),(#342192,#342193,#342194),(#342195,#342196,#342197),(#342198,
#342199,#342200),(#342201,#342202,#342203),(#342204,#342205,#342206),(#342207,
#342208,#342209),(#342210,#342211,#342212),(#342213,#342214,#342215),(#342216,
#342217,#342218),(#342219,#342220,#342221),(#342222,#342223,#342224),(#342225,
#342226,#342227),(#342228,#342229,#342230),(#342231,#342232,#342233),(#342234,
#342235,#342236),(#342237,#342238,#342239),(#342240,#342241,#342242),(#342243,
#342244,#342245),(#342246,#342247,#342248),(#342249,#342250,#342251),(#342252,
#342253,#342254),(#342255,#342256,#342257),(#342258,#342259,#342260),(#342261,
#342262,#342263),(#342264,#342265,#342266),(#342267,#342268,#342269),(#342270,
#342271,#342272),(#342273,#342274,#342275),(#342276,#342277,#342278),(#342279,
#342280,#342281),(#342282,#342283,#342284),(#342285,#342286,#342287),(#342288,
#342289,#342290),(#342291,#342292,#342293),(#342294,#342295,#342296),(#342297,
#342298,#342299),(#342300,#342301,#342302),(#342303,#342304,#342305),(#342306,
#342307,#342308),(#342309,#342310,#342311),(#342312,#342313,#342314),(#342315,
#342316,#342317),(#342318,#342319,#342320),(#342321,#342322,#342323),(#342324,
#342325,#342326),(#342327,#342328,#342329),(#342330,#342331,#342332),(#342333,
#342334,#342335),(#342336,#342337,#342338),(#342339,#342340,#342341),(#342342,
#342343,#342344),(#342345,#342346,#342347),(#342348,#342349,#342350),(#342351,
#342352,#342353),(#342354,#342355,#342356),(#342357,#342358,#342359),(#342360,
#342361,#342362),(#342363,#342364,#342365),(#342366,#342367,#342368),(#342369,
#342370,#342371),(#342372,#342373,#342374),(#342375,#342376,#342377),(#342378,
#342379,#342380),(#342381,#342382,#342383),(#342384,#342385,#342386),(#342387,
#342388,#342389),(#342390,#342391,#342392),(#342393,#342394,#342395),(#342396,
#342397,#342398),(#342399,#342400,#342401),(#342402,#342403,#342404),(#342405,
#342406,#342407),(#342408,#342409,#342410),(#342411,#342412,#342413),(#342414,
#342415,#342416),(#342417,#342418,#342419),(#342420,#342421,#342422),(#342423,
#342424,#342425),(#342426,#342427,#342428),(#342429,#342430,#342431),(#342432,
#342433,#342434),(#342435,#342436,#342437),(#342438,#342439,#342440),(#342441,
#342442,#342443),(#342444,#342445,#342446),(#342447,#342448,#342449),(#342450,
#342451,#342452),(#342453,#342454,#342455),(#342456,#342457,#342458),(#342459,
#342460,#342461),(#342462,#342463,#342464),(#342465,#342466,#342467),(#342468,
#342469,#342470),(#342471,#342472,#342473),(#342474,#342475,#342476),(#342477,
#342478,#342479),(#342480,#342481,#342482),(#342483,#342484,#342485),(#342486,
#342487,#342488),(#342489,#342490,#342491),(#342492,#342493,#342494),(#342495,
#342496,#342497),(#342498,#342499,#342500),(#342501,#342502,#342503),(#342504,
#342505,#342506),(#342507,#342508,#342509),(#342510,#342511,#342512),(#342513,
#342514,#342515),(#342516,#342517,#342518),(#342519,#342520,#342521),(#342522,
#342523,#342524),(#342525,#342526,#342527),(#342528,#342529,#342530),(#342531,
#342532,#342533),(#342534,#342535,#342536),(#342537,#342538,#342539),(#342540,
#342541,#342542),(#342543,#342544,#342545),(#342546,#342547,#342548),(#342549,
#342550,#342551),(#342552,#342553,#342554),(#342555,#342556,#342557),(#342558,
#342559,#342560),(#342561,#342562,#342563),(#342564,#342565,#342566),(#342567,
#342568,#342569),(#342570,#342571,#342572),(#342573,#342574,#342575),(#342576,
#342577,#342578),(#342579,#342580,#342581),(#342582,#342583,#342584),(#342585,
#342586,#342587),(#342588,#342589,#342590),(#342591,#342592,#342593),(#342594,
#342595,#342596),(#342597,#342598,#342599),(#342600,#342601,#342602),(#342603,
#342604,#342605),(#342606,#342607,#342608),(#342609,#342610,#342611),(#342612,
#342613,#342614),(#342615,#342616,#342617),(#342618,#342619,#342620),(#342621,
#342622,#342623),(#342624,#342625,#342626),(#342627,#342628,#342629),(#342630,
#342631,#342632),(#342633,#342634,#342635),(#342636,#342637,#342638),(#342639,
#342640,#342641),(#342642,#342643,#342644),(#342645,#342646,#342647),(#342648,
#342649,#342650),(#342651,#342652,#342653),(#342654,#342655,#342656),(#342657,
#342658,#342659),(#342660,#342661,#342662),(#342663,#342664,#342665),(#342666,
#342667,#342668),(#342669,#342670,#342671),(#342672,#342673,#342674),(#342675,
#342676,#342677),(#342678,#342679,#342680),(#342681,#342682,#342683),(#342684,
#342685,#342686),(#342687,#342688,#342689),(#342690,#342691,#342692),(#342693,
#342694,#342695),(#342696,#342697,#342698),(#342699,#342700,#342701),(#342702,
#342703,#342704),(#342705,#342706,#342707),(#342708,#342709,#342710),(#342711,
#342712,#342713),(#342714,#342715,#342716),(#342717,#342718,#342719),(#342720,
#342721,#342722),(#342723,#342724,#342725),(#342726,#342727,#342728),(#342729,
#342730,#342731),(#342732,#342733,#342734),(#342735,#342736,#342737),(#342738,
#342739,#342740),(#342741,#342742,#342743),(#342744,#342745,#342746),(#342747,
#342748,#342749),(#342750,#342751,#342752),(#342753,#342754,#342755),(#342756,
#342757,#342758),(#342759,#342760,#342761),(#342762,#342763,#342764),(#342765,
#342766,#342767),(#342768,#342769,#342770),(#342771,#342772,#342773),(#342774,
#342775,#342776),(#342777,#342778,#342779),(#342780,#342781,#342782),(#342783,
#342784,#342785),(#342786,#342787,#342788),(#342789,#342790,#342791),(#342792,
#342793,#342794),(#342795,#342796,#342797),(#342798,#342799,#342800),(#342801,
#342802,#342803),(#342804,#342805,#342806),(#342807,#342808,#342809),(#342810,
#342811,#342812),(#342813,#342814,#342815),(#342816,#342817,#342818),(#342819,
#342820,#342821),(#342822,#342823,#342824),(#342825,#342826,#342827),(#342828,
#342829,#342830),(#342831,#342832,#342833),(#342834,#342835,#342836),(#342837,
#342838,#342839),(#342840,#342841,#342842),(#342843,#342844,#342845),(#342846,
#342847,#342848),(#342849,#342850,#342851),(#342852,#342853,#342854),(#342855,
#342856,#342857),(#342858,#342859,#342860),(#342861,#342862,#342863),(#342864,
#342865,#342866),(#342867,#342868,#342869),(#342870,#342871,#342872),(#342873,
#342874,#342875),(#342876,#342877,#342878),(#342879,#342880,#342881),(#342882,
#342883,#342884),(#342885,#342886,#342887),(#342888,#342889,#342890),(#342891,
#342892,#342893),(#342894,#342895,#342896),(#342897,#342898,#342899),(#342900,
#342901,#342902),(#342903,#342904,#342905),(#342906,#342907,#342908),(#342909,
#342910,#342911),(#342912,#342913,#342914),(#342915,#342916,#342917),(#342918,
#342919,#342920),(#342921,#342922,#342923),(#342924,#342925,#342926),(#342927,
#342928,#342929),(#342930,#342931,#342932),(#342933,#342934,#342935),(#342936,
#342937,#342938),(#342939,#342940,#342941),(#342942,#342943,#342944),(#342945,
#342946,#342947),(#342948,#342949,#342950),(#342951,#342952,#342953),(#342954,
#342955,#342956),(#342957,#342958,#342959),(#342960,#342961,#342962),(#342963,
#342964,#342965),(#342966,#342967,#342968),(#342969,#342970,#342971),(#342972,
#342973,#342974),(#342975,#342976,#342977),(#342978,#342979,#342980),(#342981,
#342982,#342983),(#342984,#342985,#342986),(#342987,#342988,#342989),(#342990,
#342991,#342992),(#342993,#342994,#342995),(#342996,#342997,#342998),(#342999,
#343000,#343001),(#343002,#343003,#343004),(#343005,#343006,#343007),(#343008,
#343009,#343010),(#343011,#343012,#343013),(#343014,#343015,#343016),(#343017,
#343018,#343019),(#343020,#343021,#343022),(#343023,#343024,#343025),(#343026,
#343027,#343028),(#343029,#343030,#343031),(#343032,#343033,#343034),(#343035,
#343036,#343037),(#343038,#343039,#343040),(#343041,#343042,#343043),(#343044,
#343045,#343046),(#343047,#343048,#343049),(#343050,#343051,#343052),(#343053,
#343054,#343055),(#343056,#343057,#343058),(#343059,#343060,#343061),(#343062,
#343063,#343064),(#343065,#343066,#343067),(#343068,#343069,#343070),(#343071,
#343072,#343073),(#343074,#343075,#343076),(#343077,#343078,#343079),(#343080,
#343081,#343082),(#343083,#343084,#343085),(#343086,#343087,#343088),(#343089,
#343090,#343091),(#343092,#343093,#343094),(#343095,#343096,#343097),(#343098,
#343099,#343100),(#343101,#343102,#343103),(#343104,#343105,#343106),(#343107,
#343108,#343109),(#343110,#343111,#343112),(#343113,#343114,#343115),(#343116,
#343117,#343118),(#343119,#343120,#343121),(#343122,#343123,#343124),(#343125,
#343126,#343127),(#343128,#343129,#343130),(#343131,#343132,#343133),(#343134,
#343135,#343136),(#343137,#343138,#343139),(#343140,#343141,#343142),(#343143,
#343144,#343145),(#343146,#343147,#343148),(#343149,#343150,#343151),(#343152,
#343153,#343154),(#343155,#343156,#343157),(#343158,#343159,#343160),(#343161,
#343162,#343163),(#343164,#343165,#343166),(#343167,#343168,#343169),(#343170,
#343171,#343172),(#343173,#343174,#343175),(#343176,#343177,#343178),(#343179,
#343180,#343181),(#343182,#343183,#343184),(#343185,#343186,#343187),(#343188,
#343189,#343190),(#343191,#343192,#343193),(#343194,#343195,#343196),(#343197,
#343198,#343199),(#343200,#343201,#343202),(#343203,#343204,#343205),(#343206,
#343207,#343208),(#343209,#343210,#343211),(#343212,#343213,#343214),(#343215,
#343216,#343217),(#343218,#343219,#343220),(#343221,#343222,#343223),(#343224,
#343225,#343226),(#343227,#343228,#343229),(#343230,#343231,#343232),(#343233,
#343234,#343235),(#343236,#343237,#343238),(#343239,#343240,#343241)),
 .UNSPECIFIED.,.F.,.F.,.F.,(6,1,1,1,1,1,1,1,1,1,1,1,1,1,1,1,1,1,1,1,1,1,
1,1,1,1,1,1,1,1,1,1,1,1,1,1,1,1,1,1,1,1,1,1,1,1,1,1,1,1,1,1,1,1,1,1,1,1,
1,1,1,1,1,1,1,1,1,1,1,1,1,1,1,1,1,1,1,1,1,1,1,1,1,1,1,1,1,1,1,1,1,1,1,1,
1,1,1,1,1,1,1,1,1,1,1,1,1,1,1,1,1,1,1,1,1,1,1,1,1,1,1,1,1,1,1,1,1,1,1,1,
1,1,1,1,1,1,1,1,1,1,1,1,1,1,1,1,1,1,1,1,1,1,1,1,1,1,1,1,1,1,1,1,1,1,1,1,
1,1,1,1,1,1,1,1,1,1,1,1,1,1,1,1,1,1,1,1,1,1,1,1,1,1,1,1,1,1,1,1,1,1,1,1,
1,1,1,1,1,1,1,1,1,1,1,1,1,1,1,1,1,1,1,1,1,1,1,1,1,1,1,1,1,1,1,1,1,1,1,1,
1,1,1,1,1,1,1,1,1,1,1,1,1,1,1,1,1,1,1,1,1,1,1,1,1,1,1,1,1,1,1,1,1,1,1,1,
1,1,1,1,1,1,1,1,1,1,1,1,1,1,1,1,1,1,1,1,1,1,1,1,1,1,1,1,1,1,1,1,1,1,1,1,
1,1,1,1,1,1,1,1,1,1,1,1,1,1,1,1,1,1,1,1,1,1,1,1,1,1,1,1,1,1,1,1,1,1,1,1,
1,1,1,1,1,1,1,1,1,1,1,1,1,1,1,1,1,1,1,1,1,1,1,1,1,1,1,1,1,1,1,1,1,1,1,1,
1,1,1,1,1,1,1,1,1,1,1,1,1,1,1,1,1,1,1,1,1,1,1,1,1,1,1,1,1,1,1,1,1,1,1,1,
1,1,1,1,1,1,1,1,1,1,1,1,1,1,1,1,1,1,1,1,1,1,1,1,1,1,1,1,1,1,1,1,1,1,1,1,
1,1,1,1,1,1,1,1,1,1,1,1,1,1,1,1,1,1,1,1,1,1,1,1,1,1,1,1,1,1,1,1,1,1,1,1,
1,1,1,1,1,1,1,1,1,1,1,1,1,1,1,1,1,1,1,1,1,1,1,1,1,1,1,1,1,1,1,1,1,1,1,1,
1,1,1,1,1,1,1,1,1,1,1,1,1,1,1,1,1,1,1,6),(2,1,2),(-1.,-0.998165138,-0.996330275,
-0.994495413,-0.99266055,-0.990825688,-0.988990826,-0.987155963,-0.985321101,
-0.983486239,-0.981651376,-0.979816514,-0.977981651,-0.976146789,-0.974311927,
-0.972477064,-0.970642202,-0.968807339,-0.966972477,-0.965137615,-0.963302752,
-0.96146789,-0.959633028,-0.957798165,-0.955963303,-0.95412844,-0.952293578,
-0.950458716,-0.948623853,-0.946788991,-0.944954128,-0.943119266,-0.941284404,
-0.939449541,-0.937614679,-0.935779817,-0.933944954,-0.932110092,-0.930275229,
-0.928440367,-0.926605505,-0.924770642,-0.92293578,-0.921100917,-0.919266055,
-0.917431193,-0.91559633,-0.913761468,-0.911926606,-0.910091743,-0.908256881,
-0.906422018,-0.904587156,-0.902752294,-0.900917431,-0.899082569,-0.897247706,
-0.895412844,-0.893577982,-0.891743119,-0.889908257,-0.888073394,-0.886238532,
-0.88440367,-0.882568807,-0.880733945,-0.878899083,-0.87706422,-0.875229358,
-0.873394495,-0.871559633,-0.869724771,-0.867889908,-0.866055046,-0.864220183,
-0.862385321,-0.860550459,-0.858715596,-0.856880734,-0.855045872,-0.853211009,
-0.851376147,-0.849541284,-0.847706422,-0.84587156,-0.844036697,-0.842201835,
-0.840366972,-0.83853211,-0.836697248,-0.834862385,-0.833027523,-0.831192661,
-0.829357798,-0.827522936,-0.825688073,-0.823853211,-0.822018349,-0.820183486,
-0.818348624,-0.816513761,-0.814678899,-0.812844037,-0.811009174,-0.809174312,
-0.80733945,-0.805504587,-0.803669725,-0.801834862,-0.8,-0.798165138,-0.796330275,
-0.794495413,-0.79266055,-0.790825688,-0.788990826,-0.787155963,-0.785321101,
-0.783486239,-0.781651376,-0.779816514,-0.777981651,-0.776146789,-0.774311927,
-0.772477064,-0.770642202,-0.768807339,-0.766972477,-0.765137615,-0.763302752,
-0.76146789,-0.759633028,-0.757798165,-0.755963303,-0.75412844,-0.752293578,
-0.750458716,-0.748623853,-0.746788991,-0.744954128,-0.743119266,-0.741284404,
-0.739449541,-0.737614679,-0.735779817,-0.733944954,-0.732110092,-0.730275229,
-0.728440367,-0.726605505,-0.724770642,-0.72293578,-0.721100917,-0.719266055,
-0.717431193,-0.71559633,-0.713761468,-0.711926606,-0.710091743,-0.708256881,
-0.706422018,-0.704587156,-0.702752294,-0.700917431,-0.699082569,-0.697247706,
-0.695412844,-0.693577982,-0.691743119,-0.689908257,-0.688073394,-0.686238532,
-0.68440367,-0.682568807,-0.680733945,-0.678899083,-0.67706422,-0.675229358,
-0.673394495,-0.671559633,-0.669724771,-0.667889908,-0.666055046,-0.664220183,
-0.662385321,-0.660550459,-0.658715596,-0.656880734,-0.655045872,-0.653211009,
-0.651376147,-0.649541284,-0.647706422,-0.64587156,-0.644036697,-0.642201835,
-0.640366972,-0.63853211,-0.636697248,-0.634862385,-0.633027523,-0.631192661,
-0.629357798,-0.627522936,-0.625688073,-0.623853211,-0.622018349,-0.620183486,
-0.618348624,-0.616513761,-0.614678899,-0.612844037,-0.611009174,-0.609174312,
-0.60733945,-0.605504587,-0.603669725,-0.601834862,-0.6,-0.598165138,-0.596330275,
-0.594495413,-0.59266055,-0.590825688,-0.588990826,-0.587155963,-0.585321101,
-0.583486239,-0.581651376,-0.579816514,-0.577981651,-0.576146789,-0.574311927,
-0.572477064,-0.570642202,-0.568807339,-0.566972477,-0.565137615,-0.563302752,
-0.56146789,-0.559633028,-0.557798165,-0.555963303,-0.55412844,-0.552293578,
-0.550458716,-0.548623853,-0.546788991,-0.544954128,-0.543119266,-0.541284404,
-0.539449541,-0.537614679,-0.535779817,-0.533944954,-0.532110092,-0.530275229,
-0.528440367,-0.526605505,-0.524770642,-0.52293578,-0.521100917,-0.519266055,
-0.517431193,-0.51559633,-0.513761468,-0.511926606,-0.510091743,-0.508256881,
-0.506422018,-0.504587156,-0.502752294,-0.500917431,-0.499082569,-0.497247706,
-0.495412844,-0.493577982,-0.491743119,-0.489908257,-0.488073394,-0.486238532,
-0.48440367,-0.482568807,-0.480733945,-0.478899083,-0.47706422,-0.475229358,
-0.473394495,-0.471559633,-0.469724771,-0.467889908,-0.466055046,-0.464220183,
-0.462385321,-0.460550459,-0.458715596,-0.456880734,-0.455045872,-0.453211009,
-0.451376147,-0.449541284,-0.447706422,-0.44587156,-0.444036697,-0.442201835,
-0.440366972,-0.43853211,-0.436697248,-0.434862385,-0.433027523,-0.431192661,
-0.429357798,-0.427522936,-0.425688073,-0.423853211,-0.422018349,-0.420183486,
-0.418348624,-0.416513761,-0.414678899,-0.412844037,-0.411009174,-0.409174312,
-0.40733945,-0.405504587,-0.403669725,-0.401834862,-0.4,-0.398165138,-0.396330275,
-0.394495413,-0.39266055,-0.390825688,-0.388990826,-0.387155963,-0.385321101,
-0.383486239,-0.381651376,-0.379816514,-0.377981651,-0.376146789,-0.374311927,
-0.372477064,-0.370642202,-0.368807339,-0.366972477,-0.365137615,-0.363302752,
-0.36146789,-0.359633028,-0.357798165,-0.355963303,-0.35412844,-0.352293578,
-0.350458716,-0.348623853,-0.346788991,-0.344954128,-0.343119266,-0.341284404,
-0.339449541,-0.337614679,-0.335779817,-0.333944954,-0.332110092,-0.330275229,
-0.328440367,-0.326605505,-0.324770642,-0.32293578,-0.321100917,-0.319266055,
-0.317431193,-0.31559633,-0.313761468,-0.311926606,-0.310091743,-0.308256881,
-0.306422018,-0.304587156,-0.302752294,-0.300917431,-0.299082569,-0.297247706,
-0.295412844,-0.293577982,-0.291743119,-0.289908257,-0.288073394,-0.286238532,
-0.28440367,-0.282568807,-0.280733945,-0.278899083,-0.27706422,-0.275229358,
-0.273394495,-0.271559633,-0.269724771,-0.267889908,-0.266055046,-0.264220183,
-0.262385321,-0.260550459,-0.258715596,-0.256880734,-0.255045872,-0.253211009,
-0.251376147,-0.249541284,-0.247706422,-0.24587156,-0.244036697,-0.242201835,
-0.240366972,-0.23853211,-0.236697248,-0.234862385,-0.233027523,-0.231192661,
-0.229357798,-0.227522936,-0.225688073,-0.223853211,-0.222018349,-0.220183486,
-0.218348624,-0.216513761,-0.214678899,-0.212844037,-0.211009174,-0.209174312,
-0.20733945,-0.205504587,-0.203669725,-0.201834862,-0.2,-0.198165138,-0.196330275,
-0.194495413,-0.19266055,-0.190825688,-0.188990826,-0.187155963,-0.185321101,
-0.183486239,-0.181651376,-0.179816514,-0.177981651,-0.176146789,-0.174311927,
-0.172477064,-0.170642202,-0.168807339,-0.166972477,-0.165137615,-0.163302752,
-0.16146789,-0.159633028,-0.157798165,-0.155963303,-0.15412844,-0.152293578,
-0.150458716,-0.148623853,-0.146788991,-0.144954128,-0.143119266,-0.141284404,
-0.139449541,-0.137614679,-0.135779817,-0.133944954,-0.132110092,-0.130275229,
-0.128440367,-0.126605505,-0.124770642,-0.12293578,-0.121100917,-0.119266055,
-0.117431193,-0.11559633,-0.113761468,-0.111926606,-0.110091743,-0.108256881,
-0.106422018,-0.104587156,-0.102752294,-0.100917431,-0.099082569,-0.097247706,
-0.095412844,-0.093577982,-0.091743119,-0.089908257,-0.088073394,-0.086238532,
-0.08440367,-0.082568807,-0.080733945,-0.078899083,-0.07706422,-0.075229358,
-0.073394495,-0.071559633,-0.069724771,-0.067889908,-0.066055046,-0.064220183,
-0.062385321,-0.060550459,-0.058715596,-0.056880734,-0.055045872,-0.053211009,
-0.051376147,-0.049541284,-0.047706422,-0.04587156,-0.044036697,-0.042201835,
-0.040366972,-0.03853211,-0.036697248,-0.034862385,-0.033027523,-0.031192661,
-0.029357798,-0.027522936,-0.025688073,-0.023853211,-0.022018349,-0.020183486,
-0.018348624,-0.016513761,-0.014678899,-0.012844037,-0.011009174,-0.009174312,
-0.00733945,-0.005504587,-0.003669725,-0.001834862,0.),(0.3,1.,1.3),
 .UNSPECIFIED.);
#6328=B_SPLINE_SURFACE_WITH_KNOTS('',5,1,((#343245,#343246,#343247),(#343248,
#343249,#343250),(#343251,#343252,#343253),(#343254,#343255,#343256),(#343257,
#343258,#343259),(#343260,#343261,#343262),(#343263,#343264,#343265),(#343266,
#343267,#343268),(#343269,#343270,#343271),(#343272,#343273,#343274),(#343275,
#343276,#343277),(#343278,#343279,#343280),(#343281,#343282,#343283),(#343284,
#343285,#343286),(#343287,#343288,#343289),(#343290,#343291,#343292),(#343293,
#343294,#343295),(#343296,#343297,#343298),(#343299,#343300,#343301),(#343302,
#343303,#343304),(#343305,#343306,#343307),(#343308,#343309,#343310),(#343311,
#343312,#343313),(#343314,#343315,#343316),(#343317,#343318,#343319),(#343320,
#343321,#343322),(#343323,#343324,#343325),(#343326,#343327,#343328),(#343329,
#343330,#343331),(#343332,#343333,#343334),(#343335,#343336,#343337),(#343338,
#343339,#343340),(#343341,#343342,#343343),(#343344,#343345,#343346),(#343347,
#343348,#343349),(#343350,#343351,#343352),(#343353,#343354,#343355),(#343356,
#343357,#343358),(#343359,#343360,#343361),(#343362,#343363,#343364),(#343365,
#343366,#343367),(#343368,#343369,#343370),(#343371,#343372,#343373),(#343374,
#343375,#343376),(#343377,#343378,#343379),(#343380,#343381,#343382),(#343383,
#343384,#343385),(#343386,#343387,#343388),(#343389,#343390,#343391),(#343392,
#343393,#343394),(#343395,#343396,#343397),(#343398,#343399,#343400),(#343401,
#343402,#343403),(#343404,#343405,#343406),(#343407,#343408,#343409),(#343410,
#343411,#343412),(#343413,#343414,#343415),(#343416,#343417,#343418),(#343419,
#343420,#343421),(#343422,#343423,#343424),(#343425,#343426,#343427),(#343428,
#343429,#343430),(#343431,#343432,#343433),(#343434,#343435,#343436),(#343437,
#343438,#343439),(#343440,#343441,#343442),(#343443,#343444,#343445),(#343446,
#343447,#343448),(#343449,#343450,#343451),(#343452,#343453,#343454),(#343455,
#343456,#343457),(#343458,#343459,#343460),(#343461,#343462,#343463),(#343464,
#343465,#343466),(#343467,#343468,#343469),(#343470,#343471,#343472),(#343473,
#343474,#343475),(#343476,#343477,#343478),(#343479,#343480,#343481),(#343482,
#343483,#343484),(#343485,#343486,#343487),(#343488,#343489,#343490),(#343491,
#343492,#343493),(#343494,#343495,#343496),(#343497,#343498,#343499),(#343500,
#343501,#343502),(#343503,#343504,#343505),(#343506,#343507,#343508),(#343509,
#343510,#343511),(#343512,#343513,#343514),(#343515,#343516,#343517),(#343518,
#343519,#343520),(#343521,#343522,#343523),(#343524,#343525,#343526),(#343527,
#343528,#343529),(#343530,#343531,#343532),(#343533,#343534,#343535),(#343536,
#343537,#343538),(#343539,#343540,#343541),(#343542,#343543,#343544),(#343545,
#343546,#343547),(#343548,#343549,#343550),(#343551,#343552,#343553),(#343554,
#343555,#343556),(#343557,#343558,#343559),(#343560,#343561,#343562),(#343563,
#343564,#343565),(#343566,#343567,#343568),(#343569,#343570,#343571),(#343572,
#343573,#343574),(#343575,#343576,#343577),(#343578,#343579,#343580),(#343581,
#343582,#343583),(#343584,#343585,#343586),(#343587,#343588,#343589),(#343590,
#343591,#343592),(#343593,#343594,#343595),(#343596,#343597,#343598),(#343599,
#343600,#343601),(#343602,#343603,#343604),(#343605,#343606,#343607),(#343608,
#343609,#343610),(#343611,#343612,#343613),(#343614,#343615,#343616),(#343617,
#343618,#343619),(#343620,#343621,#343622),(#343623,#343624,#343625),(#343626,
#343627,#343628),(#343629,#343630,#343631),(#343632,#343633,#343634),(#343635,
#343636,#343637),(#343638,#343639,#343640),(#343641,#343642,#343643),(#343644,
#343645,#343646),(#343647,#343648,#343649),(#343650,#343651,#343652),(#343653,
#343654,#343655),(#343656,#343657,#343658),(#343659,#343660,#343661),(#343662,
#343663,#343664),(#343665,#343666,#343667),(#343668,#343669,#343670),(#343671,
#343672,#343673),(#343674,#343675,#343676),(#343677,#343678,#343679),(#343680,
#343681,#343682),(#343683,#343684,#343685),(#343686,#343687,#343688),(#343689,
#343690,#343691),(#343692,#343693,#343694),(#343695,#343696,#343697),(#343698,
#343699,#343700),(#343701,#343702,#343703),(#343704,#343705,#343706),(#343707,
#343708,#343709),(#343710,#343711,#343712),(#343713,#343714,#343715),(#343716,
#343717,#343718),(#343719,#343720,#343721),(#343722,#343723,#343724),(#343725,
#343726,#343727),(#343728,#343729,#343730),(#343731,#343732,#343733),(#343734,
#343735,#343736),(#343737,#343738,#343739),(#343740,#343741,#343742),(#343743,
#343744,#343745),(#343746,#343747,#343748),(#343749,#343750,#343751),(#343752,
#343753,#343754),(#343755,#343756,#343757),(#343758,#343759,#343760),(#343761,
#343762,#343763),(#343764,#343765,#343766),(#343767,#343768,#343769),(#343770,
#343771,#343772),(#343773,#343774,#343775),(#343776,#343777,#343778),(#343779,
#343780,#343781),(#343782,#343783,#343784),(#343785,#343786,#343787),(#343788,
#343789,#343790),(#343791,#343792,#343793),(#343794,#343795,#343796),(#343797,
#343798,#343799),(#343800,#343801,#343802),(#343803,#343804,#343805),(#343806,
#343807,#343808),(#343809,#343810,#343811),(#343812,#343813,#343814),(#343815,
#343816,#343817),(#343818,#343819,#343820),(#343821,#343822,#343823),(#343824,
#343825,#343826),(#343827,#343828,#343829),(#343830,#343831,#343832),(#343833,
#343834,#343835),(#343836,#343837,#343838),(#343839,#343840,#343841),(#343842,
#343843,#343844),(#343845,#343846,#343847),(#343848,#343849,#343850),(#343851,
#343852,#343853),(#343854,#343855,#343856),(#343857,#343858,#343859),(#343860,
#343861,#343862),(#343863,#343864,#343865),(#343866,#343867,#343868),(#343869,
#343870,#343871),(#343872,#343873,#343874),(#343875,#343876,#343877),(#343878,
#343879,#343880),(#343881,#343882,#343883),(#343884,#343885,#343886),(#343887,
#343888,#343889),(#343890,#343891,#343892),(#343893,#343894,#343895),(#343896,
#343897,#343898),(#343899,#343900,#343901),(#343902,#343903,#343904),(#343905,
#343906,#343907),(#343908,#343909,#343910),(#343911,#343912,#343913),(#343914,
#343915,#343916),(#343917,#343918,#343919),(#343920,#343921,#343922),(#343923,
#343924,#343925),(#343926,#343927,#343928),(#343929,#343930,#343931),(#343932,
#343933,#343934),(#343935,#343936,#343937),(#343938,#343939,#343940),(#343941,
#343942,#343943),(#343944,#343945,#343946),(#343947,#343948,#343949),(#343950,
#343951,#343952),(#343953,#343954,#343955),(#343956,#343957,#343958),(#343959,
#343960,#343961),(#343962,#343963,#343964),(#343965,#343966,#343967),(#343968,
#343969,#343970),(#343971,#343972,#343973),(#343974,#343975,#343976),(#343977,
#343978,#343979),(#343980,#343981,#343982),(#343983,#343984,#343985),(#343986,
#343987,#343988),(#343989,#343990,#343991),(#343992,#343993,#343994),(#343995,
#343996,#343997),(#343998,#343999,#344000),(#344001,#344002,#344003),(#344004,
#344005,#344006),(#344007,#344008,#344009),(#344010,#344011,#344012),(#344013,
#344014,#344015),(#344016,#344017,#344018),(#344019,#344020,#344021),(#344022,
#344023,#344024),(#344025,#344026,#344027),(#344028,#344029,#344030),(#344031,
#344032,#344033),(#344034,#344035,#344036),(#344037,#344038,#344039),(#344040,
#344041,#344042),(#344043,#344044,#344045),(#344046,#344047,#344048),(#344049,
#344050,#344051),(#344052,#344053,#344054),(#344055,#344056,#344057),(#344058,
#344059,#344060),(#344061,#344062,#344063),(#344064,#344065,#344066),(#344067,
#344068,#344069),(#344070,#344071,#344072),(#344073,#344074,#344075),(#344076,
#344077,#344078),(#344079,#344080,#344081),(#344082,#344083,#344084),(#344085,
#344086,#344087),(#344088,#344089,#344090),(#344091,#344092,#344093),(#344094,
#344095,#344096),(#344097,#344098,#344099),(#344100,#344101,#344102),(#344103,
#344104,#344105),(#344106,#344107,#344108),(#344109,#344110,#344111),(#344112,
#344113,#344114),(#344115,#344116,#344117),(#344118,#344119,#344120),(#344121,
#344122,#344123),(#344124,#344125,#344126),(#344127,#344128,#344129),(#344130,
#344131,#344132),(#344133,#344134,#344135),(#344136,#344137,#344138),(#344139,
#344140,#344141),(#344142,#344143,#344144),(#344145,#344146,#344147),(#344148,
#344149,#344150),(#344151,#344152,#344153),(#344154,#344155,#344156),(#344157,
#344158,#344159),(#344160,#344161,#344162),(#344163,#344164,#344165),(#344166,
#344167,#344168),(#344169,#344170,#344171),(#344172,#344173,#344174),(#344175,
#344176,#344177),(#344178,#344179,#344180),(#344181,#344182,#344183),(#344184,
#344185,#344186),(#344187,#344188,#344189),(#344190,#344191,#344192),(#344193,
#344194,#344195),(#344196,#344197,#344198),(#344199,#344200,#344201),(#344202,
#344203,#344204),(#344205,#344206,#344207),(#344208,#344209,#344210),(#344211,
#344212,#344213),(#344214,#344215,#344216),(#344217,#344218,#344219),(#344220,
#344221,#344222),(#344223,#344224,#344225),(#344226,#344227,#344228),(#344229,
#344230,#344231),(#344232,#344233,#344234),(#344235,#344236,#344237),(#344238,
#344239,#344240),(#344241,#344242,#344243),(#344244,#344245,#344246),(#344247,
#344248,#344249),(#344250,#344251,#344252),(#344253,#344254,#344255),(#344256,
#344257,#344258),(#344259,#344260,#344261),(#344262,#344263,#344264),(#344265,
#344266,#344267),(#344268,#344269,#344270),(#344271,#344272,#344273),(#344274,
#344275,#344276),(#344277,#344278,#344279),(#344280,#344281,#344282),(#344283,
#344284,#344285),(#344286,#344287,#344288),(#344289,#344290,#344291),(#344292,
#344293,#344294),(#344295,#344296,#344297),(#344298,#344299,#344300),(#344301,
#344302,#344303),(#344304,#344305,#344306),(#344307,#344308,#344309),(#344310,
#344311,#344312),(#344313,#344314,#344315),(#344316,#344317,#344318),(#344319,
#344320,#344321),(#344322,#344323,#344324),(#344325,#344326,#344327),(#344328,
#344329,#344330),(#344331,#344332,#344333),(#344334,#344335,#344336),(#344337,
#344338,#344339),(#344340,#344341,#344342),(#344343,#344344,#344345),(#344346,
#344347,#344348),(#344349,#344350,#344351),(#344352,#344353,#344354),(#344355,
#344356,#344357),(#344358,#344359,#344360),(#344361,#344362,#344363),(#344364,
#344365,#344366),(#344367,#344368,#344369),(#344370,#344371,#344372),(#344373,
#344374,#344375),(#344376,#344377,#344378),(#344379,#344380,#344381),(#344382,
#344383,#344384),(#344385,#344386,#344387),(#344388,#344389,#344390),(#344391,
#344392,#344393),(#344394,#344395,#344396),(#344397,#344398,#344399),(#344400,
#344401,#344402),(#344403,#344404,#344405),(#344406,#344407,#344408),(#344409,
#344410,#344411),(#344412,#344413,#344414),(#344415,#344416,#344417),(#344418,
#344419,#344420),(#344421,#344422,#344423),(#344424,#344425,#344426),(#344427,
#344428,#344429),(#344430,#344431,#344432),(#344433,#344434,#344435),(#344436,
#344437,#344438),(#344439,#344440,#344441),(#344442,#344443,#344444),(#344445,
#344446,#344447),(#344448,#344449,#344450),(#344451,#344452,#344453),(#344454,
#344455,#344456),(#344457,#344458,#344459),(#344460,#344461,#344462),(#344463,
#344464,#344465),(#344466,#344467,#344468),(#344469,#344470,#344471),(#344472,
#344473,#344474),(#344475,#344476,#344477),(#344478,#344479,#344480),(#344481,
#344482,#344483),(#344484,#344485,#344486),(#344487,#344488,#344489),(#344490,
#344491,#344492),(#344493,#344494,#344495),(#344496,#344497,#344498),(#344499,
#344500,#344501),(#344502,#344503,#344504),(#344505,#344506,#344507),(#344508,
#344509,#344510),(#344511,#344512,#344513),(#344514,#344515,#344516),(#344517,
#344518,#344519),(#344520,#344521,#344522),(#344523,#344524,#344525),(#344526,
#344527,#344528),(#344529,#344530,#344531),(#344532,#344533,#344534),(#344535,
#344536,#344537),(#344538,#344539,#344540),(#344541,#344542,#344543),(#344544,
#344545,#344546),(#344547,#344548,#344549),(#344550,#344551,#344552),(#344553,
#344554,#344555),(#344556,#344557,#344558),(#344559,#344560,#344561),(#344562,
#344563,#344564),(#344565,#344566,#344567),(#344568,#344569,#344570),(#344571,
#344572,#344573),(#344574,#344575,#344576),(#344577,#344578,#344579),(#344580,
#344581,#344582),(#344583,#344584,#344585),(#344586,#344587,#344588),(#344589,
#344590,#344591),(#344592,#344593,#344594),(#344595,#344596,#344597),(#344598,
#344599,#344600),(#344601,#344602,#344603),(#344604,#344605,#344606),(#344607,
#344608,#344609),(#344610,#344611,#344612),(#344613,#344614,#344615),(#344616,
#344617,#344618),(#344619,#344620,#344621),(#344622,#344623,#344624),(#344625,
#344626,#344627),(#344628,#344629,#344630),(#344631,#344632,#344633),(#344634,
#344635,#344636),(#344637,#344638,#344639),(#344640,#344641,#344642),(#344643,
#344644,#344645),(#344646,#344647,#344648),(#344649,#344650,#344651),(#344652,
#344653,#344654),(#344655,#344656,#344657),(#344658,#344659,#344660),(#344661,
#344662,#344663),(#344664,#344665,#344666),(#344667,#344668,#344669),(#344670,
#344671,#344672),(#344673,#344674,#344675),(#344676,#344677,#344678),(#344679,
#344680,#344681),(#344682,#344683,#344684),(#344685,#344686,#344687),(#344688,
#344689,#344690),(#344691,#344692,#344693),(#344694,#344695,#344696),(#344697,
#344698,#344699),(#344700,#344701,#344702),(#344703,#344704,#344705),(#344706,
#344707,#344708),(#344709,#344710,#344711),(#344712,#344713,#344714),(#344715,
#344716,#344717),(#344718,#344719,#344720),(#344721,#344722,#344723),(#344724,
#344725,#344726),(#344727,#344728,#344729),(#344730,#344731,#344732),(#344733,
#344734,#344735),(#344736,#344737,#344738),(#344739,#344740,#344741),(#344742,
#344743,#344744),(#344745,#344746,#344747),(#344748,#344749,#344750),(#344751,
#344752,#344753),(#344754,#344755,#344756),(#344757,#344758,#344759),(#344760,
#344761,#344762),(#344763,#344764,#344765),(#344766,#344767,#344768),(#344769,
#344770,#344771),(#344772,#344773,#344774),(#344775,#344776,#344777),(#344778,
#344779,#344780),(#344781,#344782,#344783),(#344784,#344785,#344786),(#344787,
#344788,#344789),(#344790,#344791,#344792),(#344793,#344794,#344795),(#344796,
#344797,#344798),(#344799,#344800,#344801),(#344802,#344803,#344804),(#344805,
#344806,#344807),(#344808,#344809,#344810),(#344811,#344812,#344813),(#344814,
#344815,#344816),(#344817,#344818,#344819),(#344820,#344821,#344822),(#344823,
#344824,#344825),(#344826,#344827,#344828),(#344829,#344830,#344831),(#344832,
#344833,#344834),(#344835,#344836,#344837),(#344838,#344839,#344840),(#344841,
#344842,#344843),(#344844,#344845,#344846),(#344847,#344848,#344849),(#344850,
#344851,#344852),(#344853,#344854,#344855),(#344856,#344857,#344858),(#344859,
#344860,#344861),(#344862,#344863,#344864),(#344865,#344866,#344867),(#344868,
#344869,#344870),(#344871,#344872,#344873),(#344874,#344875,#344876),(#344877,
#344878,#344879),(#344880,#344881,#344882),(#344883,#344884,#344885),(#344886,
#344887,#344888),(#344889,#344890,#344891),(#344892,#344893,#344894),(#344895,
#344896,#344897)),.UNSPECIFIED.,.F.,.F.,.F.,(6,1,1,1,1,1,1,1,1,1,1,1,1,
1,1,1,1,1,1,1,1,1,1,1,1,1,1,1,1,1,1,1,1,1,1,1,1,1,1,1,1,1,1,1,1,1,1,1,1,
1,1,1,1,1,1,1,1,1,1,1,1,1,1,1,1,1,1,1,1,1,1,1,1,1,1,1,1,1,1,1,1,1,1,1,1,
1,1,1,1,1,1,1,1,1,1,1,1,1,1,1,1,1,1,1,1,1,1,1,1,1,1,1,1,1,1,1,1,1,1,1,1,
1,1,1,1,1,1,1,1,1,1,1,1,1,1,1,1,1,1,1,1,1,1,1,1,1,1,1,1,1,1,1,1,1,1,1,1,
1,1,1,1,1,1,1,1,1,1,1,1,1,1,1,1,1,1,1,1,1,1,1,1,1,1,1,1,1,1,1,1,1,1,1,1,
1,1,1,1,1,1,1,1,1,1,1,1,1,1,1,1,1,1,1,1,1,1,1,1,1,1,1,1,1,1,1,1,1,1,1,1,
1,1,1,1,1,1,1,1,1,1,1,1,1,1,1,1,1,1,1,1,1,1,1,1,1,1,1,1,1,1,1,1,1,1,1,1,
1,1,1,1,1,1,1,1,1,1,1,1,1,1,1,1,1,1,1,1,1,1,1,1,1,1,1,1,1,1,1,1,1,1,1,1,
1,1,1,1,1,1,1,1,1,1,1,1,1,1,1,1,1,1,1,1,1,1,1,1,1,1,1,1,1,1,1,1,1,1,1,1,
1,1,1,1,1,1,1,1,1,1,1,1,1,1,1,1,1,1,1,1,1,1,1,1,1,1,1,1,1,1,1,1,1,1,1,1,
1,1,1,1,1,1,1,1,1,1,1,1,1,1,1,1,1,1,1,1,1,1,1,1,1,1,1,1,1,1,1,1,1,1,1,1,
1,1,1,1,1,1,1,1,1,1,1,1,1,1,1,1,1,1,1,1,1,1,1,1,1,1,1,1,1,1,1,1,1,1,1,1,
1,1,1,1,1,1,1,1,1,1,1,1,1,1,1,1,1,1,1,1,1,1,1,1,1,1,1,1,1,1,1,1,1,1,1,1,
1,1,1,1,1,1,1,1,1,1,1,1,1,1,1,1,1,1,1,1,1,1,1,1,1,1,1,1,1,1,1,1,1,1,1,1,
1,1,1,1,1,1,1,1,1,1,1,1,1,1,1,1,1,1,1,1,1,1,1,1,1,1,1,1,1,6),(2,1,2),(-0.00196417,
0.,0.001834862,0.003669725,0.005504587,0.00733945,0.009174312,0.011009174,
0.012844037,0.014678899,0.016513761,0.018348624,0.020183486,0.022018349,
0.023853211,0.025688073,0.027522936,0.029357798,0.031192661,0.033027523,
0.034862385,0.036697248,0.03853211,0.040366972,0.042201835,0.044036697,
0.04587156,0.047706422,0.049541284,0.051376147,0.053211009,0.055045872,
0.056880734,0.058715596,0.060550459,0.062385321,0.064220183,0.066055046,
0.067889908,0.069724771,0.071559633,0.073394495,0.075229358,0.07706422,
0.078899083,0.080733945,0.082568807,0.08440367,0.086238532,0.088073394,
0.089908257,0.091743119,0.093577982,0.095412844,0.097247706,0.099082569,
0.100917431,0.102752294,0.104587156,0.106422018,0.108256881,0.110091743,
0.111926606,0.113761468,0.11559633,0.117431193,0.119266055,0.121100917,
0.12293578,0.124770642,0.126605505,0.128440367,0.130275229,0.132110092,
0.133944954,0.135779817,0.137614679,0.139449541,0.141284404,0.143119266,
0.144954128,0.146788991,0.148623853,0.150458716,0.152293578,0.15412844,
0.155963303,0.157798165,0.159633028,0.16146789,0.163302752,0.165137615,
0.166972477,0.168807339,0.170642202,0.172477064,0.174311927,0.176146789,
0.177981651,0.179816514,0.181651376,0.183486239,0.185321101,0.187155963,
0.188990826,0.190825688,0.19266055,0.194495413,0.196330275,0.198165138,
0.2,0.201834862,0.203669725,0.205504587,0.20733945,0.209174312,0.211009174,
0.212844037,0.214678899,0.216513761,0.218348624,0.220183486,0.222018349,
0.223853211,0.225688073,0.227522936,0.229357798,0.231192661,0.233027523,
0.234862385,0.236697248,0.23853211,0.240366972,0.242201835,0.244036697,
0.24587156,0.247706422,0.249541284,0.251376147,0.253211009,0.255045872,
0.256880734,0.258715596,0.260550459,0.262385321,0.264220183,0.266055046,
0.267889908,0.269724771,0.271559633,0.273394495,0.275229358,0.27706422,
0.278899083,0.280733945,0.282568807,0.28440367,0.286238532,0.288073394,
0.289908257,0.291743119,0.293577982,0.295412844,0.297247706,0.299082569,
0.300917431,0.302752294,0.304587156,0.306422018,0.308256881,0.310091743,
0.311926606,0.313761468,0.31559633,0.317431193,0.319266055,0.321100917,
0.32293578,0.324770642,0.326605505,0.328440367,0.330275229,0.332110092,
0.333944954,0.335779817,0.337614679,0.339449541,0.341284404,0.343119266,
0.344954128,0.346788991,0.348623853,0.350458716,0.352293578,0.35412844,
0.355963303,0.357798165,0.359633028,0.36146789,0.363302752,0.365137615,
0.366972477,0.368807339,0.370642202,0.372477064,0.374311927,0.376146789,
0.377981651,0.379816514,0.381651376,0.383486239,0.385321101,0.387155963,
0.388990826,0.390825688,0.39266055,0.394495413,0.396330275,0.398165138,
0.4,0.401834862,0.403669725,0.405504587,0.40733945,0.409174312,0.411009174,
0.412844037,0.414678899,0.416513761,0.418348624,0.420183486,0.422018349,
0.423853211,0.425688073,0.427522936,0.429357798,0.431192661,0.433027523,
0.434862385,0.436697248,0.43853211,0.440366972,0.442201835,0.444036697,
0.44587156,0.447706422,0.449541284,0.451376147,0.453211009,0.455045872,
0.456880734,0.458715596,0.460550459,0.462385321,0.464220183,0.466055046,
0.467889908,0.469724771,0.471559633,0.473394495,0.475229358,0.47706422,
0.478899083,0.480733945,0.482568807,0.48440367,0.486238532,0.488073394,
0.489908257,0.491743119,0.493577982,0.495412844,0.497247706,0.499082569,
0.500917431,0.502752294,0.504587156,0.506422018,0.508256881,0.510091743,
0.511926606,0.513761468,0.51559633,0.517431193,0.519266055,0.521100917,
0.52293578,0.524770642,0.526605505,0.528440367,0.530275229,0.532110092,
0.533944954,0.535779817,0.537614679,0.539449541,0.541284404,0.543119266,
0.544954128,0.546788991,0.548623853,0.550458716,0.552293578,0.55412844,
0.555963303,0.557798165,0.559633028,0.56146789,0.563302752,0.565137615,
0.566972477,0.568807339,0.570642202,0.572477064,0.574311927,0.576146789,
0.577981651,0.579816514,0.581651376,0.583486239,0.585321101,0.587155963,
0.588990826,0.590825688,0.59266055,0.594495413,0.596330275,0.598165138,
0.6,0.601834862,0.603669725,0.605504587,0.60733945,0.609174312,0.611009174,
0.612844037,0.614678899,0.616513761,0.618348624,0.620183486,0.622018349,
0.623853211,0.625688073,0.627522936,0.629357798,0.631192661,0.633027523,
0.634862385,0.636697248,0.63853211,0.640366972,0.642201835,0.644036697,
0.64587156,0.647706422,0.649541284,0.651376147,0.653211009,0.655045872,
0.656880734,0.658715596,0.660550459,0.662385321,0.664220183,0.666055046,
0.667889908,0.669724771,0.671559633,0.673394495,0.675229358,0.67706422,
0.678899083,0.680733945,0.682568807,0.68440367,0.686238532,0.688073394,
0.689908257,0.691743119,0.693577982,0.695412844,0.697247706,0.699082569,
0.700917431,0.702752294,0.704587156,0.706422018,0.708256881,0.710091743,
0.711926606,0.713761468,0.71559633,0.717431193,0.719266055,0.721100917,
0.72293578,0.724770642,0.726605505,0.728440367,0.730275229,0.732110092,
0.733944954,0.735779817,0.737614679,0.739449541,0.741284404,0.743119266,
0.744954128,0.746788991,0.748623853,0.750458716,0.752293578,0.75412844,
0.755963303,0.757798165,0.759633028,0.76146789,0.763302752,0.765137615,
0.766972477,0.768807339,0.770642202,0.772477064,0.774311927,0.776146789,
0.777981651,0.779816514,0.781651376,0.783486239,0.785321101,0.787155963,
0.788990826,0.790825688,0.79266055,0.794495413,0.796330275,0.798165138,
0.8,0.801834862,0.803669725,0.805504587,0.80733945,0.809174312,0.811009174,
0.812844037,0.814678899,0.816513761,0.818348624,0.820183486,0.822018349,
0.823853211,0.825688073,0.827522936,0.829357798,0.831192661,0.833027523,
0.834862385,0.836697248,0.83853211,0.840366972,0.842201835,0.844036697,
0.84587156,0.847706422,0.849541284,0.851376147,0.853211009,0.855045872,
0.856880734,0.858715596,0.860550459,0.862385321,0.864220183,0.866055046,
0.867889908,0.869724771,0.871559633,0.873394495,0.875229358,0.87706422,
0.878899083,0.880733945,0.882568807,0.88440367,0.886238532,0.888073394,
0.889908257,0.891743119,0.893577982,0.895412844,0.897247706,0.899082569,
0.900917431,0.902752294,0.904587156,0.906422018,0.908256881,0.910091743,
0.911926606,0.913761468,0.91559633,0.917431193,0.919266055,0.921100917,
0.92293578,0.924770642,0.926605505,0.928440367,0.930275229,0.932110092,
0.933944954,0.935779817,0.937614679,0.939449541,0.941284404,0.943119266,
0.944954128,0.946788991,0.948623853,0.950458716,0.952293578,0.95412844,
0.955963303,0.957798165,0.959633028,0.96146789,0.963302752,0.965137615,
0.966972477,0.968807339,0.970642202,0.972477064,0.974311927,0.976146789,
0.977981651,0.979816514,0.981651376,0.983486239,0.985321101,0.987155963,
0.988990826,0.990825688,0.99266055,0.994495413,0.996330275,0.998165138,
1.000000000285),(0.3,1.,1.3),.UNSPECIFIED.);
#6329=B_SPLINE_SURFACE_WITH_KNOTS('',5,1,((#344909,#344910,#344911),(#344912,
#344913,#344914),(#344915,#344916,#344917),(#344918,#344919,#344920),(#344921,
#344922,#344923),(#344924,#344925,#344926),(#344927,#344928,#344929),(#344930,
#344931,#344932),(#344933,#344934,#344935),(#344936,#344937,#344938),(#344939,
#344940,#344941),(#344942,#344943,#344944),(#344945,#344946,#344947),(#344948,
#344949,#344950),(#344951,#344952,#344953),(#344954,#344955,#344956),(#344957,
#344958,#344959),(#344960,#344961,#344962),(#344963,#344964,#344965),(#344966,
#344967,#344968),(#344969,#344970,#344971),(#344972,#344973,#344974),(#344975,
#344976,#344977),(#344978,#344979,#344980),(#344981,#344982,#344983),(#344984,
#344985,#344986),(#344987,#344988,#344989),(#344990,#344991,#344992),(#344993,
#344994,#344995),(#344996,#344997,#344998),(#344999,#345000,#345001),(#345002,
#345003,#345004),(#345005,#345006,#345007),(#345008,#345009,#345010),(#345011,
#345012,#345013),(#345014,#345015,#345016),(#345017,#345018,#345019),(#345020,
#345021,#345022),(#345023,#345024,#345025),(#345026,#345027,#345028),(#345029,
#345030,#345031),(#345032,#345033,#345034),(#345035,#345036,#345037),(#345038,
#345039,#345040),(#345041,#345042,#345043),(#345044,#345045,#345046),(#345047,
#345048,#345049),(#345050,#345051,#345052),(#345053,#345054,#345055),(#345056,
#345057,#345058),(#345059,#345060,#345061),(#345062,#345063,#345064),(#345065,
#345066,#345067),(#345068,#345069,#345070),(#345071,#345072,#345073),(#345074,
#345075,#345076),(#345077,#345078,#345079),(#345080,#345081,#345082),(#345083,
#345084,#345085),(#345086,#345087,#345088),(#345089,#345090,#345091),(#345092,
#345093,#345094),(#345095,#345096,#345097),(#345098,#345099,#345100),(#345101,
#345102,#345103),(#345104,#345105,#345106),(#345107,#345108,#345109),(#345110,
#345111,#345112),(#345113,#345114,#345115),(#345116,#345117,#345118),(#345119,
#345120,#345121),(#345122,#345123,#345124),(#345125,#345126,#345127),(#345128,
#345129,#345130),(#345131,#345132,#345133),(#345134,#345135,#345136),(#345137,
#345138,#345139),(#345140,#345141,#345142),(#345143,#345144,#345145),(#345146,
#345147,#345148),(#345149,#345150,#345151),(#345152,#345153,#345154),(#345155,
#345156,#345157),(#345158,#345159,#345160),(#345161,#345162,#345163),(#345164,
#345165,#345166),(#345167,#345168,#345169),(#345170,#345171,#345172),(#345173,
#345174,#345175),(#345176,#345177,#345178),(#345179,#345180,#345181),(#345182,
#345183,#345184),(#345185,#345186,#345187),(#345188,#345189,#345190),(#345191,
#345192,#345193),(#345194,#345195,#345196),(#345197,#345198,#345199),(#345200,
#345201,#345202),(#345203,#345204,#345205),(#345206,#345207,#345208),(#345209,
#345210,#345211),(#345212,#345213,#345214),(#345215,#345216,#345217),(#345218,
#345219,#345220),(#345221,#345222,#345223),(#345224,#345225,#345226),(#345227,
#345228,#345229),(#345230,#345231,#345232),(#345233,#345234,#345235),(#345236,
#345237,#345238),(#345239,#345240,#345241),(#345242,#345243,#345244),(#345245,
#345246,#345247),(#345248,#345249,#345250),(#345251,#345252,#345253),(#345254,
#345255,#345256),(#345257,#345258,#345259),(#345260,#345261,#345262),(#345263,
#345264,#345265),(#345266,#345267,#345268),(#345269,#345270,#345271),(#345272,
#345273,#345274),(#345275,#345276,#345277),(#345278,#345279,#345280),(#345281,
#345282,#345283),(#345284,#345285,#345286),(#345287,#345288,#345289),(#345290,
#345291,#345292),(#345293,#345294,#345295),(#345296,#345297,#345298),(#345299,
#345300,#345301),(#345302,#345303,#345304),(#345305,#345306,#345307),(#345308,
#345309,#345310),(#345311,#345312,#345313),(#345314,#345315,#345316),(#345317,
#345318,#345319),(#345320,#345321,#345322),(#345323,#345324,#345325),(#345326,
#345327,#345328),(#345329,#345330,#345331),(#345332,#345333,#345334),(#345335,
#345336,#345337),(#345338,#345339,#345340),(#345341,#345342,#345343),(#345344,
#345345,#345346),(#345347,#345348,#345349),(#345350,#345351,#345352),(#345353,
#345354,#345355),(#345356,#345357,#345358),(#345359,#345360,#345361),(#345362,
#345363,#345364),(#345365,#345366,#345367),(#345368,#345369,#345370),(#345371,
#345372,#345373),(#345374,#345375,#345376),(#345377,#345378,#345379),(#345380,
#345381,#345382),(#345383,#345384,#345385),(#345386,#345387,#345388),(#345389,
#345390,#345391),(#345392,#345393,#345394),(#345395,#345396,#345397),(#345398,
#345399,#345400),(#345401,#345402,#345403),(#345404,#345405,#345406),(#345407,
#345408,#345409),(#345410,#345411,#345412),(#345413,#345414,#345415),(#345416,
#345417,#345418),(#345419,#345420,#345421),(#345422,#345423,#345424),(#345425,
#345426,#345427),(#345428,#345429,#345430),(#345431,#345432,#345433),(#345434,
#345435,#345436),(#345437,#345438,#345439),(#345440,#345441,#345442),(#345443,
#345444,#345445),(#345446,#345447,#345448),(#345449,#345450,#345451),(#345452,
#345453,#345454),(#345455,#345456,#345457),(#345458,#345459,#345460),(#345461,
#345462,#345463),(#345464,#345465,#345466),(#345467,#345468,#345469),(#345470,
#345471,#345472),(#345473,#345474,#345475),(#345476,#345477,#345478),(#345479,
#345480,#345481),(#345482,#345483,#345484),(#345485,#345486,#345487),(#345488,
#345489,#345490),(#345491,#345492,#345493),(#345494,#345495,#345496),(#345497,
#345498,#345499),(#345500,#345501,#345502),(#345503,#345504,#345505),(#345506,
#345507,#345508),(#345509,#345510,#345511),(#345512,#345513,#345514),(#345515,
#345516,#345517),(#345518,#345519,#345520),(#345521,#345522,#345523),(#345524,
#345525,#345526),(#345527,#345528,#345529),(#345530,#345531,#345532),(#345533,
#345534,#345535),(#345536,#345537,#345538),(#345539,#345540,#345541),(#345542,
#345543,#345544),(#345545,#345546,#345547),(#345548,#345549,#345550),(#345551,
#345552,#345553),(#345554,#345555,#345556),(#345557,#345558,#345559),(#345560,
#345561,#345562),(#345563,#345564,#345565),(#345566,#345567,#345568),(#345569,
#345570,#345571),(#345572,#345573,#345574),(#345575,#345576,#345577),(#345578,
#345579,#345580),(#345581,#345582,#345583),(#345584,#345585,#345586),(#345587,
#345588,#345589),(#345590,#345591,#345592),(#345593,#345594,#345595),(#345596,
#345597,#345598),(#345599,#345600,#345601),(#345602,#345603,#345604),(#345605,
#345606,#345607),(#345608,#345609,#345610),(#345611,#345612,#345613),(#345614,
#345615,#345616),(#345617,#345618,#345619),(#345620,#345621,#345622),(#345623,
#345624,#345625),(#345626,#345627,#345628),(#345629,#345630,#345631),(#345632,
#345633,#345634),(#345635,#345636,#345637),(#345638,#345639,#345640),(#345641,
#345642,#345643),(#345644,#345645,#345646),(#345647,#345648,#345649),(#345650,
#345651,#345652),(#345653,#345654,#345655),(#345656,#345657,#345658),(#345659,
#345660,#345661),(#345662,#345663,#345664),(#345665,#345666,#345667),(#345668,
#345669,#345670),(#345671,#345672,#345673),(#345674,#345675,#345676),(#345677,
#345678,#345679),(#345680,#345681,#345682),(#345683,#345684,#345685),(#345686,
#345687,#345688),(#345689,#345690,#345691),(#345692,#345693,#345694),(#345695,
#345696,#345697),(#345698,#345699,#345700),(#345701,#345702,#345703),(#345704,
#345705,#345706),(#345707,#345708,#345709),(#345710,#345711,#345712),(#345713,
#345714,#345715),(#345716,#345717,#345718),(#345719,#345720,#345721),(#345722,
#345723,#345724),(#345725,#345726,#345727),(#345728,#345729,#345730),(#345731,
#345732,#345733),(#345734,#345735,#345736),(#345737,#345738,#345739),(#345740,
#345741,#345742),(#345743,#345744,#345745),(#345746,#345747,#345748),(#345749,
#345750,#345751),(#345752,#345753,#345754),(#345755,#345756,#345757),(#345758,
#345759,#345760),(#345761,#345762,#345763),(#345764,#345765,#345766),(#345767,
#345768,#345769),(#345770,#345771,#345772),(#345773,#345774,#345775),(#345776,
#345777,#345778),(#345779,#345780,#345781),(#345782,#345783,#345784),(#345785,
#345786,#345787),(#345788,#345789,#345790),(#345791,#345792,#345793),(#345794,
#345795,#345796),(#345797,#345798,#345799),(#345800,#345801,#345802),(#345803,
#345804,#345805),(#345806,#345807,#345808),(#345809,#345810,#345811),(#345812,
#345813,#345814),(#345815,#345816,#345817),(#345818,#345819,#345820),(#345821,
#345822,#345823),(#345824,#345825,#345826),(#345827,#345828,#345829),(#345830,
#345831,#345832),(#345833,#345834,#345835),(#345836,#345837,#345838),(#345839,
#345840,#345841),(#345842,#345843,#345844),(#345845,#345846,#345847),(#345848,
#345849,#345850),(#345851,#345852,#345853),(#345854,#345855,#345856),(#345857,
#345858,#345859),(#345860,#345861,#345862),(#345863,#345864,#345865),(#345866,
#345867,#345868),(#345869,#345870,#345871),(#345872,#345873,#345874),(#345875,
#345876,#345877),(#345878,#345879,#345880),(#345881,#345882,#345883),(#345884,
#345885,#345886),(#345887,#345888,#345889),(#345890,#345891,#345892),(#345893,
#345894,#345895),(#345896,#345897,#345898),(#345899,#345900,#345901),(#345902,
#345903,#345904),(#345905,#345906,#345907),(#345908,#345909,#345910),(#345911,
#345912,#345913),(#345914,#345915,#345916),(#345917,#345918,#345919),(#345920,
#345921,#345922),(#345923,#345924,#345925),(#345926,#345927,#345928),(#345929,
#345930,#345931),(#345932,#345933,#345934),(#345935,#345936,#345937),(#345938,
#345939,#345940),(#345941,#345942,#345943),(#345944,#345945,#345946),(#345947,
#345948,#345949),(#345950,#345951,#345952),(#345953,#345954,#345955),(#345956,
#345957,#345958),(#345959,#345960,#345961),(#345962,#345963,#345964),(#345965,
#345966,#345967),(#345968,#345969,#345970),(#345971,#345972,#345973),(#345974,
#345975,#345976),(#345977,#345978,#345979),(#345980,#345981,#345982),(#345983,
#345984,#345985),(#345986,#345987,#345988),(#345989,#345990,#345991),(#345992,
#345993,#345994),(#345995,#345996,#345997),(#345998,#345999,#346000),(#346001,
#346002,#346003),(#346004,#346005,#346006),(#346007,#346008,#346009),(#346010,
#346011,#346012),(#346013,#346014,#346015),(#346016,#346017,#346018),(#346019,
#346020,#346021),(#346022,#346023,#346024),(#346025,#346026,#346027),(#346028,
#346029,#346030),(#346031,#346032,#346033),(#346034,#346035,#346036),(#346037,
#346038,#346039),(#346040,#346041,#346042),(#346043,#346044,#346045),(#346046,
#346047,#346048),(#346049,#346050,#346051),(#346052,#346053,#346054),(#346055,
#346056,#346057),(#346058,#346059,#346060),(#346061,#346062,#346063),(#346064,
#346065,#346066),(#346067,#346068,#346069),(#346070,#346071,#346072),(#346073,
#346074,#346075),(#346076,#346077,#346078),(#346079,#346080,#346081),(#346082,
#346083,#346084),(#346085,#346086,#346087),(#346088,#346089,#346090),(#346091,
#346092,#346093),(#346094,#346095,#346096),(#346097,#346098,#346099),(#346100,
#346101,#346102),(#346103,#346104,#346105),(#346106,#346107,#346108),(#346109,
#346110,#346111),(#346112,#346113,#346114),(#346115,#346116,#346117),(#346118,
#346119,#346120),(#346121,#346122,#346123),(#346124,#346125,#346126),(#346127,
#346128,#346129),(#346130,#346131,#346132),(#346133,#346134,#346135),(#346136,
#346137,#346138),(#346139,#346140,#346141),(#346142,#346143,#346144),(#346145,
#346146,#346147),(#346148,#346149,#346150),(#346151,#346152,#346153),(#346154,
#346155,#346156),(#346157,#346158,#346159),(#346160,#346161,#346162),(#346163,
#346164,#346165),(#346166,#346167,#346168),(#346169,#346170,#346171),(#346172,
#346173,#346174),(#346175,#346176,#346177),(#346178,#346179,#346180),(#346181,
#346182,#346183),(#346184,#346185,#346186),(#346187,#346188,#346189),(#346190,
#346191,#346192),(#346193,#346194,#346195),(#346196,#346197,#346198),(#346199,
#346200,#346201),(#346202,#346203,#346204),(#346205,#346206,#346207),(#346208,
#346209,#346210),(#346211,#346212,#346213),(#346214,#346215,#346216),(#346217,
#346218,#346219),(#346220,#346221,#346222),(#346223,#346224,#346225),(#346226,
#346227,#346228),(#346229,#346230,#346231),(#346232,#346233,#346234),(#346235,
#346236,#346237),(#346238,#346239,#346240),(#346241,#346242,#346243),(#346244,
#346245,#346246),(#346247,#346248,#346249),(#346250,#346251,#346252),(#346253,
#346254,#346255),(#346256,#346257,#346258),(#346259,#346260,#346261),(#346262,
#346263,#346264),(#346265,#346266,#346267),(#346268,#346269,#346270),(#346271,
#346272,#346273),(#346274,#346275,#346276),(#346277,#346278,#346279),(#346280,
#346281,#346282),(#346283,#346284,#346285),(#346286,#346287,#346288),(#346289,
#346290,#346291),(#346292,#346293,#346294),(#346295,#346296,#346297),(#346298,
#346299,#346300),(#346301,#346302,#346303),(#346304,#346305,#346306),(#346307,
#346308,#346309),(#346310,#346311,#346312),(#346313,#346314,#346315),(#346316,
#346317,#346318),(#346319,#346320,#346321),(#346322,#346323,#346324),(#346325,
#346326,#346327),(#346328,#346329,#346330),(#346331,#346332,#346333),(#346334,
#346335,#346336),(#346337,#346338,#346339),(#346340,#346341,#346342),(#346343,
#346344,#346345),(#346346,#346347,#346348),(#346349,#346350,#346351),(#346352,
#346353,#346354),(#346355,#346356,#346357),(#346358,#346359,#346360),(#346361,
#346362,#346363),(#346364,#346365,#346366),(#346367,#346368,#346369),(#346370,
#346371,#346372),(#346373,#346374,#346375),(#346376,#346377,#346378),(#346379,
#346380,#346381),(#346382,#346383,#346384),(#346385,#346386,#346387),(#346388,
#346389,#346390),(#346391,#346392,#346393),(#346394,#346395,#346396),(#346397,
#346398,#346399),(#346400,#346401,#346402),(#346403,#346404,#346405),(#346406,
#346407,#346408),(#346409,#346410,#346411),(#346412,#346413,#346414),(#346415,
#346416,#346417),(#346418,#346419,#346420),(#346421,#346422,#346423),(#346424,
#346425,#346426),(#346427,#346428,#346429),(#346430,#346431,#346432),(#346433,
#346434,#346435),(#346436,#346437,#346438),(#346439,#346440,#346441),(#346442,
#346443,#346444),(#346445,#346446,#346447),(#346448,#346449,#346450),(#346451,
#346452,#346453),(#346454,#346455,#346456),(#346457,#346458,#346459),(#346460,
#346461,#346462),(#346463,#346464,#346465),(#346466,#346467,#346468),(#346469,
#346470,#346471),(#346472,#346473,#346474),(#346475,#346476,#346477),(#346478,
#346479,#346480),(#346481,#346482,#346483),(#346484,#346485,#346486),(#346487,
#346488,#346489),(#346490,#346491,#346492),(#346493,#346494,#346495),(#346496,
#346497,#346498),(#346499,#346500,#346501),(#346502,#346503,#346504),(#346505,
#346506,#346507),(#346508,#346509,#346510),(#346511,#346512,#346513),(#346514,
#346515,#346516),(#346517,#346518,#346519),(#346520,#346521,#346522),(#346523,
#346524,#346525),(#346526,#346527,#346528),(#346529,#346530,#346531),(#346532,
#346533,#346534),(#346535,#346536,#346537),(#346538,#346539,#346540),(#346541,
#346542,#346543),(#346544,#346545,#346546),(#346547,#346548,#346549),(#346550,
#346551,#346552),(#346553,#346554,#346555),(#346556,#346557,#346558)),
 .UNSPECIFIED.,.F.,.F.,.F.,(6,1,1,1,1,1,1,1,1,1,1,1,1,1,1,1,1,1,1,1,1,1,
1,1,1,1,1,1,1,1,1,1,1,1,1,1,1,1,1,1,1,1,1,1,1,1,1,1,1,1,1,1,1,1,1,1,1,1,
1,1,1,1,1,1,1,1,1,1,1,1,1,1,1,1,1,1,1,1,1,1,1,1,1,1,1,1,1,1,1,1,1,1,1,1,
1,1,1,1,1,1,1,1,1,1,1,1,1,1,1,1,1,1,1,1,1,1,1,1,1,1,1,1,1,1,1,1,1,1,1,1,
1,1,1,1,1,1,1,1,1,1,1,1,1,1,1,1,1,1,1,1,1,1,1,1,1,1,1,1,1,1,1,1,1,1,1,1,
1,1,1,1,1,1,1,1,1,1,1,1,1,1,1,1,1,1,1,1,1,1,1,1,1,1,1,1,1,1,1,1,1,1,1,1,
1,1,1,1,1,1,1,1,1,1,1,1,1,1,1,1,1,1,1,1,1,1,1,1,1,1,1,1,1,1,1,1,1,1,1,1,
1,1,1,1,1,1,1,1,1,1,1,1,1,1,1,1,1,1,1,1,1,1,1,1,1,1,1,1,1,1,1,1,1,1,1,1,
1,1,1,1,1,1,1,1,1,1,1,1,1,1,1,1,1,1,1,1,1,1,1,1,1,1,1,1,1,1,1,1,1,1,1,1,
1,1,1,1,1,1,1,1,1,1,1,1,1,1,1,1,1,1,1,1,1,1,1,1,1,1,1,1,1,1,1,1,1,1,1,1,
1,1,1,1,1,1,1,1,1,1,1,1,1,1,1,1,1,1,1,1,1,1,1,1,1,1,1,1,1,1,1,1,1,1,1,1,
1,1,1,1,1,1,1,1,1,1,1,1,1,1,1,1,1,1,1,1,1,1,1,1,1,1,1,1,1,1,1,1,1,1,1,1,
1,1,1,1,1,1,1,1,1,1,1,1,1,1,1,1,1,1,1,1,1,1,1,1,1,1,1,1,1,1,1,1,1,1,1,1,
1,1,1,1,1,1,1,1,1,1,1,1,1,1,1,1,1,1,1,1,1,1,1,1,1,1,1,1,1,1,1,1,1,1,1,1,
1,1,1,1,1,1,1,1,1,1,1,1,1,1,1,1,1,1,1,1,1,1,1,1,1,1,1,1,1,1,1,1,1,1,1,1,
1,1,1,1,1,1,1,1,1,1,1,1,1,1,1,1,1,1,1,6),(2,1,2),(-1.,-0.998165138,-0.996330275,
-0.994495413,-0.99266055,-0.990825688,-0.988990826,-0.987155963,-0.985321101,
-0.983486239,-0.981651376,-0.979816514,-0.977981651,-0.976146789,-0.974311927,
-0.972477064,-0.970642202,-0.968807339,-0.966972477,-0.965137615,-0.963302752,
-0.96146789,-0.959633028,-0.957798165,-0.955963303,-0.95412844,-0.952293578,
-0.950458716,-0.948623853,-0.946788991,-0.944954128,-0.943119266,-0.941284404,
-0.939449541,-0.937614679,-0.935779817,-0.933944954,-0.932110092,-0.930275229,
-0.928440367,-0.926605505,-0.924770642,-0.92293578,-0.921100917,-0.919266055,
-0.917431193,-0.91559633,-0.913761468,-0.911926606,-0.910091743,-0.908256881,
-0.906422018,-0.904587156,-0.902752294,-0.900917431,-0.899082569,-0.897247706,
-0.895412844,-0.893577982,-0.891743119,-0.889908257,-0.888073394,-0.886238532,
-0.88440367,-0.882568807,-0.880733945,-0.878899083,-0.87706422,-0.875229358,
-0.873394495,-0.871559633,-0.869724771,-0.867889908,-0.866055046,-0.864220183,
-0.862385321,-0.860550459,-0.858715596,-0.856880734,-0.855045872,-0.853211009,
-0.851376147,-0.849541284,-0.847706422,-0.84587156,-0.844036697,-0.842201835,
-0.840366972,-0.83853211,-0.836697248,-0.834862385,-0.833027523,-0.831192661,
-0.829357798,-0.827522936,-0.825688073,-0.823853211,-0.822018349,-0.820183486,
-0.818348624,-0.816513761,-0.814678899,-0.812844037,-0.811009174,-0.809174312,
-0.80733945,-0.805504587,-0.803669725,-0.801834862,-0.8,-0.798165138,-0.796330275,
-0.794495413,-0.79266055,-0.790825688,-0.788990826,-0.787155963,-0.785321101,
-0.783486239,-0.781651376,-0.779816514,-0.777981651,-0.776146789,-0.774311927,
-0.772477064,-0.770642202,-0.768807339,-0.766972477,-0.765137615,-0.763302752,
-0.76146789,-0.759633028,-0.757798165,-0.755963303,-0.75412844,-0.752293578,
-0.750458716,-0.748623853,-0.746788991,-0.744954128,-0.743119266,-0.741284404,
-0.739449541,-0.737614679,-0.735779817,-0.733944954,-0.732110092,-0.730275229,
-0.728440367,-0.726605505,-0.724770642,-0.72293578,-0.721100917,-0.719266055,
-0.717431193,-0.71559633,-0.713761468,-0.711926606,-0.710091743,-0.708256881,
-0.706422018,-0.704587156,-0.702752294,-0.700917431,-0.699082569,-0.697247706,
-0.695412844,-0.693577982,-0.691743119,-0.689908257,-0.688073394,-0.686238532,
-0.68440367,-0.682568807,-0.680733945,-0.678899083,-0.67706422,-0.675229358,
-0.673394495,-0.671559633,-0.669724771,-0.667889908,-0.666055046,-0.664220183,
-0.662385321,-0.660550459,-0.658715596,-0.656880734,-0.655045872,-0.653211009,
-0.651376147,-0.649541284,-0.647706422,-0.64587156,-0.644036697,-0.642201835,
-0.640366972,-0.63853211,-0.636697248,-0.634862385,-0.633027523,-0.631192661,
-0.629357798,-0.627522936,-0.625688073,-0.623853211,-0.622018349,-0.620183486,
-0.618348624,-0.616513761,-0.614678899,-0.612844037,-0.611009174,-0.609174312,
-0.60733945,-0.605504587,-0.603669725,-0.601834862,-0.6,-0.598165138,-0.596330275,
-0.594495413,-0.59266055,-0.590825688,-0.588990826,-0.587155963,-0.585321101,
-0.583486239,-0.581651376,-0.579816514,-0.577981651,-0.576146789,-0.574311927,
-0.572477064,-0.570642202,-0.568807339,-0.566972477,-0.565137615,-0.563302752,
-0.56146789,-0.559633028,-0.557798165,-0.555963303,-0.55412844,-0.552293578,
-0.550458716,-0.548623853,-0.546788991,-0.544954128,-0.543119266,-0.541284404,
-0.539449541,-0.537614679,-0.535779817,-0.533944954,-0.532110092,-0.530275229,
-0.528440367,-0.526605505,-0.524770642,-0.52293578,-0.521100917,-0.519266055,
-0.517431193,-0.51559633,-0.513761468,-0.511926606,-0.510091743,-0.508256881,
-0.506422018,-0.504587156,-0.502752294,-0.500917431,-0.499082569,-0.497247706,
-0.495412844,-0.493577982,-0.491743119,-0.489908257,-0.488073394,-0.486238532,
-0.48440367,-0.482568807,-0.480733945,-0.478899083,-0.47706422,-0.475229358,
-0.473394495,-0.471559633,-0.469724771,-0.467889908,-0.466055046,-0.464220183,
-0.462385321,-0.460550459,-0.458715596,-0.456880734,-0.455045872,-0.453211009,
-0.451376147,-0.449541284,-0.447706422,-0.44587156,-0.444036697,-0.442201835,
-0.440366972,-0.43853211,-0.436697248,-0.434862385,-0.433027523,-0.431192661,
-0.429357798,-0.427522936,-0.425688073,-0.423853211,-0.422018349,-0.420183486,
-0.418348624,-0.416513761,-0.414678899,-0.412844037,-0.411009174,-0.409174312,
-0.40733945,-0.405504587,-0.403669725,-0.401834862,-0.4,-0.398165138,-0.396330275,
-0.394495413,-0.39266055,-0.390825688,-0.388990826,-0.387155963,-0.385321101,
-0.383486239,-0.381651376,-0.379816514,-0.377981651,-0.376146789,-0.374311927,
-0.372477064,-0.370642202,-0.368807339,-0.366972477,-0.365137615,-0.363302752,
-0.36146789,-0.359633028,-0.357798165,-0.355963303,-0.35412844,-0.352293578,
-0.350458716,-0.348623853,-0.346788991,-0.344954128,-0.343119266,-0.341284404,
-0.339449541,-0.337614679,-0.335779817,-0.333944954,-0.332110092,-0.330275229,
-0.328440367,-0.326605505,-0.324770642,-0.32293578,-0.321100917,-0.319266055,
-0.317431193,-0.31559633,-0.313761468,-0.311926606,-0.310091743,-0.308256881,
-0.306422018,-0.304587156,-0.302752294,-0.300917431,-0.299082569,-0.297247706,
-0.295412844,-0.293577982,-0.291743119,-0.289908257,-0.288073394,-0.286238532,
-0.28440367,-0.282568807,-0.280733945,-0.278899083,-0.27706422,-0.275229358,
-0.273394495,-0.271559633,-0.269724771,-0.267889908,-0.266055046,-0.264220183,
-0.262385321,-0.260550459,-0.258715596,-0.256880734,-0.255045872,-0.253211009,
-0.251376147,-0.249541284,-0.247706422,-0.24587156,-0.244036697,-0.242201835,
-0.240366972,-0.23853211,-0.236697248,-0.234862385,-0.233027523,-0.231192661,
-0.229357798,-0.227522936,-0.225688073,-0.223853211,-0.222018349,-0.220183486,
-0.218348624,-0.216513761,-0.214678899,-0.212844037,-0.211009174,-0.209174312,
-0.20733945,-0.205504587,-0.203669725,-0.201834862,-0.2,-0.198165138,-0.196330275,
-0.194495413,-0.19266055,-0.190825688,-0.188990826,-0.187155963,-0.185321101,
-0.183486239,-0.181651376,-0.179816514,-0.177981651,-0.176146789,-0.174311927,
-0.172477064,-0.170642202,-0.168807339,-0.166972477,-0.165137615,-0.163302752,
-0.16146789,-0.159633028,-0.157798165,-0.155963303,-0.15412844,-0.152293578,
-0.150458716,-0.148623853,-0.146788991,-0.144954128,-0.143119266,-0.141284404,
-0.139449541,-0.137614679,-0.135779817,-0.133944954,-0.132110092,-0.130275229,
-0.128440367,-0.126605505,-0.124770642,-0.12293578,-0.121100917,-0.119266055,
-0.117431193,-0.11559633,-0.113761468,-0.111926606,-0.110091743,-0.108256881,
-0.106422018,-0.104587156,-0.102752294,-0.100917431,-0.099082569,-0.097247706,
-0.095412844,-0.093577982,-0.091743119,-0.089908257,-0.088073394,-0.086238532,
-0.08440367,-0.082568807,-0.080733945,-0.078899083,-0.07706422,-0.075229358,
-0.073394495,-0.071559633,-0.069724771,-0.067889908,-0.066055046,-0.064220183,
-0.062385321,-0.060550459,-0.058715596,-0.056880734,-0.055045872,-0.053211009,
-0.051376147,-0.049541284,-0.047706422,-0.04587156,-0.044036697,-0.042201835,
-0.040366972,-0.03853211,-0.036697248,-0.034862385,-0.033027523,-0.031192661,
-0.029357798,-0.027522936,-0.025688073,-0.023853211,-0.022018349,-0.020183486,
-0.018348624,-0.016513761,-0.014678899,-0.012844037,-0.011009174,-0.009174312,
-0.00733945,-0.005504587,-0.003669725,-0.001834862,0.00098215),(0.3,1.,
1.3),.UNSPECIFIED.);
#6330=B_SPLINE_SURFACE_WITH_KNOTS('',5,1,((#346562,#346563,#346564),(#346565,
#346566,#346567),(#346568,#346569,#346570),(#346571,#346572,#346573),(#346574,
#346575,#346576),(#346577,#346578,#346579),(#346580,#346581,#346582),(#346583,
#346584,#346585),(#346586,#346587,#346588),(#346589,#346590,#346591),(#346592,
#346593,#346594),(#346595,#346596,#346597),(#346598,#346599,#346600),(#346601,
#346602,#346603),(#346604,#346605,#346606),(#346607,#346608,#346609),(#346610,
#346611,#346612),(#346613,#346614,#346615),(#346616,#346617,#346618),(#346619,
#346620,#346621),(#346622,#346623,#346624),(#346625,#346626,#346627),(#346628,
#346629,#346630),(#346631,#346632,#346633),(#346634,#346635,#346636),(#346637,
#346638,#346639),(#346640,#346641,#346642),(#346643,#346644,#346645),(#346646,
#346647,#346648),(#346649,#346650,#346651),(#346652,#346653,#346654),(#346655,
#346656,#346657),(#346658,#346659,#346660),(#346661,#346662,#346663),(#346664,
#346665,#346666),(#346667,#346668,#346669),(#346670,#346671,#346672),(#346673,
#346674,#346675),(#346676,#346677,#346678),(#346679,#346680,#346681),(#346682,
#346683,#346684),(#346685,#346686,#346687),(#346688,#346689,#346690),(#346691,
#346692,#346693),(#346694,#346695,#346696),(#346697,#346698,#346699),(#346700,
#346701,#346702),(#346703,#346704,#346705),(#346706,#346707,#346708),(#346709,
#346710,#346711),(#346712,#346713,#346714),(#346715,#346716,#346717),(#346718,
#346719,#346720),(#346721,#346722,#346723),(#346724,#346725,#346726),(#346727,
#346728,#346729),(#346730,#346731,#346732),(#346733,#346734,#346735),(#346736,
#346737,#346738),(#346739,#346740,#346741),(#346742,#346743,#346744),(#346745,
#346746,#346747),(#346748,#346749,#346750),(#346751,#346752,#346753),(#346754,
#346755,#346756),(#346757,#346758,#346759),(#346760,#346761,#346762),(#346763,
#346764,#346765),(#346766,#346767,#346768),(#346769,#346770,#346771),(#346772,
#346773,#346774),(#346775,#346776,#346777),(#346778,#346779,#346780),(#346781,
#346782,#346783),(#346784,#346785,#346786),(#346787,#346788,#346789),(#346790,
#346791,#346792),(#346793,#346794,#346795),(#346796,#346797,#346798),(#346799,
#346800,#346801),(#346802,#346803,#346804),(#346805,#346806,#346807),(#346808,
#346809,#346810),(#346811,#346812,#346813),(#346814,#346815,#346816),(#346817,
#346818,#346819),(#346820,#346821,#346822),(#346823,#346824,#346825),(#346826,
#346827,#346828),(#346829,#346830,#346831),(#346832,#346833,#346834),(#346835,
#346836,#346837),(#346838,#346839,#346840),(#346841,#346842,#346843),(#346844,
#346845,#346846),(#346847,#346848,#346849),(#346850,#346851,#346852),(#346853,
#346854,#346855),(#346856,#346857,#346858),(#346859,#346860,#346861),(#346862,
#346863,#346864),(#346865,#346866,#346867),(#346868,#346869,#346870),(#346871,
#346872,#346873),(#346874,#346875,#346876),(#346877,#346878,#346879),(#346880,
#346881,#346882),(#346883,#346884,#346885),(#346886,#346887,#346888),(#346889,
#346890,#346891),(#346892,#346893,#346894),(#346895,#346896,#346897),(#346898,
#346899,#346900),(#346901,#346902,#346903),(#346904,#346905,#346906),(#346907,
#346908,#346909),(#346910,#346911,#346912),(#346913,#346914,#346915),(#346916,
#346917,#346918),(#346919,#346920,#346921),(#346922,#346923,#346924),(#346925,
#346926,#346927),(#346928,#346929,#346930),(#346931,#346932,#346933),(#346934,
#346935,#346936),(#346937,#346938,#346939),(#346940,#346941,#346942),(#346943,
#346944,#346945),(#346946,#346947,#346948),(#346949,#346950,#346951),(#346952,
#346953,#346954),(#346955,#346956,#346957),(#346958,#346959,#346960),(#346961,
#346962,#346963),(#346964,#346965,#346966),(#346967,#346968,#346969),(#346970,
#346971,#346972),(#346973,#346974,#346975),(#346976,#346977,#346978),(#346979,
#346980,#346981),(#346982,#346983,#346984),(#346985,#346986,#346987),(#346988,
#346989,#346990),(#346991,#346992,#346993),(#346994,#346995,#346996),(#346997,
#346998,#346999),(#347000,#347001,#347002),(#347003,#347004,#347005),(#347006,
#347007,#347008),(#347009,#347010,#347011),(#347012,#347013,#347014),(#347015,
#347016,#347017),(#347018,#347019,#347020),(#347021,#347022,#347023),(#347024,
#347025,#347026),(#347027,#347028,#347029),(#347030,#347031,#347032),(#347033,
#347034,#347035),(#347036,#347037,#347038),(#347039,#347040,#347041),(#347042,
#347043,#347044),(#347045,#347046,#347047),(#347048,#347049,#347050),(#347051,
#347052,#347053),(#347054,#347055,#347056),(#347057,#347058,#347059),(#347060,
#347061,#347062),(#347063,#347064,#347065),(#347066,#347067,#347068),(#347069,
#347070,#347071),(#347072,#347073,#347074),(#347075,#347076,#347077),(#347078,
#347079,#347080),(#347081,#347082,#347083),(#347084,#347085,#347086),(#347087,
#347088,#347089),(#347090,#347091,#347092),(#347093,#347094,#347095),(#347096,
#347097,#347098),(#347099,#347100,#347101),(#347102,#347103,#347104),(#347105,
#347106,#347107),(#347108,#347109,#347110),(#347111,#347112,#347113),(#347114,
#347115,#347116),(#347117,#347118,#347119),(#347120,#347121,#347122),(#347123,
#347124,#347125),(#347126,#347127,#347128),(#347129,#347130,#347131),(#347132,
#347133,#347134),(#347135,#347136,#347137),(#347138,#347139,#347140),(#347141,
#347142,#347143),(#347144,#347145,#347146),(#347147,#347148,#347149),(#347150,
#347151,#347152),(#347153,#347154,#347155),(#347156,#347157,#347158),(#347159,
#347160,#347161),(#347162,#347163,#347164),(#347165,#347166,#347167),(#347168,
#347169,#347170),(#347171,#347172,#347173),(#347174,#347175,#347176),(#347177,
#347178,#347179),(#347180,#347181,#347182),(#347183,#347184,#347185),(#347186,
#347187,#347188),(#347189,#347190,#347191),(#347192,#347193,#347194),(#347195,
#347196,#347197),(#347198,#347199,#347200),(#347201,#347202,#347203),(#347204,
#347205,#347206),(#347207,#347208,#347209),(#347210,#347211,#347212),(#347213,
#347214,#347215),(#347216,#347217,#347218),(#347219,#347220,#347221),(#347222,
#347223,#347224),(#347225,#347226,#347227),(#347228,#347229,#347230),(#347231,
#347232,#347233),(#347234,#347235,#347236),(#347237,#347238,#347239),(#347240,
#347241,#347242),(#347243,#347244,#347245),(#347246,#347247,#347248),(#347249,
#347250,#347251),(#347252,#347253,#347254),(#347255,#347256,#347257),(#347258,
#347259,#347260),(#347261,#347262,#347263),(#347264,#347265,#347266),(#347267,
#347268,#347269),(#347270,#347271,#347272),(#347273,#347274,#347275),(#347276,
#347277,#347278),(#347279,#347280,#347281),(#347282,#347283,#347284),(#347285,
#347286,#347287),(#347288,#347289,#347290),(#347291,#347292,#347293),(#347294,
#347295,#347296),(#347297,#347298,#347299),(#347300,#347301,#347302),(#347303,
#347304,#347305),(#347306,#347307,#347308),(#347309,#347310,#347311),(#347312,
#347313,#347314),(#347315,#347316,#347317),(#347318,#347319,#347320),(#347321,
#347322,#347323),(#347324,#347325,#347326),(#347327,#347328,#347329),(#347330,
#347331,#347332),(#347333,#347334,#347335),(#347336,#347337,#347338),(#347339,
#347340,#347341),(#347342,#347343,#347344),(#347345,#347346,#347347),(#347348,
#347349,#347350),(#347351,#347352,#347353),(#347354,#347355,#347356),(#347357,
#347358,#347359),(#347360,#347361,#347362),(#347363,#347364,#347365),(#347366,
#347367,#347368),(#347369,#347370,#347371),(#347372,#347373,#347374),(#347375,
#347376,#347377),(#347378,#347379,#347380),(#347381,#347382,#347383),(#347384,
#347385,#347386),(#347387,#347388,#347389),(#347390,#347391,#347392),(#347393,
#347394,#347395),(#347396,#347397,#347398),(#347399,#347400,#347401),(#347402,
#347403,#347404),(#347405,#347406,#347407),(#347408,#347409,#347410),(#347411,
#347412,#347413),(#347414,#347415,#347416),(#347417,#347418,#347419),(#347420,
#347421,#347422),(#347423,#347424,#347425),(#347426,#347427,#347428),(#347429,
#347430,#347431),(#347432,#347433,#347434),(#347435,#347436,#347437),(#347438,
#347439,#347440),(#347441,#347442,#347443),(#347444,#347445,#347446),(#347447,
#347448,#347449),(#347450,#347451,#347452),(#347453,#347454,#347455),(#347456,
#347457,#347458),(#347459,#347460,#347461),(#347462,#347463,#347464),(#347465,
#347466,#347467),(#347468,#347469,#347470),(#347471,#347472,#347473),(#347474,
#347475,#347476),(#347477,#347478,#347479),(#347480,#347481,#347482),(#347483,
#347484,#347485),(#347486,#347487,#347488),(#347489,#347490,#347491),(#347492,
#347493,#347494),(#347495,#347496,#347497),(#347498,#347499,#347500),(#347501,
#347502,#347503),(#347504,#347505,#347506),(#347507,#347508,#347509),(#347510,
#347511,#347512),(#347513,#347514,#347515),(#347516,#347517,#347518),(#347519,
#347520,#347521),(#347522,#347523,#347524),(#347525,#347526,#347527),(#347528,
#347529,#347530),(#347531,#347532,#347533),(#347534,#347535,#347536),(#347537,
#347538,#347539),(#347540,#347541,#347542),(#347543,#347544,#347545),(#347546,
#347547,#347548),(#347549,#347550,#347551),(#347552,#347553,#347554),(#347555,
#347556,#347557),(#347558,#347559,#347560),(#347561,#347562,#347563),(#347564,
#347565,#347566),(#347567,#347568,#347569),(#347570,#347571,#347572),(#347573,
#347574,#347575),(#347576,#347577,#347578),(#347579,#347580,#347581),(#347582,
#347583,#347584),(#347585,#347586,#347587),(#347588,#347589,#347590),(#347591,
#347592,#347593),(#347594,#347595,#347596),(#347597,#347598,#347599),(#347600,
#347601,#347602),(#347603,#347604,#347605),(#347606,#347607,#347608),(#347609,
#347610,#347611),(#347612,#347613,#347614),(#347615,#347616,#347617),(#347618,
#347619,#347620),(#347621,#347622,#347623),(#347624,#347625,#347626),(#347627,
#347628,#347629),(#347630,#347631,#347632),(#347633,#347634,#347635),(#347636,
#347637,#347638),(#347639,#347640,#347641),(#347642,#347643,#347644),(#347645,
#347646,#347647),(#347648,#347649,#347650),(#347651,#347652,#347653),(#347654,
#347655,#347656),(#347657,#347658,#347659),(#347660,#347661,#347662),(#347663,
#347664,#347665),(#347666,#347667,#347668),(#347669,#347670,#347671),(#347672,
#347673,#347674),(#347675,#347676,#347677),(#347678,#347679,#347680),(#347681,
#347682,#347683),(#347684,#347685,#347686),(#347687,#347688,#347689),(#347690,
#347691,#347692),(#347693,#347694,#347695),(#347696,#347697,#347698),(#347699,
#347700,#347701),(#347702,#347703,#347704),(#347705,#347706,#347707),(#347708,
#347709,#347710),(#347711,#347712,#347713),(#347714,#347715,#347716),(#347717,
#347718,#347719),(#347720,#347721,#347722),(#347723,#347724,#347725),(#347726,
#347727,#347728),(#347729,#347730,#347731),(#347732,#347733,#347734),(#347735,
#347736,#347737),(#347738,#347739,#347740),(#347741,#347742,#347743),(#347744,
#347745,#347746),(#347747,#347748,#347749),(#347750,#347751,#347752),(#347753,
#347754,#347755),(#347756,#347757,#347758),(#347759,#347760,#347761),(#347762,
#347763,#347764),(#347765,#347766,#347767),(#347768,#347769,#347770),(#347771,
#347772,#347773),(#347774,#347775,#347776),(#347777,#347778,#347779),(#347780,
#347781,#347782),(#347783,#347784,#347785),(#347786,#347787,#347788),(#347789,
#347790,#347791),(#347792,#347793,#347794),(#347795,#347796,#347797),(#347798,
#347799,#347800),(#347801,#347802,#347803),(#347804,#347805,#347806),(#347807,
#347808,#347809),(#347810,#347811,#347812),(#347813,#347814,#347815),(#347816,
#347817,#347818),(#347819,#347820,#347821),(#347822,#347823,#347824),(#347825,
#347826,#347827),(#347828,#347829,#347830),(#347831,#347832,#347833),(#347834,
#347835,#347836),(#347837,#347838,#347839),(#347840,#347841,#347842),(#347843,
#347844,#347845),(#347846,#347847,#347848),(#347849,#347850,#347851),(#347852,
#347853,#347854),(#347855,#347856,#347857),(#347858,#347859,#347860),(#347861,
#347862,#347863),(#347864,#347865,#347866),(#347867,#347868,#347869),(#347870,
#347871,#347872),(#347873,#347874,#347875),(#347876,#347877,#347878),(#347879,
#347880,#347881),(#347882,#347883,#347884),(#347885,#347886,#347887),(#347888,
#347889,#347890),(#347891,#347892,#347893),(#347894,#347895,#347896),(#347897,
#347898,#347899),(#347900,#347901,#347902),(#347903,#347904,#347905),(#347906,
#347907,#347908),(#347909,#347910,#347911),(#347912,#347913,#347914),(#347915,
#347916,#347917),(#347918,#347919,#347920),(#347921,#347922,#347923),(#347924,
#347925,#347926),(#347927,#347928,#347929),(#347930,#347931,#347932),(#347933,
#347934,#347935),(#347936,#347937,#347938),(#347939,#347940,#347941),(#347942,
#347943,#347944),(#347945,#347946,#347947),(#347948,#347949,#347950),(#347951,
#347952,#347953),(#347954,#347955,#347956),(#347957,#347958,#347959),(#347960,
#347961,#347962),(#347963,#347964,#347965),(#347966,#347967,#347968),(#347969,
#347970,#347971),(#347972,#347973,#347974),(#347975,#347976,#347977),(#347978,
#347979,#347980),(#347981,#347982,#347983),(#347984,#347985,#347986),(#347987,
#347988,#347989),(#347990,#347991,#347992),(#347993,#347994,#347995),(#347996,
#347997,#347998),(#347999,#348000,#348001),(#348002,#348003,#348004),(#348005,
#348006,#348007),(#348008,#348009,#348010),(#348011,#348012,#348013),(#348014,
#348015,#348016),(#348017,#348018,#348019),(#348020,#348021,#348022),(#348023,
#348024,#348025),(#348026,#348027,#348028),(#348029,#348030,#348031),(#348032,
#348033,#348034),(#348035,#348036,#348037),(#348038,#348039,#348040),(#348041,
#348042,#348043),(#348044,#348045,#348046),(#348047,#348048,#348049),(#348050,
#348051,#348052),(#348053,#348054,#348055),(#348056,#348057,#348058),(#348059,
#348060,#348061),(#348062,#348063,#348064),(#348065,#348066,#348067),(#348068,
#348069,#348070),(#348071,#348072,#348073),(#348074,#348075,#348076),(#348077,
#348078,#348079),(#348080,#348081,#348082),(#348083,#348084,#348085),(#348086,
#348087,#348088),(#348089,#348090,#348091),(#348092,#348093,#348094),(#348095,
#348096,#348097),(#348098,#348099,#348100),(#348101,#348102,#348103),(#348104,
#348105,#348106),(#348107,#348108,#348109),(#348110,#348111,#348112),(#348113,
#348114,#348115),(#348116,#348117,#348118),(#348119,#348120,#348121),(#348122,
#348123,#348124),(#348125,#348126,#348127),(#348128,#348129,#348130),(#348131,
#348132,#348133),(#348134,#348135,#348136),(#348137,#348138,#348139),(#348140,
#348141,#348142),(#348143,#348144,#348145),(#348146,#348147,#348148),(#348149,
#348150,#348151),(#348152,#348153,#348154),(#348155,#348156,#348157),(#348158,
#348159,#348160),(#348161,#348162,#348163),(#348164,#348165,#348166),(#348167,
#348168,#348169),(#348170,#348171,#348172),(#348173,#348174,#348175),(#348176,
#348177,#348178),(#348179,#348180,#348181),(#348182,#348183,#348184),(#348185,
#348186,#348187),(#348188,#348189,#348190),(#348191,#348192,#348193),(#348194,
#348195,#348196),(#348197,#348198,#348199),(#348200,#348201,#348202),(#348203,
#348204,#348205),(#348206,#348207,#348208),(#348209,#348210,#348211),(#348212,
#348213,#348214)),.UNSPECIFIED.,.F.,.F.,.F.,(6,1,1,1,1,1,1,1,1,1,1,1,1,
1,1,1,1,1,1,1,1,1,1,1,1,1,1,1,1,1,1,1,1,1,1,1,1,1,1,1,1,1,1,1,1,1,1,1,1,
1,1,1,1,1,1,1,1,1,1,1,1,1,1,1,1,1,1,1,1,1,1,1,1,1,1,1,1,1,1,1,1,1,1,1,1,
1,1,1,1,1,1,1,1,1,1,1,1,1,1,1,1,1,1,1,1,1,1,1,1,1,1,1,1,1,1,1,1,1,1,1,1,
1,1,1,1,1,1,1,1,1,1,1,1,1,1,1,1,1,1,1,1,1,1,1,1,1,1,1,1,1,1,1,1,1,1,1,1,
1,1,1,1,1,1,1,1,1,1,1,1,1,1,1,1,1,1,1,1,1,1,1,1,1,1,1,1,1,1,1,1,1,1,1,1,
1,1,1,1,1,1,1,1,1,1,1,1,1,1,1,1,1,1,1,1,1,1,1,1,1,1,1,1,1,1,1,1,1,1,1,1,
1,1,1,1,1,1,1,1,1,1,1,1,1,1,1,1,1,1,1,1,1,1,1,1,1,1,1,1,1,1,1,1,1,1,1,1,
1,1,1,1,1,1,1,1,1,1,1,1,1,1,1,1,1,1,1,1,1,1,1,1,1,1,1,1,1,1,1,1,1,1,1,1,
1,1,1,1,1,1,1,1,1,1,1,1,1,1,1,1,1,1,1,1,1,1,1,1,1,1,1,1,1,1,1,1,1,1,1,1,
1,1,1,1,1,1,1,1,1,1,1,1,1,1,1,1,1,1,1,1,1,1,1,1,1,1,1,1,1,1,1,1,1,1,1,1,
1,1,1,1,1,1,1,1,1,1,1,1,1,1,1,1,1,1,1,1,1,1,1,1,1,1,1,1,1,1,1,1,1,1,1,1,
1,1,1,1,1,1,1,1,1,1,1,1,1,1,1,1,1,1,1,1,1,1,1,1,1,1,1,1,1,1,1,1,1,1,1,1,
1,1,1,1,1,1,1,1,1,1,1,1,1,1,1,1,1,1,1,1,1,1,1,1,1,1,1,1,1,1,1,1,1,1,1,1,
1,1,1,1,1,1,1,1,1,1,1,1,1,1,1,1,1,1,1,1,1,1,1,1,1,1,1,1,1,1,1,1,1,1,1,1,
1,1,1,1,1,1,1,1,1,1,1,1,1,1,1,1,1,1,1,1,1,1,1,1,1,1,1,1,1,6),(2,1,2),(-0.00196418,
0.,0.001834862,0.003669725,0.005504587,0.00733945,0.009174312,0.011009174,
0.012844037,0.014678899,0.016513761,0.018348624,0.020183486,0.022018349,
0.023853211,0.025688073,0.027522936,0.029357798,0.031192661,0.033027523,
0.034862385,0.036697248,0.03853211,0.040366972,0.042201835,0.044036697,
0.04587156,0.047706422,0.049541284,0.051376147,0.053211009,0.055045872,
0.056880734,0.058715596,0.060550459,0.062385321,0.064220183,0.066055046,
0.067889908,0.069724771,0.071559633,0.073394495,0.075229358,0.07706422,
0.078899083,0.080733945,0.082568807,0.08440367,0.086238532,0.088073394,
0.089908257,0.091743119,0.093577982,0.095412844,0.097247706,0.099082569,
0.100917431,0.102752294,0.104587156,0.106422018,0.108256881,0.110091743,
0.111926606,0.113761468,0.11559633,0.117431193,0.119266055,0.121100917,
0.12293578,0.124770642,0.126605505,0.128440367,0.130275229,0.132110092,
0.133944954,0.135779817,0.137614679,0.139449541,0.141284404,0.143119266,
0.144954128,0.146788991,0.148623853,0.150458716,0.152293578,0.15412844,
0.155963303,0.157798165,0.159633028,0.16146789,0.163302752,0.165137615,
0.166972477,0.168807339,0.170642202,0.172477064,0.174311927,0.176146789,
0.177981651,0.179816514,0.181651376,0.183486239,0.185321101,0.187155963,
0.188990826,0.190825688,0.19266055,0.194495413,0.196330275,0.198165138,
0.2,0.201834862,0.203669725,0.205504587,0.20733945,0.209174312,0.211009174,
0.212844037,0.214678899,0.216513761,0.218348624,0.220183486,0.222018349,
0.223853211,0.225688073,0.227522936,0.229357798,0.231192661,0.233027523,
0.234862385,0.236697248,0.23853211,0.240366972,0.242201835,0.244036697,
0.24587156,0.247706422,0.249541284,0.251376147,0.253211009,0.255045872,
0.256880734,0.258715596,0.260550459,0.262385321,0.264220183,0.266055046,
0.267889908,0.269724771,0.271559633,0.273394495,0.275229358,0.27706422,
0.278899083,0.280733945,0.282568807,0.28440367,0.286238532,0.288073394,
0.289908257,0.291743119,0.293577982,0.295412844,0.297247706,0.299082569,
0.300917431,0.302752294,0.304587156,0.306422018,0.308256881,0.310091743,
0.311926606,0.313761468,0.31559633,0.317431193,0.319266055,0.321100917,
0.32293578,0.324770642,0.326605505,0.328440367,0.330275229,0.332110092,
0.333944954,0.335779817,0.337614679,0.339449541,0.341284404,0.343119266,
0.344954128,0.346788991,0.348623853,0.350458716,0.352293578,0.35412844,
0.355963303,0.357798165,0.359633028,0.36146789,0.363302752,0.365137615,
0.366972477,0.368807339,0.370642202,0.372477064,0.374311927,0.376146789,
0.377981651,0.379816514,0.381651376,0.383486239,0.385321101,0.387155963,
0.388990826,0.390825688,0.39266055,0.394495413,0.396330275,0.398165138,
0.4,0.401834862,0.403669725,0.405504587,0.40733945,0.409174312,0.411009174,
0.412844037,0.414678899,0.416513761,0.418348624,0.420183486,0.422018349,
0.423853211,0.425688073,0.427522936,0.429357798,0.431192661,0.433027523,
0.434862385,0.436697248,0.43853211,0.440366972,0.442201835,0.444036697,
0.44587156,0.447706422,0.449541284,0.451376147,0.453211009,0.455045872,
0.456880734,0.458715596,0.460550459,0.462385321,0.464220183,0.466055046,
0.467889908,0.469724771,0.471559633,0.473394495,0.475229358,0.47706422,
0.478899083,0.480733945,0.482568807,0.48440367,0.486238532,0.488073394,
0.489908257,0.491743119,0.493577982,0.495412844,0.497247706,0.499082569,
0.500917431,0.502752294,0.504587156,0.506422018,0.508256881,0.510091743,
0.511926606,0.513761468,0.51559633,0.517431193,0.519266055,0.521100917,
0.52293578,0.524770642,0.526605505,0.528440367,0.530275229,0.532110092,
0.533944954,0.535779817,0.537614679,0.539449541,0.541284404,0.543119266,
0.544954128,0.546788991,0.548623853,0.550458716,0.552293578,0.55412844,
0.555963303,0.557798165,0.559633028,0.56146789,0.563302752,0.565137615,
0.566972477,0.568807339,0.570642202,0.572477064,0.574311927,0.576146789,
0.577981651,0.579816514,0.581651376,0.583486239,0.585321101,0.587155963,
0.588990826,0.590825688,0.59266055,0.594495413,0.596330275,0.598165138,
0.6,0.601834862,0.603669725,0.605504587,0.60733945,0.609174312,0.611009174,
0.612844037,0.614678899,0.616513761,0.618348624,0.620183486,0.622018349,
0.623853211,0.625688073,0.627522936,0.629357798,0.631192661,0.633027523,
0.634862385,0.636697248,0.63853211,0.640366972,0.642201835,0.644036697,
0.64587156,0.647706422,0.649541284,0.651376147,0.653211009,0.655045872,
0.656880734,0.658715596,0.660550459,0.662385321,0.664220183,0.666055046,
0.667889908,0.669724771,0.671559633,0.673394495,0.675229358,0.67706422,
0.678899083,0.680733945,0.682568807,0.68440367,0.686238532,0.688073394,
0.689908257,0.691743119,0.693577982,0.695412844,0.697247706,0.699082569,
0.700917431,0.702752294,0.704587156,0.706422018,0.708256881,0.710091743,
0.711926606,0.713761468,0.71559633,0.717431193,0.719266055,0.721100917,
0.72293578,0.724770642,0.726605505,0.728440367,0.730275229,0.732110092,
0.733944954,0.735779817,0.737614679,0.739449541,0.741284404,0.743119266,
0.744954128,0.746788991,0.748623853,0.750458716,0.752293578,0.75412844,
0.755963303,0.757798165,0.759633028,0.76146789,0.763302752,0.765137615,
0.766972477,0.768807339,0.770642202,0.772477064,0.774311927,0.776146789,
0.777981651,0.779816514,0.781651376,0.783486239,0.785321101,0.787155963,
0.788990826,0.790825688,0.79266055,0.794495413,0.796330275,0.798165138,
0.8,0.801834862,0.803669725,0.805504587,0.80733945,0.809174312,0.811009174,
0.812844037,0.814678899,0.816513761,0.818348624,0.820183486,0.822018349,
0.823853211,0.825688073,0.827522936,0.829357798,0.831192661,0.833027523,
0.834862385,0.836697248,0.83853211,0.840366972,0.842201835,0.844036697,
0.84587156,0.847706422,0.849541284,0.851376147,0.853211009,0.855045872,
0.856880734,0.858715596,0.860550459,0.862385321,0.864220183,0.866055046,
0.867889908,0.869724771,0.871559633,0.873394495,0.875229358,0.87706422,
0.878899083,0.880733945,0.882568807,0.88440367,0.886238532,0.888073394,
0.889908257,0.891743119,0.893577982,0.895412844,0.897247706,0.899082569,
0.900917431,0.902752294,0.904587156,0.906422018,0.908256881,0.910091743,
0.911926606,0.913761468,0.91559633,0.917431193,0.919266055,0.921100917,
0.92293578,0.924770642,0.926605505,0.928440367,0.930275229,0.932110092,
0.933944954,0.935779817,0.937614679,0.939449541,0.941284404,0.943119266,
0.944954128,0.946788991,0.948623853,0.950458716,0.952293578,0.95412844,
0.955963303,0.957798165,0.959633028,0.96146789,0.963302752,0.965137615,
0.966972477,0.968807339,0.970642202,0.972477064,0.974311927,0.976146789,
0.977981651,0.979816514,0.981651376,0.983486239,0.985321101,0.987155963,
0.988990826,0.990825688,0.99266055,0.994495413,0.996330275,0.998165138,
1.),(0.3,1.,1.3),.UNSPECIFIED.);
#6331=B_SPLINE_SURFACE_WITH_KNOTS('',5,1,((#348221,#348222,#348223),(#348224,
#348225,#348226),(#348227,#348228,#348229),(#348230,#348231,#348232),(#348233,
#348234,#348235),(#348236,#348237,#348238),(#348239,#348240,#348241),(#348242,
#348243,#348244),(#348245,#348246,#348247),(#348248,#348249,#348250),(#348251,
#348252,#348253),(#348254,#348255,#348256),(#348257,#348258,#348259),(#348260,
#348261,#348262),(#348263,#348264,#348265),(#348266,#348267,#348268),(#348269,
#348270,#348271),(#348272,#348273,#348274),(#348275,#348276,#348277),(#348278,
#348279,#348280),(#348281,#348282,#348283),(#348284,#348285,#348286),(#348287,
#348288,#348289),(#348290,#348291,#348292),(#348293,#348294,#348295),(#348296,
#348297,#348298),(#348299,#348300,#348301),(#348302,#348303,#348304),(#348305,
#348306,#348307),(#348308,#348309,#348310),(#348311,#348312,#348313),(#348314,
#348315,#348316),(#348317,#348318,#348319),(#348320,#348321,#348322),(#348323,
#348324,#348325),(#348326,#348327,#348328),(#348329,#348330,#348331),(#348332,
#348333,#348334),(#348335,#348336,#348337),(#348338,#348339,#348340),(#348341,
#348342,#348343),(#348344,#348345,#348346),(#348347,#348348,#348349),(#348350,
#348351,#348352),(#348353,#348354,#348355),(#348356,#348357,#348358),(#348359,
#348360,#348361),(#348362,#348363,#348364),(#348365,#348366,#348367),(#348368,
#348369,#348370),(#348371,#348372,#348373),(#348374,#348375,#348376),(#348377,
#348378,#348379),(#348380,#348381,#348382),(#348383,#348384,#348385),(#348386,
#348387,#348388),(#348389,#348390,#348391),(#348392,#348393,#348394),(#348395,
#348396,#348397),(#348398,#348399,#348400),(#348401,#348402,#348403),(#348404,
#348405,#348406),(#348407,#348408,#348409),(#348410,#348411,#348412),(#348413,
#348414,#348415),(#348416,#348417,#348418),(#348419,#348420,#348421),(#348422,
#348423,#348424),(#348425,#348426,#348427),(#348428,#348429,#348430),(#348431,
#348432,#348433),(#348434,#348435,#348436),(#348437,#348438,#348439),(#348440,
#348441,#348442),(#348443,#348444,#348445),(#348446,#348447,#348448),(#348449,
#348450,#348451),(#348452,#348453,#348454),(#348455,#348456,#348457),(#348458,
#348459,#348460),(#348461,#348462,#348463),(#348464,#348465,#348466),(#348467,
#348468,#348469),(#348470,#348471,#348472),(#348473,#348474,#348475),(#348476,
#348477,#348478),(#348479,#348480,#348481),(#348482,#348483,#348484),(#348485,
#348486,#348487),(#348488,#348489,#348490),(#348491,#348492,#348493),(#348494,
#348495,#348496),(#348497,#348498,#348499),(#348500,#348501,#348502),(#348503,
#348504,#348505),(#348506,#348507,#348508),(#348509,#348510,#348511),(#348512,
#348513,#348514),(#348515,#348516,#348517),(#348518,#348519,#348520),(#348521,
#348522,#348523),(#348524,#348525,#348526),(#348527,#348528,#348529),(#348530,
#348531,#348532),(#348533,#348534,#348535),(#348536,#348537,#348538),(#348539,
#348540,#348541),(#348542,#348543,#348544),(#348545,#348546,#348547),(#348548,
#348549,#348550),(#348551,#348552,#348553),(#348554,#348555,#348556),(#348557,
#348558,#348559),(#348560,#348561,#348562),(#348563,#348564,#348565),(#348566,
#348567,#348568),(#348569,#348570,#348571),(#348572,#348573,#348574),(#348575,
#348576,#348577),(#348578,#348579,#348580),(#348581,#348582,#348583),(#348584,
#348585,#348586),(#348587,#348588,#348589),(#348590,#348591,#348592),(#348593,
#348594,#348595),(#348596,#348597,#348598),(#348599,#348600,#348601),(#348602,
#348603,#348604),(#348605,#348606,#348607),(#348608,#348609,#348610),(#348611,
#348612,#348613),(#348614,#348615,#348616),(#348617,#348618,#348619),(#348620,
#348621,#348622),(#348623,#348624,#348625),(#348626,#348627,#348628),(#348629,
#348630,#348631),(#348632,#348633,#348634),(#348635,#348636,#348637),(#348638,
#348639,#348640),(#348641,#348642,#348643),(#348644,#348645,#348646),(#348647,
#348648,#348649),(#348650,#348651,#348652),(#348653,#348654,#348655),(#348656,
#348657,#348658),(#348659,#348660,#348661),(#348662,#348663,#348664),(#348665,
#348666,#348667),(#348668,#348669,#348670),(#348671,#348672,#348673),(#348674,
#348675,#348676),(#348677,#348678,#348679),(#348680,#348681,#348682),(#348683,
#348684,#348685),(#348686,#348687,#348688),(#348689,#348690,#348691),(#348692,
#348693,#348694),(#348695,#348696,#348697),(#348698,#348699,#348700),(#348701,
#348702,#348703),(#348704,#348705,#348706),(#348707,#348708,#348709),(#348710,
#348711,#348712),(#348713,#348714,#348715),(#348716,#348717,#348718),(#348719,
#348720,#348721),(#348722,#348723,#348724),(#348725,#348726,#348727),(#348728,
#348729,#348730),(#348731,#348732,#348733),(#348734,#348735,#348736),(#348737,
#348738,#348739),(#348740,#348741,#348742),(#348743,#348744,#348745),(#348746,
#348747,#348748),(#348749,#348750,#348751),(#348752,#348753,#348754),(#348755,
#348756,#348757),(#348758,#348759,#348760),(#348761,#348762,#348763),(#348764,
#348765,#348766),(#348767,#348768,#348769),(#348770,#348771,#348772),(#348773,
#348774,#348775),(#348776,#348777,#348778),(#348779,#348780,#348781),(#348782,
#348783,#348784),(#348785,#348786,#348787),(#348788,#348789,#348790),(#348791,
#348792,#348793),(#348794,#348795,#348796),(#348797,#348798,#348799),(#348800,
#348801,#348802),(#348803,#348804,#348805),(#348806,#348807,#348808),(#348809,
#348810,#348811),(#348812,#348813,#348814),(#348815,#348816,#348817),(#348818,
#348819,#348820),(#348821,#348822,#348823),(#348824,#348825,#348826),(#348827,
#348828,#348829),(#348830,#348831,#348832),(#348833,#348834,#348835),(#348836,
#348837,#348838),(#348839,#348840,#348841),(#348842,#348843,#348844),(#348845,
#348846,#348847),(#348848,#348849,#348850),(#348851,#348852,#348853),(#348854,
#348855,#348856),(#348857,#348858,#348859),(#348860,#348861,#348862),(#348863,
#348864,#348865),(#348866,#348867,#348868),(#348869,#348870,#348871),(#348872,
#348873,#348874),(#348875,#348876,#348877),(#348878,#348879,#348880),(#348881,
#348882,#348883),(#348884,#348885,#348886),(#348887,#348888,#348889),(#348890,
#348891,#348892),(#348893,#348894,#348895),(#348896,#348897,#348898),(#348899,
#348900,#348901),(#348902,#348903,#348904),(#348905,#348906,#348907),(#348908,
#348909,#348910),(#348911,#348912,#348913),(#348914,#348915,#348916),(#348917,
#348918,#348919),(#348920,#348921,#348922),(#348923,#348924,#348925),(#348926,
#348927,#348928),(#348929,#348930,#348931),(#348932,#348933,#348934),(#348935,
#348936,#348937),(#348938,#348939,#348940),(#348941,#348942,#348943),(#348944,
#348945,#348946),(#348947,#348948,#348949),(#348950,#348951,#348952),(#348953,
#348954,#348955),(#348956,#348957,#348958),(#348959,#348960,#348961),(#348962,
#348963,#348964),(#348965,#348966,#348967),(#348968,#348969,#348970),(#348971,
#348972,#348973),(#348974,#348975,#348976),(#348977,#348978,#348979),(#348980,
#348981,#348982),(#348983,#348984,#348985),(#348986,#348987,#348988),(#348989,
#348990,#348991),(#348992,#348993,#348994),(#348995,#348996,#348997),(#348998,
#348999,#349000),(#349001,#349002,#349003),(#349004,#349005,#349006),(#349007,
#349008,#349009),(#349010,#349011,#349012),(#349013,#349014,#349015),(#349016,
#349017,#349018),(#349019,#349020,#349021),(#349022,#349023,#349024),(#349025,
#349026,#349027),(#349028,#349029,#349030),(#349031,#349032,#349033),(#349034,
#349035,#349036),(#349037,#349038,#349039),(#349040,#349041,#349042),(#349043,
#349044,#349045),(#349046,#349047,#349048),(#349049,#349050,#349051),(#349052,
#349053,#349054),(#349055,#349056,#349057),(#349058,#349059,#349060),(#349061,
#349062,#349063),(#349064,#349065,#349066),(#349067,#349068,#349069),(#349070,
#349071,#349072),(#349073,#349074,#349075),(#349076,#349077,#349078),(#349079,
#349080,#349081),(#349082,#349083,#349084),(#349085,#349086,#349087),(#349088,
#349089,#349090),(#349091,#349092,#349093),(#349094,#349095,#349096),(#349097,
#349098,#349099),(#349100,#349101,#349102),(#349103,#349104,#349105),(#349106,
#349107,#349108),(#349109,#349110,#349111),(#349112,#349113,#349114),(#349115,
#349116,#349117),(#349118,#349119,#349120),(#349121,#349122,#349123),(#349124,
#349125,#349126),(#349127,#349128,#349129),(#349130,#349131,#349132),(#349133,
#349134,#349135),(#349136,#349137,#349138),(#349139,#349140,#349141),(#349142,
#349143,#349144),(#349145,#349146,#349147),(#349148,#349149,#349150),(#349151,
#349152,#349153),(#349154,#349155,#349156),(#349157,#349158,#349159),(#349160,
#349161,#349162),(#349163,#349164,#349165),(#349166,#349167,#349168),(#349169,
#349170,#349171),(#349172,#349173,#349174),(#349175,#349176,#349177),(#349178,
#349179,#349180),(#349181,#349182,#349183),(#349184,#349185,#349186),(#349187,
#349188,#349189),(#349190,#349191,#349192),(#349193,#349194,#349195),(#349196,
#349197,#349198),(#349199,#349200,#349201),(#349202,#349203,#349204),(#349205,
#349206,#349207),(#349208,#349209,#349210),(#349211,#349212,#349213),(#349214,
#349215,#349216),(#349217,#349218,#349219),(#349220,#349221,#349222),(#349223,
#349224,#349225),(#349226,#349227,#349228),(#349229,#349230,#349231),(#349232,
#349233,#349234),(#349235,#349236,#349237),(#349238,#349239,#349240),(#349241,
#349242,#349243),(#349244,#349245,#349246),(#349247,#349248,#349249),(#349250,
#349251,#349252),(#349253,#349254,#349255),(#349256,#349257,#349258),(#349259,
#349260,#349261),(#349262,#349263,#349264),(#349265,#349266,#349267),(#349268,
#349269,#349270),(#349271,#349272,#349273),(#349274,#349275,#349276),(#349277,
#349278,#349279),(#349280,#349281,#349282),(#349283,#349284,#349285),(#349286,
#349287,#349288),(#349289,#349290,#349291),(#349292,#349293,#349294),(#349295,
#349296,#349297),(#349298,#349299,#349300),(#349301,#349302,#349303),(#349304,
#349305,#349306),(#349307,#349308,#349309),(#349310,#349311,#349312),(#349313,
#349314,#349315),(#349316,#349317,#349318),(#349319,#349320,#349321),(#349322,
#349323,#349324),(#349325,#349326,#349327),(#349328,#349329,#349330),(#349331,
#349332,#349333),(#349334,#349335,#349336),(#349337,#349338,#349339),(#349340,
#349341,#349342),(#349343,#349344,#349345),(#349346,#349347,#349348),(#349349,
#349350,#349351),(#349352,#349353,#349354),(#349355,#349356,#349357),(#349358,
#349359,#349360),(#349361,#349362,#349363),(#349364,#349365,#349366),(#349367,
#349368,#349369),(#349370,#349371,#349372),(#349373,#349374,#349375),(#349376,
#349377,#349378),(#349379,#349380,#349381),(#349382,#349383,#349384),(#349385,
#349386,#349387),(#349388,#349389,#349390),(#349391,#349392,#349393),(#349394,
#349395,#349396),(#349397,#349398,#349399),(#349400,#349401,#349402),(#349403,
#349404,#349405),(#349406,#349407,#349408),(#349409,#349410,#349411),(#349412,
#349413,#349414),(#349415,#349416,#349417),(#349418,#349419,#349420),(#349421,
#349422,#349423),(#349424,#349425,#349426),(#349427,#349428,#349429),(#349430,
#349431,#349432),(#349433,#349434,#349435),(#349436,#349437,#349438),(#349439,
#349440,#349441),(#349442,#349443,#349444),(#349445,#349446,#349447),(#349448,
#349449,#349450),(#349451,#349452,#349453),(#349454,#349455,#349456),(#349457,
#349458,#349459),(#349460,#349461,#349462),(#349463,#349464,#349465),(#349466,
#349467,#349468),(#349469,#349470,#349471),(#349472,#349473,#349474),(#349475,
#349476,#349477),(#349478,#349479,#349480),(#349481,#349482,#349483),(#349484,
#349485,#349486),(#349487,#349488,#349489),(#349490,#349491,#349492),(#349493,
#349494,#349495),(#349496,#349497,#349498),(#349499,#349500,#349501),(#349502,
#349503,#349504),(#349505,#349506,#349507),(#349508,#349509,#349510),(#349511,
#349512,#349513),(#349514,#349515,#349516),(#349517,#349518,#349519),(#349520,
#349521,#349522),(#349523,#349524,#349525),(#349526,#349527,#349528),(#349529,
#349530,#349531),(#349532,#349533,#349534),(#349535,#349536,#349537),(#349538,
#349539,#349540),(#349541,#349542,#349543),(#349544,#349545,#349546),(#349547,
#349548,#349549),(#349550,#349551,#349552),(#349553,#349554,#349555),(#349556,
#349557,#349558),(#349559,#349560,#349561),(#349562,#349563,#349564),(#349565,
#349566,#349567),(#349568,#349569,#349570),(#349571,#349572,#349573),(#349574,
#349575,#349576),(#349577,#349578,#349579),(#349580,#349581,#349582),(#349583,
#349584,#349585),(#349586,#349587,#349588),(#349589,#349590,#349591),(#349592,
#349593,#349594),(#349595,#349596,#349597),(#349598,#349599,#349600),(#349601,
#349602,#349603),(#349604,#349605,#349606),(#349607,#349608,#349609),(#349610,
#349611,#349612),(#349613,#349614,#349615),(#349616,#349617,#349618),(#349619,
#349620,#349621),(#349622,#349623,#349624),(#349625,#349626,#349627),(#349628,
#349629,#349630),(#349631,#349632,#349633),(#349634,#349635,#349636),(#349637,
#349638,#349639),(#349640,#349641,#349642),(#349643,#349644,#349645),(#349646,
#349647,#349648),(#349649,#349650,#349651),(#349652,#349653,#349654),(#349655,
#349656,#349657),(#349658,#349659,#349660),(#349661,#349662,#349663),(#349664,
#349665,#349666),(#349667,#349668,#349669),(#349670,#349671,#349672),(#349673,
#349674,#349675),(#349676,#349677,#349678),(#349679,#349680,#349681),(#349682,
#349683,#349684),(#349685,#349686,#349687),(#349688,#349689,#349690),(#349691,
#349692,#349693),(#349694,#349695,#349696),(#349697,#349698,#349699),(#349700,
#349701,#349702),(#349703,#349704,#349705),(#349706,#349707,#349708),(#349709,
#349710,#349711),(#349712,#349713,#349714),(#349715,#349716,#349717),(#349718,
#349719,#349720),(#349721,#349722,#349723),(#349724,#349725,#349726),(#349727,
#349728,#349729),(#349730,#349731,#349732),(#349733,#349734,#349735),(#349736,
#349737,#349738),(#349739,#349740,#349741),(#349742,#349743,#349744),(#349745,
#349746,#349747),(#349748,#349749,#349750),(#349751,#349752,#349753),(#349754,
#349755,#349756),(#349757,#349758,#349759),(#349760,#349761,#349762),(#349763,
#349764,#349765),(#349766,#349767,#349768),(#349769,#349770,#349771),(#349772,
#349773,#349774),(#349775,#349776,#349777),(#349778,#349779,#349780),(#349781,
#349782,#349783),(#349784,#349785,#349786),(#349787,#349788,#349789),(#349790,
#349791,#349792),(#349793,#349794,#349795),(#349796,#349797,#349798),(#349799,
#349800,#349801),(#349802,#349803,#349804),(#349805,#349806,#349807),(#349808,
#349809,#349810),(#349811,#349812,#349813),(#349814,#349815,#349816),(#349817,
#349818,#349819),(#349820,#349821,#349822),(#349823,#349824,#349825),(#349826,
#349827,#349828),(#349829,#349830,#349831),(#349832,#349833,#349834),(#349835,
#349836,#349837),(#349838,#349839,#349840),(#349841,#349842,#349843),(#349844,
#349845,#349846),(#349847,#349848,#349849),(#349850,#349851,#349852),(#349853,
#349854,#349855),(#349856,#349857,#349858),(#349859,#349860,#349861),(#349862,
#349863,#349864),(#349865,#349866,#349867),(#349868,#349869,#349870)),
 .UNSPECIFIED.,.F.,.F.,.F.,(6,1,1,1,1,1,1,1,1,1,1,1,1,1,1,1,1,1,1,1,1,1,
1,1,1,1,1,1,1,1,1,1,1,1,1,1,1,1,1,1,1,1,1,1,1,1,1,1,1,1,1,1,1,1,1,1,1,1,
1,1,1,1,1,1,1,1,1,1,1,1,1,1,1,1,1,1,1,1,1,1,1,1,1,1,1,1,1,1,1,1,1,1,1,1,
1,1,1,1,1,1,1,1,1,1,1,1,1,1,1,1,1,1,1,1,1,1,1,1,1,1,1,1,1,1,1,1,1,1,1,1,
1,1,1,1,1,1,1,1,1,1,1,1,1,1,1,1,1,1,1,1,1,1,1,1,1,1,1,1,1,1,1,1,1,1,1,1,
1,1,1,1,1,1,1,1,1,1,1,1,1,1,1,1,1,1,1,1,1,1,1,1,1,1,1,1,1,1,1,1,1,1,1,1,
1,1,1,1,1,1,1,1,1,1,1,1,1,1,1,1,1,1,1,1,1,1,1,1,1,1,1,1,1,1,1,1,1,1,1,1,
1,1,1,1,1,1,1,1,1,1,1,1,1,1,1,1,1,1,1,1,1,1,1,1,1,1,1,1,1,1,1,1,1,1,1,1,
1,1,1,1,1,1,1,1,1,1,1,1,1,1,1,1,1,1,1,1,1,1,1,1,1,1,1,1,1,1,1,1,1,1,1,1,
1,1,1,1,1,1,1,1,1,1,1,1,1,1,1,1,1,1,1,1,1,1,1,1,1,1,1,1,1,1,1,1,1,1,1,1,
1,1,1,1,1,1,1,1,1,1,1,1,1,1,1,1,1,1,1,1,1,1,1,1,1,1,1,1,1,1,1,1,1,1,1,1,
1,1,1,1,1,1,1,1,1,1,1,1,1,1,1,1,1,1,1,1,1,1,1,1,1,1,1,1,1,1,1,1,1,1,1,1,
1,1,1,1,1,1,1,1,1,1,1,1,1,1,1,1,1,1,1,1,1,1,1,1,1,1,1,1,1,1,1,1,1,1,1,1,
1,1,1,1,1,1,1,1,1,1,1,1,1,1,1,1,1,1,1,1,1,1,1,1,1,1,1,1,1,1,1,1,1,1,1,1,
1,1,1,1,1,1,1,1,1,1,1,1,1,1,1,1,1,1,1,1,1,1,1,1,1,1,1,1,1,1,1,1,1,1,1,1,
1,1,1,1,1,1,1,1,1,1,1,1,1,1,1,1,1,1,1,6),(2,1,2),(-1.,-0.998165138,-0.996330275,
-0.994495413,-0.99266055,-0.990825688,-0.988990826,-0.987155963,-0.985321101,
-0.983486239,-0.981651376,-0.979816514,-0.977981651,-0.976146789,-0.974311927,
-0.972477064,-0.970642202,-0.968807339,-0.966972477,-0.965137615,-0.963302752,
-0.96146789,-0.959633028,-0.957798165,-0.955963303,-0.95412844,-0.952293578,
-0.950458716,-0.948623853,-0.946788991,-0.944954128,-0.943119266,-0.941284404,
-0.939449541,-0.937614679,-0.935779817,-0.933944954,-0.932110092,-0.930275229,
-0.928440367,-0.926605505,-0.924770642,-0.92293578,-0.921100917,-0.919266055,
-0.917431193,-0.91559633,-0.913761468,-0.911926606,-0.910091743,-0.908256881,
-0.906422018,-0.904587156,-0.902752294,-0.900917431,-0.899082569,-0.897247706,
-0.895412844,-0.893577982,-0.891743119,-0.889908257,-0.888073394,-0.886238532,
-0.88440367,-0.882568807,-0.880733945,-0.878899083,-0.87706422,-0.875229358,
-0.873394495,-0.871559633,-0.869724771,-0.867889908,-0.866055046,-0.864220183,
-0.862385321,-0.860550459,-0.858715596,-0.856880734,-0.855045872,-0.853211009,
-0.851376147,-0.849541284,-0.847706422,-0.84587156,-0.844036697,-0.842201835,
-0.840366972,-0.83853211,-0.836697248,-0.834862385,-0.833027523,-0.831192661,
-0.829357798,-0.827522936,-0.825688073,-0.823853211,-0.822018349,-0.820183486,
-0.818348624,-0.816513761,-0.814678899,-0.812844037,-0.811009174,-0.809174312,
-0.80733945,-0.805504587,-0.803669725,-0.801834862,-0.8,-0.798165138,-0.796330275,
-0.794495413,-0.79266055,-0.790825688,-0.788990826,-0.787155963,-0.785321101,
-0.783486239,-0.781651376,-0.779816514,-0.777981651,-0.776146789,-0.774311927,
-0.772477064,-0.770642202,-0.768807339,-0.766972477,-0.765137615,-0.763302752,
-0.76146789,-0.759633028,-0.757798165,-0.755963303,-0.75412844,-0.752293578,
-0.750458716,-0.748623853,-0.746788991,-0.744954128,-0.743119266,-0.741284404,
-0.739449541,-0.737614679,-0.735779817,-0.733944954,-0.732110092,-0.730275229,
-0.728440367,-0.726605505,-0.724770642,-0.72293578,-0.721100917,-0.719266055,
-0.717431193,-0.71559633,-0.713761468,-0.711926606,-0.710091743,-0.708256881,
-0.706422018,-0.704587156,-0.702752294,-0.700917431,-0.699082569,-0.697247706,
-0.695412844,-0.693577982,-0.691743119,-0.689908257,-0.688073394,-0.686238532,
-0.68440367,-0.682568807,-0.680733945,-0.678899083,-0.67706422,-0.675229358,
-0.673394495,-0.671559633,-0.669724771,-0.667889908,-0.666055046,-0.664220183,
-0.662385321,-0.660550459,-0.658715596,-0.656880734,-0.655045872,-0.653211009,
-0.651376147,-0.649541284,-0.647706422,-0.64587156,-0.644036697,-0.642201835,
-0.640366972,-0.63853211,-0.636697248,-0.634862385,-0.633027523,-0.631192661,
-0.629357798,-0.627522936,-0.625688073,-0.623853211,-0.622018349,-0.620183486,
-0.618348624,-0.616513761,-0.614678899,-0.612844037,-0.611009174,-0.609174312,
-0.60733945,-0.605504587,-0.603669725,-0.601834862,-0.6,-0.598165138,-0.596330275,
-0.594495413,-0.59266055,-0.590825688,-0.588990826,-0.587155963,-0.585321101,
-0.583486239,-0.581651376,-0.579816514,-0.577981651,-0.576146789,-0.574311927,
-0.572477064,-0.570642202,-0.568807339,-0.566972477,-0.565137615,-0.563302752,
-0.56146789,-0.559633028,-0.557798165,-0.555963303,-0.55412844,-0.552293578,
-0.550458716,-0.548623853,-0.546788991,-0.544954128,-0.543119266,-0.541284404,
-0.539449541,-0.537614679,-0.535779817,-0.533944954,-0.532110092,-0.530275229,
-0.528440367,-0.526605505,-0.524770642,-0.52293578,-0.521100917,-0.519266055,
-0.517431193,-0.51559633,-0.513761468,-0.511926606,-0.510091743,-0.508256881,
-0.506422018,-0.504587156,-0.502752294,-0.500917431,-0.499082569,-0.497247706,
-0.495412844,-0.493577982,-0.491743119,-0.489908257,-0.488073394,-0.486238532,
-0.48440367,-0.482568807,-0.480733945,-0.478899083,-0.47706422,-0.475229358,
-0.473394495,-0.471559633,-0.469724771,-0.467889908,-0.466055046,-0.464220183,
-0.462385321,-0.460550459,-0.458715596,-0.456880734,-0.455045872,-0.453211009,
-0.451376147,-0.449541284,-0.447706422,-0.44587156,-0.444036697,-0.442201835,
-0.440366972,-0.43853211,-0.436697248,-0.434862385,-0.433027523,-0.431192661,
-0.429357798,-0.427522936,-0.425688073,-0.423853211,-0.422018349,-0.420183486,
-0.418348624,-0.416513761,-0.414678899,-0.412844037,-0.411009174,-0.409174312,
-0.40733945,-0.405504587,-0.403669725,-0.401834862,-0.4,-0.398165138,-0.396330275,
-0.394495413,-0.39266055,-0.390825688,-0.388990826,-0.387155963,-0.385321101,
-0.383486239,-0.381651376,-0.379816514,-0.377981651,-0.376146789,-0.374311927,
-0.372477064,-0.370642202,-0.368807339,-0.366972477,-0.365137615,-0.363302752,
-0.36146789,-0.359633028,-0.357798165,-0.355963303,-0.35412844,-0.352293578,
-0.350458716,-0.348623853,-0.346788991,-0.344954128,-0.343119266,-0.341284404,
-0.339449541,-0.337614679,-0.335779817,-0.333944954,-0.332110092,-0.330275229,
-0.328440367,-0.326605505,-0.324770642,-0.32293578,-0.321100917,-0.319266055,
-0.317431193,-0.31559633,-0.313761468,-0.311926606,-0.310091743,-0.308256881,
-0.306422018,-0.304587156,-0.302752294,-0.300917431,-0.299082569,-0.297247706,
-0.295412844,-0.293577982,-0.291743119,-0.289908257,-0.288073394,-0.286238532,
-0.28440367,-0.282568807,-0.280733945,-0.278899083,-0.27706422,-0.275229358,
-0.273394495,-0.271559633,-0.269724771,-0.267889908,-0.266055046,-0.264220183,
-0.262385321,-0.260550459,-0.258715596,-0.256880734,-0.255045872,-0.253211009,
-0.251376147,-0.249541284,-0.247706422,-0.24587156,-0.244036697,-0.242201835,
-0.240366972,-0.23853211,-0.236697248,-0.234862385,-0.233027523,-0.231192661,
-0.229357798,-0.227522936,-0.225688073,-0.223853211,-0.222018349,-0.220183486,
-0.218348624,-0.216513761,-0.214678899,-0.212844037,-0.211009174,-0.209174312,
-0.20733945,-0.205504587,-0.203669725,-0.201834862,-0.2,-0.198165138,-0.196330275,
-0.194495413,-0.19266055,-0.190825688,-0.188990826,-0.187155963,-0.185321101,
-0.183486239,-0.181651376,-0.179816514,-0.177981651,-0.176146789,-0.174311927,
-0.172477064,-0.170642202,-0.168807339,-0.166972477,-0.165137615,-0.163302752,
-0.16146789,-0.159633028,-0.157798165,-0.155963303,-0.15412844,-0.152293578,
-0.150458716,-0.148623853,-0.146788991,-0.144954128,-0.143119266,-0.141284404,
-0.139449541,-0.137614679,-0.135779817,-0.133944954,-0.132110092,-0.130275229,
-0.128440367,-0.126605505,-0.124770642,-0.12293578,-0.121100917,-0.119266055,
-0.117431193,-0.11559633,-0.113761468,-0.111926606,-0.110091743,-0.108256881,
-0.106422018,-0.104587156,-0.102752294,-0.100917431,-0.099082569,-0.097247706,
-0.095412844,-0.093577982,-0.091743119,-0.089908257,-0.088073394,-0.086238532,
-0.08440367,-0.082568807,-0.080733945,-0.078899083,-0.07706422,-0.075229358,
-0.073394495,-0.071559633,-0.069724771,-0.067889908,-0.066055046,-0.064220183,
-0.062385321,-0.060550459,-0.058715596,-0.056880734,-0.055045872,-0.053211009,
-0.051376147,-0.049541284,-0.047706422,-0.04587156,-0.044036697,-0.042201835,
-0.040366972,-0.03853211,-0.036697248,-0.034862385,-0.033027523,-0.031192661,
-0.029357798,-0.027522936,-0.025688073,-0.023853211,-0.022018349,-0.020183486,
-0.018348624,-0.016513761,-0.014678899,-0.012844037,-0.011009174,-0.009174312,
-0.00733945,-0.005504587,-0.003669725,-0.001834862,0.000982119),(0.3,1.,
1.3),.UNSPECIFIED.);
#6332=B_SPLINE_SURFACE_WITH_KNOTS('',5,1,((#349874,#349875,#349876),(#349877,
#349878,#349879),(#349880,#349881,#349882),(#349883,#349884,#349885),(#349886,
#349887,#349888),(#349889,#349890,#349891),(#349892,#349893,#349894),(#349895,
#349896,#349897),(#349898,#349899,#349900),(#349901,#349902,#349903),(#349904,
#349905,#349906),(#349907,#349908,#349909),(#349910,#349911,#349912),(#349913,
#349914,#349915),(#349916,#349917,#349918),(#349919,#349920,#349921),(#349922,
#349923,#349924),(#349925,#349926,#349927),(#349928,#349929,#349930),(#349931,
#349932,#349933),(#349934,#349935,#349936),(#349937,#349938,#349939),(#349940,
#349941,#349942),(#349943,#349944,#349945),(#349946,#349947,#349948),(#349949,
#349950,#349951),(#349952,#349953,#349954),(#349955,#349956,#349957),(#349958,
#349959,#349960),(#349961,#349962,#349963),(#349964,#349965,#349966),(#349967,
#349968,#349969),(#349970,#349971,#349972),(#349973,#349974,#349975),(#349976,
#349977,#349978),(#349979,#349980,#349981),(#349982,#349983,#349984),(#349985,
#349986,#349987),(#349988,#349989,#349990),(#349991,#349992,#349993),(#349994,
#349995,#349996),(#349997,#349998,#349999),(#350000,#350001,#350002),(#350003,
#350004,#350005),(#350006,#350007,#350008),(#350009,#350010,#350011),(#350012,
#350013,#350014),(#350015,#350016,#350017),(#350018,#350019,#350020),(#350021,
#350022,#350023),(#350024,#350025,#350026),(#350027,#350028,#350029),(#350030,
#350031,#350032),(#350033,#350034,#350035),(#350036,#350037,#350038),(#350039,
#350040,#350041),(#350042,#350043,#350044),(#350045,#350046,#350047),(#350048,
#350049,#350050),(#350051,#350052,#350053),(#350054,#350055,#350056),(#350057,
#350058,#350059),(#350060,#350061,#350062),(#350063,#350064,#350065),(#350066,
#350067,#350068),(#350069,#350070,#350071),(#350072,#350073,#350074),(#350075,
#350076,#350077),(#350078,#350079,#350080),(#350081,#350082,#350083),(#350084,
#350085,#350086),(#350087,#350088,#350089),(#350090,#350091,#350092),(#350093,
#350094,#350095),(#350096,#350097,#350098),(#350099,#350100,#350101),(#350102,
#350103,#350104),(#350105,#350106,#350107),(#350108,#350109,#350110),(#350111,
#350112,#350113),(#350114,#350115,#350116),(#350117,#350118,#350119),(#350120,
#350121,#350122),(#350123,#350124,#350125),(#350126,#350127,#350128),(#350129,
#350130,#350131),(#350132,#350133,#350134),(#350135,#350136,#350137),(#350138,
#350139,#350140),(#350141,#350142,#350143),(#350144,#350145,#350146),(#350147,
#350148,#350149),(#350150,#350151,#350152),(#350153,#350154,#350155),(#350156,
#350157,#350158),(#350159,#350160,#350161),(#350162,#350163,#350164),(#350165,
#350166,#350167),(#350168,#350169,#350170),(#350171,#350172,#350173),(#350174,
#350175,#350176),(#350177,#350178,#350179),(#350180,#350181,#350182),(#350183,
#350184,#350185),(#350186,#350187,#350188),(#350189,#350190,#350191),(#350192,
#350193,#350194),(#350195,#350196,#350197),(#350198,#350199,#350200),(#350201,
#350202,#350203),(#350204,#350205,#350206),(#350207,#350208,#350209),(#350210,
#350211,#350212),(#350213,#350214,#350215),(#350216,#350217,#350218),(#350219,
#350220,#350221),(#350222,#350223,#350224),(#350225,#350226,#350227),(#350228,
#350229,#350230),(#350231,#350232,#350233),(#350234,#350235,#350236),(#350237,
#350238,#350239),(#350240,#350241,#350242),(#350243,#350244,#350245),(#350246,
#350247,#350248),(#350249,#350250,#350251),(#350252,#350253,#350254),(#350255,
#350256,#350257),(#350258,#350259,#350260),(#350261,#350262,#350263),(#350264,
#350265,#350266),(#350267,#350268,#350269),(#350270,#350271,#350272),(#350273,
#350274,#350275),(#350276,#350277,#350278),(#350279,#350280,#350281),(#350282,
#350283,#350284),(#350285,#350286,#350287),(#350288,#350289,#350290),(#350291,
#350292,#350293),(#350294,#350295,#350296),(#350297,#350298,#350299),(#350300,
#350301,#350302),(#350303,#350304,#350305),(#350306,#350307,#350308),(#350309,
#350310,#350311),(#350312,#350313,#350314),(#350315,#350316,#350317),(#350318,
#350319,#350320),(#350321,#350322,#350323),(#350324,#350325,#350326),(#350327,
#350328,#350329),(#350330,#350331,#350332),(#350333,#350334,#350335),(#350336,
#350337,#350338),(#350339,#350340,#350341),(#350342,#350343,#350344),(#350345,
#350346,#350347),(#350348,#350349,#350350),(#350351,#350352,#350353),(#350354,
#350355,#350356),(#350357,#350358,#350359),(#350360,#350361,#350362),(#350363,
#350364,#350365),(#350366,#350367,#350368),(#350369,#350370,#350371),(#350372,
#350373,#350374),(#350375,#350376,#350377),(#350378,#350379,#350380),(#350381,
#350382,#350383),(#350384,#350385,#350386),(#350387,#350388,#350389),(#350390,
#350391,#350392),(#350393,#350394,#350395),(#350396,#350397,#350398),(#350399,
#350400,#350401),(#350402,#350403,#350404),(#350405,#350406,#350407),(#350408,
#350409,#350410),(#350411,#350412,#350413),(#350414,#350415,#350416),(#350417,
#350418,#350419),(#350420,#350421,#350422),(#350423,#350424,#350425),(#350426,
#350427,#350428),(#350429,#350430,#350431),(#350432,#350433,#350434),(#350435,
#350436,#350437),(#350438,#350439,#350440),(#350441,#350442,#350443),(#350444,
#350445,#350446),(#350447,#350448,#350449),(#350450,#350451,#350452),(#350453,
#350454,#350455),(#350456,#350457,#350458),(#350459,#350460,#350461),(#350462,
#350463,#350464),(#350465,#350466,#350467),(#350468,#350469,#350470),(#350471,
#350472,#350473),(#350474,#350475,#350476),(#350477,#350478,#350479),(#350480,
#350481,#350482),(#350483,#350484,#350485),(#350486,#350487,#350488),(#350489,
#350490,#350491),(#350492,#350493,#350494),(#350495,#350496,#350497),(#350498,
#350499,#350500),(#350501,#350502,#350503),(#350504,#350505,#350506),(#350507,
#350508,#350509),(#350510,#350511,#350512),(#350513,#350514,#350515),(#350516,
#350517,#350518),(#350519,#350520,#350521),(#350522,#350523,#350524),(#350525,
#350526,#350527),(#350528,#350529,#350530),(#350531,#350532,#350533),(#350534,
#350535,#350536),(#350537,#350538,#350539),(#350540,#350541,#350542),(#350543,
#350544,#350545),(#350546,#350547,#350548),(#350549,#350550,#350551),(#350552,
#350553,#350554),(#350555,#350556,#350557),(#350558,#350559,#350560),(#350561,
#350562,#350563),(#350564,#350565,#350566),(#350567,#350568,#350569),(#350570,
#350571,#350572),(#350573,#350574,#350575),(#350576,#350577,#350578),(#350579,
#350580,#350581),(#350582,#350583,#350584),(#350585,#350586,#350587),(#350588,
#350589,#350590),(#350591,#350592,#350593),(#350594,#350595,#350596),(#350597,
#350598,#350599),(#350600,#350601,#350602),(#350603,#350604,#350605),(#350606,
#350607,#350608),(#350609,#350610,#350611),(#350612,#350613,#350614),(#350615,
#350616,#350617),(#350618,#350619,#350620),(#350621,#350622,#350623),(#350624,
#350625,#350626),(#350627,#350628,#350629),(#350630,#350631,#350632),(#350633,
#350634,#350635),(#350636,#350637,#350638),(#350639,#350640,#350641),(#350642,
#350643,#350644),(#350645,#350646,#350647),(#350648,#350649,#350650),(#350651,
#350652,#350653),(#350654,#350655,#350656),(#350657,#350658,#350659),(#350660,
#350661,#350662),(#350663,#350664,#350665),(#350666,#350667,#350668),(#350669,
#350670,#350671),(#350672,#350673,#350674),(#350675,#350676,#350677),(#350678,
#350679,#350680),(#350681,#350682,#350683),(#350684,#350685,#350686),(#350687,
#350688,#350689),(#350690,#350691,#350692),(#350693,#350694,#350695),(#350696,
#350697,#350698),(#350699,#350700,#350701),(#350702,#350703,#350704),(#350705,
#350706,#350707),(#350708,#350709,#350710),(#350711,#350712,#350713),(#350714,
#350715,#350716),(#350717,#350718,#350719),(#350720,#350721,#350722),(#350723,
#350724,#350725),(#350726,#350727,#350728),(#350729,#350730,#350731),(#350732,
#350733,#350734),(#350735,#350736,#350737),(#350738,#350739,#350740),(#350741,
#350742,#350743),(#350744,#350745,#350746),(#350747,#350748,#350749),(#350750,
#350751,#350752),(#350753,#350754,#350755),(#350756,#350757,#350758),(#350759,
#350760,#350761),(#350762,#350763,#350764),(#350765,#350766,#350767),(#350768,
#350769,#350770),(#350771,#350772,#350773),(#350774,#350775,#350776),(#350777,
#350778,#350779),(#350780,#350781,#350782),(#350783,#350784,#350785),(#350786,
#350787,#350788),(#350789,#350790,#350791),(#350792,#350793,#350794),(#350795,
#350796,#350797),(#350798,#350799,#350800),(#350801,#350802,#350803),(#350804,
#350805,#350806),(#350807,#350808,#350809),(#350810,#350811,#350812),(#350813,
#350814,#350815),(#350816,#350817,#350818),(#350819,#350820,#350821),(#350822,
#350823,#350824),(#350825,#350826,#350827),(#350828,#350829,#350830),(#350831,
#350832,#350833),(#350834,#350835,#350836),(#350837,#350838,#350839),(#350840,
#350841,#350842),(#350843,#350844,#350845),(#350846,#350847,#350848),(#350849,
#350850,#350851),(#350852,#350853,#350854),(#350855,#350856,#350857),(#350858,
#350859,#350860),(#350861,#350862,#350863),(#350864,#350865,#350866),(#350867,
#350868,#350869),(#350870,#350871,#350872),(#350873,#350874,#350875),(#350876,
#350877,#350878),(#350879,#350880,#350881),(#350882,#350883,#350884),(#350885,
#350886,#350887),(#350888,#350889,#350890),(#350891,#350892,#350893),(#350894,
#350895,#350896),(#350897,#350898,#350899),(#350900,#350901,#350902),(#350903,
#350904,#350905),(#350906,#350907,#350908),(#350909,#350910,#350911),(#350912,
#350913,#350914),(#350915,#350916,#350917),(#350918,#350919,#350920),(#350921,
#350922,#350923),(#350924,#350925,#350926),(#350927,#350928,#350929),(#350930,
#350931,#350932),(#350933,#350934,#350935),(#350936,#350937,#350938),(#350939,
#350940,#350941),(#350942,#350943,#350944),(#350945,#350946,#350947),(#350948,
#350949,#350950),(#350951,#350952,#350953),(#350954,#350955,#350956),(#350957,
#350958,#350959),(#350960,#350961,#350962),(#350963,#350964,#350965),(#350966,
#350967,#350968),(#350969,#350970,#350971),(#350972,#350973,#350974),(#350975,
#350976,#350977),(#350978,#350979,#350980),(#350981,#350982,#350983),(#350984,
#350985,#350986),(#350987,#350988,#350989),(#350990,#350991,#350992),(#350993,
#350994,#350995),(#350996,#350997,#350998),(#350999,#351000,#351001),(#351002,
#351003,#351004),(#351005,#351006,#351007),(#351008,#351009,#351010),(#351011,
#351012,#351013),(#351014,#351015,#351016),(#351017,#351018,#351019),(#351020,
#351021,#351022),(#351023,#351024,#351025),(#351026,#351027,#351028),(#351029,
#351030,#351031),(#351032,#351033,#351034),(#351035,#351036,#351037),(#351038,
#351039,#351040),(#351041,#351042,#351043),(#351044,#351045,#351046),(#351047,
#351048,#351049),(#351050,#351051,#351052),(#351053,#351054,#351055),(#351056,
#351057,#351058),(#351059,#351060,#351061),(#351062,#351063,#351064),(#351065,
#351066,#351067),(#351068,#351069,#351070),(#351071,#351072,#351073),(#351074,
#351075,#351076),(#351077,#351078,#351079),(#351080,#351081,#351082),(#351083,
#351084,#351085),(#351086,#351087,#351088),(#351089,#351090,#351091),(#351092,
#351093,#351094),(#351095,#351096,#351097),(#351098,#351099,#351100),(#351101,
#351102,#351103),(#351104,#351105,#351106),(#351107,#351108,#351109),(#351110,
#351111,#351112),(#351113,#351114,#351115),(#351116,#351117,#351118),(#351119,
#351120,#351121),(#351122,#351123,#351124),(#351125,#351126,#351127),(#351128,
#351129,#351130),(#351131,#351132,#351133),(#351134,#351135,#351136),(#351137,
#351138,#351139),(#351140,#351141,#351142),(#351143,#351144,#351145),(#351146,
#351147,#351148),(#351149,#351150,#351151),(#351152,#351153,#351154),(#351155,
#351156,#351157),(#351158,#351159,#351160),(#351161,#351162,#351163),(#351164,
#351165,#351166),(#351167,#351168,#351169),(#351170,#351171,#351172),(#351173,
#351174,#351175),(#351176,#351177,#351178),(#351179,#351180,#351181),(#351182,
#351183,#351184),(#351185,#351186,#351187),(#351188,#351189,#351190),(#351191,
#351192,#351193),(#351194,#351195,#351196),(#351197,#351198,#351199),(#351200,
#351201,#351202),(#351203,#351204,#351205),(#351206,#351207,#351208),(#351209,
#351210,#351211),(#351212,#351213,#351214),(#351215,#351216,#351217),(#351218,
#351219,#351220),(#351221,#351222,#351223),(#351224,#351225,#351226),(#351227,
#351228,#351229),(#351230,#351231,#351232),(#351233,#351234,#351235),(#351236,
#351237,#351238),(#351239,#351240,#351241),(#351242,#351243,#351244),(#351245,
#351246,#351247),(#351248,#351249,#351250),(#351251,#351252,#351253),(#351254,
#351255,#351256),(#351257,#351258,#351259),(#351260,#351261,#351262),(#351263,
#351264,#351265),(#351266,#351267,#351268),(#351269,#351270,#351271),(#351272,
#351273,#351274),(#351275,#351276,#351277),(#351278,#351279,#351280),(#351281,
#351282,#351283),(#351284,#351285,#351286),(#351287,#351288,#351289),(#351290,
#351291,#351292),(#351293,#351294,#351295),(#351296,#351297,#351298),(#351299,
#351300,#351301),(#351302,#351303,#351304),(#351305,#351306,#351307),(#351308,
#351309,#351310),(#351311,#351312,#351313),(#351314,#351315,#351316),(#351317,
#351318,#351319),(#351320,#351321,#351322),(#351323,#351324,#351325),(#351326,
#351327,#351328),(#351329,#351330,#351331),(#351332,#351333,#351334),(#351335,
#351336,#351337),(#351338,#351339,#351340),(#351341,#351342,#351343),(#351344,
#351345,#351346),(#351347,#351348,#351349),(#351350,#351351,#351352),(#351353,
#351354,#351355),(#351356,#351357,#351358),(#351359,#351360,#351361),(#351362,
#351363,#351364),(#351365,#351366,#351367),(#351368,#351369,#351370),(#351371,
#351372,#351373),(#351374,#351375,#351376),(#351377,#351378,#351379),(#351380,
#351381,#351382),(#351383,#351384,#351385),(#351386,#351387,#351388),(#351389,
#351390,#351391),(#351392,#351393,#351394),(#351395,#351396,#351397),(#351398,
#351399,#351400),(#351401,#351402,#351403),(#351404,#351405,#351406),(#351407,
#351408,#351409),(#351410,#351411,#351412),(#351413,#351414,#351415),(#351416,
#351417,#351418),(#351419,#351420,#351421),(#351422,#351423,#351424),(#351425,
#351426,#351427),(#351428,#351429,#351430),(#351431,#351432,#351433),(#351434,
#351435,#351436),(#351437,#351438,#351439),(#351440,#351441,#351442),(#351443,
#351444,#351445),(#351446,#351447,#351448),(#351449,#351450,#351451),(#351452,
#351453,#351454),(#351455,#351456,#351457),(#351458,#351459,#351460),(#351461,
#351462,#351463),(#351464,#351465,#351466),(#351467,#351468,#351469),(#351470,
#351471,#351472),(#351473,#351474,#351475),(#351476,#351477,#351478),(#351479,
#351480,#351481),(#351482,#351483,#351484),(#351485,#351486,#351487),(#351488,
#351489,#351490),(#351491,#351492,#351493),(#351494,#351495,#351496),(#351497,
#351498,#351499),(#351500,#351501,#351502),(#351503,#351504,#351505),(#351506,
#351507,#351508),(#351509,#351510,#351511),(#351512,#351513,#351514),(#351515,
#351516,#351517),(#351518,#351519,#351520),(#351521,#351522,#351523),(#351524,
#351525,#351526)),.UNSPECIFIED.,.F.,.F.,.F.,(6,1,1,1,1,1,1,1,1,1,1,1,1,
1,1,1,1,1,1,1,1,1,1,1,1,1,1,1,1,1,1,1,1,1,1,1,1,1,1,1,1,1,1,1,1,1,1,1,1,
1,1,1,1,1,1,1,1,1,1,1,1,1,1,1,1,1,1,1,1,1,1,1,1,1,1,1,1,1,1,1,1,1,1,1,1,
1,1,1,1,1,1,1,1,1,1,1,1,1,1,1,1,1,1,1,1,1,1,1,1,1,1,1,1,1,1,1,1,1,1,1,1,
1,1,1,1,1,1,1,1,1,1,1,1,1,1,1,1,1,1,1,1,1,1,1,1,1,1,1,1,1,1,1,1,1,1,1,1,
1,1,1,1,1,1,1,1,1,1,1,1,1,1,1,1,1,1,1,1,1,1,1,1,1,1,1,1,1,1,1,1,1,1,1,1,
1,1,1,1,1,1,1,1,1,1,1,1,1,1,1,1,1,1,1,1,1,1,1,1,1,1,1,1,1,1,1,1,1,1,1,1,
1,1,1,1,1,1,1,1,1,1,1,1,1,1,1,1,1,1,1,1,1,1,1,1,1,1,1,1,1,1,1,1,1,1,1,1,
1,1,1,1,1,1,1,1,1,1,1,1,1,1,1,1,1,1,1,1,1,1,1,1,1,1,1,1,1,1,1,1,1,1,1,1,
1,1,1,1,1,1,1,1,1,1,1,1,1,1,1,1,1,1,1,1,1,1,1,1,1,1,1,1,1,1,1,1,1,1,1,1,
1,1,1,1,1,1,1,1,1,1,1,1,1,1,1,1,1,1,1,1,1,1,1,1,1,1,1,1,1,1,1,1,1,1,1,1,
1,1,1,1,1,1,1,1,1,1,1,1,1,1,1,1,1,1,1,1,1,1,1,1,1,1,1,1,1,1,1,1,1,1,1,1,
1,1,1,1,1,1,1,1,1,1,1,1,1,1,1,1,1,1,1,1,1,1,1,1,1,1,1,1,1,1,1,1,1,1,1,1,
1,1,1,1,1,1,1,1,1,1,1,1,1,1,1,1,1,1,1,1,1,1,1,1,1,1,1,1,1,1,1,1,1,1,1,1,
1,1,1,1,1,1,1,1,1,1,1,1,1,1,1,1,1,1,1,1,1,1,1,1,1,1,1,1,1,1,1,1,1,1,1,1,
1,1,1,1,1,1,1,1,1,1,1,1,1,1,1,1,1,1,1,1,1,1,1,1,1,1,1,1,1,6),(2,1,2),(-0.001964172,
0.,0.001834862,0.003669725,0.005504587,0.00733945,0.009174312,0.011009174,
0.012844037,0.014678899,0.016513761,0.018348624,0.020183486,0.022018349,
0.023853211,0.025688073,0.027522936,0.029357798,0.031192661,0.033027523,
0.034862385,0.036697248,0.03853211,0.040366972,0.042201835,0.044036697,
0.04587156,0.047706422,0.049541284,0.051376147,0.053211009,0.055045872,
0.056880734,0.058715596,0.060550459,0.062385321,0.064220183,0.066055046,
0.067889908,0.069724771,0.071559633,0.073394495,0.075229358,0.07706422,
0.078899083,0.080733945,0.082568807,0.08440367,0.086238532,0.088073394,
0.089908257,0.091743119,0.093577982,0.095412844,0.097247706,0.099082569,
0.100917431,0.102752294,0.104587156,0.106422018,0.108256881,0.110091743,
0.111926606,0.113761468,0.11559633,0.117431193,0.119266055,0.121100917,
0.12293578,0.124770642,0.126605505,0.128440367,0.130275229,0.132110092,
0.133944954,0.135779817,0.137614679,0.139449541,0.141284404,0.143119266,
0.144954128,0.146788991,0.148623853,0.150458716,0.152293578,0.15412844,
0.155963303,0.157798165,0.159633028,0.16146789,0.163302752,0.165137615,
0.166972477,0.168807339,0.170642202,0.172477064,0.174311927,0.176146789,
0.177981651,0.179816514,0.181651376,0.183486239,0.185321101,0.187155963,
0.188990826,0.190825688,0.19266055,0.194495413,0.196330275,0.198165138,
0.2,0.201834862,0.203669725,0.205504587,0.20733945,0.209174312,0.211009174,
0.212844037,0.214678899,0.216513761,0.218348624,0.220183486,0.222018349,
0.223853211,0.225688073,0.227522936,0.229357798,0.231192661,0.233027523,
0.234862385,0.236697248,0.23853211,0.240366972,0.242201835,0.244036697,
0.24587156,0.247706422,0.249541284,0.251376147,0.253211009,0.255045872,
0.256880734,0.258715596,0.260550459,0.262385321,0.264220183,0.266055046,
0.267889908,0.269724771,0.271559633,0.273394495,0.275229358,0.27706422,
0.278899083,0.280733945,0.282568807,0.28440367,0.286238532,0.288073394,
0.289908257,0.291743119,0.293577982,0.295412844,0.297247706,0.299082569,
0.300917431,0.302752294,0.304587156,0.306422018,0.308256881,0.310091743,
0.311926606,0.313761468,0.31559633,0.317431193,0.319266055,0.321100917,
0.32293578,0.324770642,0.326605505,0.328440367,0.330275229,0.332110092,
0.333944954,0.335779817,0.337614679,0.339449541,0.341284404,0.343119266,
0.344954128,0.346788991,0.348623853,0.350458716,0.352293578,0.35412844,
0.355963303,0.357798165,0.359633028,0.36146789,0.363302752,0.365137615,
0.366972477,0.368807339,0.370642202,0.372477064,0.374311927,0.376146789,
0.377981651,0.379816514,0.381651376,0.383486239,0.385321101,0.387155963,
0.388990826,0.390825688,0.39266055,0.394495413,0.396330275,0.398165138,
0.4,0.401834862,0.403669725,0.405504587,0.40733945,0.409174312,0.411009174,
0.412844037,0.414678899,0.416513761,0.418348624,0.420183486,0.422018349,
0.423853211,0.425688073,0.427522936,0.429357798,0.431192661,0.433027523,
0.434862385,0.436697248,0.43853211,0.440366972,0.442201835,0.444036697,
0.44587156,0.447706422,0.449541284,0.451376147,0.453211009,0.455045872,
0.456880734,0.458715596,0.460550459,0.462385321,0.464220183,0.466055046,
0.467889908,0.469724771,0.471559633,0.473394495,0.475229358,0.47706422,
0.478899083,0.480733945,0.482568807,0.48440367,0.486238532,0.488073394,
0.489908257,0.491743119,0.493577982,0.495412844,0.497247706,0.499082569,
0.500917431,0.502752294,0.504587156,0.506422018,0.508256881,0.510091743,
0.511926606,0.513761468,0.51559633,0.517431193,0.519266055,0.521100917,
0.52293578,0.524770642,0.526605505,0.528440367,0.530275229,0.532110092,
0.533944954,0.535779817,0.537614679,0.539449541,0.541284404,0.543119266,
0.544954128,0.546788991,0.548623853,0.550458716,0.552293578,0.55412844,
0.555963303,0.557798165,0.559633028,0.56146789,0.563302752,0.565137615,
0.566972477,0.568807339,0.570642202,0.572477064,0.574311927,0.576146789,
0.577981651,0.579816514,0.581651376,0.583486239,0.585321101,0.587155963,
0.588990826,0.590825688,0.59266055,0.594495413,0.596330275,0.598165138,
0.6,0.601834862,0.603669725,0.605504587,0.60733945,0.609174312,0.611009174,
0.612844037,0.614678899,0.616513761,0.618348624,0.620183486,0.622018349,
0.623853211,0.625688073,0.627522936,0.629357798,0.631192661,0.633027523,
0.634862385,0.636697248,0.63853211,0.640366972,0.642201835,0.644036697,
0.64587156,0.647706422,0.649541284,0.651376147,0.653211009,0.655045872,
0.656880734,0.658715596,0.660550459,0.662385321,0.664220183,0.666055046,
0.667889908,0.669724771,0.671559633,0.673394495,0.675229358,0.67706422,
0.678899083,0.680733945,0.682568807,0.68440367,0.686238532,0.688073394,
0.689908257,0.691743119,0.693577982,0.695412844,0.697247706,0.699082569,
0.700917431,0.702752294,0.704587156,0.706422018,0.708256881,0.710091743,
0.711926606,0.713761468,0.71559633,0.717431193,0.719266055,0.721100917,
0.72293578,0.724770642,0.726605505,0.728440367,0.730275229,0.732110092,
0.733944954,0.735779817,0.737614679,0.739449541,0.741284404,0.743119266,
0.744954128,0.746788991,0.748623853,0.750458716,0.752293578,0.75412844,
0.755963303,0.757798165,0.759633028,0.76146789,0.763302752,0.765137615,
0.766972477,0.768807339,0.770642202,0.772477064,0.774311927,0.776146789,
0.777981651,0.779816514,0.781651376,0.783486239,0.785321101,0.787155963,
0.788990826,0.790825688,0.79266055,0.794495413,0.796330275,0.798165138,
0.8,0.801834862,0.803669725,0.805504587,0.80733945,0.809174312,0.811009174,
0.812844037,0.814678899,0.816513761,0.818348624,0.820183486,0.822018349,
0.823853211,0.825688073,0.827522936,0.829357798,0.831192661,0.833027523,
0.834862385,0.836697248,0.83853211,0.840366972,0.842201835,0.844036697,
0.84587156,0.847706422,0.849541284,0.851376147,0.853211009,0.855045872,
0.856880734,0.858715596,0.860550459,0.862385321,0.864220183,0.866055046,
0.867889908,0.869724771,0.871559633,0.873394495,0.875229358,0.87706422,
0.878899083,0.880733945,0.882568807,0.88440367,0.886238532,0.888073394,
0.889908257,0.891743119,0.893577982,0.895412844,0.897247706,0.899082569,
0.900917431,0.902752294,0.904587156,0.906422018,0.908256881,0.910091743,
0.911926606,0.913761468,0.91559633,0.917431193,0.919266055,0.921100917,
0.92293578,0.924770642,0.926605505,0.928440367,0.930275229,0.932110092,
0.933944954,0.935779817,0.937614679,0.939449541,0.941284404,0.943119266,
0.944954128,0.946788991,0.948623853,0.950458716,0.952293578,0.95412844,
0.955963303,0.957798165,0.959633028,0.96146789,0.963302752,0.965137615,
0.966972477,0.968807339,0.970642202,0.972477064,0.974311927,0.976146789,
0.977981651,0.979816514,0.981651376,0.983486239,0.985321101,0.987155963,
0.988990826,0.990825688,0.99266055,0.994495413,0.996330275,0.998165138,
1.),(0.3,1.,1.3),.UNSPECIFIED.);
#6333=B_SPLINE_SURFACE_WITH_KNOTS('',5,1,((#351531,#351532,#351533),(#351534,
#351535,#351536),(#351537,#351538,#351539),(#351540,#351541,#351542),(#351543,
#351544,#351545),(#351546,#351547,#351548),(#351549,#351550,#351551),(#351552,
#351553,#351554),(#351555,#351556,#351557),(#351558,#351559,#351560),(#351561,
#351562,#351563),(#351564,#351565,#351566),(#351567,#351568,#351569),(#351570,
#351571,#351572),(#351573,#351574,#351575),(#351576,#351577,#351578),(#351579,
#351580,#351581),(#351582,#351583,#351584),(#351585,#351586,#351587),(#351588,
#351589,#351590),(#351591,#351592,#351593),(#351594,#351595,#351596),(#351597,
#351598,#351599),(#351600,#351601,#351602),(#351603,#351604,#351605),(#351606,
#351607,#351608),(#351609,#351610,#351611),(#351612,#351613,#351614),(#351615,
#351616,#351617),(#351618,#351619,#351620),(#351621,#351622,#351623),(#351624,
#351625,#351626),(#351627,#351628,#351629),(#351630,#351631,#351632),(#351633,
#351634,#351635),(#351636,#351637,#351638),(#351639,#351640,#351641),(#351642,
#351643,#351644),(#351645,#351646,#351647),(#351648,#351649,#351650),(#351651,
#351652,#351653),(#351654,#351655,#351656),(#351657,#351658,#351659),(#351660,
#351661,#351662),(#351663,#351664,#351665),(#351666,#351667,#351668),(#351669,
#351670,#351671),(#351672,#351673,#351674),(#351675,#351676,#351677),(#351678,
#351679,#351680),(#351681,#351682,#351683),(#351684,#351685,#351686),(#351687,
#351688,#351689),(#351690,#351691,#351692),(#351693,#351694,#351695),(#351696,
#351697,#351698),(#351699,#351700,#351701),(#351702,#351703,#351704),(#351705,
#351706,#351707),(#351708,#351709,#351710),(#351711,#351712,#351713),(#351714,
#351715,#351716),(#351717,#351718,#351719),(#351720,#351721,#351722),(#351723,
#351724,#351725),(#351726,#351727,#351728),(#351729,#351730,#351731),(#351732,
#351733,#351734),(#351735,#351736,#351737),(#351738,#351739,#351740),(#351741,
#351742,#351743),(#351744,#351745,#351746),(#351747,#351748,#351749),(#351750,
#351751,#351752),(#351753,#351754,#351755),(#351756,#351757,#351758),(#351759,
#351760,#351761),(#351762,#351763,#351764),(#351765,#351766,#351767),(#351768,
#351769,#351770),(#351771,#351772,#351773),(#351774,#351775,#351776),(#351777,
#351778,#351779),(#351780,#351781,#351782),(#351783,#351784,#351785),(#351786,
#351787,#351788),(#351789,#351790,#351791),(#351792,#351793,#351794),(#351795,
#351796,#351797),(#351798,#351799,#351800),(#351801,#351802,#351803),(#351804,
#351805,#351806),(#351807,#351808,#351809),(#351810,#351811,#351812),(#351813,
#351814,#351815),(#351816,#351817,#351818),(#351819,#351820,#351821),(#351822,
#351823,#351824),(#351825,#351826,#351827),(#351828,#351829,#351830),(#351831,
#351832,#351833),(#351834,#351835,#351836),(#351837,#351838,#351839),(#351840,
#351841,#351842),(#351843,#351844,#351845),(#351846,#351847,#351848),(#351849,
#351850,#351851),(#351852,#351853,#351854),(#351855,#351856,#351857),(#351858,
#351859,#351860),(#351861,#351862,#351863),(#351864,#351865,#351866),(#351867,
#351868,#351869),(#351870,#351871,#351872),(#351873,#351874,#351875),(#351876,
#351877,#351878),(#351879,#351880,#351881),(#351882,#351883,#351884),(#351885,
#351886,#351887),(#351888,#351889,#351890),(#351891,#351892,#351893),(#351894,
#351895,#351896),(#351897,#351898,#351899),(#351900,#351901,#351902),(#351903,
#351904,#351905),(#351906,#351907,#351908),(#351909,#351910,#351911),(#351912,
#351913,#351914),(#351915,#351916,#351917),(#351918,#351919,#351920),(#351921,
#351922,#351923),(#351924,#351925,#351926),(#351927,#351928,#351929),(#351930,
#351931,#351932),(#351933,#351934,#351935),(#351936,#351937,#351938),(#351939,
#351940,#351941),(#351942,#351943,#351944),(#351945,#351946,#351947),(#351948,
#351949,#351950),(#351951,#351952,#351953),(#351954,#351955,#351956),(#351957,
#351958,#351959),(#351960,#351961,#351962),(#351963,#351964,#351965),(#351966,
#351967,#351968),(#351969,#351970,#351971),(#351972,#351973,#351974),(#351975,
#351976,#351977),(#351978,#351979,#351980),(#351981,#351982,#351983),(#351984,
#351985,#351986),(#351987,#351988,#351989),(#351990,#351991,#351992),(#351993,
#351994,#351995),(#351996,#351997,#351998),(#351999,#352000,#352001),(#352002,
#352003,#352004),(#352005,#352006,#352007),(#352008,#352009,#352010),(#352011,
#352012,#352013),(#352014,#352015,#352016),(#352017,#352018,#352019),(#352020,
#352021,#352022),(#352023,#352024,#352025),(#352026,#352027,#352028),(#352029,
#352030,#352031),(#352032,#352033,#352034),(#352035,#352036,#352037),(#352038,
#352039,#352040),(#352041,#352042,#352043),(#352044,#352045,#352046),(#352047,
#352048,#352049),(#352050,#352051,#352052),(#352053,#352054,#352055),(#352056,
#352057,#352058),(#352059,#352060,#352061),(#352062,#352063,#352064),(#352065,
#352066,#352067),(#352068,#352069,#352070),(#352071,#352072,#352073),(#352074,
#352075,#352076),(#352077,#352078,#352079),(#352080,#352081,#352082),(#352083,
#352084,#352085),(#352086,#352087,#352088),(#352089,#352090,#352091),(#352092,
#352093,#352094),(#352095,#352096,#352097),(#352098,#352099,#352100),(#352101,
#352102,#352103),(#352104,#352105,#352106),(#352107,#352108,#352109),(#352110,
#352111,#352112),(#352113,#352114,#352115),(#352116,#352117,#352118),(#352119,
#352120,#352121),(#352122,#352123,#352124),(#352125,#352126,#352127),(#352128,
#352129,#352130),(#352131,#352132,#352133),(#352134,#352135,#352136),(#352137,
#352138,#352139),(#352140,#352141,#352142),(#352143,#352144,#352145),(#352146,
#352147,#352148),(#352149,#352150,#352151),(#352152,#352153,#352154),(#352155,
#352156,#352157),(#352158,#352159,#352160),(#352161,#352162,#352163),(#352164,
#352165,#352166),(#352167,#352168,#352169),(#352170,#352171,#352172),(#352173,
#352174,#352175),(#352176,#352177,#352178),(#352179,#352180,#352181),(#352182,
#352183,#352184),(#352185,#352186,#352187),(#352188,#352189,#352190),(#352191,
#352192,#352193),(#352194,#352195,#352196),(#352197,#352198,#352199),(#352200,
#352201,#352202),(#352203,#352204,#352205),(#352206,#352207,#352208),(#352209,
#352210,#352211),(#352212,#352213,#352214),(#352215,#352216,#352217),(#352218,
#352219,#352220),(#352221,#352222,#352223),(#352224,#352225,#352226),(#352227,
#352228,#352229),(#352230,#352231,#352232),(#352233,#352234,#352235),(#352236,
#352237,#352238),(#352239,#352240,#352241),(#352242,#352243,#352244),(#352245,
#352246,#352247),(#352248,#352249,#352250),(#352251,#352252,#352253),(#352254,
#352255,#352256),(#352257,#352258,#352259),(#352260,#352261,#352262),(#352263,
#352264,#352265),(#352266,#352267,#352268),(#352269,#352270,#352271),(#352272,
#352273,#352274),(#352275,#352276,#352277),(#352278,#352279,#352280),(#352281,
#352282,#352283),(#352284,#352285,#352286),(#352287,#352288,#352289),(#352290,
#352291,#352292),(#352293,#352294,#352295),(#352296,#352297,#352298),(#352299,
#352300,#352301),(#352302,#352303,#352304),(#352305,#352306,#352307),(#352308,
#352309,#352310),(#352311,#352312,#352313),(#352314,#352315,#352316),(#352317,
#352318,#352319),(#352320,#352321,#352322),(#352323,#352324,#352325),(#352326,
#352327,#352328),(#352329,#352330,#352331),(#352332,#352333,#352334),(#352335,
#352336,#352337),(#352338,#352339,#352340),(#352341,#352342,#352343),(#352344,
#352345,#352346),(#352347,#352348,#352349),(#352350,#352351,#352352),(#352353,
#352354,#352355),(#352356,#352357,#352358),(#352359,#352360,#352361),(#352362,
#352363,#352364),(#352365,#352366,#352367),(#352368,#352369,#352370),(#352371,
#352372,#352373),(#352374,#352375,#352376),(#352377,#352378,#352379),(#352380,
#352381,#352382),(#352383,#352384,#352385),(#352386,#352387,#352388),(#352389,
#352390,#352391),(#352392,#352393,#352394),(#352395,#352396,#352397),(#352398,
#352399,#352400),(#352401,#352402,#352403),(#352404,#352405,#352406),(#352407,
#352408,#352409),(#352410,#352411,#352412),(#352413,#352414,#352415),(#352416,
#352417,#352418),(#352419,#352420,#352421),(#352422,#352423,#352424),(#352425,
#352426,#352427),(#352428,#352429,#352430),(#352431,#352432,#352433),(#352434,
#352435,#352436),(#352437,#352438,#352439),(#352440,#352441,#352442),(#352443,
#352444,#352445),(#352446,#352447,#352448),(#352449,#352450,#352451),(#352452,
#352453,#352454),(#352455,#352456,#352457),(#352458,#352459,#352460),(#352461,
#352462,#352463),(#352464,#352465,#352466),(#352467,#352468,#352469),(#352470,
#352471,#352472),(#352473,#352474,#352475),(#352476,#352477,#352478),(#352479,
#352480,#352481),(#352482,#352483,#352484),(#352485,#352486,#352487),(#352488,
#352489,#352490),(#352491,#352492,#352493),(#352494,#352495,#352496),(#352497,
#352498,#352499),(#352500,#352501,#352502),(#352503,#352504,#352505),(#352506,
#352507,#352508),(#352509,#352510,#352511),(#352512,#352513,#352514),(#352515,
#352516,#352517),(#352518,#352519,#352520),(#352521,#352522,#352523),(#352524,
#352525,#352526),(#352527,#352528,#352529),(#352530,#352531,#352532),(#352533,
#352534,#352535),(#352536,#352537,#352538),(#352539,#352540,#352541),(#352542,
#352543,#352544),(#352545,#352546,#352547),(#352548,#352549,#352550),(#352551,
#352552,#352553),(#352554,#352555,#352556),(#352557,#352558,#352559),(#352560,
#352561,#352562),(#352563,#352564,#352565),(#352566,#352567,#352568),(#352569,
#352570,#352571),(#352572,#352573,#352574),(#352575,#352576,#352577),(#352578,
#352579,#352580),(#352581,#352582,#352583),(#352584,#352585,#352586),(#352587,
#352588,#352589),(#352590,#352591,#352592),(#352593,#352594,#352595),(#352596,
#352597,#352598),(#352599,#352600,#352601),(#352602,#352603,#352604),(#352605,
#352606,#352607),(#352608,#352609,#352610),(#352611,#352612,#352613),(#352614,
#352615,#352616),(#352617,#352618,#352619),(#352620,#352621,#352622),(#352623,
#352624,#352625),(#352626,#352627,#352628),(#352629,#352630,#352631),(#352632,
#352633,#352634),(#352635,#352636,#352637),(#352638,#352639,#352640),(#352641,
#352642,#352643),(#352644,#352645,#352646),(#352647,#352648,#352649),(#352650,
#352651,#352652),(#352653,#352654,#352655),(#352656,#352657,#352658),(#352659,
#352660,#352661),(#352662,#352663,#352664),(#352665,#352666,#352667),(#352668,
#352669,#352670),(#352671,#352672,#352673),(#352674,#352675,#352676),(#352677,
#352678,#352679),(#352680,#352681,#352682),(#352683,#352684,#352685),(#352686,
#352687,#352688),(#352689,#352690,#352691),(#352692,#352693,#352694),(#352695,
#352696,#352697),(#352698,#352699,#352700),(#352701,#352702,#352703),(#352704,
#352705,#352706),(#352707,#352708,#352709),(#352710,#352711,#352712),(#352713,
#352714,#352715),(#352716,#352717,#352718),(#352719,#352720,#352721),(#352722,
#352723,#352724),(#352725,#352726,#352727),(#352728,#352729,#352730),(#352731,
#352732,#352733),(#352734,#352735,#352736),(#352737,#352738,#352739),(#352740,
#352741,#352742),(#352743,#352744,#352745),(#352746,#352747,#352748),(#352749,
#352750,#352751),(#352752,#352753,#352754),(#352755,#352756,#352757),(#352758,
#352759,#352760),(#352761,#352762,#352763),(#352764,#352765,#352766),(#352767,
#352768,#352769),(#352770,#352771,#352772),(#352773,#352774,#352775),(#352776,
#352777,#352778),(#352779,#352780,#352781),(#352782,#352783,#352784),(#352785,
#352786,#352787),(#352788,#352789,#352790),(#352791,#352792,#352793),(#352794,
#352795,#352796),(#352797,#352798,#352799),(#352800,#352801,#352802),(#352803,
#352804,#352805),(#352806,#352807,#352808),(#352809,#352810,#352811),(#352812,
#352813,#352814),(#352815,#352816,#352817),(#352818,#352819,#352820),(#352821,
#352822,#352823),(#352824,#352825,#352826),(#352827,#352828,#352829),(#352830,
#352831,#352832),(#352833,#352834,#352835),(#352836,#352837,#352838),(#352839,
#352840,#352841),(#352842,#352843,#352844),(#352845,#352846,#352847),(#352848,
#352849,#352850),(#352851,#352852,#352853),(#352854,#352855,#352856),(#352857,
#352858,#352859),(#352860,#352861,#352862),(#352863,#352864,#352865),(#352866,
#352867,#352868),(#352869,#352870,#352871),(#352872,#352873,#352874),(#352875,
#352876,#352877),(#352878,#352879,#352880),(#352881,#352882,#352883),(#352884,
#352885,#352886),(#352887,#352888,#352889),(#352890,#352891,#352892),(#352893,
#352894,#352895),(#352896,#352897,#352898),(#352899,#352900,#352901),(#352902,
#352903,#352904),(#352905,#352906,#352907),(#352908,#352909,#352910),(#352911,
#352912,#352913),(#352914,#352915,#352916),(#352917,#352918,#352919),(#352920,
#352921,#352922),(#352923,#352924,#352925),(#352926,#352927,#352928),(#352929,
#352930,#352931),(#352932,#352933,#352934),(#352935,#352936,#352937),(#352938,
#352939,#352940),(#352941,#352942,#352943),(#352944,#352945,#352946),(#352947,
#352948,#352949),(#352950,#352951,#352952),(#352953,#352954,#352955),(#352956,
#352957,#352958),(#352959,#352960,#352961),(#352962,#352963,#352964),(#352965,
#352966,#352967),(#352968,#352969,#352970),(#352971,#352972,#352973),(#352974,
#352975,#352976),(#352977,#352978,#352979),(#352980,#352981,#352982),(#352983,
#352984,#352985),(#352986,#352987,#352988),(#352989,#352990,#352991),(#352992,
#352993,#352994),(#352995,#352996,#352997),(#352998,#352999,#353000),(#353001,
#353002,#353003),(#353004,#353005,#353006),(#353007,#353008,#353009),(#353010,
#353011,#353012),(#353013,#353014,#353015),(#353016,#353017,#353018),(#353019,
#353020,#353021),(#353022,#353023,#353024),(#353025,#353026,#353027),(#353028,
#353029,#353030),(#353031,#353032,#353033),(#353034,#353035,#353036),(#353037,
#353038,#353039),(#353040,#353041,#353042),(#353043,#353044,#353045),(#353046,
#353047,#353048),(#353049,#353050,#353051),(#353052,#353053,#353054),(#353055,
#353056,#353057),(#353058,#353059,#353060),(#353061,#353062,#353063),(#353064,
#353065,#353066),(#353067,#353068,#353069),(#353070,#353071,#353072),(#353073,
#353074,#353075),(#353076,#353077,#353078),(#353079,#353080,#353081),(#353082,
#353083,#353084),(#353085,#353086,#353087),(#353088,#353089,#353090),(#353091,
#353092,#353093),(#353094,#353095,#353096),(#353097,#353098,#353099),(#353100,
#353101,#353102),(#353103,#353104,#353105),(#353106,#353107,#353108),(#353109,
#353110,#353111),(#353112,#353113,#353114),(#353115,#353116,#353117),(#353118,
#353119,#353120),(#353121,#353122,#353123),(#353124,#353125,#353126),(#353127,
#353128,#353129),(#353130,#353131,#353132),(#353133,#353134,#353135),(#353136,
#353137,#353138),(#353139,#353140,#353141),(#353142,#353143,#353144),(#353145,
#353146,#353147),(#353148,#353149,#353150),(#353151,#353152,#353153),(#353154,
#353155,#353156),(#353157,#353158,#353159),(#353160,#353161,#353162),(#353163,
#353164,#353165),(#353166,#353167,#353168),(#353169,#353170,#353171),(#353172,
#353173,#353174),(#353175,#353176,#353177),(#353178,#353179,#353180)),
 .UNSPECIFIED.,.F.,.F.,.F.,(6,1,1,1,1,1,1,1,1,1,1,1,1,1,1,1,1,1,1,1,1,1,
1,1,1,1,1,1,1,1,1,1,1,1,1,1,1,1,1,1,1,1,1,1,1,1,1,1,1,1,1,1,1,1,1,1,1,1,
1,1,1,1,1,1,1,1,1,1,1,1,1,1,1,1,1,1,1,1,1,1,1,1,1,1,1,1,1,1,1,1,1,1,1,1,
1,1,1,1,1,1,1,1,1,1,1,1,1,1,1,1,1,1,1,1,1,1,1,1,1,1,1,1,1,1,1,1,1,1,1,1,
1,1,1,1,1,1,1,1,1,1,1,1,1,1,1,1,1,1,1,1,1,1,1,1,1,1,1,1,1,1,1,1,1,1,1,1,
1,1,1,1,1,1,1,1,1,1,1,1,1,1,1,1,1,1,1,1,1,1,1,1,1,1,1,1,1,1,1,1,1,1,1,1,
1,1,1,1,1,1,1,1,1,1,1,1,1,1,1,1,1,1,1,1,1,1,1,1,1,1,1,1,1,1,1,1,1,1,1,1,
1,1,1,1,1,1,1,1,1,1,1,1,1,1,1,1,1,1,1,1,1,1,1,1,1,1,1,1,1,1,1,1,1,1,1,1,
1,1,1,1,1,1,1,1,1,1,1,1,1,1,1,1,1,1,1,1,1,1,1,1,1,1,1,1,1,1,1,1,1,1,1,1,
1,1,1,1,1,1,1,1,1,1,1,1,1,1,1,1,1,1,1,1,1,1,1,1,1,1,1,1,1,1,1,1,1,1,1,1,
1,1,1,1,1,1,1,1,1,1,1,1,1,1,1,1,1,1,1,1,1,1,1,1,1,1,1,1,1,1,1,1,1,1,1,1,
1,1,1,1,1,1,1,1,1,1,1,1,1,1,1,1,1,1,1,1,1,1,1,1,1,1,1,1,1,1,1,1,1,1,1,1,
1,1,1,1,1,1,1,1,1,1,1,1,1,1,1,1,1,1,1,1,1,1,1,1,1,1,1,1,1,1,1,1,1,1,1,1,
1,1,1,1,1,1,1,1,1,1,1,1,1,1,1,1,1,1,1,1,1,1,1,1,1,1,1,1,1,1,1,1,1,1,1,1,
1,1,1,1,1,1,1,1,1,1,1,1,1,1,1,1,1,1,1,1,1,1,1,1,1,1,1,1,1,1,1,1,1,1,1,1,
1,1,1,1,1,1,1,1,1,1,1,1,1,1,1,1,1,1,1,6),(2,1,2),(-1.,-0.998165138,-0.996330275,
-0.994495413,-0.99266055,-0.990825688,-0.988990826,-0.987155963,-0.985321101,
-0.983486239,-0.981651376,-0.979816514,-0.977981651,-0.976146789,-0.974311927,
-0.972477064,-0.970642202,-0.968807339,-0.966972477,-0.965137615,-0.963302752,
-0.96146789,-0.959633028,-0.957798165,-0.955963303,-0.95412844,-0.952293578,
-0.950458716,-0.948623853,-0.946788991,-0.944954128,-0.943119266,-0.941284404,
-0.939449541,-0.937614679,-0.935779817,-0.933944954,-0.932110092,-0.930275229,
-0.928440367,-0.926605505,-0.924770642,-0.92293578,-0.921100917,-0.919266055,
-0.917431193,-0.91559633,-0.913761468,-0.911926606,-0.910091743,-0.908256881,
-0.906422018,-0.904587156,-0.902752294,-0.900917431,-0.899082569,-0.897247706,
-0.895412844,-0.893577982,-0.891743119,-0.889908257,-0.888073394,-0.886238532,
-0.88440367,-0.882568807,-0.880733945,-0.878899083,-0.87706422,-0.875229358,
-0.873394495,-0.871559633,-0.869724771,-0.867889908,-0.866055046,-0.864220183,
-0.862385321,-0.860550459,-0.858715596,-0.856880734,-0.855045872,-0.853211009,
-0.851376147,-0.849541284,-0.847706422,-0.84587156,-0.844036697,-0.842201835,
-0.840366972,-0.83853211,-0.836697248,-0.834862385,-0.833027523,-0.831192661,
-0.829357798,-0.827522936,-0.825688073,-0.823853211,-0.822018349,-0.820183486,
-0.818348624,-0.816513761,-0.814678899,-0.812844037,-0.811009174,-0.809174312,
-0.80733945,-0.805504587,-0.803669725,-0.801834862,-0.8,-0.798165138,-0.796330275,
-0.794495413,-0.79266055,-0.790825688,-0.788990826,-0.787155963,-0.785321101,
-0.783486239,-0.781651376,-0.779816514,-0.777981651,-0.776146789,-0.774311927,
-0.772477064,-0.770642202,-0.768807339,-0.766972477,-0.765137615,-0.763302752,
-0.76146789,-0.759633028,-0.757798165,-0.755963303,-0.75412844,-0.752293578,
-0.750458716,-0.748623853,-0.746788991,-0.744954128,-0.743119266,-0.741284404,
-0.739449541,-0.737614679,-0.735779817,-0.733944954,-0.732110092,-0.730275229,
-0.728440367,-0.726605505,-0.724770642,-0.72293578,-0.721100917,-0.719266055,
-0.717431193,-0.71559633,-0.713761468,-0.711926606,-0.710091743,-0.708256881,
-0.706422018,-0.704587156,-0.702752294,-0.700917431,-0.699082569,-0.697247706,
-0.695412844,-0.693577982,-0.691743119,-0.689908257,-0.688073394,-0.686238532,
-0.68440367,-0.682568807,-0.680733945,-0.678899083,-0.67706422,-0.675229358,
-0.673394495,-0.671559633,-0.669724771,-0.667889908,-0.666055046,-0.664220183,
-0.662385321,-0.660550459,-0.658715596,-0.656880734,-0.655045872,-0.653211009,
-0.651376147,-0.649541284,-0.647706422,-0.64587156,-0.644036697,-0.642201835,
-0.640366972,-0.63853211,-0.636697248,-0.634862385,-0.633027523,-0.631192661,
-0.629357798,-0.627522936,-0.625688073,-0.623853211,-0.622018349,-0.620183486,
-0.618348624,-0.616513761,-0.614678899,-0.612844037,-0.611009174,-0.609174312,
-0.60733945,-0.605504587,-0.603669725,-0.601834862,-0.6,-0.598165138,-0.596330275,
-0.594495413,-0.59266055,-0.590825688,-0.588990826,-0.587155963,-0.585321101,
-0.583486239,-0.581651376,-0.579816514,-0.577981651,-0.576146789,-0.574311927,
-0.572477064,-0.570642202,-0.568807339,-0.566972477,-0.565137615,-0.563302752,
-0.56146789,-0.559633028,-0.557798165,-0.555963303,-0.55412844,-0.552293578,
-0.550458716,-0.548623853,-0.546788991,-0.544954128,-0.543119266,-0.541284404,
-0.539449541,-0.537614679,-0.535779817,-0.533944954,-0.532110092,-0.530275229,
-0.528440367,-0.526605505,-0.524770642,-0.52293578,-0.521100917,-0.519266055,
-0.517431193,-0.51559633,-0.513761468,-0.511926606,-0.510091743,-0.508256881,
-0.506422018,-0.504587156,-0.502752294,-0.500917431,-0.499082569,-0.497247706,
-0.495412844,-0.493577982,-0.491743119,-0.489908257,-0.488073394,-0.486238532,
-0.48440367,-0.482568807,-0.480733945,-0.478899083,-0.47706422,-0.475229358,
-0.473394495,-0.471559633,-0.469724771,-0.467889908,-0.466055046,-0.464220183,
-0.462385321,-0.460550459,-0.458715596,-0.456880734,-0.455045872,-0.453211009,
-0.451376147,-0.449541284,-0.447706422,-0.44587156,-0.444036697,-0.442201835,
-0.440366972,-0.43853211,-0.436697248,-0.434862385,-0.433027523,-0.431192661,
-0.429357798,-0.427522936,-0.425688073,-0.423853211,-0.422018349,-0.420183486,
-0.418348624,-0.416513761,-0.414678899,-0.412844037,-0.411009174,-0.409174312,
-0.40733945,-0.405504587,-0.403669725,-0.401834862,-0.4,-0.398165138,-0.396330275,
-0.394495413,-0.39266055,-0.390825688,-0.388990826,-0.387155963,-0.385321101,
-0.383486239,-0.381651376,-0.379816514,-0.377981651,-0.376146789,-0.374311927,
-0.372477064,-0.370642202,-0.368807339,-0.366972477,-0.365137615,-0.363302752,
-0.36146789,-0.359633028,-0.357798165,-0.355963303,-0.35412844,-0.352293578,
-0.350458716,-0.348623853,-0.346788991,-0.344954128,-0.343119266,-0.341284404,
-0.339449541,-0.337614679,-0.335779817,-0.333944954,-0.332110092,-0.330275229,
-0.328440367,-0.326605505,-0.324770642,-0.32293578,-0.321100917,-0.319266055,
-0.317431193,-0.31559633,-0.313761468,-0.311926606,-0.310091743,-0.308256881,
-0.306422018,-0.304587156,-0.302752294,-0.300917431,-0.299082569,-0.297247706,
-0.295412844,-0.293577982,-0.291743119,-0.289908257,-0.288073394,-0.286238532,
-0.28440367,-0.282568807,-0.280733945,-0.278899083,-0.27706422,-0.275229358,
-0.273394495,-0.271559633,-0.269724771,-0.267889908,-0.266055046,-0.264220183,
-0.262385321,-0.260550459,-0.258715596,-0.256880734,-0.255045872,-0.253211009,
-0.251376147,-0.249541284,-0.247706422,-0.24587156,-0.244036697,-0.242201835,
-0.240366972,-0.23853211,-0.236697248,-0.234862385,-0.233027523,-0.231192661,
-0.229357798,-0.227522936,-0.225688073,-0.223853211,-0.222018349,-0.220183486,
-0.218348624,-0.216513761,-0.214678899,-0.212844037,-0.211009174,-0.209174312,
-0.20733945,-0.205504587,-0.203669725,-0.201834862,-0.2,-0.198165138,-0.196330275,
-0.194495413,-0.19266055,-0.190825688,-0.188990826,-0.187155963,-0.185321101,
-0.183486239,-0.181651376,-0.179816514,-0.177981651,-0.176146789,-0.174311927,
-0.172477064,-0.170642202,-0.168807339,-0.166972477,-0.165137615,-0.163302752,
-0.16146789,-0.159633028,-0.157798165,-0.155963303,-0.15412844,-0.152293578,
-0.150458716,-0.148623853,-0.146788991,-0.144954128,-0.143119266,-0.141284404,
-0.139449541,-0.137614679,-0.135779817,-0.133944954,-0.132110092,-0.130275229,
-0.128440367,-0.126605505,-0.124770642,-0.12293578,-0.121100917,-0.119266055,
-0.117431193,-0.11559633,-0.113761468,-0.111926606,-0.110091743,-0.108256881,
-0.106422018,-0.104587156,-0.102752294,-0.100917431,-0.099082569,-0.097247706,
-0.095412844,-0.093577982,-0.091743119,-0.089908257,-0.088073394,-0.086238532,
-0.08440367,-0.082568807,-0.080733945,-0.078899083,-0.07706422,-0.075229358,
-0.073394495,-0.071559633,-0.069724771,-0.067889908,-0.066055046,-0.064220183,
-0.062385321,-0.060550459,-0.058715596,-0.056880734,-0.055045872,-0.053211009,
-0.051376147,-0.049541284,-0.047706422,-0.04587156,-0.044036697,-0.042201835,
-0.040366972,-0.03853211,-0.036697248,-0.034862385,-0.033027523,-0.031192661,
-0.029357798,-0.027522936,-0.025688073,-0.023853211,-0.022018349,-0.020183486,
-0.018348624,-0.016513761,-0.014678899,-0.012844037,-0.011009174,-0.009174312,
-0.00733945,-0.005504587,-0.003669725,-0.001834862,0.000982134),(0.3,1.,
1.3),.UNSPECIFIED.);
#6334=B_SPLINE_SURFACE_WITH_KNOTS('',5,1,((#353184,#353185,#353186),(#353187,
#353188,#353189),(#353190,#353191,#353192),(#353193,#353194,#353195),(#353196,
#353197,#353198),(#353199,#353200,#353201),(#353202,#353203,#353204),(#353205,
#353206,#353207),(#353208,#353209,#353210),(#353211,#353212,#353213),(#353214,
#353215,#353216),(#353217,#353218,#353219),(#353220,#353221,#353222),(#353223,
#353224,#353225),(#353226,#353227,#353228),(#353229,#353230,#353231),(#353232,
#353233,#353234),(#353235,#353236,#353237),(#353238,#353239,#353240),(#353241,
#353242,#353243),(#353244,#353245,#353246),(#353247,#353248,#353249),(#353250,
#353251,#353252),(#353253,#353254,#353255),(#353256,#353257,#353258),(#353259,
#353260,#353261),(#353262,#353263,#353264),(#353265,#353266,#353267),(#353268,
#353269,#353270),(#353271,#353272,#353273),(#353274,#353275,#353276),(#353277,
#353278,#353279),(#353280,#353281,#353282),(#353283,#353284,#353285),(#353286,
#353287,#353288),(#353289,#353290,#353291),(#353292,#353293,#353294),(#353295,
#353296,#353297),(#353298,#353299,#353300),(#353301,#353302,#353303),(#353304,
#353305,#353306),(#353307,#353308,#353309),(#353310,#353311,#353312),(#353313,
#353314,#353315),(#353316,#353317,#353318),(#353319,#353320,#353321),(#353322,
#353323,#353324),(#353325,#353326,#353327),(#353328,#353329,#353330),(#353331,
#353332,#353333),(#353334,#353335,#353336),(#353337,#353338,#353339),(#353340,
#353341,#353342),(#353343,#353344,#353345),(#353346,#353347,#353348),(#353349,
#353350,#353351),(#353352,#353353,#353354),(#353355,#353356,#353357),(#353358,
#353359,#353360),(#353361,#353362,#353363),(#353364,#353365,#353366),(#353367,
#353368,#353369),(#353370,#353371,#353372),(#353373,#353374,#353375),(#353376,
#353377,#353378),(#353379,#353380,#353381),(#353382,#353383,#353384),(#353385,
#353386,#353387),(#353388,#353389,#353390),(#353391,#353392,#353393),(#353394,
#353395,#353396),(#353397,#353398,#353399),(#353400,#353401,#353402),(#353403,
#353404,#353405),(#353406,#353407,#353408),(#353409,#353410,#353411),(#353412,
#353413,#353414),(#353415,#353416,#353417),(#353418,#353419,#353420),(#353421,
#353422,#353423),(#353424,#353425,#353426),(#353427,#353428,#353429),(#353430,
#353431,#353432),(#353433,#353434,#353435),(#353436,#353437,#353438),(#353439,
#353440,#353441),(#353442,#353443,#353444),(#353445,#353446,#353447),(#353448,
#353449,#353450),(#353451,#353452,#353453),(#353454,#353455,#353456),(#353457,
#353458,#353459),(#353460,#353461,#353462),(#353463,#353464,#353465),(#353466,
#353467,#353468),(#353469,#353470,#353471),(#353472,#353473,#353474),(#353475,
#353476,#353477),(#353478,#353479,#353480),(#353481,#353482,#353483),(#353484,
#353485,#353486),(#353487,#353488,#353489),(#353490,#353491,#353492),(#353493,
#353494,#353495),(#353496,#353497,#353498),(#353499,#353500,#353501),(#353502,
#353503,#353504),(#353505,#353506,#353507),(#353508,#353509,#353510),(#353511,
#353512,#353513),(#353514,#353515,#353516),(#353517,#353518,#353519),(#353520,
#353521,#353522),(#353523,#353524,#353525),(#353526,#353527,#353528),(#353529,
#353530,#353531),(#353532,#353533,#353534),(#353535,#353536,#353537),(#353538,
#353539,#353540),(#353541,#353542,#353543),(#353544,#353545,#353546),(#353547,
#353548,#353549),(#353550,#353551,#353552),(#353553,#353554,#353555),(#353556,
#353557,#353558),(#353559,#353560,#353561),(#353562,#353563,#353564),(#353565,
#353566,#353567),(#353568,#353569,#353570),(#353571,#353572,#353573),(#353574,
#353575,#353576),(#353577,#353578,#353579),(#353580,#353581,#353582),(#353583,
#353584,#353585),(#353586,#353587,#353588),(#353589,#353590,#353591),(#353592,
#353593,#353594),(#353595,#353596,#353597),(#353598,#353599,#353600),(#353601,
#353602,#353603),(#353604,#353605,#353606),(#353607,#353608,#353609),(#353610,
#353611,#353612),(#353613,#353614,#353615),(#353616,#353617,#353618),(#353619,
#353620,#353621),(#353622,#353623,#353624),(#353625,#353626,#353627),(#353628,
#353629,#353630),(#353631,#353632,#353633),(#353634,#353635,#353636),(#353637,
#353638,#353639),(#353640,#353641,#353642),(#353643,#353644,#353645),(#353646,
#353647,#353648),(#353649,#353650,#353651),(#353652,#353653,#353654),(#353655,
#353656,#353657),(#353658,#353659,#353660),(#353661,#353662,#353663),(#353664,
#353665,#353666),(#353667,#353668,#353669),(#353670,#353671,#353672),(#353673,
#353674,#353675),(#353676,#353677,#353678),(#353679,#353680,#353681),(#353682,
#353683,#353684),(#353685,#353686,#353687),(#353688,#353689,#353690),(#353691,
#353692,#353693),(#353694,#353695,#353696),(#353697,#353698,#353699),(#353700,
#353701,#353702),(#353703,#353704,#353705),(#353706,#353707,#353708),(#353709,
#353710,#353711),(#353712,#353713,#353714),(#353715,#353716,#353717),(#353718,
#353719,#353720),(#353721,#353722,#353723),(#353724,#353725,#353726),(#353727,
#353728,#353729),(#353730,#353731,#353732),(#353733,#353734,#353735),(#353736,
#353737,#353738),(#353739,#353740,#353741),(#353742,#353743,#353744),(#353745,
#353746,#353747),(#353748,#353749,#353750),(#353751,#353752,#353753),(#353754,
#353755,#353756),(#353757,#353758,#353759),(#353760,#353761,#353762),(#353763,
#353764,#353765),(#353766,#353767,#353768),(#353769,#353770,#353771),(#353772,
#353773,#353774),(#353775,#353776,#353777),(#353778,#353779,#353780),(#353781,
#353782,#353783),(#353784,#353785,#353786),(#353787,#353788,#353789),(#353790,
#353791,#353792),(#353793,#353794,#353795),(#353796,#353797,#353798),(#353799,
#353800,#353801),(#353802,#353803,#353804),(#353805,#353806,#353807),(#353808,
#353809,#353810),(#353811,#353812,#353813),(#353814,#353815,#353816),(#353817,
#353818,#353819),(#353820,#353821,#353822),(#353823,#353824,#353825),(#353826,
#353827,#353828),(#353829,#353830,#353831),(#353832,#353833,#353834),(#353835,
#353836,#353837),(#353838,#353839,#353840),(#353841,#353842,#353843),(#353844,
#353845,#353846),(#353847,#353848,#353849),(#353850,#353851,#353852),(#353853,
#353854,#353855),(#353856,#353857,#353858),(#353859,#353860,#353861),(#353862,
#353863,#353864),(#353865,#353866,#353867),(#353868,#353869,#353870),(#353871,
#353872,#353873),(#353874,#353875,#353876),(#353877,#353878,#353879),(#353880,
#353881,#353882),(#353883,#353884,#353885),(#353886,#353887,#353888),(#353889,
#353890,#353891),(#353892,#353893,#353894),(#353895,#353896,#353897),(#353898,
#353899,#353900),(#353901,#353902,#353903),(#353904,#353905,#353906),(#353907,
#353908,#353909),(#353910,#353911,#353912),(#353913,#353914,#353915),(#353916,
#353917,#353918),(#353919,#353920,#353921),(#353922,#353923,#353924),(#353925,
#353926,#353927),(#353928,#353929,#353930),(#353931,#353932,#353933),(#353934,
#353935,#353936),(#353937,#353938,#353939),(#353940,#353941,#353942),(#353943,
#353944,#353945),(#353946,#353947,#353948),(#353949,#353950,#353951),(#353952,
#353953,#353954),(#353955,#353956,#353957),(#353958,#353959,#353960),(#353961,
#353962,#353963),(#353964,#353965,#353966),(#353967,#353968,#353969),(#353970,
#353971,#353972),(#353973,#353974,#353975),(#353976,#353977,#353978),(#353979,
#353980,#353981),(#353982,#353983,#353984),(#353985,#353986,#353987),(#353988,
#353989,#353990),(#353991,#353992,#353993),(#353994,#353995,#353996),(#353997,
#353998,#353999),(#354000,#354001,#354002),(#354003,#354004,#354005),(#354006,
#354007,#354008),(#354009,#354010,#354011),(#354012,#354013,#354014),(#354015,
#354016,#354017),(#354018,#354019,#354020),(#354021,#354022,#354023),(#354024,
#354025,#354026),(#354027,#354028,#354029),(#354030,#354031,#354032),(#354033,
#354034,#354035),(#354036,#354037,#354038),(#354039,#354040,#354041),(#354042,
#354043,#354044),(#354045,#354046,#354047),(#354048,#354049,#354050),(#354051,
#354052,#354053),(#354054,#354055,#354056),(#354057,#354058,#354059),(#354060,
#354061,#354062),(#354063,#354064,#354065),(#354066,#354067,#354068),(#354069,
#354070,#354071),(#354072,#354073,#354074),(#354075,#354076,#354077),(#354078,
#354079,#354080),(#354081,#354082,#354083),(#354084,#354085,#354086),(#354087,
#354088,#354089),(#354090,#354091,#354092),(#354093,#354094,#354095),(#354096,
#354097,#354098),(#354099,#354100,#354101),(#354102,#354103,#354104),(#354105,
#354106,#354107),(#354108,#354109,#354110),(#354111,#354112,#354113),(#354114,
#354115,#354116),(#354117,#354118,#354119),(#354120,#354121,#354122),(#354123,
#354124,#354125),(#354126,#354127,#354128),(#354129,#354130,#354131),(#354132,
#354133,#354134),(#354135,#354136,#354137),(#354138,#354139,#354140),(#354141,
#354142,#354143),(#354144,#354145,#354146),(#354147,#354148,#354149),(#354150,
#354151,#354152),(#354153,#354154,#354155),(#354156,#354157,#354158),(#354159,
#354160,#354161),(#354162,#354163,#354164),(#354165,#354166,#354167),(#354168,
#354169,#354170),(#354171,#354172,#354173),(#354174,#354175,#354176),(#354177,
#354178,#354179),(#354180,#354181,#354182),(#354183,#354184,#354185),(#354186,
#354187,#354188),(#354189,#354190,#354191),(#354192,#354193,#354194),(#354195,
#354196,#354197),(#354198,#354199,#354200),(#354201,#354202,#354203),(#354204,
#354205,#354206),(#354207,#354208,#354209),(#354210,#354211,#354212),(#354213,
#354214,#354215),(#354216,#354217,#354218),(#354219,#354220,#354221),(#354222,
#354223,#354224),(#354225,#354226,#354227),(#354228,#354229,#354230),(#354231,
#354232,#354233),(#354234,#354235,#354236),(#354237,#354238,#354239),(#354240,
#354241,#354242),(#354243,#354244,#354245),(#354246,#354247,#354248),(#354249,
#354250,#354251),(#354252,#354253,#354254),(#354255,#354256,#354257),(#354258,
#354259,#354260),(#354261,#354262,#354263),(#354264,#354265,#354266),(#354267,
#354268,#354269),(#354270,#354271,#354272),(#354273,#354274,#354275),(#354276,
#354277,#354278),(#354279,#354280,#354281),(#354282,#354283,#354284),(#354285,
#354286,#354287),(#354288,#354289,#354290),(#354291,#354292,#354293),(#354294,
#354295,#354296),(#354297,#354298,#354299),(#354300,#354301,#354302),(#354303,
#354304,#354305),(#354306,#354307,#354308),(#354309,#354310,#354311),(#354312,
#354313,#354314),(#354315,#354316,#354317),(#354318,#354319,#354320),(#354321,
#354322,#354323),(#354324,#354325,#354326),(#354327,#354328,#354329),(#354330,
#354331,#354332),(#354333,#354334,#354335),(#354336,#354337,#354338),(#354339,
#354340,#354341),(#354342,#354343,#354344),(#354345,#354346,#354347),(#354348,
#354349,#354350),(#354351,#354352,#354353),(#354354,#354355,#354356),(#354357,
#354358,#354359),(#354360,#354361,#354362),(#354363,#354364,#354365),(#354366,
#354367,#354368),(#354369,#354370,#354371),(#354372,#354373,#354374),(#354375,
#354376,#354377),(#354378,#354379,#354380),(#354381,#354382,#354383),(#354384,
#354385,#354386),(#354387,#354388,#354389),(#354390,#354391,#354392),(#354393,
#354394,#354395),(#354396,#354397,#354398),(#354399,#354400,#354401),(#354402,
#354403,#354404),(#354405,#354406,#354407),(#354408,#354409,#354410),(#354411,
#354412,#354413),(#354414,#354415,#354416),(#354417,#354418,#354419),(#354420,
#354421,#354422),(#354423,#354424,#354425),(#354426,#354427,#354428),(#354429,
#354430,#354431),(#354432,#354433,#354434),(#354435,#354436,#354437),(#354438,
#354439,#354440),(#354441,#354442,#354443),(#354444,#354445,#354446),(#354447,
#354448,#354449),(#354450,#354451,#354452),(#354453,#354454,#354455),(#354456,
#354457,#354458),(#354459,#354460,#354461),(#354462,#354463,#354464),(#354465,
#354466,#354467),(#354468,#354469,#354470),(#354471,#354472,#354473),(#354474,
#354475,#354476),(#354477,#354478,#354479),(#354480,#354481,#354482),(#354483,
#354484,#354485),(#354486,#354487,#354488),(#354489,#354490,#354491),(#354492,
#354493,#354494),(#354495,#354496,#354497),(#354498,#354499,#354500),(#354501,
#354502,#354503),(#354504,#354505,#354506),(#354507,#354508,#354509),(#354510,
#354511,#354512),(#354513,#354514,#354515),(#354516,#354517,#354518),(#354519,
#354520,#354521),(#354522,#354523,#354524),(#354525,#354526,#354527),(#354528,
#354529,#354530),(#354531,#354532,#354533),(#354534,#354535,#354536),(#354537,
#354538,#354539),(#354540,#354541,#354542),(#354543,#354544,#354545),(#354546,
#354547,#354548),(#354549,#354550,#354551),(#354552,#354553,#354554),(#354555,
#354556,#354557),(#354558,#354559,#354560),(#354561,#354562,#354563),(#354564,
#354565,#354566),(#354567,#354568,#354569),(#354570,#354571,#354572),(#354573,
#354574,#354575),(#354576,#354577,#354578),(#354579,#354580,#354581),(#354582,
#354583,#354584),(#354585,#354586,#354587),(#354588,#354589,#354590),(#354591,
#354592,#354593),(#354594,#354595,#354596),(#354597,#354598,#354599),(#354600,
#354601,#354602),(#354603,#354604,#354605),(#354606,#354607,#354608),(#354609,
#354610,#354611),(#354612,#354613,#354614),(#354615,#354616,#354617),(#354618,
#354619,#354620),(#354621,#354622,#354623),(#354624,#354625,#354626),(#354627,
#354628,#354629),(#354630,#354631,#354632),(#354633,#354634,#354635),(#354636,
#354637,#354638),(#354639,#354640,#354641),(#354642,#354643,#354644),(#354645,
#354646,#354647),(#354648,#354649,#354650),(#354651,#354652,#354653),(#354654,
#354655,#354656),(#354657,#354658,#354659),(#354660,#354661,#354662),(#354663,
#354664,#354665),(#354666,#354667,#354668),(#354669,#354670,#354671),(#354672,
#354673,#354674),(#354675,#354676,#354677),(#354678,#354679,#354680),(#354681,
#354682,#354683),(#354684,#354685,#354686),(#354687,#354688,#354689),(#354690,
#354691,#354692),(#354693,#354694,#354695),(#354696,#354697,#354698),(#354699,
#354700,#354701),(#354702,#354703,#354704),(#354705,#354706,#354707),(#354708,
#354709,#354710),(#354711,#354712,#354713),(#354714,#354715,#354716),(#354717,
#354718,#354719),(#354720,#354721,#354722),(#354723,#354724,#354725),(#354726,
#354727,#354728),(#354729,#354730,#354731),(#354732,#354733,#354734),(#354735,
#354736,#354737),(#354738,#354739,#354740),(#354741,#354742,#354743),(#354744,
#354745,#354746),(#354747,#354748,#354749),(#354750,#354751,#354752),(#354753,
#354754,#354755),(#354756,#354757,#354758),(#354759,#354760,#354761),(#354762,
#354763,#354764),(#354765,#354766,#354767),(#354768,#354769,#354770),(#354771,
#354772,#354773),(#354774,#354775,#354776),(#354777,#354778,#354779),(#354780,
#354781,#354782),(#354783,#354784,#354785),(#354786,#354787,#354788),(#354789,
#354790,#354791),(#354792,#354793,#354794),(#354795,#354796,#354797),(#354798,
#354799,#354800),(#354801,#354802,#354803),(#354804,#354805,#354806),(#354807,
#354808,#354809),(#354810,#354811,#354812),(#354813,#354814,#354815),(#354816,
#354817,#354818),(#354819,#354820,#354821),(#354822,#354823,#354824),(#354825,
#354826,#354827),(#354828,#354829,#354830),(#354831,#354832,#354833),(#354834,
#354835,#354836)),.UNSPECIFIED.,.F.,.F.,.F.,(6,1,1,1,1,1,1,1,1,1,1,1,1,
1,1,1,1,1,1,1,1,1,1,1,1,1,1,1,1,1,1,1,1,1,1,1,1,1,1,1,1,1,1,1,1,1,1,1,1,
1,1,1,1,1,1,1,1,1,1,1,1,1,1,1,1,1,1,1,1,1,1,1,1,1,1,1,1,1,1,1,1,1,1,1,1,
1,1,1,1,1,1,1,1,1,1,1,1,1,1,1,1,1,1,1,1,1,1,1,1,1,1,1,1,1,1,1,1,1,1,1,1,
1,1,1,1,1,1,1,1,1,1,1,1,1,1,1,1,1,1,1,1,1,1,1,1,1,1,1,1,1,1,1,1,1,1,1,1,
1,1,1,1,1,1,1,1,1,1,1,1,1,1,1,1,1,1,1,1,1,1,1,1,1,1,1,1,1,1,1,1,1,1,1,1,
1,1,1,1,1,1,1,1,1,1,1,1,1,1,1,1,1,1,1,1,1,1,1,1,1,1,1,1,1,1,1,1,1,1,1,1,
1,1,1,1,1,1,1,1,1,1,1,1,1,1,1,1,1,1,1,1,1,1,1,1,1,1,1,1,1,1,1,1,1,1,1,1,
1,1,1,1,1,1,1,1,1,1,1,1,1,1,1,1,1,1,1,1,1,1,1,1,1,1,1,1,1,1,1,1,1,1,1,1,
1,1,1,1,1,1,1,1,1,1,1,1,1,1,1,1,1,1,1,1,1,1,1,1,1,1,1,1,1,1,1,1,1,1,1,1,
1,1,1,1,1,1,1,1,1,1,1,1,1,1,1,1,1,1,1,1,1,1,1,1,1,1,1,1,1,1,1,1,1,1,1,1,
1,1,1,1,1,1,1,1,1,1,1,1,1,1,1,1,1,1,1,1,1,1,1,1,1,1,1,1,1,1,1,1,1,1,1,1,
1,1,1,1,1,1,1,1,1,1,1,1,1,1,1,1,1,1,1,1,1,1,1,1,1,1,1,1,1,1,1,1,1,1,1,1,
1,1,1,1,1,1,1,1,1,1,1,1,1,1,1,1,1,1,1,1,1,1,1,1,1,1,1,1,1,1,1,1,1,1,1,1,
1,1,1,1,1,1,1,1,1,1,1,1,1,1,1,1,1,1,1,1,1,1,1,1,1,1,1,1,1,1,1,1,1,1,1,1,
1,1,1,1,1,1,1,1,1,1,1,1,1,1,1,1,1,1,1,1,1,1,1,1,1,1,1,1,1,6),(2,1,2),(-0.001964168,
0.,0.001834862,0.003669725,0.005504587,0.00733945,0.009174312,0.011009174,
0.012844037,0.014678899,0.016513761,0.018348624,0.020183486,0.022018349,
0.023853211,0.025688073,0.027522936,0.029357798,0.031192661,0.033027523,
0.034862385,0.036697248,0.03853211,0.040366972,0.042201835,0.044036697,
0.04587156,0.047706422,0.049541284,0.051376147,0.053211009,0.055045872,
0.056880734,0.058715596,0.060550459,0.062385321,0.064220183,0.066055046,
0.067889908,0.069724771,0.071559633,0.073394495,0.075229358,0.07706422,
0.078899083,0.080733945,0.082568807,0.08440367,0.086238532,0.088073394,
0.089908257,0.091743119,0.093577982,0.095412844,0.097247706,0.099082569,
0.100917431,0.102752294,0.104587156,0.106422018,0.108256881,0.110091743,
0.111926606,0.113761468,0.11559633,0.117431193,0.119266055,0.121100917,
0.12293578,0.124770642,0.126605505,0.128440367,0.130275229,0.132110092,
0.133944954,0.135779817,0.137614679,0.139449541,0.141284404,0.143119266,
0.144954128,0.146788991,0.148623853,0.150458716,0.152293578,0.15412844,
0.155963303,0.157798165,0.159633028,0.16146789,0.163302752,0.165137615,
0.166972477,0.168807339,0.170642202,0.172477064,0.174311927,0.176146789,
0.177981651,0.179816514,0.181651376,0.183486239,0.185321101,0.187155963,
0.188990826,0.190825688,0.19266055,0.194495413,0.196330275,0.198165138,
0.2,0.201834862,0.203669725,0.205504587,0.20733945,0.209174312,0.211009174,
0.212844037,0.214678899,0.216513761,0.218348624,0.220183486,0.222018349,
0.223853211,0.225688073,0.227522936,0.229357798,0.231192661,0.233027523,
0.234862385,0.236697248,0.23853211,0.240366972,0.242201835,0.244036697,
0.24587156,0.247706422,0.249541284,0.251376147,0.253211009,0.255045872,
0.256880734,0.258715596,0.260550459,0.262385321,0.264220183,0.266055046,
0.267889908,0.269724771,0.271559633,0.273394495,0.275229358,0.27706422,
0.278899083,0.280733945,0.282568807,0.28440367,0.286238532,0.288073394,
0.289908257,0.291743119,0.293577982,0.295412844,0.297247706,0.299082569,
0.300917431,0.302752294,0.304587156,0.306422018,0.308256881,0.310091743,
0.311926606,0.313761468,0.31559633,0.317431193,0.319266055,0.321100917,
0.32293578,0.324770642,0.326605505,0.328440367,0.330275229,0.332110092,
0.333944954,0.335779817,0.337614679,0.339449541,0.341284404,0.343119266,
0.344954128,0.346788991,0.348623853,0.350458716,0.352293578,0.35412844,
0.355963303,0.357798165,0.359633028,0.36146789,0.363302752,0.365137615,
0.366972477,0.368807339,0.370642202,0.372477064,0.374311927,0.376146789,
0.377981651,0.379816514,0.381651376,0.383486239,0.385321101,0.387155963,
0.388990826,0.390825688,0.39266055,0.394495413,0.396330275,0.398165138,
0.4,0.401834862,0.403669725,0.405504587,0.40733945,0.409174312,0.411009174,
0.412844037,0.414678899,0.416513761,0.418348624,0.420183486,0.422018349,
0.423853211,0.425688073,0.427522936,0.429357798,0.431192661,0.433027523,
0.434862385,0.436697248,0.43853211,0.440366972,0.442201835,0.444036697,
0.44587156,0.447706422,0.449541284,0.451376147,0.453211009,0.455045872,
0.456880734,0.458715596,0.460550459,0.462385321,0.464220183,0.466055046,
0.467889908,0.469724771,0.471559633,0.473394495,0.475229358,0.47706422,
0.478899083,0.480733945,0.482568807,0.48440367,0.486238532,0.488073394,
0.489908257,0.491743119,0.493577982,0.495412844,0.497247706,0.499082569,
0.500917431,0.502752294,0.504587156,0.506422018,0.508256881,0.510091743,
0.511926606,0.513761468,0.51559633,0.517431193,0.519266055,0.521100917,
0.52293578,0.524770642,0.526605505,0.528440367,0.530275229,0.532110092,
0.533944954,0.535779817,0.537614679,0.539449541,0.541284404,0.543119266,
0.544954128,0.546788991,0.548623853,0.550458716,0.552293578,0.55412844,
0.555963303,0.557798165,0.559633028,0.56146789,0.563302752,0.565137615,
0.566972477,0.568807339,0.570642202,0.572477064,0.574311927,0.576146789,
0.577981651,0.579816514,0.581651376,0.583486239,0.585321101,0.587155963,
0.588990826,0.590825688,0.59266055,0.594495413,0.596330275,0.598165138,
0.6,0.601834862,0.603669725,0.605504587,0.60733945,0.609174312,0.611009174,
0.612844037,0.614678899,0.616513761,0.618348624,0.620183486,0.622018349,
0.623853211,0.625688073,0.627522936,0.629357798,0.631192661,0.633027523,
0.634862385,0.636697248,0.63853211,0.640366972,0.642201835,0.644036697,
0.64587156,0.647706422,0.649541284,0.651376147,0.653211009,0.655045872,
0.656880734,0.658715596,0.660550459,0.662385321,0.664220183,0.666055046,
0.667889908,0.669724771,0.671559633,0.673394495,0.675229358,0.67706422,
0.678899083,0.680733945,0.682568807,0.68440367,0.686238532,0.688073394,
0.689908257,0.691743119,0.693577982,0.695412844,0.697247706,0.699082569,
0.700917431,0.702752294,0.704587156,0.706422018,0.708256881,0.710091743,
0.711926606,0.713761468,0.71559633,0.717431193,0.719266055,0.721100917,
0.72293578,0.724770642,0.726605505,0.728440367,0.730275229,0.732110092,
0.733944954,0.735779817,0.737614679,0.739449541,0.741284404,0.743119266,
0.744954128,0.746788991,0.748623853,0.750458716,0.752293578,0.75412844,
0.755963303,0.757798165,0.759633028,0.76146789,0.763302752,0.765137615,
0.766972477,0.768807339,0.770642202,0.772477064,0.774311927,0.776146789,
0.777981651,0.779816514,0.781651376,0.783486239,0.785321101,0.787155963,
0.788990826,0.790825688,0.79266055,0.794495413,0.796330275,0.798165138,
0.8,0.801834862,0.803669725,0.805504587,0.80733945,0.809174312,0.811009174,
0.812844037,0.814678899,0.816513761,0.818348624,0.820183486,0.822018349,
0.823853211,0.825688073,0.827522936,0.829357798,0.831192661,0.833027523,
0.834862385,0.836697248,0.83853211,0.840366972,0.842201835,0.844036697,
0.84587156,0.847706422,0.849541284,0.851376147,0.853211009,0.855045872,
0.856880734,0.858715596,0.860550459,0.862385321,0.864220183,0.866055046,
0.867889908,0.869724771,0.871559633,0.873394495,0.875229358,0.87706422,
0.878899083,0.880733945,0.882568807,0.88440367,0.886238532,0.888073394,
0.889908257,0.891743119,0.893577982,0.895412844,0.897247706,0.899082569,
0.900917431,0.902752294,0.904587156,0.906422018,0.908256881,0.910091743,
0.911926606,0.913761468,0.91559633,0.917431193,0.919266055,0.921100917,
0.92293578,0.924770642,0.926605505,0.928440367,0.930275229,0.932110092,
0.933944954,0.935779817,0.937614679,0.939449541,0.941284404,0.943119266,
0.944954128,0.946788991,0.948623853,0.950458716,0.952293578,0.95412844,
0.955963303,0.957798165,0.959633028,0.96146789,0.963302752,0.965137615,
0.966972477,0.968807339,0.970642202,0.972477064,0.974311927,0.976146789,
0.977981651,0.979816514,0.981651376,0.983486239,0.985321101,0.987155963,
0.988990826,0.990825688,0.99266055,0.994495413,0.996330275,0.998165138,
1.),(0.3,1.,1.3),.UNSPECIFIED.);
#6335=B_SPLINE_SURFACE_WITH_KNOTS('',5,1,((#354848,#354849,#354850),(#354851,
#354852,#354853),(#354854,#354855,#354856),(#354857,#354858,#354859),(#354860,
#354861,#354862),(#354863,#354864,#354865),(#354866,#354867,#354868),(#354869,
#354870,#354871),(#354872,#354873,#354874),(#354875,#354876,#354877),(#354878,
#354879,#354880),(#354881,#354882,#354883),(#354884,#354885,#354886),(#354887,
#354888,#354889),(#354890,#354891,#354892),(#354893,#354894,#354895),(#354896,
#354897,#354898),(#354899,#354900,#354901),(#354902,#354903,#354904),(#354905,
#354906,#354907),(#354908,#354909,#354910),(#354911,#354912,#354913),(#354914,
#354915,#354916),(#354917,#354918,#354919),(#354920,#354921,#354922),(#354923,
#354924,#354925),(#354926,#354927,#354928),(#354929,#354930,#354931),(#354932,
#354933,#354934),(#354935,#354936,#354937),(#354938,#354939,#354940),(#354941,
#354942,#354943),(#354944,#354945,#354946),(#354947,#354948,#354949),(#354950,
#354951,#354952),(#354953,#354954,#354955),(#354956,#354957,#354958),(#354959,
#354960,#354961),(#354962,#354963,#354964),(#354965,#354966,#354967),(#354968,
#354969,#354970),(#354971,#354972,#354973),(#354974,#354975,#354976),(#354977,
#354978,#354979),(#354980,#354981,#354982),(#354983,#354984,#354985),(#354986,
#354987,#354988),(#354989,#354990,#354991),(#354992,#354993,#354994),(#354995,
#354996,#354997),(#354998,#354999,#355000),(#355001,#355002,#355003),(#355004,
#355005,#355006),(#355007,#355008,#355009),(#355010,#355011,#355012),(#355013,
#355014,#355015),(#355016,#355017,#355018),(#355019,#355020,#355021),(#355022,
#355023,#355024),(#355025,#355026,#355027),(#355028,#355029,#355030),(#355031,
#355032,#355033),(#355034,#355035,#355036),(#355037,#355038,#355039),(#355040,
#355041,#355042),(#355043,#355044,#355045),(#355046,#355047,#355048),(#355049,
#355050,#355051),(#355052,#355053,#355054),(#355055,#355056,#355057),(#355058,
#355059,#355060),(#355061,#355062,#355063),(#355064,#355065,#355066),(#355067,
#355068,#355069),(#355070,#355071,#355072),(#355073,#355074,#355075),(#355076,
#355077,#355078),(#355079,#355080,#355081),(#355082,#355083,#355084),(#355085,
#355086,#355087),(#355088,#355089,#355090),(#355091,#355092,#355093),(#355094,
#355095,#355096),(#355097,#355098,#355099),(#355100,#355101,#355102),(#355103,
#355104,#355105),(#355106,#355107,#355108),(#355109,#355110,#355111),(#355112,
#355113,#355114),(#355115,#355116,#355117),(#355118,#355119,#355120),(#355121,
#355122,#355123),(#355124,#355125,#355126),(#355127,#355128,#355129),(#355130,
#355131,#355132),(#355133,#355134,#355135),(#355136,#355137,#355138),(#355139,
#355140,#355141),(#355142,#355143,#355144),(#355145,#355146,#355147),(#355148,
#355149,#355150),(#355151,#355152,#355153),(#355154,#355155,#355156),(#355157,
#355158,#355159),(#355160,#355161,#355162),(#355163,#355164,#355165),(#355166,
#355167,#355168),(#355169,#355170,#355171),(#355172,#355173,#355174),(#355175,
#355176,#355177),(#355178,#355179,#355180),(#355181,#355182,#355183),(#355184,
#355185,#355186),(#355187,#355188,#355189),(#355190,#355191,#355192),(#355193,
#355194,#355195),(#355196,#355197,#355198),(#355199,#355200,#355201),(#355202,
#355203,#355204),(#355205,#355206,#355207),(#355208,#355209,#355210),(#355211,
#355212,#355213),(#355214,#355215,#355216),(#355217,#355218,#355219),(#355220,
#355221,#355222),(#355223,#355224,#355225),(#355226,#355227,#355228),(#355229,
#355230,#355231),(#355232,#355233,#355234),(#355235,#355236,#355237),(#355238,
#355239,#355240),(#355241,#355242,#355243),(#355244,#355245,#355246),(#355247,
#355248,#355249),(#355250,#355251,#355252),(#355253,#355254,#355255),(#355256,
#355257,#355258),(#355259,#355260,#355261),(#355262,#355263,#355264),(#355265,
#355266,#355267),(#355268,#355269,#355270),(#355271,#355272,#355273),(#355274,
#355275,#355276),(#355277,#355278,#355279),(#355280,#355281,#355282),(#355283,
#355284,#355285),(#355286,#355287,#355288),(#355289,#355290,#355291),(#355292,
#355293,#355294),(#355295,#355296,#355297),(#355298,#355299,#355300),(#355301,
#355302,#355303),(#355304,#355305,#355306),(#355307,#355308,#355309),(#355310,
#355311,#355312),(#355313,#355314,#355315),(#355316,#355317,#355318),(#355319,
#355320,#355321),(#355322,#355323,#355324),(#355325,#355326,#355327),(#355328,
#355329,#355330),(#355331,#355332,#355333),(#355334,#355335,#355336),(#355337,
#355338,#355339),(#355340,#355341,#355342),(#355343,#355344,#355345),(#355346,
#355347,#355348),(#355349,#355350,#355351),(#355352,#355353,#355354),(#355355,
#355356,#355357),(#355358,#355359,#355360),(#355361,#355362,#355363),(#355364,
#355365,#355366),(#355367,#355368,#355369),(#355370,#355371,#355372),(#355373,
#355374,#355375),(#355376,#355377,#355378),(#355379,#355380,#355381),(#355382,
#355383,#355384),(#355385,#355386,#355387),(#355388,#355389,#355390),(#355391,
#355392,#355393),(#355394,#355395,#355396),(#355397,#355398,#355399),(#355400,
#355401,#355402),(#355403,#355404,#355405),(#355406,#355407,#355408),(#355409,
#355410,#355411),(#355412,#355413,#355414),(#355415,#355416,#355417),(#355418,
#355419,#355420),(#355421,#355422,#355423),(#355424,#355425,#355426),(#355427,
#355428,#355429),(#355430,#355431,#355432),(#355433,#355434,#355435),(#355436,
#355437,#355438),(#355439,#355440,#355441),(#355442,#355443,#355444),(#355445,
#355446,#355447),(#355448,#355449,#355450),(#355451,#355452,#355453),(#355454,
#355455,#355456),(#355457,#355458,#355459),(#355460,#355461,#355462),(#355463,
#355464,#355465),(#355466,#355467,#355468),(#355469,#355470,#355471),(#355472,
#355473,#355474),(#355475,#355476,#355477),(#355478,#355479,#355480),(#355481,
#355482,#355483),(#355484,#355485,#355486),(#355487,#355488,#355489),(#355490,
#355491,#355492),(#355493,#355494,#355495),(#355496,#355497,#355498),(#355499,
#355500,#355501),(#355502,#355503,#355504),(#355505,#355506,#355507),(#355508,
#355509,#355510),(#355511,#355512,#355513),(#355514,#355515,#355516),(#355517,
#355518,#355519),(#355520,#355521,#355522),(#355523,#355524,#355525),(#355526,
#355527,#355528),(#355529,#355530,#355531),(#355532,#355533,#355534),(#355535,
#355536,#355537),(#355538,#355539,#355540),(#355541,#355542,#355543),(#355544,
#355545,#355546),(#355547,#355548,#355549),(#355550,#355551,#355552),(#355553,
#355554,#355555),(#355556,#355557,#355558),(#355559,#355560,#355561),(#355562,
#355563,#355564),(#355565,#355566,#355567),(#355568,#355569,#355570),(#355571,
#355572,#355573),(#355574,#355575,#355576),(#355577,#355578,#355579),(#355580,
#355581,#355582),(#355583,#355584,#355585),(#355586,#355587,#355588),(#355589,
#355590,#355591),(#355592,#355593,#355594),(#355595,#355596,#355597),(#355598,
#355599,#355600),(#355601,#355602,#355603),(#355604,#355605,#355606),(#355607,
#355608,#355609),(#355610,#355611,#355612),(#355613,#355614,#355615),(#355616,
#355617,#355618),(#355619,#355620,#355621),(#355622,#355623,#355624),(#355625,
#355626,#355627),(#355628,#355629,#355630),(#355631,#355632,#355633),(#355634,
#355635,#355636),(#355637,#355638,#355639),(#355640,#355641,#355642),(#355643,
#355644,#355645),(#355646,#355647,#355648),(#355649,#355650,#355651),(#355652,
#355653,#355654),(#355655,#355656,#355657),(#355658,#355659,#355660),(#355661,
#355662,#355663),(#355664,#355665,#355666),(#355667,#355668,#355669),(#355670,
#355671,#355672),(#355673,#355674,#355675),(#355676,#355677,#355678),(#355679,
#355680,#355681),(#355682,#355683,#355684),(#355685,#355686,#355687),(#355688,
#355689,#355690),(#355691,#355692,#355693),(#355694,#355695,#355696),(#355697,
#355698,#355699),(#355700,#355701,#355702),(#355703,#355704,#355705),(#355706,
#355707,#355708),(#355709,#355710,#355711),(#355712,#355713,#355714),(#355715,
#355716,#355717),(#355718,#355719,#355720),(#355721,#355722,#355723),(#355724,
#355725,#355726),(#355727,#355728,#355729),(#355730,#355731,#355732),(#355733,
#355734,#355735),(#355736,#355737,#355738),(#355739,#355740,#355741),(#355742,
#355743,#355744),(#355745,#355746,#355747),(#355748,#355749,#355750),(#355751,
#355752,#355753),(#355754,#355755,#355756),(#355757,#355758,#355759),(#355760,
#355761,#355762),(#355763,#355764,#355765),(#355766,#355767,#355768),(#355769,
#355770,#355771),(#355772,#355773,#355774),(#355775,#355776,#355777),(#355778,
#355779,#355780),(#355781,#355782,#355783),(#355784,#355785,#355786),(#355787,
#355788,#355789),(#355790,#355791,#355792),(#355793,#355794,#355795),(#355796,
#355797,#355798),(#355799,#355800,#355801),(#355802,#355803,#355804),(#355805,
#355806,#355807),(#355808,#355809,#355810),(#355811,#355812,#355813),(#355814,
#355815,#355816),(#355817,#355818,#355819),(#355820,#355821,#355822),(#355823,
#355824,#355825),(#355826,#355827,#355828),(#355829,#355830,#355831),(#355832,
#355833,#355834),(#355835,#355836,#355837),(#355838,#355839,#355840),(#355841,
#355842,#355843),(#355844,#355845,#355846),(#355847,#355848,#355849),(#355850,
#355851,#355852),(#355853,#355854,#355855),(#355856,#355857,#355858),(#355859,
#355860,#355861),(#355862,#355863,#355864),(#355865,#355866,#355867),(#355868,
#355869,#355870),(#355871,#355872,#355873),(#355874,#355875,#355876),(#355877,
#355878,#355879),(#355880,#355881,#355882),(#355883,#355884,#355885),(#355886,
#355887,#355888),(#355889,#355890,#355891),(#355892,#355893,#355894),(#355895,
#355896,#355897),(#355898,#355899,#355900),(#355901,#355902,#355903),(#355904,
#355905,#355906),(#355907,#355908,#355909),(#355910,#355911,#355912),(#355913,
#355914,#355915),(#355916,#355917,#355918),(#355919,#355920,#355921),(#355922,
#355923,#355924),(#355925,#355926,#355927),(#355928,#355929,#355930),(#355931,
#355932,#355933),(#355934,#355935,#355936),(#355937,#355938,#355939),(#355940,
#355941,#355942),(#355943,#355944,#355945),(#355946,#355947,#355948),(#355949,
#355950,#355951),(#355952,#355953,#355954),(#355955,#355956,#355957),(#355958,
#355959,#355960),(#355961,#355962,#355963),(#355964,#355965,#355966),(#355967,
#355968,#355969),(#355970,#355971,#355972),(#355973,#355974,#355975),(#355976,
#355977,#355978),(#355979,#355980,#355981),(#355982,#355983,#355984),(#355985,
#355986,#355987),(#355988,#355989,#355990),(#355991,#355992,#355993),(#355994,
#355995,#355996),(#355997,#355998,#355999),(#356000,#356001,#356002),(#356003,
#356004,#356005),(#356006,#356007,#356008),(#356009,#356010,#356011),(#356012,
#356013,#356014),(#356015,#356016,#356017),(#356018,#356019,#356020),(#356021,
#356022,#356023),(#356024,#356025,#356026),(#356027,#356028,#356029),(#356030,
#356031,#356032),(#356033,#356034,#356035),(#356036,#356037,#356038),(#356039,
#356040,#356041),(#356042,#356043,#356044),(#356045,#356046,#356047),(#356048,
#356049,#356050),(#356051,#356052,#356053),(#356054,#356055,#356056),(#356057,
#356058,#356059),(#356060,#356061,#356062),(#356063,#356064,#356065),(#356066,
#356067,#356068),(#356069,#356070,#356071),(#356072,#356073,#356074),(#356075,
#356076,#356077),(#356078,#356079,#356080),(#356081,#356082,#356083),(#356084,
#356085,#356086),(#356087,#356088,#356089),(#356090,#356091,#356092),(#356093,
#356094,#356095),(#356096,#356097,#356098),(#356099,#356100,#356101),(#356102,
#356103,#356104),(#356105,#356106,#356107),(#356108,#356109,#356110),(#356111,
#356112,#356113),(#356114,#356115,#356116),(#356117,#356118,#356119),(#356120,
#356121,#356122),(#356123,#356124,#356125),(#356126,#356127,#356128),(#356129,
#356130,#356131),(#356132,#356133,#356134),(#356135,#356136,#356137),(#356138,
#356139,#356140),(#356141,#356142,#356143),(#356144,#356145,#356146),(#356147,
#356148,#356149),(#356150,#356151,#356152),(#356153,#356154,#356155),(#356156,
#356157,#356158),(#356159,#356160,#356161),(#356162,#356163,#356164),(#356165,
#356166,#356167),(#356168,#356169,#356170),(#356171,#356172,#356173),(#356174,
#356175,#356176),(#356177,#356178,#356179),(#356180,#356181,#356182),(#356183,
#356184,#356185),(#356186,#356187,#356188),(#356189,#356190,#356191),(#356192,
#356193,#356194),(#356195,#356196,#356197),(#356198,#356199,#356200),(#356201,
#356202,#356203),(#356204,#356205,#356206),(#356207,#356208,#356209),(#356210,
#356211,#356212),(#356213,#356214,#356215),(#356216,#356217,#356218),(#356219,
#356220,#356221),(#356222,#356223,#356224),(#356225,#356226,#356227),(#356228,
#356229,#356230),(#356231,#356232,#356233),(#356234,#356235,#356236),(#356237,
#356238,#356239),(#356240,#356241,#356242),(#356243,#356244,#356245),(#356246,
#356247,#356248),(#356249,#356250,#356251),(#356252,#356253,#356254),(#356255,
#356256,#356257),(#356258,#356259,#356260),(#356261,#356262,#356263),(#356264,
#356265,#356266),(#356267,#356268,#356269),(#356270,#356271,#356272),(#356273,
#356274,#356275),(#356276,#356277,#356278),(#356279,#356280,#356281),(#356282,
#356283,#356284),(#356285,#356286,#356287),(#356288,#356289,#356290),(#356291,
#356292,#356293),(#356294,#356295,#356296),(#356297,#356298,#356299),(#356300,
#356301,#356302),(#356303,#356304,#356305),(#356306,#356307,#356308),(#356309,
#356310,#356311),(#356312,#356313,#356314),(#356315,#356316,#356317),(#356318,
#356319,#356320),(#356321,#356322,#356323),(#356324,#356325,#356326),(#356327,
#356328,#356329),(#356330,#356331,#356332),(#356333,#356334,#356335),(#356336,
#356337,#356338),(#356339,#356340,#356341),(#356342,#356343,#356344),(#356345,
#356346,#356347),(#356348,#356349,#356350),(#356351,#356352,#356353),(#356354,
#356355,#356356),(#356357,#356358,#356359),(#356360,#356361,#356362),(#356363,
#356364,#356365),(#356366,#356367,#356368),(#356369,#356370,#356371),(#356372,
#356373,#356374),(#356375,#356376,#356377),(#356378,#356379,#356380),(#356381,
#356382,#356383),(#356384,#356385,#356386),(#356387,#356388,#356389),(#356390,
#356391,#356392),(#356393,#356394,#356395),(#356396,#356397,#356398),(#356399,
#356400,#356401),(#356402,#356403,#356404),(#356405,#356406,#356407),(#356408,
#356409,#356410),(#356411,#356412,#356413),(#356414,#356415,#356416),(#356417,
#356418,#356419),(#356420,#356421,#356422),(#356423,#356424,#356425),(#356426,
#356427,#356428),(#356429,#356430,#356431),(#356432,#356433,#356434),(#356435,
#356436,#356437),(#356438,#356439,#356440),(#356441,#356442,#356443),(#356444,
#356445,#356446),(#356447,#356448,#356449),(#356450,#356451,#356452),(#356453,
#356454,#356455),(#356456,#356457,#356458),(#356459,#356460,#356461),(#356462,
#356463,#356464),(#356465,#356466,#356467),(#356468,#356469,#356470),(#356471,
#356472,#356473),(#356474,#356475,#356476),(#356477,#356478,#356479),(#356480,
#356481,#356482),(#356483,#356484,#356485),(#356486,#356487,#356488),(#356489,
#356490,#356491),(#356492,#356493,#356494),(#356495,#356496,#356497)),
 .UNSPECIFIED.,.F.,.F.,.F.,(6,1,1,1,1,1,1,1,1,1,1,1,1,1,1,1,1,1,1,1,1,1,
1,1,1,1,1,1,1,1,1,1,1,1,1,1,1,1,1,1,1,1,1,1,1,1,1,1,1,1,1,1,1,1,1,1,1,1,
1,1,1,1,1,1,1,1,1,1,1,1,1,1,1,1,1,1,1,1,1,1,1,1,1,1,1,1,1,1,1,1,1,1,1,1,
1,1,1,1,1,1,1,1,1,1,1,1,1,1,1,1,1,1,1,1,1,1,1,1,1,1,1,1,1,1,1,1,1,1,1,1,
1,1,1,1,1,1,1,1,1,1,1,1,1,1,1,1,1,1,1,1,1,1,1,1,1,1,1,1,1,1,1,1,1,1,1,1,
1,1,1,1,1,1,1,1,1,1,1,1,1,1,1,1,1,1,1,1,1,1,1,1,1,1,1,1,1,1,1,1,1,1,1,1,
1,1,1,1,1,1,1,1,1,1,1,1,1,1,1,1,1,1,1,1,1,1,1,1,1,1,1,1,1,1,1,1,1,1,1,1,
1,1,1,1,1,1,1,1,1,1,1,1,1,1,1,1,1,1,1,1,1,1,1,1,1,1,1,1,1,1,1,1,1,1,1,1,
1,1,1,1,1,1,1,1,1,1,1,1,1,1,1,1,1,1,1,1,1,1,1,1,1,1,1,1,1,1,1,1,1,1,1,1,
1,1,1,1,1,1,1,1,1,1,1,1,1,1,1,1,1,1,1,1,1,1,1,1,1,1,1,1,1,1,1,1,1,1,1,1,
1,1,1,1,1,1,1,1,1,1,1,1,1,1,1,1,1,1,1,1,1,1,1,1,1,1,1,1,1,1,1,1,1,1,1,1,
1,1,1,1,1,1,1,1,1,1,1,1,1,1,1,1,1,1,1,1,1,1,1,1,1,1,1,1,1,1,1,1,1,1,1,1,
1,1,1,1,1,1,1,1,1,1,1,1,1,1,1,1,1,1,1,1,1,1,1,1,1,1,1,1,1,1,1,1,1,1,1,1,
1,1,1,1,1,1,1,1,1,1,1,1,1,1,1,1,1,1,1,1,1,1,1,1,1,1,1,1,1,1,1,1,1,1,1,1,
1,1,1,1,1,1,1,1,1,1,1,1,1,1,1,1,1,1,1,1,1,1,1,1,1,1,1,1,1,1,1,1,1,1,1,1,
1,1,1,1,1,1,1,1,1,1,1,1,1,1,1,1,1,1,1,6),(2,1,2),(-1.,-0.998165138,-0.996330275,
-0.994495413,-0.99266055,-0.990825688,-0.988990826,-0.987155963,-0.985321101,
-0.983486239,-0.981651376,-0.979816514,-0.977981651,-0.976146789,-0.974311927,
-0.972477064,-0.970642202,-0.968807339,-0.966972477,-0.965137615,-0.963302752,
-0.96146789,-0.959633028,-0.957798165,-0.955963303,-0.95412844,-0.952293578,
-0.950458716,-0.948623853,-0.946788991,-0.944954128,-0.943119266,-0.941284404,
-0.939449541,-0.937614679,-0.935779817,-0.933944954,-0.932110092,-0.930275229,
-0.928440367,-0.926605505,-0.924770642,-0.92293578,-0.921100917,-0.919266055,
-0.917431193,-0.91559633,-0.913761468,-0.911926606,-0.910091743,-0.908256881,
-0.906422018,-0.904587156,-0.902752294,-0.900917431,-0.899082569,-0.897247706,
-0.895412844,-0.893577982,-0.891743119,-0.889908257,-0.888073394,-0.886238532,
-0.88440367,-0.882568807,-0.880733945,-0.878899083,-0.87706422,-0.875229358,
-0.873394495,-0.871559633,-0.869724771,-0.867889908,-0.866055046,-0.864220183,
-0.862385321,-0.860550459,-0.858715596,-0.856880734,-0.855045872,-0.853211009,
-0.851376147,-0.849541284,-0.847706422,-0.84587156,-0.844036697,-0.842201835,
-0.840366972,-0.83853211,-0.836697248,-0.834862385,-0.833027523,-0.831192661,
-0.829357798,-0.827522936,-0.825688073,-0.823853211,-0.822018349,-0.820183486,
-0.818348624,-0.816513761,-0.814678899,-0.812844037,-0.811009174,-0.809174312,
-0.80733945,-0.805504587,-0.803669725,-0.801834862,-0.8,-0.798165138,-0.796330275,
-0.794495413,-0.79266055,-0.790825688,-0.788990826,-0.787155963,-0.785321101,
-0.783486239,-0.781651376,-0.779816514,-0.777981651,-0.776146789,-0.774311927,
-0.772477064,-0.770642202,-0.768807339,-0.766972477,-0.765137615,-0.763302752,
-0.76146789,-0.759633028,-0.757798165,-0.755963303,-0.75412844,-0.752293578,
-0.750458716,-0.748623853,-0.746788991,-0.744954128,-0.743119266,-0.741284404,
-0.739449541,-0.737614679,-0.735779817,-0.733944954,-0.732110092,-0.730275229,
-0.728440367,-0.726605505,-0.724770642,-0.72293578,-0.721100917,-0.719266055,
-0.717431193,-0.71559633,-0.713761468,-0.711926606,-0.710091743,-0.708256881,
-0.706422018,-0.704587156,-0.702752294,-0.700917431,-0.699082569,-0.697247706,
-0.695412844,-0.693577982,-0.691743119,-0.689908257,-0.688073394,-0.686238532,
-0.68440367,-0.682568807,-0.680733945,-0.678899083,-0.67706422,-0.675229358,
-0.673394495,-0.671559633,-0.669724771,-0.667889908,-0.666055046,-0.664220183,
-0.662385321,-0.660550459,-0.658715596,-0.656880734,-0.655045872,-0.653211009,
-0.651376147,-0.649541284,-0.647706422,-0.64587156,-0.644036697,-0.642201835,
-0.640366972,-0.63853211,-0.636697248,-0.634862385,-0.633027523,-0.631192661,
-0.629357798,-0.627522936,-0.625688073,-0.623853211,-0.622018349,-0.620183486,
-0.618348624,-0.616513761,-0.614678899,-0.612844037,-0.611009174,-0.609174312,
-0.60733945,-0.605504587,-0.603669725,-0.601834862,-0.6,-0.598165138,-0.596330275,
-0.594495413,-0.59266055,-0.590825688,-0.588990826,-0.587155963,-0.585321101,
-0.583486239,-0.581651376,-0.579816514,-0.577981651,-0.576146789,-0.574311927,
-0.572477064,-0.570642202,-0.568807339,-0.566972477,-0.565137615,-0.563302752,
-0.56146789,-0.559633028,-0.557798165,-0.555963303,-0.55412844,-0.552293578,
-0.550458716,-0.548623853,-0.546788991,-0.544954128,-0.543119266,-0.541284404,
-0.539449541,-0.537614679,-0.535779817,-0.533944954,-0.532110092,-0.530275229,
-0.528440367,-0.526605505,-0.524770642,-0.52293578,-0.521100917,-0.519266055,
-0.517431193,-0.51559633,-0.513761468,-0.511926606,-0.510091743,-0.508256881,
-0.506422018,-0.504587156,-0.502752294,-0.500917431,-0.499082569,-0.497247706,
-0.495412844,-0.493577982,-0.491743119,-0.489908257,-0.488073394,-0.486238532,
-0.48440367,-0.482568807,-0.480733945,-0.478899083,-0.47706422,-0.475229358,
-0.473394495,-0.471559633,-0.469724771,-0.467889908,-0.466055046,-0.464220183,
-0.462385321,-0.460550459,-0.458715596,-0.456880734,-0.455045872,-0.453211009,
-0.451376147,-0.449541284,-0.447706422,-0.44587156,-0.444036697,-0.442201835,
-0.440366972,-0.43853211,-0.436697248,-0.434862385,-0.433027523,-0.431192661,
-0.429357798,-0.427522936,-0.425688073,-0.423853211,-0.422018349,-0.420183486,
-0.418348624,-0.416513761,-0.414678899,-0.412844037,-0.411009174,-0.409174312,
-0.40733945,-0.405504587,-0.403669725,-0.401834862,-0.4,-0.398165138,-0.396330275,
-0.394495413,-0.39266055,-0.390825688,-0.388990826,-0.387155963,-0.385321101,
-0.383486239,-0.381651376,-0.379816514,-0.377981651,-0.376146789,-0.374311927,
-0.372477064,-0.370642202,-0.368807339,-0.366972477,-0.365137615,-0.363302752,
-0.36146789,-0.359633028,-0.357798165,-0.355963303,-0.35412844,-0.352293578,
-0.350458716,-0.348623853,-0.346788991,-0.344954128,-0.343119266,-0.341284404,
-0.339449541,-0.337614679,-0.335779817,-0.333944954,-0.332110092,-0.330275229,
-0.328440367,-0.326605505,-0.324770642,-0.32293578,-0.321100917,-0.319266055,
-0.317431193,-0.31559633,-0.313761468,-0.311926606,-0.310091743,-0.308256881,
-0.306422018,-0.304587156,-0.302752294,-0.300917431,-0.299082569,-0.297247706,
-0.295412844,-0.293577982,-0.291743119,-0.289908257,-0.288073394,-0.286238532,
-0.28440367,-0.282568807,-0.280733945,-0.278899083,-0.27706422,-0.275229358,
-0.273394495,-0.271559633,-0.269724771,-0.267889908,-0.266055046,-0.264220183,
-0.262385321,-0.260550459,-0.258715596,-0.256880734,-0.255045872,-0.253211009,
-0.251376147,-0.249541284,-0.247706422,-0.24587156,-0.244036697,-0.242201835,
-0.240366972,-0.23853211,-0.236697248,-0.234862385,-0.233027523,-0.231192661,
-0.229357798,-0.227522936,-0.225688073,-0.223853211,-0.222018349,-0.220183486,
-0.218348624,-0.216513761,-0.214678899,-0.212844037,-0.211009174,-0.209174312,
-0.20733945,-0.205504587,-0.203669725,-0.201834862,-0.2,-0.198165138,-0.196330275,
-0.194495413,-0.19266055,-0.190825688,-0.188990826,-0.187155963,-0.185321101,
-0.183486239,-0.181651376,-0.179816514,-0.177981651,-0.176146789,-0.174311927,
-0.172477064,-0.170642202,-0.168807339,-0.166972477,-0.165137615,-0.163302752,
-0.16146789,-0.159633028,-0.157798165,-0.155963303,-0.15412844,-0.152293578,
-0.150458716,-0.148623853,-0.146788991,-0.144954128,-0.143119266,-0.141284404,
-0.139449541,-0.137614679,-0.135779817,-0.133944954,-0.132110092,-0.130275229,
-0.128440367,-0.126605505,-0.124770642,-0.12293578,-0.121100917,-0.119266055,
-0.117431193,-0.11559633,-0.113761468,-0.111926606,-0.110091743,-0.108256881,
-0.106422018,-0.104587156,-0.102752294,-0.100917431,-0.099082569,-0.097247706,
-0.095412844,-0.093577982,-0.091743119,-0.089908257,-0.088073394,-0.086238532,
-0.08440367,-0.082568807,-0.080733945,-0.078899083,-0.07706422,-0.075229358,
-0.073394495,-0.071559633,-0.069724771,-0.067889908,-0.066055046,-0.064220183,
-0.062385321,-0.060550459,-0.058715596,-0.056880734,-0.055045872,-0.053211009,
-0.051376147,-0.049541284,-0.047706422,-0.04587156,-0.044036697,-0.042201835,
-0.040366972,-0.03853211,-0.036697248,-0.034862385,-0.033027523,-0.031192661,
-0.029357798,-0.027522936,-0.025688073,-0.023853211,-0.022018349,-0.020183486,
-0.018348624,-0.016513761,-0.014678899,-0.012844037,-0.011009174,-0.009174312,
-0.00733945,-0.005504587,-0.003669725,-0.001834862,0.000982074616),(0.3,
1.,1.3),.UNSPECIFIED.);
#6336=B_SPLINE_SURFACE_WITH_KNOTS('',5,1,((#356501,#356502,#356503),(#356504,
#356505,#356506),(#356507,#356508,#356509),(#356510,#356511,#356512),(#356513,
#356514,#356515),(#356516,#356517,#356518),(#356519,#356520,#356521),(#356522,
#356523,#356524),(#356525,#356526,#356527),(#356528,#356529,#356530),(#356531,
#356532,#356533),(#356534,#356535,#356536),(#356537,#356538,#356539),(#356540,
#356541,#356542),(#356543,#356544,#356545),(#356546,#356547,#356548),(#356549,
#356550,#356551),(#356552,#356553,#356554),(#356555,#356556,#356557),(#356558,
#356559,#356560),(#356561,#356562,#356563),(#356564,#356565,#356566),(#356567,
#356568,#356569),(#356570,#356571,#356572),(#356573,#356574,#356575),(#356576,
#356577,#356578),(#356579,#356580,#356581),(#356582,#356583,#356584),(#356585,
#356586,#356587),(#356588,#356589,#356590),(#356591,#356592,#356593),(#356594,
#356595,#356596),(#356597,#356598,#356599),(#356600,#356601,#356602),(#356603,
#356604,#356605),(#356606,#356607,#356608),(#356609,#356610,#356611),(#356612,
#356613,#356614),(#356615,#356616,#356617),(#356618,#356619,#356620),(#356621,
#356622,#356623),(#356624,#356625,#356626),(#356627,#356628,#356629),(#356630,
#356631,#356632),(#356633,#356634,#356635),(#356636,#356637,#356638),(#356639,
#356640,#356641),(#356642,#356643,#356644),(#356645,#356646,#356647),(#356648,
#356649,#356650),(#356651,#356652,#356653),(#356654,#356655,#356656),(#356657,
#356658,#356659),(#356660,#356661,#356662),(#356663,#356664,#356665),(#356666,
#356667,#356668),(#356669,#356670,#356671),(#356672,#356673,#356674),(#356675,
#356676,#356677),(#356678,#356679,#356680),(#356681,#356682,#356683),(#356684,
#356685,#356686),(#356687,#356688,#356689),(#356690,#356691,#356692),(#356693,
#356694,#356695),(#356696,#356697,#356698),(#356699,#356700,#356701),(#356702,
#356703,#356704),(#356705,#356706,#356707),(#356708,#356709,#356710),(#356711,
#356712,#356713),(#356714,#356715,#356716),(#356717,#356718,#356719),(#356720,
#356721,#356722),(#356723,#356724,#356725),(#356726,#356727,#356728),(#356729,
#356730,#356731),(#356732,#356733,#356734),(#356735,#356736,#356737),(#356738,
#356739,#356740),(#356741,#356742,#356743),(#356744,#356745,#356746),(#356747,
#356748,#356749),(#356750,#356751,#356752),(#356753,#356754,#356755),(#356756,
#356757,#356758),(#356759,#356760,#356761),(#356762,#356763,#356764),(#356765,
#356766,#356767),(#356768,#356769,#356770),(#356771,#356772,#356773),(#356774,
#356775,#356776),(#356777,#356778,#356779),(#356780,#356781,#356782),(#356783,
#356784,#356785),(#356786,#356787,#356788),(#356789,#356790,#356791),(#356792,
#356793,#356794),(#356795,#356796,#356797),(#356798,#356799,#356800),(#356801,
#356802,#356803),(#356804,#356805,#356806),(#356807,#356808,#356809),(#356810,
#356811,#356812),(#356813,#356814,#356815),(#356816,#356817,#356818),(#356819,
#356820,#356821),(#356822,#356823,#356824),(#356825,#356826,#356827),(#356828,
#356829,#356830),(#356831,#356832,#356833),(#356834,#356835,#356836),(#356837,
#356838,#356839),(#356840,#356841,#356842),(#356843,#356844,#356845),(#356846,
#356847,#356848),(#356849,#356850,#356851),(#356852,#356853,#356854),(#356855,
#356856,#356857),(#356858,#356859,#356860),(#356861,#356862,#356863),(#356864,
#356865,#356866),(#356867,#356868,#356869),(#356870,#356871,#356872),(#356873,
#356874,#356875),(#356876,#356877,#356878),(#356879,#356880,#356881),(#356882,
#356883,#356884),(#356885,#356886,#356887),(#356888,#356889,#356890),(#356891,
#356892,#356893),(#356894,#356895,#356896),(#356897,#356898,#356899),(#356900,
#356901,#356902),(#356903,#356904,#356905),(#356906,#356907,#356908),(#356909,
#356910,#356911),(#356912,#356913,#356914),(#356915,#356916,#356917),(#356918,
#356919,#356920),(#356921,#356922,#356923),(#356924,#356925,#356926),(#356927,
#356928,#356929),(#356930,#356931,#356932),(#356933,#356934,#356935),(#356936,
#356937,#356938),(#356939,#356940,#356941),(#356942,#356943,#356944),(#356945,
#356946,#356947),(#356948,#356949,#356950),(#356951,#356952,#356953),(#356954,
#356955,#356956),(#356957,#356958,#356959),(#356960,#356961,#356962),(#356963,
#356964,#356965),(#356966,#356967,#356968),(#356969,#356970,#356971),(#356972,
#356973,#356974),(#356975,#356976,#356977),(#356978,#356979,#356980),(#356981,
#356982,#356983),(#356984,#356985,#356986),(#356987,#356988,#356989),(#356990,
#356991,#356992),(#356993,#356994,#356995),(#356996,#356997,#356998),(#356999,
#357000,#357001),(#357002,#357003,#357004),(#357005,#357006,#357007),(#357008,
#357009,#357010),(#357011,#357012,#357013),(#357014,#357015,#357016),(#357017,
#357018,#357019),(#357020,#357021,#357022),(#357023,#357024,#357025),(#357026,
#357027,#357028),(#357029,#357030,#357031),(#357032,#357033,#357034),(#357035,
#357036,#357037),(#357038,#357039,#357040),(#357041,#357042,#357043),(#357044,
#357045,#357046),(#357047,#357048,#357049),(#357050,#357051,#357052),(#357053,
#357054,#357055),(#357056,#357057,#357058),(#357059,#357060,#357061),(#357062,
#357063,#357064),(#357065,#357066,#357067),(#357068,#357069,#357070),(#357071,
#357072,#357073),(#357074,#357075,#357076),(#357077,#357078,#357079),(#357080,
#357081,#357082),(#357083,#357084,#357085),(#357086,#357087,#357088),(#357089,
#357090,#357091),(#357092,#357093,#357094),(#357095,#357096,#357097),(#357098,
#357099,#357100),(#357101,#357102,#357103),(#357104,#357105,#357106),(#357107,
#357108,#357109),(#357110,#357111,#357112),(#357113,#357114,#357115),(#357116,
#357117,#357118),(#357119,#357120,#357121),(#357122,#357123,#357124),(#357125,
#357126,#357127),(#357128,#357129,#357130),(#357131,#357132,#357133),(#357134,
#357135,#357136),(#357137,#357138,#357139),(#357140,#357141,#357142),(#357143,
#357144,#357145),(#357146,#357147,#357148),(#357149,#357150,#357151),(#357152,
#357153,#357154),(#357155,#357156,#357157),(#357158,#357159,#357160),(#357161,
#357162,#357163),(#357164,#357165,#357166),(#357167,#357168,#357169),(#357170,
#357171,#357172),(#357173,#357174,#357175),(#357176,#357177,#357178),(#357179,
#357180,#357181),(#357182,#357183,#357184),(#357185,#357186,#357187),(#357188,
#357189,#357190),(#357191,#357192,#357193),(#357194,#357195,#357196),(#357197,
#357198,#357199),(#357200,#357201,#357202),(#357203,#357204,#357205),(#357206,
#357207,#357208),(#357209,#357210,#357211),(#357212,#357213,#357214),(#357215,
#357216,#357217),(#357218,#357219,#357220),(#357221,#357222,#357223),(#357224,
#357225,#357226),(#357227,#357228,#357229),(#357230,#357231,#357232),(#357233,
#357234,#357235),(#357236,#357237,#357238),(#357239,#357240,#357241),(#357242,
#357243,#357244),(#357245,#357246,#357247),(#357248,#357249,#357250),(#357251,
#357252,#357253),(#357254,#357255,#357256),(#357257,#357258,#357259),(#357260,
#357261,#357262),(#357263,#357264,#357265),(#357266,#357267,#357268),(#357269,
#357270,#357271),(#357272,#357273,#357274),(#357275,#357276,#357277),(#357278,
#357279,#357280),(#357281,#357282,#357283),(#357284,#357285,#357286),(#357287,
#357288,#357289),(#357290,#357291,#357292),(#357293,#357294,#357295),(#357296,
#357297,#357298),(#357299,#357300,#357301),(#357302,#357303,#357304),(#357305,
#357306,#357307),(#357308,#357309,#357310),(#357311,#357312,#357313),(#357314,
#357315,#357316),(#357317,#357318,#357319),(#357320,#357321,#357322),(#357323,
#357324,#357325),(#357326,#357327,#357328),(#357329,#357330,#357331),(#357332,
#357333,#357334),(#357335,#357336,#357337),(#357338,#357339,#357340),(#357341,
#357342,#357343),(#357344,#357345,#357346),(#357347,#357348,#357349),(#357350,
#357351,#357352),(#357353,#357354,#357355),(#357356,#357357,#357358),(#357359,
#357360,#357361),(#357362,#357363,#357364),(#357365,#357366,#357367),(#357368,
#357369,#357370),(#357371,#357372,#357373),(#357374,#357375,#357376),(#357377,
#357378,#357379),(#357380,#357381,#357382),(#357383,#357384,#357385),(#357386,
#357387,#357388),(#357389,#357390,#357391),(#357392,#357393,#357394),(#357395,
#357396,#357397),(#357398,#357399,#357400),(#357401,#357402,#357403),(#357404,
#357405,#357406),(#357407,#357408,#357409),(#357410,#357411,#357412),(#357413,
#357414,#357415),(#357416,#357417,#357418),(#357419,#357420,#357421),(#357422,
#357423,#357424),(#357425,#357426,#357427),(#357428,#357429,#357430),(#357431,
#357432,#357433),(#357434,#357435,#357436),(#357437,#357438,#357439),(#357440,
#357441,#357442),(#357443,#357444,#357445),(#357446,#357447,#357448),(#357449,
#357450,#357451),(#357452,#357453,#357454),(#357455,#357456,#357457),(#357458,
#357459,#357460),(#357461,#357462,#357463),(#357464,#357465,#357466),(#357467,
#357468,#357469),(#357470,#357471,#357472),(#357473,#357474,#357475),(#357476,
#357477,#357478),(#357479,#357480,#357481),(#357482,#357483,#357484),(#357485,
#357486,#357487),(#357488,#357489,#357490),(#357491,#357492,#357493),(#357494,
#357495,#357496),(#357497,#357498,#357499),(#357500,#357501,#357502),(#357503,
#357504,#357505),(#357506,#357507,#357508),(#357509,#357510,#357511),(#357512,
#357513,#357514),(#357515,#357516,#357517),(#357518,#357519,#357520),(#357521,
#357522,#357523),(#357524,#357525,#357526),(#357527,#357528,#357529),(#357530,
#357531,#357532),(#357533,#357534,#357535),(#357536,#357537,#357538),(#357539,
#357540,#357541),(#357542,#357543,#357544),(#357545,#357546,#357547),(#357548,
#357549,#357550),(#357551,#357552,#357553),(#357554,#357555,#357556),(#357557,
#357558,#357559),(#357560,#357561,#357562),(#357563,#357564,#357565),(#357566,
#357567,#357568),(#357569,#357570,#357571),(#357572,#357573,#357574),(#357575,
#357576,#357577),(#357578,#357579,#357580),(#357581,#357582,#357583),(#357584,
#357585,#357586),(#357587,#357588,#357589),(#357590,#357591,#357592),(#357593,
#357594,#357595),(#357596,#357597,#357598),(#357599,#357600,#357601),(#357602,
#357603,#357604),(#357605,#357606,#357607),(#357608,#357609,#357610),(#357611,
#357612,#357613),(#357614,#357615,#357616),(#357617,#357618,#357619),(#357620,
#357621,#357622),(#357623,#357624,#357625),(#357626,#357627,#357628),(#357629,
#357630,#357631),(#357632,#357633,#357634),(#357635,#357636,#357637),(#357638,
#357639,#357640),(#357641,#357642,#357643),(#357644,#357645,#357646),(#357647,
#357648,#357649),(#357650,#357651,#357652),(#357653,#357654,#357655),(#357656,
#357657,#357658),(#357659,#357660,#357661),(#357662,#357663,#357664),(#357665,
#357666,#357667),(#357668,#357669,#357670),(#357671,#357672,#357673),(#357674,
#357675,#357676),(#357677,#357678,#357679),(#357680,#357681,#357682),(#357683,
#357684,#357685),(#357686,#357687,#357688),(#357689,#357690,#357691),(#357692,
#357693,#357694),(#357695,#357696,#357697),(#357698,#357699,#357700),(#357701,
#357702,#357703),(#357704,#357705,#357706),(#357707,#357708,#357709),(#357710,
#357711,#357712),(#357713,#357714,#357715),(#357716,#357717,#357718),(#357719,
#357720,#357721),(#357722,#357723,#357724),(#357725,#357726,#357727),(#357728,
#357729,#357730),(#357731,#357732,#357733),(#357734,#357735,#357736),(#357737,
#357738,#357739),(#357740,#357741,#357742),(#357743,#357744,#357745),(#357746,
#357747,#357748),(#357749,#357750,#357751),(#357752,#357753,#357754),(#357755,
#357756,#357757),(#357758,#357759,#357760),(#357761,#357762,#357763),(#357764,
#357765,#357766),(#357767,#357768,#357769),(#357770,#357771,#357772),(#357773,
#357774,#357775),(#357776,#357777,#357778),(#357779,#357780,#357781),(#357782,
#357783,#357784),(#357785,#357786,#357787),(#357788,#357789,#357790),(#357791,
#357792,#357793),(#357794,#357795,#357796),(#357797,#357798,#357799),(#357800,
#357801,#357802),(#357803,#357804,#357805),(#357806,#357807,#357808),(#357809,
#357810,#357811),(#357812,#357813,#357814),(#357815,#357816,#357817),(#357818,
#357819,#357820),(#357821,#357822,#357823),(#357824,#357825,#357826),(#357827,
#357828,#357829),(#357830,#357831,#357832),(#357833,#357834,#357835),(#357836,
#357837,#357838),(#357839,#357840,#357841),(#357842,#357843,#357844),(#357845,
#357846,#357847),(#357848,#357849,#357850),(#357851,#357852,#357853),(#357854,
#357855,#357856),(#357857,#357858,#357859),(#357860,#357861,#357862),(#357863,
#357864,#357865),(#357866,#357867,#357868),(#357869,#357870,#357871),(#357872,
#357873,#357874),(#357875,#357876,#357877),(#357878,#357879,#357880),(#357881,
#357882,#357883),(#357884,#357885,#357886),(#357887,#357888,#357889),(#357890,
#357891,#357892),(#357893,#357894,#357895),(#357896,#357897,#357898),(#357899,
#357900,#357901),(#357902,#357903,#357904),(#357905,#357906,#357907),(#357908,
#357909,#357910),(#357911,#357912,#357913),(#357914,#357915,#357916),(#357917,
#357918,#357919),(#357920,#357921,#357922),(#357923,#357924,#357925),(#357926,
#357927,#357928),(#357929,#357930,#357931),(#357932,#357933,#357934),(#357935,
#357936,#357937),(#357938,#357939,#357940),(#357941,#357942,#357943),(#357944,
#357945,#357946),(#357947,#357948,#357949),(#357950,#357951,#357952),(#357953,
#357954,#357955),(#357956,#357957,#357958),(#357959,#357960,#357961),(#357962,
#357963,#357964),(#357965,#357966,#357967),(#357968,#357969,#357970),(#357971,
#357972,#357973),(#357974,#357975,#357976),(#357977,#357978,#357979),(#357980,
#357981,#357982),(#357983,#357984,#357985),(#357986,#357987,#357988),(#357989,
#357990,#357991),(#357992,#357993,#357994),(#357995,#357996,#357997),(#357998,
#357999,#358000),(#358001,#358002,#358003),(#358004,#358005,#358006),(#358007,
#358008,#358009),(#358010,#358011,#358012),(#358013,#358014,#358015),(#358016,
#358017,#358018),(#358019,#358020,#358021),(#358022,#358023,#358024),(#358025,
#358026,#358027),(#358028,#358029,#358030),(#358031,#358032,#358033),(#358034,
#358035,#358036),(#358037,#358038,#358039),(#358040,#358041,#358042),(#358043,
#358044,#358045),(#358046,#358047,#358048),(#358049,#358050,#358051),(#358052,
#358053,#358054),(#358055,#358056,#358057),(#358058,#358059,#358060),(#358061,
#358062,#358063),(#358064,#358065,#358066),(#358067,#358068,#358069),(#358070,
#358071,#358072),(#358073,#358074,#358075),(#358076,#358077,#358078),(#358079,
#358080,#358081),(#358082,#358083,#358084),(#358085,#358086,#358087),(#358088,
#358089,#358090),(#358091,#358092,#358093),(#358094,#358095,#358096),(#358097,
#358098,#358099),(#358100,#358101,#358102),(#358103,#358104,#358105),(#358106,
#358107,#358108),(#358109,#358110,#358111),(#358112,#358113,#358114),(#358115,
#358116,#358117),(#358118,#358119,#358120),(#358121,#358122,#358123),(#358124,
#358125,#358126),(#358127,#358128,#358129),(#358130,#358131,#358132),(#358133,
#358134,#358135),(#358136,#358137,#358138),(#358139,#358140,#358141),(#358142,
#358143,#358144),(#358145,#358146,#358147),(#358148,#358149,#358150),(#358151,
#358152,#358153)),.UNSPECIFIED.,.F.,.F.,.F.,(6,1,1,1,1,1,1,1,1,1,1,1,1,
1,1,1,1,1,1,1,1,1,1,1,1,1,1,1,1,1,1,1,1,1,1,1,1,1,1,1,1,1,1,1,1,1,1,1,1,
1,1,1,1,1,1,1,1,1,1,1,1,1,1,1,1,1,1,1,1,1,1,1,1,1,1,1,1,1,1,1,1,1,1,1,1,
1,1,1,1,1,1,1,1,1,1,1,1,1,1,1,1,1,1,1,1,1,1,1,1,1,1,1,1,1,1,1,1,1,1,1,1,
1,1,1,1,1,1,1,1,1,1,1,1,1,1,1,1,1,1,1,1,1,1,1,1,1,1,1,1,1,1,1,1,1,1,1,1,
1,1,1,1,1,1,1,1,1,1,1,1,1,1,1,1,1,1,1,1,1,1,1,1,1,1,1,1,1,1,1,1,1,1,1,1,
1,1,1,1,1,1,1,1,1,1,1,1,1,1,1,1,1,1,1,1,1,1,1,1,1,1,1,1,1,1,1,1,1,1,1,1,
1,1,1,1,1,1,1,1,1,1,1,1,1,1,1,1,1,1,1,1,1,1,1,1,1,1,1,1,1,1,1,1,1,1,1,1,
1,1,1,1,1,1,1,1,1,1,1,1,1,1,1,1,1,1,1,1,1,1,1,1,1,1,1,1,1,1,1,1,1,1,1,1,
1,1,1,1,1,1,1,1,1,1,1,1,1,1,1,1,1,1,1,1,1,1,1,1,1,1,1,1,1,1,1,1,1,1,1,1,
1,1,1,1,1,1,1,1,1,1,1,1,1,1,1,1,1,1,1,1,1,1,1,1,1,1,1,1,1,1,1,1,1,1,1,1,
1,1,1,1,1,1,1,1,1,1,1,1,1,1,1,1,1,1,1,1,1,1,1,1,1,1,1,1,1,1,1,1,1,1,1,1,
1,1,1,1,1,1,1,1,1,1,1,1,1,1,1,1,1,1,1,1,1,1,1,1,1,1,1,1,1,1,1,1,1,1,1,1,
1,1,1,1,1,1,1,1,1,1,1,1,1,1,1,1,1,1,1,1,1,1,1,1,1,1,1,1,1,1,1,1,1,1,1,1,
1,1,1,1,1,1,1,1,1,1,1,1,1,1,1,1,1,1,1,1,1,1,1,1,1,1,1,1,1,1,1,1,1,1,1,1,
1,1,1,1,1,1,1,1,1,1,1,1,1,1,1,1,1,1,1,1,1,1,1,1,1,1,1,1,1,6),(2,1,2),(-0.001964179,
0.,0.001834862,0.003669725,0.005504587,0.00733945,0.009174312,0.011009174,
0.012844037,0.014678899,0.016513761,0.018348624,0.020183486,0.022018349,
0.023853211,0.025688073,0.027522936,0.029357798,0.031192661,0.033027523,
0.034862385,0.036697248,0.03853211,0.040366972,0.042201835,0.044036697,
0.04587156,0.047706422,0.049541284,0.051376147,0.053211009,0.055045872,
0.056880734,0.058715596,0.060550459,0.062385321,0.064220183,0.066055046,
0.067889908,0.069724771,0.071559633,0.073394495,0.075229358,0.07706422,
0.078899083,0.080733945,0.082568807,0.08440367,0.086238532,0.088073394,
0.089908257,0.091743119,0.093577982,0.095412844,0.097247706,0.099082569,
0.100917431,0.102752294,0.104587156,0.106422018,0.108256881,0.110091743,
0.111926606,0.113761468,0.11559633,0.117431193,0.119266055,0.121100917,
0.12293578,0.124770642,0.126605505,0.128440367,0.130275229,0.132110092,
0.133944954,0.135779817,0.137614679,0.139449541,0.141284404,0.143119266,
0.144954128,0.146788991,0.148623853,0.150458716,0.152293578,0.15412844,
0.155963303,0.157798165,0.159633028,0.16146789,0.163302752,0.165137615,
0.166972477,0.168807339,0.170642202,0.172477064,0.174311927,0.176146789,
0.177981651,0.179816514,0.181651376,0.183486239,0.185321101,0.187155963,
0.188990826,0.190825688,0.19266055,0.194495413,0.196330275,0.198165138,
0.2,0.201834862,0.203669725,0.205504587,0.20733945,0.209174312,0.211009174,
0.212844037,0.214678899,0.216513761,0.218348624,0.220183486,0.222018349,
0.223853211,0.225688073,0.227522936,0.229357798,0.231192661,0.233027523,
0.234862385,0.236697248,0.23853211,0.240366972,0.242201835,0.244036697,
0.24587156,0.247706422,0.249541284,0.251376147,0.253211009,0.255045872,
0.256880734,0.258715596,0.260550459,0.262385321,0.264220183,0.266055046,
0.267889908,0.269724771,0.271559633,0.273394495,0.275229358,0.27706422,
0.278899083,0.280733945,0.282568807,0.28440367,0.286238532,0.288073394,
0.289908257,0.291743119,0.293577982,0.295412844,0.297247706,0.299082569,
0.300917431,0.302752294,0.304587156,0.306422018,0.308256881,0.310091743,
0.311926606,0.313761468,0.31559633,0.317431193,0.319266055,0.321100917,
0.32293578,0.324770642,0.326605505,0.328440367,0.330275229,0.332110092,
0.333944954,0.335779817,0.337614679,0.339449541,0.341284404,0.343119266,
0.344954128,0.346788991,0.348623853,0.350458716,0.352293578,0.35412844,
0.355963303,0.357798165,0.359633028,0.36146789,0.363302752,0.365137615,
0.366972477,0.368807339,0.370642202,0.372477064,0.374311927,0.376146789,
0.377981651,0.379816514,0.381651376,0.383486239,0.385321101,0.387155963,
0.388990826,0.390825688,0.39266055,0.394495413,0.396330275,0.398165138,
0.4,0.401834862,0.403669725,0.405504587,0.40733945,0.409174312,0.411009174,
0.412844037,0.414678899,0.416513761,0.418348624,0.420183486,0.422018349,
0.423853211,0.425688073,0.427522936,0.429357798,0.431192661,0.433027523,
0.434862385,0.436697248,0.43853211,0.440366972,0.442201835,0.444036697,
0.44587156,0.447706422,0.449541284,0.451376147,0.453211009,0.455045872,
0.456880734,0.458715596,0.460550459,0.462385321,0.464220183,0.466055046,
0.467889908,0.469724771,0.471559633,0.473394495,0.475229358,0.47706422,
0.478899083,0.480733945,0.482568807,0.48440367,0.486238532,0.488073394,
0.489908257,0.491743119,0.493577982,0.495412844,0.497247706,0.499082569,
0.500917431,0.502752294,0.504587156,0.506422018,0.508256881,0.510091743,
0.511926606,0.513761468,0.51559633,0.517431193,0.519266055,0.521100917,
0.52293578,0.524770642,0.526605505,0.528440367,0.530275229,0.532110092,
0.533944954,0.535779817,0.537614679,0.539449541,0.541284404,0.543119266,
0.544954128,0.546788991,0.548623853,0.550458716,0.552293578,0.55412844,
0.555963303,0.557798165,0.559633028,0.56146789,0.563302752,0.565137615,
0.566972477,0.568807339,0.570642202,0.572477064,0.574311927,0.576146789,
0.577981651,0.579816514,0.581651376,0.583486239,0.585321101,0.587155963,
0.588990826,0.590825688,0.59266055,0.594495413,0.596330275,0.598165138,
0.6,0.601834862,0.603669725,0.605504587,0.60733945,0.609174312,0.611009174,
0.612844037,0.614678899,0.616513761,0.618348624,0.620183486,0.622018349,
0.623853211,0.625688073,0.627522936,0.629357798,0.631192661,0.633027523,
0.634862385,0.636697248,0.63853211,0.640366972,0.642201835,0.644036697,
0.64587156,0.647706422,0.649541284,0.651376147,0.653211009,0.655045872,
0.656880734,0.658715596,0.660550459,0.662385321,0.664220183,0.666055046,
0.667889908,0.669724771,0.671559633,0.673394495,0.675229358,0.67706422,
0.678899083,0.680733945,0.682568807,0.68440367,0.686238532,0.688073394,
0.689908257,0.691743119,0.693577982,0.695412844,0.697247706,0.699082569,
0.700917431,0.702752294,0.704587156,0.706422018,0.708256881,0.710091743,
0.711926606,0.713761468,0.71559633,0.717431193,0.719266055,0.721100917,
0.72293578,0.724770642,0.726605505,0.728440367,0.730275229,0.732110092,
0.733944954,0.735779817,0.737614679,0.739449541,0.741284404,0.743119266,
0.744954128,0.746788991,0.748623853,0.750458716,0.752293578,0.75412844,
0.755963303,0.757798165,0.759633028,0.76146789,0.763302752,0.765137615,
0.766972477,0.768807339,0.770642202,0.772477064,0.774311927,0.776146789,
0.777981651,0.779816514,0.781651376,0.783486239,0.785321101,0.787155963,
0.788990826,0.790825688,0.79266055,0.794495413,0.796330275,0.798165138,
0.8,0.801834862,0.803669725,0.805504587,0.80733945,0.809174312,0.811009174,
0.812844037,0.814678899,0.816513761,0.818348624,0.820183486,0.822018349,
0.823853211,0.825688073,0.827522936,0.829357798,0.831192661,0.833027523,
0.834862385,0.836697248,0.83853211,0.840366972,0.842201835,0.844036697,
0.84587156,0.847706422,0.849541284,0.851376147,0.853211009,0.855045872,
0.856880734,0.858715596,0.860550459,0.862385321,0.864220183,0.866055046,
0.867889908,0.869724771,0.871559633,0.873394495,0.875229358,0.87706422,
0.878899083,0.880733945,0.882568807,0.88440367,0.886238532,0.888073394,
0.889908257,0.891743119,0.893577982,0.895412844,0.897247706,0.899082569,
0.900917431,0.902752294,0.904587156,0.906422018,0.908256881,0.910091743,
0.911926606,0.913761468,0.91559633,0.917431193,0.919266055,0.921100917,
0.92293578,0.924770642,0.926605505,0.928440367,0.930275229,0.932110092,
0.933944954,0.935779817,0.937614679,0.939449541,0.941284404,0.943119266,
0.944954128,0.946788991,0.948623853,0.950458716,0.952293578,0.95412844,
0.955963303,0.957798165,0.959633028,0.96146789,0.963302752,0.965137615,
0.966972477,0.968807339,0.970642202,0.972477064,0.974311927,0.976146789,
0.977981651,0.979816514,0.981651376,0.983486239,0.985321101,0.987155963,
0.988990826,0.990825688,0.99266055,0.994495413,0.996330275,0.998165138,
1.),(0.3,1.,1.3),.UNSPECIFIED.);
#7942=FACE_OUTER_BOUND('',#13824,.T.);
#7943=FACE_OUTER_BOUND('',#13825,.T.);
#7944=FACE_OUTER_BOUND('',#13826,.T.);
#7945=FACE_OUTER_BOUND('',#13827,.T.);
#7946=FACE_OUTER_BOUND('',#13828,.T.);
#7947=FACE_OUTER_BOUND('',#13829,.T.);
#7948=FACE_OUTER_BOUND('',#13830,.T.);
#7949=FACE_OUTER_BOUND('',#13831,.T.);
#7950=FACE_OUTER_BOUND('',#13832,.T.);
#7951=FACE_OUTER_BOUND('',#13833,.T.);
#7952=FACE_OUTER_BOUND('',#13834,.T.);
#7953=FACE_OUTER_BOUND('',#13835,.T.);
#7954=FACE_OUTER_BOUND('',#13836,.T.);
#7955=FACE_OUTER_BOUND('',#13837,.T.);
#7956=FACE_OUTER_BOUND('',#13838,.T.);
#7957=FACE_OUTER_BOUND('',#13839,.T.);
#7958=FACE_OUTER_BOUND('',#13840,.T.);
#7959=FACE_OUTER_BOUND('',#13841,.T.);
#7960=FACE_OUTER_BOUND('',#13842,.T.);
#7961=FACE_OUTER_BOUND('',#13843,.T.);
#7962=FACE_OUTER_BOUND('',#13844,.T.);
#7963=FACE_OUTER_BOUND('',#13845,.T.);
#7964=FACE_OUTER_BOUND('',#13846,.T.);
#7965=FACE_OUTER_BOUND('',#13847,.T.);
#7966=FACE_OUTER_BOUND('',#13848,.T.);
#7967=FACE_OUTER_BOUND('',#13849,.T.);
#7968=FACE_OUTER_BOUND('',#13850,.T.);
#7969=FACE_OUTER_BOUND('',#13851,.T.);
#7970=FACE_OUTER_BOUND('',#13852,.T.);
#7971=FACE_OUTER_BOUND('',#13853,.T.);
#7972=FACE_OUTER_BOUND('',#13854,.T.);
#7973=FACE_OUTER_BOUND('',#13855,.T.);
#7974=FACE_OUTER_BOUND('',#13856,.T.);
#7975=FACE_OUTER_BOUND('',#13857,.T.);
#7976=FACE_OUTER_BOUND('',#13858,.T.);
#7977=FACE_OUTER_BOUND('',#13859,.T.);
#7978=FACE_OUTER_BOUND('',#13860,.T.);
#7979=FACE_OUTER_BOUND('',#13861,.T.);
#7980=FACE_OUTER_BOUND('',#13862,.T.);
#7981=FACE_OUTER_BOUND('',#13863,.T.);
#7982=FACE_OUTER_BOUND('',#13864,.T.);
#7983=FACE_OUTER_BOUND('',#13865,.T.);
#7984=FACE_OUTER_BOUND('',#13866,.T.);
#7985=FACE_OUTER_BOUND('',#13867,.T.);
#7986=FACE_OUTER_BOUND('',#13868,.T.);
#7987=FACE_OUTER_BOUND('',#13869,.T.);
#7988=FACE_OUTER_BOUND('',#13870,.T.);
#7989=FACE_OUTER_BOUND('',#13871,.T.);
#7990=FACE_OUTER_BOUND('',#13872,.T.);
#7991=FACE_OUTER_BOUND('',#13873,.T.);
#7992=FACE_OUTER_BOUND('',#13874,.T.);
#7993=FACE_OUTER_BOUND('',#13875,.T.);
#7994=FACE_OUTER_BOUND('',#13876,.T.);
#7995=FACE_OUTER_BOUND('',#13877,.T.);
#7996=FACE_OUTER_BOUND('',#13878,.T.);
#7997=FACE_OUTER_BOUND('',#13879,.T.);
#7998=FACE_OUTER_BOUND('',#13880,.T.);
#7999=FACE_OUTER_BOUND('',#13881,.T.);
#8000=FACE_OUTER_BOUND('',#13882,.T.);
#8001=FACE_OUTER_BOUND('',#13883,.T.);
#8002=FACE_OUTER_BOUND('',#13884,.T.);
#8003=FACE_OUTER_BOUND('',#13885,.T.);
#8004=FACE_OUTER_BOUND('',#13886,.T.);
#8005=FACE_OUTER_BOUND('',#13887,.T.);
#8006=FACE_OUTER_BOUND('',#13888,.T.);
#8007=FACE_OUTER_BOUND('',#13889,.T.);
#8008=FACE_OUTER_BOUND('',#13890,.T.);
#8009=FACE_OUTER_BOUND('',#13891,.T.);
#8010=FACE_OUTER_BOUND('',#13892,.T.);
#8011=FACE_OUTER_BOUND('',#13893,.T.);
#8012=FACE_OUTER_BOUND('',#13894,.T.);
#8013=FACE_OUTER_BOUND('',#13895,.T.);
#8014=FACE_OUTER_BOUND('',#13896,.T.);
#8015=FACE_OUTER_BOUND('',#13897,.T.);
#8016=FACE_OUTER_BOUND('',#13898,.T.);
#8017=FACE_OUTER_BOUND('',#13899,.T.);
#8018=FACE_OUTER_BOUND('',#13900,.T.);
#8019=FACE_OUTER_BOUND('',#13901,.T.);
#8020=FACE_OUTER_BOUND('',#13902,.T.);
#8021=FACE_OUTER_BOUND('',#13903,.T.);
#8022=FACE_OUTER_BOUND('',#13904,.T.);
#8023=FACE_OUTER_BOUND('',#13905,.T.);
#8024=FACE_OUTER_BOUND('',#13906,.T.);
#8025=FACE_OUTER_BOUND('',#13907,.T.);
#8026=FACE_OUTER_BOUND('',#13908,.T.);
#8027=FACE_OUTER_BOUND('',#13909,.T.);
#8028=FACE_OUTER_BOUND('',#13910,.T.);
#8029=FACE_OUTER_BOUND('',#13911,.T.);
#8030=FACE_OUTER_BOUND('',#13912,.T.);
#8031=FACE_OUTER_BOUND('',#13913,.T.);
#8032=FACE_OUTER_BOUND('',#13914,.T.);
#8033=FACE_OUTER_BOUND('',#13915,.T.);
#8034=FACE_OUTER_BOUND('',#13916,.T.);
#8035=FACE_OUTER_BOUND('',#13917,.T.);
#8036=FACE_OUTER_BOUND('',#13918,.T.);
#8037=FACE_OUTER_BOUND('',#13919,.T.);
#8038=FACE_OUTER_BOUND('',#13920,.T.);
#8039=FACE_OUTER_BOUND('',#13921,.T.);
#8040=FACE_OUTER_BOUND('',#13922,.T.);
#8041=FACE_OUTER_BOUND('',#13923,.T.);
#8042=FACE_OUTER_BOUND('',#13924,.T.);
#8043=FACE_OUTER_BOUND('',#13925,.T.);
#8044=FACE_OUTER_BOUND('',#13926,.T.);
#8045=FACE_OUTER_BOUND('',#13927,.T.);
#8046=FACE_OUTER_BOUND('',#13928,.T.);
#8047=FACE_OUTER_BOUND('',#13929,.T.);
#8048=FACE_OUTER_BOUND('',#13930,.T.);
#8049=FACE_OUTER_BOUND('',#13931,.T.);
#8050=FACE_OUTER_BOUND('',#13932,.T.);
#8051=FACE_OUTER_BOUND('',#13933,.T.);
#8052=FACE_OUTER_BOUND('',#13934,.T.);
#8053=FACE_OUTER_BOUND('',#13935,.T.);
#8054=FACE_OUTER_BOUND('',#13936,.T.);
#8055=FACE_OUTER_BOUND('',#13937,.T.);
#8056=FACE_OUTER_BOUND('',#13938,.T.);
#8057=FACE_OUTER_BOUND('',#13939,.T.);
#8058=FACE_OUTER_BOUND('',#13940,.T.);
#8059=FACE_OUTER_BOUND('',#13941,.T.);
#8060=FACE_OUTER_BOUND('',#13942,.T.);
#8061=FACE_OUTER_BOUND('',#13943,.T.);
#8062=FACE_OUTER_BOUND('',#13944,.T.);
#8063=FACE_OUTER_BOUND('',#13945,.T.);
#8064=FACE_OUTER_BOUND('',#13946,.T.);
#8065=FACE_OUTER_BOUND('',#13947,.T.);
#8066=FACE_OUTER_BOUND('',#13948,.T.);
#8067=FACE_OUTER_BOUND('',#13949,.T.);
#8068=FACE_OUTER_BOUND('',#13950,.T.);
#8069=FACE_OUTER_BOUND('',#13951,.T.);
#8070=FACE_OUTER_BOUND('',#13952,.T.);
#8071=FACE_OUTER_BOUND('',#13953,.T.);
#8072=FACE_OUTER_BOUND('',#13954,.T.);
#8073=FACE_OUTER_BOUND('',#13955,.T.);
#8074=FACE_OUTER_BOUND('',#13956,.T.);
#8075=FACE_OUTER_BOUND('',#13957,.T.);
#8076=FACE_OUTER_BOUND('',#13958,.T.);
#8077=FACE_OUTER_BOUND('',#13959,.T.);
#8078=FACE_OUTER_BOUND('',#13960,.T.);
#8079=FACE_OUTER_BOUND('',#13961,.T.);
#8080=FACE_OUTER_BOUND('',#13962,.T.);
#8081=FACE_OUTER_BOUND('',#13963,.T.);
#8082=FACE_OUTER_BOUND('',#13964,.T.);
#8083=FACE_OUTER_BOUND('',#13965,.T.);
#8084=FACE_OUTER_BOUND('',#13966,.T.);
#8085=FACE_OUTER_BOUND('',#13967,.T.);
#8086=FACE_OUTER_BOUND('',#13968,.T.);
#8087=FACE_OUTER_BOUND('',#13969,.T.);
#8088=FACE_OUTER_BOUND('',#13970,.T.);
#8089=FACE_OUTER_BOUND('',#13971,.T.);
#8090=FACE_OUTER_BOUND('',#13972,.T.);
#8091=FACE_OUTER_BOUND('',#13973,.T.);
#8092=FACE_OUTER_BOUND('',#13974,.T.);
#8093=FACE_OUTER_BOUND('',#13975,.T.);
#8094=FACE_OUTER_BOUND('',#13976,.T.);
#8095=FACE_OUTER_BOUND('',#13977,.T.);
#8096=FACE_OUTER_BOUND('',#13978,.T.);
#8097=FACE_OUTER_BOUND('',#13979,.T.);
#8098=FACE_OUTER_BOUND('',#13980,.T.);
#8099=FACE_OUTER_BOUND('',#13981,.T.);
#8100=FACE_OUTER_BOUND('',#13982,.T.);
#8101=FACE_OUTER_BOUND('',#13983,.T.);
#8102=FACE_OUTER_BOUND('',#13984,.T.);
#8103=FACE_OUTER_BOUND('',#13985,.T.);
#8104=FACE_OUTER_BOUND('',#13986,.T.);
#8105=FACE_OUTER_BOUND('',#13987,.T.);
#8106=FACE_OUTER_BOUND('',#13988,.T.);
#8107=FACE_OUTER_BOUND('',#13989,.T.);
#8108=FACE_OUTER_BOUND('',#13990,.T.);
#8109=FACE_OUTER_BOUND('',#13991,.T.);
#8110=FACE_OUTER_BOUND('',#13992,.T.);
#8111=FACE_OUTER_BOUND('',#13993,.T.);
#8112=FACE_OUTER_BOUND('',#13994,.T.);
#8113=FACE_OUTER_BOUND('',#13995,.T.);
#8114=FACE_OUTER_BOUND('',#13997,.T.);
#8115=FACE_OUTER_BOUND('',#13998,.T.);
#8116=FACE_OUTER_BOUND('',#13999,.T.);
#8117=FACE_OUTER_BOUND('',#14000,.T.);
#8118=FACE_OUTER_BOUND('',#14001,.T.);
#8119=FACE_OUTER_BOUND('',#14002,.T.);
#8120=FACE_OUTER_BOUND('',#14003,.T.);
#8121=FACE_OUTER_BOUND('',#14005,.T.);
#8122=FACE_OUTER_BOUND('',#14006,.T.);
#8123=FACE_OUTER_BOUND('',#14007,.T.);
#8124=FACE_OUTER_BOUND('',#14008,.T.);
#8125=FACE_OUTER_BOUND('',#14009,.T.);
#8126=FACE_OUTER_BOUND('',#14011,.T.);
#8127=FACE_OUTER_BOUND('',#14012,.T.);
#8128=FACE_OUTER_BOUND('',#14014,.T.);
#8129=FACE_OUTER_BOUND('',#14015,.T.);
#8130=FACE_OUTER_BOUND('',#14016,.T.);
#8131=FACE_OUTER_BOUND('',#14017,.T.);
#8132=FACE_OUTER_BOUND('',#14018,.T.);
#8133=FACE_OUTER_BOUND('',#14019,.T.);
#8134=FACE_OUTER_BOUND('',#14020,.T.);
#8135=FACE_OUTER_BOUND('',#14021,.T.);
#8136=FACE_OUTER_BOUND('',#14022,.T.);
#8137=FACE_OUTER_BOUND('',#14023,.T.);
#8138=FACE_OUTER_BOUND('',#14024,.T.);
#8139=FACE_OUTER_BOUND('',#14025,.T.);
#8140=FACE_OUTER_BOUND('',#14026,.T.);
#8141=FACE_OUTER_BOUND('',#14027,.T.);
#8142=FACE_OUTER_BOUND('',#14028,.T.);
#8143=FACE_OUTER_BOUND('',#14029,.T.);
#8144=FACE_OUTER_BOUND('',#14030,.T.);
#8145=FACE_OUTER_BOUND('',#14031,.T.);
#8146=FACE_OUTER_BOUND('',#14032,.T.);
#8147=FACE_OUTER_BOUND('',#14033,.T.);
#8148=FACE_OUTER_BOUND('',#14034,.T.);
#8149=FACE_OUTER_BOUND('',#14035,.T.);
#8150=FACE_OUTER_BOUND('',#14036,.T.);
#8151=FACE_OUTER_BOUND('',#14037,.T.);
#8152=FACE_OUTER_BOUND('',#14038,.T.);
#8153=FACE_OUTER_BOUND('',#14039,.T.);
#8154=FACE_OUTER_BOUND('',#14040,.T.);
#8155=FACE_OUTER_BOUND('',#14041,.T.);
#8156=FACE_OUTER_BOUND('',#14042,.T.);
#8157=FACE_OUTER_BOUND('',#14043,.T.);
#8158=FACE_OUTER_BOUND('',#14044,.T.);
#8159=FACE_OUTER_BOUND('',#14045,.T.);
#8160=FACE_OUTER_BOUND('',#14046,.T.);
#8161=FACE_OUTER_BOUND('',#14047,.T.);
#8162=FACE_OUTER_BOUND('',#14048,.T.);
#8163=FACE_OUTER_BOUND('',#14049,.T.);
#8164=FACE_OUTER_BOUND('',#14050,.T.);
#8165=FACE_OUTER_BOUND('',#14051,.T.);
#8166=FACE_OUTER_BOUND('',#14052,.T.);
#8167=FACE_OUTER_BOUND('',#14053,.T.);
#8168=FACE_OUTER_BOUND('',#14054,.T.);
#8169=FACE_OUTER_BOUND('',#14055,.T.);
#8170=FACE_OUTER_BOUND('',#14056,.T.);
#8171=FACE_OUTER_BOUND('',#14057,.T.);
#8172=FACE_OUTER_BOUND('',#14058,.T.);
#8173=FACE_OUTER_BOUND('',#14059,.T.);
#8174=FACE_OUTER_BOUND('',#14060,.T.);
#8175=FACE_OUTER_BOUND('',#14061,.T.);
#8176=FACE_OUTER_BOUND('',#14062,.T.);
#8177=FACE_OUTER_BOUND('',#14063,.T.);
#8178=FACE_OUTER_BOUND('',#14064,.T.);
#8179=FACE_OUTER_BOUND('',#14065,.T.);
#8180=FACE_OUTER_BOUND('',#14067,.T.);
#8181=FACE_OUTER_BOUND('',#14068,.T.);
#8182=FACE_OUTER_BOUND('',#14069,.T.);
#8183=FACE_OUTER_BOUND('',#14070,.T.);
#8184=FACE_OUTER_BOUND('',#14071,.T.);
#8185=FACE_OUTER_BOUND('',#14072,.T.);
#8186=FACE_OUTER_BOUND('',#14073,.T.);
#8187=FACE_OUTER_BOUND('',#14074,.T.);
#8188=FACE_OUTER_BOUND('',#14075,.T.);
#8189=FACE_OUTER_BOUND('',#14076,.T.);
#8190=FACE_OUTER_BOUND('',#14077,.T.);
#8191=FACE_OUTER_BOUND('',#14078,.T.);
#8192=FACE_OUTER_BOUND('',#14079,.T.);
#8193=FACE_OUTER_BOUND('',#14080,.T.);
#8194=FACE_OUTER_BOUND('',#14081,.T.);
#8195=FACE_OUTER_BOUND('',#14082,.T.);
#8196=FACE_OUTER_BOUND('',#14083,.T.);
#8197=FACE_OUTER_BOUND('',#14084,.T.);
#8198=FACE_OUTER_BOUND('',#14085,.T.);
#8199=FACE_OUTER_BOUND('',#14086,.T.);
#8200=FACE_OUTER_BOUND('',#14087,.T.);
#8201=FACE_OUTER_BOUND('',#14088,.T.);
#8202=FACE_OUTER_BOUND('',#14089,.T.);
#8203=FACE_OUTER_BOUND('',#14090,.T.);
#8204=FACE_OUTER_BOUND('',#14091,.T.);
#8205=FACE_OUTER_BOUND('',#14092,.T.);
#8206=FACE_OUTER_BOUND('',#14093,.T.);
#8207=FACE_OUTER_BOUND('',#14094,.T.);
#8208=FACE_OUTER_BOUND('',#14095,.T.);
#8209=FACE_OUTER_BOUND('',#14096,.T.);
#8210=FACE_OUTER_BOUND('',#14097,.T.);
#8211=FACE_OUTER_BOUND('',#14098,.T.);
#8212=FACE_OUTER_BOUND('',#14099,.T.);
#8213=FACE_OUTER_BOUND('',#14100,.T.);
#8214=FACE_OUTER_BOUND('',#14101,.T.);
#8215=FACE_OUTER_BOUND('',#14102,.T.);
#8216=FACE_OUTER_BOUND('',#14103,.T.);
#8217=FACE_OUTER_BOUND('',#14104,.T.);
#8218=FACE_OUTER_BOUND('',#14105,.T.);
#8219=FACE_OUTER_BOUND('',#14106,.T.);
#8220=FACE_OUTER_BOUND('',#14107,.T.);
#8221=FACE_OUTER_BOUND('',#14108,.T.);
#8222=FACE_OUTER_BOUND('',#14109,.T.);
#8223=FACE_OUTER_BOUND('',#14110,.T.);
#8224=FACE_OUTER_BOUND('',#14111,.T.);
#8225=FACE_OUTER_BOUND('',#14112,.T.);
#8226=FACE_OUTER_BOUND('',#14113,.T.);
#8227=FACE_OUTER_BOUND('',#14114,.T.);
#8228=FACE_OUTER_BOUND('',#14115,.T.);
#8229=FACE_OUTER_BOUND('',#14116,.T.);
#8230=FACE_OUTER_BOUND('',#14117,.T.);
#8231=FACE_OUTER_BOUND('',#14118,.T.);
#8232=FACE_OUTER_BOUND('',#14119,.T.);
#13824=EDGE_LOOP('',(#66724,#66725,#66726,#66727));
#13825=EDGE_LOOP('',(#66728,#66729,#66730,#66731));
#13826=EDGE_LOOP('',(#66732,#66733,#66734,#66735));
#13827=EDGE_LOOP('',(#66736,#66737,#66738,#66739));
#13828=EDGE_LOOP('',(#66740,#66741,#66742,#66743));
#13829=EDGE_LOOP('',(#66744,#66745,#66746,#66747));
#13830=EDGE_LOOP('',(#66748,#66749,#66750,#66751));
#13831=EDGE_LOOP('',(#66752,#66753,#66754,#66755));
#13832=EDGE_LOOP('',(#66756,#66757,#66758,#66759));
#13833=EDGE_LOOP('',(#66760,#66761,#66762,#66763));
#13834=EDGE_LOOP('',(#66764,#66765,#66766,#66767));
#13835=EDGE_LOOP('',(#66768,#66769,#66770,#66771));
#13836=EDGE_LOOP('',(#66772,#66773,#66774,#66775));
#13837=EDGE_LOOP('',(#66776,#66777,#66778,#66779));
#13838=EDGE_LOOP('',(#66780,#66781,#66782,#66783));
#13839=EDGE_LOOP('',(#66784,#66785,#66786,#66787));
#13840=EDGE_LOOP('',(#66788,#66789,#66790,#66791));
#13841=EDGE_LOOP('',(#66792,#66793,#66794,#66795));
#13842=EDGE_LOOP('',(#66796,#66797,#66798,#66799));
#13843=EDGE_LOOP('',(#66800,#66801,#66802,#66803));
#13844=EDGE_LOOP('',(#66804,#66805,#66806,#66807));
#13845=EDGE_LOOP('',(#66808,#66809,#66810,#66811));
#13846=EDGE_LOOP('',(#66812,#66813,#66814,#66815));
#13847=EDGE_LOOP('',(#66816,#66817,#66818,#66819));
#13848=EDGE_LOOP('',(#66820,#66821,#66822,#66823));
#13849=EDGE_LOOP('',(#66824,#66825,#66826,#66827));
#13850=EDGE_LOOP('',(#66828,#66829,#66830,#66831));
#13851=EDGE_LOOP('',(#66832,#66833,#66834,#66835));
#13852=EDGE_LOOP('',(#66836,#66837,#66838,#66839));
#13853=EDGE_LOOP('',(#66840,#66841,#66842,#66843));
#13854=EDGE_LOOP('',(#66844,#66845,#66846,#66847));
#13855=EDGE_LOOP('',(#66848,#66849,#66850,#66851));
#13856=EDGE_LOOP('',(#66852,#66853,#66854,#66855));
#13857=EDGE_LOOP('',(#66856,#66857,#66858,#66859));
#13858=EDGE_LOOP('',(#66860,#66861,#66862,#66863));
#13859=EDGE_LOOP('',(#66864,#66865,#66866,#66867));
#13860=EDGE_LOOP('',(#66868,#66869,#66870,#66871));
#13861=EDGE_LOOP('',(#66872,#66873,#66874,#66875));
#13862=EDGE_LOOP('',(#66876,#66877,#66878,#66879));
#13863=EDGE_LOOP('',(#66880,#66881,#66882,#66883));
#13864=EDGE_LOOP('',(#66884,#66885,#66886,#66887));
#13865=EDGE_LOOP('',(#66888,#66889,#66890,#66891));
#13866=EDGE_LOOP('',(#66892,#66893,#66894,#66895));
#13867=EDGE_LOOP('',(#66896,#66897,#66898,#66899));
#13868=EDGE_LOOP('',(#66900,#66901,#66902,#66903));
#13869=EDGE_LOOP('',(#66904,#66905,#66906,#66907));
#13870=EDGE_LOOP('',(#66908,#66909,#66910,#66911));
#13871=EDGE_LOOP('',(#66912,#66913,#66914,#66915));
#13872=EDGE_LOOP('',(#66916,#66917,#66918,#66919));
#13873=EDGE_LOOP('',(#66920,#66921,#66922,#66923));
#13874=EDGE_LOOP('',(#66924,#66925,#66926,#66927));
#13875=EDGE_LOOP('',(#66928,#66929,#66930,#66931));
#13876=EDGE_LOOP('',(#66932,#66933,#66934,#66935));
#13877=EDGE_LOOP('',(#66936,#66937,#66938,#66939));
#13878=EDGE_LOOP('',(#66940,#66941,#66942,#66943));
#13879=EDGE_LOOP('',(#66944,#66945,#66946,#66947));
#13880=EDGE_LOOP('',(#66948,#66949,#66950,#66951));
#13881=EDGE_LOOP('',(#66952,#66953,#66954,#66955));
#13882=EDGE_LOOP('',(#66956,#66957,#66958,#66959));
#13883=EDGE_LOOP('',(#66960,#66961,#66962,#66963));
#13884=EDGE_LOOP('',(#66964,#66965,#66966,#66967));
#13885=EDGE_LOOP('',(#66968,#66969,#66970,#66971));
#13886=EDGE_LOOP('',(#66972,#66973,#66974,#66975));
#13887=EDGE_LOOP('',(#66976,#66977,#66978,#66979));
#13888=EDGE_LOOP('',(#66980,#66981,#66982,#66983));
#13889=EDGE_LOOP('',(#66984,#66985,#66986,#66987));
#13890=EDGE_LOOP('',(#66988,#66989,#66990,#66991));
#13891=EDGE_LOOP('',(#66992,#66993,#66994,#66995));
#13892=EDGE_LOOP('',(#66996,#66997,#66998,#66999));
#13893=EDGE_LOOP('',(#67000,#67001,#67002,#67003));
#13894=EDGE_LOOP('',(#67004,#67005,#67006,#67007));
#13895=EDGE_LOOP('',(#67008,#67009,#67010,#67011));
#13896=EDGE_LOOP('',(#67012,#67013,#67014,#67015));
#13897=EDGE_LOOP('',(#67016,#67017,#67018,#67019));
#13898=EDGE_LOOP('',(#67020,#67021,#67022,#67023));
#13899=EDGE_LOOP('',(#67024,#67025,#67026,#67027));
#13900=EDGE_LOOP('',(#67028,#67029,#67030,#67031));
#13901=EDGE_LOOP('',(#67032,#67033,#67034,#67035));
#13902=EDGE_LOOP('',(#67036,#67037,#67038,#67039));
#13903=EDGE_LOOP('',(#67040,#67041,#67042,#67043));
#13904=EDGE_LOOP('',(#67044,#67045,#67046,#67047));
#13905=EDGE_LOOP('',(#67048,#67049,#67050,#67051));
#13906=EDGE_LOOP('',(#67052,#67053,#67054,#67055));
#13907=EDGE_LOOP('',(#67056,#67057,#67058,#67059));
#13908=EDGE_LOOP('',(#67060,#67061,#67062,#67063));
#13909=EDGE_LOOP('',(#67064,#67065,#67066,#67067));
#13910=EDGE_LOOP('',(#67068,#67069,#67070,#67071));
#13911=EDGE_LOOP('',(#67072,#67073,#67074,#67075));
#13912=EDGE_LOOP('',(#67076,#67077,#67078,#67079));
#13913=EDGE_LOOP('',(#67080,#67081,#67082,#67083));
#13914=EDGE_LOOP('',(#67084,#67085,#67086,#67087));
#13915=EDGE_LOOP('',(#67088,#67089,#67090,#67091));
#13916=EDGE_LOOP('',(#67092,#67093,#67094,#67095));
#13917=EDGE_LOOP('',(#67096,#67097,#67098,#67099));
#13918=EDGE_LOOP('',(#67100,#67101,#67102,#67103));
#13919=EDGE_LOOP('',(#67104,#67105,#67106,#67107));
#13920=EDGE_LOOP('',(#67108,#67109,#67110,#67111));
#13921=EDGE_LOOP('',(#67112,#67113,#67114,#67115));
#13922=EDGE_LOOP('',(#67116,#67117,#67118,#67119));
#13923=EDGE_LOOP('',(#67120,#67121,#67122,#67123));
#13924=EDGE_LOOP('',(#67124,#67125,#67126,#67127));
#13925=EDGE_LOOP('',(#67128,#67129,#67130,#67131));
#13926=EDGE_LOOP('',(#67132,#67133,#67134,#67135));
#13927=EDGE_LOOP('',(#67136,#67137,#67138,#67139));
#13928=EDGE_LOOP('',(#67140,#67141,#67142,#67143));
#13929=EDGE_LOOP('',(#67144,#67145,#67146,#67147));
#13930=EDGE_LOOP('',(#67148,#67149,#67150,#67151));
#13931=EDGE_LOOP('',(#67152,#67153,#67154,#67155));
#13932=EDGE_LOOP('',(#67156,#67157,#67158,#67159));
#13933=EDGE_LOOP('',(#67160,#67161,#67162,#67163));
#13934=EDGE_LOOP('',(#67164,#67165,#67166,#67167));
#13935=EDGE_LOOP('',(#67168,#67169,#67170,#67171));
#13936=EDGE_LOOP('',(#67172,#67173,#67174,#67175));
#13937=EDGE_LOOP('',(#67176,#67177,#67178,#67179));
#13938=EDGE_LOOP('',(#67180,#67181,#67182,#67183));
#13939=EDGE_LOOP('',(#67184,#67185,#67186,#67187));
#13940=EDGE_LOOP('',(#67188,#67189,#67190,#67191));
#13941=EDGE_LOOP('',(#67192,#67193,#67194,#67195));
#13942=EDGE_LOOP('',(#67196,#67197,#67198,#67199));
#13943=EDGE_LOOP('',(#67200,#67201,#67202,#67203));
#13944=EDGE_LOOP('',(#67204,#67205,#67206,#67207));
#13945=EDGE_LOOP('',(#67208,#67209,#67210,#67211));
#13946=EDGE_LOOP('',(#67212,#67213,#67214,#67215));
#13947=EDGE_LOOP('',(#67216,#67217,#67218,#67219));
#13948=EDGE_LOOP('',(#67220,#67221,#67222,#67223));
#13949=EDGE_LOOP('',(#67224,#67225,#67226,#67227));
#13950=EDGE_LOOP('',(#67228,#67229,#67230,#67231));
#13951=EDGE_LOOP('',(#67232,#67233,#67234,#67235));
#13952=EDGE_LOOP('',(#67236,#67237,#67238,#67239));
#13953=EDGE_LOOP('',(#67240,#67241,#67242,#67243));
#13954=EDGE_LOOP('',(#67244,#67245,#67246,#67247));
#13955=EDGE_LOOP('',(#67248,#67249,#67250,#67251));
#13956=EDGE_LOOP('',(#67252,#67253,#67254,#67255));
#13957=EDGE_LOOP('',(#67256,#67257,#67258,#67259));
#13958=EDGE_LOOP('',(#67260,#67261,#67262,#67263));
#13959=EDGE_LOOP('',(#67264,#67265,#67266,#67267));
#13960=EDGE_LOOP('',(#67268,#67269,#67270,#67271));
#13961=EDGE_LOOP('',(#67272,#67273,#67274,#67275));
#13962=EDGE_LOOP('',(#67276,#67277,#67278,#67279));
#13963=EDGE_LOOP('',(#67280,#67281,#67282,#67283));
#13964=EDGE_LOOP('',(#67284,#67285,#67286,#67287));
#13965=EDGE_LOOP('',(#67288,#67289,#67290,#67291));
#13966=EDGE_LOOP('',(#67292,#67293,#67294,#67295));
#13967=EDGE_LOOP('',(#67296,#67297,#67298,#67299));
#13968=EDGE_LOOP('',(#67300,#67301,#67302,#67303));
#13969=EDGE_LOOP('',(#67304,#67305,#67306,#67307));
#13970=EDGE_LOOP('',(#67308,#67309,#67310,#67311));
#13971=EDGE_LOOP('',(#67312,#67313,#67314,#67315));
#13972=EDGE_LOOP('',(#67316,#67317,#67318,#67319));
#13973=EDGE_LOOP('',(#67320,#67321,#67322,#67323));
#13974=EDGE_LOOP('',(#67324,#67325,#67326,#67327));
#13975=EDGE_LOOP('',(#67328,#67329,#67330,#67331));
#13976=EDGE_LOOP('',(#67332,#67333,#67334,#67335));
#13977=EDGE_LOOP('',(#67336,#67337,#67338,#67339));
#13978=EDGE_LOOP('',(#67340,#67341,#67342,#67343));
#13979=EDGE_LOOP('',(#67344,#67345,#67346,#67347));
#13980=EDGE_LOOP('',(#67348,#67349,#67350,#67351));
#13981=EDGE_LOOP('',(#67352,#67353,#67354,#67355));
#13982=EDGE_LOOP('',(#67356,#67357,#67358,#67359));
#13983=EDGE_LOOP('',(#67360,#67361,#67362,#67363));
#13984=EDGE_LOOP('',(#67364,#67365,#67366,#67367));
#13985=EDGE_LOOP('',(#67368,#67369,#67370,#67371));
#13986=EDGE_LOOP('',(#67372,#67373,#67374,#67375));
#13987=EDGE_LOOP('',(#67376,#67377,#67378,#67379));
#13988=EDGE_LOOP('',(#67380,#67381,#67382,#67383));
#13989=EDGE_LOOP('',(#67384,#67385,#67386,#67387));
#13990=EDGE_LOOP('',(#67388,#67389,#67390,#67391));
#13991=EDGE_LOOP('',(#67392,#67393,#67394,#67395));
#13992=EDGE_LOOP('',(#67396,#67397,#67398,#67399));
#13993=EDGE_LOOP('',(#67400,#67401,#67402,#67403));
#13994=EDGE_LOOP('',(#67404,#67405,#67406,#67407));
#13995=EDGE_LOOP('',(#67408,#67409,#67410,#67411,#67412,#67413,#67414,#67415,
#67416,#67417,#67418,#67419,#67420,#67421,#67422,#67423,#67424,#67425,#67426,
#67427,#67428,#67429,#67430,#67431,#67432,#67433,#67434,#67435,#67436,#67437,
#67438,#67439,#67440,#67441,#67442,#67443,#67444,#67445,#67446,#67447,#67448,
#67449,#67450,#67451,#67452,#67453,#67454,#67455,#67456,#67457,#67458,#67459,
#67460,#67461,#67462,#67463,#67464,#67465,#67466,#67467,#67468,#67469,#67470,
#67471,#67472,#67473,#67474,#67475,#67476,#67477,#67478,#67479,#67480,#67481,
#67482,#67483,#67484,#67485,#67486,#67487,#67488,#67489,#67490,#67491,#67492,
#67493,#67494,#67495,#67496,#67497,#67498,#67499,#67500,#67501,#67502,#67503,
#67504,#67505,#67506,#67507,#67508,#67509,#67510,#67511,#67512,#67513,#67514,
#67515,#67516,#67517,#67518,#67519,#67520,#67521,#67522,#67523,#67524,#67525,
#67526,#67527,#67528,#67529,#67530,#67531,#67532,#67533,#67534,#67535,#67536,
#67537,#67538,#67539,#67540,#67541,#67542,#67543,#67544,#67545,#67546,#67547,
#67548,#67549,#67550,#67551,#67552,#67553,#67554,#67555,#67556,#67557,#67558,
#67559,#67560,#67561,#67562,#67563,#67564,#67565,#67566,#67567,#67568,#67569,
#67570,#67571,#67572,#67573,#67574,#67575,#67576,#67577,#67578,#67579,#67580,
#67581,#67582,#67583));
#13996=EDGE_LOOP('',(#67584));
#13997=EDGE_LOOP('',(#67585,#67586,#67587,#67588));
#13998=EDGE_LOOP('',(#67589,#67590,#67591,#67592));
#13999=EDGE_LOOP('',(#67593,#67594,#67595,#67596));
#14000=EDGE_LOOP('',(#67597,#67598,#67599,#67600));
#14001=EDGE_LOOP('',(#67601,#67602,#67603,#67604));
#14002=EDGE_LOOP('',(#67605,#67606,#67607,#67608));
#14003=EDGE_LOOP('',(#67609,#67610,#67611,#67612,#67613,#67614,#67615,#67616,
#67617,#67618,#67619,#67620,#67621,#67622,#67623,#67624,#67625,#67626,#67627,
#67628,#67629,#67630,#67631,#67632,#67633,#67634,#67635,#67636,#67637,#67638,
#67639,#67640,#67641,#67642,#67643,#67644,#67645,#67646,#67647,#67648,#67649,
#67650,#67651,#67652,#67653,#67654,#67655,#67656,#67657,#67658,#67659,#67660,
#67661,#67662,#67663,#67664,#67665,#67666,#67667,#67668,#67669,#67670,#67671,
#67672,#67673,#67674,#67675,#67676,#67677,#67678,#67679,#67680,#67681,#67682,
#67683,#67684,#67685,#67686,#67687,#67688,#67689,#67690,#67691,#67692,#67693,
#67694,#67695,#67696,#67697,#67698,#67699,#67700,#67701,#67702,#67703,#67704,
#67705,#67706,#67707,#67708,#67709,#67710,#67711,#67712,#67713,#67714,#67715,
#67716,#67717,#67718,#67719,#67720,#67721,#67722,#67723,#67724,#67725,#67726,
#67727,#67728,#67729,#67730,#67731,#67732,#67733,#67734,#67735,#67736,#67737,
#67738,#67739,#67740,#67741,#67742,#67743,#67744,#67745,#67746,#67747,#67748,
#67749,#67750,#67751,#67752,#67753,#67754,#67755,#67756,#67757,#67758,#67759,
#67760,#67761,#67762,#67763,#67764,#67765,#67766,#67767,#67768,#67769,#67770,
#67771,#67772,#67773,#67774,#67775,#67776,#67777,#67778,#67779,#67780,#67781,
#67782,#67783,#67784));
#14004=EDGE_LOOP('',(#67785));
#14005=EDGE_LOOP('',(#67786,#67787,#67788,#67789));
#14006=EDGE_LOOP('',(#67790,#67791,#67792,#67793));
#14007=EDGE_LOOP('',(#67794));
#14008=EDGE_LOOP('',(#67795));
#14009=EDGE_LOOP('',(#67796,#67797,#67798,#67799,#67800,#67801,#67802,#67803,
#67804,#67805,#67806,#67807,#67808,#67809,#67810,#67811,#67812,#67813,#67814,
#67815,#67816,#67817,#67818,#67819,#67820,#67821,#67822,#67823,#67824,#67825,
#67826,#67827,#67828,#67829,#67830,#67831,#67832,#67833,#67834,#67835,#67836,
#67837,#67838,#67839,#67840,#67841,#67842,#67843,#67844,#67845,#67846,#67847,
#67848,#67849,#67850,#67851,#67852,#67853,#67854,#67855,#67856,#67857,#67858,
#67859,#67860,#67861,#67862,#67863,#67864,#67865,#67866,#67867,#67868,#67869,
#67870,#67871,#67872,#67873,#67874,#67875,#67876,#67877,#67878,#67879,#67880,
#67881,#67882,#67883,#67884,#67885,#67886,#67887,#67888,#67889,#67890,#67891,
#67892,#67893,#67894,#67895,#67896,#67897));
#14010=EDGE_LOOP('',(#67898));
#14011=EDGE_LOOP('',(#67899,#67900,#67901,#67902));
#14012=EDGE_LOOP('',(#67903));
#14013=EDGE_LOOP('',(#67904));
#14014=EDGE_LOOP('',(#67905,#67906,#67907,#67908));
#14015=EDGE_LOOP('',(#67909,#67910,#67911,#67912));
#14016=EDGE_LOOP('',(#67913,#67914,#67915,#67916));
#14017=EDGE_LOOP('',(#67917,#67918,#67919,#67920));
#14018=EDGE_LOOP('',(#67921,#67922,#67923,#67924));
#14019=EDGE_LOOP('',(#67925,#67926,#67927,#67928));
#14020=EDGE_LOOP('',(#67929,#67930,#67931,#67932));
#14021=EDGE_LOOP('',(#67933,#67934,#67935,#67936));
#14022=EDGE_LOOP('',(#67937,#67938,#67939,#67940));
#14023=EDGE_LOOP('',(#67941,#67942,#67943,#67944));
#14024=EDGE_LOOP('',(#67945,#67946,#67947,#67948));
#14025=EDGE_LOOP('',(#67949,#67950,#67951,#67952));
#14026=EDGE_LOOP('',(#67953,#67954,#67955,#67956));
#14027=EDGE_LOOP('',(#67957,#67958,#67959,#67960));
#14028=EDGE_LOOP('',(#67961,#67962,#67963,#67964));
#14029=EDGE_LOOP('',(#67965,#67966,#67967,#67968));
#14030=EDGE_LOOP('',(#67969,#67970,#67971,#67972));
#14031=EDGE_LOOP('',(#67973,#67974,#67975,#67976));
#14032=EDGE_LOOP('',(#67977,#67978,#67979,#67980));
#14033=EDGE_LOOP('',(#67981,#67982,#67983,#67984));
#14034=EDGE_LOOP('',(#67985,#67986,#67987,#67988));
#14035=EDGE_LOOP('',(#67989,#67990,#67991,#67992));
#14036=EDGE_LOOP('',(#67993,#67994,#67995,#67996));
#14037=EDGE_LOOP('',(#67997,#67998,#67999,#68000));
#14038=EDGE_LOOP('',(#68001,#68002,#68003,#68004));
#14039=EDGE_LOOP('',(#68005,#68006,#68007,#68008));
#14040=EDGE_LOOP('',(#68009,#68010,#68011,#68012));
#14041=EDGE_LOOP('',(#68013,#68014,#68015,#68016));
#14042=EDGE_LOOP('',(#68017,#68018,#68019,#68020));
#14043=EDGE_LOOP('',(#68021,#68022,#68023,#68024));
#14044=EDGE_LOOP('',(#68025,#68026,#68027,#68028));
#14045=EDGE_LOOP('',(#68029,#68030,#68031,#68032));
#14046=EDGE_LOOP('',(#68033,#68034,#68035,#68036));
#14047=EDGE_LOOP('',(#68037,#68038,#68039,#68040));
#14048=EDGE_LOOP('',(#68041,#68042,#68043,#68044));
#14049=EDGE_LOOP('',(#68045,#68046,#68047,#68048));
#14050=EDGE_LOOP('',(#68049,#68050,#68051,#68052));
#14051=EDGE_LOOP('',(#68053,#68054,#68055,#68056));
#14052=EDGE_LOOP('',(#68057,#68058,#68059,#68060));
#14053=EDGE_LOOP('',(#68061,#68062,#68063,#68064));
#14054=EDGE_LOOP('',(#68065,#68066,#68067,#68068));
#14055=EDGE_LOOP('',(#68069,#68070,#68071,#68072));
#14056=EDGE_LOOP('',(#68073,#68074,#68075,#68076));
#14057=EDGE_LOOP('',(#68077,#68078,#68079,#68080));
#14058=EDGE_LOOP('',(#68081,#68082,#68083,#68084));
#14059=EDGE_LOOP('',(#68085,#68086,#68087,#68088));
#14060=EDGE_LOOP('',(#68089,#68090,#68091,#68092));
#14061=EDGE_LOOP('',(#68093,#68094,#68095,#68096));
#14062=EDGE_LOOP('',(#68097,#68098,#68099,#68100));
#14063=EDGE_LOOP('',(#68101,#68102,#68103,#68104));
#14064=EDGE_LOOP('',(#68105,#68106,#68107,#68108));
#14065=EDGE_LOOP('',(#68109,#68110,#68111,#68112,#68113,#68114,#68115,#68116,
#68117,#68118,#68119,#68120,#68121,#68122,#68123,#68124,#68125,#68126,#68127,
#68128,#68129,#68130,#68131,#68132,#68133,#68134,#68135,#68136,#68137,#68138,
#68139,#68140,#68141,#68142,#68143,#68144,#68145,#68146,#68147,#68148,#68149,
#68150,#68151,#68152,#68153,#68154,#68155,#68156,#68157,#68158,#68159,#68160,
#68161,#68162,#68163,#68164,#68165,#68166,#68167,#68168,#68169,#68170,#68171,
#68172,#68173,#68174,#68175,#68176,#68177,#68178,#68179,#68180,#68181,#68182,
#68183,#68184,#68185,#68186,#68187,#68188,#68189,#68190,#68191,#68192,#68193,
#68194,#68195,#68196,#68197,#68198,#68199,#68200,#68201,#68202,#68203,#68204,
#68205,#68206,#68207,#68208,#68209,#68210));
#14066=EDGE_LOOP('',(#68211));
#14067=EDGE_LOOP('',(#68212,#68213,#68214,#68215));
#14068=EDGE_LOOP('',(#68216,#68217,#68218,#68219));
#14069=EDGE_LOOP('',(#68220,#68221,#68222,#68223));
#14070=EDGE_LOOP('',(#68224,#68225,#68226,#68227));
#14071=EDGE_LOOP('',(#68228,#68229,#68230,#68231));
#14072=EDGE_LOOP('',(#68232,#68233,#68234,#68235));
#14073=EDGE_LOOP('',(#68236,#68237,#68238,#68239));
#14074=EDGE_LOOP('',(#68240,#68241,#68242,#68243));
#14075=EDGE_LOOP('',(#68244,#68245,#68246,#68247));
#14076=EDGE_LOOP('',(#68248,#68249,#68250,#68251));
#14077=EDGE_LOOP('',(#68252,#68253,#68254,#68255));
#14078=EDGE_LOOP('',(#68256,#68257,#68258,#68259));
#14079=EDGE_LOOP('',(#68260,#68261,#68262,#68263));
#14080=EDGE_LOOP('',(#68264,#68265,#68266,#68267));
#14081=EDGE_LOOP('',(#68268,#68269,#68270,#68271));
#14082=EDGE_LOOP('',(#68272,#68273,#68274,#68275));
#14083=EDGE_LOOP('',(#68276,#68277,#68278,#68279));
#14084=EDGE_LOOP('',(#68280,#68281,#68282,#68283));
#14085=EDGE_LOOP('',(#68284,#68285,#68286,#68287));
#14086=EDGE_LOOP('',(#68288,#68289,#68290,#68291));
#14087=EDGE_LOOP('',(#68292,#68293,#68294,#68295));
#14088=EDGE_LOOP('',(#68296,#68297,#68298,#68299));
#14089=EDGE_LOOP('',(#68300,#68301,#68302,#68303));
#14090=EDGE_LOOP('',(#68304,#68305,#68306,#68307));
#14091=EDGE_LOOP('',(#68308,#68309,#68310,#68311));
#14092=EDGE_LOOP('',(#68312,#68313,#68314,#68315));
#14093=EDGE_LOOP('',(#68316,#68317,#68318,#68319));
#14094=EDGE_LOOP('',(#68320,#68321,#68322,#68323));
#14095=EDGE_LOOP('',(#68324,#68325,#68326,#68327));
#14096=EDGE_LOOP('',(#68328,#68329,#68330,#68331));
#14097=EDGE_LOOP('',(#68332,#68333,#68334,#68335));
#14098=EDGE_LOOP('',(#68336,#68337,#68338,#68339));
#14099=EDGE_LOOP('',(#68340,#68341,#68342,#68343));
#14100=EDGE_LOOP('',(#68344,#68345,#68346,#68347));
#14101=EDGE_LOOP('',(#68348,#68349,#68350,#68351));
#14102=EDGE_LOOP('',(#68352,#68353,#68354,#68355));
#14103=EDGE_LOOP('',(#68356,#68357,#68358,#68359));
#14104=EDGE_LOOP('',(#68360,#68361,#68362,#68363));
#14105=EDGE_LOOP('',(#68364,#68365,#68366,#68367));
#14106=EDGE_LOOP('',(#68368,#68369,#68370,#68371));
#14107=EDGE_LOOP('',(#68372,#68373,#68374,#68375));
#14108=EDGE_LOOP('',(#68376,#68377,#68378,#68379));
#14109=EDGE_LOOP('',(#68380,#68381,#68382,#68383));
#14110=EDGE_LOOP('',(#68384,#68385,#68386,#68387));
#14111=EDGE_LOOP('',(#68388,#68389,#68390,#68391));
#14112=EDGE_LOOP('',(#68392,#68393,#68394,#68395));
#14113=EDGE_LOOP('',(#68396,#68397,#68398,#68399));
#14114=EDGE_LOOP('',(#68400,#68401,#68402,#68403));
#14115=EDGE_LOOP('',(#68404,#68405,#68406,#68407));
#14116=EDGE_LOOP('',(#68408,#68409,#68410,#68411));
#14117=EDGE_LOOP('',(#68412,#68413,#68414,#68415));
#14118=EDGE_LOOP('',(#68416,#68417,#68418,#68419));
#14119=EDGE_LOOP('',(#68420));
#14120=EDGE_LOOP('',(#68421));
#20150=CIRCLE('',#98434,11.5);
#20151=CIRCLE('',#98435,11.5);
#20152=CIRCLE('',#98437,10.375);
#20153=CIRCLE('',#98438,10.375);
#20154=CIRCLE('',#98440,11.5);
#20155=CIRCLE('',#98441,11.5);
#20156=CIRCLE('',#98443,10.375);
#20157=CIRCLE('',#98444,10.375);
#20158=CIRCLE('',#98446,11.5);
#20159=CIRCLE('',#98447,11.5);
#20160=CIRCLE('',#98449,10.375);
#20161=CIRCLE('',#98450,10.375);
#20162=CIRCLE('',#98452,11.5);
#20163=CIRCLE('',#98453,11.5);
#20164=CIRCLE('',#98455,10.375);
#20165=CIRCLE('',#98456,10.375);
#20166=CIRCLE('',#98458,11.5);
#20167=CIRCLE('',#98459,11.5);
#20168=CIRCLE('',#98461,10.375);
#20169=CIRCLE('',#98462,10.375);
#20170=CIRCLE('',#98464,11.5);
#20171=CIRCLE('',#98465,11.5);
#20172=CIRCLE('',#98467,10.375);
#20173=CIRCLE('',#98468,10.375);
#20174=CIRCLE('',#98470,11.5);
#20175=CIRCLE('',#98471,11.5);
#20176=CIRCLE('',#98473,10.375);
#20177=CIRCLE('',#98474,10.375);
#20178=CIRCLE('',#98476,11.5);
#20179=CIRCLE('',#98477,11.5);
#20180=CIRCLE('',#98479,10.375);
#20181=CIRCLE('',#98480,10.375);
#20182=CIRCLE('',#98482,11.5);
#20183=CIRCLE('',#98483,11.5);
#20184=CIRCLE('',#98485,10.375);
#20185=CIRCLE('',#98486,10.375);
#20186=CIRCLE('',#98488,11.5);
#20187=CIRCLE('',#98489,11.5);
#20188=CIRCLE('',#98491,10.375);
#20189=CIRCLE('',#98492,10.375);
#20190=CIRCLE('',#98494,11.5);
#20191=CIRCLE('',#98495,11.5);
#20192=CIRCLE('',#98497,10.375);
#20193=CIRCLE('',#98498,10.375);
#20194=CIRCLE('',#98500,11.5);
#20195=CIRCLE('',#98501,11.5);
#20196=CIRCLE('',#98503,10.375);
#20197=CIRCLE('',#98504,10.375);
#20198=CIRCLE('',#98506,11.5);
#20199=CIRCLE('',#98507,11.5);
#20200=CIRCLE('',#98509,10.375);
#20201=CIRCLE('',#98510,10.375);
#20202=CIRCLE('',#98512,11.5);
#20203=CIRCLE('',#98513,11.5);
#20204=CIRCLE('',#98515,10.375);
#20205=CIRCLE('',#98516,10.375);
#20206=CIRCLE('',#98518,11.5);
#20207=CIRCLE('',#98519,11.5);
#20208=CIRCLE('',#98521,10.375);
#20209=CIRCLE('',#98522,10.375);
#20210=CIRCLE('',#98524,11.5);
#20211=CIRCLE('',#98525,11.5);
#20212=CIRCLE('',#98527,10.375);
#20213=CIRCLE('',#98528,10.375);
#20214=CIRCLE('',#98530,11.5);
#20215=CIRCLE('',#98531,11.5);
#20216=CIRCLE('',#98533,10.375);
#20217=CIRCLE('',#98534,10.375);
#20218=CIRCLE('',#98536,11.5);
#20219=CIRCLE('',#98537,11.5);
#20220=CIRCLE('',#98539,10.375);
#20221=CIRCLE('',#98540,10.375);
#20222=CIRCLE('',#98542,11.5);
#20223=CIRCLE('',#98543,11.5);
#20224=CIRCLE('',#98545,10.375);
#20225=CIRCLE('',#98546,10.375);
#20226=CIRCLE('',#98548,11.5);
#20227=CIRCLE('',#98549,11.5);
#20228=CIRCLE('',#98551,10.375);
#20229=CIRCLE('',#98552,10.375);
#20230=CIRCLE('',#98554,11.5);
#20231=CIRCLE('',#98555,11.5);
#20232=CIRCLE('',#98557,10.375);
#20233=CIRCLE('',#98558,10.375);
#20234=CIRCLE('',#98560,11.5);
#20235=CIRCLE('',#98561,11.5);
#20236=CIRCLE('',#98563,10.375);
#20237=CIRCLE('',#98564,10.375);
#20238=CIRCLE('',#98566,11.5);
#20239=CIRCLE('',#98567,11.5);
#20240=CIRCLE('',#98569,10.375);
#20241=CIRCLE('',#98570,10.375);
#20242=CIRCLE('',#98572,11.5);
#20243=CIRCLE('',#98573,11.5);
#20244=CIRCLE('',#98575,10.375);
#20245=CIRCLE('',#98576,10.375);
#20246=CIRCLE('',#98578,11.5);
#20247=CIRCLE('',#98579,11.5);
#20248=CIRCLE('',#98581,10.375);
#20249=CIRCLE('',#98582,10.375);
#20250=CIRCLE('',#98584,11.5);
#20251=CIRCLE('',#98585,11.5);
#20252=CIRCLE('',#98587,10.375);
#20253=CIRCLE('',#98588,10.375);
#20254=CIRCLE('',#98590,11.5);
#20255=CIRCLE('',#98591,11.5);
#20256=CIRCLE('',#98593,10.375);
#20257=CIRCLE('',#98594,10.375);
#20258=CIRCLE('',#98596,11.5);
#20259=CIRCLE('',#98597,11.5);
#20260=CIRCLE('',#98599,10.375);
#20261=CIRCLE('',#98600,10.375);
#20262=CIRCLE('',#98602,11.5);
#20263=CIRCLE('',#98603,11.5);
#20264=CIRCLE('',#98605,10.375);
#20265=CIRCLE('',#98606,10.375);
#20266=CIRCLE('',#98608,11.5);
#20267=CIRCLE('',#98609,11.5);
#20268=CIRCLE('',#98611,10.375);
#20269=CIRCLE('',#98612,10.375);
#20270=CIRCLE('',#98614,11.5);
#20271=CIRCLE('',#98615,11.5);
#20272=CIRCLE('',#98617,10.375);
#20273=CIRCLE('',#98618,10.375);
#20274=CIRCLE('',#98620,11.5);
#20275=CIRCLE('',#98621,11.5);
#20276=CIRCLE('',#98623,10.375);
#20277=CIRCLE('',#98624,10.375);
#20278=CIRCLE('',#98626,11.5);
#20279=CIRCLE('',#98627,11.5);
#20280=CIRCLE('',#98629,10.375);
#20281=CIRCLE('',#98630,10.375);
#20282=CIRCLE('',#98632,11.5);
#20283=CIRCLE('',#98633,11.5);
#20284=CIRCLE('',#98635,10.375);
#20285=CIRCLE('',#98636,10.375);
#20286=CIRCLE('',#98638,11.5);
#20287=CIRCLE('',#98639,11.5);
#20288=CIRCLE('',#98641,10.375);
#20289=CIRCLE('',#98642,10.375);
#20290=CIRCLE('',#98644,11.5);
#20291=CIRCLE('',#98645,11.5);
#20292=CIRCLE('',#98647,10.375);
#20293=CIRCLE('',#98648,10.375);
#20294=CIRCLE('',#98650,11.5);
#20295=CIRCLE('',#98651,11.5);
#20296=CIRCLE('',#98653,10.375);
#20297=CIRCLE('',#98654,10.375);
#20298=CIRCLE('',#98656,11.5);
#20299=CIRCLE('',#98657,11.5);
#20300=CIRCLE('',#98659,10.375);
#20301=CIRCLE('',#98660,10.375);
#20302=CIRCLE('',#98662,11.5);
#20303=CIRCLE('',#98663,11.5);
#20304=CIRCLE('',#98665,10.375);
#20305=CIRCLE('',#98666,10.375);
#20306=CIRCLE('',#98668,11.5);
#20307=CIRCLE('',#98669,11.5);
#20308=CIRCLE('',#98671,10.375);
#20309=CIRCLE('',#98672,10.375);
#20310=CIRCLE('',#98674,11.5);
#20311=CIRCLE('',#98675,11.5);
#20312=CIRCLE('',#98677,10.375);
#20313=CIRCLE('',#98678,10.375);
#20314=CIRCLE('',#98680,11.5);
#20315=CIRCLE('',#98681,11.5);
#20316=CIRCLE('',#98683,10.375);
#20317=CIRCLE('',#98684,10.375);
#20318=CIRCLE('',#98686,11.5);
#20319=CIRCLE('',#98687,11.5);
#20320=CIRCLE('',#98689,10.375);
#20321=CIRCLE('',#98690,10.375);
#20322=CIRCLE('',#98691,11.5);
#20323=CIRCLE('',#98692,3.5);
#20324=CIRCLE('',#98694,10.375);
#20325=CIRCLE('',#98696,10.375);
#20326=CIRCLE('',#98698,11.5);
#20327=CIRCLE('',#98700,3.5);
#20328=CIRCLE('',#98703,1.5);
#20329=CIRCLE('',#98704,1.5);
#20330=CIRCLE('',#98706,1.5);
#20331=CIRCLE('',#98707,1.5);
#20332=CIRCLE('',#98711,3.625);
#20333=CIRCLE('',#98712,4.75);
#20334=CIRCLE('',#98713,3.625);
#20335=CIRCLE('',#98714,4.75);
#20336=CIRCLE('',#98715,3.625);
#20337=CIRCLE('',#98716,4.75);
#20338=CIRCLE('',#98717,3.625);
#20339=CIRCLE('',#98718,4.75);
#20340=CIRCLE('',#98719,3.625);
#20341=CIRCLE('',#98720,4.75);
#20342=CIRCLE('',#98721,3.625);
#20343=CIRCLE('',#98722,4.75);
#20344=CIRCLE('',#98723,3.625);
#20345=CIRCLE('',#98724,4.75);
#20346=CIRCLE('',#98725,3.625);
#20347=CIRCLE('',#98726,4.75);
#20348=CIRCLE('',#98727,3.625);
#20349=CIRCLE('',#98728,4.75);
#20350=CIRCLE('',#98729,3.625);
#20351=CIRCLE('',#98730,4.75);
#20352=CIRCLE('',#98731,3.625);
#20353=CIRCLE('',#98732,4.75);
#20354=CIRCLE('',#98733,3.625);
#20355=CIRCLE('',#98734,4.75);
#20356=CIRCLE('',#98735,3.625);
#20357=CIRCLE('',#98736,4.75);
#20358=CIRCLE('',#98737,3.625);
#20359=CIRCLE('',#98738,4.75);
#20360=CIRCLE('',#98739,3.625);
#20361=CIRCLE('',#98740,4.75);
#20362=CIRCLE('',#98741,3.625);
#20363=CIRCLE('',#98742,4.75);
#20364=CIRCLE('',#98743,3.625);
#20365=CIRCLE('',#98744,4.75);
#20366=CIRCLE('',#98745,3.5);
#20367=CIRCLE('',#98747,3.);
#20368=CIRCLE('',#98748,3.);
#20369=CIRCLE('',#98751,4.75);
#20370=CIRCLE('',#98754,3.625);
#20371=CIRCLE('',#98757,4.75);
#20372=CIRCLE('',#98760,3.625);
#20373=CIRCLE('',#98763,4.75);
#20374=CIRCLE('',#98766,3.625);
#20375=CIRCLE('',#98769,4.75);
#20376=CIRCLE('',#98772,3.625);
#20377=CIRCLE('',#98775,4.75);
#20378=CIRCLE('',#98778,3.625);
#20379=CIRCLE('',#98781,4.75);
#20380=CIRCLE('',#98784,3.625);
#20381=CIRCLE('',#98787,4.75);
#20382=CIRCLE('',#98790,3.625);
#20383=CIRCLE('',#98793,4.75);
#20384=CIRCLE('',#98796,3.625);
#20385=CIRCLE('',#98799,4.75);
#20386=CIRCLE('',#98802,3.625);
#20387=CIRCLE('',#98803,4.75);
#20388=CIRCLE('',#98804,3.625);
#20389=CIRCLE('',#98805,4.75);
#20390=CIRCLE('',#98806,3.625);
#20391=CIRCLE('',#98807,4.75);
#20392=CIRCLE('',#98808,3.625);
#20393=CIRCLE('',#98809,4.75);
#20394=CIRCLE('',#98810,3.625);
#20395=CIRCLE('',#98811,4.75);
#20396=CIRCLE('',#98812,3.625);
#20397=CIRCLE('',#98813,4.75);
#20398=CIRCLE('',#98814,3.625);
#20399=CIRCLE('',#98815,4.75);
#20400=CIRCLE('',#98816,3.625);
#20401=CIRCLE('',#98817,4.75);
#20402=CIRCLE('',#98818,3.625);
#20403=CIRCLE('',#98854,3.5);
#24319=B_SPLINE_CURVE_WITH_KNOTS('',5,(#154494,#154495,#154496,#154497,
#154498,#154499,#154500,#154501,#154502,#154503,#154504,#154505,#154506,
#154507,#154508,#154509,#154510,#154511,#154512,#154513,#154514,#154515,
#154516,#154517,#154518,#154519,#154520,#154521,#154522,#154523,#154524,
#154525,#154526,#154527,#154528,#154529,#154530,#154531,#154532,#154533,
#154534,#154535,#154536,#154537,#154538,#154539,#154540,#154541,#154542,
#154543,#154544,#154545,#154546,#154547,#154548,#154549,#154550,#154551,
#154552,#154553,#154554,#154555,#154556,#154557,#154558,#154559,#154560,
#154561,#154562,#154563,#154564,#154565,#154566,#154567,#154568,#154569,
#154570,#154571,#154572,#154573,#154574,#154575,#154576,#154577,#154578,
#154579,#154580,#154581,#154582,#154583,#154584,#154585,#154586,#154587,
#154588,#154589,#154590,#154591,#154592,#154593,#154594,#154595,#154596,
#154597,#154598,#154599,#154600,#154601,#154602,#154603,#154604,#154605,
#154606,#154607,#154608,#154609,#154610,#154611,#154612,#154613,#154614,
#154615,#154616,#154617,#154618,#154619,#154620,#154621,#154622,#154623,
#154624,#154625,#154626,#154627,#154628,#154629,#154630,#154631,#154632,
#154633,#154634,#154635,#154636,#154637,#154638,#154639,#154640,#154641,
#154642,#154643,#154644,#154645,#154646,#154647,#154648,#154649,#154650,
#154651,#154652,#154653,#154654,#154655,#154656,#154657,#154658,#154659,
#154660,#154661,#154662,#154663,#154664,#154665,#154666,#154667,#154668,
#154669,#154670,#154671,#154672,#154673,#154674,#154675,#154676,#154677,
#154678,#154679,#154680,#154681,#154682,#154683,#154684,#154685,#154686,
#154687,#154688,#154689,#154690,#154691,#154692,#154693,#154694,#154695,
#154696,#154697,#154698,#154699,#154700,#154701,#154702,#154703,#154704,
#154705,#154706,#154707,#154708,#154709,#154710,#154711,#154712,#154713,
#154714,#154715,#154716,#154717,#154718,#154719,#154720,#154721,#154722,
#154723,#154724,#154725,#154726,#154727,#154728,#154729,#154730,#154731,
#154732,#154733,#154734,#154735,#154736,#154737,#154738,#154739,#154740,
#154741,#154742,#154743,#154744,#154745,#154746,#154747,#154748,#154749,
#154750,#154751,#154752,#154753,#154754,#154755,#154756,#154757,#154758,
#154759,#154760,#154761,#154762,#154763,#154764,#154765,#154766,#154767,
#154768,#154769,#154770,#154771,#154772,#154773,#154774,#154775,#154776,
#154777,#154778,#154779,#154780,#154781,#154782,#154783,#154784,#154785,
#154786,#154787,#154788,#154789,#154790,#154791,#154792,#154793,#154794,
#154795,#154796,#154797,#154798,#154799,#154800,#154801,#154802,#154803,
#154804,#154805,#154806,#154807,#154808,#154809,#154810,#154811,#154812,
#154813,#154814,#154815,#154816,#154817,#154818,#154819,#154820,#154821,
#154822,#154823,#154824,#154825,#154826,#154827,#154828,#154829,#154830,
#154831,#154832,#154833,#154834,#154835,#154836,#154837,#154838,#154839,
#154840,#154841,#154842,#154843,#154844,#154845,#154846,#154847,#154848,
#154849,#154850,#154851,#154852,#154853,#154854,#154855,#154856,#154857,
#154858,#154859,#154860,#154861,#154862,#154863,#154864,#154865,#154866,
#154867,#154868,#154869,#154870,#154871,#154872,#154873,#154874,#154875,
#154876,#154877,#154878,#154879,#154880,#154881,#154882,#154883,#154884,
#154885,#154886,#154887,#154888,#154889,#154890,#154891,#154892,#154893,
#154894,#154895,#154896,#154897,#154898,#154899,#154900,#154901,#154902,
#154903,#154904,#154905,#154906,#154907,#154908,#154909,#154910,#154911,
#154912,#154913,#154914,#154915,#154916,#154917,#154918,#154919,#154920,
#154921,#154922,#154923,#154924,#154925,#154926,#154927,#154928,#154929,
#154930,#154931,#154932,#154933,#154934,#154935,#154936,#154937,#154938,
#154939,#154940,#154941,#154942,#154943,#154944,#154945,#154946,#154947,
#154948,#154949,#154950,#154951,#154952,#154953,#154954,#154955,#154956,
#154957,#154958,#154959,#154960,#154961,#154962,#154963,#154964),
 .UNSPECIFIED.,.F.,.F.,(6,1,1,1,1,1,1,1,1,1,1,1,1,1,1,1,1,1,1,1,1,1,1,1,
1,1,1,1,1,1,1,1,1,1,1,1,1,1,1,1,1,1,1,1,1,1,1,1,1,1,1,1,1,1,1,1,1,1,1,1,
1,1,1,1,1,1,1,1,1,1,1,1,1,1,1,1,1,1,1,1,1,1,1,1,1,1,1,1,1,1,1,1,1,1,1,1,
1,1,1,1,1,1,1,1,1,1,1,1,1,1,1,1,1,1,1,1,1,1,1,1,1,1,1,1,1,1,1,1,1,1,1,1,
1,1,1,1,1,1,1,1,1,1,1,1,1,1,1,1,1,1,1,1,1,1,1,1,1,1,1,1,1,1,1,1,1,1,1,1,
1,1,1,1,1,1,1,1,1,1,1,1,1,1,1,1,1,1,1,1,1,1,1,1,1,1,1,1,1,1,1,1,1,1,1,1,
1,1,1,1,1,1,1,1,1,1,1,1,1,1,1,1,1,1,1,1,1,1,1,1,1,1,1,1,1,1,1,1,1,1,1,1,
1,1,1,1,1,1,1,1,1,1,1,1,1,1,1,1,1,1,1,1,1,1,1,1,1,1,1,1,1,1,1,1,1,1,1,1,
1,1,1,1,1,1,1,1,1,1,1,1,1,1,1,1,1,1,1,1,1,1,1,1,1,1,1,1,1,1,1,1,1,1,1,1,
1,1,1,1,1,1,1,1,1,1,1,1,1,1,1,1,1,1,1,1,1,1,1,1,1,1,1,1,1,1,1,1,1,1,1,1,
1,1,1,1,1,1,1,1,1,1,1,1,1,1,1,1,1,1,1,1,1,1,1,1,1,1,1,1,1,1,1,1,1,1,1,1,
1,1,1,1,1,1,1,1,1,1,1,1,1,1,1,1,1,1,1,1,1,1,1,1,1,1,1,1,1,1,1,1,1,1,1,1,
1,1,1,1,1,1,1,1,1,1,1,1,1,1,1,1,1,1,1,1,1,1,1,1,1,1,1,1,1,1,1,1,1,1,1,1,
1,1,1,1,1,1,1,1,1,1,6),(0.143172102,0.144954128,0.146788991,0.148623853,
0.150458716,0.152293578,0.15412844,0.155963303,0.157798165,0.159633028,
0.16146789,0.163302752,0.165137615,0.166972477,0.168807339,0.170642202,
0.172477064,0.174311927,0.176146789,0.177981651,0.179816514,0.181651376,
0.183486239,0.185321101,0.187155963,0.188990826,0.190825688,0.19266055,
0.194495413,0.196330275,0.198165138,0.2,0.201834862,0.203669725,0.205504587,
0.20733945,0.209174312,0.211009174,0.212844037,0.214678899,0.216513761,
0.218348624,0.220183486,0.222018349,0.223853211,0.225688073,0.227522936,
0.231192661,0.233027523,0.234862385,0.236697248,0.23853211,0.240366972,
0.242201835,0.244036697,0.24587156,0.247706422,0.249541284,0.251376147,
0.253211009,0.255045872,0.256880734,0.258715596,0.260550459,0.262385321,
0.264220183,0.266055046,0.267889908,0.269724771,0.271559633,0.273394495,
0.275229358,0.27706422,0.278899083,0.280733945,0.282568807,0.28440367,0.286238532,
0.288073394,0.289908257,0.291743119,0.293577982,0.295412844,0.297247706,
0.299082569,0.300917431,0.302752294,0.304587156,0.306422018,0.308256881,
0.310091743,0.311926606,0.313761468,0.31559633,0.317431193,0.319266055,
0.321100917,0.32293578,0.324770642,0.326605505,0.328440367,0.330275229,
0.332110092,0.333944954,0.335779817,0.337614679,0.339449541,0.341284404,
0.343119266,0.344954128,0.346788991,0.348623853,0.350458716,0.352293578,
0.35412844,0.355963303,0.357798165,0.359633028,0.36146789,0.363302752,0.365137615,
0.366972477,0.368807339,0.370642202,0.372477064,0.374311927,0.376146789,
0.377981651,0.379816514,0.381651376,0.383486239,0.385321101,0.387155963,
0.388990826,0.390825688,0.39266055,0.394495413,0.396330275,0.398165138,
0.4,0.401834862,0.403669725,0.405504587,0.40733945,0.409174312,0.411009174,
0.412844037,0.414678899,0.416513761,0.418348624,0.420183486,0.422018349,
0.423853211,0.425688073,0.427522936,0.429357798,0.431192661,0.433027523,
0.434862385,0.436697248,0.43853211,0.440366972,0.442201835,0.444036697,
0.44587156,0.447706422,0.449541284,0.451376147,0.453211009,0.455045872,
0.456880734,0.458715596,0.460550459,0.462385321,0.464220183,0.466055046,
0.467889908,0.469724771,0.471559633,0.473394495,0.475229358,0.47706422,
0.478899083,0.480733945,0.482568807,0.48440367,0.486238532,0.488073394,
0.489908257,0.491743119,0.493577982,0.495412844,0.497247706,0.499082569,
0.500917431,0.502752294,0.504587156,0.506422018,0.508256881,0.510091743,
0.511926606,0.513761468,0.51559633,0.517431193,0.519266055,0.521100917,
0.52293578,0.524770642,0.526605505,0.528440367,0.530275229,0.532110092,
0.533944954,0.535779817,0.537614679,0.539449541,0.541284404,0.543119266,
0.544954128,0.546788991,0.548623853,0.550458716,0.552293578,0.55412844,
0.555963303,0.557798165,0.559633028,0.56146789,0.563302752,0.565137615,
0.566972477,0.568807339,0.570642202,0.572477064,0.574311927,0.576146789,
0.577981651,0.579816514,0.581651376,0.583486239,0.585321101,0.587155963,
0.588990826,0.590825688,0.59266055,0.594495413,0.596330275,0.598165138,
0.6,0.601834862,0.603669725,0.605504587,0.60733945,0.609174312,0.611009174,
0.612844037,0.614678899,0.616513761,0.618348624,0.620183486,0.622018349,
0.623853211,0.625688073,0.627522936,0.629357798,0.631192661,0.633027523,
0.634862385,0.636697248,0.63853211,0.640366972,0.642201835,0.644036697,
0.64587156,0.647706422,0.649541284,0.651376147,0.653211009,0.655045872,
0.656880734,0.658715596,0.660550459,0.662385321,0.664220183,0.666055046,
0.667889908,0.669724771,0.671559633,0.673394495,0.675229358,0.67706422,
0.678899083,0.680733945,0.682568807,0.68440367,0.686238532,0.688073394,
0.689908257,0.691743119,0.693577982,0.695412844,0.697247706,0.699082569,
0.700917431,0.702752294,0.704587156,0.706422018,0.708256881,0.710091743,
0.711926606,0.713761468,0.71559633,0.717431193,0.719266055,0.721100917,
0.72293578,0.724770642,0.726605505,0.728440367,0.730275229,0.732110092,
0.733944954,0.735779817,0.737614679,0.739449541,0.741284404,0.743119266,
0.744954128,0.746788991,0.748623853,0.750458716,0.752293578,0.75412844,
0.755963303,0.757798165,0.759633028,0.76146789,0.763302752,0.765137615,
0.766972477,0.768807339,0.770642202,0.772477064,0.774311927,0.776146789,
0.777981651,0.779816514,0.781651376,0.783486239,0.785321101,0.787155963,
0.788990826,0.790825688,0.79266055,0.794495413,0.796330275,0.798165138,
0.8,0.801834862,0.803669725,0.805504587,0.80733945,0.809174312,0.811009174,
0.812844037,0.814678899,0.816513761,0.818348624,0.820183486,0.822018349,
0.823853211,0.825688073,0.827522936,0.829357798,0.831192661,0.833027523,
0.834862385,0.836697248,0.83853211,0.840366972,0.842201835,0.844036697,
0.84587156,0.847706422,0.849541284,0.851376147,0.853211009,0.855045872,
0.856880734,0.858715596,0.860550459,0.862385321,0.864220183,0.866055046,
0.867889908,0.869724771,0.871559633,0.873394495,0.875229358,0.87706422,
0.878899083,0.880733945,0.882568807,0.88440367,0.886238532,0.888073394,
0.889908257,0.891743119,0.893577982,0.895412844,0.897247706,0.899082569,
0.900917431,0.902752294,0.904587156,0.906422018,0.908256881,0.910091743,
0.911926606,0.913761468,0.91559633,0.917431193,0.919266055,0.921100917,
0.92293578,0.924770642,0.926605505,0.928440367,0.930275229,0.932110092,
0.933944954,0.935779817,0.937614679,0.939449541,0.941284404,0.943119266,
0.944954128,0.946788991,0.948623853,0.950458716,0.952293578,0.95412844,
0.955963303,0.957798165,0.959633028,0.96146789,0.963302752,0.965137615,
0.966972477,0.968807339,0.970642202,0.972477064,0.974311927,0.976146789,
0.977981651,0.979816514,0.981651376,0.983486239,0.985321101,0.987155963,
0.988990826,0.990825688,0.99266055,0.994495413,0.996330275,0.998165138,
1.),.UNSPECIFIED.);
#24320=B_SPLINE_CURVE_WITH_KNOTS('',5,(#154965,#154966,#154967,#154968,
#154969,#154970,#154971,#154972,#154973,#154974,#154975,#154976,#154977,
#154978,#154979,#154980,#154981,#154982,#154983,#154984,#154985,#154986,
#154987,#154988,#154989,#154990,#154991,#154992,#154993,#154994,#154995,
#154996,#154997,#154998,#154999,#155000,#155001,#155002,#155003,#155004,
#155005,#155006,#155007,#155008,#155009,#155010,#155011,#155012,#155013,
#155014,#155015,#155016,#155017,#155018,#155019,#155020,#155021,#155022,
#155023,#155024,#155025,#155026,#155027,#155028,#155029,#155030,#155031,
#155032,#155033,#155034,#155035,#155036,#155037,#155038,#155039,#155040,
#155041,#155042,#155043,#155044,#155045,#155046,#155047,#155048,#155049,
#155050,#155051,#155052,#155053,#155054,#155055,#155056,#155057,#155058,
#155059,#155060,#155061,#155062,#155063,#155064,#155065,#155066,#155067,
#155068,#155069,#155070,#155071,#155072,#155073,#155074,#155075,#155076,
#155077,#155078,#155079,#155080,#155081,#155082,#155083,#155084,#155085,
#155086,#155087,#155088,#155089,#155090,#155091,#155092,#155093,#155094,
#155095,#155096,#155097,#155098,#155099,#155100,#155101,#155102,#155103,
#155104,#155105,#155106,#155107,#155108,#155109,#155110,#155111,#155112,
#155113,#155114,#155115,#155116,#155117,#155118,#155119,#155120,#155121,
#155122,#155123,#155124,#155125,#155126,#155127,#155128,#155129,#155130,
#155131,#155132,#155133,#155134,#155135,#155136,#155137,#155138,#155139,
#155140,#155141,#155142,#155143,#155144,#155145,#155146,#155147,#155148,
#155149,#155150,#155151,#155152,#155153,#155154,#155155,#155156,#155157,
#155158,#155159,#155160,#155161,#155162,#155163,#155164,#155165,#155166,
#155167,#155168,#155169,#155170,#155171,#155172,#155173,#155174,#155175,
#155176,#155177,#155178,#155179,#155180,#155181,#155182,#155183,#155184,
#155185,#155186,#155187,#155188,#155189,#155190,#155191,#155192,#155193,
#155194,#155195,#155196,#155197,#155198,#155199,#155200,#155201,#155202,
#155203,#155204,#155205,#155206,#155207,#155208,#155209,#155210,#155211,
#155212,#155213,#155214,#155215,#155216,#155217,#155218,#155219,#155220,
#155221,#155222,#155223,#155224,#155225,#155226,#155227,#155228,#155229,
#155230,#155231,#155232,#155233,#155234,#155235,#155236,#155237,#155238,
#155239,#155240,#155241,#155242,#155243,#155244,#155245,#155246,#155247,
#155248,#155249,#155250,#155251,#155252,#155253,#155254,#155255,#155256,
#155257,#155258,#155259,#155260,#155261,#155262,#155263,#155264,#155265,
#155266,#155267,#155268,#155269,#155270,#155271,#155272,#155273,#155274,
#155275,#155276,#155277,#155278,#155279,#155280,#155281,#155282,#155283,
#155284,#155285,#155286,#155287,#155288,#155289,#155290,#155291,#155292,
#155293,#155294,#155295,#155296,#155297,#155298,#155299,#155300,#155301,
#155302,#155303,#155304,#155305,#155306,#155307,#155308,#155309,#155310,
#155311,#155312,#155313,#155314,#155315,#155316,#155317,#155318,#155319,
#155320,#155321,#155322,#155323,#155324,#155325,#155326,#155327,#155328,
#155329,#155330,#155331,#155332,#155333,#155334,#155335,#155336,#155337,
#155338,#155339,#155340,#155341,#155342,#155343,#155344,#155345,#155346,
#155347,#155348,#155349,#155350,#155351,#155352,#155353,#155354,#155355,
#155356,#155357,#155358,#155359,#155360,#155361,#155362,#155363,#155364,
#155365,#155366,#155367,#155368,#155369,#155370,#155371,#155372,#155373,
#155374,#155375,#155376,#155377,#155378,#155379,#155380,#155381,#155382,
#155383,#155384,#155385,#155386,#155387,#155388,#155389,#155390,#155391,
#155392,#155393,#155394,#155395,#155396,#155397,#155398,#155399,#155400,
#155401,#155402,#155403,#155404,#155405,#155406,#155407,#155408,#155409,
#155410,#155411,#155412,#155413,#155414,#155415,#155416,#155417,#155418,
#155419,#155420,#155421,#155422,#155423,#155424,#155425,#155426,#155427,
#155428,#155429,#155430,#155431,#155432,#155433,#155434,#155435),
 .UNSPECIFIED.,.F.,.F.,(6,1,1,1,1,1,1,1,1,1,1,1,1,1,1,1,1,1,1,1,1,1,1,1,
1,1,1,1,1,1,1,1,1,1,1,1,1,1,1,1,1,1,1,1,1,1,1,1,1,1,1,1,1,1,1,1,1,1,1,1,
1,1,1,1,1,1,1,1,1,1,1,1,1,1,1,1,1,1,1,1,1,1,1,1,1,1,1,1,1,1,1,1,1,1,1,1,
1,1,1,1,1,1,1,1,1,1,1,1,1,1,1,1,1,1,1,1,1,1,1,1,1,1,1,1,1,1,1,1,1,1,1,1,
1,1,1,1,1,1,1,1,1,1,1,1,1,1,1,1,1,1,1,1,1,1,1,1,1,1,1,1,1,1,1,1,1,1,1,1,
1,1,1,1,1,1,1,1,1,1,1,1,1,1,1,1,1,1,1,1,1,1,1,1,1,1,1,1,1,1,1,1,1,1,1,1,
1,1,1,1,1,1,1,1,1,1,1,1,1,1,1,1,1,1,1,1,1,1,1,1,1,1,1,1,1,1,1,1,1,1,1,1,
1,1,1,1,1,1,1,1,1,1,1,1,1,1,1,1,1,1,1,1,1,1,1,1,1,1,1,1,1,1,1,1,1,1,1,1,
1,1,1,1,1,1,1,1,1,1,1,1,1,1,1,1,1,1,1,1,1,1,1,1,1,1,1,1,1,1,1,1,1,1,1,1,
1,1,1,1,1,1,1,1,1,1,1,1,1,1,1,1,1,1,1,1,1,1,1,1,1,1,1,1,1,1,1,1,1,1,1,1,
1,1,1,1,1,1,1,1,1,1,1,1,1,1,1,1,1,1,1,1,1,1,1,1,1,1,1,1,1,1,1,1,1,1,1,1,
1,1,1,1,1,1,1,1,1,1,1,1,1,1,1,1,1,1,1,1,1,1,1,1,1,1,1,1,1,1,1,1,1,1,1,1,
1,1,1,1,1,1,1,1,1,1,1,1,1,1,1,1,1,1,1,1,1,1,1,1,1,1,1,1,1,1,1,1,1,1,1,1,
1,1,1,1,1,1,1,1,1,1,6),(0.143172102,0.144954128,0.146788991,0.148623853,
0.150458716,0.152293578,0.15412844,0.155963303,0.157798165,0.159633028,
0.16146789,0.163302752,0.165137615,0.166972477,0.168807339,0.170642202,
0.172477064,0.174311927,0.176146789,0.177981651,0.179816514,0.181651376,
0.183486239,0.185321101,0.187155963,0.188990826,0.190825688,0.19266055,
0.194495413,0.196330275,0.198165138,0.2,0.201834862,0.203669725,0.205504587,
0.20733945,0.209174312,0.211009174,0.212844037,0.214678899,0.216513761,
0.218348624,0.220183486,0.222018349,0.223853211,0.225688073,0.227522936,
0.231192661,0.233027523,0.234862385,0.236697248,0.23853211,0.240366972,
0.242201835,0.244036697,0.24587156,0.247706422,0.249541284,0.251376147,
0.253211009,0.255045872,0.256880734,0.258715596,0.260550459,0.262385321,
0.264220183,0.266055046,0.267889908,0.269724771,0.271559633,0.273394495,
0.275229358,0.27706422,0.278899083,0.280733945,0.282568807,0.28440367,0.286238532,
0.288073394,0.289908257,0.291743119,0.293577982,0.295412844,0.297247706,
0.299082569,0.300917431,0.302752294,0.304587156,0.306422018,0.308256881,
0.310091743,0.311926606,0.313761468,0.31559633,0.317431193,0.319266055,
0.321100917,0.32293578,0.324770642,0.326605505,0.328440367,0.330275229,
0.332110092,0.333944954,0.335779817,0.337614679,0.339449541,0.341284404,
0.343119266,0.344954128,0.346788991,0.348623853,0.350458716,0.352293578,
0.35412844,0.355963303,0.357798165,0.359633028,0.36146789,0.363302752,0.365137615,
0.366972477,0.368807339,0.370642202,0.372477064,0.374311927,0.376146789,
0.377981651,0.379816514,0.381651376,0.383486239,0.385321101,0.387155963,
0.388990826,0.390825688,0.39266055,0.394495413,0.396330275,0.398165138,
0.4,0.401834862,0.403669725,0.405504587,0.40733945,0.409174312,0.411009174,
0.412844037,0.414678899,0.416513761,0.418348624,0.420183486,0.422018349,
0.423853211,0.425688073,0.427522936,0.429357798,0.431192661,0.433027523,
0.434862385,0.436697248,0.43853211,0.440366972,0.442201835,0.444036697,
0.44587156,0.447706422,0.449541284,0.451376147,0.453211009,0.455045872,
0.456880734,0.458715596,0.460550459,0.462385321,0.464220183,0.466055046,
0.467889908,0.469724771,0.471559633,0.473394495,0.475229358,0.47706422,
0.478899083,0.480733945,0.482568807,0.48440367,0.486238532,0.488073394,
0.489908257,0.491743119,0.493577982,0.495412844,0.497247706,0.499082569,
0.500917431,0.502752294,0.504587156,0.506422018,0.508256881,0.510091743,
0.511926606,0.513761468,0.51559633,0.517431193,0.519266055,0.521100917,
0.52293578,0.524770642,0.526605505,0.528440367,0.530275229,0.532110092,
0.533944954,0.535779817,0.537614679,0.539449541,0.541284404,0.543119266,
0.544954128,0.546788991,0.548623853,0.550458716,0.552293578,0.55412844,
0.555963303,0.557798165,0.559633028,0.56146789,0.563302752,0.565137615,
0.566972477,0.568807339,0.570642202,0.572477064,0.574311927,0.576146789,
0.577981651,0.579816514,0.581651376,0.583486239,0.585321101,0.587155963,
0.588990826,0.590825688,0.59266055,0.594495413,0.596330275,0.598165138,
0.6,0.601834862,0.603669725,0.605504587,0.60733945,0.609174312,0.611009174,
0.612844037,0.614678899,0.616513761,0.618348624,0.620183486,0.622018349,
0.623853211,0.625688073,0.627522936,0.629357798,0.631192661,0.633027523,
0.634862385,0.636697248,0.63853211,0.640366972,0.642201835,0.644036697,
0.64587156,0.647706422,0.649541284,0.651376147,0.653211009,0.655045872,
0.656880734,0.658715596,0.660550459,0.662385321,0.664220183,0.666055046,
0.667889908,0.669724771,0.671559633,0.673394495,0.675229358,0.67706422,
0.678899083,0.680733945,0.682568807,0.68440367,0.686238532,0.688073394,
0.689908257,0.691743119,0.693577982,0.695412844,0.697247706,0.699082569,
0.700917431,0.702752294,0.704587156,0.706422018,0.708256881,0.710091743,
0.711926606,0.713761468,0.71559633,0.717431193,0.719266055,0.721100917,
0.72293578,0.724770642,0.726605505,0.728440367,0.730275229,0.732110092,
0.733944954,0.735779817,0.737614679,0.739449541,0.741284404,0.743119266,
0.744954128,0.746788991,0.748623853,0.750458716,0.752293578,0.75412844,
0.755963303,0.757798165,0.759633028,0.76146789,0.763302752,0.765137615,
0.766972477,0.768807339,0.770642202,0.772477064,0.774311927,0.776146789,
0.777981651,0.779816514,0.781651376,0.783486239,0.785321101,0.787155963,
0.788990826,0.790825688,0.79266055,0.794495413,0.796330275,0.798165138,
0.8,0.801834862,0.803669725,0.805504587,0.80733945,0.809174312,0.811009174,
0.812844037,0.814678899,0.816513761,0.818348624,0.820183486,0.822018349,
0.823853211,0.825688073,0.827522936,0.829357798,0.831192661,0.833027523,
0.834862385,0.836697248,0.83853211,0.840366972,0.842201835,0.844036697,
0.84587156,0.847706422,0.849541284,0.851376147,0.853211009,0.855045872,
0.856880734,0.858715596,0.860550459,0.862385321,0.864220183,0.866055046,
0.867889908,0.869724771,0.871559633,0.873394495,0.875229358,0.87706422,
0.878899083,0.880733945,0.882568807,0.88440367,0.886238532,0.888073394,
0.889908257,0.891743119,0.893577982,0.895412844,0.897247706,0.899082569,
0.900917431,0.902752294,0.904587156,0.906422018,0.908256881,0.910091743,
0.911926606,0.913761468,0.91559633,0.917431193,0.919266055,0.921100917,
0.92293578,0.924770642,0.926605505,0.928440367,0.930275229,0.932110092,
0.933944954,0.935779817,0.937614679,0.939449541,0.941284404,0.943119266,
0.944954128,0.946788991,0.948623853,0.950458716,0.952293578,0.95412844,
0.955963303,0.957798165,0.959633028,0.96146789,0.963302752,0.965137615,
0.966972477,0.968807339,0.970642202,0.972477064,0.974311927,0.976146789,
0.977981651,0.979816514,0.981651376,0.983486239,0.985321101,0.987155963,
0.988990826,0.990825688,0.99266055,0.994495413,0.996330275,0.998165138,
1.),.UNSPECIFIED.);
#24321=B_SPLINE_CURVE_WITH_KNOTS('',5,(#156383,#156384,#156385,#156386,
#156387,#156388,#156389,#156390,#156391,#156392,#156393,#156394,#156395,
#156396,#156397,#156398,#156399,#156400,#156401,#156402,#156403,#156404,
#156405,#156406,#156407,#156408,#156409,#156410,#156411,#156412,#156413,
#156414,#156415,#156416,#156417,#156418,#156419,#156420,#156421,#156422,
#156423,#156424,#156425,#156426,#156427,#156428,#156429,#156430,#156431,
#156432,#156433,#156434,#156435,#156436,#156437,#156438,#156439,#156440,
#156441,#156442,#156443,#156444,#156445,#156446,#156447,#156448,#156449,
#156450,#156451,#156452,#156453,#156454,#156455,#156456,#156457,#156458,
#156459,#156460,#156461,#156462,#156463,#156464,#156465,#156466,#156467,
#156468,#156469,#156470,#156471,#156472,#156473,#156474,#156475,#156476,
#156477,#156478,#156479,#156480,#156481,#156482,#156483,#156484,#156485,
#156486,#156487,#156488,#156489,#156490,#156491,#156492,#156493,#156494,
#156495,#156496,#156497,#156498,#156499,#156500,#156501,#156502,#156503,
#156504,#156505,#156506,#156507,#156508,#156509,#156510,#156511,#156512,
#156513,#156514,#156515,#156516,#156517,#156518,#156519,#156520,#156521,
#156522,#156523,#156524,#156525,#156526,#156527,#156528,#156529,#156530,
#156531,#156532,#156533,#156534,#156535,#156536,#156537,#156538,#156539,
#156540,#156541,#156542,#156543,#156544,#156545,#156546,#156547,#156548,
#156549,#156550,#156551,#156552,#156553,#156554,#156555,#156556,#156557,
#156558,#156559,#156560,#156561,#156562,#156563,#156564,#156565,#156566,
#156567,#156568,#156569,#156570,#156571,#156572,#156573,#156574,#156575,
#156576,#156577,#156578,#156579,#156580,#156581,#156582,#156583,#156584,
#156585,#156586,#156587,#156588,#156589,#156590,#156591,#156592,#156593,
#156594,#156595,#156596,#156597,#156598,#156599,#156600,#156601,#156602,
#156603,#156604,#156605,#156606,#156607,#156608,#156609,#156610,#156611,
#156612,#156613,#156614,#156615,#156616,#156617,#156618,#156619,#156620,
#156621,#156622,#156623,#156624,#156625,#156626,#156627,#156628,#156629,
#156630,#156631,#156632,#156633,#156634,#156635,#156636,#156637,#156638,
#156639,#156640,#156641,#156642,#156643,#156644,#156645,#156646,#156647,
#156648,#156649,#156650,#156651,#156652,#156653,#156654,#156655,#156656,
#156657,#156658,#156659,#156660,#156661,#156662,#156663,#156664,#156665,
#156666,#156667,#156668,#156669,#156670,#156671,#156672,#156673,#156674,
#156675,#156676,#156677,#156678,#156679,#156680,#156681,#156682,#156683,
#156684,#156685,#156686,#156687,#156688,#156689,#156690,#156691,#156692,
#156693,#156694,#156695,#156696,#156697,#156698,#156699,#156700,#156701,
#156702,#156703,#156704,#156705,#156706,#156707,#156708,#156709,#156710,
#156711,#156712,#156713,#156714,#156715,#156716,#156717,#156718,#156719,
#156720,#156721,#156722,#156723,#156724,#156725,#156726,#156727,#156728,
#156729,#156730,#156731,#156732,#156733,#156734,#156735,#156736,#156737,
#156738,#156739,#156740,#156741,#156742,#156743,#156744,#156745,#156746,
#156747,#156748,#156749,#156750,#156751,#156752,#156753,#156754,#156755,
#156756,#156757,#156758,#156759,#156760,#156761,#156762,#156763,#156764,
#156765,#156766,#156767,#156768,#156769,#156770,#156771,#156772,#156773,
#156774,#156775,#156776,#156777,#156778,#156779,#156780,#156781,#156782,
#156783,#156784,#156785,#156786,#156787,#156788,#156789,#156790,#156791,
#156792,#156793,#156794,#156795,#156796,#156797,#156798,#156799,#156800,
#156801,#156802,#156803,#156804,#156805,#156806,#156807,#156808,#156809,
#156810,#156811,#156812,#156813,#156814,#156815,#156816,#156817,#156818,
#156819,#156820,#156821,#156822,#156823,#156824,#156825,#156826,#156827,
#156828,#156829,#156830,#156831,#156832,#156833,#156834,#156835,#156836,
#156837,#156838,#156839,#156840,#156841,#156842,#156843,#156844,#156845,
#156846,#156847,#156848,#156849,#156850,#156851,#156852,#156853,#156854),
 .UNSPECIFIED.,.F.,.F.,(6,1,1,1,1,1,1,1,1,1,1,1,1,1,1,1,1,1,1,1,1,1,1,1,
1,1,1,1,1,1,1,1,1,1,1,1,1,1,1,1,1,1,1,1,1,1,1,1,1,1,1,1,1,1,1,1,1,1,1,1,
1,1,1,1,1,1,1,1,1,1,1,1,1,1,1,1,1,1,1,1,1,1,1,1,1,1,1,1,1,1,1,1,1,1,1,1,
1,1,1,1,1,1,1,1,1,1,1,1,1,1,1,1,1,1,1,1,1,1,1,1,1,1,1,1,1,1,1,1,1,1,1,1,
1,1,1,1,1,1,1,1,1,1,1,1,1,1,1,1,1,1,1,1,1,1,1,1,1,1,1,1,1,1,1,1,1,1,1,1,
1,1,1,1,1,1,1,1,1,1,1,1,1,1,1,1,1,1,1,1,1,1,1,1,1,1,1,1,1,1,1,1,1,1,1,1,
1,1,1,1,1,1,1,1,1,1,1,1,1,1,1,1,1,1,1,1,1,1,1,1,1,1,1,1,1,1,1,1,1,1,1,1,
1,1,1,1,1,1,1,1,1,1,1,1,1,1,1,1,1,1,1,1,1,1,1,1,1,1,1,1,1,1,1,1,1,1,1,1,
1,1,1,1,1,1,1,1,1,1,1,1,1,1,1,1,1,1,1,1,1,1,1,1,1,1,1,1,1,1,1,1,1,1,1,1,
1,1,1,1,1,1,1,1,1,1,1,1,1,1,1,1,1,1,1,1,1,1,1,1,1,1,1,1,1,1,1,1,1,1,1,1,
1,1,1,1,1,1,1,1,1,1,1,1,1,1,1,1,1,1,1,1,1,1,1,1,1,1,1,1,1,1,1,1,1,1,1,1,
1,1,1,1,1,1,1,1,1,1,1,1,1,1,1,1,1,1,1,1,1,1,1,1,1,1,1,1,1,1,1,1,1,1,1,1,
1,1,1,1,1,1,1,1,1,1,1,1,1,1,1,1,1,1,1,1,1,1,1,1,1,1,1,1,1,1,1,1,1,1,1,1,
1,1,1,1,1,1,1,1,1,1,1,6),(-1.,-0.998165138,-0.996330275,-0.994495413,-0.99266055,
-0.990825688,-0.988990826,-0.987155963,-0.985321101,-0.983486239,-0.981651376,
-0.979816514,-0.977981651,-0.976146789,-0.974311927,-0.972477064,-0.970642202,
-0.968807339,-0.966972477,-0.965137615,-0.963302752,-0.96146789,-0.959633028,
-0.957798165,-0.955963303,-0.95412844,-0.952293578,-0.950458716,-0.948623853,
-0.946788991,-0.944954128,-0.943119266,-0.941284404,-0.939449541,-0.937614679,
-0.935779817,-0.933944954,-0.932110092,-0.930275229,-0.928440367,-0.926605505,
-0.924770642,-0.92293578,-0.921100917,-0.919266055,-0.917431193,-0.91559633,
-0.913761468,-0.911926606,-0.910091743,-0.908256881,-0.906422018,-0.904587156,
-0.902752294,-0.900917431,-0.899082569,-0.897247706,-0.895412844,-0.893577982,
-0.891743119,-0.889908257,-0.888073394,-0.886238532,-0.88440367,-0.882568807,
-0.880733945,-0.878899083,-0.87706422,-0.875229358,-0.873394495,-0.871559633,
-0.869724771,-0.867889908,-0.866055046,-0.864220183,-0.862385321,-0.860550459,
-0.858715596,-0.856880734,-0.855045872,-0.853211009,-0.851376147,-0.849541284,
-0.847706422,-0.84587156,-0.844036697,-0.842201835,-0.840366972,-0.83853211,
-0.836697248,-0.834862385,-0.833027523,-0.831192661,-0.829357798,-0.827522936,
-0.825688073,-0.823853211,-0.822018349,-0.820183486,-0.818348624,-0.816513761,
-0.814678899,-0.812844037,-0.811009174,-0.809174312,-0.80733945,-0.805504587,
-0.803669725,-0.801834862,-0.8,-0.798165138,-0.796330275,-0.794495413,-0.79266055,
-0.790825688,-0.788990826,-0.787155963,-0.785321101,-0.783486239,-0.781651376,
-0.779816514,-0.777981651,-0.776146789,-0.774311927,-0.772477064,-0.770642202,
-0.768807339,-0.766972477,-0.765137615,-0.763302752,-0.76146789,-0.759633028,
-0.757798165,-0.755963303,-0.75412844,-0.752293578,-0.750458716,-0.748623853,
-0.746788991,-0.744954128,-0.743119266,-0.741284404,-0.739449541,-0.737614679,
-0.735779817,-0.733944954,-0.732110092,-0.730275229,-0.728440367,-0.726605505,
-0.724770642,-0.72293578,-0.721100917,-0.719266055,-0.717431193,-0.71559633,
-0.713761468,-0.711926606,-0.710091743,-0.708256881,-0.706422018,-0.704587156,
-0.702752294,-0.700917431,-0.699082569,-0.697247706,-0.695412844,-0.693577982,
-0.691743119,-0.689908257,-0.688073394,-0.686238532,-0.68440367,-0.682568807,
-0.680733945,-0.678899083,-0.67706422,-0.675229358,-0.673394495,-0.671559633,
-0.669724771,-0.667889908,-0.666055046,-0.664220183,-0.662385321,-0.660550459,
-0.658715596,-0.656880734,-0.655045872,-0.653211009,-0.651376147,-0.649541284,
-0.647706422,-0.64587156,-0.644036697,-0.642201835,-0.640366972,-0.63853211,
-0.636697248,-0.634862385,-0.633027523,-0.631192661,-0.629357798,-0.627522936,
-0.625688073,-0.623853211,-0.622018349,-0.620183486,-0.618348624,-0.616513761,
-0.614678899,-0.612844037,-0.611009174,-0.609174312,-0.60733945,-0.605504587,
-0.603669725,-0.601834862,-0.6,-0.598165138,-0.596330275,-0.594495413,-0.59266055,
-0.590825688,-0.588990826,-0.587155963,-0.585321101,-0.583486239,-0.581651376,
-0.579816514,-0.577981651,-0.576146789,-0.574311927,-0.572477064,-0.570642202,
-0.568807339,-0.566972477,-0.565137615,-0.563302752,-0.56146789,-0.559633028,
-0.557798165,-0.555963303,-0.55412844,-0.552293578,-0.550458716,-0.548623853,
-0.546788991,-0.544954128,-0.543119266,-0.541284404,-0.539449541,-0.537614679,
-0.535779817,-0.533944954,-0.532110092,-0.530275229,-0.528440367,-0.526605505,
-0.524770642,-0.52293578,-0.521100917,-0.519266055,-0.517431193,-0.51559633,
-0.513761468,-0.511926606,-0.510091743,-0.508256881,-0.506422018,-0.504587156,
-0.502752294,-0.500917431,-0.499082569,-0.497247706,-0.495412844,-0.493577982,
-0.491743119,-0.489908257,-0.488073394,-0.486238532,-0.48440367,-0.482568807,
-0.480733945,-0.478899083,-0.47706422,-0.475229358,-0.473394495,-0.471559633,
-0.469724771,-0.467889908,-0.466055046,-0.464220183,-0.462385321,-0.460550459,
-0.458715596,-0.456880734,-0.455045872,-0.453211009,-0.451376147,-0.449541284,
-0.447706422,-0.44587156,-0.444036697,-0.442201835,-0.440366972,-0.43853211,
-0.436697248,-0.434862385,-0.433027523,-0.431192661,-0.429357798,-0.427522936,
-0.425688073,-0.423853211,-0.422018349,-0.420183486,-0.418348624,-0.416513761,
-0.414678899,-0.412844037,-0.411009174,-0.409174312,-0.40733945,-0.405504587,
-0.403669725,-0.401834862,-0.4,-0.398165138,-0.396330275,-0.394495413,-0.39266055,
-0.390825688,-0.388990826,-0.387155963,-0.385321101,-0.383486239,-0.381651376,
-0.379816514,-0.377981651,-0.376146789,-0.374311927,-0.372477064,-0.370642202,
-0.368807339,-0.366972477,-0.365137615,-0.363302752,-0.36146789,-0.359633028,
-0.357798165,-0.355963303,-0.35412844,-0.352293578,-0.350458716,-0.348623853,
-0.346788991,-0.344954128,-0.343119266,-0.341284404,-0.339449541,-0.337614679,
-0.335779817,-0.333944954,-0.332110092,-0.330275229,-0.328440367,-0.326605505,
-0.324770642,-0.32293578,-0.321100917,-0.319266055,-0.317431193,-0.31559633,
-0.313761468,-0.311926606,-0.310091743,-0.308256881,-0.306422018,-0.304587156,
-0.302752294,-0.300917431,-0.299082569,-0.297247706,-0.295412844,-0.293577982,
-0.291743119,-0.289908257,-0.288073394,-0.286238532,-0.28440367,-0.282568807,
-0.280733945,-0.278899083,-0.27706422,-0.275229358,-0.273394495,-0.271559633,
-0.269724771,-0.267889908,-0.266055046,-0.264220183,-0.262385321,-0.260550459,
-0.258715596,-0.256880734,-0.255045872,-0.253211009,-0.251376147,-0.249541284,
-0.247706422,-0.24587156,-0.244036697,-0.242201835,-0.240366972,-0.23853211,
-0.236697248,-0.234862385,-0.233027523,-0.231192661,-0.229357798,-0.227522936,
-0.225688073,-0.223853211,-0.222018349,-0.220183486,-0.218348624,-0.216513761,
-0.214678899,-0.212844037,-0.211009174,-0.209174312,-0.20733945,-0.205504587,
-0.203669725,-0.201834862,-0.2,-0.198165138,-0.196330275,-0.194495413,-0.19266055,
-0.190825688,-0.188990826,-0.187155963,-0.185321101,-0.183486239,-0.181651376,
-0.179816514,-0.177981651,-0.176146789,-0.174311927,-0.172477064,-0.170642202,
-0.168807339,-0.166972477,-0.165137615,-0.163302752,-0.16146789,-0.159633028,
-0.157798165,-0.155963303,-0.15412844,-0.152293578,-0.150458716,-0.148623853,
-0.146788991,-0.144954128,-0.143172102),.UNSPECIFIED.);
#24322=B_SPLINE_CURVE_WITH_KNOTS('',5,(#156855,#156856,#156857,#156858,
#156859,#156860,#156861,#156862,#156863,#156864,#156865,#156866,#156867,
#156868,#156869,#156870,#156871,#156872,#156873,#156874,#156875,#156876,
#156877,#156878,#156879,#156880,#156881,#156882,#156883,#156884,#156885,
#156886,#156887,#156888,#156889,#156890,#156891,#156892,#156893,#156894,
#156895,#156896,#156897,#156898,#156899,#156900,#156901,#156902,#156903,
#156904,#156905,#156906,#156907,#156908,#156909,#156910,#156911,#156912,
#156913,#156914,#156915,#156916,#156917,#156918,#156919,#156920,#156921,
#156922,#156923,#156924,#156925,#156926,#156927,#156928,#156929,#156930,
#156931,#156932,#156933,#156934,#156935,#156936,#156937,#156938,#156939,
#156940,#156941,#156942,#156943,#156944,#156945,#156946,#156947,#156948,
#156949,#156950,#156951,#156952,#156953,#156954,#156955,#156956,#156957,
#156958,#156959,#156960,#156961,#156962,#156963,#156964,#156965,#156966,
#156967,#156968,#156969,#156970,#156971,#156972,#156973,#156974,#156975,
#156976,#156977,#156978,#156979,#156980,#156981,#156982,#156983,#156984,
#156985,#156986,#156987,#156988,#156989,#156990,#156991,#156992,#156993,
#156994,#156995,#156996,#156997,#156998,#156999,#157000,#157001,#157002,
#157003,#157004,#157005,#157006,#157007,#157008,#157009,#157010,#157011,
#157012,#157013,#157014,#157015,#157016,#157017,#157018,#157019,#157020,
#157021,#157022,#157023,#157024,#157025,#157026,#157027,#157028,#157029,
#157030,#157031,#157032,#157033,#157034,#157035,#157036,#157037,#157038,
#157039,#157040,#157041,#157042,#157043,#157044,#157045,#157046,#157047,
#157048,#157049,#157050,#157051,#157052,#157053,#157054,#157055,#157056,
#157057,#157058,#157059,#157060,#157061,#157062,#157063,#157064,#157065,
#157066,#157067,#157068,#157069,#157070,#157071,#157072,#157073,#157074,
#157075,#157076,#157077,#157078,#157079,#157080,#157081,#157082,#157083,
#157084,#157085,#157086,#157087,#157088,#157089,#157090,#157091,#157092,
#157093,#157094,#157095,#157096,#157097,#157098,#157099,#157100,#157101,
#157102,#157103,#157104,#157105,#157106,#157107,#157108,#157109,#157110,
#157111,#157112,#157113,#157114,#157115,#157116,#157117,#157118,#157119,
#157120,#157121,#157122,#157123,#157124,#157125,#157126,#157127,#157128,
#157129,#157130,#157131,#157132,#157133,#157134,#157135,#157136,#157137,
#157138,#157139,#157140,#157141,#157142,#157143,#157144,#157145,#157146,
#157147,#157148,#157149,#157150,#157151,#157152,#157153,#157154,#157155,
#157156,#157157,#157158,#157159,#157160,#157161,#157162,#157163,#157164,
#157165,#157166,#157167,#157168,#157169,#157170,#157171,#157172,#157173,
#157174,#157175,#157176,#157177,#157178,#157179,#157180,#157181,#157182,
#157183,#157184,#157185,#157186,#157187,#157188,#157189,#157190,#157191,
#157192,#157193,#157194,#157195,#157196,#157197,#157198,#157199,#157200,
#157201,#157202,#157203,#157204,#157205,#157206,#157207,#157208,#157209,
#157210,#157211,#157212,#157213,#157214,#157215,#157216,#157217,#157218,
#157219,#157220,#157221,#157222,#157223,#157224,#157225,#157226,#157227,
#157228,#157229,#157230,#157231,#157232,#157233,#157234,#157235,#157236,
#157237,#157238,#157239,#157240,#157241,#157242,#157243,#157244,#157245,
#157246,#157247,#157248,#157249,#157250,#157251,#157252,#157253,#157254,
#157255,#157256,#157257,#157258,#157259,#157260,#157261,#157262,#157263,
#157264,#157265,#157266,#157267,#157268,#157269,#157270,#157271,#157272,
#157273,#157274,#157275,#157276,#157277,#157278,#157279,#157280,#157281,
#157282,#157283,#157284,#157285,#157286,#157287,#157288,#157289,#157290,
#157291,#157292,#157293,#157294,#157295,#157296,#157297,#157298,#157299,
#157300,#157301,#157302,#157303,#157304,#157305,#157306,#157307,#157308,
#157309,#157310,#157311,#157312,#157313,#157314,#157315,#157316,#157317,
#157318,#157319,#157320,#157321,#157322,#157323,#157324,#157325,#157326),
 .UNSPECIFIED.,.F.,.F.,(6,1,1,1,1,1,1,1,1,1,1,1,1,1,1,1,1,1,1,1,1,1,1,1,
1,1,1,1,1,1,1,1,1,1,1,1,1,1,1,1,1,1,1,1,1,1,1,1,1,1,1,1,1,1,1,1,1,1,1,1,
1,1,1,1,1,1,1,1,1,1,1,1,1,1,1,1,1,1,1,1,1,1,1,1,1,1,1,1,1,1,1,1,1,1,1,1,
1,1,1,1,1,1,1,1,1,1,1,1,1,1,1,1,1,1,1,1,1,1,1,1,1,1,1,1,1,1,1,1,1,1,1,1,
1,1,1,1,1,1,1,1,1,1,1,1,1,1,1,1,1,1,1,1,1,1,1,1,1,1,1,1,1,1,1,1,1,1,1,1,
1,1,1,1,1,1,1,1,1,1,1,1,1,1,1,1,1,1,1,1,1,1,1,1,1,1,1,1,1,1,1,1,1,1,1,1,
1,1,1,1,1,1,1,1,1,1,1,1,1,1,1,1,1,1,1,1,1,1,1,1,1,1,1,1,1,1,1,1,1,1,1,1,
1,1,1,1,1,1,1,1,1,1,1,1,1,1,1,1,1,1,1,1,1,1,1,1,1,1,1,1,1,1,1,1,1,1,1,1,
1,1,1,1,1,1,1,1,1,1,1,1,1,1,1,1,1,1,1,1,1,1,1,1,1,1,1,1,1,1,1,1,1,1,1,1,
1,1,1,1,1,1,1,1,1,1,1,1,1,1,1,1,1,1,1,1,1,1,1,1,1,1,1,1,1,1,1,1,1,1,1,1,
1,1,1,1,1,1,1,1,1,1,1,1,1,1,1,1,1,1,1,1,1,1,1,1,1,1,1,1,1,1,1,1,1,1,1,1,
1,1,1,1,1,1,1,1,1,1,1,1,1,1,1,1,1,1,1,1,1,1,1,1,1,1,1,1,1,1,1,1,1,1,1,1,
1,1,1,1,1,1,1,1,1,1,1,1,1,1,1,1,1,1,1,1,1,1,1,1,1,1,1,1,1,1,1,1,1,1,1,1,
1,1,1,1,1,1,1,1,1,1,1,6),(0.143172102,0.144954128,0.146788991,0.148623853,
0.150458716,0.152293578,0.15412844,0.155963303,0.157798165,0.159633028,
0.16146789,0.163302752,0.165137615,0.166972477,0.168807339,0.170642202,
0.172477064,0.174311927,0.176146789,0.177981651,0.179816514,0.181651376,
0.183486239,0.185321101,0.187155963,0.188990826,0.190825688,0.19266055,
0.194495413,0.196330275,0.198165138,0.2,0.201834862,0.203669725,0.205504587,
0.20733945,0.209174312,0.211009174,0.212844037,0.214678899,0.216513761,
0.218348624,0.220183486,0.222018349,0.223853211,0.225688073,0.227522936,
0.229357798,0.231192661,0.233027523,0.234862385,0.236697248,0.23853211,
0.240366972,0.242201835,0.244036697,0.24587156,0.247706422,0.249541284,
0.251376147,0.253211009,0.255045872,0.256880734,0.258715596,0.260550459,
0.262385321,0.264220183,0.266055046,0.267889908,0.269724771,0.271559633,
0.273394495,0.275229358,0.27706422,0.278899083,0.280733945,0.282568807,
0.28440367,0.286238532,0.288073394,0.289908257,0.291743119,0.293577982,
0.295412844,0.297247706,0.299082569,0.300917431,0.302752294,0.304587156,
0.306422018,0.308256881,0.310091743,0.311926606,0.313761468,0.31559633,
0.317431193,0.319266055,0.321100917,0.32293578,0.324770642,0.326605505,
0.328440367,0.330275229,0.332110092,0.333944954,0.335779817,0.337614679,
0.339449541,0.341284404,0.343119266,0.344954128,0.346788991,0.348623853,
0.350458716,0.352293578,0.35412844,0.355963303,0.357798165,0.359633028,
0.36146789,0.363302752,0.365137615,0.366972477,0.368807339,0.370642202,
0.372477064,0.374311927,0.376146789,0.377981651,0.379816514,0.381651376,
0.383486239,0.385321101,0.387155963,0.388990826,0.390825688,0.39266055,
0.394495413,0.396330275,0.398165138,0.4,0.401834862,0.403669725,0.405504587,
0.40733945,0.409174312,0.411009174,0.412844037,0.414678899,0.416513761,
0.418348624,0.420183486,0.422018349,0.423853211,0.425688073,0.427522936,
0.429357798,0.431192661,0.433027523,0.434862385,0.436697248,0.43853211,
0.440366972,0.442201835,0.444036697,0.44587156,0.447706422,0.449541284,
0.451376147,0.453211009,0.455045872,0.456880734,0.458715596,0.460550459,
0.462385321,0.464220183,0.466055046,0.467889908,0.469724771,0.471559633,
0.473394495,0.475229358,0.47706422,0.478899083,0.480733945,0.482568807,
0.48440367,0.486238532,0.488073394,0.489908257,0.491743119,0.493577982,
0.495412844,0.497247706,0.499082569,0.500917431,0.502752294,0.504587156,
0.506422018,0.508256881,0.510091743,0.511926606,0.513761468,0.51559633,
0.517431193,0.519266055,0.521100917,0.52293578,0.524770642,0.526605505,
0.528440367,0.530275229,0.532110092,0.533944954,0.535779817,0.537614679,
0.539449541,0.541284404,0.543119266,0.544954128,0.546788991,0.548623853,
0.550458716,0.552293578,0.55412844,0.555963303,0.557798165,0.559633028,
0.56146789,0.563302752,0.565137615,0.566972477,0.568807339,0.570642202,
0.572477064,0.574311927,0.576146789,0.577981651,0.579816514,0.581651376,
0.583486239,0.585321101,0.587155963,0.588990826,0.590825688,0.59266055,
0.594495413,0.596330275,0.598165138,0.6,0.601834862,0.603669725,0.605504587,
0.60733945,0.609174312,0.611009174,0.612844037,0.614678899,0.616513761,
0.618348624,0.620183486,0.622018349,0.623853211,0.625688073,0.627522936,
0.629357798,0.631192661,0.633027523,0.634862385,0.636697248,0.63853211,
0.640366972,0.642201835,0.644036697,0.64587156,0.647706422,0.649541284,
0.651376147,0.653211009,0.655045872,0.656880734,0.658715596,0.660550459,
0.662385321,0.664220183,0.666055046,0.667889908,0.669724771,0.671559633,
0.673394495,0.675229358,0.67706422,0.678899083,0.680733945,0.682568807,
0.68440367,0.686238532,0.688073394,0.689908257,0.691743119,0.693577982,
0.695412844,0.697247706,0.699082569,0.700917431,0.702752294,0.704587156,
0.706422018,0.708256881,0.710091743,0.711926606,0.713761468,0.71559633,
0.717431193,0.719266055,0.721100917,0.72293578,0.724770642,0.726605505,
0.728440367,0.730275229,0.732110092,0.733944954,0.735779817,0.737614679,
0.739449541,0.741284404,0.743119266,0.744954128,0.746788991,0.748623853,
0.750458716,0.752293578,0.75412844,0.755963303,0.757798165,0.759633028,
0.76146789,0.763302752,0.765137615,0.766972477,0.768807339,0.770642202,
0.772477064,0.774311927,0.776146789,0.777981651,0.779816514,0.781651376,
0.783486239,0.785321101,0.787155963,0.788990826,0.790825688,0.79266055,
0.794495413,0.796330275,0.798165138,0.8,0.801834862,0.803669725,0.805504587,
0.80733945,0.809174312,0.811009174,0.812844037,0.814678899,0.816513761,
0.818348624,0.820183486,0.822018349,0.823853211,0.825688073,0.827522936,
0.829357798,0.831192661,0.833027523,0.834862385,0.836697248,0.83853211,
0.840366972,0.842201835,0.844036697,0.84587156,0.847706422,0.849541284,
0.851376147,0.853211009,0.855045872,0.856880734,0.858715596,0.860550459,
0.862385321,0.864220183,0.866055046,0.867889908,0.869724771,0.871559633,
0.873394495,0.875229358,0.87706422,0.878899083,0.880733945,0.882568807,
0.88440367,0.886238532,0.888073394,0.889908257,0.891743119,0.893577982,
0.895412844,0.897247706,0.899082569,0.900917431,0.902752294,0.904587156,
0.906422018,0.908256881,0.910091743,0.911926606,0.913761468,0.91559633,
0.917431193,0.919266055,0.921100917,0.92293578,0.924770642,0.926605505,
0.928440367,0.930275229,0.932110092,0.933944954,0.935779817,0.937614679,
0.939449541,0.941284404,0.943119266,0.944954128,0.946788991,0.948623853,
0.950458716,0.952293578,0.95412844,0.955963303,0.957798165,0.959633028,
0.96146789,0.963302752,0.965137615,0.966972477,0.968807339,0.970642202,
0.972477064,0.974311927,0.976146789,0.977981651,0.979816514,0.981651376,
0.983486239,0.985321101,0.987155963,0.988990826,0.990825688,0.99266055,
0.994495413,0.996330275,0.998165138,1.),.UNSPECIFIED.);
#24323=B_SPLINE_CURVE_WITH_KNOTS('',3,(#158289,#158290,#158291,#158292,
#158293,#158294,#158295,#158296,#158297,#158298,#158299,#158300,#158301,
#158302,#158303,#158304,#158305,#158306,#158307,#158308,#158309,#158310,
#158311,#158312,#158313,#158314,#158315,#158316,#158317,#158318,#158319,
#158320,#158321,#158322,#158323,#158324,#158325,#158326,#158327,#158328,
#158329,#158330,#158331,#158332,#158333,#158334,#158335,#158336,#158337,
#158338,#158339,#158340,#158341,#158342,#158343,#158344,#158345,#158346,
#158347,#158348,#158349,#158350,#158351,#158352,#158353,#158354,#158355,
#158356,#158357,#158358,#158359,#158360,#158361,#158362,#158363,#158364,
#158365,#158366,#158367,#158368,#158369,#158370,#158371,#158372,#158373,
#158374,#158375,#158376,#158377,#158378,#158379,#158380,#158381,#158382,
#158383,#158384,#158385,#158386,#158387,#158388,#158389,#158390,#158391,
#158392,#158393,#158394,#158395,#158396,#158397,#158398,#158399,#158400,
#158401,#158402,#158403,#158404,#158405,#158406,#158407,#158408,#158409,
#158410,#158411,#158412,#158413,#158414,#158415,#158416,#158417,#158418,
#158419,#158420,#158421,#158422,#158423,#158424,#158425,#158426,#158427,
#158428,#158429,#158430,#158431,#158432,#158433,#158434,#158435,#158436,
#158437,#158438,#158439,#158440,#158441,#158442,#158443,#158444,#158445,
#158446,#158447,#158448,#158449,#158450,#158451,#158452,#158453,#158454,
#158455,#158456,#158457,#158458,#158459,#158460,#158461,#158462,#158463,
#158464,#158465,#158466,#158467,#158468,#158469,#158470,#158471,#158472,
#158473,#158474,#158475,#158476,#158477,#158478,#158479,#158480,#158481,
#158482,#158483,#158484,#158485,#158486,#158487,#158488,#158489,#158490,
#158491,#158492,#158493,#158494,#158495,#158496,#158497,#158498,#158499,
#158500,#158501,#158502,#158503,#158504,#158505,#158506,#158507,#158508,
#158509,#158510,#158511,#158512,#158513,#158514,#158515,#158516,#158517,
#158518,#158519,#158520,#158521,#158522,#158523,#158524,#158525,#158526,
#158527,#158528,#158529,#158530,#158531,#158532,#158533,#158534,#158535,
#158536,#158537,#158538,#158539,#158540,#158541,#158542,#158543,#158544,
#158545,#158546,#158547,#158548,#158549,#158550,#158551,#158552,#158553,
#158554,#158555,#158556,#158557,#158558,#158559,#158560,#158561,#158562,
#158563,#158564,#158565,#158566,#158567,#158568,#158569,#158570,#158571,
#158572,#158573,#158574,#158575,#158576,#158577,#158578,#158579,#158580,
#158581,#158582,#158583,#158584,#158585,#158586,#158587,#158588,#158589,
#158590,#158591,#158592,#158593,#158594,#158595,#158596,#158597,#158598,
#158599,#158600,#158601,#158602,#158603,#158604,#158605,#158606,#158607,
#158608,#158609,#158610),.UNSPECIFIED.,.F.,.F.,(4,3,3,3,3,3,3,3,3,3,3,3,
3,3,3,3,3,3,3,3,3,3,3,3,3,3,3,3,3,3,3,3,3,3,3,3,3,3,3,3,3,3,3,3,3,3,3,3,
3,3,3,3,3,3,3,3,3,3,3,3,3,3,3,3,3,3,3,3,3,3,3,3,3,3,3,3,3,3,3,3,3,3,3,3,
3,3,3,3,3,3,3,3,3,3,3,3,3,3,3,3,3,3,3,3,3,3,3,4),(-1.,-0.994495413,-0.988990826,
-0.983486239,-0.977981651,-0.968807339,-0.963302752,-0.957798165,-0.952293578,
-0.946788991,-0.941284404,-0.935779817,-0.930275229,-0.924770642,-0.919266055,
-0.913761468,-0.908256881,-0.902752294,-0.897247706,-0.891743119,-0.886238532,
-0.880733945,-0.875229358,-0.867889908,-0.862385321,-0.856880734,-0.849541284,
-0.842201835,-0.836697248,-0.831192661,-0.825688073,-0.820183486,-0.814678899,
-0.809174312,-0.801834862,-0.794495413,-0.787155963,-0.779816514,-0.772477064,
-0.765137615,-0.757798165,-0.750458716,-0.741284404,-0.733944954,-0.726605505,
-0.719266055,-0.711926606,-0.704587156,-0.697247706,-0.689908257,-0.678899083,
-0.671559633,-0.664220183,-0.656880734,-0.649541284,-0.642201835,-0.631192661,
-0.623853211,-0.616513761,-0.609174312,-0.601834862,-0.594495413,-0.587155963,
-0.579816514,-0.572477064,-0.565137615,-0.557798165,-0.550458716,-0.543119266,
-0.533944954,-0.524770642,-0.51559633,-0.506422018,-0.497247706,-0.488073394,
-0.478899083,-0.469724771,-0.460550459,-0.451376147,-0.442201835,-0.433027523,
-0.423853211,-0.414678899,-0.405504587,-0.396330275,-0.387155963,-0.374311927,
-0.363302752,-0.352293578,-0.341284404,-0.330275229,-0.319266055,-0.308256881,
-0.297247706,-0.286238532,-0.275229358,-0.264220183,-0.253211009,-0.242201835,
-0.231192661,-0.220183486,-0.209174312,-0.198165138,-0.187155963,-0.176146789,
-0.165137615,-0.15412844,-0.143172102),.UNSPECIFIED.);
#24324=B_SPLINE_CURVE_WITH_KNOTS('',3,(#158611,#158612,#158613,#158614,
#158615,#158616,#158617,#158618,#158619,#158620,#158621,#158622,#158623,
#158624,#158625,#158626,#158627,#158628,#158629,#158630,#158631,#158632,
#158633,#158634,#158635,#158636,#158637,#158638,#158639,#158640,#158641,
#158642,#158643,#158644,#158645,#158646,#158647,#158648,#158649,#158650,
#158651,#158652,#158653,#158654,#158655,#158656,#158657,#158658,#158659,
#158660,#158661,#158662,#158663,#158664,#158665,#158666,#158667,#158668,
#158669,#158670,#158671,#158672,#158673,#158674,#158675,#158676,#158677,
#158678,#158679,#158680,#158681,#158682,#158683,#158684,#158685,#158686,
#158687,#158688,#158689,#158690,#158691,#158692,#158693,#158694,#158695,
#158696,#158697,#158698,#158699,#158700,#158701,#158702,#158703,#158704,
#158705,#158706,#158707,#158708,#158709,#158710,#158711,#158712,#158713,
#158714,#158715,#158716,#158717,#158718,#158719,#158720,#158721,#158722,
#158723,#158724,#158725,#158726,#158727,#158728,#158729,#158730,#158731,
#158732,#158733,#158734,#158735,#158736,#158737,#158738,#158739,#158740,
#158741,#158742,#158743,#158744,#158745,#158746,#158747,#158748,#158749,
#158750,#158751,#158752,#158753,#158754,#158755,#158756,#158757,#158758,
#158759,#158760,#158761,#158762,#158763,#158764,#158765,#158766,#158767,
#158768,#158769,#158770,#158771,#158772,#158773,#158774,#158775,#158776,
#158777,#158778,#158779,#158780,#158781,#158782,#158783,#158784,#158785,
#158786,#158787,#158788,#158789,#158790,#158791,#158792,#158793,#158794,
#158795,#158796,#158797,#158798,#158799,#158800,#158801,#158802,#158803,
#158804,#158805,#158806,#158807,#158808,#158809,#158810,#158811,#158812,
#158813,#158814,#158815,#158816,#158817,#158818,#158819,#158820,#158821,
#158822,#158823,#158824,#158825,#158826,#158827,#158828,#158829,#158830,
#158831,#158832,#158833,#158834,#158835,#158836,#158837,#158838,#158839,
#158840,#158841,#158842,#158843,#158844,#158845,#158846,#158847,#158848,
#158849,#158850,#158851,#158852,#158853,#158854,#158855,#158856,#158857,
#158858,#158859,#158860,#158861,#158862,#158863,#158864,#158865,#158866,
#158867,#158868,#158869,#158870,#158871,#158872,#158873,#158874,#158875,
#158876,#158877,#158878,#158879,#158880,#158881,#158882,#158883,#158884,
#158885,#158886,#158887,#158888,#158889,#158890,#158891,#158892,#158893,
#158894,#158895,#158896,#158897,#158898,#158899,#158900,#158901,#158902,
#158903,#158904,#158905,#158906,#158907,#158908,#158909,#158910,#158911,
#158912,#158913,#158914,#158915,#158916,#158917,#158918,#158919,#158920,
#158921,#158922,#158923,#158924,#158925,#158926),.UNSPECIFIED.,.F.,.F.,
(4,3,3,3,3,3,3,3,3,3,3,3,3,3,3,3,3,3,3,3,3,3,3,3,3,3,3,3,3,3,3,3,3,3,3,
3,3,3,3,3,3,3,3,3,3,3,3,3,3,3,3,3,3,3,3,3,3,3,3,3,3,3,3,3,3,3,3,3,3,3,3,
3,3,3,3,3,3,3,3,3,3,3,3,3,3,3,3,3,3,3,3,3,3,3,3,3,3,3,3,3,3,3,3,3,3,4),
(0.143172102,0.15412844,0.165137615,0.176146789,0.187155963,0.198165138,
0.209174312,0.220183486,0.231192661,0.242201835,0.253211009,0.264220183,
0.275229358,0.286238532,0.297247706,0.310091743,0.321100917,0.332110092,
0.343119266,0.35412844,0.365137615,0.377981651,0.390825688,0.4,0.411009174,
0.420183486,0.429357798,0.43853211,0.447706422,0.456880734,0.466055046,
0.475229358,0.48440367,0.493577982,0.502752294,0.513761468,0.524770642,
0.533944954,0.541284404,0.548623853,0.557798165,0.565137615,0.572477064,
0.579816514,0.587155963,0.594495413,0.601834862,0.609174312,0.616513761,
0.623853211,0.631192661,0.63853211,0.64587156,0.653211009,0.660550459,0.667889908,
0.675229358,0.682568807,0.691743119,0.700917431,0.708256881,0.71559633,
0.72293578,0.730275229,0.737614679,0.744954128,0.752293578,0.759633028,
0.766972477,0.776146789,0.783486239,0.790825688,0.798165138,0.805504587,
0.812844037,0.820183486,0.825688073,0.831192661,0.840366972,0.84587156,
0.853211009,0.858715596,0.864220183,0.869724771,0.87706422,0.882568807,
0.888073394,0.893577982,0.900917431,0.906422018,0.911926606,0.919266055,
0.924770642,0.930275229,0.935779817,0.941284404,0.946788991,0.952293578,
0.957798165,0.963302752,0.968807339,0.974311927,0.979816514,0.985321101,
0.990825688,1.),.UNSPECIFIED.);
#24325=B_SPLINE_CURVE_WITH_KNOTS('',5,(#159871,#159872,#159873,#159874,
#159875,#159876,#159877,#159878,#159879,#159880,#159881,#159882,#159883,
#159884,#159885,#159886,#159887,#159888,#159889,#159890,#159891,#159892,
#159893,#159894,#159895,#159896,#159897,#159898,#159899,#159900,#159901,
#159902,#159903,#159904,#159905,#159906,#159907,#159908,#159909,#159910,
#159911,#159912,#159913,#159914,#159915,#159916,#159917,#159918,#159919,
#159920,#159921,#159922,#159923,#159924,#159925,#159926,#159927,#159928,
#159929,#159930,#159931,#159932,#159933,#159934,#159935,#159936,#159937,
#159938,#159939,#159940,#159941,#159942,#159943,#159944,#159945,#159946,
#159947,#159948,#159949,#159950,#159951,#159952,#159953,#159954,#159955,
#159956,#159957,#159958,#159959,#159960,#159961,#159962,#159963,#159964,
#159965,#159966,#159967,#159968,#159969,#159970,#159971,#159972,#159973,
#159974,#159975,#159976,#159977,#159978,#159979,#159980,#159981,#159982,
#159983,#159984,#159985,#159986,#159987,#159988,#159989,#159990,#159991,
#159992,#159993,#159994,#159995,#159996,#159997,#159998,#159999,#160000,
#160001,#160002,#160003,#160004,#160005,#160006,#160007,#160008,#160009,
#160010,#160011,#160012,#160013,#160014,#160015,#160016,#160017,#160018,
#160019,#160020,#160021,#160022,#160023,#160024,#160025,#160026,#160027,
#160028,#160029,#160030,#160031,#160032,#160033,#160034,#160035,#160036,
#160037,#160038,#160039,#160040,#160041,#160042,#160043,#160044,#160045,
#160046,#160047,#160048,#160049,#160050,#160051,#160052,#160053,#160054,
#160055,#160056,#160057,#160058,#160059,#160060,#160061,#160062,#160063,
#160064,#160065,#160066,#160067,#160068,#160069,#160070,#160071,#160072,
#160073,#160074,#160075,#160076,#160077,#160078,#160079,#160080,#160081,
#160082,#160083,#160084,#160085,#160086,#160087,#160088,#160089,#160090,
#160091,#160092,#160093,#160094,#160095,#160096,#160097,#160098,#160099,
#160100,#160101,#160102,#160103,#160104,#160105,#160106,#160107,#160108,
#160109,#160110,#160111,#160112,#160113,#160114,#160115,#160116,#160117,
#160118,#160119,#160120,#160121,#160122,#160123,#160124,#160125,#160126,
#160127,#160128,#160129,#160130,#160131,#160132,#160133,#160134,#160135,
#160136,#160137,#160138,#160139,#160140,#160141,#160142,#160143,#160144,
#160145,#160146,#160147,#160148,#160149,#160150,#160151,#160152,#160153,
#160154,#160155,#160156,#160157,#160158,#160159,#160160,#160161,#160162,
#160163,#160164,#160165,#160166,#160167,#160168,#160169,#160170,#160171,
#160172,#160173,#160174,#160175,#160176,#160177,#160178,#160179,#160180,
#160181,#160182,#160183,#160184,#160185,#160186,#160187,#160188,#160189,
#160190,#160191,#160192,#160193,#160194,#160195,#160196,#160197,#160198,
#160199,#160200,#160201,#160202,#160203,#160204,#160205,#160206,#160207,
#160208,#160209,#160210,#160211,#160212,#160213,#160214,#160215,#160216,
#160217,#160218,#160219,#160220,#160221,#160222,#160223,#160224,#160225,
#160226,#160227,#160228,#160229,#160230,#160231,#160232,#160233,#160234,
#160235,#160236,#160237,#160238,#160239,#160240,#160241,#160242,#160243,
#160244,#160245,#160246,#160247,#160248,#160249,#160250,#160251,#160252,
#160253,#160254,#160255,#160256,#160257,#160258,#160259,#160260,#160261,
#160262,#160263,#160264,#160265,#160266,#160267,#160268,#160269,#160270,
#160271,#160272,#160273,#160274,#160275,#160276,#160277,#160278,#160279,
#160280,#160281,#160282,#160283,#160284,#160285,#160286,#160287,#160288,
#160289,#160290,#160291,#160292,#160293,#160294,#160295,#160296,#160297,
#160298,#160299,#160300,#160301,#160302,#160303,#160304,#160305,#160306,
#160307,#160308,#160309,#160310,#160311,#160312,#160313,#160314,#160315,
#160316,#160317,#160318,#160319,#160320,#160321,#160322,#160323,#160324,
#160325,#160326,#160327,#160328,#160329,#160330,#160331,#160332,#160333,
#160334,#160335,#160336,#160337,#160338,#160339,#160340,#160341,#160342),
 .UNSPECIFIED.,.F.,.F.,(6,1,1,1,1,1,1,1,1,1,1,1,1,1,1,1,1,1,1,1,1,1,1,1,
1,1,1,1,1,1,1,1,1,1,1,1,1,1,1,1,1,1,1,1,1,1,1,1,1,1,1,1,1,1,1,1,1,1,1,1,
1,1,1,1,1,1,1,1,1,1,1,1,1,1,1,1,1,1,1,1,1,1,1,1,1,1,1,1,1,1,1,1,1,1,1,1,
1,1,1,1,1,1,1,1,1,1,1,1,1,1,1,1,1,1,1,1,1,1,1,1,1,1,1,1,1,1,1,1,1,1,1,1,
1,1,1,1,1,1,1,1,1,1,1,1,1,1,1,1,1,1,1,1,1,1,1,1,1,1,1,1,1,1,1,1,1,1,1,1,
1,1,1,1,1,1,1,1,1,1,1,1,1,1,1,1,1,1,1,1,1,1,1,1,1,1,1,1,1,1,1,1,1,1,1,1,
1,1,1,1,1,1,1,1,1,1,1,1,1,1,1,1,1,1,1,1,1,1,1,1,1,1,1,1,1,1,1,1,1,1,1,1,
1,1,1,1,1,1,1,1,1,1,1,1,1,1,1,1,1,1,1,1,1,1,1,1,1,1,1,1,1,1,1,1,1,1,1,1,
1,1,1,1,1,1,1,1,1,1,1,1,1,1,1,1,1,1,1,1,1,1,1,1,1,1,1,1,1,1,1,1,1,1,1,1,
1,1,1,1,1,1,1,1,1,1,1,1,1,1,1,1,1,1,1,1,1,1,1,1,1,1,1,1,1,1,1,1,1,1,1,1,
1,1,1,1,1,1,1,1,1,1,1,1,1,1,1,1,1,1,1,1,1,1,1,1,1,1,1,1,1,1,1,1,1,1,1,1,
1,1,1,1,1,1,1,1,1,1,1,1,1,1,1,1,1,1,1,1,1,1,1,1,1,1,1,1,1,1,1,1,1,1,1,1,
1,1,1,1,1,1,1,1,1,1,1,1,1,1,1,1,1,1,1,1,1,1,1,1,1,1,1,1,1,1,1,1,1,1,1,1,
1,1,1,1,1,1,1,1,1,1,1,6),(0.143172102,0.144954128,0.146788991,0.148623853,
0.150458716,0.152293578,0.15412844,0.155963303,0.157798165,0.159633028,
0.16146789,0.163302752,0.165137615,0.166972477,0.168807339,0.170642202,
0.172477064,0.174311927,0.176146789,0.177981651,0.179816514,0.181651376,
0.183486239,0.185321101,0.187155963,0.188990826,0.190825688,0.19266055,
0.194495413,0.196330275,0.198165138,0.2,0.201834862,0.203669725,0.205504587,
0.20733945,0.209174312,0.211009174,0.212844037,0.214678899,0.216513761,
0.218348624,0.220183486,0.222018349,0.223853211,0.225688073,0.227522936,
0.229357798,0.231192661,0.233027523,0.234862385,0.236697248,0.23853211,
0.240366972,0.242201835,0.244036697,0.24587156,0.247706422,0.249541284,
0.251376147,0.253211009,0.255045872,0.256880734,0.258715596,0.260550459,
0.262385321,0.264220183,0.266055046,0.267889908,0.269724771,0.271559633,
0.273394495,0.275229358,0.27706422,0.278899083,0.280733945,0.282568807,
0.28440367,0.286238532,0.288073394,0.289908257,0.291743119,0.293577982,
0.295412844,0.297247706,0.299082569,0.300917431,0.302752294,0.304587156,
0.306422018,0.308256881,0.310091743,0.311926606,0.313761468,0.31559633,
0.317431193,0.319266055,0.321100917,0.32293578,0.324770642,0.326605505,
0.328440367,0.330275229,0.332110092,0.333944954,0.335779817,0.337614679,
0.339449541,0.341284404,0.343119266,0.344954128,0.346788991,0.348623853,
0.350458716,0.352293578,0.35412844,0.355963303,0.357798165,0.359633028,
0.36146789,0.363302752,0.365137615,0.366972477,0.368807339,0.370642202,
0.372477064,0.374311927,0.376146789,0.377981651,0.379816514,0.381651376,
0.383486239,0.385321101,0.387155963,0.388990826,0.390825688,0.39266055,
0.394495413,0.396330275,0.398165138,0.4,0.401834862,0.403669725,0.405504587,
0.40733945,0.409174312,0.411009174,0.412844037,0.414678899,0.416513761,
0.418348624,0.420183486,0.422018349,0.423853211,0.425688073,0.427522936,
0.429357798,0.431192661,0.433027523,0.434862385,0.436697248,0.43853211,
0.440366972,0.442201835,0.444036697,0.44587156,0.447706422,0.449541284,
0.451376147,0.453211009,0.455045872,0.456880734,0.458715596,0.460550459,
0.462385321,0.464220183,0.466055046,0.467889908,0.469724771,0.471559633,
0.473394495,0.475229358,0.47706422,0.478899083,0.480733945,0.482568807,
0.48440367,0.486238532,0.488073394,0.489908257,0.491743119,0.493577982,
0.495412844,0.497247706,0.499082569,0.500917431,0.502752294,0.504587156,
0.506422018,0.508256881,0.510091743,0.511926606,0.513761468,0.51559633,
0.517431193,0.519266055,0.521100917,0.52293578,0.524770642,0.526605505,
0.528440367,0.530275229,0.532110092,0.533944954,0.535779817,0.537614679,
0.539449541,0.541284404,0.543119266,0.544954128,0.546788991,0.548623853,
0.550458716,0.552293578,0.55412844,0.555963303,0.557798165,0.559633028,
0.56146789,0.563302752,0.565137615,0.566972477,0.568807339,0.570642202,
0.572477064,0.574311927,0.576146789,0.577981651,0.579816514,0.581651376,
0.583486239,0.585321101,0.587155963,0.588990826,0.590825688,0.59266055,
0.594495413,0.596330275,0.598165138,0.6,0.601834862,0.603669725,0.605504587,
0.60733945,0.609174312,0.611009174,0.612844037,0.614678899,0.616513761,
0.618348624,0.620183486,0.622018349,0.623853211,0.625688073,0.627522936,
0.629357798,0.631192661,0.633027523,0.634862385,0.636697248,0.63853211,
0.640366972,0.642201835,0.644036697,0.64587156,0.647706422,0.649541284,
0.651376147,0.653211009,0.655045872,0.656880734,0.658715596,0.660550459,
0.662385321,0.664220183,0.666055046,0.667889908,0.669724771,0.671559633,
0.673394495,0.675229358,0.67706422,0.678899083,0.680733945,0.682568807,
0.68440367,0.686238532,0.688073394,0.689908257,0.691743119,0.693577982,
0.695412844,0.697247706,0.699082569,0.700917431,0.702752294,0.704587156,
0.706422018,0.708256881,0.710091743,0.711926606,0.713761468,0.71559633,
0.717431193,0.719266055,0.721100917,0.72293578,0.724770642,0.726605505,
0.728440367,0.730275229,0.732110092,0.733944954,0.735779817,0.737614679,
0.739449541,0.741284404,0.743119266,0.744954128,0.746788991,0.748623853,
0.750458716,0.752293578,0.75412844,0.755963303,0.757798165,0.759633028,
0.76146789,0.763302752,0.765137615,0.766972477,0.768807339,0.770642202,
0.772477064,0.774311927,0.776146789,0.777981651,0.779816514,0.781651376,
0.783486239,0.785321101,0.787155963,0.788990826,0.790825688,0.79266055,
0.794495413,0.796330275,0.798165138,0.8,0.801834862,0.803669725,0.805504587,
0.80733945,0.809174312,0.811009174,0.812844037,0.814678899,0.816513761,
0.818348624,0.820183486,0.822018349,0.823853211,0.825688073,0.827522936,
0.829357798,0.831192661,0.833027523,0.834862385,0.836697248,0.83853211,
0.840366972,0.842201835,0.844036697,0.84587156,0.847706422,0.849541284,
0.851376147,0.853211009,0.855045872,0.856880734,0.858715596,0.860550459,
0.862385321,0.864220183,0.866055046,0.867889908,0.869724771,0.871559633,
0.873394495,0.875229358,0.87706422,0.878899083,0.880733945,0.882568807,
0.88440367,0.886238532,0.888073394,0.889908257,0.891743119,0.893577982,
0.895412844,0.897247706,0.899082569,0.900917431,0.902752294,0.904587156,
0.906422018,0.908256881,0.910091743,0.911926606,0.913761468,0.91559633,
0.917431193,0.919266055,0.921100917,0.92293578,0.924770642,0.926605505,
0.928440367,0.930275229,0.932110092,0.933944954,0.935779817,0.937614679,
0.939449541,0.941284404,0.943119266,0.944954128,0.946788991,0.948623853,
0.950458716,0.952293578,0.95412844,0.955963303,0.957798165,0.959633028,
0.96146789,0.963302752,0.965137615,0.966972477,0.968807339,0.970642202,
0.972477064,0.974311927,0.976146789,0.977981651,0.979816514,0.981651376,
0.983486239,0.985321101,0.987155963,0.988990826,0.990825688,0.99266055,
0.994495413,0.996330275,0.998165138,1.),.UNSPECIFIED.);
#24326=B_SPLINE_CURVE_WITH_KNOTS('',5,(#160343,#160344,#160345,#160346,
#160347,#160348,#160349,#160350,#160351,#160352,#160353,#160354,#160355,
#160356,#160357,#160358,#160359,#160360,#160361,#160362,#160363,#160364,
#160365,#160366,#160367,#160368,#160369,#160370,#160371,#160372,#160373,
#160374,#160375,#160376,#160377,#160378,#160379,#160380,#160381,#160382,
#160383,#160384,#160385,#160386,#160387,#160388,#160389,#160390,#160391,
#160392,#160393,#160394,#160395,#160396,#160397,#160398,#160399,#160400,
#160401,#160402,#160403,#160404,#160405,#160406,#160407,#160408,#160409,
#160410,#160411,#160412,#160413,#160414,#160415,#160416,#160417,#160418,
#160419,#160420,#160421,#160422,#160423,#160424,#160425,#160426,#160427,
#160428,#160429,#160430,#160431,#160432,#160433,#160434,#160435,#160436,
#160437,#160438,#160439,#160440,#160441,#160442,#160443,#160444,#160445,
#160446,#160447,#160448,#160449,#160450,#160451,#160452,#160453,#160454,
#160455,#160456,#160457,#160458,#160459,#160460,#160461,#160462,#160463,
#160464,#160465,#160466,#160467,#160468,#160469,#160470,#160471,#160472,
#160473,#160474,#160475,#160476,#160477,#160478,#160479,#160480,#160481,
#160482,#160483,#160484,#160485,#160486,#160487,#160488,#160489,#160490,
#160491,#160492,#160493,#160494,#160495,#160496,#160497,#160498,#160499,
#160500,#160501,#160502,#160503,#160504,#160505,#160506,#160507,#160508,
#160509,#160510,#160511,#160512,#160513,#160514,#160515,#160516,#160517,
#160518,#160519,#160520,#160521,#160522,#160523,#160524,#160525,#160526,
#160527,#160528,#160529,#160530,#160531,#160532,#160533,#160534,#160535,
#160536,#160537,#160538,#160539,#160540,#160541,#160542,#160543,#160544,
#160545,#160546,#160547,#160548,#160549,#160550,#160551,#160552,#160553,
#160554,#160555,#160556,#160557,#160558,#160559,#160560,#160561,#160562,
#160563,#160564,#160565,#160566,#160567,#160568,#160569,#160570,#160571,
#160572,#160573,#160574,#160575,#160576,#160577,#160578,#160579,#160580,
#160581,#160582,#160583,#160584,#160585,#160586,#160587,#160588,#160589,
#160590,#160591,#160592,#160593,#160594,#160595,#160596,#160597,#160598,
#160599,#160600,#160601,#160602,#160603,#160604,#160605,#160606,#160607,
#160608,#160609,#160610,#160611,#160612,#160613,#160614,#160615,#160616,
#160617,#160618,#160619,#160620,#160621,#160622,#160623,#160624,#160625,
#160626,#160627,#160628,#160629,#160630,#160631,#160632,#160633,#160634,
#160635,#160636,#160637,#160638,#160639,#160640,#160641,#160642,#160643,
#160644,#160645,#160646,#160647,#160648,#160649,#160650,#160651,#160652,
#160653,#160654,#160655,#160656,#160657,#160658,#160659,#160660,#160661,
#160662,#160663,#160664,#160665,#160666,#160667,#160668,#160669,#160670,
#160671,#160672,#160673,#160674,#160675,#160676,#160677,#160678,#160679,
#160680,#160681,#160682,#160683,#160684,#160685,#160686,#160687,#160688,
#160689,#160690,#160691,#160692,#160693,#160694,#160695,#160696,#160697,
#160698,#160699,#160700,#160701,#160702,#160703,#160704,#160705,#160706,
#160707,#160708,#160709,#160710,#160711,#160712,#160713,#160714,#160715,
#160716,#160717,#160718,#160719,#160720,#160721,#160722,#160723,#160724,
#160725,#160726,#160727,#160728,#160729,#160730,#160731,#160732,#160733,
#160734,#160735,#160736,#160737,#160738,#160739,#160740,#160741,#160742,
#160743,#160744,#160745,#160746,#160747,#160748,#160749,#160750,#160751,
#160752,#160753,#160754,#160755,#160756,#160757,#160758,#160759,#160760,
#160761,#160762,#160763,#160764,#160765,#160766,#160767,#160768,#160769,
#160770,#160771,#160772,#160773,#160774,#160775,#160776,#160777,#160778,
#160779,#160780,#160781,#160782,#160783,#160784,#160785,#160786,#160787,
#160788,#160789,#160790,#160791,#160792,#160793,#160794,#160795,#160796,
#160797,#160798,#160799,#160800,#160801,#160802,#160803,#160804,#160805,
#160806,#160807,#160808,#160809,#160810,#160811,#160812,#160813,#160814),
 .UNSPECIFIED.,.F.,.F.,(6,1,1,1,1,1,1,1,1,1,1,1,1,1,1,1,1,1,1,1,1,1,1,1,
1,1,1,1,1,1,1,1,1,1,1,1,1,1,1,1,1,1,1,1,1,1,1,1,1,1,1,1,1,1,1,1,1,1,1,1,
1,1,1,1,1,1,1,1,1,1,1,1,1,1,1,1,1,1,1,1,1,1,1,1,1,1,1,1,1,1,1,1,1,1,1,1,
1,1,1,1,1,1,1,1,1,1,1,1,1,1,1,1,1,1,1,1,1,1,1,1,1,1,1,1,1,1,1,1,1,1,1,1,
1,1,1,1,1,1,1,1,1,1,1,1,1,1,1,1,1,1,1,1,1,1,1,1,1,1,1,1,1,1,1,1,1,1,1,1,
1,1,1,1,1,1,1,1,1,1,1,1,1,1,1,1,1,1,1,1,1,1,1,1,1,1,1,1,1,1,1,1,1,1,1,1,
1,1,1,1,1,1,1,1,1,1,1,1,1,1,1,1,1,1,1,1,1,1,1,1,1,1,1,1,1,1,1,1,1,1,1,1,
1,1,1,1,1,1,1,1,1,1,1,1,1,1,1,1,1,1,1,1,1,1,1,1,1,1,1,1,1,1,1,1,1,1,1,1,
1,1,1,1,1,1,1,1,1,1,1,1,1,1,1,1,1,1,1,1,1,1,1,1,1,1,1,1,1,1,1,1,1,1,1,1,
1,1,1,1,1,1,1,1,1,1,1,1,1,1,1,1,1,1,1,1,1,1,1,1,1,1,1,1,1,1,1,1,1,1,1,1,
1,1,1,1,1,1,1,1,1,1,1,1,1,1,1,1,1,1,1,1,1,1,1,1,1,1,1,1,1,1,1,1,1,1,1,1,
1,1,1,1,1,1,1,1,1,1,1,1,1,1,1,1,1,1,1,1,1,1,1,1,1,1,1,1,1,1,1,1,1,1,1,1,
1,1,1,1,1,1,1,1,1,1,1,1,1,1,1,1,1,1,1,1,1,1,1,1,1,1,1,1,1,1,1,1,1,1,1,1,
1,1,1,1,1,1,1,1,1,1,1,6),(0.143172102,0.144954128,0.146788991,0.148623853,
0.150458716,0.152293578,0.15412844,0.155963303,0.157798165,0.159633028,
0.16146789,0.163302752,0.165137615,0.166972477,0.168807339,0.170642202,
0.172477064,0.174311927,0.176146789,0.177981651,0.179816514,0.181651376,
0.183486239,0.185321101,0.187155963,0.188990826,0.190825688,0.19266055,
0.194495413,0.196330275,0.198165138,0.2,0.201834862,0.203669725,0.205504587,
0.20733945,0.209174312,0.211009174,0.212844037,0.214678899,0.216513761,
0.218348624,0.220183486,0.222018349,0.223853211,0.225688073,0.227522936,
0.229357798,0.231192661,0.233027523,0.234862385,0.236697248,0.23853211,
0.240366972,0.242201835,0.244036697,0.24587156,0.247706422,0.249541284,
0.251376147,0.253211009,0.255045872,0.256880734,0.258715596,0.260550459,
0.262385321,0.264220183,0.266055046,0.267889908,0.269724771,0.271559633,
0.273394495,0.275229358,0.27706422,0.278899083,0.280733945,0.282568807,
0.28440367,0.286238532,0.288073394,0.289908257,0.291743119,0.293577982,
0.295412844,0.297247706,0.299082569,0.300917431,0.302752294,0.304587156,
0.306422018,0.308256881,0.310091743,0.311926606,0.313761468,0.31559633,
0.317431193,0.319266055,0.321100917,0.32293578,0.324770642,0.326605505,
0.328440367,0.330275229,0.332110092,0.333944954,0.335779817,0.337614679,
0.339449541,0.341284404,0.343119266,0.344954128,0.346788991,0.348623853,
0.350458716,0.352293578,0.35412844,0.355963303,0.357798165,0.359633028,
0.36146789,0.363302752,0.365137615,0.366972477,0.368807339,0.370642202,
0.372477064,0.374311927,0.376146789,0.377981651,0.379816514,0.381651376,
0.383486239,0.385321101,0.387155963,0.388990826,0.390825688,0.39266055,
0.394495413,0.396330275,0.398165138,0.4,0.401834862,0.403669725,0.405504587,
0.40733945,0.409174312,0.411009174,0.412844037,0.414678899,0.416513761,
0.418348624,0.420183486,0.422018349,0.423853211,0.425688073,0.427522936,
0.429357798,0.431192661,0.433027523,0.434862385,0.436697248,0.43853211,
0.440366972,0.442201835,0.444036697,0.44587156,0.447706422,0.449541284,
0.451376147,0.453211009,0.455045872,0.456880734,0.458715596,0.460550459,
0.462385321,0.464220183,0.466055046,0.467889908,0.469724771,0.471559633,
0.473394495,0.475229358,0.47706422,0.478899083,0.480733945,0.482568807,
0.48440367,0.486238532,0.488073394,0.489908257,0.491743119,0.493577982,
0.495412844,0.497247706,0.499082569,0.500917431,0.502752294,0.504587156,
0.506422018,0.508256881,0.510091743,0.511926606,0.513761468,0.51559633,
0.517431193,0.519266055,0.521100917,0.52293578,0.524770642,0.526605505,
0.528440367,0.530275229,0.532110092,0.533944954,0.535779817,0.537614679,
0.539449541,0.541284404,0.543119266,0.544954128,0.546788991,0.548623853,
0.550458716,0.552293578,0.55412844,0.555963303,0.557798165,0.559633028,
0.56146789,0.563302752,0.565137615,0.566972477,0.568807339,0.570642202,
0.572477064,0.574311927,0.576146789,0.577981651,0.579816514,0.581651376,
0.583486239,0.585321101,0.587155963,0.588990826,0.590825688,0.59266055,
0.594495413,0.596330275,0.598165138,0.6,0.601834862,0.603669725,0.605504587,
0.60733945,0.609174312,0.611009174,0.612844037,0.614678899,0.616513761,
0.618348624,0.620183486,0.622018349,0.623853211,0.625688073,0.627522936,
0.629357798,0.631192661,0.633027523,0.634862385,0.636697248,0.63853211,
0.640366972,0.642201835,0.644036697,0.64587156,0.647706422,0.649541284,
0.651376147,0.653211009,0.655045872,0.656880734,0.658715596,0.660550459,
0.662385321,0.664220183,0.666055046,0.667889908,0.669724771,0.671559633,
0.673394495,0.675229358,0.67706422,0.678899083,0.680733945,0.682568807,
0.68440367,0.686238532,0.688073394,0.689908257,0.691743119,0.693577982,
0.695412844,0.697247706,0.699082569,0.700917431,0.702752294,0.704587156,
0.706422018,0.708256881,0.710091743,0.711926606,0.713761468,0.71559633,
0.717431193,0.719266055,0.721100917,0.72293578,0.724770642,0.726605505,
0.728440367,0.730275229,0.732110092,0.733944954,0.735779817,0.737614679,
0.739449541,0.741284404,0.743119266,0.744954128,0.746788991,0.748623853,
0.750458716,0.752293578,0.75412844,0.755963303,0.757798165,0.759633028,
0.76146789,0.763302752,0.765137615,0.766972477,0.768807339,0.770642202,
0.772477064,0.774311927,0.776146789,0.777981651,0.779816514,0.781651376,
0.783486239,0.785321101,0.787155963,0.788990826,0.790825688,0.79266055,
0.794495413,0.796330275,0.798165138,0.8,0.801834862,0.803669725,0.805504587,
0.80733945,0.809174312,0.811009174,0.812844037,0.814678899,0.816513761,
0.818348624,0.820183486,0.822018349,0.823853211,0.825688073,0.827522936,
0.829357798,0.831192661,0.833027523,0.834862385,0.836697248,0.83853211,
0.840366972,0.842201835,0.844036697,0.84587156,0.847706422,0.849541284,
0.851376147,0.853211009,0.855045872,0.856880734,0.858715596,0.860550459,
0.862385321,0.864220183,0.866055046,0.867889908,0.869724771,0.871559633,
0.873394495,0.875229358,0.87706422,0.878899083,0.880733945,0.882568807,
0.88440367,0.886238532,0.888073394,0.889908257,0.891743119,0.893577982,
0.895412844,0.897247706,0.899082569,0.900917431,0.902752294,0.904587156,
0.906422018,0.908256881,0.910091743,0.911926606,0.913761468,0.91559633,
0.917431193,0.919266055,0.921100917,0.92293578,0.924770642,0.926605505,
0.928440367,0.930275229,0.932110092,0.933944954,0.935779817,0.937614679,
0.939449541,0.941284404,0.943119266,0.944954128,0.946788991,0.948623853,
0.950458716,0.952293578,0.95412844,0.955963303,0.957798165,0.959633028,
0.96146789,0.963302752,0.965137615,0.966972477,0.968807339,0.970642202,
0.972477064,0.974311927,0.976146789,0.977981651,0.979816514,0.981651376,
0.983486239,0.985321101,0.987155963,0.988990826,0.990825688,0.99266055,
0.994495413,0.996330275,0.998165138,1.),.UNSPECIFIED.);
#24327=B_SPLINE_CURVE_WITH_KNOTS('',3,(#161774,#161775,#161776,#161777,
#161778,#161779,#161780,#161781,#161782,#161783,#161784,#161785,#161786,
#161787,#161788,#161789,#161790,#161791,#161792,#161793,#161794,#161795,
#161796,#161797,#161798,#161799,#161800,#161801,#161802,#161803,#161804,
#161805,#161806,#161807,#161808,#161809,#161810,#161811,#161812,#161813,
#161814,#161815,#161816,#161817,#161818,#161819,#161820,#161821,#161822,
#161823,#161824,#161825,#161826,#161827,#161828,#161829,#161830,#161831,
#161832,#161833,#161834,#161835,#161836,#161837,#161838,#161839,#161840,
#161841,#161842,#161843,#161844,#161845,#161846,#161847,#161848,#161849,
#161850,#161851,#161852,#161853,#161854,#161855,#161856,#161857,#161858,
#161859,#161860,#161861,#161862,#161863,#161864,#161865,#161866,#161867,
#161868,#161869,#161870,#161871,#161872,#161873,#161874,#161875,#161876,
#161877,#161878,#161879,#161880,#161881,#161882,#161883,#161884,#161885,
#161886,#161887,#161888,#161889,#161890,#161891,#161892,#161893,#161894,
#161895,#161896,#161897,#161898,#161899,#161900,#161901,#161902,#161903,
#161904,#161905,#161906,#161907,#161908,#161909,#161910,#161911,#161912,
#161913,#161914,#161915,#161916,#161917,#161918,#161919,#161920,#161921,
#161922,#161923,#161924,#161925,#161926,#161927,#161928,#161929,#161930,
#161931,#161932,#161933,#161934,#161935,#161936,#161937,#161938,#161939,
#161940,#161941,#161942,#161943,#161944,#161945,#161946,#161947,#161948,
#161949,#161950,#161951,#161952,#161953,#161954,#161955,#161956,#161957,
#161958,#161959,#161960,#161961,#161962,#161963,#161964,#161965,#161966,
#161967,#161968,#161969,#161970,#161971,#161972,#161973,#161974,#161975,
#161976,#161977,#161978,#161979,#161980,#161981,#161982,#161983,#161984,
#161985,#161986,#161987,#161988,#161989,#161990,#161991,#161992,#161993,
#161994,#161995,#161996,#161997,#161998,#161999,#162000,#162001,#162002,
#162003,#162004,#162005,#162006,#162007,#162008,#162009,#162010,#162011,
#162012,#162013,#162014,#162015,#162016,#162017,#162018,#162019,#162020,
#162021,#162022,#162023,#162024,#162025,#162026,#162027,#162028,#162029,
#162030,#162031,#162032,#162033,#162034,#162035,#162036,#162037,#162038,
#162039,#162040,#162041,#162042,#162043,#162044,#162045,#162046,#162047,
#162048,#162049,#162050,#162051,#162052,#162053,#162054,#162055,#162056,
#162057,#162058,#162059,#162060,#162061,#162062,#162063,#162064,#162065,
#162066,#162067,#162068,#162069,#162070,#162071,#162072,#162073,#162074,
#162075,#162076,#162077,#162078,#162079,#162080,#162081,#162082,#162083,
#162084,#162085,#162086,#162087,#162088,#162089,#162090,#162091,#162092,
#162093,#162094,#162095,#162096,#162097,#162098,#162099,#162100,#162101,
#162102,#162103,#162104),.UNSPECIFIED.,.F.,.F.,(4,3,3,3,3,3,3,3,3,3,3,3,
3,3,3,3,3,3,3,3,3,3,3,3,3,3,3,3,3,3,3,3,3,3,3,3,3,3,3,3,3,3,3,3,3,3,3,3,
3,3,3,3,3,3,3,3,3,3,3,3,3,3,3,3,3,3,3,3,3,3,3,3,3,3,3,3,3,3,3,3,3,3,3,3,
3,3,3,3,3,3,3,3,3,3,3,3,3,3,3,3,3,3,3,3,3,3,3,3,3,3,4),(0.143172102,0.15412844,
0.165137615,0.176146789,0.187155963,0.198165138,0.209174312,0.220183486,
0.231192661,0.242201835,0.253211009,0.264220183,0.275229358,0.286238532,
0.297247706,0.308256881,0.319266055,0.330275229,0.341284404,0.352293578,
0.365137615,0.376146789,0.388990826,0.398165138,0.40733945,0.416513761,
0.425688073,0.434862385,0.444036697,0.453211009,0.462385321,0.471559633,
0.480733945,0.489908257,0.499082569,0.508256881,0.517431193,0.526605505,
0.533944954,0.541284404,0.548623853,0.555963303,0.563302752,0.570642202,
0.577981651,0.585321101,0.59266055,0.6,0.60733945,0.614678899,0.622018349,
0.629357798,0.636697248,0.644036697,0.651376147,0.658715596,0.666055046,
0.673394495,0.680733945,0.688073394,0.695412844,0.702752294,0.711926606,
0.719266055,0.726605505,0.733944954,0.741284404,0.748623853,0.755963303,
0.763302752,0.770642202,0.777981651,0.785321101,0.79266055,0.8,0.80733945,
0.812844037,0.818348624,0.823853211,0.829357798,0.834862385,0.840366972,
0.84587156,0.851376147,0.856880734,0.862385321,0.867889908,0.873394495,
0.878899083,0.88440367,0.889908257,0.895412844,0.900917431,0.906422018,
0.911926606,0.917431193,0.92293578,0.928440367,0.933944954,0.939449541,
0.944954128,0.950458716,0.955963303,0.96146789,0.966972477,0.972477064,
0.977981651,0.983486239,0.988990826,0.994495413,1.),.UNSPECIFIED.);
#24328=B_SPLINE_CURVE_WITH_KNOTS('',3,(#162105,#162106,#162107,#162108,
#162109,#162110,#162111,#162112,#162113,#162114,#162115,#162116,#162117,
#162118,#162119,#162120,#162121,#162122,#162123,#162124,#162125,#162126,
#162127,#162128,#162129,#162130,#162131,#162132,#162133,#162134,#162135,
#162136,#162137,#162138,#162139,#162140,#162141,#162142,#162143,#162144,
#162145,#162146,#162147,#162148,#162149,#162150,#162151,#162152,#162153,
#162154,#162155,#162156,#162157,#162158,#162159,#162160,#162161,#162162,
#162163,#162164,#162165,#162166,#162167,#162168,#162169,#162170,#162171,
#162172,#162173,#162174,#162175,#162176,#162177,#162178,#162179,#162180,
#162181,#162182,#162183,#162184,#162185,#162186,#162187,#162188,#162189,
#162190,#162191,#162192,#162193,#162194,#162195,#162196,#162197,#162198,
#162199,#162200,#162201,#162202,#162203,#162204,#162205,#162206,#162207,
#162208,#162209,#162210,#162211,#162212,#162213,#162214,#162215,#162216,
#162217,#162218,#162219,#162220,#162221,#162222,#162223,#162224,#162225,
#162226,#162227,#162228,#162229,#162230,#162231,#162232,#162233,#162234,
#162235,#162236,#162237,#162238,#162239,#162240,#162241,#162242,#162243,
#162244,#162245,#162246,#162247,#162248,#162249,#162250,#162251,#162252,
#162253,#162254,#162255,#162256,#162257,#162258,#162259,#162260,#162261,
#162262,#162263,#162264,#162265,#162266,#162267,#162268,#162269,#162270,
#162271,#162272,#162273,#162274,#162275,#162276,#162277,#162278,#162279,
#162280,#162281,#162282,#162283,#162284,#162285,#162286,#162287,#162288,
#162289,#162290,#162291,#162292,#162293,#162294,#162295,#162296,#162297,
#162298,#162299,#162300,#162301,#162302,#162303,#162304,#162305,#162306,
#162307,#162308,#162309,#162310,#162311,#162312,#162313,#162314,#162315,
#162316,#162317,#162318,#162319,#162320,#162321,#162322,#162323,#162324,
#162325,#162326,#162327,#162328,#162329,#162330,#162331,#162332,#162333,
#162334,#162335,#162336,#162337,#162338,#162339,#162340,#162341,#162342,
#162343,#162344,#162345,#162346,#162347,#162348,#162349,#162350,#162351,
#162352,#162353,#162354,#162355,#162356,#162357,#162358,#162359,#162360,
#162361,#162362,#162363,#162364,#162365,#162366,#162367,#162368,#162369,
#162370,#162371,#162372,#162373,#162374,#162375,#162376,#162377,#162378,
#162379,#162380,#162381,#162382,#162383,#162384,#162385,#162386,#162387,
#162388,#162389,#162390,#162391,#162392,#162393,#162394,#162395,#162396,
#162397,#162398,#162399,#162400,#162401,#162402,#162403,#162404,#162405,
#162406,#162407,#162408,#162409,#162410,#162411,#162412,#162413,#162414,
#162415,#162416,#162417,#162418,#162419,#162420,#162421,#162422,#162423,
#162424,#162425,#162426,#162427,#162428,#162429),.UNSPECIFIED.,.F.,.F.,
(4,3,3,3,3,3,3,3,3,3,3,3,3,3,3,3,3,3,3,3,3,3,3,3,3,3,3,3,3,3,3,3,3,3,3,
3,3,3,3,3,3,3,3,3,3,3,3,3,3,3,3,3,3,3,3,3,3,3,3,3,3,3,3,3,3,3,3,3,3,3,3,
3,3,3,3,3,3,3,3,3,3,3,3,3,3,3,3,3,3,3,3,3,3,3,3,3,3,3,3,3,3,3,3,3,3,3,3,
3,4),(0.143172102,0.15412844,0.165137615,0.176146789,0.187155963,0.198165138,
0.209174312,0.220183486,0.231192661,0.242201835,0.253211009,0.264220183,
0.275229358,0.286238532,0.297247706,0.308256881,0.319266055,0.330275229,
0.341284404,0.352293578,0.363302752,0.374311927,0.385321101,0.396330275,
0.405504587,0.414678899,0.423853211,0.433027523,0.442201835,0.451376147,
0.460550459,0.469724771,0.478899083,0.488073394,0.497247706,0.506422018,
0.51559633,0.524770642,0.533944954,0.543119266,0.550458716,0.557798165,
0.565137615,0.572477064,0.579816514,0.587155963,0.594495413,0.601834862,
0.609174312,0.616513761,0.623853211,0.631192661,0.63853211,0.64587156,0.653211009,
0.660550459,0.667889908,0.67706422,0.68440367,0.691743119,0.699082569,0.706422018,
0.713761468,0.721100917,0.728440367,0.735779817,0.743119266,0.750458716,
0.757798165,0.765137615,0.772477064,0.779816514,0.787155963,0.794495413,
0.803669725,0.811009174,0.816513761,0.822018349,0.827522936,0.833027523,
0.83853211,0.844036697,0.849541284,0.855045872,0.860550459,0.866055046,
0.871559633,0.87706422,0.882568807,0.888073394,0.893577982,0.899082569,
0.904587156,0.910091743,0.91559633,0.921100917,0.926605505,0.933944954,
0.939449541,0.944954128,0.950458716,0.955963303,0.96146789,0.968807339,
0.974311927,0.979816514,0.985321101,0.990825688,1.),.UNSPECIFIED.);
#24329=B_SPLINE_CURVE_WITH_KNOTS('',3,(#163377,#163378,#163379,#163380,
#163381,#163382,#163383,#163384,#163385,#163386,#163387,#163388,#163389,
#163390,#163391,#163392,#163393,#163394,#163395,#163396,#163397,#163398,
#163399,#163400,#163401,#163402,#163403,#163404,#163405,#163406,#163407,
#163408,#163409,#163410,#163411,#163412,#163413,#163414,#163415,#163416,
#163417,#163418,#163419,#163420,#163421,#163422,#163423,#163424,#163425,
#163426,#163427,#163428,#163429,#163430,#163431,#163432,#163433,#163434,
#163435,#163436,#163437,#163438,#163439,#163440,#163441,#163442,#163443,
#163444,#163445,#163446,#163447,#163448,#163449,#163450,#163451,#163452,
#163453,#163454,#163455,#163456,#163457,#163458,#163459,#163460,#163461,
#163462,#163463,#163464,#163465,#163466,#163467,#163468,#163469,#163470,
#163471,#163472,#163473,#163474,#163475,#163476,#163477,#163478,#163479,
#163480,#163481,#163482,#163483,#163484,#163485,#163486,#163487,#163488,
#163489,#163490,#163491,#163492,#163493,#163494,#163495,#163496,#163497,
#163498,#163499,#163500,#163501,#163502,#163503,#163504,#163505,#163506,
#163507,#163508,#163509,#163510,#163511,#163512,#163513,#163514,#163515,
#163516,#163517,#163518,#163519,#163520,#163521,#163522,#163523,#163524,
#163525,#163526,#163527,#163528,#163529,#163530,#163531,#163532,#163533,
#163534,#163535,#163536,#163537,#163538,#163539,#163540,#163541,#163542,
#163543,#163544,#163545,#163546,#163547,#163548,#163549,#163550,#163551,
#163552,#163553,#163554,#163555,#163556,#163557,#163558,#163559,#163560,
#163561,#163562,#163563,#163564,#163565,#163566,#163567,#163568,#163569,
#163570,#163571,#163572,#163573,#163574,#163575,#163576,#163577,#163578,
#163579,#163580,#163581,#163582,#163583,#163584,#163585,#163586,#163587,
#163588,#163589,#163590,#163591,#163592,#163593,#163594,#163595,#163596,
#163597,#163598,#163599,#163600,#163601,#163602,#163603,#163604,#163605,
#163606,#163607,#163608,#163609,#163610,#163611,#163612,#163613,#163614,
#163615,#163616,#163617,#163618,#163619,#163620,#163621,#163622,#163623,
#163624,#163625,#163626,#163627,#163628,#163629,#163630,#163631,#163632,
#163633,#163634,#163635,#163636,#163637,#163638,#163639,#163640,#163641,
#163642,#163643,#163644,#163645,#163646,#163647,#163648,#163649,#163650,
#163651,#163652,#163653,#163654,#163655,#163656,#163657,#163658,#163659,
#163660,#163661,#163662,#163663,#163664,#163665,#163666,#163667,#163668,
#163669,#163670,#163671,#163672,#163673,#163674,#163675,#163676,#163677,
#163678,#163679,#163680,#163681,#163682,#163683,#163684,#163685,#163686,
#163687,#163688,#163689,#163690,#163691,#163692,#163693,#163694,#163695,
#163696,#163697,#163698),.UNSPECIFIED.,.F.,.F.,(4,3,3,3,3,3,3,3,3,3,3,3,
3,3,3,3,3,3,3,3,3,3,3,3,3,3,3,3,3,3,3,3,3,3,3,3,3,3,3,3,3,3,3,3,3,3,3,3,
3,3,3,3,3,3,3,3,3,3,3,3,3,3,3,3,3,3,3,3,3,3,3,3,3,3,3,3,3,3,3,3,3,3,3,3,
3,3,3,3,3,3,3,3,3,3,3,3,3,3,3,3,3,3,3,3,3,3,3,4),(-1.,-0.994495413,-0.988990826,
-0.983486239,-0.977981651,-0.972477064,-0.965137615,-0.957798165,-0.952293578,
-0.946788991,-0.939449541,-0.933944954,-0.928440367,-0.92293578,-0.917431193,
-0.911926606,-0.906422018,-0.900917431,-0.895412844,-0.889908257,-0.88440367,
-0.87706422,-0.871559633,-0.866055046,-0.860550459,-0.855045872,-0.849541284,
-0.840366972,-0.834862385,-0.829357798,-0.823853211,-0.818348624,-0.812844037,
-0.80733945,-0.8,-0.79266055,-0.783486239,-0.776146789,-0.768807339,-0.76146789,
-0.75412844,-0.746788991,-0.739449541,-0.732110092,-0.724770642,-0.717431193,
-0.708256881,-0.700917431,-0.691743119,-0.68440367,-0.67706422,-0.669724771,
-0.662385321,-0.655045872,-0.647706422,-0.640366972,-0.633027523,-0.625688073,
-0.618348624,-0.611009174,-0.603669725,-0.596330275,-0.588990826,-0.579816514,
-0.572477064,-0.565137615,-0.557798165,-0.550458716,-0.543119266,-0.535779817,
-0.528440367,-0.519266055,-0.510091743,-0.499082569,-0.489908257,-0.480733945,
-0.471559633,-0.462385321,-0.453211009,-0.444036697,-0.434862385,-0.425688073,
-0.416513761,-0.40733945,-0.398165138,-0.388990826,-0.377981651,-0.366972477,
-0.355963303,-0.344954128,-0.333944954,-0.32293578,-0.311926606,-0.300917431,
-0.289908257,-0.278899083,-0.267889908,-0.256880734,-0.24587156,-0.234862385,
-0.223853211,-0.212844037,-0.201834862,-0.190825688,-0.179816514,-0.168807339,
-0.157798165,-0.143172102),.UNSPECIFIED.);
#24330=B_SPLINE_CURVE_WITH_KNOTS('',3,(#163699,#163700,#163701,#163702,
#163703,#163704,#163705,#163706,#163707,#163708,#163709,#163710,#163711,
#163712,#163713,#163714,#163715,#163716,#163717,#163718,#163719,#163720,
#163721,#163722,#163723,#163724,#163725,#163726,#163727,#163728,#163729,
#163730,#163731,#163732,#163733,#163734,#163735,#163736,#163737,#163738,
#163739,#163740,#163741,#163742,#163743,#163744,#163745,#163746,#163747,
#163748,#163749,#163750,#163751,#163752,#163753,#163754,#163755,#163756,
#163757,#163758,#163759,#163760,#163761,#163762,#163763,#163764,#163765,
#163766,#163767,#163768,#163769,#163770,#163771,#163772,#163773,#163774,
#163775,#163776,#163777,#163778,#163779,#163780,#163781,#163782,#163783,
#163784,#163785,#163786,#163787,#163788,#163789,#163790,#163791,#163792,
#163793,#163794,#163795,#163796,#163797,#163798,#163799,#163800,#163801,
#163802,#163803,#163804,#163805,#163806,#163807,#163808,#163809,#163810,
#163811,#163812,#163813,#163814,#163815,#163816,#163817,#163818,#163819,
#163820,#163821,#163822,#163823,#163824,#163825,#163826,#163827,#163828,
#163829,#163830,#163831,#163832,#163833,#163834,#163835,#163836,#163837,
#163838,#163839,#163840,#163841,#163842,#163843,#163844,#163845,#163846,
#163847,#163848,#163849,#163850,#163851,#163852,#163853,#163854,#163855,
#163856,#163857,#163858,#163859,#163860,#163861,#163862,#163863,#163864,
#163865,#163866,#163867,#163868,#163869,#163870,#163871,#163872,#163873,
#163874,#163875,#163876,#163877,#163878,#163879,#163880,#163881,#163882,
#163883,#163884,#163885,#163886,#163887,#163888,#163889,#163890,#163891,
#163892,#163893,#163894,#163895,#163896,#163897,#163898,#163899,#163900,
#163901,#163902,#163903,#163904,#163905,#163906,#163907,#163908,#163909,
#163910,#163911,#163912,#163913,#163914,#163915,#163916,#163917,#163918,
#163919,#163920,#163921,#163922,#163923,#163924,#163925,#163926,#163927,
#163928,#163929,#163930,#163931,#163932,#163933,#163934,#163935,#163936,
#163937,#163938,#163939,#163940,#163941,#163942,#163943,#163944,#163945,
#163946,#163947,#163948,#163949,#163950,#163951,#163952,#163953,#163954,
#163955,#163956,#163957,#163958,#163959,#163960,#163961,#163962,#163963,
#163964,#163965,#163966,#163967,#163968,#163969,#163970,#163971,#163972,
#163973,#163974,#163975,#163976,#163977,#163978,#163979,#163980,#163981,
#163982,#163983,#163984,#163985,#163986,#163987,#163988,#163989,#163990,
#163991,#163992,#163993,#163994,#163995,#163996,#163997,#163998,#163999,
#164000,#164001,#164002,#164003,#164004,#164005,#164006,#164007,#164008,
#164009,#164010,#164011,#164012,#164013,#164014),.UNSPECIFIED.,.F.,.F.,
(4,3,3,3,3,3,3,3,3,3,3,3,3,3,3,3,3,3,3,3,3,3,3,3,3,3,3,3,3,3,3,3,3,3,3,
3,3,3,3,3,3,3,3,3,3,3,3,3,3,3,3,3,3,3,3,3,3,3,3,3,3,3,3,3,3,3,3,3,3,3,3,
3,3,3,3,3,3,3,3,3,3,3,3,3,3,3,3,3,3,3,3,3,3,3,3,3,3,3,3,3,3,3,3,3,3,4),
(0.143172102,0.15412844,0.165137615,0.176146789,0.187155963,0.198165138,
0.209174312,0.220183486,0.231192661,0.242201835,0.255045872,0.266055046,
0.27706422,0.288073394,0.299082569,0.310091743,0.321100917,0.332110092,
0.343119266,0.35412844,0.365137615,0.376146789,0.387155963,0.396330275,
0.405504587,0.414678899,0.423853211,0.433027523,0.442201835,0.451376147,
0.460550459,0.469724771,0.478899083,0.488073394,0.497247706,0.506422018,
0.51559633,0.524770642,0.533944954,0.541284404,0.548623853,0.557798165,
0.565137615,0.572477064,0.579816514,0.588990826,0.596330275,0.603669725,
0.611009174,0.618348624,0.625688073,0.633027523,0.640366972,0.647706422,
0.655045872,0.662385321,0.671559633,0.678899083,0.686238532,0.693577982,
0.700917431,0.710091743,0.717431193,0.724770642,0.733944954,0.743119266,
0.750458716,0.757798165,0.766972477,0.776146789,0.783486239,0.790825688,
0.798165138,0.805504587,0.811009174,0.820183486,0.825688073,0.831192661,
0.840366972,0.84587156,0.853211009,0.858715596,0.864220183,0.869724771,
0.87706422,0.882568807,0.888073394,0.893577982,0.900917431,0.906422018,
0.911926606,0.919266055,0.924770642,0.930275229,0.935779817,0.941284404,
0.946788991,0.952293578,0.957798165,0.963302752,0.968807339,0.974311927,
0.979816514,0.985321101,0.990825688,1.),.UNSPECIFIED.);
#24331=B_SPLINE_CURVE_WITH_KNOTS('',3,(#164977,#164978,#164979,#164980,
#164981,#164982,#164983,#164984,#164985,#164986,#164987,#164988,#164989,
#164990,#164991,#164992,#164993,#164994,#164995,#164996,#164997,#164998,
#164999,#165000,#165001,#165002,#165003,#165004,#165005,#165006,#165007,
#165008,#165009,#165010,#165011,#165012,#165013,#165014,#165015,#165016,
#165017,#165018,#165019,#165020,#165021,#165022,#165023,#165024,#165025,
#165026,#165027,#165028,#165029,#165030,#165031,#165032,#165033,#165034,
#165035,#165036,#165037,#165038,#165039,#165040,#165041,#165042,#165043,
#165044,#165045,#165046,#165047,#165048,#165049,#165050,#165051,#165052,
#165053,#165054,#165055,#165056,#165057,#165058,#165059,#165060,#165061,
#165062,#165063,#165064,#165065,#165066,#165067,#165068,#165069,#165070,
#165071,#165072,#165073,#165074,#165075,#165076,#165077,#165078,#165079,
#165080,#165081,#165082,#165083,#165084,#165085,#165086,#165087,#165088,
#165089,#165090,#165091,#165092,#165093,#165094,#165095,#165096,#165097,
#165098,#165099,#165100,#165101,#165102,#165103,#165104,#165105,#165106,
#165107,#165108,#165109,#165110,#165111,#165112,#165113,#165114,#165115,
#165116,#165117,#165118,#165119,#165120,#165121,#165122,#165123,#165124,
#165125,#165126,#165127,#165128,#165129,#165130,#165131,#165132,#165133,
#165134,#165135,#165136,#165137,#165138,#165139,#165140,#165141,#165142,
#165143,#165144,#165145,#165146,#165147,#165148,#165149,#165150,#165151,
#165152,#165153,#165154,#165155,#165156,#165157,#165158,#165159,#165160,
#165161,#165162,#165163,#165164,#165165,#165166,#165167,#165168,#165169,
#165170,#165171,#165172,#165173,#165174,#165175,#165176,#165177,#165178,
#165179,#165180,#165181,#165182,#165183,#165184,#165185,#165186,#165187,
#165188,#165189,#165190,#165191,#165192,#165193,#165194,#165195,#165196,
#165197,#165198,#165199,#165200,#165201,#165202,#165203,#165204,#165205,
#165206,#165207,#165208,#165209,#165210,#165211,#165212,#165213,#165214,
#165215,#165216,#165217,#165218,#165219,#165220,#165221,#165222,#165223,
#165224,#165225,#165226,#165227,#165228,#165229,#165230,#165231,#165232,
#165233,#165234,#165235,#165236,#165237,#165238,#165239,#165240,#165241,
#165242,#165243,#165244,#165245,#165246,#165247,#165248,#165249,#165250,
#165251,#165252,#165253,#165254,#165255,#165256,#165257,#165258,#165259,
#165260,#165261,#165262,#165263,#165264,#165265,#165266,#165267,#165268,
#165269,#165270,#165271,#165272,#165273,#165274,#165275,#165276,#165277,
#165278,#165279,#165280,#165281,#165282,#165283,#165284,#165285,#165286,
#165287,#165288,#165289,#165290,#165291,#165292,#165293,#165294,#165295,
#165296,#165297,#165298,#165299,#165300,#165301),.UNSPECIFIED.,.F.,.F.,
(4,3,3,3,3,3,3,3,3,3,3,3,3,3,3,3,3,3,3,3,3,3,3,3,3,3,3,3,3,3,3,3,3,3,3,
3,3,3,3,3,3,3,3,3,3,3,3,3,3,3,3,3,3,3,3,3,3,3,3,3,3,3,3,3,3,3,3,3,3,3,3,
3,3,3,3,3,3,3,3,3,3,3,3,3,3,3,3,3,3,3,3,3,3,3,3,3,3,3,3,3,3,3,3,3,3,3,3,
3,4),(-1.,-0.994495413,-0.988990826,-0.981651376,-0.976146789,-0.968807339,
-0.963302752,-0.957798165,-0.952293578,-0.946788991,-0.941284404,-0.935779817,
-0.930275229,-0.924770642,-0.919266055,-0.913761468,-0.908256881,-0.900917431,
-0.895412844,-0.889908257,-0.88440367,-0.878899083,-0.873394495,-0.867889908,
-0.862385321,-0.856880734,-0.851376147,-0.84587156,-0.840366972,-0.834862385,
-0.829357798,-0.823853211,-0.818348624,-0.812844037,-0.80733945,-0.8,-0.79266055,
-0.783486239,-0.776146789,-0.768807339,-0.76146789,-0.75412844,-0.746788991,
-0.739449541,-0.732110092,-0.724770642,-0.717431193,-0.708256881,-0.700917431,
-0.693577982,-0.686238532,-0.678899083,-0.671559633,-0.664220183,-0.656880734,
-0.649541284,-0.642201835,-0.634862385,-0.627522936,-0.620183486,-0.612844037,
-0.605504587,-0.598165138,-0.590825688,-0.583486239,-0.576146789,-0.568807339,
-0.56146789,-0.55412844,-0.546788991,-0.539449541,-0.532110092,-0.52293578,
-0.513761468,-0.504587156,-0.495412844,-0.486238532,-0.47706422,-0.467889908,
-0.458715596,-0.449541284,-0.440366972,-0.431192661,-0.422018349,-0.412844037,
-0.403669725,-0.394495413,-0.383486239,-0.372477064,-0.36146789,-0.350458716,
-0.339449541,-0.328440367,-0.31559633,-0.304587156,-0.293577982,-0.282568807,
-0.271559633,-0.258715596,-0.247706422,-0.236697248,-0.225688073,-0.214678899,
-0.203669725,-0.19266055,-0.181651376,-0.170642202,-0.159633028,-0.143172102),
 .UNSPECIFIED.);
#24332=B_SPLINE_CURVE_WITH_KNOTS('',3,(#165302,#165303,#165304,#165305,
#165306,#165307,#165308,#165309,#165310,#165311,#165312,#165313,#165314,
#165315,#165316,#165317,#165318,#165319,#165320,#165321,#165322,#165323,
#165324,#165325,#165326,#165327,#165328,#165329,#165330,#165331,#165332,
#165333,#165334,#165335,#165336,#165337,#165338,#165339,#165340,#165341,
#165342,#165343,#165344,#165345,#165346,#165347,#165348,#165349,#165350,
#165351,#165352,#165353,#165354,#165355,#165356,#165357,#165358,#165359,
#165360,#165361,#165362,#165363,#165364,#165365,#165366,#165367,#165368,
#165369,#165370,#165371,#165372,#165373,#165374,#165375,#165376,#165377,
#165378,#165379,#165380,#165381,#165382,#165383,#165384,#165385,#165386,
#165387,#165388,#165389,#165390,#165391,#165392,#165393,#165394,#165395,
#165396,#165397,#165398,#165399,#165400,#165401,#165402,#165403,#165404,
#165405,#165406,#165407,#165408,#165409,#165410,#165411,#165412,#165413,
#165414,#165415,#165416,#165417,#165418,#165419,#165420,#165421,#165422,
#165423,#165424,#165425,#165426,#165427,#165428,#165429,#165430,#165431,
#165432,#165433,#165434,#165435,#165436,#165437,#165438,#165439,#165440,
#165441,#165442,#165443,#165444,#165445,#165446,#165447,#165448,#165449,
#165450,#165451,#165452,#165453,#165454,#165455,#165456,#165457,#165458,
#165459,#165460,#165461,#165462,#165463,#165464,#165465,#165466,#165467,
#165468,#165469,#165470,#165471,#165472,#165473,#165474,#165475,#165476,
#165477,#165478,#165479,#165480,#165481,#165482,#165483,#165484,#165485,
#165486,#165487,#165488,#165489,#165490,#165491,#165492,#165493,#165494,
#165495,#165496,#165497,#165498,#165499,#165500,#165501,#165502,#165503,
#165504,#165505,#165506,#165507,#165508,#165509,#165510,#165511,#165512,
#165513,#165514,#165515,#165516,#165517,#165518,#165519,#165520,#165521,
#165522,#165523,#165524,#165525,#165526,#165527,#165528,#165529,#165530,
#165531,#165532,#165533,#165534,#165535,#165536,#165537,#165538,#165539,
#165540,#165541,#165542,#165543,#165544,#165545,#165546,#165547,#165548,
#165549,#165550,#165551,#165552,#165553,#165554,#165555,#165556,#165557,
#165558,#165559,#165560,#165561,#165562,#165563,#165564,#165565,#165566,
#165567,#165568,#165569,#165570,#165571,#165572,#165573,#165574,#165575,
#165576,#165577,#165578,#165579,#165580,#165581,#165582,#165583,#165584,
#165585,#165586,#165587,#165588,#165589,#165590,#165591,#165592,#165593,
#165594,#165595,#165596,#165597,#165598,#165599,#165600,#165601,#165602,
#165603,#165604,#165605,#165606,#165607,#165608,#165609,#165610,#165611,
#165612,#165613,#165614,#165615,#165616,#165617,#165618,#165619,#165620,
#165621,#165622,#165623,#165624,#165625,#165626),.UNSPECIFIED.,.F.,.F.,
(4,3,3,3,3,3,3,3,3,3,3,3,3,3,3,3,3,3,3,3,3,3,3,3,3,3,3,3,3,3,3,3,3,3,3,
3,3,3,3,3,3,3,3,3,3,3,3,3,3,3,3,3,3,3,3,3,3,3,3,3,3,3,3,3,3,3,3,3,3,3,3,
3,3,3,3,3,3,3,3,3,3,3,3,3,3,3,3,3,3,3,3,3,3,3,3,3,3,3,3,3,3,3,3,3,3,3,3,
3,4),(0.143172102,0.15412844,0.165137615,0.176146789,0.187155963,0.198165138,
0.209174312,0.220183486,0.231192661,0.242201835,0.256880734,0.267889908,
0.278899083,0.289908257,0.300917431,0.311926606,0.32293578,0.333944954,
0.344954128,0.355963303,0.366972477,0.377981651,0.388990826,0.398165138,
0.40733945,0.416513761,0.425688073,0.434862385,0.444036697,0.453211009,
0.462385321,0.471559633,0.480733945,0.489908257,0.499082569,0.510091743,
0.519266055,0.528440367,0.535779817,0.543119266,0.550458716,0.557798165,
0.565137615,0.572477064,0.579816514,0.587155963,0.594495413,0.601834862,
0.609174312,0.616513761,0.623853211,0.631192661,0.63853211,0.64587156,0.653211009,
0.660550459,0.667889908,0.675229358,0.682568807,0.689908257,0.697247706,
0.704587156,0.711926606,0.719266055,0.726605505,0.733944954,0.741284404,
0.748623853,0.755963303,0.763302752,0.772477064,0.779816514,0.787155963,
0.794495413,0.801834862,0.809174312,0.814678899,0.820183486,0.825688073,
0.831192661,0.840366972,0.84587156,0.851376147,0.856880734,0.862385321,
0.867889908,0.873394495,0.878899083,0.88440367,0.891743119,0.897247706,
0.902752294,0.908256881,0.913761468,0.919266055,0.924770642,0.930275229,
0.935779817,0.941284404,0.946788991,0.952293578,0.957798165,0.963302752,
0.968807339,0.974311927,0.981651376,0.987155963,0.99266055,1.),
 .UNSPECIFIED.);
#24333=B_SPLINE_CURVE_WITH_KNOTS('',3,(#166571,#166572,#166573,#166574,
#166575,#166576,#166577,#166578,#166579,#166580,#166581,#166582,#166583,
#166584,#166585,#166586,#166587,#166588,#166589,#166590,#166591,#166592,
#166593,#166594,#166595,#166596,#166597,#166598,#166599,#166600,#166601,
#166602,#166603,#166604,#166605,#166606,#166607,#166608,#166609,#166610,
#166611,#166612,#166613,#166614,#166615,#166616,#166617,#166618,#166619,
#166620,#166621,#166622,#166623,#166624,#166625,#166626,#166627,#166628,
#166629,#166630,#166631,#166632,#166633,#166634,#166635,#166636,#166637,
#166638,#166639,#166640,#166641,#166642,#166643,#166644,#166645,#166646,
#166647,#166648,#166649,#166650,#166651,#166652,#166653,#166654,#166655,
#166656,#166657,#166658,#166659,#166660,#166661,#166662,#166663,#166664,
#166665,#166666,#166667,#166668,#166669,#166670,#166671,#166672,#166673,
#166674,#166675,#166676,#166677,#166678,#166679,#166680,#166681,#166682,
#166683,#166684,#166685,#166686,#166687,#166688,#166689,#166690,#166691,
#166692,#166693,#166694,#166695,#166696,#166697,#166698,#166699,#166700,
#166701,#166702,#166703,#166704,#166705,#166706,#166707,#166708,#166709,
#166710,#166711,#166712,#166713,#166714,#166715,#166716,#166717,#166718,
#166719,#166720,#166721,#166722,#166723,#166724,#166725,#166726,#166727,
#166728,#166729,#166730,#166731,#166732,#166733,#166734,#166735,#166736,
#166737,#166738,#166739,#166740,#166741,#166742,#166743,#166744,#166745,
#166746,#166747,#166748,#166749,#166750,#166751,#166752,#166753,#166754,
#166755,#166756,#166757,#166758,#166759,#166760,#166761,#166762,#166763,
#166764,#166765,#166766,#166767,#166768,#166769,#166770,#166771,#166772,
#166773,#166774,#166775,#166776,#166777,#166778,#166779,#166780,#166781,
#166782,#166783,#166784,#166785,#166786,#166787,#166788,#166789,#166790,
#166791,#166792,#166793,#166794,#166795,#166796,#166797,#166798,#166799,
#166800,#166801,#166802,#166803,#166804,#166805,#166806,#166807,#166808,
#166809,#166810,#166811,#166812,#166813,#166814,#166815,#166816,#166817,
#166818,#166819,#166820,#166821,#166822,#166823,#166824,#166825,#166826,
#166827,#166828,#166829,#166830,#166831,#166832,#166833,#166834,#166835,
#166836,#166837,#166838,#166839,#166840,#166841,#166842,#166843,#166844,
#166845,#166846,#166847,#166848,#166849,#166850,#166851,#166852,#166853,
#166854,#166855,#166856,#166857,#166858,#166859,#166860,#166861,#166862,
#166863,#166864,#166865,#166866,#166867,#166868,#166869,#166870,#166871,
#166872,#166873,#166874,#166875,#166876,#166877,#166878,#166879,#166880,
#166881,#166882,#166883,#166884,#166885,#166886,#166887,#166888,#166889,
#166890,#166891,#166892),.UNSPECIFIED.,.F.,.F.,(4,3,3,3,3,3,3,3,3,3,3,3,
3,3,3,3,3,3,3,3,3,3,3,3,3,3,3,3,3,3,3,3,3,3,3,3,3,3,3,3,3,3,3,3,3,3,3,3,
3,3,3,3,3,3,3,3,3,3,3,3,3,3,3,3,3,3,3,3,3,3,3,3,3,3,3,3,3,3,3,3,3,3,3,3,
3,3,3,3,3,3,3,3,3,3,3,3,3,3,3,3,3,3,3,3,3,3,3,4),(0.143172102,0.15412844,
0.165137615,0.176146789,0.187155963,0.198165138,0.209174312,0.220183486,
0.231192661,0.242201835,0.253211009,0.264220183,0.275229358,0.286238532,
0.299082569,0.310091743,0.321100917,0.332110092,0.343119266,0.35412844,
0.365137615,0.376146789,0.387155963,0.398165138,0.40733945,0.416513761,
0.425688073,0.436697248,0.44587156,0.455045872,0.464220183,0.473394495,
0.482568807,0.495412844,0.504587156,0.513761468,0.52293578,0.532110092,
0.539449541,0.546788991,0.55412844,0.56146789,0.568807339,0.576146789,0.583486239,
0.590825688,0.598165138,0.60733945,0.614678899,0.622018349,0.631192661,
0.63853211,0.64587156,0.653211009,0.660550459,0.669724771,0.678899083,0.686238532,
0.693577982,0.702752294,0.710091743,0.717431193,0.724770642,0.732110092,
0.741284404,0.748623853,0.755963303,0.763302752,0.770642202,0.777981651,
0.785321101,0.79266055,0.8,0.80733945,0.812844037,0.818348624,0.823853211,
0.829357798,0.834862385,0.840366972,0.84587156,0.851376147,0.856880734,
0.862385321,0.869724771,0.875229358,0.880733945,0.886238532,0.891743119,
0.897247706,0.902752294,0.908256881,0.913761468,0.919266055,0.924770642,
0.932110092,0.937614679,0.943119266,0.948623853,0.95412844,0.959633028,
0.965137615,0.970642202,0.976146789,0.981651376,0.987155963,0.99266055,
1.),.UNSPECIFIED.);
#24334=B_SPLINE_CURVE_WITH_KNOTS('',3,(#166893,#166894,#166895,#166896,
#166897,#166898,#166899,#166900,#166901,#166902,#166903,#166904,#166905,
#166906,#166907,#166908,#166909,#166910,#166911,#166912,#166913,#166914,
#166915,#166916,#166917,#166918,#166919,#166920,#166921,#166922,#166923,
#166924,#166925,#166926,#166927,#166928,#166929,#166930,#166931,#166932,
#166933,#166934,#166935,#166936,#166937,#166938,#166939,#166940,#166941,
#166942,#166943,#166944,#166945,#166946,#166947,#166948,#166949,#166950,
#166951,#166952,#166953,#166954,#166955,#166956,#166957,#166958,#166959,
#166960,#166961,#166962,#166963,#166964,#166965,#166966,#166967,#166968,
#166969,#166970,#166971,#166972,#166973,#166974,#166975,#166976,#166977,
#166978,#166979,#166980,#166981,#166982,#166983,#166984,#166985,#166986,
#166987,#166988,#166989,#166990,#166991,#166992,#166993,#166994,#166995,
#166996,#166997,#166998,#166999,#167000,#167001,#167002,#167003,#167004,
#167005,#167006,#167007,#167008,#167009,#167010,#167011,#167012,#167013,
#167014,#167015,#167016,#167017,#167018,#167019,#167020,#167021,#167022,
#167023,#167024,#167025,#167026,#167027,#167028,#167029,#167030,#167031,
#167032,#167033,#167034,#167035,#167036,#167037,#167038,#167039,#167040,
#167041,#167042,#167043,#167044,#167045,#167046,#167047,#167048,#167049,
#167050,#167051,#167052,#167053,#167054,#167055,#167056,#167057,#167058,
#167059,#167060,#167061,#167062,#167063,#167064,#167065,#167066,#167067,
#167068,#167069,#167070,#167071,#167072,#167073,#167074,#167075,#167076,
#167077,#167078,#167079,#167080,#167081,#167082,#167083,#167084,#167085,
#167086,#167087,#167088,#167089,#167090,#167091,#167092,#167093,#167094,
#167095,#167096,#167097,#167098,#167099,#167100,#167101,#167102,#167103,
#167104,#167105,#167106,#167107,#167108,#167109,#167110,#167111,#167112,
#167113,#167114,#167115,#167116,#167117,#167118,#167119,#167120,#167121,
#167122,#167123,#167124,#167125,#167126,#167127,#167128,#167129,#167130,
#167131,#167132,#167133,#167134,#167135,#167136,#167137,#167138,#167139,
#167140,#167141,#167142,#167143,#167144,#167145,#167146,#167147,#167148,
#167149,#167150,#167151,#167152,#167153,#167154,#167155,#167156,#167157,
#167158,#167159,#167160,#167161,#167162,#167163,#167164,#167165,#167166,
#167167,#167168,#167169,#167170,#167171,#167172,#167173,#167174,#167175,
#167176,#167177,#167178,#167179,#167180,#167181,#167182,#167183,#167184,
#167185,#167186,#167187,#167188,#167189,#167190,#167191,#167192,#167193,
#167194,#167195,#167196,#167197,#167198,#167199,#167200,#167201,#167202,
#167203,#167204,#167205,#167206,#167207,#167208,#167209,#167210,#167211,
#167212,#167213,#167214),.UNSPECIFIED.,.F.,.F.,(4,3,3,3,3,3,3,3,3,3,3,3,
3,3,3,3,3,3,3,3,3,3,3,3,3,3,3,3,3,3,3,3,3,3,3,3,3,3,3,3,3,3,3,3,3,3,3,3,
3,3,3,3,3,3,3,3,3,3,3,3,3,3,3,3,3,3,3,3,3,3,3,3,3,3,3,3,3,3,3,3,3,3,3,3,
3,3,3,3,3,3,3,3,3,3,3,3,3,3,3,3,3,3,3,3,3,3,3,4),(0.143172102,0.15412844,
0.165137615,0.176146789,0.187155963,0.198165138,0.209174312,0.220183486,
0.231192661,0.242201835,0.253211009,0.264220183,0.275229358,0.286238532,
0.299082569,0.310091743,0.321100917,0.332110092,0.343119266,0.35412844,
0.365137615,0.376146789,0.387155963,0.396330275,0.405504587,0.414678899,
0.423853211,0.433027523,0.442201835,0.451376147,0.460550459,0.469724771,
0.478899083,0.488073394,0.499082569,0.508256881,0.517431193,0.526605505,
0.533944954,0.541284404,0.550458716,0.557798165,0.565137615,0.572477064,
0.579816514,0.587155963,0.594495413,0.601834862,0.609174312,0.616513761,
0.623853211,0.631192661,0.63853211,0.64587156,0.653211009,0.660550459,0.667889908,
0.67706422,0.68440367,0.691743119,0.700917431,0.710091743,0.717431193,0.724770642,
0.732110092,0.739449541,0.746788991,0.75412844,0.76146789,0.770642202,0.777981651,
0.785321101,0.794495413,0.801834862,0.809174312,0.814678899,0.820183486,
0.825688073,0.831192661,0.836697248,0.842201835,0.847706422,0.853211009,
0.858715596,0.866055046,0.871559633,0.87706422,0.882568807,0.888073394,
0.893577982,0.900917431,0.906422018,0.911926606,0.919266055,0.924770642,
0.930275229,0.935779817,0.941284404,0.946788991,0.952293578,0.959633028,
0.965137615,0.970642202,0.976146789,0.981651376,0.987155963,0.994495413,
1.),.UNSPECIFIED.);
#24335=B_SPLINE_CURVE_WITH_KNOTS('',5,(#168174,#168175,#168176,#168177,
#168178,#168179,#168180,#168181,#168182,#168183,#168184,#168185,#168186,
#168187,#168188,#168189,#168190,#168191,#168192,#168193,#168194,#168195,
#168196,#168197,#168198,#168199,#168200,#168201,#168202,#168203,#168204,
#168205,#168206,#168207,#168208,#168209,#168210,#168211,#168212,#168213,
#168214,#168215,#168216,#168217,#168218,#168219,#168220,#168221,#168222,
#168223,#168224,#168225,#168226,#168227,#168228,#168229,#168230,#168231,
#168232,#168233,#168234,#168235,#168236,#168237,#168238,#168239,#168240,
#168241,#168242,#168243,#168244,#168245,#168246,#168247,#168248,#168249,
#168250,#168251,#168252,#168253,#168254,#168255,#168256,#168257,#168258,
#168259,#168260,#168261,#168262,#168263,#168264,#168265,#168266,#168267,
#168268,#168269,#168270,#168271,#168272,#168273,#168274,#168275,#168276,
#168277,#168278,#168279,#168280,#168281,#168282,#168283,#168284,#168285,
#168286,#168287,#168288,#168289,#168290,#168291,#168292,#168293,#168294,
#168295,#168296,#168297,#168298,#168299,#168300,#168301,#168302,#168303,
#168304,#168305,#168306,#168307,#168308,#168309,#168310,#168311,#168312,
#168313,#168314,#168315,#168316,#168317,#168318,#168319,#168320,#168321,
#168322,#168323,#168324,#168325,#168326,#168327,#168328,#168329,#168330,
#168331,#168332,#168333,#168334,#168335,#168336,#168337,#168338,#168339,
#168340,#168341,#168342,#168343,#168344,#168345,#168346,#168347,#168348,
#168349,#168350,#168351,#168352,#168353,#168354,#168355,#168356,#168357,
#168358,#168359,#168360,#168361,#168362,#168363,#168364,#168365,#168366,
#168367,#168368,#168369,#168370,#168371,#168372,#168373,#168374,#168375,
#168376,#168377,#168378,#168379,#168380,#168381,#168382,#168383,#168384,
#168385,#168386,#168387,#168388,#168389,#168390,#168391,#168392,#168393,
#168394,#168395,#168396,#168397,#168398,#168399,#168400,#168401,#168402,
#168403,#168404,#168405,#168406,#168407,#168408,#168409,#168410,#168411,
#168412,#168413,#168414,#168415,#168416,#168417,#168418,#168419,#168420,
#168421,#168422,#168423,#168424,#168425,#168426,#168427,#168428,#168429,
#168430,#168431,#168432,#168433,#168434,#168435,#168436,#168437,#168438,
#168439,#168440,#168441,#168442,#168443,#168444,#168445,#168446,#168447,
#168448,#168449,#168450,#168451,#168452,#168453,#168454,#168455,#168456,
#168457,#168458,#168459,#168460,#168461,#168462,#168463,#168464,#168465,
#168466,#168467,#168468,#168469,#168470,#168471,#168472,#168473,#168474,
#168475,#168476,#168477,#168478,#168479,#168480,#168481,#168482,#168483,
#168484,#168485,#168486,#168487,#168488,#168489,#168490,#168491,#168492,
#168493,#168494,#168495,#168496,#168497,#168498,#168499,#168500,#168501,
#168502,#168503,#168504,#168505,#168506,#168507,#168508,#168509,#168510,
#168511,#168512,#168513,#168514,#168515,#168516,#168517,#168518,#168519,
#168520,#168521,#168522,#168523,#168524,#168525,#168526,#168527,#168528,
#168529,#168530,#168531,#168532,#168533,#168534,#168535,#168536,#168537,
#168538,#168539,#168540,#168541,#168542,#168543,#168544,#168545,#168546,
#168547,#168548,#168549,#168550,#168551,#168552,#168553,#168554,#168555,
#168556,#168557,#168558,#168559,#168560,#168561,#168562,#168563,#168564,
#168565,#168566,#168567,#168568,#168569,#168570,#168571,#168572,#168573,
#168574,#168575,#168576,#168577,#168578,#168579,#168580,#168581,#168582,
#168583,#168584,#168585,#168586,#168587,#168588,#168589,#168590,#168591,
#168592,#168593,#168594,#168595,#168596,#168597,#168598,#168599,#168600,
#168601,#168602,#168603,#168604,#168605,#168606,#168607,#168608,#168609,
#168610,#168611,#168612,#168613,#168614,#168615,#168616,#168617,#168618,
#168619,#168620,#168621,#168622,#168623,#168624,#168625,#168626,#168627,
#168628,#168629,#168630,#168631,#168632,#168633,#168634,#168635,#168636,
#168637,#168638,#168639,#168640,#168641,#168642,#168643,#168644,#168645),
 .UNSPECIFIED.,.F.,.F.,(6,1,1,1,1,1,1,1,1,1,1,1,1,1,1,1,1,1,1,1,1,1,1,1,
1,1,1,1,1,1,1,1,1,1,1,1,1,1,1,1,1,1,1,1,1,1,1,1,1,1,1,1,1,1,1,1,1,1,1,1,
1,1,1,1,1,1,1,1,1,1,1,1,1,1,1,1,1,1,1,1,1,1,1,1,1,1,1,1,1,1,1,1,1,1,1,1,
1,1,1,1,1,1,1,1,1,1,1,1,1,1,1,1,1,1,1,1,1,1,1,1,1,1,1,1,1,1,1,1,1,1,1,1,
1,1,1,1,1,1,1,1,1,1,1,1,1,1,1,1,1,1,1,1,1,1,1,1,1,1,1,1,1,1,1,1,1,1,1,1,
1,1,1,1,1,1,1,1,1,1,1,1,1,1,1,1,1,1,1,1,1,1,1,1,1,1,1,1,1,1,1,1,1,1,1,1,
1,1,1,1,1,1,1,1,1,1,1,1,1,1,1,1,1,1,1,1,1,1,1,1,1,1,1,1,1,1,1,1,1,1,1,1,
1,1,1,1,1,1,1,1,1,1,1,1,1,1,1,1,1,1,1,1,1,1,1,1,1,1,1,1,1,1,1,1,1,1,1,1,
1,1,1,1,1,1,1,1,1,1,1,1,1,1,1,1,1,1,1,1,1,1,1,1,1,1,1,1,1,1,1,1,1,1,1,1,
1,1,1,1,1,1,1,1,1,1,1,1,1,1,1,1,1,1,1,1,1,1,1,1,1,1,1,1,1,1,1,1,1,1,1,1,
1,1,1,1,1,1,1,1,1,1,1,1,1,1,1,1,1,1,1,1,1,1,1,1,1,1,1,1,1,1,1,1,1,1,1,1,
1,1,1,1,1,1,1,1,1,1,1,1,1,1,1,1,1,1,1,1,1,1,1,1,1,1,1,1,1,1,1,1,1,1,1,1,
1,1,1,1,1,1,1,1,1,1,1,1,1,1,1,1,1,1,1,1,1,1,1,1,1,1,1,1,1,1,1,1,1,1,1,1,
1,1,1,1,1,1,1,1,1,1,1,6),(0.143172102,0.144954128,0.146788991,0.148623853,
0.150458716,0.152293578,0.15412844,0.155963303,0.157798165,0.159633028,
0.16146789,0.163302752,0.165137615,0.166972477,0.168807339,0.170642202,
0.172477064,0.174311927,0.176146789,0.177981651,0.179816514,0.181651376,
0.183486239,0.185321101,0.187155963,0.188990826,0.190825688,0.19266055,
0.194495413,0.196330275,0.198165138,0.2,0.201834862,0.203669725,0.205504587,
0.20733945,0.209174312,0.211009174,0.212844037,0.214678899,0.216513761,
0.218348624,0.220183486,0.222018349,0.223853211,0.225688073,0.227522936,
0.229357798,0.231192661,0.233027523,0.234862385,0.236697248,0.23853211,
0.240366972,0.242201835,0.244036697,0.24587156,0.247706422,0.249541284,
0.251376147,0.253211009,0.255045872,0.256880734,0.258715596,0.260550459,
0.262385321,0.264220183,0.266055046,0.267889908,0.269724771,0.271559633,
0.273394495,0.275229358,0.27706422,0.278899083,0.280733945,0.282568807,
0.28440367,0.286238532,0.288073394,0.289908257,0.291743119,0.293577982,
0.295412844,0.297247706,0.299082569,0.300917431,0.302752294,0.304587156,
0.306422018,0.308256881,0.310091743,0.311926606,0.313761468,0.31559633,
0.317431193,0.319266055,0.321100917,0.32293578,0.324770642,0.326605505,
0.328440367,0.330275229,0.332110092,0.333944954,0.335779817,0.337614679,
0.339449541,0.341284404,0.343119266,0.344954128,0.346788991,0.348623853,
0.350458716,0.352293578,0.35412844,0.355963303,0.357798165,0.359633028,
0.36146789,0.363302752,0.365137615,0.366972477,0.368807339,0.370642202,
0.372477064,0.374311927,0.376146789,0.377981651,0.379816514,0.381651376,
0.383486239,0.385321101,0.387155963,0.388990826,0.390825688,0.39266055,
0.394495413,0.396330275,0.398165138,0.4,0.401834862,0.403669725,0.405504587,
0.40733945,0.409174312,0.411009174,0.412844037,0.414678899,0.416513761,
0.418348624,0.420183486,0.422018349,0.423853211,0.425688073,0.427522936,
0.429357798,0.431192661,0.433027523,0.434862385,0.436697248,0.43853211,
0.440366972,0.442201835,0.444036697,0.44587156,0.447706422,0.449541284,
0.451376147,0.453211009,0.455045872,0.456880734,0.458715596,0.460550459,
0.462385321,0.464220183,0.466055046,0.467889908,0.469724771,0.471559633,
0.473394495,0.475229358,0.47706422,0.478899083,0.480733945,0.482568807,
0.48440367,0.486238532,0.488073394,0.489908257,0.491743119,0.493577982,
0.495412844,0.497247706,0.499082569,0.500917431,0.502752294,0.504587156,
0.506422018,0.508256881,0.510091743,0.511926606,0.513761468,0.51559633,
0.517431193,0.519266055,0.521100917,0.52293578,0.524770642,0.526605505,
0.528440367,0.530275229,0.532110092,0.533944954,0.535779817,0.537614679,
0.539449541,0.541284404,0.543119266,0.544954128,0.546788991,0.548623853,
0.550458716,0.552293578,0.55412844,0.555963303,0.557798165,0.559633028,
0.56146789,0.563302752,0.565137615,0.566972477,0.568807339,0.570642202,
0.572477064,0.574311927,0.576146789,0.577981651,0.579816514,0.581651376,
0.583486239,0.585321101,0.587155963,0.588990826,0.590825688,0.59266055,
0.594495413,0.596330275,0.598165138,0.6,0.601834862,0.603669725,0.605504587,
0.60733945,0.609174312,0.611009174,0.612844037,0.614678899,0.616513761,
0.618348624,0.620183486,0.622018349,0.623853211,0.625688073,0.627522936,
0.629357798,0.631192661,0.633027523,0.634862385,0.636697248,0.63853211,
0.640366972,0.642201835,0.644036697,0.64587156,0.647706422,0.649541284,
0.651376147,0.653211009,0.655045872,0.656880734,0.658715596,0.660550459,
0.662385321,0.664220183,0.666055046,0.667889908,0.669724771,0.671559633,
0.673394495,0.675229358,0.67706422,0.678899083,0.680733945,0.682568807,
0.68440367,0.686238532,0.688073394,0.689908257,0.691743119,0.693577982,
0.695412844,0.697247706,0.699082569,0.700917431,0.702752294,0.704587156,
0.706422018,0.708256881,0.710091743,0.711926606,0.713761468,0.71559633,
0.717431193,0.719266055,0.721100917,0.72293578,0.724770642,0.726605505,
0.728440367,0.730275229,0.732110092,0.733944954,0.735779817,0.737614679,
0.739449541,0.741284404,0.743119266,0.744954128,0.746788991,0.748623853,
0.750458716,0.752293578,0.75412844,0.755963303,0.757798165,0.759633028,
0.76146789,0.763302752,0.765137615,0.766972477,0.768807339,0.770642202,
0.772477064,0.774311927,0.776146789,0.777981651,0.779816514,0.781651376,
0.783486239,0.785321101,0.787155963,0.788990826,0.790825688,0.79266055,
0.794495413,0.796330275,0.798165138,0.8,0.801834862,0.803669725,0.805504587,
0.80733945,0.809174312,0.811009174,0.812844037,0.814678899,0.816513761,
0.818348624,0.820183486,0.822018349,0.823853211,0.825688073,0.827522936,
0.829357798,0.831192661,0.833027523,0.834862385,0.836697248,0.83853211,
0.840366972,0.842201835,0.844036697,0.84587156,0.847706422,0.849541284,
0.851376147,0.853211009,0.855045872,0.856880734,0.858715596,0.860550459,
0.862385321,0.864220183,0.866055046,0.867889908,0.869724771,0.871559633,
0.873394495,0.875229358,0.87706422,0.878899083,0.880733945,0.882568807,
0.88440367,0.886238532,0.888073394,0.889908257,0.891743119,0.893577982,
0.895412844,0.897247706,0.899082569,0.900917431,0.902752294,0.904587156,
0.906422018,0.908256881,0.910091743,0.911926606,0.913761468,0.91559633,
0.917431193,0.919266055,0.921100917,0.92293578,0.924770642,0.926605505,
0.928440367,0.930275229,0.932110092,0.933944954,0.935779817,0.937614679,
0.939449541,0.941284404,0.943119266,0.944954128,0.946788991,0.948623853,
0.950458716,0.952293578,0.95412844,0.955963303,0.957798165,0.959633028,
0.96146789,0.963302752,0.965137615,0.966972477,0.968807339,0.970642202,
0.972477064,0.974311927,0.976146789,0.977981651,0.979816514,0.981651376,
0.983486239,0.985321101,0.987155963,0.988990826,0.990825688,0.99266055,
0.994495413,0.996330275,0.998165138,1.),.UNSPECIFIED.);
#24336=B_SPLINE_CURVE_WITH_KNOTS('',5,(#168646,#168647,#168648,#168649,
#168650,#168651,#168652,#168653,#168654,#168655,#168656,#168657,#168658,
#168659,#168660,#168661,#168662,#168663,#168664,#168665,#168666,#168667,
#168668,#168669,#168670,#168671,#168672,#168673,#168674,#168675,#168676,
#168677,#168678,#168679,#168680,#168681,#168682,#168683,#168684,#168685,
#168686,#168687,#168688,#168689,#168690,#168691,#168692,#168693,#168694,
#168695,#168696,#168697,#168698,#168699,#168700,#168701,#168702,#168703,
#168704,#168705,#168706,#168707,#168708,#168709,#168710,#168711,#168712,
#168713,#168714,#168715,#168716,#168717,#168718,#168719,#168720,#168721,
#168722,#168723,#168724,#168725,#168726,#168727,#168728,#168729,#168730,
#168731,#168732,#168733,#168734,#168735,#168736,#168737,#168738,#168739,
#168740,#168741,#168742,#168743,#168744,#168745,#168746,#168747,#168748,
#168749,#168750,#168751,#168752,#168753,#168754,#168755,#168756,#168757,
#168758,#168759,#168760,#168761,#168762,#168763,#168764,#168765,#168766,
#168767,#168768,#168769,#168770,#168771,#168772,#168773,#168774,#168775,
#168776,#168777,#168778,#168779,#168780,#168781,#168782,#168783,#168784,
#168785,#168786,#168787,#168788,#168789,#168790,#168791,#168792,#168793,
#168794,#168795,#168796,#168797,#168798,#168799,#168800,#168801,#168802,
#168803,#168804,#168805,#168806,#168807,#168808,#168809,#168810,#168811,
#168812,#168813,#168814,#168815,#168816,#168817,#168818,#168819,#168820,
#168821,#168822,#168823,#168824,#168825,#168826,#168827,#168828,#168829,
#168830,#168831,#168832,#168833,#168834,#168835,#168836,#168837,#168838,
#168839,#168840,#168841,#168842,#168843,#168844,#168845,#168846,#168847,
#168848,#168849,#168850,#168851,#168852,#168853,#168854,#168855,#168856,
#168857,#168858,#168859,#168860,#168861,#168862,#168863,#168864,#168865,
#168866,#168867,#168868,#168869,#168870,#168871,#168872,#168873,#168874,
#168875,#168876,#168877,#168878,#168879,#168880,#168881,#168882,#168883,
#168884,#168885,#168886,#168887,#168888,#168889,#168890,#168891,#168892,
#168893,#168894,#168895,#168896,#168897,#168898,#168899,#168900,#168901,
#168902,#168903,#168904,#168905,#168906,#168907,#168908,#168909,#168910,
#168911,#168912,#168913,#168914,#168915,#168916,#168917,#168918,#168919,
#168920,#168921,#168922,#168923,#168924,#168925,#168926,#168927,#168928,
#168929,#168930,#168931,#168932,#168933,#168934,#168935,#168936,#168937,
#168938,#168939,#168940,#168941,#168942,#168943,#168944,#168945,#168946,
#168947,#168948,#168949,#168950,#168951,#168952,#168953,#168954,#168955,
#168956,#168957,#168958,#168959,#168960,#168961,#168962,#168963,#168964,
#168965,#168966,#168967,#168968,#168969,#168970,#168971,#168972,#168973,
#168974,#168975,#168976,#168977,#168978,#168979,#168980,#168981,#168982,
#168983,#168984,#168985,#168986,#168987,#168988,#168989,#168990,#168991,
#168992,#168993,#168994,#168995,#168996,#168997,#168998,#168999,#169000,
#169001,#169002,#169003,#169004,#169005,#169006,#169007,#169008,#169009,
#169010,#169011,#169012,#169013,#169014,#169015,#169016,#169017,#169018,
#169019,#169020,#169021,#169022,#169023,#169024,#169025,#169026,#169027,
#169028,#169029,#169030,#169031,#169032,#169033,#169034,#169035,#169036,
#169037,#169038,#169039,#169040,#169041,#169042,#169043,#169044,#169045,
#169046,#169047,#169048,#169049,#169050,#169051,#169052,#169053,#169054,
#169055,#169056,#169057,#169058,#169059,#169060,#169061,#169062,#169063,
#169064,#169065,#169066,#169067,#169068,#169069,#169070,#169071,#169072,
#169073,#169074,#169075,#169076,#169077,#169078,#169079,#169080,#169081,
#169082,#169083,#169084,#169085,#169086,#169087,#169088,#169089,#169090,
#169091,#169092,#169093,#169094,#169095,#169096,#169097,#169098,#169099,
#169100,#169101,#169102,#169103,#169104,#169105,#169106,#169107,#169108,
#169109,#169110,#169111,#169112,#169113,#169114,#169115,#169116,#169117),
 .UNSPECIFIED.,.F.,.F.,(6,1,1,1,1,1,1,1,1,1,1,1,1,1,1,1,1,1,1,1,1,1,1,1,
1,1,1,1,1,1,1,1,1,1,1,1,1,1,1,1,1,1,1,1,1,1,1,1,1,1,1,1,1,1,1,1,1,1,1,1,
1,1,1,1,1,1,1,1,1,1,1,1,1,1,1,1,1,1,1,1,1,1,1,1,1,1,1,1,1,1,1,1,1,1,1,1,
1,1,1,1,1,1,1,1,1,1,1,1,1,1,1,1,1,1,1,1,1,1,1,1,1,1,1,1,1,1,1,1,1,1,1,1,
1,1,1,1,1,1,1,1,1,1,1,1,1,1,1,1,1,1,1,1,1,1,1,1,1,1,1,1,1,1,1,1,1,1,1,1,
1,1,1,1,1,1,1,1,1,1,1,1,1,1,1,1,1,1,1,1,1,1,1,1,1,1,1,1,1,1,1,1,1,1,1,1,
1,1,1,1,1,1,1,1,1,1,1,1,1,1,1,1,1,1,1,1,1,1,1,1,1,1,1,1,1,1,1,1,1,1,1,1,
1,1,1,1,1,1,1,1,1,1,1,1,1,1,1,1,1,1,1,1,1,1,1,1,1,1,1,1,1,1,1,1,1,1,1,1,
1,1,1,1,1,1,1,1,1,1,1,1,1,1,1,1,1,1,1,1,1,1,1,1,1,1,1,1,1,1,1,1,1,1,1,1,
1,1,1,1,1,1,1,1,1,1,1,1,1,1,1,1,1,1,1,1,1,1,1,1,1,1,1,1,1,1,1,1,1,1,1,1,
1,1,1,1,1,1,1,1,1,1,1,1,1,1,1,1,1,1,1,1,1,1,1,1,1,1,1,1,1,1,1,1,1,1,1,1,
1,1,1,1,1,1,1,1,1,1,1,1,1,1,1,1,1,1,1,1,1,1,1,1,1,1,1,1,1,1,1,1,1,1,1,1,
1,1,1,1,1,1,1,1,1,1,1,1,1,1,1,1,1,1,1,1,1,1,1,1,1,1,1,1,1,1,1,1,1,1,1,1,
1,1,1,1,1,1,1,1,1,1,1,6),(0.143172102,0.144954128,0.146788991,0.148623853,
0.150458716,0.152293578,0.15412844,0.155963303,0.157798165,0.159633028,
0.16146789,0.163302752,0.165137615,0.166972477,0.168807339,0.170642202,
0.172477064,0.174311927,0.176146789,0.177981651,0.179816514,0.181651376,
0.183486239,0.185321101,0.187155963,0.188990826,0.190825688,0.19266055,
0.194495413,0.196330275,0.198165138,0.2,0.201834862,0.203669725,0.205504587,
0.20733945,0.209174312,0.211009174,0.212844037,0.214678899,0.216513761,
0.218348624,0.220183486,0.222018349,0.223853211,0.225688073,0.227522936,
0.229357798,0.231192661,0.233027523,0.234862385,0.236697248,0.23853211,
0.240366972,0.242201835,0.244036697,0.24587156,0.247706422,0.249541284,
0.251376147,0.253211009,0.255045872,0.256880734,0.258715596,0.260550459,
0.262385321,0.264220183,0.266055046,0.267889908,0.269724771,0.271559633,
0.273394495,0.275229358,0.27706422,0.278899083,0.280733945,0.282568807,
0.28440367,0.286238532,0.288073394,0.289908257,0.291743119,0.293577982,
0.295412844,0.297247706,0.299082569,0.300917431,0.302752294,0.304587156,
0.306422018,0.308256881,0.310091743,0.311926606,0.313761468,0.31559633,
0.317431193,0.319266055,0.321100917,0.32293578,0.324770642,0.326605505,
0.328440367,0.330275229,0.332110092,0.333944954,0.335779817,0.337614679,
0.339449541,0.341284404,0.343119266,0.344954128,0.346788991,0.348623853,
0.350458716,0.352293578,0.35412844,0.355963303,0.357798165,0.359633028,
0.36146789,0.363302752,0.365137615,0.366972477,0.368807339,0.370642202,
0.372477064,0.374311927,0.376146789,0.377981651,0.379816514,0.381651376,
0.383486239,0.385321101,0.387155963,0.388990826,0.390825688,0.39266055,
0.394495413,0.396330275,0.398165138,0.4,0.401834862,0.403669725,0.405504587,
0.40733945,0.409174312,0.411009174,0.412844037,0.414678899,0.416513761,
0.418348624,0.420183486,0.422018349,0.423853211,0.425688073,0.427522936,
0.429357798,0.431192661,0.433027523,0.434862385,0.436697248,0.43853211,
0.440366972,0.442201835,0.444036697,0.44587156,0.447706422,0.449541284,
0.451376147,0.453211009,0.455045872,0.456880734,0.458715596,0.460550459,
0.462385321,0.464220183,0.466055046,0.467889908,0.469724771,0.471559633,
0.473394495,0.475229358,0.47706422,0.478899083,0.480733945,0.482568807,
0.48440367,0.486238532,0.488073394,0.489908257,0.491743119,0.493577982,
0.495412844,0.497247706,0.499082569,0.500917431,0.502752294,0.504587156,
0.506422018,0.508256881,0.510091743,0.511926606,0.513761468,0.51559633,
0.517431193,0.519266055,0.521100917,0.52293578,0.524770642,0.526605505,
0.528440367,0.530275229,0.532110092,0.533944954,0.535779817,0.537614679,
0.539449541,0.541284404,0.543119266,0.544954128,0.546788991,0.548623853,
0.550458716,0.552293578,0.55412844,0.555963303,0.557798165,0.559633028,
0.56146789,0.563302752,0.565137615,0.566972477,0.568807339,0.570642202,
0.572477064,0.574311927,0.576146789,0.577981651,0.579816514,0.581651376,
0.583486239,0.585321101,0.587155963,0.588990826,0.590825688,0.59266055,
0.594495413,0.596330275,0.598165138,0.6,0.601834862,0.603669725,0.605504587,
0.60733945,0.609174312,0.611009174,0.612844037,0.614678899,0.616513761,
0.618348624,0.620183486,0.622018349,0.623853211,0.625688073,0.627522936,
0.629357798,0.631192661,0.633027523,0.634862385,0.636697248,0.63853211,
0.640366972,0.642201835,0.644036697,0.64587156,0.647706422,0.649541284,
0.651376147,0.653211009,0.655045872,0.656880734,0.658715596,0.660550459,
0.662385321,0.664220183,0.666055046,0.667889908,0.669724771,0.671559633,
0.673394495,0.675229358,0.67706422,0.678899083,0.680733945,0.682568807,
0.68440367,0.686238532,0.688073394,0.689908257,0.691743119,0.693577982,
0.695412844,0.697247706,0.699082569,0.700917431,0.702752294,0.704587156,
0.706422018,0.708256881,0.710091743,0.711926606,0.713761468,0.71559633,
0.717431193,0.719266055,0.721100917,0.72293578,0.724770642,0.726605505,
0.728440367,0.730275229,0.732110092,0.733944954,0.735779817,0.737614679,
0.739449541,0.741284404,0.743119266,0.744954128,0.746788991,0.748623853,
0.750458716,0.752293578,0.75412844,0.755963303,0.757798165,0.759633028,
0.76146789,0.763302752,0.765137615,0.766972477,0.768807339,0.770642202,
0.772477064,0.774311927,0.776146789,0.777981651,0.779816514,0.781651376,
0.783486239,0.785321101,0.787155963,0.788990826,0.790825688,0.79266055,
0.794495413,0.796330275,0.798165138,0.8,0.801834862,0.803669725,0.805504587,
0.80733945,0.809174312,0.811009174,0.812844037,0.814678899,0.816513761,
0.818348624,0.820183486,0.822018349,0.823853211,0.825688073,0.827522936,
0.829357798,0.831192661,0.833027523,0.834862385,0.836697248,0.83853211,
0.840366972,0.842201835,0.844036697,0.84587156,0.847706422,0.849541284,
0.851376147,0.853211009,0.855045872,0.856880734,0.858715596,0.860550459,
0.862385321,0.864220183,0.866055046,0.867889908,0.869724771,0.871559633,
0.873394495,0.875229358,0.87706422,0.878899083,0.880733945,0.882568807,
0.88440367,0.886238532,0.888073394,0.889908257,0.891743119,0.893577982,
0.895412844,0.897247706,0.899082569,0.900917431,0.902752294,0.904587156,
0.906422018,0.908256881,0.910091743,0.911926606,0.913761468,0.91559633,
0.917431193,0.919266055,0.921100917,0.92293578,0.924770642,0.926605505,
0.928440367,0.930275229,0.932110092,0.933944954,0.935779817,0.937614679,
0.939449541,0.941284404,0.943119266,0.944954128,0.946788991,0.948623853,
0.950458716,0.952293578,0.95412844,0.955963303,0.957798165,0.959633028,
0.96146789,0.963302752,0.965137615,0.966972477,0.968807339,0.970642202,
0.972477064,0.974311927,0.976146789,0.977981651,0.979816514,0.981651376,
0.983486239,0.985321101,0.987155963,0.988990826,0.990825688,0.99266055,
0.994495413,0.996330275,0.998165138,1.),.UNSPECIFIED.);
#24337=B_SPLINE_CURVE_WITH_KNOTS('',5,(#170065,#170066,#170067,#170068,
#170069,#170070,#170071,#170072,#170073,#170074,#170075,#170076,#170077,
#170078,#170079,#170080,#170081,#170082,#170083,#170084,#170085,#170086,
#170087,#170088,#170089,#170090,#170091,#170092,#170093,#170094,#170095,
#170096,#170097,#170098,#170099,#170100,#170101,#170102,#170103,#170104,
#170105,#170106,#170107,#170108,#170109,#170110,#170111,#170112,#170113,
#170114,#170115,#170116,#170117,#170118,#170119,#170120,#170121,#170122,
#170123,#170124,#170125,#170126,#170127,#170128,#170129,#170130,#170131,
#170132,#170133,#170134,#170135,#170136,#170137,#170138,#170139,#170140,
#170141,#170142,#170143,#170144,#170145,#170146,#170147,#170148,#170149,
#170150,#170151,#170152,#170153,#170154,#170155,#170156,#170157,#170158,
#170159,#170160,#170161,#170162,#170163,#170164,#170165,#170166,#170167,
#170168,#170169,#170170,#170171,#170172,#170173,#170174,#170175,#170176,
#170177,#170178,#170179,#170180,#170181,#170182,#170183,#170184,#170185,
#170186,#170187,#170188,#170189,#170190,#170191,#170192,#170193,#170194,
#170195,#170196,#170197,#170198,#170199,#170200,#170201,#170202,#170203,
#170204,#170205,#170206,#170207,#170208,#170209,#170210,#170211,#170212,
#170213,#170214,#170215,#170216,#170217,#170218,#170219,#170220,#170221,
#170222,#170223,#170224,#170225,#170226,#170227,#170228,#170229,#170230,
#170231,#170232,#170233,#170234,#170235,#170236,#170237,#170238,#170239,
#170240,#170241,#170242,#170243,#170244,#170245,#170246,#170247,#170248,
#170249,#170250,#170251,#170252,#170253,#170254,#170255,#170256,#170257,
#170258,#170259,#170260,#170261,#170262,#170263,#170264,#170265,#170266,
#170267,#170268,#170269,#170270,#170271,#170272,#170273,#170274,#170275,
#170276,#170277,#170278,#170279,#170280,#170281,#170282,#170283,#170284,
#170285,#170286,#170287,#170288,#170289,#170290,#170291,#170292,#170293,
#170294,#170295,#170296,#170297,#170298,#170299,#170300,#170301,#170302,
#170303,#170304,#170305,#170306,#170307,#170308,#170309,#170310,#170311,
#170312,#170313,#170314,#170315,#170316,#170317,#170318,#170319,#170320,
#170321,#170322,#170323,#170324,#170325,#170326,#170327,#170328,#170329,
#170330,#170331,#170332,#170333,#170334,#170335,#170336,#170337,#170338,
#170339,#170340,#170341,#170342,#170343,#170344,#170345,#170346,#170347,
#170348,#170349,#170350,#170351,#170352,#170353,#170354,#170355,#170356,
#170357,#170358,#170359,#170360,#170361,#170362,#170363,#170364,#170365,
#170366,#170367,#170368,#170369,#170370,#170371,#170372,#170373,#170374,
#170375,#170376,#170377,#170378,#170379,#170380,#170381,#170382,#170383,
#170384,#170385,#170386,#170387,#170388,#170389,#170390,#170391,#170392,
#170393,#170394,#170395,#170396,#170397,#170398,#170399,#170400,#170401,
#170402,#170403,#170404,#170405,#170406,#170407,#170408,#170409,#170410,
#170411,#170412,#170413,#170414,#170415,#170416,#170417,#170418,#170419,
#170420,#170421,#170422,#170423,#170424,#170425,#170426,#170427,#170428,
#170429,#170430,#170431,#170432,#170433,#170434,#170435,#170436,#170437,
#170438,#170439,#170440,#170441,#170442,#170443,#170444,#170445,#170446,
#170447,#170448,#170449,#170450,#170451,#170452,#170453,#170454,#170455,
#170456,#170457,#170458,#170459,#170460,#170461,#170462,#170463,#170464,
#170465,#170466,#170467,#170468,#170469,#170470,#170471,#170472,#170473,
#170474,#170475,#170476,#170477,#170478,#170479,#170480,#170481,#170482,
#170483,#170484,#170485,#170486,#170487,#170488,#170489,#170490,#170491,
#170492,#170493,#170494,#170495,#170496,#170497,#170498,#170499,#170500,
#170501,#170502,#170503,#170504,#170505,#170506,#170507,#170508,#170509,
#170510,#170511,#170512,#170513,#170514,#170515,#170516,#170517,#170518,
#170519,#170520,#170521,#170522,#170523,#170524,#170525,#170526,#170527,
#170528,#170529,#170530,#170531,#170532,#170533,#170534,#170535,#170536),
 .UNSPECIFIED.,.F.,.F.,(6,1,1,1,1,1,1,1,1,1,1,1,1,1,1,1,1,1,1,1,1,1,1,1,
1,1,1,1,1,1,1,1,1,1,1,1,1,1,1,1,1,1,1,1,1,1,1,1,1,1,1,1,1,1,1,1,1,1,1,1,
1,1,1,1,1,1,1,1,1,1,1,1,1,1,1,1,1,1,1,1,1,1,1,1,1,1,1,1,1,1,1,1,1,1,1,1,
1,1,1,1,1,1,1,1,1,1,1,1,1,1,1,1,1,1,1,1,1,1,1,1,1,1,1,1,1,1,1,1,1,1,1,1,
1,1,1,1,1,1,1,1,1,1,1,1,1,1,1,1,1,1,1,1,1,1,1,1,1,1,1,1,1,1,1,1,1,1,1,1,
1,1,1,1,1,1,1,1,1,1,1,1,1,1,1,1,1,1,1,1,1,1,1,1,1,1,1,1,1,1,1,1,1,1,1,1,
1,1,1,1,1,1,1,1,1,1,1,1,1,1,1,1,1,1,1,1,1,1,1,1,1,1,1,1,1,1,1,1,1,1,1,1,
1,1,1,1,1,1,1,1,1,1,1,1,1,1,1,1,1,1,1,1,1,1,1,1,1,1,1,1,1,1,1,1,1,1,1,1,
1,1,1,1,1,1,1,1,1,1,1,1,1,1,1,1,1,1,1,1,1,1,1,1,1,1,1,1,1,1,1,1,1,1,1,1,
1,1,1,1,1,1,1,1,1,1,1,1,1,1,1,1,1,1,1,1,1,1,1,1,1,1,1,1,1,1,1,1,1,1,1,1,
1,1,1,1,1,1,1,1,1,1,1,1,1,1,1,1,1,1,1,1,1,1,1,1,1,1,1,1,1,1,1,1,1,1,1,1,
1,1,1,1,1,1,1,1,1,1,1,1,1,1,1,1,1,1,1,1,1,1,1,1,1,1,1,1,1,1,1,1,1,1,1,1,
1,1,1,1,1,1,1,1,1,1,1,1,1,1,1,1,1,1,1,1,1,1,1,1,1,1,1,1,1,1,1,1,1,1,1,1,
1,1,1,1,1,1,1,1,1,1,1,6),(-1.,-0.998165138,-0.996330275,-0.994495413,-0.99266055,
-0.990825688,-0.988990826,-0.987155963,-0.985321101,-0.983486239,-0.981651376,
-0.979816514,-0.977981651,-0.976146789,-0.974311927,-0.972477064,-0.970642202,
-0.968807339,-0.966972477,-0.965137615,-0.963302752,-0.96146789,-0.959633028,
-0.957798165,-0.955963303,-0.95412844,-0.952293578,-0.950458716,-0.948623853,
-0.946788991,-0.944954128,-0.943119266,-0.941284404,-0.939449541,-0.937614679,
-0.935779817,-0.933944954,-0.932110092,-0.930275229,-0.928440367,-0.926605505,
-0.924770642,-0.92293578,-0.921100917,-0.919266055,-0.917431193,-0.91559633,
-0.913761468,-0.911926606,-0.910091743,-0.908256881,-0.906422018,-0.904587156,
-0.902752294,-0.900917431,-0.899082569,-0.897247706,-0.895412844,-0.893577982,
-0.891743119,-0.889908257,-0.888073394,-0.886238532,-0.88440367,-0.882568807,
-0.880733945,-0.878899083,-0.87706422,-0.875229358,-0.873394495,-0.871559633,
-0.869724771,-0.867889908,-0.866055046,-0.864220183,-0.862385321,-0.860550459,
-0.858715596,-0.856880734,-0.855045872,-0.853211009,-0.851376147,-0.849541284,
-0.847706422,-0.84587156,-0.844036697,-0.842201835,-0.840366972,-0.83853211,
-0.836697248,-0.834862385,-0.833027523,-0.831192661,-0.829357798,-0.827522936,
-0.825688073,-0.823853211,-0.822018349,-0.820183486,-0.818348624,-0.816513761,
-0.814678899,-0.812844037,-0.811009174,-0.809174312,-0.80733945,-0.805504587,
-0.803669725,-0.801834862,-0.8,-0.798165138,-0.796330275,-0.794495413,-0.79266055,
-0.790825688,-0.788990826,-0.787155963,-0.785321101,-0.783486239,-0.781651376,
-0.779816514,-0.777981651,-0.776146789,-0.774311927,-0.772477064,-0.770642202,
-0.768807339,-0.766972477,-0.765137615,-0.763302752,-0.76146789,-0.759633028,
-0.757798165,-0.755963303,-0.75412844,-0.752293578,-0.750458716,-0.748623853,
-0.746788991,-0.744954128,-0.743119266,-0.741284404,-0.739449541,-0.737614679,
-0.735779817,-0.733944954,-0.732110092,-0.730275229,-0.728440367,-0.726605505,
-0.724770642,-0.72293578,-0.721100917,-0.719266055,-0.717431193,-0.71559633,
-0.713761468,-0.711926606,-0.710091743,-0.708256881,-0.706422018,-0.704587156,
-0.702752294,-0.700917431,-0.699082569,-0.697247706,-0.695412844,-0.693577982,
-0.691743119,-0.689908257,-0.688073394,-0.686238532,-0.68440367,-0.682568807,
-0.680733945,-0.678899083,-0.67706422,-0.675229358,-0.673394495,-0.671559633,
-0.669724771,-0.667889908,-0.666055046,-0.664220183,-0.662385321,-0.660550459,
-0.658715596,-0.656880734,-0.655045872,-0.653211009,-0.651376147,-0.649541284,
-0.647706422,-0.64587156,-0.644036697,-0.642201835,-0.640366972,-0.63853211,
-0.636697248,-0.634862385,-0.633027523,-0.631192661,-0.629357798,-0.627522936,
-0.625688073,-0.623853211,-0.622018349,-0.620183486,-0.618348624,-0.616513761,
-0.614678899,-0.612844037,-0.611009174,-0.609174312,-0.60733945,-0.605504587,
-0.603669725,-0.601834862,-0.6,-0.598165138,-0.596330275,-0.594495413,-0.59266055,
-0.590825688,-0.588990826,-0.587155963,-0.585321101,-0.583486239,-0.581651376,
-0.579816514,-0.577981651,-0.576146789,-0.574311927,-0.572477064,-0.570642202,
-0.568807339,-0.566972477,-0.565137615,-0.563302752,-0.56146789,-0.559633028,
-0.557798165,-0.555963303,-0.55412844,-0.552293578,-0.550458716,-0.548623853,
-0.546788991,-0.544954128,-0.543119266,-0.541284404,-0.539449541,-0.537614679,
-0.535779817,-0.533944954,-0.532110092,-0.530275229,-0.528440367,-0.526605505,
-0.524770642,-0.52293578,-0.521100917,-0.519266055,-0.517431193,-0.51559633,
-0.513761468,-0.511926606,-0.510091743,-0.508256881,-0.506422018,-0.504587156,
-0.502752294,-0.500917431,-0.499082569,-0.497247706,-0.495412844,-0.493577982,
-0.491743119,-0.489908257,-0.488073394,-0.486238532,-0.48440367,-0.482568807,
-0.480733945,-0.478899083,-0.47706422,-0.475229358,-0.473394495,-0.471559633,
-0.469724771,-0.467889908,-0.466055046,-0.464220183,-0.462385321,-0.460550459,
-0.458715596,-0.456880734,-0.455045872,-0.453211009,-0.451376147,-0.449541284,
-0.447706422,-0.44587156,-0.444036697,-0.442201835,-0.440366972,-0.43853211,
-0.436697248,-0.434862385,-0.433027523,-0.431192661,-0.429357798,-0.427522936,
-0.425688073,-0.423853211,-0.422018349,-0.420183486,-0.418348624,-0.416513761,
-0.414678899,-0.412844037,-0.411009174,-0.409174312,-0.40733945,-0.405504587,
-0.403669725,-0.401834862,-0.4,-0.398165138,-0.396330275,-0.394495413,-0.39266055,
-0.390825688,-0.388990826,-0.387155963,-0.385321101,-0.383486239,-0.381651376,
-0.379816514,-0.377981651,-0.376146789,-0.374311927,-0.372477064,-0.370642202,
-0.368807339,-0.366972477,-0.365137615,-0.363302752,-0.36146789,-0.359633028,
-0.357798165,-0.355963303,-0.35412844,-0.352293578,-0.350458716,-0.348623853,
-0.346788991,-0.344954128,-0.343119266,-0.341284404,-0.339449541,-0.337614679,
-0.335779817,-0.333944954,-0.332110092,-0.330275229,-0.328440367,-0.326605505,
-0.324770642,-0.32293578,-0.321100917,-0.319266055,-0.317431193,-0.31559633,
-0.313761468,-0.311926606,-0.310091743,-0.308256881,-0.306422018,-0.304587156,
-0.302752294,-0.300917431,-0.299082569,-0.297247706,-0.295412844,-0.293577982,
-0.291743119,-0.289908257,-0.288073394,-0.286238532,-0.28440367,-0.282568807,
-0.280733945,-0.278899083,-0.27706422,-0.275229358,-0.273394495,-0.271559633,
-0.269724771,-0.267889908,-0.266055046,-0.264220183,-0.262385321,-0.260550459,
-0.258715596,-0.256880734,-0.255045872,-0.253211009,-0.251376147,-0.249541284,
-0.247706422,-0.24587156,-0.244036697,-0.242201835,-0.240366972,-0.23853211,
-0.236697248,-0.234862385,-0.233027523,-0.231192661,-0.229357798,-0.227522936,
-0.225688073,-0.223853211,-0.222018349,-0.220183486,-0.218348624,-0.216513761,
-0.214678899,-0.212844037,-0.211009174,-0.209174312,-0.20733945,-0.205504587,
-0.203669725,-0.201834862,-0.2,-0.198165138,-0.196330275,-0.194495413,-0.19266055,
-0.190825688,-0.188990826,-0.187155963,-0.185321101,-0.183486239,-0.181651376,
-0.179816514,-0.177981651,-0.176146789,-0.174311927,-0.172477064,-0.170642202,
-0.168807339,-0.166972477,-0.165137615,-0.163302752,-0.16146789,-0.159633028,
-0.157798165,-0.155963303,-0.15412844,-0.152293578,-0.150458716,-0.148623853,
-0.146788991,-0.144954128,-0.143172102),.UNSPECIFIED.);
#24338=B_SPLINE_CURVE_WITH_KNOTS('',5,(#170537,#170538,#170539,#170540,
#170541,#170542,#170543,#170544,#170545,#170546,#170547,#170548,#170549,
#170550,#170551,#170552,#170553,#170554,#170555,#170556,#170557,#170558,
#170559,#170560,#170561,#170562,#170563,#170564,#170565,#170566,#170567,
#170568,#170569,#170570,#170571,#170572,#170573,#170574,#170575,#170576,
#170577,#170578,#170579,#170580,#170581,#170582,#170583,#170584,#170585,
#170586,#170587,#170588,#170589,#170590,#170591,#170592,#170593,#170594,
#170595,#170596,#170597,#170598,#170599,#170600,#170601,#170602,#170603,
#170604,#170605,#170606,#170607,#170608,#170609,#170610,#170611,#170612,
#170613,#170614,#170615,#170616,#170617,#170618,#170619,#170620,#170621,
#170622,#170623,#170624,#170625,#170626,#170627,#170628,#170629,#170630,
#170631,#170632,#170633,#170634,#170635,#170636,#170637,#170638,#170639,
#170640,#170641,#170642,#170643,#170644,#170645,#170646,#170647,#170648,
#170649,#170650,#170651,#170652,#170653,#170654,#170655,#170656,#170657,
#170658,#170659,#170660,#170661,#170662,#170663,#170664,#170665,#170666,
#170667,#170668,#170669,#170670,#170671,#170672,#170673,#170674,#170675,
#170676,#170677,#170678,#170679,#170680,#170681,#170682,#170683,#170684,
#170685,#170686,#170687,#170688,#170689,#170690,#170691,#170692,#170693,
#170694,#170695,#170696,#170697,#170698,#170699,#170700,#170701,#170702,
#170703,#170704,#170705,#170706,#170707,#170708,#170709,#170710,#170711,
#170712,#170713,#170714,#170715,#170716,#170717,#170718,#170719,#170720,
#170721,#170722,#170723,#170724,#170725,#170726,#170727,#170728,#170729,
#170730,#170731,#170732,#170733,#170734,#170735,#170736,#170737,#170738,
#170739,#170740,#170741,#170742,#170743,#170744,#170745,#170746,#170747,
#170748,#170749,#170750,#170751,#170752,#170753,#170754,#170755,#170756,
#170757,#170758,#170759,#170760,#170761,#170762,#170763,#170764,#170765,
#170766,#170767,#170768,#170769,#170770,#170771,#170772,#170773,#170774,
#170775,#170776,#170777,#170778,#170779,#170780,#170781,#170782,#170783,
#170784,#170785,#170786,#170787,#170788,#170789,#170790,#170791,#170792,
#170793,#170794,#170795,#170796,#170797,#170798,#170799,#170800,#170801,
#170802,#170803,#170804,#170805,#170806,#170807,#170808,#170809,#170810,
#170811,#170812,#170813,#170814,#170815,#170816,#170817,#170818,#170819,
#170820,#170821,#170822,#170823,#170824,#170825,#170826,#170827,#170828,
#170829,#170830,#170831,#170832,#170833,#170834,#170835,#170836,#170837,
#170838,#170839,#170840,#170841,#170842,#170843,#170844,#170845,#170846,
#170847,#170848,#170849,#170850,#170851,#170852,#170853,#170854,#170855,
#170856,#170857,#170858,#170859,#170860,#170861,#170862,#170863,#170864,
#170865,#170866,#170867,#170868,#170869,#170870,#170871,#170872,#170873,
#170874,#170875,#170876,#170877,#170878,#170879,#170880,#170881,#170882,
#170883,#170884,#170885,#170886,#170887,#170888,#170889,#170890,#170891,
#170892,#170893,#170894,#170895,#170896,#170897,#170898,#170899,#170900,
#170901,#170902,#170903,#170904,#170905,#170906,#170907,#170908,#170909,
#170910,#170911,#170912,#170913,#170914,#170915,#170916,#170917,#170918,
#170919,#170920,#170921,#170922,#170923,#170924,#170925,#170926,#170927,
#170928,#170929,#170930,#170931,#170932,#170933,#170934,#170935,#170936,
#170937,#170938,#170939,#170940,#170941,#170942,#170943,#170944,#170945,
#170946,#170947,#170948,#170949,#170950,#170951,#170952,#170953,#170954,
#170955,#170956,#170957,#170958,#170959,#170960,#170961,#170962,#170963,
#170964,#170965,#170966,#170967,#170968,#170969,#170970,#170971,#170972,
#170973,#170974,#170975,#170976,#170977,#170978,#170979,#170980,#170981,
#170982,#170983,#170984,#170985,#170986,#170987,#170988,#170989,#170990,
#170991,#170992,#170993,#170994,#170995,#170996,#170997,#170998,#170999,
#171000,#171001,#171002,#171003,#171004,#171005,#171006,#171007,#171008),
 .UNSPECIFIED.,.F.,.F.,(6,1,1,1,1,1,1,1,1,1,1,1,1,1,1,1,1,1,1,1,1,1,1,1,
1,1,1,1,1,1,1,1,1,1,1,1,1,1,1,1,1,1,1,1,1,1,1,1,1,1,1,1,1,1,1,1,1,1,1,1,
1,1,1,1,1,1,1,1,1,1,1,1,1,1,1,1,1,1,1,1,1,1,1,1,1,1,1,1,1,1,1,1,1,1,1,1,
1,1,1,1,1,1,1,1,1,1,1,1,1,1,1,1,1,1,1,1,1,1,1,1,1,1,1,1,1,1,1,1,1,1,1,1,
1,1,1,1,1,1,1,1,1,1,1,1,1,1,1,1,1,1,1,1,1,1,1,1,1,1,1,1,1,1,1,1,1,1,1,1,
1,1,1,1,1,1,1,1,1,1,1,1,1,1,1,1,1,1,1,1,1,1,1,1,1,1,1,1,1,1,1,1,1,1,1,1,
1,1,1,1,1,1,1,1,1,1,1,1,1,1,1,1,1,1,1,1,1,1,1,1,1,1,1,1,1,1,1,1,1,1,1,1,
1,1,1,1,1,1,1,1,1,1,1,1,1,1,1,1,1,1,1,1,1,1,1,1,1,1,1,1,1,1,1,1,1,1,1,1,
1,1,1,1,1,1,1,1,1,1,1,1,1,1,1,1,1,1,1,1,1,1,1,1,1,1,1,1,1,1,1,1,1,1,1,1,
1,1,1,1,1,1,1,1,1,1,1,1,1,1,1,1,1,1,1,1,1,1,1,1,1,1,1,1,1,1,1,1,1,1,1,1,
1,1,1,1,1,1,1,1,1,1,1,1,1,1,1,1,1,1,1,1,1,1,1,1,1,1,1,1,1,1,1,1,1,1,1,1,
1,1,1,1,1,1,1,1,1,1,1,1,1,1,1,1,1,1,1,1,1,1,1,1,1,1,1,1,1,1,1,1,1,1,1,1,
1,1,1,1,1,1,1,1,1,1,1,1,1,1,1,1,1,1,1,1,1,1,1,1,1,1,1,1,1,1,1,1,1,1,1,1,
1,1,1,1,1,1,1,1,1,1,1,6),(0.143172102,0.144954128,0.146788991,0.148623853,
0.150458716,0.152293578,0.15412844,0.155963303,0.157798165,0.159633028,
0.16146789,0.163302752,0.165137615,0.166972477,0.168807339,0.170642202,
0.172477064,0.174311927,0.176146789,0.177981651,0.179816514,0.181651376,
0.183486239,0.185321101,0.187155963,0.188990826,0.190825688,0.19266055,
0.194495413,0.196330275,0.198165138,0.2,0.201834862,0.203669725,0.205504587,
0.20733945,0.209174312,0.211009174,0.212844037,0.214678899,0.216513761,
0.218348624,0.220183486,0.222018349,0.223853211,0.225688073,0.227522936,
0.229357798,0.231192661,0.233027523,0.234862385,0.236697248,0.23853211,
0.240366972,0.242201835,0.244036697,0.24587156,0.247706422,0.249541284,
0.251376147,0.253211009,0.255045872,0.256880734,0.258715596,0.260550459,
0.262385321,0.264220183,0.266055046,0.267889908,0.269724771,0.271559633,
0.273394495,0.275229358,0.27706422,0.278899083,0.280733945,0.282568807,
0.28440367,0.286238532,0.288073394,0.289908257,0.291743119,0.293577982,
0.295412844,0.297247706,0.299082569,0.300917431,0.302752294,0.304587156,
0.306422018,0.308256881,0.310091743,0.311926606,0.313761468,0.31559633,
0.317431193,0.319266055,0.321100917,0.32293578,0.324770642,0.326605505,
0.328440367,0.330275229,0.332110092,0.333944954,0.335779817,0.337614679,
0.339449541,0.341284404,0.343119266,0.344954128,0.346788991,0.348623853,
0.350458716,0.352293578,0.35412844,0.355963303,0.357798165,0.359633028,
0.36146789,0.363302752,0.365137615,0.366972477,0.368807339,0.370642202,
0.372477064,0.374311927,0.376146789,0.377981651,0.379816514,0.381651376,
0.383486239,0.385321101,0.387155963,0.388990826,0.390825688,0.39266055,
0.394495413,0.396330275,0.398165138,0.4,0.401834862,0.403669725,0.405504587,
0.40733945,0.409174312,0.411009174,0.412844037,0.414678899,0.416513761,
0.418348624,0.420183486,0.422018349,0.423853211,0.425688073,0.427522936,
0.429357798,0.431192661,0.433027523,0.434862385,0.436697248,0.43853211,
0.440366972,0.442201835,0.444036697,0.44587156,0.447706422,0.449541284,
0.451376147,0.453211009,0.455045872,0.456880734,0.458715596,0.460550459,
0.462385321,0.464220183,0.466055046,0.467889908,0.469724771,0.471559633,
0.473394495,0.475229358,0.47706422,0.478899083,0.480733945,0.482568807,
0.48440367,0.486238532,0.488073394,0.489908257,0.491743119,0.493577982,
0.495412844,0.497247706,0.499082569,0.500917431,0.502752294,0.504587156,
0.506422018,0.508256881,0.510091743,0.511926606,0.513761468,0.51559633,
0.517431193,0.519266055,0.521100917,0.52293578,0.524770642,0.526605505,
0.528440367,0.530275229,0.532110092,0.533944954,0.535779817,0.537614679,
0.539449541,0.541284404,0.543119266,0.544954128,0.546788991,0.548623853,
0.550458716,0.552293578,0.55412844,0.555963303,0.557798165,0.559633028,
0.56146789,0.563302752,0.565137615,0.566972477,0.568807339,0.570642202,
0.572477064,0.574311927,0.576146789,0.577981651,0.579816514,0.581651376,
0.583486239,0.585321101,0.587155963,0.588990826,0.590825688,0.59266055,
0.594495413,0.596330275,0.598165138,0.6,0.601834862,0.603669725,0.605504587,
0.60733945,0.609174312,0.611009174,0.612844037,0.614678899,0.616513761,
0.618348624,0.620183486,0.622018349,0.623853211,0.625688073,0.627522936,
0.629357798,0.631192661,0.633027523,0.634862385,0.636697248,0.63853211,
0.640366972,0.642201835,0.644036697,0.64587156,0.647706422,0.649541284,
0.651376147,0.653211009,0.655045872,0.656880734,0.658715596,0.660550459,
0.662385321,0.664220183,0.666055046,0.667889908,0.669724771,0.671559633,
0.673394495,0.675229358,0.67706422,0.678899083,0.680733945,0.682568807,
0.68440367,0.686238532,0.688073394,0.689908257,0.691743119,0.693577982,
0.695412844,0.697247706,0.699082569,0.700917431,0.702752294,0.704587156,
0.706422018,0.708256881,0.710091743,0.711926606,0.713761468,0.71559633,
0.717431193,0.719266055,0.721100917,0.72293578,0.724770642,0.726605505,
0.728440367,0.730275229,0.732110092,0.733944954,0.735779817,0.737614679,
0.739449541,0.741284404,0.743119266,0.744954128,0.746788991,0.748623853,
0.750458716,0.752293578,0.75412844,0.755963303,0.757798165,0.759633028,
0.76146789,0.763302752,0.765137615,0.766972477,0.768807339,0.770642202,
0.772477064,0.774311927,0.776146789,0.777981651,0.779816514,0.781651376,
0.783486239,0.785321101,0.787155963,0.788990826,0.790825688,0.79266055,
0.794495413,0.796330275,0.798165138,0.8,0.801834862,0.803669725,0.805504587,
0.80733945,0.809174312,0.811009174,0.812844037,0.814678899,0.816513761,
0.818348624,0.820183486,0.822018349,0.823853211,0.825688073,0.827522936,
0.829357798,0.831192661,0.833027523,0.834862385,0.836697248,0.83853211,
0.840366972,0.842201835,0.844036697,0.84587156,0.847706422,0.849541284,
0.851376147,0.853211009,0.855045872,0.856880734,0.858715596,0.860550459,
0.862385321,0.864220183,0.866055046,0.867889908,0.869724771,0.871559633,
0.873394495,0.875229358,0.87706422,0.878899083,0.880733945,0.882568807,
0.88440367,0.886238532,0.888073394,0.889908257,0.891743119,0.893577982,
0.895412844,0.897247706,0.899082569,0.900917431,0.902752294,0.904587156,
0.906422018,0.908256881,0.910091743,0.911926606,0.913761468,0.91559633,
0.917431193,0.919266055,0.921100917,0.92293578,0.924770642,0.926605505,
0.928440367,0.930275229,0.932110092,0.933944954,0.935779817,0.937614679,
0.939449541,0.941284404,0.943119266,0.944954128,0.946788991,0.948623853,
0.950458716,0.952293578,0.95412844,0.955963303,0.957798165,0.959633028,
0.96146789,0.963302752,0.965137615,0.966972477,0.968807339,0.970642202,
0.972477064,0.974311927,0.976146789,0.977981651,0.979816514,0.981651376,
0.983486239,0.985321101,0.987155963,0.988990826,0.990825688,0.99266055,
0.994495413,0.996330275,0.998165138,1.),.UNSPECIFIED.);
#24339=B_SPLINE_CURVE_WITH_KNOTS('',5,(#171971,#171972,#171973,#171974,
#171975,#171976,#171977,#171978,#171979,#171980,#171981,#171982,#171983,
#171984,#171985,#171986,#171987,#171988,#171989,#171990,#171991,#171992,
#171993,#171994,#171995,#171996,#171997,#171998,#171999,#172000,#172001,
#172002,#172003,#172004,#172005,#172006,#172007,#172008,#172009,#172010,
#172011,#172012,#172013,#172014,#172015,#172016,#172017,#172018,#172019,
#172020,#172021,#172022,#172023,#172024,#172025,#172026,#172027,#172028,
#172029,#172030,#172031,#172032,#172033,#172034,#172035,#172036,#172037,
#172038,#172039,#172040,#172041,#172042,#172043,#172044,#172045,#172046,
#172047,#172048,#172049,#172050,#172051,#172052,#172053,#172054,#172055,
#172056,#172057,#172058,#172059,#172060,#172061,#172062,#172063,#172064,
#172065,#172066,#172067,#172068,#172069,#172070,#172071,#172072,#172073,
#172074,#172075,#172076,#172077,#172078,#172079,#172080,#172081,#172082,
#172083,#172084,#172085,#172086,#172087,#172088,#172089,#172090,#172091,
#172092,#172093,#172094,#172095,#172096,#172097,#172098,#172099,#172100,
#172101,#172102,#172103,#172104,#172105,#172106,#172107,#172108,#172109,
#172110,#172111,#172112,#172113,#172114,#172115,#172116,#172117,#172118,
#172119,#172120,#172121,#172122,#172123,#172124,#172125,#172126,#172127,
#172128,#172129,#172130,#172131,#172132,#172133,#172134,#172135,#172136,
#172137,#172138,#172139,#172140,#172141,#172142,#172143,#172144,#172145,
#172146,#172147,#172148,#172149,#172150,#172151,#172152,#172153,#172154,
#172155,#172156,#172157,#172158,#172159,#172160,#172161,#172162,#172163,
#172164,#172165,#172166,#172167,#172168,#172169,#172170,#172171,#172172,
#172173,#172174,#172175,#172176,#172177,#172178,#172179,#172180,#172181,
#172182,#172183,#172184,#172185,#172186,#172187,#172188,#172189,#172190,
#172191,#172192,#172193,#172194,#172195,#172196,#172197,#172198,#172199,
#172200,#172201,#172202,#172203,#172204,#172205,#172206,#172207,#172208,
#172209,#172210,#172211,#172212,#172213,#172214,#172215,#172216,#172217,
#172218,#172219,#172220,#172221,#172222,#172223,#172224,#172225,#172226,
#172227,#172228,#172229,#172230,#172231,#172232,#172233,#172234,#172235,
#172236,#172237,#172238,#172239,#172240,#172241,#172242,#172243,#172244,
#172245,#172246,#172247,#172248,#172249,#172250,#172251,#172252,#172253,
#172254,#172255,#172256,#172257,#172258,#172259,#172260,#172261,#172262,
#172263,#172264,#172265,#172266,#172267,#172268,#172269,#172270,#172271,
#172272,#172273,#172274,#172275,#172276,#172277,#172278,#172279,#172280,
#172281,#172282,#172283,#172284,#172285,#172286,#172287,#172288,#172289,
#172290,#172291,#172292,#172293,#172294,#172295,#172296,#172297,#172298,
#172299,#172300,#172301,#172302,#172303,#172304,#172305,#172306,#172307,
#172308,#172309,#172310,#172311,#172312,#172313,#172314,#172315,#172316,
#172317,#172318,#172319,#172320,#172321,#172322,#172323,#172324,#172325,
#172326,#172327,#172328,#172329,#172330,#172331,#172332,#172333,#172334,
#172335,#172336,#172337,#172338,#172339,#172340,#172341,#172342,#172343,
#172344,#172345,#172346,#172347,#172348,#172349,#172350,#172351,#172352,
#172353,#172354,#172355,#172356,#172357,#172358,#172359,#172360,#172361,
#172362,#172363,#172364,#172365,#172366,#172367,#172368,#172369,#172370,
#172371,#172372,#172373,#172374,#172375,#172376,#172377,#172378,#172379,
#172380,#172381,#172382,#172383,#172384,#172385,#172386,#172387,#172388,
#172389,#172390,#172391,#172392,#172393,#172394,#172395,#172396,#172397,
#172398,#172399,#172400,#172401,#172402,#172403,#172404,#172405,#172406,
#172407,#172408,#172409,#172410,#172411,#172412,#172413,#172414,#172415,
#172416,#172417,#172418,#172419,#172420,#172421,#172422,#172423,#172424,
#172425,#172426,#172427,#172428,#172429,#172430,#172431,#172432,#172433,
#172434,#172435,#172436,#172437,#172438,#172439),.UNSPECIFIED.,.F.,.F.,
(6,1,1,1,1,1,1,1,1,1,1,1,1,1,1,1,1,1,1,1,1,1,1,1,1,1,1,1,1,1,1,1,1,1,1,
1,1,1,1,1,1,1,1,1,1,1,1,1,1,1,1,1,1,1,1,1,1,1,1,1,1,1,1,1,1,1,1,1,1,1,1,
1,1,1,1,1,1,1,1,1,1,1,1,1,1,1,1,1,1,1,1,1,1,1,1,1,1,1,1,1,1,1,1,1,1,1,1,
1,1,1,1,1,1,1,1,1,1,1,1,1,1,1,1,1,1,1,1,1,1,1,1,1,1,1,1,1,1,1,1,1,1,1,1,
1,1,1,1,1,1,1,1,1,1,1,1,1,1,1,1,1,1,1,1,1,1,1,1,1,1,1,1,1,1,1,1,1,1,1,1,
1,1,1,1,1,1,1,1,1,1,1,1,1,1,1,1,1,1,1,1,1,1,1,1,1,1,1,1,1,1,1,1,1,1,1,1,
1,1,1,1,1,1,1,1,1,1,1,1,1,1,1,1,1,1,1,1,1,1,1,1,1,1,1,1,1,1,1,1,1,1,1,1,
1,1,1,1,1,1,1,1,1,1,1,1,1,1,1,1,1,1,1,1,1,1,1,1,1,1,1,1,1,1,1,1,1,1,1,1,
1,1,1,1,1,1,1,1,1,1,1,1,1,1,1,1,1,1,1,1,1,1,1,1,1,1,1,1,1,1,1,1,1,1,1,1,
1,1,1,1,1,1,1,1,1,1,1,1,1,1,1,1,1,1,1,1,1,1,1,1,1,1,1,1,1,1,1,1,1,1,1,1,
1,1,1,1,1,1,1,1,1,1,1,1,1,1,1,1,1,1,1,1,1,1,1,1,1,1,1,1,1,1,1,1,1,1,1,1,
1,1,1,1,1,1,1,1,1,1,1,1,1,1,1,1,1,1,1,1,1,1,1,1,1,1,1,1,1,1,1,1,1,1,1,1,
1,1,1,1,1,1,1,1,1,1,1,1,1,1,1,1,1,1,1,1,1,1,1,1,1,1,1,1,1,1,1,1,1,6),(-1.,
-0.998165138,-0.996330275,-0.994495413,-0.99266055,-0.990825688,-0.988990826,
-0.987155963,-0.985321101,-0.983486239,-0.981651376,-0.979816514,-0.977981651,
-0.974311927,-0.972477064,-0.970642202,-0.968807339,-0.966972477,-0.965137615,
-0.963302752,-0.96146789,-0.959633028,-0.957798165,-0.955963303,-0.95412844,
-0.952293578,-0.950458716,-0.948623853,-0.946788991,-0.944954128,-0.943119266,
-0.941284404,-0.939449541,-0.937614679,-0.935779817,-0.933944954,-0.932110092,
-0.930275229,-0.928440367,-0.926605505,-0.924770642,-0.92293578,-0.921100917,
-0.919266055,-0.917431193,-0.91559633,-0.913761468,-0.911926606,-0.910091743,
-0.908256881,-0.906422018,-0.904587156,-0.902752294,-0.900917431,-0.899082569,
-0.897247706,-0.895412844,-0.893577982,-0.891743119,-0.889908257,-0.888073394,
-0.886238532,-0.88440367,-0.882568807,-0.880733945,-0.878899083,-0.87706422,
-0.875229358,-0.873394495,-0.871559633,-0.869724771,-0.867889908,-0.866055046,
-0.864220183,-0.862385321,-0.860550459,-0.858715596,-0.856880734,-0.855045872,
-0.853211009,-0.851376147,-0.849541284,-0.847706422,-0.84587156,-0.844036697,
-0.842201835,-0.840366972,-0.83853211,-0.836697248,-0.834862385,-0.833027523,
-0.831192661,-0.829357798,-0.827522936,-0.825688073,-0.823853211,-0.822018349,
-0.820183486,-0.818348624,-0.816513761,-0.814678899,-0.812844037,-0.811009174,
-0.809174312,-0.80733945,-0.805504587,-0.803669725,-0.801834862,-0.8,-0.798165138,
-0.796330275,-0.794495413,-0.79266055,-0.790825688,-0.788990826,-0.787155963,
-0.785321101,-0.783486239,-0.781651376,-0.779816514,-0.777981651,-0.776146789,
-0.774311927,-0.772477064,-0.770642202,-0.768807339,-0.766972477,-0.765137615,
-0.763302752,-0.76146789,-0.759633028,-0.757798165,-0.755963303,-0.75412844,
-0.752293578,-0.750458716,-0.748623853,-0.744954128,-0.743119266,-0.741284404,
-0.739449541,-0.737614679,-0.735779817,-0.733944954,-0.732110092,-0.730275229,
-0.728440367,-0.726605505,-0.724770642,-0.72293578,-0.721100917,-0.719266055,
-0.717431193,-0.71559633,-0.713761468,-0.711926606,-0.710091743,-0.708256881,
-0.706422018,-0.704587156,-0.702752294,-0.700917431,-0.699082569,-0.697247706,
-0.695412844,-0.693577982,-0.691743119,-0.689908257,-0.688073394,-0.686238532,
-0.68440367,-0.682568807,-0.680733945,-0.678899083,-0.67706422,-0.675229358,
-0.673394495,-0.671559633,-0.669724771,-0.667889908,-0.666055046,-0.664220183,
-0.662385321,-0.660550459,-0.658715596,-0.656880734,-0.655045872,-0.653211009,
-0.651376147,-0.649541284,-0.647706422,-0.64587156,-0.644036697,-0.642201835,
-0.640366972,-0.63853211,-0.636697248,-0.634862385,-0.633027523,-0.631192661,
-0.629357798,-0.627522936,-0.625688073,-0.623853211,-0.622018349,-0.620183486,
-0.618348624,-0.616513761,-0.614678899,-0.612844037,-0.611009174,-0.609174312,
-0.60733945,-0.605504587,-0.603669725,-0.601834862,-0.6,-0.598165138,-0.596330275,
-0.594495413,-0.59266055,-0.590825688,-0.588990826,-0.587155963,-0.585321101,
-0.583486239,-0.581651376,-0.579816514,-0.577981651,-0.576146789,-0.574311927,
-0.572477064,-0.570642202,-0.568807339,-0.566972477,-0.565137615,-0.563302752,
-0.56146789,-0.559633028,-0.557798165,-0.555963303,-0.55412844,-0.552293578,
-0.550458716,-0.548623853,-0.546788991,-0.544954128,-0.543119266,-0.541284404,
-0.539449541,-0.537614679,-0.535779817,-0.533944954,-0.532110092,-0.530275229,
-0.528440367,-0.526605505,-0.524770642,-0.52293578,-0.521100917,-0.519266055,
-0.517431193,-0.51559633,-0.513761468,-0.511926606,-0.510091743,-0.508256881,
-0.506422018,-0.504587156,-0.502752294,-0.500917431,-0.499082569,-0.497247706,
-0.495412844,-0.493577982,-0.491743119,-0.489908257,-0.488073394,-0.486238532,
-0.48440367,-0.482568807,-0.480733945,-0.478899083,-0.47706422,-0.475229358,
-0.473394495,-0.471559633,-0.469724771,-0.467889908,-0.466055046,-0.464220183,
-0.462385321,-0.460550459,-0.458715596,-0.456880734,-0.455045872,-0.453211009,
-0.451376147,-0.449541284,-0.447706422,-0.44587156,-0.444036697,-0.442201835,
-0.440366972,-0.43853211,-0.436697248,-0.434862385,-0.433027523,-0.431192661,
-0.429357798,-0.427522936,-0.425688073,-0.423853211,-0.422018349,-0.420183486,
-0.418348624,-0.416513761,-0.414678899,-0.412844037,-0.411009174,-0.409174312,
-0.40733945,-0.405504587,-0.403669725,-0.401834862,-0.4,-0.398165138,-0.396330275,
-0.394495413,-0.39266055,-0.390825688,-0.388990826,-0.387155963,-0.385321101,
-0.383486239,-0.381651376,-0.379816514,-0.377981651,-0.376146789,-0.374311927,
-0.372477064,-0.370642202,-0.368807339,-0.366972477,-0.365137615,-0.363302752,
-0.36146789,-0.359633028,-0.357798165,-0.355963303,-0.35412844,-0.352293578,
-0.350458716,-0.348623853,-0.346788991,-0.344954128,-0.343119266,-0.341284404,
-0.339449541,-0.337614679,-0.335779817,-0.333944954,-0.332110092,-0.328440367,
-0.326605505,-0.324770642,-0.32293578,-0.321100917,-0.319266055,-0.317431193,
-0.31559633,-0.313761468,-0.311926606,-0.310091743,-0.308256881,-0.306422018,
-0.304587156,-0.302752294,-0.300917431,-0.299082569,-0.297247706,-0.295412844,
-0.293577982,-0.291743119,-0.289908257,-0.288073394,-0.286238532,-0.28440367,
-0.282568807,-0.280733945,-0.278899083,-0.27706422,-0.275229358,-0.273394495,
-0.271559633,-0.269724771,-0.267889908,-0.266055046,-0.264220183,-0.262385321,
-0.260550459,-0.258715596,-0.256880734,-0.255045872,-0.253211009,-0.251376147,
-0.249541284,-0.247706422,-0.24587156,-0.244036697,-0.242201835,-0.240366972,
-0.23853211,-0.236697248,-0.234862385,-0.233027523,-0.231192661,-0.229357798,
-0.227522936,-0.225688073,-0.223853211,-0.222018349,-0.220183486,-0.218348624,
-0.216513761,-0.214678899,-0.212844037,-0.211009174,-0.209174312,-0.20733945,
-0.205504587,-0.203669725,-0.201834862,-0.2,-0.198165138,-0.196330275,-0.194495413,
-0.19266055,-0.190825688,-0.188990826,-0.187155963,-0.185321101,-0.183486239,
-0.181651376,-0.179816514,-0.177981651,-0.176146789,-0.174311927,-0.172477064,
-0.170642202,-0.168807339,-0.166972477,-0.165137615,-0.163302752,-0.16146789,
-0.159633028,-0.157798165,-0.155963303,-0.15412844,-0.152293578,-0.150458716,
-0.148623853,-0.146788991,-0.144954128,-0.143172102),.UNSPECIFIED.);
#24340=B_SPLINE_CURVE_WITH_KNOTS('',5,(#172440,#172441,#172442,#172443,
#172444,#172445,#172446,#172447,#172448,#172449,#172450,#172451,#172452,
#172453,#172454,#172455,#172456,#172457,#172458,#172459,#172460,#172461,
#172462,#172463,#172464,#172465,#172466,#172467,#172468,#172469,#172470,
#172471,#172472,#172473,#172474,#172475,#172476,#172477,#172478,#172479,
#172480,#172481,#172482,#172483,#172484,#172485,#172486,#172487,#172488,
#172489,#172490,#172491,#172492,#172493,#172494,#172495,#172496,#172497,
#172498,#172499,#172500,#172501,#172502,#172503,#172504,#172505,#172506,
#172507,#172508,#172509,#172510,#172511,#172512,#172513,#172514,#172515,
#172516,#172517,#172518,#172519,#172520,#172521,#172522,#172523,#172524,
#172525,#172526,#172527,#172528,#172529,#172530,#172531,#172532,#172533,
#172534,#172535,#172536,#172537,#172538,#172539,#172540,#172541,#172542,
#172543,#172544,#172545,#172546,#172547,#172548,#172549,#172550,#172551,
#172552,#172553,#172554,#172555,#172556,#172557,#172558,#172559,#172560,
#172561,#172562,#172563,#172564,#172565,#172566,#172567,#172568,#172569,
#172570,#172571,#172572,#172573,#172574,#172575,#172576,#172577,#172578,
#172579,#172580,#172581,#172582,#172583,#172584,#172585,#172586,#172587,
#172588,#172589,#172590,#172591,#172592,#172593,#172594,#172595,#172596,
#172597,#172598,#172599,#172600,#172601,#172602,#172603,#172604,#172605,
#172606,#172607,#172608,#172609,#172610,#172611,#172612,#172613,#172614,
#172615,#172616,#172617,#172618,#172619,#172620,#172621,#172622,#172623,
#172624,#172625,#172626,#172627,#172628,#172629,#172630,#172631,#172632,
#172633,#172634,#172635,#172636,#172637,#172638,#172639,#172640,#172641,
#172642,#172643,#172644,#172645,#172646,#172647,#172648,#172649,#172650,
#172651,#172652,#172653,#172654,#172655,#172656,#172657,#172658,#172659,
#172660,#172661,#172662,#172663,#172664,#172665,#172666,#172667,#172668,
#172669,#172670,#172671,#172672,#172673,#172674,#172675,#172676,#172677,
#172678,#172679,#172680,#172681,#172682,#172683,#172684,#172685,#172686,
#172687,#172688,#172689,#172690,#172691,#172692,#172693,#172694,#172695,
#172696,#172697,#172698,#172699,#172700,#172701,#172702,#172703,#172704,
#172705,#172706,#172707,#172708,#172709,#172710,#172711,#172712,#172713,
#172714,#172715,#172716,#172717,#172718,#172719,#172720,#172721,#172722,
#172723,#172724,#172725,#172726,#172727,#172728,#172729,#172730,#172731,
#172732,#172733,#172734,#172735,#172736,#172737,#172738,#172739,#172740,
#172741,#172742,#172743,#172744,#172745,#172746,#172747,#172748,#172749,
#172750,#172751,#172752,#172753,#172754,#172755,#172756,#172757,#172758,
#172759,#172760,#172761,#172762,#172763,#172764,#172765,#172766,#172767,
#172768,#172769,#172770,#172771,#172772,#172773,#172774,#172775,#172776,
#172777,#172778,#172779,#172780,#172781,#172782,#172783,#172784,#172785,
#172786,#172787,#172788,#172789,#172790,#172791,#172792,#172793,#172794,
#172795,#172796,#172797,#172798,#172799,#172800,#172801,#172802,#172803,
#172804,#172805,#172806,#172807,#172808,#172809,#172810,#172811,#172812,
#172813,#172814,#172815,#172816,#172817,#172818,#172819,#172820,#172821,
#172822,#172823,#172824,#172825,#172826,#172827,#172828,#172829,#172830,
#172831,#172832,#172833,#172834,#172835,#172836,#172837,#172838,#172839,
#172840,#172841,#172842,#172843,#172844,#172845,#172846,#172847,#172848,
#172849,#172850,#172851,#172852,#172853,#172854,#172855,#172856,#172857,
#172858,#172859,#172860,#172861,#172862,#172863,#172864,#172865,#172866,
#172867,#172868,#172869,#172870,#172871,#172872,#172873,#172874,#172875,
#172876,#172877,#172878,#172879,#172880,#172881,#172882,#172883,#172884,
#172885,#172886,#172887,#172888,#172889,#172890,#172891,#172892,#172893,
#172894,#172895,#172896,#172897,#172898,#172899,#172900,#172901,#172902,
#172903,#172904,#172905,#172906,#172907,#172908),.UNSPECIFIED.,.F.,.F.,
(6,1,1,1,1,1,1,1,1,1,1,1,1,1,1,1,1,1,1,1,1,1,1,1,1,1,1,1,1,1,1,1,1,1,1,
1,1,1,1,1,1,1,1,1,1,1,1,1,1,1,1,1,1,1,1,1,1,1,1,1,1,1,1,1,1,1,1,1,1,1,1,
1,1,1,1,1,1,1,1,1,1,1,1,1,1,1,1,1,1,1,1,1,1,1,1,1,1,1,1,1,1,1,1,1,1,1,1,
1,1,1,1,1,1,1,1,1,1,1,1,1,1,1,1,1,1,1,1,1,1,1,1,1,1,1,1,1,1,1,1,1,1,1,1,
1,1,1,1,1,1,1,1,1,1,1,1,1,1,1,1,1,1,1,1,1,1,1,1,1,1,1,1,1,1,1,1,1,1,1,1,
1,1,1,1,1,1,1,1,1,1,1,1,1,1,1,1,1,1,1,1,1,1,1,1,1,1,1,1,1,1,1,1,1,1,1,1,
1,1,1,1,1,1,1,1,1,1,1,1,1,1,1,1,1,1,1,1,1,1,1,1,1,1,1,1,1,1,1,1,1,1,1,1,
1,1,1,1,1,1,1,1,1,1,1,1,1,1,1,1,1,1,1,1,1,1,1,1,1,1,1,1,1,1,1,1,1,1,1,1,
1,1,1,1,1,1,1,1,1,1,1,1,1,1,1,1,1,1,1,1,1,1,1,1,1,1,1,1,1,1,1,1,1,1,1,1,
1,1,1,1,1,1,1,1,1,1,1,1,1,1,1,1,1,1,1,1,1,1,1,1,1,1,1,1,1,1,1,1,1,1,1,1,
1,1,1,1,1,1,1,1,1,1,1,1,1,1,1,1,1,1,1,1,1,1,1,1,1,1,1,1,1,1,1,1,1,1,1,1,
1,1,1,1,1,1,1,1,1,1,1,1,1,1,1,1,1,1,1,1,1,1,1,1,1,1,1,1,1,1,1,1,1,1,1,1,
1,1,1,1,1,1,1,1,1,1,1,1,1,1,1,1,1,1,1,1,1,1,1,1,1,1,1,1,1,1,1,1,1,6),(0.143172102,
0.144954128,0.146788991,0.148623853,0.150458716,0.152293578,0.15412844,
0.155963303,0.157798165,0.159633028,0.16146789,0.163302752,0.165137615,
0.166972477,0.168807339,0.170642202,0.172477064,0.174311927,0.176146789,
0.177981651,0.179816514,0.181651376,0.183486239,0.185321101,0.187155963,
0.188990826,0.190825688,0.19266055,0.194495413,0.196330275,0.198165138,
0.2,0.201834862,0.203669725,0.205504587,0.20733945,0.209174312,0.211009174,
0.212844037,0.214678899,0.216513761,0.218348624,0.220183486,0.222018349,
0.223853211,0.225688073,0.227522936,0.229357798,0.231192661,0.233027523,
0.234862385,0.236697248,0.23853211,0.240366972,0.242201835,0.244036697,
0.24587156,0.247706422,0.249541284,0.251376147,0.253211009,0.255045872,
0.256880734,0.258715596,0.260550459,0.262385321,0.264220183,0.266055046,
0.267889908,0.269724771,0.271559633,0.273394495,0.275229358,0.27706422,
0.278899083,0.280733945,0.282568807,0.28440367,0.286238532,0.288073394,
0.289908257,0.291743119,0.293577982,0.295412844,0.297247706,0.299082569,
0.300917431,0.302752294,0.304587156,0.306422018,0.308256881,0.310091743,
0.311926606,0.313761468,0.31559633,0.317431193,0.319266055,0.321100917,
0.32293578,0.324770642,0.326605505,0.328440367,0.332110092,0.333944954,
0.335779817,0.337614679,0.339449541,0.341284404,0.343119266,0.344954128,
0.346788991,0.348623853,0.350458716,0.352293578,0.35412844,0.355963303,
0.357798165,0.359633028,0.36146789,0.363302752,0.365137615,0.366972477,
0.368807339,0.370642202,0.372477064,0.374311927,0.376146789,0.377981651,
0.379816514,0.381651376,0.383486239,0.385321101,0.387155963,0.388990826,
0.390825688,0.39266055,0.394495413,0.396330275,0.398165138,0.4,0.401834862,
0.403669725,0.405504587,0.40733945,0.409174312,0.411009174,0.412844037,
0.414678899,0.416513761,0.418348624,0.420183486,0.422018349,0.423853211,
0.425688073,0.427522936,0.429357798,0.431192661,0.433027523,0.434862385,
0.436697248,0.43853211,0.440366972,0.442201835,0.444036697,0.44587156,0.447706422,
0.449541284,0.451376147,0.453211009,0.455045872,0.456880734,0.458715596,
0.460550459,0.462385321,0.464220183,0.466055046,0.467889908,0.469724771,
0.471559633,0.473394495,0.475229358,0.47706422,0.478899083,0.480733945,
0.482568807,0.48440367,0.486238532,0.488073394,0.489908257,0.491743119,
0.493577982,0.495412844,0.497247706,0.499082569,0.500917431,0.502752294,
0.504587156,0.506422018,0.508256881,0.510091743,0.511926606,0.513761468,
0.51559633,0.517431193,0.519266055,0.521100917,0.52293578,0.524770642,0.526605505,
0.528440367,0.530275229,0.532110092,0.533944954,0.535779817,0.537614679,
0.539449541,0.541284404,0.543119266,0.544954128,0.546788991,0.548623853,
0.550458716,0.552293578,0.55412844,0.555963303,0.557798165,0.559633028,
0.56146789,0.563302752,0.565137615,0.566972477,0.568807339,0.570642202,
0.572477064,0.574311927,0.576146789,0.577981651,0.579816514,0.581651376,
0.583486239,0.585321101,0.587155963,0.588990826,0.590825688,0.59266055,
0.594495413,0.596330275,0.598165138,0.6,0.601834862,0.603669725,0.605504587,
0.60733945,0.609174312,0.611009174,0.612844037,0.614678899,0.616513761,
0.618348624,0.620183486,0.622018349,0.623853211,0.625688073,0.627522936,
0.629357798,0.631192661,0.633027523,0.634862385,0.636697248,0.63853211,
0.640366972,0.642201835,0.644036697,0.64587156,0.647706422,0.649541284,
0.651376147,0.653211009,0.655045872,0.656880734,0.658715596,0.660550459,
0.662385321,0.664220183,0.666055046,0.667889908,0.669724771,0.671559633,
0.673394495,0.675229358,0.67706422,0.678899083,0.680733945,0.682568807,
0.68440367,0.686238532,0.688073394,0.689908257,0.691743119,0.693577982,
0.695412844,0.697247706,0.699082569,0.700917431,0.702752294,0.704587156,
0.706422018,0.708256881,0.710091743,0.711926606,0.713761468,0.71559633,
0.717431193,0.719266055,0.721100917,0.72293578,0.724770642,0.726605505,
0.728440367,0.730275229,0.732110092,0.733944954,0.735779817,0.737614679,
0.739449541,0.741284404,0.743119266,0.744954128,0.748623853,0.750458716,
0.752293578,0.75412844,0.755963303,0.757798165,0.759633028,0.76146789,0.763302752,
0.765137615,0.766972477,0.768807339,0.770642202,0.772477064,0.774311927,
0.776146789,0.777981651,0.779816514,0.781651376,0.783486239,0.785321101,
0.787155963,0.788990826,0.790825688,0.79266055,0.794495413,0.796330275,
0.798165138,0.8,0.801834862,0.803669725,0.805504587,0.80733945,0.809174312,
0.811009174,0.812844037,0.814678899,0.816513761,0.818348624,0.820183486,
0.822018349,0.823853211,0.825688073,0.827522936,0.829357798,0.831192661,
0.833027523,0.834862385,0.836697248,0.83853211,0.840366972,0.842201835,
0.844036697,0.84587156,0.847706422,0.849541284,0.851376147,0.853211009,
0.855045872,0.856880734,0.858715596,0.860550459,0.862385321,0.864220183,
0.866055046,0.867889908,0.869724771,0.871559633,0.873394495,0.875229358,
0.87706422,0.878899083,0.880733945,0.882568807,0.88440367,0.886238532,0.888073394,
0.889908257,0.891743119,0.893577982,0.895412844,0.897247706,0.899082569,
0.900917431,0.902752294,0.904587156,0.906422018,0.908256881,0.910091743,
0.911926606,0.913761468,0.91559633,0.917431193,0.919266055,0.921100917,
0.92293578,0.924770642,0.926605505,0.928440367,0.930275229,0.932110092,
0.933944954,0.935779817,0.937614679,0.939449541,0.941284404,0.943119266,
0.944954128,0.946788991,0.948623853,0.950458716,0.952293578,0.95412844,
0.955963303,0.957798165,0.959633028,0.96146789,0.963302752,0.965137615,
0.966972477,0.968807339,0.970642202,0.972477064,0.974311927,0.977981651,
0.979816514,0.981651376,0.983486239,0.985321101,0.987155963,0.988990826,
0.990825688,0.99266055,0.994495413,0.996330275,0.998165138,1.),
 .UNSPECIFIED.);
#24341=B_SPLINE_CURVE_WITH_KNOTS('',3,(#173853,#173854,#173855,#173856,
#173857,#173858,#173859,#173860,#173861,#173862,#173863,#173864,#173865,
#173866,#173867,#173868,#173869,#173870,#173871,#173872,#173873,#173874,
#173875,#173876,#173877,#173878,#173879,#173880,#173881,#173882,#173883,
#173884,#173885,#173886,#173887,#173888,#173889,#173890,#173891,#173892,
#173893,#173894,#173895,#173896,#173897,#173898,#173899,#173900,#173901,
#173902,#173903,#173904,#173905,#173906,#173907,#173908,#173909,#173910,
#173911,#173912,#173913,#173914,#173915,#173916,#173917,#173918,#173919,
#173920,#173921,#173922,#173923,#173924,#173925,#173926,#173927,#173928,
#173929,#173930,#173931,#173932,#173933,#173934,#173935,#173936,#173937,
#173938,#173939,#173940,#173941,#173942,#173943,#173944,#173945,#173946,
#173947,#173948,#173949,#173950,#173951,#173952,#173953,#173954,#173955,
#173956,#173957,#173958,#173959,#173960,#173961,#173962,#173963,#173964,
#173965,#173966,#173967,#173968,#173969,#173970,#173971,#173972,#173973,
#173974,#173975,#173976,#173977,#173978,#173979,#173980,#173981,#173982,
#173983,#173984,#173985,#173986,#173987,#173988,#173989,#173990,#173991,
#173992,#173993,#173994,#173995,#173996,#173997,#173998,#173999,#174000,
#174001,#174002,#174003,#174004,#174005,#174006,#174007,#174008,#174009,
#174010,#174011,#174012,#174013,#174014,#174015,#174016,#174017,#174018,
#174019,#174020,#174021,#174022,#174023,#174024,#174025,#174026,#174027,
#174028,#174029,#174030,#174031,#174032,#174033,#174034,#174035,#174036,
#174037,#174038,#174039,#174040,#174041,#174042,#174043,#174044,#174045,
#174046,#174047,#174048,#174049,#174050,#174051,#174052,#174053,#174054,
#174055,#174056,#174057,#174058,#174059,#174060,#174061,#174062,#174063,
#174064,#174065,#174066,#174067,#174068,#174069,#174070,#174071,#174072,
#174073,#174074,#174075,#174076,#174077,#174078,#174079,#174080,#174081,
#174082,#174083,#174084,#174085,#174086,#174087,#174088,#174089,#174090,
#174091,#174092,#174093,#174094,#174095,#174096,#174097,#174098,#174099,
#174100,#174101,#174102,#174103,#174104,#174105,#174106,#174107,#174108,
#174109,#174110,#174111,#174112,#174113,#174114,#174115,#174116,#174117,
#174118,#174119,#174120,#174121,#174122,#174123,#174124,#174125,#174126,
#174127,#174128,#174129,#174130,#174131,#174132,#174133,#174134,#174135,
#174136,#174137,#174138,#174139,#174140,#174141,#174142,#174143,#174144,
#174145,#174146,#174147,#174148,#174149,#174150,#174151,#174152,#174153,
#174154,#174155,#174156,#174157,#174158,#174159,#174160,#174161,#174162,
#174163,#174164,#174165,#174166,#174167,#174168,#174169,#174170,#174171,
#174172,#174173,#174174),.UNSPECIFIED.,.F.,.F.,(4,3,3,3,3,3,3,3,3,3,3,3,
3,3,3,3,3,3,3,3,3,3,3,3,3,3,3,3,3,3,3,3,3,3,3,3,3,3,3,3,3,3,3,3,3,3,3,3,
3,3,3,3,3,3,3,3,3,3,3,3,3,3,3,3,3,3,3,3,3,3,3,3,3,3,3,3,3,3,3,3,3,3,3,3,
3,3,3,3,3,3,3,3,3,3,3,3,3,3,3,3,3,3,3,3,3,3,3,4),(0.143172102,0.15412844,
0.165137615,0.176146789,0.187155963,0.198165138,0.209174312,0.220183486,
0.231192661,0.242201835,0.253211009,0.264220183,0.275229358,0.286238532,
0.297247706,0.308256881,0.319266055,0.330275229,0.341284404,0.352293578,
0.365137615,0.376146789,0.387155963,0.396330275,0.405504587,0.414678899,
0.423853211,0.433027523,0.442201835,0.451376147,0.460550459,0.469724771,
0.478899083,0.488073394,0.497247706,0.508256881,0.517431193,0.526605505,
0.533944954,0.541284404,0.548623853,0.555963303,0.563302752,0.570642202,
0.577981651,0.588990826,0.598165138,0.605504587,0.612844037,0.620183486,
0.627522936,0.636697248,0.644036697,0.651376147,0.658715596,0.666055046,
0.673394495,0.680733945,0.688073394,0.695412844,0.704587156,0.711926606,
0.719266055,0.726605505,0.735779817,0.743119266,0.750458716,0.757798165,
0.765137615,0.772477064,0.779816514,0.787155963,0.794495413,0.801834862,
0.809174312,0.816513761,0.822018349,0.827522936,0.833027523,0.840366972,
0.84587156,0.851376147,0.856880734,0.862385321,0.867889908,0.873394495,
0.878899083,0.88440367,0.889908257,0.895412844,0.902752294,0.908256881,
0.913761468,0.919266055,0.924770642,0.930275229,0.935779817,0.941284404,
0.946788991,0.952293578,0.957798165,0.963302752,0.970642202,0.976146789,
0.981651376,0.987155963,0.99266055,1.),.UNSPECIFIED.);
#24342=B_SPLINE_CURVE_WITH_KNOTS('',3,(#174175,#174176,#174177,#174178,
#174179,#174180,#174181,#174182,#174183,#174184,#174185,#174186,#174187,
#174188,#174189,#174190,#174191,#174192,#174193,#174194,#174195,#174196,
#174197,#174198,#174199,#174200,#174201,#174202,#174203,#174204,#174205,
#174206,#174207,#174208,#174209,#174210,#174211,#174212,#174213,#174214,
#174215,#174216,#174217,#174218,#174219,#174220,#174221,#174222,#174223,
#174224,#174225,#174226,#174227,#174228,#174229,#174230,#174231,#174232,
#174233,#174234,#174235,#174236,#174237,#174238,#174239,#174240,#174241,
#174242,#174243,#174244,#174245,#174246,#174247,#174248,#174249,#174250,
#174251,#174252,#174253,#174254,#174255,#174256,#174257,#174258,#174259,
#174260,#174261,#174262,#174263,#174264,#174265,#174266,#174267,#174268,
#174269,#174270,#174271,#174272,#174273,#174274,#174275,#174276,#174277,
#174278,#174279,#174280,#174281,#174282,#174283,#174284,#174285,#174286,
#174287,#174288,#174289,#174290,#174291,#174292,#174293,#174294,#174295,
#174296,#174297,#174298,#174299,#174300,#174301,#174302,#174303,#174304,
#174305,#174306,#174307,#174308,#174309,#174310,#174311,#174312,#174313,
#174314,#174315,#174316,#174317,#174318,#174319,#174320,#174321,#174322,
#174323,#174324,#174325,#174326,#174327,#174328,#174329,#174330,#174331,
#174332,#174333,#174334,#174335,#174336,#174337,#174338,#174339,#174340,
#174341,#174342,#174343,#174344,#174345,#174346,#174347,#174348,#174349,
#174350,#174351,#174352,#174353,#174354,#174355,#174356,#174357,#174358,
#174359,#174360,#174361,#174362,#174363,#174364,#174365,#174366,#174367,
#174368,#174369,#174370,#174371,#174372,#174373,#174374,#174375,#174376,
#174377,#174378,#174379,#174380,#174381,#174382,#174383,#174384,#174385,
#174386,#174387,#174388,#174389,#174390,#174391,#174392,#174393,#174394,
#174395,#174396,#174397,#174398,#174399,#174400,#174401,#174402,#174403,
#174404,#174405,#174406,#174407,#174408,#174409,#174410,#174411,#174412,
#174413,#174414,#174415,#174416,#174417,#174418,#174419,#174420,#174421,
#174422,#174423,#174424,#174425,#174426,#174427,#174428,#174429,#174430,
#174431,#174432,#174433,#174434,#174435,#174436,#174437,#174438,#174439,
#174440,#174441,#174442,#174443,#174444,#174445,#174446,#174447,#174448,
#174449,#174450,#174451,#174452,#174453,#174454,#174455,#174456,#174457,
#174458,#174459,#174460,#174461,#174462,#174463,#174464,#174465,#174466,
#174467,#174468,#174469,#174470,#174471,#174472,#174473,#174474,#174475,
#174476,#174477,#174478,#174479,#174480,#174481,#174482,#174483,#174484,
#174485,#174486,#174487,#174488,#174489,#174490,#174491,#174492,#174493,
#174494,#174495,#174496),.UNSPECIFIED.,.F.,.F.,(4,3,3,3,3,3,3,3,3,3,3,3,
3,3,3,3,3,3,3,3,3,3,3,3,3,3,3,3,3,3,3,3,3,3,3,3,3,3,3,3,3,3,3,3,3,3,3,3,
3,3,3,3,3,3,3,3,3,3,3,3,3,3,3,3,3,3,3,3,3,3,3,3,3,3,3,3,3,3,3,3,3,3,3,3,
3,3,3,3,3,3,3,3,3,3,3,3,3,3,3,3,3,3,3,3,3,3,3,4),(0.143172102,0.15412844,
0.165137615,0.176146789,0.187155963,0.198165138,0.209174312,0.220183486,
0.231192661,0.242201835,0.253211009,0.264220183,0.275229358,0.286238532,
0.297247706,0.308256881,0.319266055,0.330275229,0.341284404,0.352293578,
0.363302752,0.374311927,0.385321101,0.396330275,0.405504587,0.414678899,
0.423853211,0.433027523,0.442201835,0.451376147,0.460550459,0.469724771,
0.478899083,0.488073394,0.497247706,0.508256881,0.517431193,0.526605505,
0.533944954,0.541284404,0.548623853,0.557798165,0.565137615,0.572477064,
0.579816514,0.587155963,0.594495413,0.601834862,0.609174312,0.616513761,
0.623853211,0.631192661,0.63853211,0.64587156,0.653211009,0.660550459,0.667889908,
0.675229358,0.682568807,0.689908257,0.697247706,0.704587156,0.711926606,
0.719266055,0.726605505,0.733944954,0.743119266,0.750458716,0.757798165,
0.765137615,0.772477064,0.779816514,0.787155963,0.794495413,0.801834862,
0.809174312,0.814678899,0.820183486,0.825688073,0.831192661,0.83853211,
0.844036697,0.849541284,0.855045872,0.860550459,0.867889908,0.873394495,
0.878899083,0.88440367,0.889908257,0.895412844,0.900917431,0.906422018,
0.911926606,0.917431193,0.92293578,0.930275229,0.937614679,0.943119266,
0.948623853,0.95412844,0.96146789,0.966972477,0.974311927,0.979816514,0.985321101,
0.994495413,1.),.UNSPECIFIED.);
#24343=B_SPLINE_CURVE_WITH_KNOTS('',3,(#175456,#175457,#175458,#175459,
#175460,#175461,#175462,#175463,#175464,#175465,#175466,#175467,#175468,
#175469,#175470,#175471,#175472,#175473,#175474,#175475,#175476,#175477,
#175478,#175479,#175480,#175481,#175482,#175483,#175484,#175485,#175486,
#175487,#175488,#175489,#175490,#175491,#175492,#175493,#175494,#175495,
#175496,#175497,#175498,#175499,#175500,#175501,#175502,#175503,#175504,
#175505,#175506,#175507,#175508,#175509,#175510,#175511,#175512,#175513,
#175514,#175515,#175516,#175517,#175518,#175519,#175520,#175521,#175522,
#175523,#175524,#175525,#175526,#175527,#175528,#175529,#175530,#175531,
#175532,#175533,#175534,#175535,#175536,#175537,#175538,#175539,#175540,
#175541,#175542,#175543,#175544,#175545,#175546,#175547,#175548,#175549,
#175550,#175551,#175552,#175553,#175554,#175555,#175556,#175557,#175558,
#175559,#175560,#175561,#175562,#175563,#175564,#175565,#175566,#175567,
#175568,#175569,#175570,#175571,#175572,#175573,#175574,#175575,#175576,
#175577,#175578,#175579,#175580,#175581,#175582,#175583,#175584,#175585,
#175586,#175587,#175588,#175589,#175590,#175591,#175592,#175593,#175594,
#175595,#175596,#175597,#175598,#175599,#175600,#175601,#175602,#175603,
#175604,#175605,#175606,#175607,#175608,#175609,#175610,#175611,#175612,
#175613,#175614,#175615,#175616,#175617,#175618,#175619,#175620,#175621,
#175622,#175623,#175624,#175625,#175626,#175627,#175628,#175629,#175630,
#175631,#175632,#175633,#175634,#175635,#175636,#175637,#175638,#175639,
#175640,#175641,#175642,#175643,#175644,#175645,#175646,#175647,#175648,
#175649,#175650,#175651,#175652,#175653,#175654,#175655,#175656,#175657,
#175658,#175659,#175660,#175661,#175662,#175663,#175664,#175665,#175666,
#175667,#175668,#175669,#175670,#175671,#175672,#175673,#175674,#175675,
#175676,#175677,#175678,#175679,#175680,#175681,#175682,#175683,#175684,
#175685,#175686,#175687,#175688,#175689,#175690,#175691,#175692,#175693,
#175694,#175695,#175696,#175697,#175698,#175699,#175700,#175701,#175702,
#175703,#175704,#175705,#175706,#175707,#175708,#175709,#175710,#175711,
#175712,#175713,#175714,#175715,#175716,#175717,#175718,#175719,#175720,
#175721,#175722,#175723,#175724,#175725,#175726,#175727,#175728,#175729,
#175730,#175731,#175732,#175733,#175734,#175735,#175736,#175737,#175738,
#175739,#175740,#175741,#175742,#175743,#175744,#175745,#175746,#175747,
#175748,#175749,#175750,#175751,#175752,#175753,#175754,#175755,#175756,
#175757,#175758,#175759,#175760,#175761,#175762,#175763,#175764,#175765,
#175766,#175767,#175768,#175769,#175770,#175771,#175772,#175773,#175774,
#175775,#175776,#175777,#175778,#175779,#175780),.UNSPECIFIED.,.F.,.F.,
(4,3,3,3,3,3,3,3,3,3,3,3,3,3,3,3,3,3,3,3,3,3,3,3,3,3,3,3,3,3,3,3,3,3,3,
3,3,3,3,3,3,3,3,3,3,3,3,3,3,3,3,3,3,3,3,3,3,3,3,3,3,3,3,3,3,3,3,3,3,3,3,
3,3,3,3,3,3,3,3,3,3,3,3,3,3,3,3,3,3,3,3,3,3,3,3,3,3,3,3,3,3,3,3,3,3,3,3,
3,4),(0.143172102,0.15412844,0.165137615,0.176146789,0.187155963,0.198165138,
0.209174312,0.220183486,0.231192661,0.242201835,0.253211009,0.264220183,
0.275229358,0.286238532,0.297247706,0.308256881,0.319266055,0.330275229,
0.341284404,0.352293578,0.363302752,0.374311927,0.385321101,0.396330275,
0.405504587,0.414678899,0.423853211,0.433027523,0.442201835,0.451376147,
0.462385321,0.471559633,0.480733945,0.489908257,0.499082569,0.508256881,
0.517431193,0.526605505,0.533944954,0.541284404,0.548623853,0.555963303,
0.563302752,0.570642202,0.577981651,0.585321101,0.59266055,0.6,0.60733945,
0.614678899,0.622018349,0.631192661,0.63853211,0.64587156,0.655045872,0.662385321,
0.671559633,0.678899083,0.686238532,0.693577982,0.700917431,0.708256881,
0.71559633,0.72293578,0.730275229,0.737614679,0.744954128,0.752293578,0.759633028,
0.766972477,0.774311927,0.781651376,0.788990826,0.796330275,0.803669725,
0.811009174,0.816513761,0.822018349,0.827522936,0.833027523,0.840366972,
0.84587156,0.851376147,0.856880734,0.862385321,0.867889908,0.873394495,
0.878899083,0.88440367,0.889908257,0.895412844,0.900917431,0.906422018,
0.911926606,0.917431193,0.92293578,0.928440367,0.935779817,0.941284404,
0.946788991,0.952293578,0.957798165,0.963302752,0.970642202,0.976146789,
0.983486239,0.988990826,0.994495413,1.),.UNSPECIFIED.);
#24344=B_SPLINE_CURVE_WITH_KNOTS('',3,(#175781,#175782,#175783,#175784,
#175785,#175786,#175787,#175788,#175789,#175790,#175791,#175792,#175793,
#175794,#175795,#175796,#175797,#175798,#175799,#175800,#175801,#175802,
#175803,#175804,#175805,#175806,#175807,#175808,#175809,#175810,#175811,
#175812,#175813,#175814,#175815,#175816,#175817,#175818,#175819,#175820,
#175821,#175822,#175823,#175824,#175825,#175826,#175827,#175828,#175829,
#175830,#175831,#175832,#175833,#175834,#175835,#175836,#175837,#175838,
#175839,#175840,#175841,#175842,#175843,#175844,#175845,#175846,#175847,
#175848,#175849,#175850,#175851,#175852,#175853,#175854,#175855,#175856,
#175857,#175858,#175859,#175860,#175861,#175862,#175863,#175864,#175865,
#175866,#175867,#175868,#175869,#175870,#175871,#175872,#175873,#175874,
#175875,#175876,#175877,#175878,#175879,#175880,#175881,#175882,#175883,
#175884,#175885,#175886,#175887,#175888,#175889,#175890,#175891,#175892,
#175893,#175894,#175895,#175896,#175897,#175898,#175899,#175900,#175901,
#175902,#175903,#175904,#175905,#175906,#175907,#175908,#175909,#175910,
#175911,#175912,#175913,#175914,#175915,#175916,#175917,#175918,#175919,
#175920,#175921,#175922,#175923,#175924,#175925,#175926,#175927,#175928,
#175929,#175930,#175931,#175932,#175933,#175934,#175935,#175936,#175937,
#175938,#175939,#175940,#175941,#175942,#175943,#175944,#175945,#175946,
#175947,#175948,#175949,#175950,#175951,#175952,#175953,#175954,#175955,
#175956,#175957,#175958,#175959,#175960,#175961,#175962,#175963,#175964,
#175965,#175966,#175967,#175968,#175969,#175970,#175971,#175972,#175973,
#175974,#175975,#175976,#175977,#175978,#175979,#175980,#175981,#175982,
#175983,#175984,#175985,#175986,#175987,#175988,#175989,#175990,#175991,
#175992,#175993,#175994,#175995,#175996,#175997,#175998,#175999,#176000,
#176001,#176002,#176003,#176004,#176005,#176006,#176007,#176008,#176009,
#176010,#176011,#176012,#176013,#176014,#176015,#176016,#176017,#176018,
#176019,#176020,#176021,#176022,#176023,#176024,#176025,#176026,#176027,
#176028,#176029,#176030,#176031,#176032,#176033,#176034,#176035,#176036,
#176037,#176038,#176039,#176040,#176041,#176042,#176043,#176044,#176045,
#176046,#176047,#176048,#176049,#176050,#176051,#176052,#176053,#176054,
#176055,#176056,#176057,#176058,#176059,#176060,#176061,#176062,#176063,
#176064,#176065,#176066,#176067,#176068,#176069,#176070,#176071,#176072,
#176073,#176074,#176075,#176076,#176077,#176078,#176079,#176080,#176081,
#176082,#176083,#176084,#176085,#176086,#176087,#176088,#176089,#176090,
#176091,#176092,#176093,#176094,#176095,#176096,#176097,#176098,#176099,
#176100,#176101,#176102,#176103,#176104,#176105,#176106,#176107,#176108),
 .UNSPECIFIED.,.F.,.F.,(4,3,3,3,3,3,3,3,3,3,3,3,3,3,3,3,3,3,3,3,3,3,3,3,
3,3,3,3,3,3,3,3,3,3,3,3,3,3,3,3,3,3,3,3,3,3,3,3,3,3,3,3,3,3,3,3,3,3,3,3,
3,3,3,3,3,3,3,3,3,3,3,3,3,3,3,3,3,3,3,3,3,3,3,3,3,3,3,3,3,3,3,3,3,3,3,3,
3,3,3,3,3,3,3,3,3,3,3,3,3,4),(0.143172102,0.15412844,0.165137615,0.176146789,
0.187155963,0.198165138,0.209174312,0.220183486,0.231192661,0.242201835,
0.253211009,0.264220183,0.275229358,0.286238532,0.297247706,0.308256881,
0.319266055,0.330275229,0.341284404,0.352293578,0.363302752,0.374311927,
0.385321101,0.396330275,0.405504587,0.414678899,0.423853211,0.433027523,
0.442201835,0.451376147,0.460550459,0.469724771,0.478899083,0.488073394,
0.497247706,0.506422018,0.51559633,0.524770642,0.533944954,0.541284404,
0.548623853,0.555963303,0.563302752,0.570642202,0.577981651,0.585321101,
0.59266055,0.6,0.60733945,0.614678899,0.622018349,0.629357798,0.636697248,
0.644036697,0.651376147,0.658715596,0.666055046,0.673394495,0.680733945,
0.688073394,0.695412844,0.704587156,0.711926606,0.719266055,0.726605505,
0.733944954,0.741284404,0.748623853,0.755963303,0.763302752,0.770642202,
0.777981651,0.785321101,0.79266055,0.8,0.809174312,0.814678899,0.820183486,
0.825688073,0.831192661,0.836697248,0.842201835,0.847706422,0.853211009,
0.858715596,0.864220183,0.869724771,0.875229358,0.880733945,0.886238532,
0.891743119,0.897247706,0.902752294,0.908256881,0.913761468,0.919266055,
0.924770642,0.930275229,0.935779817,0.941284404,0.946788991,0.952293578,
0.957798165,0.963302752,0.970642202,0.976146789,0.981651376,0.987155963,
0.99266055,1.),.UNSPECIFIED.);
#24345=B_SPLINE_CURVE_WITH_KNOTS('',3,(#177056,#177057,#177058,#177059,
#177060,#177061,#177062,#177063,#177064,#177065,#177066,#177067,#177068,
#177069,#177070,#177071,#177072,#177073,#177074,#177075,#177076,#177077,
#177078,#177079,#177080,#177081,#177082,#177083,#177084,#177085,#177086,
#177087,#177088,#177089,#177090,#177091,#177092,#177093,#177094,#177095,
#177096,#177097,#177098,#177099,#177100,#177101,#177102,#177103,#177104,
#177105,#177106,#177107,#177108,#177109,#177110,#177111,#177112,#177113,
#177114,#177115,#177116,#177117,#177118,#177119,#177120,#177121,#177122,
#177123,#177124,#177125,#177126,#177127,#177128,#177129,#177130,#177131,
#177132,#177133,#177134,#177135,#177136,#177137,#177138,#177139,#177140,
#177141,#177142,#177143,#177144,#177145,#177146,#177147,#177148,#177149,
#177150,#177151,#177152,#177153,#177154,#177155,#177156,#177157,#177158,
#177159,#177160,#177161,#177162,#177163,#177164,#177165,#177166,#177167,
#177168,#177169,#177170,#177171,#177172,#177173,#177174,#177175,#177176,
#177177,#177178,#177179,#177180,#177181,#177182,#177183,#177184,#177185,
#177186,#177187,#177188,#177189,#177190,#177191,#177192,#177193,#177194,
#177195,#177196,#177197,#177198,#177199,#177200,#177201,#177202,#177203,
#177204,#177205,#177206,#177207,#177208,#177209,#177210,#177211,#177212,
#177213,#177214,#177215,#177216,#177217,#177218,#177219,#177220,#177221,
#177222,#177223,#177224,#177225,#177226,#177227,#177228,#177229,#177230,
#177231,#177232,#177233,#177234,#177235,#177236,#177237,#177238,#177239,
#177240,#177241,#177242,#177243,#177244,#177245,#177246,#177247,#177248,
#177249,#177250,#177251,#177252,#177253,#177254,#177255,#177256,#177257,
#177258,#177259,#177260,#177261,#177262,#177263,#177264,#177265,#177266,
#177267,#177268,#177269,#177270,#177271,#177272,#177273,#177274,#177275,
#177276,#177277,#177278,#177279,#177280,#177281,#177282,#177283,#177284,
#177285,#177286,#177287,#177288,#177289,#177290,#177291,#177292,#177293,
#177294,#177295,#177296,#177297,#177298,#177299,#177300,#177301,#177302,
#177303,#177304,#177305,#177306,#177307,#177308,#177309,#177310,#177311,
#177312,#177313,#177314,#177315,#177316,#177317,#177318,#177319,#177320,
#177321,#177322,#177323,#177324,#177325,#177326,#177327,#177328,#177329,
#177330,#177331,#177332,#177333,#177334,#177335,#177336,#177337,#177338,
#177339,#177340,#177341,#177342,#177343,#177344,#177345,#177346,#177347,
#177348,#177349,#177350,#177351,#177352,#177353,#177354,#177355,#177356,
#177357,#177358,#177359,#177360,#177361,#177362,#177363,#177364,#177365,
#177366,#177367,#177368,#177369,#177370,#177371,#177372,#177373,#177374,
#177375,#177376,#177377,#177378,#177379,#177380),.UNSPECIFIED.,.F.,.F.,
(4,3,3,3,3,3,3,3,3,3,3,3,3,3,3,3,3,3,3,3,3,3,3,3,3,3,3,3,3,3,3,3,3,3,3,
3,3,3,3,3,3,3,3,3,3,3,3,3,3,3,3,3,3,3,3,3,3,3,3,3,3,3,3,3,3,3,3,3,3,3,3,
3,3,3,3,3,3,3,3,3,3,3,3,3,3,3,3,3,3,3,3,3,3,3,3,3,3,3,3,3,3,3,3,3,3,3,3,
3,4),(-0.999999999770594,-0.994495413,-0.988990826,-0.981651376,-0.976146789,
-0.970642202,-0.965137615,-0.957798165,-0.952293578,-0.946788991,-0.941284404,
-0.935779817,-0.930275229,-0.924770642,-0.919266055,-0.913761468,-0.908256881,
-0.902752294,-0.897247706,-0.891743119,-0.886238532,-0.880733945,-0.875229358,
-0.867889908,-0.862385321,-0.856880734,-0.851376147,-0.844036697,-0.83853211,
-0.833027523,-0.827522936,-0.822018349,-0.816513761,-0.811009174,-0.805504587,
-0.798165138,-0.790825688,-0.783486239,-0.776146789,-0.768807339,-0.76146789,
-0.75412844,-0.746788991,-0.737614679,-0.730275229,-0.72293578,-0.713761468,
-0.706422018,-0.699082569,-0.691743119,-0.68440367,-0.67706422,-0.669724771,
-0.662385321,-0.655045872,-0.647706422,-0.640366972,-0.633027523,-0.625688073,
-0.618348624,-0.611009174,-0.603669725,-0.596330275,-0.588990826,-0.581651376,
-0.574311927,-0.566972477,-0.559633028,-0.552293578,-0.544954128,-0.537614679,
-0.530275229,-0.521100917,-0.511926606,-0.502752294,-0.493577982,-0.48440367,
-0.475229358,-0.466055046,-0.456880734,-0.447706422,-0.43853211,-0.429357798,
-0.420183486,-0.411009174,-0.401834862,-0.39266055,-0.381651376,-0.370642202,
-0.359633028,-0.348623853,-0.337614679,-0.326605505,-0.31559633,-0.304587156,
-0.293577982,-0.282568807,-0.271559633,-0.260550459,-0.249541284,-0.23853211,
-0.227522936,-0.216513761,-0.205504587,-0.194495413,-0.183486239,-0.172477064,
-0.16146789,-0.143172102),.UNSPECIFIED.);
#24346=B_SPLINE_CURVE_WITH_KNOTS('',3,(#177381,#177382,#177383,#177384,
#177385,#177386,#177387,#177388,#177389,#177390,#177391,#177392,#177393,
#177394,#177395,#177396,#177397,#177398,#177399,#177400,#177401,#177402,
#177403,#177404,#177405,#177406,#177407,#177408,#177409,#177410,#177411,
#177412,#177413,#177414,#177415,#177416,#177417,#177418,#177419,#177420,
#177421,#177422,#177423,#177424,#177425,#177426,#177427,#177428,#177429,
#177430,#177431,#177432,#177433,#177434,#177435,#177436,#177437,#177438,
#177439,#177440,#177441,#177442,#177443,#177444,#177445,#177446,#177447,
#177448,#177449,#177450,#177451,#177452,#177453,#177454,#177455,#177456,
#177457,#177458,#177459,#177460,#177461,#177462,#177463,#177464,#177465,
#177466,#177467,#177468,#177469,#177470,#177471,#177472,#177473,#177474,
#177475,#177476,#177477,#177478,#177479,#177480,#177481,#177482,#177483,
#177484,#177485,#177486,#177487,#177488,#177489,#177490,#177491,#177492,
#177493,#177494,#177495,#177496,#177497,#177498,#177499,#177500,#177501,
#177502,#177503,#177504,#177505,#177506,#177507,#177508,#177509,#177510,
#177511,#177512,#177513,#177514,#177515,#177516,#177517,#177518,#177519,
#177520,#177521,#177522,#177523,#177524,#177525,#177526,#177527,#177528,
#177529,#177530,#177531,#177532,#177533,#177534,#177535,#177536,#177537,
#177538,#177539,#177540,#177541,#177542,#177543,#177544,#177545,#177546,
#177547,#177548,#177549,#177550,#177551,#177552,#177553,#177554,#177555,
#177556,#177557,#177558,#177559,#177560,#177561,#177562,#177563,#177564,
#177565,#177566,#177567,#177568,#177569,#177570,#177571,#177572,#177573,
#177574,#177575,#177576,#177577,#177578,#177579,#177580,#177581,#177582,
#177583,#177584,#177585,#177586,#177587,#177588,#177589,#177590,#177591,
#177592,#177593,#177594,#177595,#177596,#177597,#177598,#177599,#177600,
#177601,#177602,#177603,#177604,#177605,#177606,#177607,#177608,#177609,
#177610,#177611,#177612,#177613,#177614,#177615,#177616,#177617,#177618,
#177619,#177620,#177621,#177622,#177623,#177624,#177625,#177626,#177627,
#177628,#177629,#177630,#177631,#177632,#177633,#177634,#177635,#177636,
#177637,#177638,#177639,#177640,#177641,#177642,#177643,#177644,#177645,
#177646,#177647,#177648,#177649,#177650,#177651,#177652,#177653,#177654,
#177655,#177656,#177657,#177658,#177659,#177660,#177661,#177662,#177663,
#177664,#177665,#177666,#177667,#177668,#177669,#177670,#177671,#177672,
#177673,#177674,#177675,#177676,#177677,#177678,#177679,#177680,#177681,
#177682,#177683,#177684,#177685,#177686,#177687,#177688,#177689,#177690,
#177691,#177692,#177693,#177694,#177695,#177696,#177697,#177698,#177699,
#177700,#177701,#177702,#177703,#177704,#177705),.UNSPECIFIED.,.F.,.F.,
(4,3,3,3,3,3,3,3,3,3,3,3,3,3,3,3,3,3,3,3,3,3,3,3,3,3,3,3,3,3,3,3,3,3,3,
3,3,3,3,3,3,3,3,3,3,3,3,3,3,3,3,3,3,3,3,3,3,3,3,3,3,3,3,3,3,3,3,3,3,3,3,
3,3,3,3,3,3,3,3,3,3,3,3,3,3,3,3,3,3,3,3,3,3,3,3,3,3,3,3,3,3,3,3,3,3,3,3,
3,4),(0.143172102,0.15412844,0.165137615,0.176146789,0.187155963,0.198165138,
0.209174312,0.220183486,0.231192661,0.242201835,0.253211009,0.264220183,
0.275229358,0.286238532,0.297247706,0.308256881,0.319266055,0.330275229,
0.341284404,0.352293578,0.363302752,0.374311927,0.385321101,0.396330275,
0.405504587,0.414678899,0.423853211,0.433027523,0.442201835,0.451376147,
0.462385321,0.471559633,0.480733945,0.489908257,0.499082569,0.508256881,
0.517431193,0.526605505,0.533944954,0.543119266,0.550458716,0.557798165,
0.565137615,0.572477064,0.581651376,0.588990826,0.596330275,0.605504587,
0.612844037,0.620183486,0.627522936,0.634862385,0.642201835,0.649541284,
0.656880734,0.664220183,0.671559633,0.678899083,0.686238532,0.693577982,
0.700917431,0.708256881,0.71559633,0.72293578,0.730275229,0.737614679,0.744954128,
0.752293578,0.759633028,0.766972477,0.776146789,0.783486239,0.790825688,
0.798165138,0.805504587,0.811009174,0.818348624,0.823853211,0.829357798,
0.834862385,0.840366972,0.84587156,0.851376147,0.856880734,0.862385321,
0.867889908,0.873394495,0.878899083,0.88440367,0.889908257,0.895412844,
0.900917431,0.906422018,0.911926606,0.917431193,0.92293578,0.930275229,
0.935779817,0.941284404,0.946788991,0.952293578,0.957798165,0.963302752,
0.968807339,0.974311927,0.981651376,0.987155963,0.99266055,0.999999999770594),
 .UNSPECIFIED.);
#24347=B_SPLINE_CURVE_WITH_KNOTS('',5,(#178668,#178669,#178670,#178671,
#178672,#178673,#178674,#178675,#178676,#178677,#178678,#178679,#178680,
#178681,#178682,#178683,#178684,#178685,#178686,#178687,#178688,#178689,
#178690,#178691,#178692,#178693,#178694,#178695,#178696,#178697,#178698,
#178699,#178700,#178701,#178702,#178703,#178704,#178705,#178706,#178707,
#178708,#178709,#178710,#178711,#178712,#178713,#178714,#178715,#178716,
#178717,#178718,#178719,#178720,#178721,#178722,#178723,#178724,#178725,
#178726,#178727,#178728,#178729,#178730,#178731,#178732,#178733,#178734,
#178735,#178736,#178737,#178738,#178739,#178740,#178741,#178742,#178743,
#178744,#178745,#178746,#178747,#178748,#178749,#178750,#178751,#178752,
#178753,#178754,#178755,#178756,#178757,#178758,#178759,#178760,#178761,
#178762,#178763,#178764,#178765,#178766,#178767,#178768,#178769,#178770,
#178771,#178772,#178773,#178774,#178775,#178776,#178777,#178778,#178779,
#178780,#178781,#178782,#178783,#178784,#178785,#178786,#178787,#178788,
#178789,#178790,#178791,#178792,#178793,#178794,#178795,#178796,#178797,
#178798,#178799,#178800,#178801,#178802,#178803,#178804,#178805,#178806,
#178807,#178808,#178809,#178810,#178811,#178812,#178813,#178814,#178815,
#178816,#178817,#178818,#178819,#178820,#178821,#178822,#178823,#178824,
#178825,#178826,#178827,#178828,#178829,#178830,#178831,#178832,#178833,
#178834,#178835,#178836,#178837,#178838,#178839,#178840,#178841,#178842,
#178843,#178844,#178845,#178846,#178847,#178848,#178849,#178850,#178851,
#178852,#178853,#178854,#178855,#178856,#178857,#178858,#178859,#178860,
#178861,#178862,#178863,#178864,#178865,#178866,#178867,#178868,#178869,
#178870,#178871,#178872,#178873,#178874,#178875,#178876,#178877,#178878,
#178879,#178880,#178881,#178882,#178883,#178884,#178885,#178886,#178887,
#178888,#178889,#178890,#178891,#178892,#178893,#178894,#178895,#178896,
#178897,#178898,#178899,#178900,#178901,#178902,#178903,#178904,#178905,
#178906,#178907,#178908,#178909,#178910,#178911,#178912,#178913,#178914,
#178915,#178916,#178917,#178918,#178919,#178920,#178921,#178922,#178923,
#178924,#178925,#178926,#178927,#178928,#178929,#178930,#178931,#178932,
#178933,#178934,#178935,#178936,#178937,#178938,#178939,#178940,#178941,
#178942,#178943,#178944,#178945,#178946,#178947,#178948,#178949,#178950,
#178951,#178952,#178953,#178954,#178955,#178956,#178957,#178958,#178959,
#178960,#178961,#178962,#178963,#178964,#178965,#178966,#178967,#178968,
#178969,#178970,#178971,#178972,#178973,#178974,#178975,#178976,#178977,
#178978,#178979,#178980,#178981,#178982,#178983,#178984,#178985,#178986,
#178987,#178988,#178989,#178990,#178991,#178992,#178993,#178994,#178995,
#178996,#178997,#178998,#178999,#179000,#179001,#179002,#179003,#179004,
#179005,#179006,#179007,#179008,#179009,#179010,#179011,#179012,#179013,
#179014,#179015,#179016,#179017,#179018,#179019,#179020,#179021,#179022,
#179023,#179024,#179025,#179026,#179027,#179028,#179029,#179030,#179031,
#179032,#179033,#179034,#179035,#179036,#179037,#179038,#179039,#179040,
#179041,#179042,#179043,#179044,#179045,#179046,#179047,#179048,#179049,
#179050,#179051,#179052,#179053,#179054,#179055,#179056,#179057,#179058,
#179059,#179060,#179061,#179062,#179063,#179064,#179065,#179066,#179067,
#179068,#179069,#179070,#179071,#179072,#179073,#179074,#179075,#179076,
#179077,#179078,#179079,#179080,#179081,#179082,#179083,#179084,#179085,
#179086,#179087,#179088,#179089,#179090,#179091,#179092,#179093,#179094,
#179095,#179096,#179097,#179098,#179099,#179100,#179101,#179102,#179103,
#179104,#179105,#179106,#179107,#179108,#179109,#179110,#179111,#179112,
#179113,#179114,#179115,#179116,#179117,#179118,#179119,#179120,#179121,
#179122,#179123,#179124,#179125,#179126,#179127,#179128,#179129,#179130,
#179131,#179132,#179133,#179134,#179135,#179136,#179137,#179138,#179139),
 .UNSPECIFIED.,.F.,.F.,(6,1,1,1,1,1,1,1,1,1,1,1,1,1,1,1,1,1,1,1,1,1,1,1,
1,1,1,1,1,1,1,1,1,1,1,1,1,1,1,1,1,1,1,1,1,1,1,1,1,1,1,1,1,1,1,1,1,1,1,1,
1,1,1,1,1,1,1,1,1,1,1,1,1,1,1,1,1,1,1,1,1,1,1,1,1,1,1,1,1,1,1,1,1,1,1,1,
1,1,1,1,1,1,1,1,1,1,1,1,1,1,1,1,1,1,1,1,1,1,1,1,1,1,1,1,1,1,1,1,1,1,1,1,
1,1,1,1,1,1,1,1,1,1,1,1,1,1,1,1,1,1,1,1,1,1,1,1,1,1,1,1,1,1,1,1,1,1,1,1,
1,1,1,1,1,1,1,1,1,1,1,1,1,1,1,1,1,1,1,1,1,1,1,1,1,1,1,1,1,1,1,1,1,1,1,1,
1,1,1,1,1,1,1,1,1,1,1,1,1,1,1,1,1,1,1,1,1,1,1,1,1,1,1,1,1,1,1,1,1,1,1,1,
1,1,1,1,1,1,1,1,1,1,1,1,1,1,1,1,1,1,1,1,1,1,1,1,1,1,1,1,1,1,1,1,1,1,1,1,
1,1,1,1,1,1,1,1,1,1,1,1,1,1,1,1,1,1,1,1,1,1,1,1,1,1,1,1,1,1,1,1,1,1,1,1,
1,1,1,1,1,1,1,1,1,1,1,1,1,1,1,1,1,1,1,1,1,1,1,1,1,1,1,1,1,1,1,1,1,1,1,1,
1,1,1,1,1,1,1,1,1,1,1,1,1,1,1,1,1,1,1,1,1,1,1,1,1,1,1,1,1,1,1,1,1,1,1,1,
1,1,1,1,1,1,1,1,1,1,1,1,1,1,1,1,1,1,1,1,1,1,1,1,1,1,1,1,1,1,1,1,1,1,1,1,
1,1,1,1,1,1,1,1,1,1,1,1,1,1,1,1,1,1,1,1,1,1,1,1,1,1,1,1,1,1,1,1,1,1,1,1,
1,1,1,1,1,1,1,1,1,1,1,6),(-1.,-0.998165138,-0.996330275,-0.994495413,-0.99266055,
-0.990825688,-0.988990826,-0.987155963,-0.985321101,-0.983486239,-0.981651376,
-0.979816514,-0.977981651,-0.976146789,-0.974311927,-0.972477064,-0.970642202,
-0.968807339,-0.966972477,-0.965137615,-0.963302752,-0.96146789,-0.959633028,
-0.957798165,-0.955963303,-0.95412844,-0.952293578,-0.950458716,-0.948623853,
-0.946788991,-0.944954128,-0.943119266,-0.941284404,-0.939449541,-0.937614679,
-0.935779817,-0.933944954,-0.932110092,-0.930275229,-0.928440367,-0.926605505,
-0.924770642,-0.92293578,-0.921100917,-0.919266055,-0.917431193,-0.91559633,
-0.913761468,-0.911926606,-0.910091743,-0.908256881,-0.906422018,-0.904587156,
-0.902752294,-0.900917431,-0.899082569,-0.897247706,-0.895412844,-0.893577982,
-0.891743119,-0.889908257,-0.888073394,-0.886238532,-0.88440367,-0.882568807,
-0.880733945,-0.878899083,-0.87706422,-0.875229358,-0.873394495,-0.871559633,
-0.869724771,-0.867889908,-0.866055046,-0.864220183,-0.862385321,-0.860550459,
-0.858715596,-0.856880734,-0.855045872,-0.853211009,-0.851376147,-0.849541284,
-0.847706422,-0.84587156,-0.844036697,-0.842201835,-0.840366972,-0.83853211,
-0.836697248,-0.834862385,-0.833027523,-0.831192661,-0.829357798,-0.827522936,
-0.825688073,-0.823853211,-0.822018349,-0.820183486,-0.818348624,-0.816513761,
-0.814678899,-0.812844037,-0.811009174,-0.809174312,-0.80733945,-0.805504587,
-0.803669725,-0.801834862,-0.8,-0.798165138,-0.796330275,-0.794495413,-0.79266055,
-0.790825688,-0.788990826,-0.787155963,-0.785321101,-0.783486239,-0.781651376,
-0.779816514,-0.777981651,-0.776146789,-0.774311927,-0.772477064,-0.770642202,
-0.768807339,-0.766972477,-0.765137615,-0.763302752,-0.76146789,-0.759633028,
-0.757798165,-0.755963303,-0.75412844,-0.752293578,-0.750458716,-0.748623853,
-0.746788991,-0.744954128,-0.743119266,-0.741284404,-0.739449541,-0.737614679,
-0.735779817,-0.733944954,-0.732110092,-0.730275229,-0.728440367,-0.726605505,
-0.724770642,-0.72293578,-0.721100917,-0.719266055,-0.717431193,-0.71559633,
-0.713761468,-0.711926606,-0.710091743,-0.708256881,-0.706422018,-0.704587156,
-0.702752294,-0.700917431,-0.699082569,-0.697247706,-0.695412844,-0.693577982,
-0.691743119,-0.689908257,-0.688073394,-0.686238532,-0.68440367,-0.682568807,
-0.680733945,-0.678899083,-0.67706422,-0.675229358,-0.673394495,-0.671559633,
-0.669724771,-0.667889908,-0.666055046,-0.664220183,-0.662385321,-0.660550459,
-0.658715596,-0.656880734,-0.655045872,-0.653211009,-0.651376147,-0.649541284,
-0.647706422,-0.64587156,-0.644036697,-0.642201835,-0.640366972,-0.63853211,
-0.636697248,-0.634862385,-0.633027523,-0.631192661,-0.629357798,-0.627522936,
-0.625688073,-0.623853211,-0.622018349,-0.620183486,-0.618348624,-0.616513761,
-0.614678899,-0.612844037,-0.611009174,-0.609174312,-0.60733945,-0.605504587,
-0.603669725,-0.601834862,-0.6,-0.598165138,-0.596330275,-0.594495413,-0.59266055,
-0.590825688,-0.588990826,-0.587155963,-0.585321101,-0.583486239,-0.581651376,
-0.579816514,-0.577981651,-0.576146789,-0.574311927,-0.572477064,-0.570642202,
-0.568807339,-0.566972477,-0.565137615,-0.563302752,-0.56146789,-0.559633028,
-0.557798165,-0.555963303,-0.55412844,-0.552293578,-0.550458716,-0.548623853,
-0.546788991,-0.544954128,-0.543119266,-0.541284404,-0.539449541,-0.537614679,
-0.535779817,-0.533944954,-0.532110092,-0.530275229,-0.528440367,-0.526605505,
-0.524770642,-0.52293578,-0.521100917,-0.519266055,-0.517431193,-0.51559633,
-0.513761468,-0.511926606,-0.510091743,-0.508256881,-0.506422018,-0.504587156,
-0.502752294,-0.500917431,-0.499082569,-0.497247706,-0.495412844,-0.493577982,
-0.491743119,-0.489908257,-0.488073394,-0.486238532,-0.48440367,-0.482568807,
-0.480733945,-0.478899083,-0.47706422,-0.475229358,-0.473394495,-0.471559633,
-0.469724771,-0.467889908,-0.466055046,-0.464220183,-0.462385321,-0.460550459,
-0.458715596,-0.456880734,-0.455045872,-0.453211009,-0.451376147,-0.449541284,
-0.447706422,-0.44587156,-0.444036697,-0.442201835,-0.440366972,-0.43853211,
-0.436697248,-0.434862385,-0.433027523,-0.431192661,-0.429357798,-0.427522936,
-0.425688073,-0.423853211,-0.422018349,-0.420183486,-0.418348624,-0.416513761,
-0.414678899,-0.412844037,-0.411009174,-0.409174312,-0.40733945,-0.405504587,
-0.403669725,-0.401834862,-0.4,-0.398165138,-0.396330275,-0.394495413,-0.39266055,
-0.390825688,-0.388990826,-0.387155963,-0.385321101,-0.383486239,-0.381651376,
-0.379816514,-0.377981651,-0.376146789,-0.374311927,-0.372477064,-0.370642202,
-0.368807339,-0.366972477,-0.365137615,-0.363302752,-0.36146789,-0.359633028,
-0.357798165,-0.355963303,-0.35412844,-0.352293578,-0.350458716,-0.348623853,
-0.346788991,-0.344954128,-0.343119266,-0.341284404,-0.339449541,-0.337614679,
-0.335779817,-0.333944954,-0.332110092,-0.330275229,-0.328440367,-0.326605505,
-0.324770642,-0.32293578,-0.321100917,-0.319266055,-0.317431193,-0.31559633,
-0.313761468,-0.311926606,-0.310091743,-0.308256881,-0.306422018,-0.304587156,
-0.302752294,-0.300917431,-0.299082569,-0.297247706,-0.295412844,-0.293577982,
-0.291743119,-0.289908257,-0.288073394,-0.286238532,-0.28440367,-0.282568807,
-0.280733945,-0.278899083,-0.27706422,-0.275229358,-0.273394495,-0.271559633,
-0.269724771,-0.267889908,-0.266055046,-0.264220183,-0.262385321,-0.260550459,
-0.258715596,-0.256880734,-0.255045872,-0.253211009,-0.251376147,-0.249541284,
-0.247706422,-0.24587156,-0.244036697,-0.242201835,-0.240366972,-0.23853211,
-0.236697248,-0.234862385,-0.233027523,-0.231192661,-0.229357798,-0.227522936,
-0.225688073,-0.223853211,-0.222018349,-0.220183486,-0.218348624,-0.216513761,
-0.214678899,-0.212844037,-0.211009174,-0.209174312,-0.20733945,-0.205504587,
-0.203669725,-0.201834862,-0.2,-0.198165138,-0.196330275,-0.194495413,-0.19266055,
-0.190825688,-0.188990826,-0.187155963,-0.185321101,-0.183486239,-0.181651376,
-0.179816514,-0.177981651,-0.176146789,-0.174311927,-0.172477064,-0.170642202,
-0.168807339,-0.166972477,-0.165137615,-0.163302752,-0.16146789,-0.159633028,
-0.157798165,-0.155963303,-0.15412844,-0.152293578,-0.150458716,-0.148623853,
-0.146788991,-0.144954128,-0.143172102),.UNSPECIFIED.);
#24348=B_SPLINE_CURVE_WITH_KNOTS('',5,(#179140,#179141,#179142,#179143,
#179144,#179145,#179146,#179147,#179148,#179149,#179150,#179151,#179152,
#179153,#179154,#179155,#179156,#179157,#179158,#179159,#179160,#179161,
#179162,#179163,#179164,#179165,#179166,#179167,#179168,#179169,#179170,
#179171,#179172,#179173,#179174,#179175,#179176,#179177,#179178,#179179,
#179180,#179181,#179182,#179183,#179184,#179185,#179186,#179187,#179188,
#179189,#179190,#179191,#179192,#179193,#179194,#179195,#179196,#179197,
#179198,#179199,#179200,#179201,#179202,#179203,#179204,#179205,#179206,
#179207,#179208,#179209,#179210,#179211,#179212,#179213,#179214,#179215,
#179216,#179217,#179218,#179219,#179220,#179221,#179222,#179223,#179224,
#179225,#179226,#179227,#179228,#179229,#179230,#179231,#179232,#179233,
#179234,#179235,#179236,#179237,#179238,#179239,#179240,#179241,#179242,
#179243,#179244,#179245,#179246,#179247,#179248,#179249,#179250,#179251,
#179252,#179253,#179254,#179255,#179256,#179257,#179258,#179259,#179260,
#179261,#179262,#179263,#179264,#179265,#179266,#179267,#179268,#179269,
#179270,#179271,#179272,#179273,#179274,#179275,#179276,#179277,#179278,
#179279,#179280,#179281,#179282,#179283,#179284,#179285,#179286,#179287,
#179288,#179289,#179290,#179291,#179292,#179293,#179294,#179295,#179296,
#179297,#179298,#179299,#179300,#179301,#179302,#179303,#179304,#179305,
#179306,#179307,#179308,#179309,#179310,#179311,#179312,#179313,#179314,
#179315,#179316,#179317,#179318,#179319,#179320,#179321,#179322,#179323,
#179324,#179325,#179326,#179327,#179328,#179329,#179330,#179331,#179332,
#179333,#179334,#179335,#179336,#179337,#179338,#179339,#179340,#179341,
#179342,#179343,#179344,#179345,#179346,#179347,#179348,#179349,#179350,
#179351,#179352,#179353,#179354,#179355,#179356,#179357,#179358,#179359,
#179360,#179361,#179362,#179363,#179364,#179365,#179366,#179367,#179368,
#179369,#179370,#179371,#179372,#179373,#179374,#179375,#179376,#179377,
#179378,#179379,#179380,#179381,#179382,#179383,#179384,#179385,#179386,
#179387,#179388,#179389,#179390,#179391,#179392,#179393,#179394,#179395,
#179396,#179397,#179398,#179399,#179400,#179401,#179402,#179403,#179404,
#179405,#179406,#179407,#179408,#179409,#179410,#179411,#179412,#179413,
#179414,#179415,#179416,#179417,#179418,#179419,#179420,#179421,#179422,
#179423,#179424,#179425,#179426,#179427,#179428,#179429,#179430,#179431,
#179432,#179433,#179434,#179435,#179436,#179437,#179438,#179439,#179440,
#179441,#179442,#179443,#179444,#179445,#179446,#179447,#179448,#179449,
#179450,#179451,#179452,#179453,#179454,#179455,#179456,#179457,#179458,
#179459,#179460,#179461,#179462,#179463,#179464,#179465,#179466,#179467,
#179468,#179469,#179470,#179471,#179472,#179473,#179474,#179475,#179476,
#179477,#179478,#179479,#179480,#179481,#179482,#179483,#179484,#179485,
#179486,#179487,#179488,#179489,#179490,#179491,#179492,#179493,#179494,
#179495,#179496,#179497,#179498,#179499,#179500,#179501,#179502,#179503,
#179504,#179505,#179506,#179507,#179508,#179509,#179510,#179511,#179512,
#179513,#179514,#179515,#179516,#179517,#179518,#179519,#179520,#179521,
#179522,#179523,#179524,#179525,#179526,#179527,#179528,#179529,#179530,
#179531,#179532,#179533,#179534,#179535,#179536,#179537,#179538,#179539,
#179540,#179541,#179542,#179543,#179544,#179545,#179546,#179547,#179548,
#179549,#179550,#179551,#179552,#179553,#179554,#179555,#179556,#179557,
#179558,#179559,#179560,#179561,#179562,#179563,#179564,#179565,#179566,
#179567,#179568,#179569,#179570,#179571,#179572,#179573,#179574,#179575,
#179576,#179577,#179578,#179579,#179580,#179581,#179582,#179583,#179584,
#179585,#179586,#179587,#179588,#179589,#179590,#179591,#179592,#179593,
#179594,#179595,#179596,#179597,#179598,#179599,#179600,#179601,#179602,
#179603,#179604,#179605,#179606,#179607,#179608,#179609,#179610,#179611),
 .UNSPECIFIED.,.F.,.F.,(6,1,1,1,1,1,1,1,1,1,1,1,1,1,1,1,1,1,1,1,1,1,1,1,
1,1,1,1,1,1,1,1,1,1,1,1,1,1,1,1,1,1,1,1,1,1,1,1,1,1,1,1,1,1,1,1,1,1,1,1,
1,1,1,1,1,1,1,1,1,1,1,1,1,1,1,1,1,1,1,1,1,1,1,1,1,1,1,1,1,1,1,1,1,1,1,1,
1,1,1,1,1,1,1,1,1,1,1,1,1,1,1,1,1,1,1,1,1,1,1,1,1,1,1,1,1,1,1,1,1,1,1,1,
1,1,1,1,1,1,1,1,1,1,1,1,1,1,1,1,1,1,1,1,1,1,1,1,1,1,1,1,1,1,1,1,1,1,1,1,
1,1,1,1,1,1,1,1,1,1,1,1,1,1,1,1,1,1,1,1,1,1,1,1,1,1,1,1,1,1,1,1,1,1,1,1,
1,1,1,1,1,1,1,1,1,1,1,1,1,1,1,1,1,1,1,1,1,1,1,1,1,1,1,1,1,1,1,1,1,1,1,1,
1,1,1,1,1,1,1,1,1,1,1,1,1,1,1,1,1,1,1,1,1,1,1,1,1,1,1,1,1,1,1,1,1,1,1,1,
1,1,1,1,1,1,1,1,1,1,1,1,1,1,1,1,1,1,1,1,1,1,1,1,1,1,1,1,1,1,1,1,1,1,1,1,
1,1,1,1,1,1,1,1,1,1,1,1,1,1,1,1,1,1,1,1,1,1,1,1,1,1,1,1,1,1,1,1,1,1,1,1,
1,1,1,1,1,1,1,1,1,1,1,1,1,1,1,1,1,1,1,1,1,1,1,1,1,1,1,1,1,1,1,1,1,1,1,1,
1,1,1,1,1,1,1,1,1,1,1,1,1,1,1,1,1,1,1,1,1,1,1,1,1,1,1,1,1,1,1,1,1,1,1,1,
1,1,1,1,1,1,1,1,1,1,1,1,1,1,1,1,1,1,1,1,1,1,1,1,1,1,1,1,1,1,1,1,1,1,1,1,
1,1,1,1,1,1,1,1,1,1,1,6),(0.143172102,0.144954128,0.146788991,0.148623853,
0.150458716,0.152293578,0.15412844,0.155963303,0.157798165,0.159633028,
0.16146789,0.163302752,0.165137615,0.166972477,0.168807339,0.170642202,
0.172477064,0.174311927,0.176146789,0.177981651,0.179816514,0.181651376,
0.183486239,0.185321101,0.187155963,0.188990826,0.190825688,0.19266055,
0.194495413,0.196330275,0.198165138,0.2,0.201834862,0.203669725,0.205504587,
0.20733945,0.209174312,0.211009174,0.212844037,0.214678899,0.216513761,
0.218348624,0.220183486,0.222018349,0.223853211,0.225688073,0.227522936,
0.229357798,0.231192661,0.233027523,0.234862385,0.236697248,0.23853211,
0.240366972,0.242201835,0.244036697,0.24587156,0.247706422,0.249541284,
0.251376147,0.253211009,0.255045872,0.256880734,0.258715596,0.260550459,
0.262385321,0.264220183,0.266055046,0.267889908,0.269724771,0.271559633,
0.273394495,0.275229358,0.27706422,0.278899083,0.280733945,0.282568807,
0.28440367,0.286238532,0.288073394,0.289908257,0.291743119,0.293577982,
0.295412844,0.297247706,0.299082569,0.300917431,0.302752294,0.304587156,
0.306422018,0.308256881,0.310091743,0.311926606,0.313761468,0.31559633,
0.317431193,0.319266055,0.321100917,0.32293578,0.324770642,0.326605505,
0.328440367,0.330275229,0.332110092,0.333944954,0.335779817,0.337614679,
0.339449541,0.341284404,0.343119266,0.344954128,0.346788991,0.348623853,
0.350458716,0.352293578,0.35412844,0.355963303,0.357798165,0.359633028,
0.36146789,0.363302752,0.365137615,0.366972477,0.368807339,0.370642202,
0.372477064,0.374311927,0.376146789,0.377981651,0.379816514,0.381651376,
0.383486239,0.385321101,0.387155963,0.388990826,0.390825688,0.39266055,
0.394495413,0.396330275,0.398165138,0.4,0.401834862,0.403669725,0.405504587,
0.40733945,0.409174312,0.411009174,0.412844037,0.414678899,0.416513761,
0.418348624,0.420183486,0.422018349,0.423853211,0.425688073,0.427522936,
0.429357798,0.431192661,0.433027523,0.434862385,0.436697248,0.43853211,
0.440366972,0.442201835,0.444036697,0.44587156,0.447706422,0.449541284,
0.451376147,0.453211009,0.455045872,0.456880734,0.458715596,0.460550459,
0.462385321,0.464220183,0.466055046,0.467889908,0.469724771,0.471559633,
0.473394495,0.475229358,0.47706422,0.478899083,0.480733945,0.482568807,
0.48440367,0.486238532,0.488073394,0.489908257,0.491743119,0.493577982,
0.495412844,0.497247706,0.499082569,0.500917431,0.502752294,0.504587156,
0.506422018,0.508256881,0.510091743,0.511926606,0.513761468,0.51559633,
0.517431193,0.519266055,0.521100917,0.52293578,0.524770642,0.526605505,
0.528440367,0.530275229,0.532110092,0.533944954,0.535779817,0.537614679,
0.539449541,0.541284404,0.543119266,0.544954128,0.546788991,0.548623853,
0.550458716,0.552293578,0.55412844,0.555963303,0.557798165,0.559633028,
0.56146789,0.563302752,0.565137615,0.566972477,0.568807339,0.570642202,
0.572477064,0.574311927,0.576146789,0.577981651,0.579816514,0.581651376,
0.583486239,0.585321101,0.587155963,0.588990826,0.590825688,0.59266055,
0.594495413,0.596330275,0.598165138,0.6,0.601834862,0.603669725,0.605504587,
0.60733945,0.609174312,0.611009174,0.612844037,0.614678899,0.616513761,
0.618348624,0.620183486,0.622018349,0.623853211,0.625688073,0.627522936,
0.629357798,0.631192661,0.633027523,0.634862385,0.636697248,0.63853211,
0.640366972,0.642201835,0.644036697,0.64587156,0.647706422,0.649541284,
0.651376147,0.653211009,0.655045872,0.656880734,0.658715596,0.660550459,
0.662385321,0.664220183,0.666055046,0.667889908,0.669724771,0.671559633,
0.673394495,0.675229358,0.67706422,0.678899083,0.680733945,0.682568807,
0.68440367,0.686238532,0.688073394,0.689908257,0.691743119,0.693577982,
0.695412844,0.697247706,0.699082569,0.700917431,0.702752294,0.704587156,
0.706422018,0.708256881,0.710091743,0.711926606,0.713761468,0.71559633,
0.717431193,0.719266055,0.721100917,0.72293578,0.724770642,0.726605505,
0.728440367,0.730275229,0.732110092,0.733944954,0.735779817,0.737614679,
0.739449541,0.741284404,0.743119266,0.744954128,0.746788991,0.748623853,
0.750458716,0.752293578,0.75412844,0.755963303,0.757798165,0.759633028,
0.76146789,0.763302752,0.765137615,0.766972477,0.768807339,0.770642202,
0.772477064,0.774311927,0.776146789,0.777981651,0.779816514,0.781651376,
0.783486239,0.785321101,0.787155963,0.788990826,0.790825688,0.79266055,
0.794495413,0.796330275,0.798165138,0.8,0.801834862,0.803669725,0.805504587,
0.80733945,0.809174312,0.811009174,0.812844037,0.814678899,0.816513761,
0.818348624,0.820183486,0.822018349,0.823853211,0.825688073,0.827522936,
0.829357798,0.831192661,0.833027523,0.834862385,0.836697248,0.83853211,
0.840366972,0.842201835,0.844036697,0.84587156,0.847706422,0.849541284,
0.851376147,0.853211009,0.855045872,0.856880734,0.858715596,0.860550459,
0.862385321,0.864220183,0.866055046,0.867889908,0.869724771,0.871559633,
0.873394495,0.875229358,0.87706422,0.878899083,0.880733945,0.882568807,
0.88440367,0.886238532,0.888073394,0.889908257,0.891743119,0.893577982,
0.895412844,0.897247706,0.899082569,0.900917431,0.902752294,0.904587156,
0.906422018,0.908256881,0.910091743,0.911926606,0.913761468,0.91559633,
0.917431193,0.919266055,0.921100917,0.92293578,0.924770642,0.926605505,
0.928440367,0.930275229,0.932110092,0.933944954,0.935779817,0.937614679,
0.939449541,0.941284404,0.943119266,0.944954128,0.946788991,0.948623853,
0.950458716,0.952293578,0.95412844,0.955963303,0.957798165,0.959633028,
0.96146789,0.963302752,0.965137615,0.966972477,0.968807339,0.970642202,
0.972477064,0.974311927,0.976146789,0.977981651,0.979816514,0.981651376,
0.983486239,0.985321101,0.987155963,0.988990826,0.990825688,0.99266055,
0.994495413,0.996330275,0.998165138,1.),.UNSPECIFIED.);
#24349=B_SPLINE_CURVE_WITH_KNOTS('',3,(#180556,#180557,#180558,#180559,
#180560,#180561,#180562,#180563,#180564,#180565,#180566,#180567,#180568,
#180569,#180570,#180571,#180572,#180573,#180574,#180575,#180576,#180577,
#180578,#180579,#180580,#180581,#180582,#180583,#180584,#180585,#180586,
#180587,#180588,#180589,#180590,#180591,#180592,#180593,#180594,#180595,
#180596,#180597,#180598,#180599,#180600,#180601,#180602,#180603,#180604,
#180605,#180606,#180607,#180608,#180609,#180610,#180611,#180612,#180613,
#180614,#180615,#180616,#180617,#180618,#180619,#180620,#180621,#180622,
#180623,#180624,#180625,#180626,#180627,#180628,#180629,#180630,#180631,
#180632,#180633,#180634,#180635,#180636,#180637,#180638,#180639,#180640,
#180641,#180642,#180643,#180644,#180645,#180646,#180647,#180648,#180649,
#180650,#180651,#180652,#180653,#180654,#180655,#180656,#180657,#180658,
#180659,#180660,#180661,#180662,#180663,#180664,#180665,#180666,#180667,
#180668,#180669,#180670,#180671,#180672,#180673,#180674,#180675,#180676,
#180677,#180678,#180679,#180680,#180681,#180682,#180683,#180684,#180685,
#180686,#180687,#180688,#180689,#180690,#180691,#180692,#180693,#180694,
#180695,#180696,#180697,#180698,#180699,#180700,#180701,#180702,#180703,
#180704,#180705,#180706,#180707,#180708,#180709,#180710,#180711,#180712,
#180713,#180714,#180715,#180716,#180717,#180718,#180719,#180720,#180721,
#180722,#180723,#180724,#180725,#180726,#180727,#180728,#180729,#180730,
#180731,#180732,#180733,#180734,#180735,#180736,#180737,#180738,#180739,
#180740,#180741,#180742,#180743,#180744,#180745,#180746,#180747,#180748,
#180749,#180750,#180751,#180752,#180753,#180754,#180755,#180756,#180757,
#180758,#180759,#180760,#180761,#180762,#180763,#180764,#180765,#180766,
#180767,#180768,#180769,#180770,#180771,#180772,#180773,#180774,#180775,
#180776,#180777,#180778,#180779,#180780,#180781,#180782,#180783,#180784,
#180785,#180786,#180787,#180788,#180789,#180790,#180791,#180792,#180793,
#180794,#180795,#180796,#180797,#180798,#180799,#180800,#180801,#180802,
#180803,#180804,#180805,#180806,#180807,#180808,#180809,#180810,#180811,
#180812,#180813,#180814,#180815,#180816,#180817,#180818,#180819,#180820,
#180821,#180822,#180823,#180824,#180825,#180826,#180827,#180828,#180829,
#180830,#180831,#180832,#180833,#180834,#180835,#180836,#180837,#180838,
#180839,#180840,#180841,#180842,#180843,#180844,#180845,#180846,#180847,
#180848,#180849,#180850,#180851,#180852,#180853,#180854,#180855,#180856,
#180857,#180858,#180859,#180860,#180861,#180862,#180863,#180864,#180865,
#180866,#180867,#180868,#180869,#180870,#180871,#180872,#180873,#180874),
 .UNSPECIFIED.,.F.,.F.,(4,3,3,3,3,3,3,3,3,3,3,3,3,3,3,3,3,3,3,3,3,3,3,3,
3,3,3,3,3,3,3,3,3,3,3,3,3,3,3,3,3,3,3,3,3,3,3,3,3,3,3,3,3,3,3,3,3,3,3,3,
3,3,3,3,3,3,3,3,3,3,3,3,3,3,3,3,3,3,3,3,3,3,3,3,3,3,3,3,3,3,3,3,3,3,3,3,
3,3,3,3,3,3,3,3,3,3,4),(0.143172102,0.15412844,0.165137615,0.176146789,
0.187155963,0.198165138,0.209174312,0.220183486,0.231192661,0.242201835,
0.253211009,0.264220183,0.275229358,0.286238532,0.297247706,0.308256881,
0.319266055,0.330275229,0.341284404,0.352293578,0.365137615,0.376146789,
0.387155963,0.398165138,0.40733945,0.416513761,0.425688073,0.434862385,
0.444036697,0.455045872,0.464220183,0.473394495,0.48440367,0.493577982,
0.502752294,0.511926606,0.521100917,0.530275229,0.537614679,0.544954128,
0.552293578,0.559633028,0.566972477,0.574311927,0.583486239,0.590825688,
0.598165138,0.60733945,0.614678899,0.622018349,0.631192661,0.63853211,0.64587156,
0.655045872,0.662385321,0.671559633,0.678899083,0.686238532,0.693577982,
0.704587156,0.711926606,0.719266055,0.726605505,0.733944954,0.741284404,
0.748623853,0.755963303,0.763302752,0.770642202,0.777981651,0.785321101,
0.79266055,0.8,0.80733945,0.812844037,0.818348624,0.823853211,0.831192661,
0.836697248,0.842201835,0.847706422,0.853211009,0.858715596,0.864220183,
0.869724771,0.875229358,0.880733945,0.886238532,0.891743119,0.897247706,
0.902752294,0.908256881,0.913761468,0.919266055,0.928440367,0.935779817,
0.941284404,0.946788991,0.952293578,0.957798165,0.963302752,0.970642202,
0.976146789,0.983486239,0.988990826,0.994495413,1.),.UNSPECIFIED.);
#24350=B_SPLINE_CURVE_WITH_KNOTS('',3,(#180875,#180876,#180877,#180878,
#180879,#180880,#180881,#180882,#180883,#180884,#180885,#180886,#180887,
#180888,#180889,#180890,#180891,#180892,#180893,#180894,#180895,#180896,
#180897,#180898,#180899,#180900,#180901,#180902,#180903,#180904,#180905,
#180906,#180907,#180908,#180909,#180910,#180911,#180912,#180913,#180914,
#180915,#180916,#180917,#180918,#180919,#180920,#180921,#180922,#180923,
#180924,#180925,#180926,#180927,#180928,#180929,#180930,#180931,#180932,
#180933,#180934,#180935,#180936,#180937,#180938,#180939,#180940,#180941,
#180942,#180943,#180944,#180945,#180946,#180947,#180948,#180949,#180950,
#180951,#180952,#180953,#180954,#180955,#180956,#180957,#180958,#180959,
#180960,#180961,#180962,#180963,#180964,#180965,#180966,#180967,#180968,
#180969,#180970,#180971,#180972,#180973,#180974,#180975,#180976,#180977,
#180978,#180979,#180980,#180981,#180982,#180983,#180984,#180985,#180986,
#180987,#180988,#180989,#180990,#180991,#180992,#180993,#180994,#180995,
#180996,#180997,#180998,#180999,#181000,#181001,#181002,#181003,#181004,
#181005,#181006,#181007,#181008,#181009,#181010,#181011,#181012,#181013,
#181014,#181015,#181016,#181017,#181018,#181019,#181020,#181021,#181022,
#181023,#181024,#181025,#181026,#181027,#181028,#181029,#181030,#181031,
#181032,#181033,#181034,#181035,#181036,#181037,#181038,#181039,#181040,
#181041,#181042,#181043,#181044,#181045,#181046,#181047,#181048,#181049,
#181050,#181051,#181052,#181053,#181054,#181055,#181056,#181057,#181058,
#181059,#181060,#181061,#181062,#181063,#181064,#181065,#181066,#181067,
#181068,#181069,#181070,#181071,#181072,#181073,#181074,#181075,#181076,
#181077,#181078,#181079,#181080,#181081,#181082,#181083,#181084,#181085,
#181086,#181087,#181088,#181089,#181090,#181091,#181092,#181093,#181094,
#181095,#181096,#181097,#181098,#181099,#181100,#181101,#181102,#181103,
#181104,#181105,#181106,#181107,#181108,#181109,#181110,#181111,#181112,
#181113,#181114,#181115,#181116,#181117,#181118,#181119,#181120,#181121,
#181122,#181123,#181124,#181125,#181126,#181127,#181128,#181129,#181130,
#181131,#181132,#181133,#181134,#181135,#181136,#181137,#181138,#181139,
#181140,#181141,#181142,#181143,#181144,#181145,#181146,#181147,#181148,
#181149,#181150,#181151,#181152,#181153,#181154,#181155,#181156,#181157,
#181158,#181159,#181160,#181161,#181162,#181163,#181164,#181165,#181166,
#181167,#181168,#181169,#181170,#181171,#181172,#181173,#181174,#181175,
#181176,#181177,#181178,#181179,#181180,#181181,#181182,#181183,#181184,
#181185,#181186,#181187,#181188,#181189,#181190,#181191,#181192,#181193,
#181194,#181195,#181196),.UNSPECIFIED.,.F.,.F.,(4,3,3,3,3,3,3,3,3,3,3,3,
3,3,3,3,3,3,3,3,3,3,3,3,3,3,3,3,3,3,3,3,3,3,3,3,3,3,3,3,3,3,3,3,3,3,3,3,
3,3,3,3,3,3,3,3,3,3,3,3,3,3,3,3,3,3,3,3,3,3,3,3,3,3,3,3,3,3,3,3,3,3,3,3,
3,3,3,3,3,3,3,3,3,3,3,3,3,3,3,3,3,3,3,3,3,3,3,4),(0.143172102,0.15412844,
0.165137615,0.176146789,0.187155963,0.198165138,0.209174312,0.220183486,
0.231192661,0.242201835,0.253211009,0.264220183,0.275229358,0.286238532,
0.297247706,0.308256881,0.319266055,0.330275229,0.341284404,0.352293578,
0.363302752,0.374311927,0.385321101,0.396330275,0.405504587,0.414678899,
0.423853211,0.433027523,0.442201835,0.451376147,0.460550459,0.469724771,
0.478899083,0.488073394,0.497247706,0.506422018,0.51559633,0.524770642,
0.533944954,0.541284404,0.548623853,0.555963303,0.563302752,0.570642202,
0.579816514,0.588990826,0.596330275,0.603669725,0.611009174,0.618348624,
0.625688073,0.633027523,0.640366972,0.647706422,0.655045872,0.664220183,
0.671559633,0.678899083,0.686238532,0.693577982,0.700917431,0.708256881,
0.71559633,0.72293578,0.730275229,0.737614679,0.744954128,0.752293578,0.759633028,
0.766972477,0.776146789,0.783486239,0.790825688,0.798165138,0.805504587,
0.811009174,0.816513761,0.822018349,0.827522936,0.833027523,0.840366972,
0.84587156,0.853211009,0.858715596,0.864220183,0.869724771,0.875229358,
0.880733945,0.888073394,0.893577982,0.899082569,0.904587156,0.910091743,
0.91559633,0.921100917,0.928440367,0.933944954,0.939449541,0.946788991,
0.952293578,0.957798165,0.963302752,0.968807339,0.974311927,0.979816514,
0.985321101,0.990825688,1.),.UNSPECIFIED.);
#24351=B_SPLINE_CURVE_WITH_KNOTS('',3,(#182156,#182157,#182158,#182159,
#182160,#182161,#182162,#182163,#182164,#182165,#182166,#182167,#182168,
#182169,#182170,#182171,#182172,#182173,#182174,#182175,#182176,#182177,
#182178,#182179,#182180,#182181,#182182,#182183,#182184,#182185,#182186,
#182187,#182188,#182189,#182190,#182191,#182192,#182193,#182194,#182195,
#182196,#182197,#182198,#182199,#182200,#182201,#182202,#182203,#182204,
#182205,#182206,#182207,#182208,#182209,#182210,#182211,#182212,#182213,
#182214,#182215,#182216,#182217,#182218,#182219,#182220,#182221,#182222,
#182223,#182224,#182225,#182226,#182227,#182228,#182229,#182230,#182231,
#182232,#182233,#182234,#182235,#182236,#182237,#182238,#182239,#182240,
#182241,#182242,#182243,#182244,#182245,#182246,#182247,#182248,#182249,
#182250,#182251,#182252,#182253,#182254,#182255,#182256,#182257,#182258,
#182259,#182260,#182261,#182262,#182263,#182264,#182265,#182266,#182267,
#182268,#182269,#182270,#182271,#182272,#182273,#182274,#182275,#182276,
#182277,#182278,#182279,#182280,#182281,#182282,#182283,#182284,#182285,
#182286,#182287,#182288,#182289,#182290,#182291,#182292,#182293,#182294,
#182295,#182296,#182297,#182298,#182299,#182300,#182301,#182302,#182303,
#182304,#182305,#182306,#182307,#182308,#182309,#182310,#182311,#182312,
#182313,#182314,#182315,#182316,#182317,#182318,#182319,#182320,#182321,
#182322,#182323,#182324,#182325,#182326,#182327,#182328,#182329,#182330,
#182331,#182332,#182333,#182334,#182335,#182336,#182337,#182338,#182339,
#182340,#182341,#182342,#182343,#182344,#182345,#182346,#182347,#182348,
#182349,#182350,#182351,#182352,#182353,#182354,#182355,#182356,#182357,
#182358,#182359,#182360,#182361,#182362,#182363,#182364,#182365,#182366,
#182367,#182368,#182369,#182370,#182371,#182372,#182373,#182374,#182375,
#182376,#182377,#182378,#182379,#182380,#182381,#182382,#182383,#182384,
#182385,#182386,#182387,#182388,#182389,#182390,#182391,#182392,#182393,
#182394,#182395,#182396,#182397,#182398,#182399,#182400,#182401,#182402,
#182403,#182404,#182405,#182406,#182407,#182408,#182409,#182410,#182411,
#182412,#182413,#182414,#182415,#182416,#182417,#182418,#182419,#182420,
#182421,#182422,#182423,#182424,#182425,#182426,#182427,#182428,#182429,
#182430,#182431,#182432,#182433,#182434,#182435,#182436,#182437,#182438,
#182439,#182440,#182441,#182442,#182443,#182444,#182445,#182446,#182447,
#182448,#182449,#182450,#182451,#182452,#182453,#182454,#182455,#182456,
#182457,#182458,#182459,#182460,#182461,#182462,#182463,#182464,#182465,
#182466,#182467,#182468,#182469,#182470,#182471),.UNSPECIFIED.,.F.,.F.,
(4,3,3,3,3,3,3,3,3,3,3,3,3,3,3,3,3,3,3,3,3,3,3,3,3,3,3,3,3,3,3,3,3,3,3,
3,3,3,3,3,3,3,3,3,3,3,3,3,3,3,3,3,3,3,3,3,3,3,3,3,3,3,3,3,3,3,3,3,3,3,3,
3,3,3,3,3,3,3,3,3,3,3,3,3,3,3,3,3,3,3,3,3,3,3,3,3,3,3,3,3,3,3,3,3,3,4),
(0.143172102,0.15412844,0.165137615,0.176146789,0.187155963,0.198165138,
0.209174312,0.220183486,0.231192661,0.242201835,0.253211009,0.264220183,
0.275229358,0.286238532,0.297247706,0.308256881,0.319266055,0.330275229,
0.341284404,0.352293578,0.363302752,0.374311927,0.385321101,0.398165138,
0.40733945,0.416513761,0.425688073,0.434862385,0.444036697,0.453211009,
0.462385321,0.471559633,0.480733945,0.489908257,0.499082569,0.508256881,
0.517431193,0.526605505,0.533944954,0.541284404,0.550458716,0.559633028,
0.566972477,0.574311927,0.583486239,0.590825688,0.598165138,0.605504587,
0.612844037,0.620183486,0.627522936,0.634862385,0.64587156,0.653211009,
0.660550459,0.671559633,0.678899083,0.686238532,0.693577982,0.704587156,
0.711926606,0.719266055,0.726605505,0.735779817,0.743119266,0.750458716,
0.759633028,0.766972477,0.774311927,0.783486239,0.790825688,0.798165138,
0.80733945,0.812844037,0.818348624,0.823853211,0.829357798,0.834862385,
0.840366972,0.84587156,0.851376147,0.856880734,0.862385321,0.867889908,
0.873394495,0.878899083,0.88440367,0.889908257,0.895412844,0.900917431,
0.906422018,0.911926606,0.917431193,0.92293578,0.928440367,0.935779817,
0.941284404,0.946788991,0.952293578,0.96146789,0.966972477,0.974311927,
0.979816514,0.985321101,0.990825688,1.),.UNSPECIFIED.);
#24352=B_SPLINE_CURVE_WITH_KNOTS('',3,(#182472,#182473,#182474,#182475,
#182476,#182477,#182478,#182479,#182480,#182481,#182482,#182483,#182484,
#182485,#182486,#182487,#182488,#182489,#182490,#182491,#182492,#182493,
#182494,#182495,#182496,#182497,#182498,#182499,#182500,#182501,#182502,
#182503,#182504,#182505,#182506,#182507,#182508,#182509,#182510,#182511,
#182512,#182513,#182514,#182515,#182516,#182517,#182518,#182519,#182520,
#182521,#182522,#182523,#182524,#182525,#182526,#182527,#182528,#182529,
#182530,#182531,#182532,#182533,#182534,#182535,#182536,#182537,#182538,
#182539,#182540,#182541,#182542,#182543,#182544,#182545,#182546,#182547,
#182548,#182549,#182550,#182551,#182552,#182553,#182554,#182555,#182556,
#182557,#182558,#182559,#182560,#182561,#182562,#182563,#182564,#182565,
#182566,#182567,#182568,#182569,#182570,#182571,#182572,#182573,#182574,
#182575,#182576,#182577,#182578,#182579,#182580,#182581,#182582,#182583,
#182584,#182585,#182586,#182587,#182588,#182589,#182590,#182591,#182592,
#182593,#182594,#182595,#182596,#182597,#182598,#182599,#182600,#182601,
#182602,#182603,#182604,#182605,#182606,#182607,#182608,#182609,#182610,
#182611,#182612,#182613,#182614,#182615,#182616,#182617,#182618,#182619,
#182620,#182621,#182622,#182623,#182624,#182625,#182626,#182627,#182628,
#182629,#182630,#182631,#182632,#182633,#182634,#182635,#182636,#182637,
#182638,#182639,#182640,#182641,#182642,#182643,#182644,#182645,#182646,
#182647,#182648,#182649,#182650,#182651,#182652,#182653,#182654,#182655,
#182656,#182657,#182658,#182659,#182660,#182661,#182662,#182663,#182664,
#182665,#182666,#182667,#182668,#182669,#182670,#182671,#182672,#182673,
#182674,#182675,#182676,#182677,#182678,#182679,#182680,#182681,#182682,
#182683,#182684,#182685,#182686,#182687,#182688,#182689,#182690,#182691,
#182692,#182693,#182694,#182695,#182696,#182697,#182698,#182699,#182700,
#182701,#182702,#182703,#182704,#182705,#182706,#182707,#182708,#182709,
#182710,#182711,#182712,#182713,#182714,#182715,#182716,#182717,#182718,
#182719,#182720,#182721,#182722,#182723,#182724,#182725,#182726,#182727,
#182728,#182729,#182730,#182731,#182732,#182733,#182734,#182735,#182736,
#182737,#182738,#182739,#182740,#182741,#182742,#182743,#182744,#182745,
#182746,#182747,#182748,#182749,#182750,#182751,#182752,#182753,#182754,
#182755,#182756,#182757,#182758,#182759,#182760,#182761,#182762,#182763,
#182764,#182765,#182766,#182767,#182768,#182769,#182770,#182771,#182772,
#182773,#182774,#182775,#182776,#182777,#182778,#182779,#182780,#182781,
#182782,#182783,#182784,#182785,#182786,#182787),.UNSPECIFIED.,.F.,.F.,
(4,3,3,3,3,3,3,3,3,3,3,3,3,3,3,3,3,3,3,3,3,3,3,3,3,3,3,3,3,3,3,3,3,3,3,
3,3,3,3,3,3,3,3,3,3,3,3,3,3,3,3,3,3,3,3,3,3,3,3,3,3,3,3,3,3,3,3,3,3,3,3,
3,3,3,3,3,3,3,3,3,3,3,3,3,3,3,3,3,3,3,3,3,3,3,3,3,3,3,3,3,3,3,3,3,3,4),
(0.143172102,0.15412844,0.165137615,0.176146789,0.187155963,0.198165138,
0.209174312,0.220183486,0.231192661,0.242201835,0.253211009,0.264220183,
0.275229358,0.286238532,0.297247706,0.308256881,0.319266055,0.330275229,
0.341284404,0.352293578,0.363302752,0.374311927,0.385321101,0.396330275,
0.405504587,0.414678899,0.423853211,0.433027523,0.442201835,0.451376147,
0.460550459,0.469724771,0.478899083,0.488073394,0.497247706,0.506422018,
0.51559633,0.524770642,0.533944954,0.543119266,0.550458716,0.557798165,
0.565137615,0.572477064,0.579816514,0.587155963,0.594495413,0.601834862,
0.609174312,0.616513761,0.623853211,0.631192661,0.63853211,0.64587156,0.653211009,
0.662385321,0.669724771,0.67706422,0.68440367,0.691743119,0.700917431,0.710091743,
0.717431193,0.724770642,0.732110092,0.743119266,0.750458716,0.757798165,
0.766972477,0.774311927,0.781651376,0.788990826,0.796330275,0.805504587,
0.811009174,0.818348624,0.823853211,0.829357798,0.834862385,0.842201835,
0.847706422,0.853211009,0.858715596,0.864220183,0.869724771,0.875229358,
0.880733945,0.888073394,0.893577982,0.899082569,0.904587156,0.910091743,
0.91559633,0.921100917,0.930275229,0.935779817,0.941284404,0.946788991,
0.952293578,0.959633028,0.968807339,0.974311927,0.979816514,0.985321101,
0.990825688,1.),.UNSPECIFIED.);
#24353=B_SPLINE_CURVE_WITH_KNOTS('',5,(#183735,#183736,#183737,#183738,
#183739,#183740,#183741,#183742,#183743,#183744,#183745,#183746,#183747,
#183748,#183749,#183750,#183751,#183752,#183753,#183754,#183755,#183756,
#183757,#183758,#183759,#183760,#183761,#183762,#183763,#183764,#183765,
#183766,#183767,#183768,#183769,#183770,#183771,#183772,#183773,#183774,
#183775,#183776,#183777,#183778,#183779,#183780,#183781,#183782,#183783,
#183784,#183785,#183786,#183787,#183788,#183789,#183790,#183791,#183792,
#183793,#183794,#183795,#183796,#183797,#183798,#183799,#183800,#183801,
#183802,#183803,#183804,#183805,#183806,#183807,#183808,#183809,#183810,
#183811,#183812,#183813,#183814,#183815,#183816,#183817,#183818,#183819,
#183820,#183821,#183822,#183823,#183824,#183825,#183826,#183827,#183828,
#183829,#183830,#183831,#183832,#183833,#183834,#183835,#183836,#183837,
#183838,#183839,#183840,#183841,#183842,#183843,#183844,#183845,#183846,
#183847,#183848,#183849,#183850,#183851,#183852,#183853,#183854,#183855,
#183856,#183857,#183858,#183859,#183860,#183861,#183862,#183863,#183864,
#183865,#183866,#183867,#183868,#183869,#183870,#183871,#183872,#183873,
#183874,#183875,#183876,#183877,#183878,#183879,#183880,#183881,#183882,
#183883,#183884,#183885,#183886,#183887,#183888,#183889,#183890,#183891,
#183892,#183893,#183894,#183895,#183896,#183897,#183898,#183899,#183900,
#183901,#183902,#183903,#183904,#183905,#183906,#183907,#183908,#183909,
#183910,#183911,#183912,#183913,#183914,#183915,#183916,#183917,#183918,
#183919,#183920,#183921,#183922,#183923,#183924,#183925,#183926,#183927,
#183928,#183929,#183930,#183931,#183932,#183933,#183934,#183935,#183936,
#183937,#183938,#183939,#183940,#183941,#183942,#183943,#183944,#183945,
#183946,#183947,#183948,#183949,#183950,#183951,#183952,#183953,#183954,
#183955,#183956,#183957,#183958,#183959,#183960,#183961,#183962,#183963,
#183964,#183965,#183966,#183967,#183968,#183969,#183970,#183971,#183972,
#183973,#183974,#183975,#183976,#183977,#183978,#183979,#183980,#183981,
#183982,#183983,#183984,#183985,#183986,#183987,#183988,#183989,#183990,
#183991,#183992,#183993,#183994,#183995,#183996,#183997,#183998,#183999,
#184000,#184001,#184002,#184003,#184004,#184005,#184006,#184007,#184008,
#184009,#184010,#184011,#184012,#184013,#184014,#184015,#184016,#184017,
#184018,#184019,#184020,#184021,#184022,#184023,#184024,#184025,#184026,
#184027,#184028,#184029,#184030,#184031,#184032,#184033,#184034,#184035,
#184036,#184037,#184038,#184039,#184040,#184041,#184042,#184043,#184044,
#184045,#184046,#184047,#184048,#184049,#184050,#184051,#184052,#184053,
#184054,#184055,#184056,#184057,#184058,#184059,#184060,#184061,#184062,
#184063,#184064,#184065,#184066,#184067,#184068,#184069,#184070,#184071,
#184072,#184073,#184074,#184075,#184076,#184077,#184078,#184079,#184080,
#184081,#184082,#184083,#184084,#184085,#184086,#184087,#184088,#184089,
#184090,#184091,#184092,#184093,#184094,#184095,#184096,#184097,#184098,
#184099,#184100,#184101,#184102,#184103,#184104,#184105,#184106,#184107,
#184108,#184109,#184110,#184111,#184112,#184113,#184114,#184115,#184116,
#184117,#184118,#184119,#184120,#184121,#184122,#184123,#184124,#184125,
#184126,#184127,#184128,#184129,#184130,#184131,#184132,#184133,#184134,
#184135,#184136,#184137,#184138,#184139,#184140,#184141,#184142,#184143,
#184144,#184145,#184146,#184147,#184148,#184149,#184150,#184151,#184152,
#184153,#184154,#184155,#184156,#184157,#184158,#184159,#184160,#184161,
#184162,#184163,#184164,#184165,#184166,#184167,#184168,#184169,#184170,
#184171,#184172,#184173,#184174,#184175,#184176,#184177,#184178,#184179,
#184180,#184181,#184182,#184183,#184184,#184185,#184186,#184187,#184188,
#184189,#184190,#184191,#184192,#184193,#184194,#184195,#184196,#184197,
#184198,#184199,#184200,#184201,#184202,#184203,#184204,#184205,#184206),
 .UNSPECIFIED.,.F.,.F.,(6,1,1,1,1,1,1,1,1,1,1,1,1,1,1,1,1,1,1,1,1,1,1,1,
1,1,1,1,1,1,1,1,1,1,1,1,1,1,1,1,1,1,1,1,1,1,1,1,1,1,1,1,1,1,1,1,1,1,1,1,
1,1,1,1,1,1,1,1,1,1,1,1,1,1,1,1,1,1,1,1,1,1,1,1,1,1,1,1,1,1,1,1,1,1,1,1,
1,1,1,1,1,1,1,1,1,1,1,1,1,1,1,1,1,1,1,1,1,1,1,1,1,1,1,1,1,1,1,1,1,1,1,1,
1,1,1,1,1,1,1,1,1,1,1,1,1,1,1,1,1,1,1,1,1,1,1,1,1,1,1,1,1,1,1,1,1,1,1,1,
1,1,1,1,1,1,1,1,1,1,1,1,1,1,1,1,1,1,1,1,1,1,1,1,1,1,1,1,1,1,1,1,1,1,1,1,
1,1,1,1,1,1,1,1,1,1,1,1,1,1,1,1,1,1,1,1,1,1,1,1,1,1,1,1,1,1,1,1,1,1,1,1,
1,1,1,1,1,1,1,1,1,1,1,1,1,1,1,1,1,1,1,1,1,1,1,1,1,1,1,1,1,1,1,1,1,1,1,1,
1,1,1,1,1,1,1,1,1,1,1,1,1,1,1,1,1,1,1,1,1,1,1,1,1,1,1,1,1,1,1,1,1,1,1,1,
1,1,1,1,1,1,1,1,1,1,1,1,1,1,1,1,1,1,1,1,1,1,1,1,1,1,1,1,1,1,1,1,1,1,1,1,
1,1,1,1,1,1,1,1,1,1,1,1,1,1,1,1,1,1,1,1,1,1,1,1,1,1,1,1,1,1,1,1,1,1,1,1,
1,1,1,1,1,1,1,1,1,1,1,1,1,1,1,1,1,1,1,1,1,1,1,1,1,1,1,1,1,1,1,1,1,1,1,1,
1,1,1,1,1,1,1,1,1,1,1,1,1,1,1,1,1,1,1,1,1,1,1,1,1,1,1,1,1,1,1,1,1,1,1,1,
1,1,1,1,1,1,1,1,1,1,1,6),(-1.,-0.998165138,-0.996330275,-0.994495413,-0.99266055,
-0.990825688,-0.988990826,-0.987155963,-0.985321101,-0.983486239,-0.981651376,
-0.979816514,-0.977981651,-0.976146789,-0.974311927,-0.972477064,-0.970642202,
-0.968807339,-0.966972477,-0.965137615,-0.963302752,-0.96146789,-0.959633028,
-0.957798165,-0.955963303,-0.95412844,-0.952293578,-0.950458716,-0.948623853,
-0.946788991,-0.944954128,-0.943119266,-0.941284404,-0.939449541,-0.937614679,
-0.935779817,-0.933944954,-0.932110092,-0.930275229,-0.928440367,-0.926605505,
-0.924770642,-0.92293578,-0.921100917,-0.919266055,-0.917431193,-0.91559633,
-0.913761468,-0.911926606,-0.910091743,-0.908256881,-0.906422018,-0.904587156,
-0.902752294,-0.900917431,-0.899082569,-0.897247706,-0.895412844,-0.893577982,
-0.891743119,-0.889908257,-0.888073394,-0.886238532,-0.88440367,-0.882568807,
-0.880733945,-0.878899083,-0.87706422,-0.875229358,-0.873394495,-0.871559633,
-0.869724771,-0.867889908,-0.866055046,-0.864220183,-0.862385321,-0.860550459,
-0.858715596,-0.856880734,-0.855045872,-0.853211009,-0.851376147,-0.849541284,
-0.847706422,-0.84587156,-0.844036697,-0.842201835,-0.840366972,-0.83853211,
-0.836697248,-0.834862385,-0.833027523,-0.831192661,-0.829357798,-0.827522936,
-0.825688073,-0.823853211,-0.822018349,-0.820183486,-0.818348624,-0.816513761,
-0.814678899,-0.812844037,-0.811009174,-0.809174312,-0.80733945,-0.805504587,
-0.803669725,-0.801834862,-0.8,-0.798165138,-0.796330275,-0.794495413,-0.79266055,
-0.790825688,-0.788990826,-0.787155963,-0.785321101,-0.783486239,-0.781651376,
-0.779816514,-0.777981651,-0.776146789,-0.774311927,-0.772477064,-0.770642202,
-0.768807339,-0.766972477,-0.765137615,-0.763302752,-0.76146789,-0.759633028,
-0.757798165,-0.755963303,-0.75412844,-0.752293578,-0.750458716,-0.748623853,
-0.746788991,-0.744954128,-0.743119266,-0.741284404,-0.739449541,-0.737614679,
-0.735779817,-0.733944954,-0.732110092,-0.730275229,-0.728440367,-0.726605505,
-0.724770642,-0.72293578,-0.721100917,-0.719266055,-0.717431193,-0.71559633,
-0.713761468,-0.711926606,-0.710091743,-0.708256881,-0.706422018,-0.704587156,
-0.702752294,-0.700917431,-0.699082569,-0.697247706,-0.695412844,-0.693577982,
-0.691743119,-0.689908257,-0.688073394,-0.686238532,-0.68440367,-0.682568807,
-0.680733945,-0.678899083,-0.67706422,-0.675229358,-0.673394495,-0.671559633,
-0.669724771,-0.667889908,-0.666055046,-0.664220183,-0.662385321,-0.660550459,
-0.658715596,-0.656880734,-0.655045872,-0.653211009,-0.651376147,-0.649541284,
-0.647706422,-0.64587156,-0.644036697,-0.642201835,-0.640366972,-0.63853211,
-0.636697248,-0.634862385,-0.633027523,-0.631192661,-0.629357798,-0.627522936,
-0.625688073,-0.623853211,-0.622018349,-0.620183486,-0.618348624,-0.616513761,
-0.614678899,-0.612844037,-0.611009174,-0.609174312,-0.60733945,-0.605504587,
-0.603669725,-0.601834862,-0.6,-0.598165138,-0.596330275,-0.594495413,-0.59266055,
-0.590825688,-0.588990826,-0.587155963,-0.585321101,-0.583486239,-0.581651376,
-0.579816514,-0.577981651,-0.576146789,-0.574311927,-0.572477064,-0.570642202,
-0.568807339,-0.566972477,-0.565137615,-0.563302752,-0.56146789,-0.559633028,
-0.557798165,-0.555963303,-0.55412844,-0.552293578,-0.550458716,-0.548623853,
-0.546788991,-0.544954128,-0.543119266,-0.541284404,-0.539449541,-0.537614679,
-0.535779817,-0.533944954,-0.532110092,-0.530275229,-0.528440367,-0.526605505,
-0.524770642,-0.52293578,-0.521100917,-0.519266055,-0.517431193,-0.51559633,
-0.513761468,-0.511926606,-0.510091743,-0.508256881,-0.506422018,-0.504587156,
-0.502752294,-0.500917431,-0.499082569,-0.497247706,-0.495412844,-0.493577982,
-0.491743119,-0.489908257,-0.488073394,-0.486238532,-0.48440367,-0.482568807,
-0.480733945,-0.478899083,-0.47706422,-0.475229358,-0.473394495,-0.471559633,
-0.469724771,-0.467889908,-0.466055046,-0.464220183,-0.462385321,-0.460550459,
-0.458715596,-0.456880734,-0.455045872,-0.453211009,-0.451376147,-0.449541284,
-0.447706422,-0.44587156,-0.444036697,-0.442201835,-0.440366972,-0.43853211,
-0.436697248,-0.434862385,-0.433027523,-0.431192661,-0.429357798,-0.427522936,
-0.425688073,-0.423853211,-0.422018349,-0.420183486,-0.418348624,-0.416513761,
-0.414678899,-0.412844037,-0.411009174,-0.409174312,-0.40733945,-0.405504587,
-0.403669725,-0.401834862,-0.4,-0.398165138,-0.396330275,-0.394495413,-0.39266055,
-0.390825688,-0.388990826,-0.387155963,-0.385321101,-0.383486239,-0.381651376,
-0.379816514,-0.377981651,-0.376146789,-0.374311927,-0.372477064,-0.370642202,
-0.368807339,-0.366972477,-0.365137615,-0.363302752,-0.36146789,-0.359633028,
-0.357798165,-0.355963303,-0.35412844,-0.352293578,-0.350458716,-0.348623853,
-0.346788991,-0.344954128,-0.343119266,-0.341284404,-0.339449541,-0.337614679,
-0.335779817,-0.333944954,-0.332110092,-0.330275229,-0.328440367,-0.326605505,
-0.324770642,-0.32293578,-0.321100917,-0.319266055,-0.317431193,-0.31559633,
-0.313761468,-0.311926606,-0.310091743,-0.308256881,-0.306422018,-0.304587156,
-0.302752294,-0.300917431,-0.299082569,-0.297247706,-0.295412844,-0.293577982,
-0.291743119,-0.289908257,-0.288073394,-0.286238532,-0.28440367,-0.282568807,
-0.280733945,-0.278899083,-0.27706422,-0.275229358,-0.273394495,-0.271559633,
-0.269724771,-0.267889908,-0.266055046,-0.264220183,-0.262385321,-0.260550459,
-0.258715596,-0.256880734,-0.255045872,-0.253211009,-0.251376147,-0.249541284,
-0.247706422,-0.24587156,-0.244036697,-0.242201835,-0.240366972,-0.23853211,
-0.236697248,-0.234862385,-0.233027523,-0.231192661,-0.229357798,-0.227522936,
-0.225688073,-0.223853211,-0.222018349,-0.220183486,-0.218348624,-0.216513761,
-0.214678899,-0.212844037,-0.211009174,-0.209174312,-0.20733945,-0.205504587,
-0.203669725,-0.201834862,-0.2,-0.198165138,-0.196330275,-0.194495413,-0.19266055,
-0.190825688,-0.188990826,-0.187155963,-0.185321101,-0.183486239,-0.181651376,
-0.179816514,-0.177981651,-0.176146789,-0.174311927,-0.172477064,-0.170642202,
-0.168807339,-0.166972477,-0.165137615,-0.163302752,-0.16146789,-0.159633028,
-0.157798165,-0.155963303,-0.15412844,-0.152293578,-0.150458716,-0.148623853,
-0.146788991,-0.144954128,-0.143172102),.UNSPECIFIED.);
#24354=B_SPLINE_CURVE_WITH_KNOTS('',5,(#184207,#184208,#184209,#184210,
#184211,#184212,#184213,#184214,#184215,#184216,#184217,#184218,#184219,
#184220,#184221,#184222,#184223,#184224,#184225,#184226,#184227,#184228,
#184229,#184230,#184231,#184232,#184233,#184234,#184235,#184236,#184237,
#184238,#184239,#184240,#184241,#184242,#184243,#184244,#184245,#184246,
#184247,#184248,#184249,#184250,#184251,#184252,#184253,#184254,#184255,
#184256,#184257,#184258,#184259,#184260,#184261,#184262,#184263,#184264,
#184265,#184266,#184267,#184268,#184269,#184270,#184271,#184272,#184273,
#184274,#184275,#184276,#184277,#184278,#184279,#184280,#184281,#184282,
#184283,#184284,#184285,#184286,#184287,#184288,#184289,#184290,#184291,
#184292,#184293,#184294,#184295,#184296,#184297,#184298,#184299,#184300,
#184301,#184302,#184303,#184304,#184305,#184306,#184307,#184308,#184309,
#184310,#184311,#184312,#184313,#184314,#184315,#184316,#184317,#184318,
#184319,#184320,#184321,#184322,#184323,#184324,#184325,#184326,#184327,
#184328,#184329,#184330,#184331,#184332,#184333,#184334,#184335,#184336,
#184337,#184338,#184339,#184340,#184341,#184342,#184343,#184344,#184345,
#184346,#184347,#184348,#184349,#184350,#184351,#184352,#184353,#184354,
#184355,#184356,#184357,#184358,#184359,#184360,#184361,#184362,#184363,
#184364,#184365,#184366,#184367,#184368,#184369,#184370,#184371,#184372,
#184373,#184374,#184375,#184376,#184377,#184378,#184379,#184380,#184381,
#184382,#184383,#184384,#184385,#184386,#184387,#184388,#184389,#184390,
#184391,#184392,#184393,#184394,#184395,#184396,#184397,#184398,#184399,
#184400,#184401,#184402,#184403,#184404,#184405,#184406,#184407,#184408,
#184409,#184410,#184411,#184412,#184413,#184414,#184415,#184416,#184417,
#184418,#184419,#184420,#184421,#184422,#184423,#184424,#184425,#184426,
#184427,#184428,#184429,#184430,#184431,#184432,#184433,#184434,#184435,
#184436,#184437,#184438,#184439,#184440,#184441,#184442,#184443,#184444,
#184445,#184446,#184447,#184448,#184449,#184450,#184451,#184452,#184453,
#184454,#184455,#184456,#184457,#184458,#184459,#184460,#184461,#184462,
#184463,#184464,#184465,#184466,#184467,#184468,#184469,#184470,#184471,
#184472,#184473,#184474,#184475,#184476,#184477,#184478,#184479,#184480,
#184481,#184482,#184483,#184484,#184485,#184486,#184487,#184488,#184489,
#184490,#184491,#184492,#184493,#184494,#184495,#184496,#184497,#184498,
#184499,#184500,#184501,#184502,#184503,#184504,#184505,#184506,#184507,
#184508,#184509,#184510,#184511,#184512,#184513,#184514,#184515,#184516,
#184517,#184518,#184519,#184520,#184521,#184522,#184523,#184524,#184525,
#184526,#184527,#184528,#184529,#184530,#184531,#184532,#184533,#184534,
#184535,#184536,#184537,#184538,#184539,#184540,#184541,#184542,#184543,
#184544,#184545,#184546,#184547,#184548,#184549,#184550,#184551,#184552,
#184553,#184554,#184555,#184556,#184557,#184558,#184559,#184560,#184561,
#184562,#184563,#184564,#184565,#184566,#184567,#184568,#184569,#184570,
#184571,#184572,#184573,#184574,#184575,#184576,#184577,#184578,#184579,
#184580,#184581,#184582,#184583,#184584,#184585,#184586,#184587,#184588,
#184589,#184590,#184591,#184592,#184593,#184594,#184595,#184596,#184597,
#184598,#184599,#184600,#184601,#184602,#184603,#184604,#184605,#184606,
#184607,#184608,#184609,#184610,#184611,#184612,#184613,#184614,#184615,
#184616,#184617,#184618,#184619,#184620,#184621,#184622,#184623,#184624,
#184625,#184626,#184627,#184628,#184629,#184630,#184631,#184632,#184633,
#184634,#184635,#184636,#184637,#184638,#184639,#184640,#184641,#184642,
#184643,#184644,#184645,#184646,#184647,#184648,#184649,#184650,#184651,
#184652,#184653,#184654,#184655,#184656,#184657,#184658,#184659,#184660,
#184661,#184662,#184663,#184664,#184665,#184666,#184667,#184668,#184669,
#184670,#184671,#184672,#184673,#184674,#184675,#184676,#184677,#184678),
 .UNSPECIFIED.,.F.,.F.,(6,1,1,1,1,1,1,1,1,1,1,1,1,1,1,1,1,1,1,1,1,1,1,1,
1,1,1,1,1,1,1,1,1,1,1,1,1,1,1,1,1,1,1,1,1,1,1,1,1,1,1,1,1,1,1,1,1,1,1,1,
1,1,1,1,1,1,1,1,1,1,1,1,1,1,1,1,1,1,1,1,1,1,1,1,1,1,1,1,1,1,1,1,1,1,1,1,
1,1,1,1,1,1,1,1,1,1,1,1,1,1,1,1,1,1,1,1,1,1,1,1,1,1,1,1,1,1,1,1,1,1,1,1,
1,1,1,1,1,1,1,1,1,1,1,1,1,1,1,1,1,1,1,1,1,1,1,1,1,1,1,1,1,1,1,1,1,1,1,1,
1,1,1,1,1,1,1,1,1,1,1,1,1,1,1,1,1,1,1,1,1,1,1,1,1,1,1,1,1,1,1,1,1,1,1,1,
1,1,1,1,1,1,1,1,1,1,1,1,1,1,1,1,1,1,1,1,1,1,1,1,1,1,1,1,1,1,1,1,1,1,1,1,
1,1,1,1,1,1,1,1,1,1,1,1,1,1,1,1,1,1,1,1,1,1,1,1,1,1,1,1,1,1,1,1,1,1,1,1,
1,1,1,1,1,1,1,1,1,1,1,1,1,1,1,1,1,1,1,1,1,1,1,1,1,1,1,1,1,1,1,1,1,1,1,1,
1,1,1,1,1,1,1,1,1,1,1,1,1,1,1,1,1,1,1,1,1,1,1,1,1,1,1,1,1,1,1,1,1,1,1,1,
1,1,1,1,1,1,1,1,1,1,1,1,1,1,1,1,1,1,1,1,1,1,1,1,1,1,1,1,1,1,1,1,1,1,1,1,
1,1,1,1,1,1,1,1,1,1,1,1,1,1,1,1,1,1,1,1,1,1,1,1,1,1,1,1,1,1,1,1,1,1,1,1,
1,1,1,1,1,1,1,1,1,1,1,1,1,1,1,1,1,1,1,1,1,1,1,1,1,1,1,1,1,1,1,1,1,1,1,1,
1,1,1,1,1,1,1,1,1,1,1,6),(0.143172102,0.144954128,0.146788991,0.148623853,
0.150458716,0.152293578,0.15412844,0.155963303,0.157798165,0.159633028,
0.16146789,0.163302752,0.165137615,0.166972477,0.168807339,0.170642202,
0.172477064,0.174311927,0.176146789,0.177981651,0.179816514,0.181651376,
0.183486239,0.185321101,0.187155963,0.188990826,0.190825688,0.19266055,
0.194495413,0.196330275,0.198165138,0.2,0.201834862,0.203669725,0.205504587,
0.20733945,0.209174312,0.211009174,0.212844037,0.214678899,0.216513761,
0.218348624,0.220183486,0.222018349,0.223853211,0.225688073,0.227522936,
0.229357798,0.231192661,0.233027523,0.234862385,0.236697248,0.23853211,
0.240366972,0.242201835,0.244036697,0.24587156,0.247706422,0.249541284,
0.251376147,0.253211009,0.255045872,0.256880734,0.258715596,0.260550459,
0.262385321,0.264220183,0.266055046,0.267889908,0.269724771,0.271559633,
0.273394495,0.275229358,0.27706422,0.278899083,0.280733945,0.282568807,
0.28440367,0.286238532,0.288073394,0.289908257,0.291743119,0.293577982,
0.295412844,0.297247706,0.299082569,0.300917431,0.302752294,0.304587156,
0.306422018,0.308256881,0.310091743,0.311926606,0.313761468,0.31559633,
0.317431193,0.319266055,0.321100917,0.32293578,0.324770642,0.326605505,
0.328440367,0.330275229,0.332110092,0.333944954,0.335779817,0.337614679,
0.339449541,0.341284404,0.343119266,0.344954128,0.346788991,0.348623853,
0.350458716,0.352293578,0.35412844,0.355963303,0.357798165,0.359633028,
0.36146789,0.363302752,0.365137615,0.366972477,0.368807339,0.370642202,
0.372477064,0.374311927,0.376146789,0.377981651,0.379816514,0.381651376,
0.383486239,0.385321101,0.387155963,0.388990826,0.390825688,0.39266055,
0.394495413,0.396330275,0.398165138,0.4,0.401834862,0.403669725,0.405504587,
0.40733945,0.409174312,0.411009174,0.412844037,0.414678899,0.416513761,
0.418348624,0.420183486,0.422018349,0.423853211,0.425688073,0.427522936,
0.429357798,0.431192661,0.433027523,0.434862385,0.436697248,0.43853211,
0.440366972,0.442201835,0.444036697,0.44587156,0.447706422,0.449541284,
0.451376147,0.453211009,0.455045872,0.456880734,0.458715596,0.460550459,
0.462385321,0.464220183,0.466055046,0.467889908,0.469724771,0.471559633,
0.473394495,0.475229358,0.47706422,0.478899083,0.480733945,0.482568807,
0.48440367,0.486238532,0.488073394,0.489908257,0.491743119,0.493577982,
0.495412844,0.497247706,0.499082569,0.500917431,0.502752294,0.504587156,
0.506422018,0.508256881,0.510091743,0.511926606,0.513761468,0.51559633,
0.517431193,0.519266055,0.521100917,0.52293578,0.524770642,0.526605505,
0.528440367,0.530275229,0.532110092,0.533944954,0.535779817,0.537614679,
0.539449541,0.541284404,0.543119266,0.544954128,0.546788991,0.548623853,
0.550458716,0.552293578,0.55412844,0.555963303,0.557798165,0.559633028,
0.56146789,0.563302752,0.565137615,0.566972477,0.568807339,0.570642202,
0.572477064,0.574311927,0.576146789,0.577981651,0.579816514,0.581651376,
0.583486239,0.585321101,0.587155963,0.588990826,0.590825688,0.59266055,
0.594495413,0.596330275,0.598165138,0.6,0.601834862,0.603669725,0.605504587,
0.60733945,0.609174312,0.611009174,0.612844037,0.614678899,0.616513761,
0.618348624,0.620183486,0.622018349,0.623853211,0.625688073,0.627522936,
0.629357798,0.631192661,0.633027523,0.634862385,0.636697248,0.63853211,
0.640366972,0.642201835,0.644036697,0.64587156,0.647706422,0.649541284,
0.651376147,0.653211009,0.655045872,0.656880734,0.658715596,0.660550459,
0.662385321,0.664220183,0.666055046,0.667889908,0.669724771,0.671559633,
0.673394495,0.675229358,0.67706422,0.678899083,0.680733945,0.682568807,
0.68440367,0.686238532,0.688073394,0.689908257,0.691743119,0.693577982,
0.695412844,0.697247706,0.699082569,0.700917431,0.702752294,0.704587156,
0.706422018,0.708256881,0.710091743,0.711926606,0.713761468,0.71559633,
0.717431193,0.719266055,0.721100917,0.72293578,0.724770642,0.726605505,
0.728440367,0.730275229,0.732110092,0.733944954,0.735779817,0.737614679,
0.739449541,0.741284404,0.743119266,0.744954128,0.746788991,0.748623853,
0.750458716,0.752293578,0.75412844,0.755963303,0.757798165,0.759633028,
0.76146789,0.763302752,0.765137615,0.766972477,0.768807339,0.770642202,
0.772477064,0.774311927,0.776146789,0.777981651,0.779816514,0.781651376,
0.783486239,0.785321101,0.787155963,0.788990826,0.790825688,0.79266055,
0.794495413,0.796330275,0.798165138,0.8,0.801834862,0.803669725,0.805504587,
0.80733945,0.809174312,0.811009174,0.812844037,0.814678899,0.816513761,
0.818348624,0.820183486,0.822018349,0.823853211,0.825688073,0.827522936,
0.829357798,0.831192661,0.833027523,0.834862385,0.836697248,0.83853211,
0.840366972,0.842201835,0.844036697,0.84587156,0.847706422,0.849541284,
0.851376147,0.853211009,0.855045872,0.856880734,0.858715596,0.860550459,
0.862385321,0.864220183,0.866055046,0.867889908,0.869724771,0.871559633,
0.873394495,0.875229358,0.87706422,0.878899083,0.880733945,0.882568807,
0.88440367,0.886238532,0.888073394,0.889908257,0.891743119,0.893577982,
0.895412844,0.897247706,0.899082569,0.900917431,0.902752294,0.904587156,
0.906422018,0.908256881,0.910091743,0.911926606,0.913761468,0.91559633,
0.917431193,0.919266055,0.921100917,0.92293578,0.924770642,0.926605505,
0.928440367,0.930275229,0.932110092,0.933944954,0.935779817,0.937614679,
0.939449541,0.941284404,0.943119266,0.944954128,0.946788991,0.948623853,
0.950458716,0.952293578,0.95412844,0.955963303,0.957798165,0.959633028,
0.96146789,0.963302752,0.965137615,0.966972477,0.968807339,0.970642202,
0.972477064,0.974311927,0.976146789,0.977981651,0.979816514,0.981651376,
0.983486239,0.985321101,0.987155963,0.988990826,0.990825688,0.99266055,
0.994495413,0.996330275,0.998165138,1.),.UNSPECIFIED.);
#24355=B_SPLINE_CURVE_WITH_KNOTS('',3,(#185641,#185642,#185643,#185644,
#185645,#185646,#185647,#185648,#185649,#185650,#185651,#185652,#185653,
#185654,#185655,#185656,#185657,#185658,#185659,#185660,#185661,#185662,
#185663,#185664,#185665,#185666,#185667,#185668,#185669,#185670,#185671,
#185672,#185673,#185674,#185675,#185676,#185677,#185678,#185679,#185680,
#185681,#185682,#185683,#185684,#185685,#185686,#185687,#185688,#185689,
#185690,#185691,#185692,#185693,#185694,#185695,#185696,#185697,#185698,
#185699,#185700,#185701,#185702,#185703,#185704,#185705,#185706,#185707,
#185708,#185709,#185710,#185711,#185712,#185713,#185714,#185715,#185716,
#185717,#185718,#185719,#185720,#185721,#185722,#185723,#185724,#185725,
#185726,#185727,#185728,#185729,#185730,#185731,#185732,#185733,#185734,
#185735,#185736,#185737,#185738,#185739,#185740,#185741,#185742,#185743,
#185744,#185745,#185746,#185747,#185748,#185749,#185750,#185751,#185752,
#185753,#185754,#185755,#185756,#185757,#185758,#185759,#185760,#185761,
#185762,#185763,#185764,#185765,#185766,#185767,#185768,#185769,#185770,
#185771,#185772,#185773,#185774,#185775,#185776,#185777,#185778,#185779,
#185780,#185781,#185782,#185783,#185784,#185785,#185786,#185787,#185788,
#185789,#185790,#185791,#185792,#185793,#185794,#185795,#185796,#185797,
#185798,#185799,#185800,#185801,#185802,#185803,#185804,#185805,#185806,
#185807,#185808,#185809,#185810,#185811,#185812,#185813,#185814,#185815,
#185816,#185817,#185818,#185819,#185820,#185821,#185822,#185823,#185824,
#185825,#185826,#185827,#185828,#185829,#185830,#185831,#185832,#185833,
#185834,#185835,#185836,#185837,#185838,#185839,#185840,#185841,#185842,
#185843,#185844,#185845,#185846,#185847,#185848,#185849,#185850,#185851,
#185852,#185853,#185854,#185855,#185856,#185857,#185858,#185859,#185860,
#185861,#185862,#185863,#185864,#185865,#185866,#185867,#185868,#185869,
#185870,#185871,#185872,#185873,#185874,#185875,#185876,#185877,#185878,
#185879,#185880,#185881,#185882,#185883,#185884,#185885,#185886,#185887,
#185888,#185889,#185890,#185891,#185892,#185893,#185894,#185895,#185896,
#185897,#185898,#185899,#185900,#185901,#185902,#185903,#185904,#185905,
#185906,#185907,#185908,#185909,#185910,#185911,#185912,#185913,#185914,
#185915,#185916,#185917,#185918,#185919,#185920,#185921,#185922,#185923,
#185924,#185925,#185926,#185927,#185928,#185929,#185930,#185931,#185932,
#185933,#185934,#185935,#185936,#185937,#185938,#185939,#185940,#185941,
#185942,#185943,#185944,#185945,#185946,#185947,#185948,#185949,#185950,
#185951,#185952,#185953,#185954,#185955,#185956,#185957,#185958,#185959,
#185960,#185961,#185962,#185963,#185964,#185965,#185966,#185967,#185968),
 .UNSPECIFIED.,.F.,.F.,(4,3,3,3,3,3,3,3,3,3,3,3,3,3,3,3,3,3,3,3,3,3,3,3,
3,3,3,3,3,3,3,3,3,3,3,3,3,3,3,3,3,3,3,3,3,3,3,3,3,3,3,3,3,3,3,3,3,3,3,3,
3,3,3,3,3,3,3,3,3,3,3,3,3,3,3,3,3,3,3,3,3,3,3,3,3,3,3,3,3,3,3,3,3,3,3,3,
3,3,3,3,3,3,3,3,3,3,3,3,3,4),(-1.,-0.994495413,-0.988990826,-0.983486239,
-0.977981651,-0.972477064,-0.966972477,-0.959633028,-0.95412844,-0.948623853,
-0.943119266,-0.937614679,-0.932110092,-0.926605505,-0.921100917,-0.91559633,
-0.910091743,-0.904587156,-0.899082569,-0.893577982,-0.888073394,-0.882568807,
-0.87706422,-0.871559633,-0.866055046,-0.860550459,-0.855045872,-0.849541284,
-0.842201835,-0.836697248,-0.831192661,-0.825688073,-0.818348624,-0.812844037,
-0.80733945,-0.8,-0.79266055,-0.785321101,-0.777981651,-0.770642202,-0.763302752,
-0.755963303,-0.748623853,-0.741284404,-0.733944954,-0.726605505,-0.719266055,
-0.711926606,-0.704587156,-0.697247706,-0.689908257,-0.682568807,-0.675229358,
-0.667889908,-0.660550459,-0.653211009,-0.64587156,-0.63853211,-0.631192661,
-0.623853211,-0.616513761,-0.609174312,-0.601834862,-0.59266055,-0.585321101,
-0.577981651,-0.570642202,-0.563302752,-0.555963303,-0.548623853,-0.541284404,
-0.533944954,-0.526605505,-0.517431193,-0.508256881,-0.499082569,-0.489908257,
-0.480733945,-0.471559633,-0.462385321,-0.453211009,-0.444036697,-0.434862385,
-0.425688073,-0.414678899,-0.405504587,-0.396330275,-0.387155963,-0.374311927,
-0.363302752,-0.352293578,-0.341284404,-0.330275229,-0.319266055,-0.308256881,
-0.297247706,-0.286238532,-0.275229358,-0.264220183,-0.253211009,-0.242201835,
-0.231192661,-0.220183486,-0.209174312,-0.198165138,-0.187155963,-0.176146789,
-0.165137615,-0.15412844,-0.143172102),.UNSPECIFIED.);
#24356=B_SPLINE_CURVE_WITH_KNOTS('',3,(#185969,#185970,#185971,#185972,
#185973,#185974,#185975,#185976,#185977,#185978,#185979,#185980,#185981,
#185982,#185983,#185984,#185985,#185986,#185987,#185988,#185989,#185990,
#185991,#185992,#185993,#185994,#185995,#185996,#185997,#185998,#185999,
#186000,#186001,#186002,#186003,#186004,#186005,#186006,#186007,#186008,
#186009,#186010,#186011,#186012,#186013,#186014,#186015,#186016,#186017,
#186018,#186019,#186020,#186021,#186022,#186023,#186024,#186025,#186026,
#186027,#186028,#186029,#186030,#186031,#186032,#186033,#186034,#186035,
#186036,#186037,#186038,#186039,#186040,#186041,#186042,#186043,#186044,
#186045,#186046,#186047,#186048,#186049,#186050,#186051,#186052,#186053,
#186054,#186055,#186056,#186057,#186058,#186059,#186060,#186061,#186062,
#186063,#186064,#186065,#186066,#186067,#186068,#186069,#186070,#186071,
#186072,#186073,#186074,#186075,#186076,#186077,#186078,#186079,#186080,
#186081,#186082,#186083,#186084,#186085,#186086,#186087,#186088,#186089,
#186090,#186091,#186092,#186093,#186094,#186095,#186096,#186097,#186098,
#186099,#186100,#186101,#186102,#186103,#186104,#186105,#186106,#186107,
#186108,#186109,#186110,#186111,#186112,#186113,#186114,#186115,#186116,
#186117,#186118,#186119,#186120,#186121,#186122,#186123,#186124,#186125,
#186126,#186127,#186128,#186129,#186130,#186131,#186132,#186133,#186134,
#186135,#186136,#186137,#186138,#186139,#186140,#186141,#186142,#186143,
#186144,#186145,#186146,#186147,#186148,#186149,#186150,#186151,#186152,
#186153,#186154,#186155,#186156,#186157,#186158,#186159,#186160,#186161,
#186162,#186163,#186164,#186165,#186166,#186167,#186168,#186169,#186170,
#186171,#186172,#186173,#186174,#186175,#186176,#186177,#186178,#186179,
#186180,#186181,#186182,#186183,#186184,#186185,#186186,#186187,#186188,
#186189,#186190,#186191,#186192,#186193,#186194,#186195,#186196,#186197,
#186198,#186199,#186200,#186201,#186202,#186203,#186204,#186205,#186206,
#186207,#186208,#186209,#186210,#186211,#186212,#186213,#186214,#186215,
#186216,#186217,#186218,#186219,#186220,#186221,#186222,#186223,#186224,
#186225,#186226,#186227,#186228,#186229,#186230,#186231,#186232,#186233,
#186234,#186235,#186236,#186237,#186238,#186239,#186240,#186241,#186242,
#186243,#186244,#186245,#186246,#186247,#186248,#186249,#186250,#186251,
#186252,#186253,#186254,#186255,#186256,#186257,#186258,#186259,#186260,
#186261,#186262,#186263,#186264,#186265,#186266,#186267,#186268,#186269,
#186270,#186271,#186272,#186273,#186274,#186275,#186276,#186277,#186278),
 .UNSPECIFIED.,.F.,.F.,(4,3,3,3,3,3,3,3,3,3,3,3,3,3,3,3,3,3,3,3,3,3,3,3,
3,3,3,3,3,3,3,3,3,3,3,3,3,3,3,3,3,3,3,3,3,3,3,3,3,3,3,3,3,3,3,3,3,3,3,3,
3,3,3,3,3,3,3,3,3,3,3,3,3,3,3,3,3,3,3,3,3,3,3,3,3,3,3,3,3,3,3,3,3,3,3,3,
3,3,3,3,3,3,3,4),(0.143172102,0.15412844,0.165137615,0.176146789,0.187155963,
0.198165138,0.209174312,0.220183486,0.231192661,0.242201835,0.253211009,
0.264220183,0.275229358,0.286238532,0.297247706,0.308256881,0.319266055,
0.330275229,0.341284404,0.352293578,0.363302752,0.374311927,0.388990826,
0.398165138,0.40733945,0.416513761,0.425688073,0.434862385,0.444036697,
0.453211009,0.462385321,0.473394495,0.482568807,0.491743119,0.504587156,
0.51559633,0.524770642,0.533944954,0.541284404,0.548623853,0.555963303,
0.563302752,0.570642202,0.577981651,0.585321101,0.59266055,0.601834862,
0.609174312,0.616513761,0.625688073,0.633027523,0.640366972,0.649541284,
0.658715596,0.666055046,0.673394495,0.680733945,0.688073394,0.695412844,
0.706422018,0.713761468,0.721100917,0.730275229,0.739449541,0.746788991,
0.75412844,0.76146789,0.768807339,0.777981651,0.785321101,0.79266055,0.8,
0.80733945,0.812844037,0.818348624,0.823853211,0.829357798,0.836697248,
0.842201835,0.849541284,0.855045872,0.860550459,0.866055046,0.871559633,
0.878899083,0.888073394,0.893577982,0.899082569,0.904587156,0.910091743,
0.917431193,0.924770642,0.930275229,0.939449541,0.944954128,0.950458716,
0.955963303,0.96146789,0.966972477,0.972477064,0.977981651,0.985321101,
0.99266055,1.),.UNSPECIFIED.);
#24357=B_SPLINE_CURVE_WITH_KNOTS('',3,(#187223,#187224,#187225,#187226,
#187227,#187228,#187229,#187230,#187231,#187232,#187233,#187234,#187235,
#187236,#187237,#187238,#187239,#187240,#187241,#187242,#187243,#187244,
#187245,#187246,#187247,#187248,#187249,#187250,#187251,#187252,#187253,
#187254,#187255,#187256,#187257,#187258,#187259,#187260,#187261,#187262,
#187263,#187264,#187265,#187266,#187267,#187268,#187269,#187270,#187271,
#187272,#187273,#187274,#187275,#187276,#187277,#187278,#187279,#187280,
#187281,#187282,#187283,#187284,#187285,#187286,#187287,#187288,#187289,
#187290,#187291,#187292,#187293,#187294,#187295,#187296,#187297,#187298,
#187299,#187300,#187301,#187302,#187303,#187304,#187305,#187306,#187307,
#187308,#187309,#187310,#187311,#187312,#187313,#187314,#187315,#187316,
#187317,#187318,#187319,#187320,#187321,#187322,#187323,#187324,#187325,
#187326,#187327,#187328,#187329,#187330,#187331,#187332,#187333,#187334,
#187335,#187336,#187337,#187338,#187339,#187340,#187341,#187342,#187343,
#187344,#187345,#187346,#187347,#187348,#187349,#187350,#187351,#187352,
#187353,#187354,#187355,#187356,#187357,#187358,#187359,#187360,#187361,
#187362,#187363,#187364,#187365,#187366,#187367,#187368,#187369,#187370,
#187371,#187372,#187373,#187374,#187375,#187376,#187377,#187378,#187379,
#187380,#187381,#187382,#187383,#187384,#187385,#187386,#187387,#187388,
#187389,#187390,#187391,#187392,#187393,#187394,#187395,#187396,#187397,
#187398,#187399,#187400,#187401,#187402,#187403,#187404,#187405,#187406,
#187407,#187408,#187409,#187410,#187411,#187412,#187413,#187414,#187415,
#187416,#187417,#187418,#187419,#187420,#187421,#187422,#187423,#187424,
#187425,#187426,#187427,#187428,#187429,#187430,#187431,#187432,#187433,
#187434,#187435,#187436,#187437,#187438,#187439,#187440,#187441,#187442,
#187443,#187444,#187445,#187446,#187447,#187448,#187449,#187450,#187451,
#187452,#187453,#187454,#187455,#187456,#187457,#187458,#187459,#187460,
#187461,#187462,#187463,#187464,#187465,#187466,#187467,#187468,#187469,
#187470,#187471,#187472,#187473,#187474,#187475,#187476,#187477,#187478,
#187479,#187480,#187481,#187482,#187483,#187484,#187485,#187486,#187487,
#187488,#187489,#187490,#187491,#187492,#187493,#187494,#187495,#187496,
#187497,#187498,#187499,#187500,#187501,#187502,#187503,#187504,#187505,
#187506,#187507,#187508,#187509,#187510,#187511,#187512,#187513,#187514,
#187515,#187516,#187517,#187518,#187519,#187520,#187521,#187522,#187523,
#187524,#187525,#187526,#187527,#187528,#187529,#187530,#187531,#187532,
#187533,#187534,#187535,#187536,#187537,#187538,#187539,#187540,#187541,
#187542,#187543,#187544),.UNSPECIFIED.,.F.,.F.,(4,3,3,3,3,3,3,3,3,3,3,3,
3,3,3,3,3,3,3,3,3,3,3,3,3,3,3,3,3,3,3,3,3,3,3,3,3,3,3,3,3,3,3,3,3,3,3,3,
3,3,3,3,3,3,3,3,3,3,3,3,3,3,3,3,3,3,3,3,3,3,3,3,3,3,3,3,3,3,3,3,3,3,3,3,
3,3,3,3,3,3,3,3,3,3,3,3,3,3,3,3,3,3,3,3,3,3,3,4),(0.143172102,0.15412844,
0.165137615,0.176146789,0.187155963,0.198165138,0.209174312,0.222018349,
0.233027523,0.244036697,0.255045872,0.266055046,0.27706422,0.288073394,
0.299082569,0.311926606,0.32293578,0.335779817,0.346788991,0.357798165,
0.368807339,0.379816514,0.390825688,0.4,0.409174312,0.418348624,0.427522936,
0.436697248,0.44587156,0.455045872,0.464220183,0.473394495,0.482568807,
0.491743119,0.500917431,0.510091743,0.519266055,0.528440367,0.535779817,
0.543119266,0.550458716,0.557798165,0.565137615,0.572477064,0.579816514,
0.587155963,0.594495413,0.601834862,0.609174312,0.616513761,0.623853211,
0.631192661,0.63853211,0.64587156,0.655045872,0.662385321,0.671559633,0.678899083,
0.686238532,0.693577982,0.700917431,0.708256881,0.71559633,0.72293578,0.730275229,
0.737614679,0.746788991,0.75412844,0.76146789,0.768807339,0.776146789,0.783486239,
0.790825688,0.798165138,0.805504587,0.811009174,0.818348624,0.823853211,
0.831192661,0.836697248,0.842201835,0.847706422,0.855045872,0.860550459,
0.869724771,0.875229358,0.880733945,0.886238532,0.891743119,0.897247706,
0.902752294,0.908256881,0.913761468,0.919266055,0.926605505,0.932110092,
0.937614679,0.943119266,0.948623853,0.95412844,0.959633028,0.966972477,
0.972477064,0.977981651,0.983486239,0.988990826,0.994495413,1.),
 .UNSPECIFIED.);
#24358=B_SPLINE_CURVE_WITH_KNOTS('',3,(#187545,#187546,#187547,#187548,
#187549,#187550,#187551,#187552,#187553,#187554,#187555,#187556,#187557,
#187558,#187559,#187560,#187561,#187562,#187563,#187564,#187565,#187566,
#187567,#187568,#187569,#187570,#187571,#187572,#187573,#187574,#187575,
#187576,#187577,#187578,#187579,#187580,#187581,#187582,#187583,#187584,
#187585,#187586,#187587,#187588,#187589,#187590,#187591,#187592,#187593,
#187594,#187595,#187596,#187597,#187598,#187599,#187600,#187601,#187602,
#187603,#187604,#187605,#187606,#187607,#187608,#187609,#187610,#187611,
#187612,#187613,#187614,#187615,#187616,#187617,#187618,#187619,#187620,
#187621,#187622,#187623,#187624,#187625,#187626,#187627,#187628,#187629,
#187630,#187631,#187632,#187633,#187634,#187635,#187636,#187637,#187638,
#187639,#187640,#187641,#187642,#187643,#187644,#187645,#187646,#187647,
#187648,#187649,#187650,#187651,#187652,#187653,#187654,#187655,#187656,
#187657,#187658,#187659,#187660,#187661,#187662,#187663,#187664,#187665,
#187666,#187667,#187668,#187669,#187670,#187671,#187672,#187673,#187674,
#187675,#187676,#187677,#187678,#187679,#187680,#187681,#187682,#187683,
#187684,#187685,#187686,#187687,#187688,#187689,#187690,#187691,#187692,
#187693,#187694,#187695,#187696,#187697,#187698,#187699,#187700,#187701,
#187702,#187703,#187704,#187705,#187706,#187707,#187708,#187709,#187710,
#187711,#187712,#187713,#187714,#187715,#187716,#187717,#187718,#187719,
#187720,#187721,#187722,#187723,#187724,#187725,#187726,#187727,#187728,
#187729,#187730,#187731,#187732,#187733,#187734,#187735,#187736,#187737,
#187738,#187739,#187740,#187741,#187742,#187743,#187744,#187745,#187746,
#187747,#187748,#187749,#187750,#187751,#187752,#187753,#187754,#187755,
#187756,#187757,#187758,#187759,#187760,#187761,#187762,#187763,#187764,
#187765,#187766,#187767,#187768,#187769,#187770,#187771,#187772,#187773,
#187774,#187775,#187776,#187777,#187778,#187779,#187780,#187781,#187782,
#187783,#187784,#187785,#187786,#187787,#187788,#187789,#187790,#187791,
#187792,#187793,#187794,#187795,#187796,#187797,#187798,#187799,#187800,
#187801,#187802,#187803,#187804,#187805,#187806,#187807,#187808,#187809,
#187810,#187811,#187812,#187813,#187814,#187815,#187816,#187817,#187818,
#187819,#187820,#187821,#187822,#187823,#187824,#187825,#187826,#187827,
#187828,#187829,#187830,#187831,#187832,#187833,#187834,#187835,#187836,
#187837,#187838,#187839,#187840,#187841,#187842,#187843,#187844,#187845,
#187846,#187847,#187848,#187849,#187850,#187851,#187852,#187853,#187854,
#187855,#187856,#187857,#187858,#187859,#187860,#187861,#187862,#187863,
#187864,#187865,#187866),.UNSPECIFIED.,.F.,.F.,(4,3,3,3,3,3,3,3,3,3,3,3,
3,3,3,3,3,3,3,3,3,3,3,3,3,3,3,3,3,3,3,3,3,3,3,3,3,3,3,3,3,3,3,3,3,3,3,3,
3,3,3,3,3,3,3,3,3,3,3,3,3,3,3,3,3,3,3,3,3,3,3,3,3,3,3,3,3,3,3,3,3,3,3,3,
3,3,3,3,3,3,3,3,3,3,3,3,3,3,3,3,3,3,3,3,3,3,3,4),(0.143172102,0.15412844,
0.165137615,0.176146789,0.187155963,0.198165138,0.209174312,0.220183486,
0.231192661,0.242201835,0.253211009,0.264220183,0.275229358,0.286238532,
0.297247706,0.308256881,0.319266055,0.330275229,0.341284404,0.352293578,
0.363302752,0.374311927,0.385321101,0.398165138,0.40733945,0.416513761,
0.425688073,0.434862385,0.444036697,0.453211009,0.464220183,0.473394495,
0.48440367,0.493577982,0.502752294,0.511926606,0.521100917,0.530275229,
0.537614679,0.544954128,0.552293578,0.559633028,0.566972477,0.574311927,
0.581651376,0.588990826,0.596330275,0.603669725,0.612844037,0.620183486,
0.627522936,0.634862385,0.642201835,0.649541284,0.656880734,0.664220183,
0.673394495,0.680733945,0.688073394,0.695412844,0.704587156,0.711926606,
0.719266055,0.726605505,0.733944954,0.741284404,0.748623853,0.755963303,
0.763302752,0.770642202,0.777981651,0.785321101,0.79266055,0.8,0.809174312,
0.814678899,0.820183486,0.825688073,0.831192661,0.836697248,0.842201835,
0.847706422,0.853211009,0.858715596,0.864220183,0.869724771,0.875229358,
0.880733945,0.888073394,0.893577982,0.899082569,0.904587156,0.910091743,
0.91559633,0.921100917,0.930275229,0.935779817,0.941284404,0.946788991,
0.952293578,0.957798165,0.963302752,0.968807339,0.974311927,0.979816514,
0.985321101,0.990825688,1.),.UNSPECIFIED.);
#24359=B_SPLINE_CURVE_WITH_KNOTS('',3,(#188826,#188827,#188828,#188829,
#188830,#188831,#188832,#188833,#188834,#188835,#188836,#188837,#188838,
#188839,#188840,#188841,#188842,#188843,#188844,#188845,#188846,#188847,
#188848,#188849,#188850,#188851,#188852,#188853,#188854,#188855,#188856,
#188857,#188858,#188859,#188860,#188861,#188862,#188863,#188864,#188865,
#188866,#188867,#188868,#188869,#188870,#188871,#188872,#188873,#188874,
#188875,#188876,#188877,#188878,#188879,#188880,#188881,#188882,#188883,
#188884,#188885,#188886,#188887,#188888,#188889,#188890,#188891,#188892,
#188893,#188894,#188895,#188896,#188897,#188898,#188899,#188900,#188901,
#188902,#188903,#188904,#188905,#188906,#188907,#188908,#188909,#188910,
#188911,#188912,#188913,#188914,#188915,#188916,#188917,#188918,#188919,
#188920,#188921,#188922,#188923,#188924,#188925,#188926,#188927,#188928,
#188929,#188930,#188931,#188932,#188933,#188934,#188935,#188936,#188937,
#188938,#188939,#188940,#188941,#188942,#188943,#188944,#188945,#188946,
#188947,#188948,#188949,#188950,#188951,#188952,#188953,#188954,#188955,
#188956,#188957,#188958,#188959,#188960,#188961,#188962,#188963,#188964,
#188965,#188966,#188967,#188968,#188969,#188970,#188971,#188972,#188973,
#188974,#188975,#188976,#188977,#188978,#188979,#188980,#188981,#188982,
#188983,#188984,#188985,#188986,#188987,#188988,#188989,#188990,#188991,
#188992,#188993,#188994,#188995,#188996,#188997,#188998,#188999,#189000,
#189001,#189002,#189003,#189004,#189005,#189006,#189007,#189008,#189009,
#189010,#189011,#189012,#189013,#189014,#189015,#189016,#189017,#189018,
#189019,#189020,#189021,#189022,#189023,#189024,#189025,#189026,#189027,
#189028,#189029,#189030,#189031,#189032,#189033,#189034,#189035,#189036,
#189037,#189038,#189039,#189040,#189041,#189042,#189043,#189044,#189045,
#189046,#189047,#189048,#189049,#189050,#189051,#189052,#189053,#189054,
#189055,#189056,#189057,#189058,#189059,#189060,#189061,#189062,#189063,
#189064,#189065,#189066,#189067,#189068,#189069,#189070,#189071,#189072,
#189073,#189074,#189075,#189076,#189077,#189078,#189079,#189080,#189081,
#189082,#189083,#189084,#189085,#189086,#189087,#189088,#189089,#189090,
#189091,#189092,#189093,#189094,#189095,#189096,#189097,#189098,#189099,
#189100,#189101,#189102,#189103,#189104,#189105,#189106,#189107,#189108,
#189109,#189110,#189111,#189112,#189113,#189114),.UNSPECIFIED.,.F.,.F.,
(4,3,3,3,3,3,3,3,3,3,3,3,3,3,3,3,3,3,3,3,3,3,3,3,3,3,3,3,3,3,3,3,3,3,3,
3,3,3,3,3,3,3,3,3,3,3,3,3,3,3,3,3,3,3,3,3,3,3,3,3,3,3,3,3,3,3,3,3,3,3,3,
3,3,3,3,3,3,3,3,3,3,3,3,3,3,3,3,3,3,3,3,3,3,3,3,3,4),(0.143172102,0.15412844,
0.165137615,0.177981651,0.188990826,0.2,0.212844037,0.223853211,0.234862385,
0.24587156,0.256880734,0.267889908,0.278899083,0.289908257,0.300917431,
0.31559633,0.328440367,0.341284404,0.352293578,0.365137615,0.376146789,
0.39266055,0.403669725,0.416513761,0.427522936,0.43853211,0.449541284,0.460550459,
0.469724771,0.480733945,0.493577982,0.504587156,0.51559633,0.524770642,
0.533944954,0.541284404,0.550458716,0.557798165,0.565137615,0.572477064,
0.583486239,0.590825688,0.598165138,0.60733945,0.614678899,0.622018349,
0.629357798,0.640366972,0.651376147,0.660550459,0.667889908,0.67706422,
0.686238532,0.693577982,0.700917431,0.713761468,0.726605505,0.733944954,
0.743119266,0.750458716,0.757798165,0.765137615,0.772477064,0.779816514,
0.788990826,0.798165138,0.80733945,0.812844037,0.818348624,0.825688073,
0.831192661,0.83853211,0.84587156,0.851376147,0.858715596,0.864220183,0.871559633,
0.87706422,0.88440367,0.893577982,0.900917431,0.910091743,0.91559633,0.92293578,
0.928440367,0.935779817,0.941284404,0.948623853,0.95412844,0.96146789,0.966972477,
0.972477064,0.977981651,0.983486239,0.988990826,0.994495413,1.),
 .UNSPECIFIED.);
#24360=B_SPLINE_CURVE_WITH_KNOTS('',3,(#189115,#189116,#189117,#189118,
#189119,#189120,#189121,#189122,#189123,#189124,#189125,#189126,#189127,
#189128,#189129,#189130,#189131,#189132,#189133,#189134,#189135,#189136,
#189137,#189138,#189139,#189140,#189141,#189142,#189143,#189144,#189145,
#189146,#189147,#189148,#189149,#189150,#189151,#189152,#189153,#189154,
#189155,#189156,#189157,#189158,#189159,#189160,#189161,#189162,#189163,
#189164,#189165,#189166,#189167,#189168,#189169,#189170,#189171,#189172,
#189173,#189174,#189175,#189176,#189177,#189178,#189179,#189180,#189181,
#189182,#189183,#189184,#189185,#189186,#189187,#189188,#189189,#189190,
#189191,#189192,#189193,#189194,#189195,#189196,#189197,#189198,#189199,
#189200,#189201,#189202,#189203,#189204,#189205,#189206,#189207,#189208,
#189209,#189210,#189211,#189212,#189213,#189214,#189215,#189216,#189217,
#189218,#189219,#189220,#189221,#189222,#189223,#189224,#189225,#189226,
#189227,#189228,#189229,#189230,#189231,#189232,#189233,#189234,#189235,
#189236,#189237,#189238,#189239,#189240,#189241,#189242,#189243,#189244,
#189245,#189246,#189247,#189248,#189249,#189250,#189251,#189252,#189253,
#189254,#189255,#189256,#189257,#189258,#189259,#189260,#189261,#189262,
#189263,#189264,#189265,#189266,#189267,#189268,#189269,#189270,#189271,
#189272,#189273,#189274,#189275,#189276,#189277,#189278,#189279,#189280,
#189281,#189282,#189283,#189284,#189285,#189286,#189287,#189288,#189289,
#189290,#189291,#189292,#189293,#189294,#189295,#189296,#189297,#189298,
#189299,#189300,#189301,#189302,#189303,#189304,#189305,#189306,#189307,
#189308,#189309,#189310,#189311,#189312,#189313,#189314,#189315,#189316,
#189317,#189318,#189319,#189320,#189321,#189322,#189323,#189324,#189325,
#189326,#189327,#189328,#189329,#189330,#189331,#189332,#189333,#189334,
#189335,#189336,#189337,#189338,#189339,#189340,#189341,#189342,#189343,
#189344,#189345,#189346,#189347,#189348,#189349,#189350,#189351,#189352,
#189353,#189354,#189355,#189356,#189357,#189358,#189359,#189360,#189361,
#189362,#189363,#189364,#189365,#189366,#189367,#189368,#189369,#189370,
#189371,#189372,#189373,#189374,#189375,#189376,#189377,#189378,#189379,
#189380,#189381,#189382,#189383,#189384,#189385,#189386,#189387,#189388,
#189389,#189390,#189391,#189392,#189393,#189394,#189395,#189396,#189397,
#189398,#189399,#189400,#189401,#189402,#189403,#189404,#189405,#189406,
#189407,#189408,#189409,#189410,#189411,#189412,#189413,#189414,#189415,
#189416,#189417,#189418,#189419,#189420,#189421,#189422,#189423,#189424,
#189425,#189426,#189427,#189428,#189429,#189430,#189431,#189432,#189433),
 .UNSPECIFIED.,.F.,.F.,(4,3,3,3,3,3,3,3,3,3,3,3,3,3,3,3,3,3,3,3,3,3,3,3,
3,3,3,3,3,3,3,3,3,3,3,3,3,3,3,3,3,3,3,3,3,3,3,3,3,3,3,3,3,3,3,3,3,3,3,3,
3,3,3,3,3,3,3,3,3,3,3,3,3,3,3,3,3,3,3,3,3,3,3,3,3,3,3,3,3,3,3,3,3,3,3,3,
3,3,3,3,3,3,3,3,3,3,4),(0.143172102,0.15412844,0.165137615,0.176146789,
0.187155963,0.198165138,0.209174312,0.220183486,0.233027523,0.244036697,
0.262385321,0.275229358,0.288073394,0.300917431,0.311926606,0.32293578,
0.333944954,0.344954128,0.355963303,0.368807339,0.379816514,0.390825688,
0.401834862,0.411009174,0.420183486,0.429357798,0.43853211,0.449541284,
0.458715596,0.467889908,0.478899083,0.488073394,0.499082569,0.508256881,
0.517431193,0.526605505,0.533944954,0.541284404,0.548623853,0.555963303,
0.563302752,0.570642202,0.577981651,0.585321101,0.59266055,0.6,0.60733945,
0.614678899,0.622018349,0.629357798,0.636697248,0.644036697,0.651376147,
0.658715596,0.667889908,0.67706422,0.68440367,0.691743119,0.699082569,0.706422018,
0.713761468,0.721100917,0.728440367,0.735779817,0.743119266,0.750458716,
0.757798165,0.765137615,0.772477064,0.781651376,0.788990826,0.796330275,
0.805504587,0.811009174,0.816513761,0.822018349,0.827522936,0.833027523,
0.83853211,0.844036697,0.849541284,0.855045872,0.860550459,0.866055046,
0.871559633,0.87706422,0.882568807,0.888073394,0.893577982,0.900917431,
0.906422018,0.911926606,0.917431193,0.92293578,0.928440367,0.933944954,
0.939449541,0.944954128,0.950458716,0.957798165,0.963302752,0.968807339,
0.974311927,0.979816514,0.985321101,0.990825688,1.),.UNSPECIFIED.);
#24361=B_SPLINE_CURVE_WITH_KNOTS('',3,(#190381,#190382,#190383,#190384,
#190385,#190386,#190387,#190388,#190389,#190390,#190391,#190392,#190393,
#190394,#190395,#190396,#190397,#190398,#190399,#190400,#190401,#190402,
#190403,#190404,#190405,#190406,#190407,#190408,#190409,#190410,#190411,
#190412,#190413,#190414,#190415,#190416,#190417,#190418,#190419,#190420,
#190421,#190422,#190423,#190424,#190425,#190426,#190427,#190428,#190429,
#190430,#190431,#190432,#190433,#190434,#190435,#190436,#190437,#190438,
#190439,#190440,#190441,#190442,#190443,#190444,#190445,#190446,#190447,
#190448,#190449,#190450,#190451,#190452,#190453,#190454,#190455,#190456,
#190457,#190458,#190459,#190460,#190461,#190462,#190463,#190464,#190465,
#190466,#190467,#190468,#190469,#190470,#190471,#190472,#190473,#190474,
#190475,#190476,#190477,#190478,#190479,#190480,#190481,#190482,#190483,
#190484,#190485,#190486,#190487,#190488,#190489,#190490,#190491,#190492,
#190493,#190494,#190495,#190496,#190497,#190498,#190499,#190500,#190501,
#190502,#190503,#190504,#190505,#190506,#190507,#190508,#190509,#190510,
#190511,#190512,#190513,#190514,#190515,#190516,#190517,#190518,#190519,
#190520,#190521,#190522,#190523,#190524,#190525,#190526,#190527,#190528,
#190529,#190530,#190531,#190532,#190533,#190534,#190535,#190536,#190537,
#190538,#190539,#190540,#190541,#190542,#190543,#190544,#190545,#190546,
#190547,#190548,#190549,#190550,#190551,#190552,#190553,#190554,#190555,
#190556,#190557,#190558,#190559,#190560,#190561,#190562,#190563,#190564,
#190565,#190566,#190567,#190568,#190569,#190570,#190571,#190572,#190573,
#190574,#190575,#190576,#190577,#190578,#190579,#190580,#190581,#190582,
#190583,#190584,#190585,#190586,#190587,#190588,#190589,#190590,#190591,
#190592,#190593,#190594,#190595,#190596,#190597,#190598,#190599,#190600,
#190601,#190602,#190603,#190604,#190605,#190606,#190607,#190608,#190609,
#190610,#190611,#190612,#190613,#190614,#190615,#190616,#190617,#190618,
#190619,#190620,#190621,#190622,#190623,#190624,#190625,#190626,#190627,
#190628,#190629,#190630,#190631,#190632,#190633,#190634,#190635,#190636,
#190637,#190638,#190639,#190640,#190641,#190642,#190643,#190644,#190645,
#190646,#190647,#190648,#190649,#190650,#190651,#190652,#190653,#190654,
#190655,#190656,#190657,#190658,#190659,#190660,#190661,#190662,#190663,
#190664,#190665,#190666,#190667,#190668,#190669,#190670,#190671,#190672,
#190673,#190674,#190675,#190676,#190677,#190678,#190679,#190680,#190681,
#190682,#190683,#190684,#190685,#190686,#190687,#190688,#190689,#190690,
#190691,#190692,#190693,#190694,#190695,#190696,#190697,#190698,#190699,
#190700,#190701,#190702),.UNSPECIFIED.,.F.,.F.,(4,3,3,3,3,3,3,3,3,3,3,3,
3,3,3,3,3,3,3,3,3,3,3,3,3,3,3,3,3,3,3,3,3,3,3,3,3,3,3,3,3,3,3,3,3,3,3,3,
3,3,3,3,3,3,3,3,3,3,3,3,3,3,3,3,3,3,3,3,3,3,3,3,3,3,3,3,3,3,3,3,3,3,3,3,
3,3,3,3,3,3,3,3,3,3,3,3,3,3,3,3,3,3,3,3,3,3,3,4),(-1.,-0.994495413,-0.988990826,
-0.983486239,-0.977981651,-0.972477064,-0.966972477,-0.96146789,-0.955963303,
-0.950458716,-0.944954128,-0.939449541,-0.933944954,-0.928440367,-0.92293578,
-0.917431193,-0.911926606,-0.906422018,-0.900917431,-0.895412844,-0.889908257,
-0.88440367,-0.878899083,-0.873394495,-0.867889908,-0.862385321,-0.855045872,
-0.849541284,-0.842201835,-0.836697248,-0.831192661,-0.825688073,-0.820183486,
-0.814678899,-0.809174312,-0.801834862,-0.794495413,-0.787155963,-0.779816514,
-0.772477064,-0.765137615,-0.757798165,-0.750458716,-0.743119266,-0.735779817,
-0.728440367,-0.721100917,-0.713761468,-0.706422018,-0.697247706,-0.689908257,
-0.682568807,-0.675229358,-0.667889908,-0.660550459,-0.653211009,-0.644036697,
-0.636697248,-0.627522936,-0.620183486,-0.612844037,-0.605504587,-0.598165138,
-0.590825688,-0.583486239,-0.576146789,-0.568807339,-0.56146789,-0.55412844,
-0.546788991,-0.539449541,-0.532110092,-0.52293578,-0.513761468,-0.504587156,
-0.495412844,-0.486238532,-0.475229358,-0.466055046,-0.453211009,-0.444036697,
-0.434862385,-0.425688073,-0.416513761,-0.40733945,-0.398165138,-0.385321101,
-0.374311927,-0.363302752,-0.352293578,-0.341284404,-0.330275229,-0.319266055,
-0.308256881,-0.297247706,-0.286238532,-0.275229358,-0.264220183,-0.253211009,
-0.240366972,-0.229357798,-0.218348624,-0.20733945,-0.196330275,-0.185321101,
-0.172477064,-0.16146789,-0.143172102),.UNSPECIFIED.);
#24362=B_SPLINE_CURVE_WITH_KNOTS('',3,(#190703,#190704,#190705,#190706,
#190707,#190708,#190709,#190710,#190711,#190712,#190713,#190714,#190715,
#190716,#190717,#190718,#190719,#190720,#190721,#190722,#190723,#190724,
#190725,#190726,#190727,#190728,#190729,#190730,#190731,#190732,#190733,
#190734,#190735,#190736,#190737,#190738,#190739,#190740,#190741,#190742,
#190743,#190744,#190745,#190746,#190747,#190748,#190749,#190750,#190751,
#190752,#190753,#190754,#190755,#190756,#190757,#190758,#190759,#190760,
#190761,#190762,#190763,#190764,#190765,#190766,#190767,#190768,#190769,
#190770,#190771,#190772,#190773,#190774,#190775,#190776,#190777,#190778,
#190779,#190780,#190781,#190782,#190783,#190784,#190785,#190786,#190787,
#190788,#190789,#190790,#190791,#190792,#190793,#190794,#190795,#190796,
#190797,#190798,#190799,#190800,#190801,#190802,#190803,#190804,#190805,
#190806,#190807,#190808,#190809,#190810,#190811,#190812,#190813,#190814,
#190815,#190816,#190817,#190818,#190819,#190820,#190821,#190822,#190823,
#190824,#190825,#190826,#190827,#190828,#190829,#190830,#190831,#190832,
#190833,#190834,#190835,#190836,#190837,#190838,#190839,#190840,#190841,
#190842,#190843,#190844,#190845,#190846,#190847,#190848,#190849,#190850,
#190851,#190852,#190853,#190854,#190855,#190856,#190857,#190858,#190859,
#190860,#190861,#190862,#190863,#190864,#190865,#190866,#190867,#190868,
#190869,#190870,#190871,#190872,#190873,#190874,#190875,#190876,#190877,
#190878,#190879,#190880,#190881,#190882,#190883,#190884,#190885,#190886,
#190887,#190888,#190889,#190890,#190891,#190892,#190893,#190894,#190895,
#190896,#190897,#190898,#190899,#190900,#190901,#190902,#190903,#190904,
#190905,#190906,#190907,#190908,#190909,#190910,#190911,#190912,#190913,
#190914,#190915,#190916,#190917,#190918,#190919,#190920,#190921,#190922,
#190923,#190924,#190925,#190926,#190927,#190928,#190929,#190930,#190931,
#190932,#190933,#190934,#190935,#190936,#190937,#190938,#190939,#190940,
#190941,#190942,#190943,#190944,#190945,#190946,#190947,#190948,#190949,
#190950,#190951,#190952,#190953,#190954,#190955,#190956,#190957,#190958,
#190959,#190960,#190961,#190962,#190963,#190964,#190965,#190966,#190967,
#190968,#190969,#190970,#190971,#190972,#190973,#190974,#190975,#190976,
#190977,#190978,#190979,#190980,#190981,#190982,#190983,#190984,#190985,
#190986,#190987,#190988,#190989,#190990,#190991,#190992,#190993,#190994,
#190995,#190996,#190997,#190998,#190999,#191000),.UNSPECIFIED.,.F.,.F.,
(4,3,3,3,3,3,3,3,3,3,3,3,3,3,3,3,3,3,3,3,3,3,3,3,3,3,3,3,3,3,3,3,3,3,3,
3,3,3,3,3,3,3,3,3,3,3,3,3,3,3,3,3,3,3,3,3,3,3,3,3,3,3,3,3,3,3,3,3,3,3,3,
3,3,3,3,3,3,3,3,3,3,3,3,3,3,3,3,3,3,3,3,3,3,3,3,3,3,3,3,4),(0.143172102,
0.15412844,0.165137615,0.179816514,0.190825688,0.201834862,0.212844037,
0.223853211,0.234862385,0.24587156,0.256880734,0.267889908,0.278899083,
0.289908257,0.300917431,0.313761468,0.324770642,0.335779817,0.346788991,
0.363302752,0.374311927,0.385321101,0.396330275,0.405504587,0.416513761,
0.425688073,0.434862385,0.444036697,0.453211009,0.464220183,0.473394495,
0.482568807,0.491743119,0.500917431,0.510091743,0.521100917,0.530275229,
0.539449541,0.550458716,0.557798165,0.568807339,0.576146789,0.583486239,
0.59266055,0.6,0.60733945,0.614678899,0.622018349,0.631192661,0.640366972,
0.649541284,0.656880734,0.664220183,0.673394495,0.680733945,0.688073394,
0.695412844,0.702752294,0.710091743,0.717431193,0.730275229,0.743119266,
0.750458716,0.763302752,0.770642202,0.777981651,0.785321101,0.79266055,
0.8,0.811009174,0.816513761,0.822018349,0.827522936,0.833027523,0.83853211,
0.847706422,0.855045872,0.862385321,0.869724771,0.875229358,0.880733945,
0.886238532,0.893577982,0.899082569,0.904587156,0.910091743,0.917431193,
0.92293578,0.928440367,0.933944954,0.939449541,0.944954128,0.950458716,
0.957798165,0.966972477,0.972477064,0.977981651,0.983486239,0.99266055,
1.),.UNSPECIFIED.);
#24363=B_SPLINE_CURVE_WITH_KNOTS('',5,(#191963,#191964,#191965,#191966,
#191967,#191968,#191969,#191970,#191971,#191972,#191973,#191974,#191975,
#191976,#191977,#191978,#191979,#191980,#191981,#191982,#191983,#191984,
#191985,#191986,#191987,#191988,#191989,#191990,#191991,#191992,#191993,
#191994,#191995,#191996,#191997,#191998,#191999,#192000,#192001,#192002,
#192003,#192004,#192005,#192006,#192007,#192008,#192009,#192010,#192011,
#192012,#192013,#192014,#192015,#192016,#192017,#192018,#192019,#192020,
#192021,#192022,#192023,#192024,#192025,#192026,#192027,#192028,#192029,
#192030,#192031,#192032,#192033,#192034,#192035,#192036,#192037,#192038,
#192039,#192040,#192041,#192042,#192043,#192044,#192045,#192046,#192047,
#192048,#192049,#192050,#192051,#192052,#192053,#192054,#192055,#192056,
#192057,#192058,#192059,#192060,#192061,#192062,#192063,#192064,#192065,
#192066,#192067,#192068,#192069,#192070,#192071,#192072,#192073,#192074,
#192075,#192076,#192077,#192078,#192079,#192080,#192081,#192082,#192083,
#192084,#192085,#192086,#192087,#192088,#192089,#192090,#192091,#192092,
#192093,#192094,#192095,#192096,#192097,#192098,#192099,#192100,#192101,
#192102,#192103,#192104,#192105,#192106,#192107,#192108,#192109,#192110,
#192111,#192112,#192113,#192114,#192115,#192116,#192117,#192118,#192119,
#192120,#192121,#192122,#192123,#192124,#192125,#192126,#192127,#192128,
#192129,#192130,#192131,#192132,#192133,#192134,#192135,#192136,#192137,
#192138,#192139,#192140,#192141,#192142,#192143,#192144,#192145,#192146,
#192147,#192148,#192149,#192150,#192151,#192152,#192153,#192154,#192155,
#192156,#192157,#192158,#192159,#192160,#192161,#192162,#192163,#192164,
#192165,#192166,#192167,#192168,#192169,#192170,#192171,#192172,#192173,
#192174,#192175,#192176,#192177,#192178,#192179,#192180,#192181,#192182,
#192183,#192184,#192185,#192186,#192187,#192188,#192189,#192190,#192191,
#192192,#192193,#192194,#192195,#192196,#192197,#192198,#192199,#192200,
#192201,#192202,#192203,#192204,#192205,#192206,#192207,#192208,#192209,
#192210,#192211,#192212,#192213,#192214,#192215,#192216,#192217,#192218,
#192219,#192220,#192221,#192222,#192223,#192224,#192225,#192226,#192227,
#192228,#192229,#192230,#192231,#192232,#192233,#192234,#192235,#192236,
#192237,#192238,#192239,#192240,#192241,#192242,#192243,#192244,#192245,
#192246,#192247,#192248,#192249,#192250,#192251,#192252,#192253,#192254,
#192255,#192256,#192257,#192258,#192259,#192260,#192261,#192262,#192263,
#192264,#192265,#192266,#192267,#192268,#192269,#192270,#192271,#192272,
#192273,#192274,#192275,#192276,#192277,#192278,#192279,#192280,#192281,
#192282,#192283,#192284,#192285,#192286,#192287,#192288,#192289,#192290,
#192291,#192292,#192293,#192294,#192295,#192296,#192297,#192298,#192299,
#192300,#192301,#192302,#192303,#192304,#192305,#192306,#192307,#192308,
#192309,#192310,#192311,#192312,#192313,#192314,#192315,#192316,#192317,
#192318,#192319,#192320,#192321,#192322,#192323,#192324,#192325,#192326,
#192327,#192328,#192329,#192330,#192331,#192332,#192333,#192334,#192335,
#192336,#192337,#192338,#192339,#192340,#192341,#192342,#192343,#192344,
#192345,#192346,#192347,#192348,#192349,#192350,#192351,#192352,#192353,
#192354,#192355,#192356,#192357,#192358,#192359,#192360,#192361,#192362,
#192363,#192364,#192365,#192366,#192367,#192368,#192369,#192370,#192371,
#192372,#192373,#192374,#192375,#192376,#192377,#192378,#192379,#192380,
#192381,#192382,#192383,#192384,#192385,#192386,#192387,#192388,#192389,
#192390,#192391,#192392,#192393,#192394,#192395,#192396,#192397,#192398,
#192399,#192400,#192401,#192402,#192403,#192404,#192405,#192406,#192407,
#192408,#192409,#192410,#192411,#192412,#192413,#192414,#192415,#192416,
#192417,#192418,#192419,#192420,#192421,#192422,#192423,#192424,#192425,
#192426,#192427,#192428,#192429,#192430,#192431,#192432,#192433),
 .UNSPECIFIED.,.F.,.F.,(6,1,1,1,1,1,1,1,1,1,1,1,1,1,1,1,1,1,1,1,1,1,1,1,
1,1,1,1,1,1,1,1,1,1,1,1,1,1,1,1,1,1,1,1,1,1,1,1,1,1,1,1,1,1,1,1,1,1,1,1,
1,1,1,1,1,1,1,1,1,1,1,1,1,1,1,1,1,1,1,1,1,1,1,1,1,1,1,1,1,1,1,1,1,1,1,1,
1,1,1,1,1,1,1,1,1,1,1,1,1,1,1,1,1,1,1,1,1,1,1,1,1,1,1,1,1,1,1,1,1,1,1,1,
1,1,1,1,1,1,1,1,1,1,1,1,1,1,1,1,1,1,1,1,1,1,1,1,1,1,1,1,1,1,1,1,1,1,1,1,
1,1,1,1,1,1,1,1,1,1,1,1,1,1,1,1,1,1,1,1,1,1,1,1,1,1,1,1,1,1,1,1,1,1,1,1,
1,1,1,1,1,1,1,1,1,1,1,1,1,1,1,1,1,1,1,1,1,1,1,1,1,1,1,1,1,1,1,1,1,1,1,1,
1,1,1,1,1,1,1,1,1,1,1,1,1,1,1,1,1,1,1,1,1,1,1,1,1,1,1,1,1,1,1,1,1,1,1,1,
1,1,1,1,1,1,1,1,1,1,1,1,1,1,1,1,1,1,1,1,1,1,1,1,1,1,1,1,1,1,1,1,1,1,1,1,
1,1,1,1,1,1,1,1,1,1,1,1,1,1,1,1,1,1,1,1,1,1,1,1,1,1,1,1,1,1,1,1,1,1,1,1,
1,1,1,1,1,1,1,1,1,1,1,1,1,1,1,1,1,1,1,1,1,1,1,1,1,1,1,1,1,1,1,1,1,1,1,1,
1,1,1,1,1,1,1,1,1,1,1,1,1,1,1,1,1,1,1,1,1,1,1,1,1,1,1,1,1,1,1,1,1,1,1,1,
1,1,1,1,1,1,1,1,1,1,1,1,1,1,1,1,1,1,1,1,1,1,1,1,1,1,1,1,1,1,1,1,1,1,1,1,
1,1,1,1,1,1,1,1,1,1,6),(-1.,-0.998165138,-0.996330275,-0.994495413,-0.99266055,
-0.990825688,-0.988990826,-0.987155963,-0.985321101,-0.983486239,-0.981651376,
-0.979816514,-0.977981651,-0.976146789,-0.974311927,-0.972477064,-0.970642202,
-0.968807339,-0.966972477,-0.965137615,-0.963302752,-0.96146789,-0.959633028,
-0.957798165,-0.955963303,-0.95412844,-0.952293578,-0.950458716,-0.948623853,
-0.946788991,-0.944954128,-0.943119266,-0.941284404,-0.939449541,-0.937614679,
-0.935779817,-0.933944954,-0.932110092,-0.930275229,-0.928440367,-0.926605505,
-0.924770642,-0.92293578,-0.921100917,-0.919266055,-0.917431193,-0.91559633,
-0.913761468,-0.911926606,-0.910091743,-0.908256881,-0.906422018,-0.904587156,
-0.902752294,-0.900917431,-0.899082569,-0.897247706,-0.895412844,-0.893577982,
-0.891743119,-0.889908257,-0.888073394,-0.886238532,-0.88440367,-0.882568807,
-0.880733945,-0.878899083,-0.87706422,-0.875229358,-0.873394495,-0.871559633,
-0.869724771,-0.867889908,-0.866055046,-0.864220183,-0.862385321,-0.860550459,
-0.858715596,-0.856880734,-0.855045872,-0.853211009,-0.851376147,-0.849541284,
-0.847706422,-0.84587156,-0.844036697,-0.842201835,-0.840366972,-0.83853211,
-0.836697248,-0.834862385,-0.833027523,-0.831192661,-0.829357798,-0.827522936,
-0.825688073,-0.823853211,-0.822018349,-0.820183486,-0.818348624,-0.816513761,
-0.814678899,-0.812844037,-0.811009174,-0.809174312,-0.80733945,-0.805504587,
-0.803669725,-0.801834862,-0.8,-0.798165138,-0.796330275,-0.794495413,-0.79266055,
-0.790825688,-0.788990826,-0.787155963,-0.785321101,-0.783486239,-0.781651376,
-0.779816514,-0.777981651,-0.776146789,-0.774311927,-0.772477064,-0.770642202,
-0.768807339,-0.766972477,-0.765137615,-0.763302752,-0.76146789,-0.759633028,
-0.757798165,-0.755963303,-0.75412844,-0.752293578,-0.750458716,-0.748623853,
-0.746788991,-0.744954128,-0.743119266,-0.741284404,-0.739449541,-0.737614679,
-0.735779817,-0.733944954,-0.732110092,-0.730275229,-0.728440367,-0.726605505,
-0.724770642,-0.72293578,-0.721100917,-0.719266055,-0.717431193,-0.71559633,
-0.713761468,-0.711926606,-0.710091743,-0.708256881,-0.706422018,-0.704587156,
-0.702752294,-0.700917431,-0.699082569,-0.697247706,-0.695412844,-0.693577982,
-0.691743119,-0.689908257,-0.688073394,-0.686238532,-0.68440367,-0.682568807,
-0.680733945,-0.678899083,-0.67706422,-0.675229358,-0.673394495,-0.671559633,
-0.669724771,-0.667889908,-0.666055046,-0.664220183,-0.662385321,-0.660550459,
-0.658715596,-0.656880734,-0.655045872,-0.653211009,-0.651376147,-0.649541284,
-0.647706422,-0.64587156,-0.644036697,-0.642201835,-0.640366972,-0.63853211,
-0.636697248,-0.634862385,-0.633027523,-0.631192661,-0.629357798,-0.627522936,
-0.625688073,-0.623853211,-0.622018349,-0.620183486,-0.618348624,-0.616513761,
-0.614678899,-0.612844037,-0.611009174,-0.609174312,-0.60733945,-0.605504587,
-0.603669725,-0.601834862,-0.6,-0.598165138,-0.596330275,-0.594495413,-0.59266055,
-0.590825688,-0.588990826,-0.587155963,-0.585321101,-0.583486239,-0.581651376,
-0.579816514,-0.577981651,-0.576146789,-0.574311927,-0.572477064,-0.570642202,
-0.568807339,-0.566972477,-0.565137615,-0.563302752,-0.56146789,-0.559633028,
-0.557798165,-0.555963303,-0.55412844,-0.552293578,-0.550458716,-0.548623853,
-0.546788991,-0.544954128,-0.543119266,-0.541284404,-0.539449541,-0.537614679,
-0.535779817,-0.533944954,-0.532110092,-0.530275229,-0.528440367,-0.526605505,
-0.524770642,-0.52293578,-0.521100917,-0.519266055,-0.517431193,-0.51559633,
-0.513761468,-0.511926606,-0.510091743,-0.508256881,-0.506422018,-0.504587156,
-0.502752294,-0.500917431,-0.499082569,-0.497247706,-0.495412844,-0.493577982,
-0.491743119,-0.489908257,-0.488073394,-0.486238532,-0.48440367,-0.482568807,
-0.480733945,-0.478899083,-0.475229358,-0.473394495,-0.471559633,-0.469724771,
-0.467889908,-0.466055046,-0.464220183,-0.462385321,-0.460550459,-0.458715596,
-0.456880734,-0.455045872,-0.453211009,-0.451376147,-0.449541284,-0.447706422,
-0.44587156,-0.444036697,-0.442201835,-0.440366972,-0.43853211,-0.436697248,
-0.434862385,-0.433027523,-0.431192661,-0.429357798,-0.427522936,-0.425688073,
-0.423853211,-0.422018349,-0.420183486,-0.418348624,-0.416513761,-0.414678899,
-0.412844037,-0.411009174,-0.409174312,-0.40733945,-0.405504587,-0.403669725,
-0.401834862,-0.4,-0.398165138,-0.396330275,-0.394495413,-0.39266055,-0.390825688,
-0.388990826,-0.387155963,-0.385321101,-0.383486239,-0.381651376,-0.379816514,
-0.377981651,-0.376146789,-0.374311927,-0.372477064,-0.370642202,-0.368807339,
-0.366972477,-0.365137615,-0.363302752,-0.36146789,-0.359633028,-0.357798165,
-0.355963303,-0.35412844,-0.352293578,-0.350458716,-0.348623853,-0.346788991,
-0.344954128,-0.343119266,-0.341284404,-0.339449541,-0.337614679,-0.335779817,
-0.333944954,-0.332110092,-0.330275229,-0.328440367,-0.326605505,-0.324770642,
-0.32293578,-0.321100917,-0.319266055,-0.317431193,-0.31559633,-0.313761468,
-0.311926606,-0.310091743,-0.308256881,-0.306422018,-0.304587156,-0.302752294,
-0.300917431,-0.299082569,-0.297247706,-0.295412844,-0.293577982,-0.291743119,
-0.289908257,-0.288073394,-0.286238532,-0.28440367,-0.282568807,-0.280733945,
-0.278899083,-0.27706422,-0.275229358,-0.273394495,-0.271559633,-0.269724771,
-0.267889908,-0.266055046,-0.264220183,-0.262385321,-0.260550459,-0.258715596,
-0.256880734,-0.255045872,-0.253211009,-0.251376147,-0.249541284,-0.247706422,
-0.24587156,-0.244036697,-0.242201835,-0.240366972,-0.23853211,-0.236697248,
-0.234862385,-0.233027523,-0.231192661,-0.229357798,-0.227522936,-0.225688073,
-0.223853211,-0.222018349,-0.220183486,-0.218348624,-0.216513761,-0.214678899,
-0.212844037,-0.211009174,-0.209174312,-0.20733945,-0.205504587,-0.203669725,
-0.201834862,-0.2,-0.198165138,-0.196330275,-0.194495413,-0.19266055,-0.190825688,
-0.188990826,-0.187155963,-0.185321101,-0.183486239,-0.181651376,-0.179816514,
-0.177981651,-0.176146789,-0.174311927,-0.172477064,-0.170642202,-0.168807339,
-0.166972477,-0.165137615,-0.163302752,-0.16146789,-0.159633028,-0.157798165,
-0.155963303,-0.15412844,-0.152293578,-0.150458716,-0.148623853,-0.146788991,
-0.144954128,-0.143172102),.UNSPECIFIED.);
#24364=B_SPLINE_CURVE_WITH_KNOTS('',5,(#192434,#192435,#192436,#192437,
#192438,#192439,#192440,#192441,#192442,#192443,#192444,#192445,#192446,
#192447,#192448,#192449,#192450,#192451,#192452,#192453,#192454,#192455,
#192456,#192457,#192458,#192459,#192460,#192461,#192462,#192463,#192464,
#192465,#192466,#192467,#192468,#192469,#192470,#192471,#192472,#192473,
#192474,#192475,#192476,#192477,#192478,#192479,#192480,#192481,#192482,
#192483,#192484,#192485,#192486,#192487,#192488,#192489,#192490,#192491,
#192492,#192493,#192494,#192495,#192496,#192497,#192498,#192499,#192500,
#192501,#192502,#192503,#192504,#192505,#192506,#192507,#192508,#192509,
#192510,#192511,#192512,#192513,#192514,#192515,#192516,#192517,#192518,
#192519,#192520,#192521,#192522,#192523,#192524,#192525,#192526,#192527,
#192528,#192529,#192530,#192531,#192532,#192533,#192534,#192535,#192536,
#192537,#192538,#192539,#192540,#192541,#192542,#192543,#192544,#192545,
#192546,#192547,#192548,#192549,#192550,#192551,#192552,#192553,#192554,
#192555,#192556,#192557,#192558,#192559,#192560,#192561,#192562,#192563,
#192564,#192565,#192566,#192567,#192568,#192569,#192570,#192571,#192572,
#192573,#192574,#192575,#192576,#192577,#192578,#192579,#192580,#192581,
#192582,#192583,#192584,#192585,#192586,#192587,#192588,#192589,#192590,
#192591,#192592,#192593,#192594,#192595,#192596,#192597,#192598,#192599,
#192600,#192601,#192602,#192603,#192604,#192605,#192606,#192607,#192608,
#192609,#192610,#192611,#192612,#192613,#192614,#192615,#192616,#192617,
#192618,#192619,#192620,#192621,#192622,#192623,#192624,#192625,#192626,
#192627,#192628,#192629,#192630,#192631,#192632,#192633,#192634,#192635,
#192636,#192637,#192638,#192639,#192640,#192641,#192642,#192643,#192644,
#192645,#192646,#192647,#192648,#192649,#192650,#192651,#192652,#192653,
#192654,#192655,#192656,#192657,#192658,#192659,#192660,#192661,#192662,
#192663,#192664,#192665,#192666,#192667,#192668,#192669,#192670,#192671,
#192672,#192673,#192674,#192675,#192676,#192677,#192678,#192679,#192680,
#192681,#192682,#192683,#192684,#192685,#192686,#192687,#192688,#192689,
#192690,#192691,#192692,#192693,#192694,#192695,#192696,#192697,#192698,
#192699,#192700,#192701,#192702,#192703,#192704,#192705,#192706,#192707,
#192708,#192709,#192710,#192711,#192712,#192713,#192714,#192715,#192716,
#192717,#192718,#192719,#192720,#192721,#192722,#192723,#192724,#192725,
#192726,#192727,#192728,#192729,#192730,#192731,#192732,#192733,#192734,
#192735,#192736,#192737,#192738,#192739,#192740,#192741,#192742,#192743,
#192744,#192745,#192746,#192747,#192748,#192749,#192750,#192751,#192752,
#192753,#192754,#192755,#192756,#192757,#192758,#192759,#192760,#192761,
#192762,#192763,#192764,#192765,#192766,#192767,#192768,#192769,#192770,
#192771,#192772,#192773,#192774,#192775,#192776,#192777,#192778,#192779,
#192780,#192781,#192782,#192783,#192784,#192785,#192786,#192787,#192788,
#192789,#192790,#192791,#192792,#192793,#192794,#192795,#192796,#192797,
#192798,#192799,#192800,#192801,#192802,#192803,#192804,#192805,#192806,
#192807,#192808,#192809,#192810,#192811,#192812,#192813,#192814,#192815,
#192816,#192817,#192818,#192819,#192820,#192821,#192822,#192823,#192824,
#192825,#192826,#192827,#192828,#192829,#192830,#192831,#192832,#192833,
#192834,#192835,#192836,#192837,#192838,#192839,#192840,#192841,#192842,
#192843,#192844,#192845,#192846,#192847,#192848,#192849,#192850,#192851,
#192852,#192853,#192854,#192855,#192856,#192857,#192858,#192859,#192860,
#192861,#192862,#192863,#192864,#192865,#192866,#192867,#192868,#192869,
#192870,#192871,#192872,#192873,#192874,#192875,#192876,#192877,#192878,
#192879,#192880,#192881,#192882,#192883,#192884,#192885,#192886,#192887,
#192888,#192889,#192890,#192891,#192892,#192893,#192894,#192895,#192896,
#192897,#192898,#192899,#192900,#192901,#192902,#192903,#192904),
 .UNSPECIFIED.,.F.,.F.,(6,1,1,1,1,1,1,1,1,1,1,1,1,1,1,1,1,1,1,1,1,1,1,1,
1,1,1,1,1,1,1,1,1,1,1,1,1,1,1,1,1,1,1,1,1,1,1,1,1,1,1,1,1,1,1,1,1,1,1,1,
1,1,1,1,1,1,1,1,1,1,1,1,1,1,1,1,1,1,1,1,1,1,1,1,1,1,1,1,1,1,1,1,1,1,1,1,
1,1,1,1,1,1,1,1,1,1,1,1,1,1,1,1,1,1,1,1,1,1,1,1,1,1,1,1,1,1,1,1,1,1,1,1,
1,1,1,1,1,1,1,1,1,1,1,1,1,1,1,1,1,1,1,1,1,1,1,1,1,1,1,1,1,1,1,1,1,1,1,1,
1,1,1,1,1,1,1,1,1,1,1,1,1,1,1,1,1,1,1,1,1,1,1,1,1,1,1,1,1,1,1,1,1,1,1,1,
1,1,1,1,1,1,1,1,1,1,1,1,1,1,1,1,1,1,1,1,1,1,1,1,1,1,1,1,1,1,1,1,1,1,1,1,
1,1,1,1,1,1,1,1,1,1,1,1,1,1,1,1,1,1,1,1,1,1,1,1,1,1,1,1,1,1,1,1,1,1,1,1,
1,1,1,1,1,1,1,1,1,1,1,1,1,1,1,1,1,1,1,1,1,1,1,1,1,1,1,1,1,1,1,1,1,1,1,1,
1,1,1,1,1,1,1,1,1,1,1,1,1,1,1,1,1,1,1,1,1,1,1,1,1,1,1,1,1,1,1,1,1,1,1,1,
1,1,1,1,1,1,1,1,1,1,1,1,1,1,1,1,1,1,1,1,1,1,1,1,1,1,1,1,1,1,1,1,1,1,1,1,
1,1,1,1,1,1,1,1,1,1,1,1,1,1,1,1,1,1,1,1,1,1,1,1,1,1,1,1,1,1,1,1,1,1,1,1,
1,1,1,1,1,1,1,1,1,1,1,1,1,1,1,1,1,1,1,1,1,1,1,1,1,1,1,1,1,1,1,1,1,1,1,1,
1,1,1,1,1,1,1,1,1,1,6),(0.143172102,0.144954128,0.146788991,0.148623853,
0.150458716,0.152293578,0.15412844,0.155963303,0.157798165,0.159633028,
0.16146789,0.163302752,0.165137615,0.166972477,0.168807339,0.170642202,
0.172477064,0.174311927,0.176146789,0.177981651,0.179816514,0.181651376,
0.183486239,0.185321101,0.187155963,0.188990826,0.190825688,0.19266055,
0.194495413,0.196330275,0.198165138,0.2,0.201834862,0.203669725,0.205504587,
0.20733945,0.209174312,0.211009174,0.212844037,0.214678899,0.216513761,
0.218348624,0.220183486,0.222018349,0.223853211,0.225688073,0.227522936,
0.229357798,0.231192661,0.233027523,0.234862385,0.236697248,0.23853211,
0.240366972,0.242201835,0.244036697,0.24587156,0.247706422,0.249541284,
0.251376147,0.253211009,0.255045872,0.256880734,0.258715596,0.260550459,
0.262385321,0.264220183,0.266055046,0.267889908,0.269724771,0.271559633,
0.273394495,0.275229358,0.27706422,0.278899083,0.280733945,0.282568807,
0.28440367,0.286238532,0.288073394,0.289908257,0.291743119,0.293577982,
0.295412844,0.297247706,0.299082569,0.300917431,0.302752294,0.304587156,
0.306422018,0.308256881,0.310091743,0.311926606,0.313761468,0.31559633,
0.317431193,0.319266055,0.321100917,0.32293578,0.324770642,0.326605505,
0.328440367,0.330275229,0.332110092,0.333944954,0.335779817,0.337614679,
0.339449541,0.341284404,0.343119266,0.344954128,0.346788991,0.348623853,
0.350458716,0.352293578,0.35412844,0.355963303,0.357798165,0.359633028,
0.36146789,0.363302752,0.365137615,0.366972477,0.368807339,0.370642202,
0.372477064,0.374311927,0.376146789,0.377981651,0.379816514,0.381651376,
0.383486239,0.385321101,0.387155963,0.388990826,0.390825688,0.39266055,
0.394495413,0.396330275,0.398165138,0.4,0.401834862,0.403669725,0.405504587,
0.40733945,0.409174312,0.411009174,0.412844037,0.414678899,0.416513761,
0.418348624,0.420183486,0.422018349,0.423853211,0.425688073,0.427522936,
0.429357798,0.431192661,0.433027523,0.434862385,0.436697248,0.43853211,
0.440366972,0.442201835,0.444036697,0.44587156,0.447706422,0.449541284,
0.451376147,0.453211009,0.455045872,0.456880734,0.458715596,0.460550459,
0.462385321,0.464220183,0.466055046,0.467889908,0.469724771,0.471559633,
0.473394495,0.475229358,0.478899083,0.480733945,0.482568807,0.48440367,
0.486238532,0.488073394,0.489908257,0.491743119,0.493577982,0.495412844,
0.497247706,0.499082569,0.500917431,0.502752294,0.504587156,0.506422018,
0.508256881,0.510091743,0.511926606,0.513761468,0.51559633,0.517431193,
0.519266055,0.521100917,0.52293578,0.524770642,0.526605505,0.528440367,
0.530275229,0.532110092,0.533944954,0.535779817,0.537614679,0.539449541,
0.541284404,0.543119266,0.544954128,0.546788991,0.548623853,0.550458716,
0.552293578,0.55412844,0.555963303,0.557798165,0.559633028,0.56146789,0.563302752,
0.565137615,0.566972477,0.568807339,0.570642202,0.572477064,0.574311927,
0.576146789,0.577981651,0.579816514,0.581651376,0.583486239,0.585321101,
0.587155963,0.588990826,0.590825688,0.59266055,0.594495413,0.596330275,
0.598165138,0.6,0.601834862,0.603669725,0.605504587,0.60733945,0.609174312,
0.611009174,0.612844037,0.614678899,0.616513761,0.618348624,0.620183486,
0.622018349,0.623853211,0.625688073,0.627522936,0.629357798,0.631192661,
0.633027523,0.634862385,0.636697248,0.63853211,0.640366972,0.642201835,
0.644036697,0.64587156,0.647706422,0.649541284,0.651376147,0.653211009,
0.655045872,0.656880734,0.658715596,0.660550459,0.662385321,0.664220183,
0.666055046,0.667889908,0.669724771,0.671559633,0.673394495,0.675229358,
0.67706422,0.678899083,0.680733945,0.682568807,0.68440367,0.686238532,0.688073394,
0.689908257,0.691743119,0.693577982,0.695412844,0.697247706,0.699082569,
0.700917431,0.702752294,0.704587156,0.706422018,0.708256881,0.710091743,
0.711926606,0.713761468,0.71559633,0.717431193,0.719266055,0.721100917,
0.72293578,0.724770642,0.726605505,0.728440367,0.730275229,0.732110092,
0.733944954,0.735779817,0.737614679,0.739449541,0.741284404,0.743119266,
0.744954128,0.746788991,0.748623853,0.750458716,0.752293578,0.75412844,
0.755963303,0.757798165,0.759633028,0.76146789,0.763302752,0.765137615,
0.766972477,0.768807339,0.770642202,0.772477064,0.774311927,0.776146789,
0.777981651,0.779816514,0.781651376,0.783486239,0.785321101,0.787155963,
0.788990826,0.790825688,0.79266055,0.794495413,0.796330275,0.798165138,
0.8,0.801834862,0.803669725,0.805504587,0.80733945,0.809174312,0.811009174,
0.812844037,0.814678899,0.816513761,0.818348624,0.820183486,0.822018349,
0.823853211,0.825688073,0.827522936,0.829357798,0.831192661,0.833027523,
0.834862385,0.836697248,0.83853211,0.840366972,0.842201835,0.844036697,
0.84587156,0.847706422,0.849541284,0.851376147,0.853211009,0.855045872,
0.856880734,0.858715596,0.860550459,0.862385321,0.864220183,0.866055046,
0.867889908,0.869724771,0.871559633,0.873394495,0.875229358,0.87706422,
0.878899083,0.880733945,0.882568807,0.88440367,0.886238532,0.888073394,
0.889908257,0.891743119,0.893577982,0.895412844,0.897247706,0.899082569,
0.900917431,0.902752294,0.904587156,0.906422018,0.908256881,0.910091743,
0.911926606,0.913761468,0.91559633,0.917431193,0.919266055,0.921100917,
0.92293578,0.924770642,0.926605505,0.928440367,0.930275229,0.932110092,
0.933944954,0.935779817,0.937614679,0.939449541,0.941284404,0.943119266,
0.944954128,0.946788991,0.948623853,0.950458716,0.952293578,0.95412844,
0.955963303,0.957798165,0.959633028,0.96146789,0.963302752,0.965137615,
0.966972477,0.968807339,0.970642202,0.972477064,0.974311927,0.976146789,
0.977981651,0.979816514,0.981651376,0.983486239,0.985321101,0.987155963,
0.988990826,0.990825688,0.99266055,0.994495413,0.996330275,0.998165138,
1.),.UNSPECIFIED.);
#24365=B_SPLINE_CURVE_WITH_KNOTS('',3,(#193849,#193850,#193851,#193852,
#193853,#193854,#193855,#193856,#193857,#193858,#193859,#193860,#193861,
#193862,#193863,#193864,#193865,#193866,#193867,#193868,#193869,#193870,
#193871,#193872,#193873,#193874,#193875,#193876,#193877,#193878,#193879,
#193880,#193881,#193882,#193883,#193884,#193885,#193886,#193887,#193888,
#193889,#193890,#193891,#193892,#193893,#193894,#193895,#193896,#193897,
#193898,#193899,#193900,#193901,#193902,#193903,#193904,#193905,#193906,
#193907,#193908,#193909,#193910,#193911,#193912,#193913,#193914,#193915,
#193916,#193917,#193918,#193919,#193920,#193921,#193922,#193923,#193924,
#193925,#193926,#193927,#193928,#193929,#193930,#193931,#193932,#193933,
#193934,#193935,#193936,#193937,#193938,#193939,#193940,#193941,#193942,
#193943,#193944,#193945,#193946,#193947,#193948,#193949,#193950,#193951,
#193952,#193953,#193954,#193955,#193956,#193957,#193958,#193959,#193960,
#193961,#193962,#193963,#193964,#193965,#193966,#193967,#193968,#193969,
#193970,#193971,#193972,#193973,#193974,#193975,#193976,#193977,#193978,
#193979,#193980,#193981,#193982,#193983,#193984,#193985,#193986,#193987,
#193988,#193989,#193990,#193991,#193992,#193993,#193994,#193995,#193996,
#193997,#193998,#193999,#194000,#194001,#194002,#194003,#194004,#194005,
#194006,#194007,#194008,#194009,#194010,#194011,#194012,#194013,#194014,
#194015,#194016,#194017,#194018,#194019,#194020,#194021,#194022,#194023,
#194024,#194025,#194026,#194027,#194028,#194029,#194030,#194031,#194032,
#194033,#194034,#194035,#194036,#194037,#194038,#194039,#194040,#194041,
#194042,#194043,#194044,#194045,#194046,#194047,#194048,#194049,#194050,
#194051,#194052,#194053,#194054,#194055,#194056,#194057,#194058,#194059,
#194060,#194061,#194062,#194063,#194064,#194065,#194066,#194067,#194068,
#194069,#194070,#194071,#194072,#194073,#194074,#194075,#194076,#194077,
#194078,#194079,#194080,#194081,#194082,#194083,#194084,#194085,#194086,
#194087,#194088,#194089,#194090,#194091,#194092,#194093,#194094,#194095,
#194096,#194097,#194098,#194099,#194100,#194101,#194102,#194103,#194104,
#194105,#194106,#194107,#194108,#194109,#194110,#194111,#194112,#194113,
#194114,#194115,#194116,#194117,#194118,#194119,#194120,#194121,#194122,
#194123,#194124,#194125,#194126,#194127,#194128,#194129,#194130,#194131,
#194132,#194133,#194134,#194135,#194136,#194137,#194138,#194139,#194140,
#194141,#194142,#194143,#194144,#194145,#194146),.UNSPECIFIED.,.F.,.F.,
(4,3,3,3,3,3,3,3,3,3,3,3,3,3,3,3,3,3,3,3,3,3,3,3,3,3,3,3,3,3,3,3,3,3,3,
3,3,3,3,3,3,3,3,3,3,3,3,3,3,3,3,3,3,3,3,3,3,3,3,3,3,3,3,3,3,3,3,3,3,3,3,
3,3,3,3,3,3,3,3,3,3,3,3,3,3,3,3,3,3,3,3,3,3,3,3,3,3,3,3,4),(0.143172102,
0.15412844,0.165137615,0.177981651,0.188990826,0.201834862,0.212844037,
0.223853211,0.234862385,0.24587156,0.256880734,0.267889908,0.278899083,
0.289908257,0.300917431,0.311926606,0.32293578,0.339449541,0.350458716,
0.36146789,0.374311927,0.385321101,0.396330275,0.40733945,0.416513761,0.425688073,
0.434862385,0.44587156,0.458715596,0.467889908,0.47706422,0.491743119,0.500917431,
0.511926606,0.521100917,0.530275229,0.537614679,0.548623853,0.555963303,
0.563302752,0.570642202,0.577981651,0.585321101,0.594495413,0.601834862,
0.609174312,0.616513761,0.623853211,0.631192661,0.640366972,0.647706422,
0.655045872,0.664220183,0.671559633,0.678899083,0.688073394,0.695412844,
0.702752294,0.711926606,0.719266055,0.726605505,0.735779817,0.744954128,
0.75412844,0.76146789,0.768807339,0.776146789,0.785321101,0.796330275,0.803669725,
0.812844037,0.820183486,0.827522936,0.836697248,0.842201835,0.849541284,
0.856880734,0.862385321,0.867889908,0.875229358,0.880733945,0.888073394,
0.893577982,0.899082569,0.906422018,0.911926606,0.917431193,0.92293578,
0.930275229,0.935779817,0.944954128,0.950458716,0.959633028,0.965137615,
0.970642202,0.976146789,0.981651376,0.987155963,0.99266055,1.),
 .UNSPECIFIED.);
#24366=B_SPLINE_CURVE_WITH_KNOTS('',3,(#194147,#194148,#194149,#194150,
#194151,#194152,#194153,#194154,#194155,#194156,#194157,#194158,#194159,
#194160,#194161,#194162,#194163,#194164,#194165,#194166,#194167,#194168,
#194169,#194170,#194171,#194172,#194173,#194174,#194175,#194176,#194177,
#194178,#194179,#194180,#194181,#194182,#194183,#194184,#194185,#194186,
#194187,#194188,#194189,#194190,#194191,#194192,#194193,#194194,#194195,
#194196,#194197,#194198,#194199,#194200,#194201,#194202,#194203,#194204,
#194205,#194206,#194207,#194208,#194209,#194210,#194211,#194212,#194213,
#194214,#194215,#194216,#194217,#194218,#194219,#194220,#194221,#194222,
#194223,#194224,#194225,#194226,#194227,#194228,#194229,#194230,#194231,
#194232,#194233,#194234,#194235,#194236,#194237,#194238,#194239,#194240,
#194241,#194242,#194243,#194244,#194245,#194246,#194247,#194248,#194249,
#194250,#194251,#194252,#194253,#194254,#194255,#194256,#194257,#194258,
#194259,#194260,#194261,#194262,#194263,#194264,#194265,#194266,#194267,
#194268,#194269,#194270,#194271,#194272,#194273,#194274,#194275,#194276,
#194277,#194278,#194279,#194280,#194281,#194282,#194283,#194284,#194285,
#194286,#194287,#194288,#194289,#194290,#194291,#194292,#194293,#194294,
#194295,#194296,#194297,#194298,#194299,#194300,#194301,#194302,#194303,
#194304,#194305,#194306,#194307,#194308,#194309,#194310,#194311,#194312,
#194313,#194314,#194315,#194316,#194317,#194318,#194319,#194320,#194321,
#194322,#194323,#194324,#194325,#194326,#194327,#194328,#194329,#194330,
#194331,#194332,#194333,#194334,#194335,#194336,#194337,#194338,#194339,
#194340,#194341,#194342,#194343,#194344,#194345,#194346,#194347,#194348,
#194349,#194350,#194351,#194352,#194353,#194354,#194355,#194356,#194357,
#194358,#194359,#194360,#194361,#194362,#194363,#194364,#194365,#194366,
#194367,#194368,#194369,#194370,#194371,#194372,#194373,#194374,#194375,
#194376,#194377,#194378,#194379,#194380,#194381,#194382,#194383,#194384,
#194385,#194386,#194387,#194388,#194389,#194390,#194391,#194392,#194393,
#194394,#194395,#194396,#194397,#194398,#194399,#194400,#194401,#194402,
#194403,#194404,#194405,#194406,#194407,#194408,#194409,#194410,#194411,
#194412,#194413,#194414,#194415,#194416,#194417,#194418,#194419,#194420,
#194421,#194422,#194423,#194424,#194425,#194426,#194427,#194428,#194429,
#194430,#194431,#194432,#194433,#194434,#194435,#194436,#194437,#194438,
#194439,#194440,#194441,#194442,#194443,#194444,#194445,#194446,#194447,
#194448,#194449,#194450,#194451,#194452,#194453,#194454,#194455,#194456,
#194457,#194458,#194459,#194460,#194461,#194462,#194463,#194464,#194465,
#194466,#194467,#194468),.UNSPECIFIED.,.F.,.F.,(4,3,3,3,3,3,3,3,3,3,3,3,
3,3,3,3,3,3,3,3,3,3,3,3,3,3,3,3,3,3,3,3,3,3,3,3,3,3,3,3,3,3,3,3,3,3,3,3,
3,3,3,3,3,3,3,3,3,3,3,3,3,3,3,3,3,3,3,3,3,3,3,3,3,3,3,3,3,3,3,3,3,3,3,3,
3,3,3,3,3,3,3,3,3,3,3,3,3,3,3,3,3,3,3,3,3,3,3,4),(0.143172102,0.15412844,
0.165137615,0.177981651,0.188990826,0.201834862,0.212844037,0.223853211,
0.234862385,0.247706422,0.258715596,0.269724771,0.280733945,0.291743119,
0.302752294,0.313761468,0.324770642,0.335779817,0.346788991,0.357798165,
0.368807339,0.379816514,0.39266055,0.401834862,0.411009174,0.420183486,
0.429357798,0.43853211,0.447706422,0.456880734,0.466055046,0.47706422,0.489908257,
0.499082569,0.508256881,0.517431193,0.526605505,0.533944954,0.541284404,
0.548623853,0.555963303,0.563302752,0.570642202,0.577981651,0.585321101,
0.59266055,0.6,0.60733945,0.614678899,0.622018349,0.629357798,0.636697248,
0.644036697,0.651376147,0.658715596,0.667889908,0.675229358,0.682568807,
0.689908257,0.697247706,0.704587156,0.711926606,0.719266055,0.726605505,
0.735779817,0.743119266,0.750458716,0.757798165,0.765137615,0.772477064,
0.779816514,0.787155963,0.794495413,0.801834862,0.809174312,0.814678899,
0.820183486,0.825688073,0.831192661,0.836697248,0.842201835,0.849541284,
0.855045872,0.860550459,0.866055046,0.871559633,0.87706422,0.882568807,
0.888073394,0.893577982,0.900917431,0.906422018,0.911926606,0.917431193,
0.92293578,0.928440367,0.933944954,0.939449541,0.944954128,0.950458716,
0.957798165,0.963302752,0.968807339,0.976146789,0.981651376,0.987155963,
0.99266055,1.),.UNSPECIFIED.);
#24367=B_SPLINE_CURVE_WITH_KNOTS('',3,(#195428,#195429,#195430,#195431,
#195432,#195433,#195434,#195435,#195436,#195437,#195438,#195439,#195440,
#195441,#195442,#195443,#195444,#195445,#195446,#195447,#195448,#195449,
#195450,#195451,#195452,#195453,#195454,#195455,#195456,#195457,#195458,
#195459,#195460,#195461,#195462,#195463,#195464,#195465,#195466,#195467,
#195468,#195469,#195470,#195471,#195472,#195473,#195474,#195475,#195476,
#195477,#195478,#195479,#195480,#195481,#195482,#195483,#195484,#195485,
#195486,#195487,#195488,#195489,#195490,#195491,#195492,#195493,#195494,
#195495,#195496,#195497,#195498,#195499,#195500,#195501,#195502,#195503,
#195504,#195505,#195506,#195507,#195508,#195509,#195510,#195511,#195512,
#195513,#195514,#195515,#195516,#195517,#195518,#195519,#195520,#195521,
#195522,#195523,#195524,#195525,#195526,#195527,#195528,#195529,#195530,
#195531,#195532,#195533,#195534,#195535,#195536,#195537,#195538,#195539,
#195540,#195541,#195542,#195543,#195544,#195545,#195546,#195547,#195548,
#195549,#195550,#195551,#195552,#195553,#195554,#195555,#195556,#195557,
#195558,#195559,#195560,#195561,#195562,#195563,#195564,#195565,#195566,
#195567,#195568,#195569,#195570,#195571,#195572,#195573,#195574,#195575,
#195576,#195577,#195578,#195579,#195580,#195581,#195582,#195583,#195584,
#195585,#195586,#195587,#195588,#195589,#195590,#195591,#195592,#195593,
#195594,#195595,#195596,#195597,#195598,#195599,#195600,#195601,#195602,
#195603,#195604,#195605,#195606,#195607,#195608,#195609,#195610,#195611,
#195612,#195613,#195614,#195615,#195616,#195617,#195618,#195619,#195620,
#195621,#195622,#195623,#195624,#195625,#195626,#195627,#195628,#195629,
#195630,#195631,#195632,#195633,#195634,#195635,#195636,#195637,#195638,
#195639,#195640,#195641,#195642,#195643,#195644,#195645,#195646,#195647,
#195648,#195649,#195650,#195651,#195652,#195653,#195654,#195655,#195656,
#195657,#195658,#195659,#195660,#195661,#195662,#195663,#195664,#195665,
#195666,#195667,#195668,#195669,#195670,#195671,#195672,#195673,#195674,
#195675,#195676,#195677,#195678,#195679,#195680,#195681,#195682,#195683,
#195684,#195685,#195686,#195687,#195688,#195689,#195690,#195691,#195692,
#195693,#195694,#195695,#195696,#195697,#195698,#195699,#195700,#195701,
#195702,#195703,#195704,#195705,#195706,#195707,#195708,#195709,#195710,
#195711,#195712,#195713,#195714,#195715,#195716,#195717,#195718,#195719,
#195720,#195721,#195722,#195723,#195724,#195725,#195726,#195727,#195728,
#195729,#195730,#195731,#195732,#195733,#195734),.UNSPECIFIED.,.F.,.F.,
(4,3,3,3,3,3,3,3,3,3,3,3,3,3,3,3,3,3,3,3,3,3,3,3,3,3,3,3,3,3,3,3,3,3,3,
3,3,3,3,3,3,3,3,3,3,3,3,3,3,3,3,3,3,3,3,3,3,3,3,3,3,3,3,3,3,3,3,3,3,3,3,
3,3,3,3,3,3,3,3,3,3,3,3,3,3,3,3,3,3,3,3,3,3,3,3,3,3,3,3,3,3,3,4),(0.143172102,
0.15412844,0.165137615,0.176146789,0.187155963,0.198165138,0.211009174,
0.222018349,0.233027523,0.244036697,0.255045872,0.266055046,0.27706422,
0.288073394,0.299082569,0.310091743,0.321100917,0.332110092,0.343119266,
0.35412844,0.365137615,0.376146789,0.387155963,0.398165138,0.40733945,0.416513761,
0.425688073,0.434862385,0.444036697,0.453211009,0.466055046,0.47706422,
0.486238532,0.497247706,0.506422018,0.51559633,0.524770642,0.533944954,
0.541284404,0.550458716,0.557798165,0.565137615,0.572477064,0.583486239,
0.59266055,0.6,0.60733945,0.616513761,0.623853211,0.631192661,0.640366972,
0.647706422,0.655045872,0.664220183,0.671559633,0.678899083,0.686238532,
0.693577982,0.702752294,0.713761468,0.721100917,0.728440367,0.735779817,
0.744954128,0.752293578,0.759633028,0.770642202,0.777981651,0.788990826,
0.796330275,0.803669725,0.812844037,0.822018349,0.829357798,0.834862385,
0.840366972,0.84587156,0.853211009,0.858715596,0.864220183,0.871559633,
0.87706422,0.882568807,0.888073394,0.893577982,0.902752294,0.908256881,
0.913761468,0.919266055,0.924770642,0.930275229,0.937614679,0.943119266,
0.948623853,0.95412844,0.96146789,0.966972477,0.972477064,0.977981651,0.983486239,
0.988990826,0.994495413,1.),.UNSPECIFIED.);
#24368=B_SPLINE_CURVE_WITH_KNOTS('',3,(#195735,#195736,#195737,#195738,
#195739,#195740,#195741,#195742,#195743,#195744,#195745,#195746,#195747,
#195748,#195749,#195750,#195751,#195752,#195753,#195754,#195755,#195756,
#195757,#195758,#195759,#195760,#195761,#195762,#195763,#195764,#195765,
#195766,#195767,#195768,#195769,#195770,#195771,#195772,#195773,#195774,
#195775,#195776,#195777,#195778,#195779,#195780,#195781,#195782,#195783,
#195784,#195785,#195786,#195787,#195788,#195789,#195790,#195791,#195792,
#195793,#195794,#195795,#195796,#195797,#195798,#195799,#195800,#195801,
#195802,#195803,#195804,#195805,#195806,#195807,#195808,#195809,#195810,
#195811,#195812,#195813,#195814,#195815,#195816,#195817,#195818,#195819,
#195820,#195821,#195822,#195823,#195824,#195825,#195826,#195827,#195828,
#195829,#195830,#195831,#195832,#195833,#195834,#195835,#195836,#195837,
#195838,#195839,#195840,#195841,#195842,#195843,#195844,#195845,#195846,
#195847,#195848,#195849,#195850,#195851,#195852,#195853,#195854,#195855,
#195856,#195857,#195858,#195859,#195860,#195861,#195862,#195863,#195864,
#195865,#195866,#195867,#195868,#195869,#195870,#195871,#195872,#195873,
#195874,#195875,#195876,#195877,#195878,#195879,#195880,#195881,#195882,
#195883,#195884,#195885,#195886,#195887,#195888,#195889,#195890,#195891,
#195892,#195893,#195894,#195895,#195896,#195897,#195898,#195899,#195900,
#195901,#195902,#195903,#195904,#195905,#195906,#195907,#195908,#195909,
#195910,#195911,#195912,#195913,#195914,#195915,#195916,#195917,#195918,
#195919,#195920,#195921,#195922,#195923,#195924,#195925,#195926,#195927,
#195928,#195929,#195930,#195931,#195932,#195933,#195934,#195935,#195936,
#195937,#195938,#195939,#195940,#195941,#195942,#195943,#195944,#195945,
#195946,#195947,#195948,#195949,#195950,#195951,#195952,#195953,#195954,
#195955,#195956,#195957,#195958,#195959,#195960,#195961,#195962,#195963,
#195964,#195965,#195966,#195967,#195968,#195969,#195970,#195971,#195972,
#195973,#195974,#195975,#195976,#195977,#195978,#195979,#195980,#195981,
#195982,#195983,#195984,#195985,#195986,#195987,#195988,#195989,#195990,
#195991,#195992,#195993,#195994,#195995,#195996,#195997,#195998,#195999,
#196000,#196001,#196002,#196003,#196004,#196005,#196006,#196007,#196008,
#196009,#196010,#196011,#196012,#196013,#196014,#196015,#196016,#196017,
#196018,#196019,#196020,#196021,#196022,#196023,#196024,#196025,#196026,
#196027,#196028,#196029,#196030,#196031,#196032,#196033,#196034,#196035,
#196036,#196037,#196038,#196039,#196040,#196041,#196042,#196043,#196044,
#196045,#196046,#196047,#196048,#196049,#196050,#196051,#196052,#196053),
 .UNSPECIFIED.,.F.,.F.,(4,3,3,3,3,3,3,3,3,3,3,3,3,3,3,3,3,3,3,3,3,3,3,3,
3,3,3,3,3,3,3,3,3,3,3,3,3,3,3,3,3,3,3,3,3,3,3,3,3,3,3,3,3,3,3,3,3,3,3,3,
3,3,3,3,3,3,3,3,3,3,3,3,3,3,3,3,3,3,3,3,3,3,3,3,3,3,3,3,3,3,3,3,3,3,3,3,
3,3,3,3,3,3,3,3,3,3,4),(0.143172102,0.15412844,0.165137615,0.176146789,
0.187155963,0.198165138,0.211009174,0.222018349,0.233027523,0.244036697,
0.255045872,0.266055046,0.27706422,0.289908257,0.300917431,0.311926606,
0.32293578,0.333944954,0.344954128,0.355963303,0.366972477,0.377981651,
0.388990826,0.398165138,0.40733945,0.416513761,0.425688073,0.434862385,
0.444036697,0.453211009,0.464220183,0.473394495,0.482568807,0.491743119,
0.500917431,0.510091743,0.519266055,0.528440367,0.535779817,0.544954128,
0.552293578,0.56146789,0.568807339,0.576146789,0.583486239,0.59266055,0.6,
0.60733945,0.614678899,0.622018349,0.629357798,0.636697248,0.644036697,
0.651376147,0.658715596,0.669724771,0.67706422,0.68440367,0.691743119,0.700917431,
0.708256881,0.71559633,0.72293578,0.730275229,0.737614679,0.744954128,0.752293578,
0.759633028,0.770642202,0.777981651,0.785321101,0.79266055,0.8,0.80733945,
0.812844037,0.820183486,0.825688073,0.831192661,0.83853211,0.844036697,
0.849541284,0.855045872,0.860550459,0.866055046,0.871559633,0.87706422,
0.882568807,0.888073394,0.893577982,0.900917431,0.906422018,0.911926606,
0.917431193,0.924770642,0.930275229,0.935779817,0.941284404,0.946788991,
0.952293578,0.957798165,0.963302752,0.968807339,0.974311927,0.979816514,
0.985321101,0.99266055,1.),.UNSPECIFIED.);
#24369=B_SPLINE_CURVE_WITH_KNOTS('',5,(#197001,#197002,#197003,#197004,
#197005,#197006,#197007,#197008,#197009,#197010,#197011,#197012,#197013,
#197014,#197015,#197016,#197017,#197018,#197019,#197020,#197021,#197022,
#197023,#197024,#197025,#197026,#197027,#197028,#197029,#197030,#197031,
#197032,#197033,#197034,#197035,#197036,#197037,#197038,#197039,#197040,
#197041,#197042,#197043,#197044,#197045,#197046,#197047,#197048,#197049,
#197050,#197051,#197052,#197053,#197054,#197055,#197056,#197057,#197058,
#197059,#197060,#197061,#197062,#197063,#197064,#197065,#197066,#197067,
#197068,#197069,#197070,#197071,#197072,#197073,#197074,#197075,#197076,
#197077,#197078,#197079,#197080,#197081,#197082,#197083,#197084,#197085,
#197086,#197087,#197088,#197089,#197090,#197091,#197092,#197093,#197094,
#197095,#197096,#197097,#197098,#197099,#197100,#197101,#197102,#197103,
#197104,#197105,#197106,#197107,#197108,#197109,#197110,#197111,#197112,
#197113,#197114,#197115,#197116,#197117,#197118,#197119,#197120,#197121,
#197122,#197123,#197124,#197125,#197126,#197127,#197128,#197129,#197130,
#197131,#197132,#197133,#197134,#197135,#197136,#197137,#197138,#197139,
#197140,#197141,#197142,#197143,#197144,#197145,#197146,#197147,#197148,
#197149,#197150,#197151,#197152,#197153,#197154,#197155,#197156,#197157,
#197158,#197159,#197160,#197161,#197162,#197163,#197164,#197165,#197166,
#197167,#197168,#197169,#197170,#197171,#197172,#197173,#197174,#197175,
#197176,#197177,#197178,#197179,#197180,#197181,#197182,#197183,#197184,
#197185,#197186,#197187,#197188,#197189,#197190,#197191,#197192,#197193,
#197194,#197195,#197196,#197197,#197198,#197199,#197200,#197201,#197202,
#197203,#197204,#197205,#197206,#197207,#197208,#197209,#197210,#197211,
#197212,#197213,#197214,#197215,#197216,#197217,#197218,#197219,#197220,
#197221,#197222,#197223,#197224,#197225,#197226,#197227,#197228,#197229,
#197230,#197231,#197232,#197233,#197234,#197235,#197236,#197237,#197238,
#197239,#197240,#197241,#197242,#197243,#197244,#197245,#197246,#197247,
#197248,#197249,#197250,#197251,#197252,#197253,#197254,#197255,#197256,
#197257,#197258,#197259,#197260,#197261,#197262,#197263,#197264,#197265,
#197266,#197267,#197268,#197269,#197270,#197271,#197272,#197273,#197274,
#197275,#197276,#197277,#197278,#197279,#197280,#197281,#197282,#197283,
#197284,#197285,#197286,#197287,#197288,#197289,#197290,#197291,#197292,
#197293,#197294,#197295,#197296,#197297,#197298,#197299,#197300,#197301,
#197302,#197303,#197304,#197305,#197306,#197307,#197308,#197309,#197310,
#197311,#197312,#197313,#197314,#197315,#197316,#197317,#197318,#197319,
#197320,#197321,#197322,#197323,#197324,#197325,#197326,#197327,#197328,
#197329,#197330,#197331,#197332,#197333,#197334,#197335,#197336,#197337,
#197338,#197339,#197340,#197341,#197342,#197343,#197344,#197345,#197346,
#197347,#197348,#197349,#197350,#197351,#197352,#197353,#197354,#197355,
#197356,#197357,#197358,#197359,#197360,#197361,#197362,#197363,#197364,
#197365,#197366,#197367,#197368,#197369,#197370,#197371,#197372,#197373,
#197374,#197375,#197376,#197377,#197378,#197379,#197380,#197381,#197382,
#197383,#197384,#197385,#197386,#197387,#197388,#197389,#197390,#197391,
#197392,#197393,#197394,#197395,#197396,#197397,#197398,#197399,#197400,
#197401,#197402,#197403,#197404,#197405,#197406,#197407,#197408,#197409,
#197410,#197411,#197412,#197413,#197414,#197415,#197416,#197417,#197418,
#197419,#197420,#197421,#197422,#197423,#197424,#197425,#197426,#197427,
#197428,#197429,#197430,#197431,#197432,#197433,#197434,#197435,#197436,
#197437,#197438,#197439,#197440,#197441,#197442,#197443,#197444,#197445,
#197446,#197447,#197448,#197449,#197450,#197451,#197452,#197453,#197454,
#197455,#197456,#197457,#197458,#197459,#197460,#197461,#197462,#197463,
#197464,#197465,#197466,#197467,#197468,#197469,#197470,#197471,#197472),
 .UNSPECIFIED.,.F.,.F.,(6,1,1,1,1,1,1,1,1,1,1,1,1,1,1,1,1,1,1,1,1,1,1,1,
1,1,1,1,1,1,1,1,1,1,1,1,1,1,1,1,1,1,1,1,1,1,1,1,1,1,1,1,1,1,1,1,1,1,1,1,
1,1,1,1,1,1,1,1,1,1,1,1,1,1,1,1,1,1,1,1,1,1,1,1,1,1,1,1,1,1,1,1,1,1,1,1,
1,1,1,1,1,1,1,1,1,1,1,1,1,1,1,1,1,1,1,1,1,1,1,1,1,1,1,1,1,1,1,1,1,1,1,1,
1,1,1,1,1,1,1,1,1,1,1,1,1,1,1,1,1,1,1,1,1,1,1,1,1,1,1,1,1,1,1,1,1,1,1,1,
1,1,1,1,1,1,1,1,1,1,1,1,1,1,1,1,1,1,1,1,1,1,1,1,1,1,1,1,1,1,1,1,1,1,1,1,
1,1,1,1,1,1,1,1,1,1,1,1,1,1,1,1,1,1,1,1,1,1,1,1,1,1,1,1,1,1,1,1,1,1,1,1,
1,1,1,1,1,1,1,1,1,1,1,1,1,1,1,1,1,1,1,1,1,1,1,1,1,1,1,1,1,1,1,1,1,1,1,1,
1,1,1,1,1,1,1,1,1,1,1,1,1,1,1,1,1,1,1,1,1,1,1,1,1,1,1,1,1,1,1,1,1,1,1,1,
1,1,1,1,1,1,1,1,1,1,1,1,1,1,1,1,1,1,1,1,1,1,1,1,1,1,1,1,1,1,1,1,1,1,1,1,
1,1,1,1,1,1,1,1,1,1,1,1,1,1,1,1,1,1,1,1,1,1,1,1,1,1,1,1,1,1,1,1,1,1,1,1,
1,1,1,1,1,1,1,1,1,1,1,1,1,1,1,1,1,1,1,1,1,1,1,1,1,1,1,1,1,1,1,1,1,1,1,1,
1,1,1,1,1,1,1,1,1,1,1,1,1,1,1,1,1,1,1,1,1,1,1,1,1,1,1,1,1,1,1,1,1,1,1,1,
1,1,1,1,1,1,1,1,1,1,1,6),(-1.,-0.998165138,-0.996330275,-0.994495413,-0.99266055,
-0.990825688,-0.988990826,-0.987155963,-0.985321101,-0.983486239,-0.981651376,
-0.979816514,-0.977981651,-0.976146789,-0.974311927,-0.972477064,-0.970642202,
-0.968807339,-0.966972477,-0.965137615,-0.963302752,-0.96146789,-0.959633028,
-0.957798165,-0.955963303,-0.95412844,-0.952293578,-0.950458716,-0.948623853,
-0.946788991,-0.944954128,-0.943119266,-0.941284404,-0.939449541,-0.937614679,
-0.935779817,-0.933944954,-0.932110092,-0.930275229,-0.928440367,-0.926605505,
-0.924770642,-0.92293578,-0.921100917,-0.919266055,-0.917431193,-0.91559633,
-0.913761468,-0.911926606,-0.910091743,-0.908256881,-0.906422018,-0.904587156,
-0.902752294,-0.900917431,-0.899082569,-0.897247706,-0.895412844,-0.893577982,
-0.891743119,-0.889908257,-0.888073394,-0.886238532,-0.88440367,-0.882568807,
-0.880733945,-0.878899083,-0.87706422,-0.875229358,-0.873394495,-0.871559633,
-0.869724771,-0.867889908,-0.866055046,-0.864220183,-0.862385321,-0.860550459,
-0.858715596,-0.856880734,-0.855045872,-0.853211009,-0.851376147,-0.849541284,
-0.847706422,-0.84587156,-0.844036697,-0.842201835,-0.840366972,-0.83853211,
-0.836697248,-0.834862385,-0.833027523,-0.831192661,-0.829357798,-0.827522936,
-0.825688073,-0.823853211,-0.822018349,-0.820183486,-0.818348624,-0.816513761,
-0.814678899,-0.812844037,-0.811009174,-0.809174312,-0.80733945,-0.805504587,
-0.803669725,-0.801834862,-0.8,-0.798165138,-0.796330275,-0.794495413,-0.79266055,
-0.790825688,-0.788990826,-0.787155963,-0.785321101,-0.783486239,-0.781651376,
-0.779816514,-0.777981651,-0.776146789,-0.774311927,-0.772477064,-0.770642202,
-0.768807339,-0.766972477,-0.765137615,-0.763302752,-0.76146789,-0.759633028,
-0.757798165,-0.755963303,-0.75412844,-0.752293578,-0.750458716,-0.748623853,
-0.746788991,-0.744954128,-0.743119266,-0.741284404,-0.739449541,-0.737614679,
-0.735779817,-0.733944954,-0.732110092,-0.730275229,-0.728440367,-0.726605505,
-0.724770642,-0.72293578,-0.721100917,-0.719266055,-0.717431193,-0.71559633,
-0.713761468,-0.711926606,-0.710091743,-0.708256881,-0.706422018,-0.704587156,
-0.702752294,-0.700917431,-0.699082569,-0.697247706,-0.695412844,-0.693577982,
-0.691743119,-0.689908257,-0.688073394,-0.686238532,-0.68440367,-0.682568807,
-0.680733945,-0.678899083,-0.67706422,-0.675229358,-0.673394495,-0.671559633,
-0.669724771,-0.667889908,-0.666055046,-0.664220183,-0.662385321,-0.660550459,
-0.658715596,-0.656880734,-0.655045872,-0.653211009,-0.651376147,-0.649541284,
-0.647706422,-0.64587156,-0.644036697,-0.642201835,-0.640366972,-0.63853211,
-0.636697248,-0.634862385,-0.633027523,-0.631192661,-0.629357798,-0.627522936,
-0.625688073,-0.623853211,-0.622018349,-0.620183486,-0.618348624,-0.616513761,
-0.614678899,-0.612844037,-0.611009174,-0.609174312,-0.60733945,-0.605504587,
-0.603669725,-0.601834862,-0.6,-0.598165138,-0.596330275,-0.594495413,-0.59266055,
-0.590825688,-0.588990826,-0.587155963,-0.585321101,-0.583486239,-0.581651376,
-0.579816514,-0.577981651,-0.576146789,-0.574311927,-0.572477064,-0.570642202,
-0.568807339,-0.566972477,-0.565137615,-0.563302752,-0.56146789,-0.559633028,
-0.557798165,-0.555963303,-0.55412844,-0.552293578,-0.550458716,-0.548623853,
-0.546788991,-0.544954128,-0.543119266,-0.541284404,-0.539449541,-0.537614679,
-0.535779817,-0.533944954,-0.532110092,-0.530275229,-0.528440367,-0.526605505,
-0.524770642,-0.52293578,-0.521100917,-0.519266055,-0.517431193,-0.51559633,
-0.513761468,-0.511926606,-0.510091743,-0.508256881,-0.506422018,-0.504587156,
-0.502752294,-0.500917431,-0.499082569,-0.497247706,-0.495412844,-0.493577982,
-0.491743119,-0.489908257,-0.488073394,-0.486238532,-0.48440367,-0.482568807,
-0.480733945,-0.478899083,-0.47706422,-0.475229358,-0.473394495,-0.471559633,
-0.469724771,-0.467889908,-0.466055046,-0.464220183,-0.462385321,-0.460550459,
-0.458715596,-0.456880734,-0.455045872,-0.453211009,-0.451376147,-0.449541284,
-0.447706422,-0.44587156,-0.444036697,-0.442201835,-0.440366972,-0.43853211,
-0.436697248,-0.434862385,-0.433027523,-0.431192661,-0.429357798,-0.427522936,
-0.425688073,-0.423853211,-0.422018349,-0.420183486,-0.418348624,-0.416513761,
-0.414678899,-0.412844037,-0.411009174,-0.409174312,-0.40733945,-0.405504587,
-0.403669725,-0.401834862,-0.4,-0.398165138,-0.396330275,-0.394495413,-0.39266055,
-0.390825688,-0.388990826,-0.387155963,-0.385321101,-0.383486239,-0.381651376,
-0.379816514,-0.377981651,-0.376146789,-0.374311927,-0.372477064,-0.370642202,
-0.368807339,-0.366972477,-0.365137615,-0.363302752,-0.36146789,-0.359633028,
-0.357798165,-0.355963303,-0.35412844,-0.352293578,-0.350458716,-0.348623853,
-0.346788991,-0.344954128,-0.343119266,-0.341284404,-0.339449541,-0.337614679,
-0.335779817,-0.333944954,-0.332110092,-0.330275229,-0.328440367,-0.326605505,
-0.324770642,-0.32293578,-0.321100917,-0.319266055,-0.317431193,-0.31559633,
-0.313761468,-0.311926606,-0.310091743,-0.308256881,-0.306422018,-0.304587156,
-0.302752294,-0.300917431,-0.299082569,-0.297247706,-0.295412844,-0.293577982,
-0.291743119,-0.289908257,-0.288073394,-0.286238532,-0.28440367,-0.282568807,
-0.280733945,-0.278899083,-0.27706422,-0.275229358,-0.273394495,-0.271559633,
-0.269724771,-0.267889908,-0.266055046,-0.264220183,-0.262385321,-0.260550459,
-0.258715596,-0.256880734,-0.255045872,-0.253211009,-0.251376147,-0.249541284,
-0.247706422,-0.24587156,-0.244036697,-0.242201835,-0.240366972,-0.23853211,
-0.236697248,-0.234862385,-0.233027523,-0.231192661,-0.229357798,-0.227522936,
-0.225688073,-0.223853211,-0.222018349,-0.220183486,-0.218348624,-0.216513761,
-0.214678899,-0.212844037,-0.211009174,-0.209174312,-0.20733945,-0.205504587,
-0.203669725,-0.201834862,-0.2,-0.198165138,-0.196330275,-0.194495413,-0.19266055,
-0.190825688,-0.188990826,-0.187155963,-0.185321101,-0.183486239,-0.181651376,
-0.179816514,-0.177981651,-0.176146789,-0.174311927,-0.172477064,-0.170642202,
-0.168807339,-0.166972477,-0.165137615,-0.163302752,-0.16146789,-0.159633028,
-0.157798165,-0.155963303,-0.15412844,-0.152293578,-0.150458716,-0.148623853,
-0.146788991,-0.144954128,-0.143172102),.UNSPECIFIED.);
#24370=B_SPLINE_CURVE_WITH_KNOTS('',5,(#197473,#197474,#197475,#197476,
#197477,#197478,#197479,#197480,#197481,#197482,#197483,#197484,#197485,
#197486,#197487,#197488,#197489,#197490,#197491,#197492,#197493,#197494,
#197495,#197496,#197497,#197498,#197499,#197500,#197501,#197502,#197503,
#197504,#197505,#197506,#197507,#197508,#197509,#197510,#197511,#197512,
#197513,#197514,#197515,#197516,#197517,#197518,#197519,#197520,#197521,
#197522,#197523,#197524,#197525,#197526,#197527,#197528,#197529,#197530,
#197531,#197532,#197533,#197534,#197535,#197536,#197537,#197538,#197539,
#197540,#197541,#197542,#197543,#197544,#197545,#197546,#197547,#197548,
#197549,#197550,#197551,#197552,#197553,#197554,#197555,#197556,#197557,
#197558,#197559,#197560,#197561,#197562,#197563,#197564,#197565,#197566,
#197567,#197568,#197569,#197570,#197571,#197572,#197573,#197574,#197575,
#197576,#197577,#197578,#197579,#197580,#197581,#197582,#197583,#197584,
#197585,#197586,#197587,#197588,#197589,#197590,#197591,#197592,#197593,
#197594,#197595,#197596,#197597,#197598,#197599,#197600,#197601,#197602,
#197603,#197604,#197605,#197606,#197607,#197608,#197609,#197610,#197611,
#197612,#197613,#197614,#197615,#197616,#197617,#197618,#197619,#197620,
#197621,#197622,#197623,#197624,#197625,#197626,#197627,#197628,#197629,
#197630,#197631,#197632,#197633,#197634,#197635,#197636,#197637,#197638,
#197639,#197640,#197641,#197642,#197643,#197644,#197645,#197646,#197647,
#197648,#197649,#197650,#197651,#197652,#197653,#197654,#197655,#197656,
#197657,#197658,#197659,#197660,#197661,#197662,#197663,#197664,#197665,
#197666,#197667,#197668,#197669,#197670,#197671,#197672,#197673,#197674,
#197675,#197676,#197677,#197678,#197679,#197680,#197681,#197682,#197683,
#197684,#197685,#197686,#197687,#197688,#197689,#197690,#197691,#197692,
#197693,#197694,#197695,#197696,#197697,#197698,#197699,#197700,#197701,
#197702,#197703,#197704,#197705,#197706,#197707,#197708,#197709,#197710,
#197711,#197712,#197713,#197714,#197715,#197716,#197717,#197718,#197719,
#197720,#197721,#197722,#197723,#197724,#197725,#197726,#197727,#197728,
#197729,#197730,#197731,#197732,#197733,#197734,#197735,#197736,#197737,
#197738,#197739,#197740,#197741,#197742,#197743,#197744,#197745,#197746,
#197747,#197748,#197749,#197750,#197751,#197752,#197753,#197754,#197755,
#197756,#197757,#197758,#197759,#197760,#197761,#197762,#197763,#197764,
#197765,#197766,#197767,#197768,#197769,#197770,#197771,#197772,#197773,
#197774,#197775,#197776,#197777,#197778,#197779,#197780,#197781,#197782,
#197783,#197784,#197785,#197786,#197787,#197788,#197789,#197790,#197791,
#197792,#197793,#197794,#197795,#197796,#197797,#197798,#197799,#197800,
#197801,#197802,#197803,#197804,#197805,#197806,#197807,#197808,#197809,
#197810,#197811,#197812,#197813,#197814,#197815,#197816,#197817,#197818,
#197819,#197820,#197821,#197822,#197823,#197824,#197825,#197826,#197827,
#197828,#197829,#197830,#197831,#197832,#197833,#197834,#197835,#197836,
#197837,#197838,#197839,#197840,#197841,#197842,#197843,#197844,#197845,
#197846,#197847,#197848,#197849,#197850,#197851,#197852,#197853,#197854,
#197855,#197856,#197857,#197858,#197859,#197860,#197861,#197862,#197863,
#197864,#197865,#197866,#197867,#197868,#197869,#197870,#197871,#197872,
#197873,#197874,#197875,#197876,#197877,#197878,#197879,#197880,#197881,
#197882,#197883,#197884,#197885,#197886,#197887,#197888,#197889,#197890,
#197891,#197892,#197893,#197894,#197895,#197896,#197897,#197898,#197899,
#197900,#197901,#197902,#197903,#197904,#197905,#197906,#197907,#197908,
#197909,#197910,#197911,#197912,#197913,#197914,#197915,#197916,#197917,
#197918,#197919,#197920,#197921,#197922,#197923,#197924,#197925,#197926,
#197927,#197928,#197929,#197930,#197931,#197932,#197933,#197934,#197935,
#197936,#197937,#197938,#197939,#197940,#197941,#197942,#197943,#197944),
 .UNSPECIFIED.,.F.,.F.,(6,1,1,1,1,1,1,1,1,1,1,1,1,1,1,1,1,1,1,1,1,1,1,1,
1,1,1,1,1,1,1,1,1,1,1,1,1,1,1,1,1,1,1,1,1,1,1,1,1,1,1,1,1,1,1,1,1,1,1,1,
1,1,1,1,1,1,1,1,1,1,1,1,1,1,1,1,1,1,1,1,1,1,1,1,1,1,1,1,1,1,1,1,1,1,1,1,
1,1,1,1,1,1,1,1,1,1,1,1,1,1,1,1,1,1,1,1,1,1,1,1,1,1,1,1,1,1,1,1,1,1,1,1,
1,1,1,1,1,1,1,1,1,1,1,1,1,1,1,1,1,1,1,1,1,1,1,1,1,1,1,1,1,1,1,1,1,1,1,1,
1,1,1,1,1,1,1,1,1,1,1,1,1,1,1,1,1,1,1,1,1,1,1,1,1,1,1,1,1,1,1,1,1,1,1,1,
1,1,1,1,1,1,1,1,1,1,1,1,1,1,1,1,1,1,1,1,1,1,1,1,1,1,1,1,1,1,1,1,1,1,1,1,
1,1,1,1,1,1,1,1,1,1,1,1,1,1,1,1,1,1,1,1,1,1,1,1,1,1,1,1,1,1,1,1,1,1,1,1,
1,1,1,1,1,1,1,1,1,1,1,1,1,1,1,1,1,1,1,1,1,1,1,1,1,1,1,1,1,1,1,1,1,1,1,1,
1,1,1,1,1,1,1,1,1,1,1,1,1,1,1,1,1,1,1,1,1,1,1,1,1,1,1,1,1,1,1,1,1,1,1,1,
1,1,1,1,1,1,1,1,1,1,1,1,1,1,1,1,1,1,1,1,1,1,1,1,1,1,1,1,1,1,1,1,1,1,1,1,
1,1,1,1,1,1,1,1,1,1,1,1,1,1,1,1,1,1,1,1,1,1,1,1,1,1,1,1,1,1,1,1,1,1,1,1,
1,1,1,1,1,1,1,1,1,1,1,1,1,1,1,1,1,1,1,1,1,1,1,1,1,1,1,1,1,1,1,1,1,1,1,1,
1,1,1,1,1,1,1,1,1,1,1,6),(0.143172102,0.144954128,0.146788991,0.148623853,
0.150458716,0.152293578,0.15412844,0.155963303,0.157798165,0.159633028,
0.16146789,0.163302752,0.165137615,0.166972477,0.168807339,0.170642202,
0.172477064,0.174311927,0.176146789,0.177981651,0.179816514,0.181651376,
0.183486239,0.185321101,0.187155963,0.188990826,0.190825688,0.19266055,
0.194495413,0.196330275,0.198165138,0.2,0.201834862,0.203669725,0.205504587,
0.20733945,0.209174312,0.211009174,0.212844037,0.214678899,0.216513761,
0.218348624,0.220183486,0.222018349,0.223853211,0.225688073,0.227522936,
0.229357798,0.231192661,0.233027523,0.234862385,0.236697248,0.23853211,
0.240366972,0.242201835,0.244036697,0.24587156,0.247706422,0.249541284,
0.251376147,0.253211009,0.255045872,0.256880734,0.258715596,0.260550459,
0.262385321,0.264220183,0.266055046,0.267889908,0.269724771,0.271559633,
0.273394495,0.275229358,0.27706422,0.278899083,0.280733945,0.282568807,
0.28440367,0.286238532,0.288073394,0.289908257,0.291743119,0.293577982,
0.295412844,0.297247706,0.299082569,0.300917431,0.302752294,0.304587156,
0.306422018,0.308256881,0.310091743,0.311926606,0.313761468,0.31559633,
0.317431193,0.319266055,0.321100917,0.32293578,0.324770642,0.326605505,
0.328440367,0.330275229,0.332110092,0.333944954,0.335779817,0.337614679,
0.339449541,0.341284404,0.343119266,0.344954128,0.346788991,0.348623853,
0.350458716,0.352293578,0.35412844,0.355963303,0.357798165,0.359633028,
0.36146789,0.363302752,0.365137615,0.366972477,0.368807339,0.370642202,
0.372477064,0.374311927,0.376146789,0.377981651,0.379816514,0.381651376,
0.383486239,0.385321101,0.387155963,0.388990826,0.390825688,0.39266055,
0.394495413,0.396330275,0.398165138,0.4,0.401834862,0.403669725,0.405504587,
0.40733945,0.409174312,0.411009174,0.412844037,0.414678899,0.416513761,
0.418348624,0.420183486,0.422018349,0.423853211,0.425688073,0.427522936,
0.429357798,0.431192661,0.433027523,0.434862385,0.436697248,0.43853211,
0.440366972,0.442201835,0.444036697,0.44587156,0.447706422,0.449541284,
0.451376147,0.453211009,0.455045872,0.456880734,0.458715596,0.460550459,
0.462385321,0.464220183,0.466055046,0.467889908,0.469724771,0.471559633,
0.473394495,0.475229358,0.47706422,0.478899083,0.480733945,0.482568807,
0.48440367,0.486238532,0.488073394,0.489908257,0.491743119,0.493577982,
0.495412844,0.497247706,0.499082569,0.500917431,0.502752294,0.504587156,
0.506422018,0.508256881,0.510091743,0.511926606,0.513761468,0.51559633,
0.517431193,0.519266055,0.521100917,0.52293578,0.524770642,0.526605505,
0.528440367,0.530275229,0.532110092,0.533944954,0.535779817,0.537614679,
0.539449541,0.541284404,0.543119266,0.544954128,0.546788991,0.548623853,
0.550458716,0.552293578,0.55412844,0.555963303,0.557798165,0.559633028,
0.56146789,0.563302752,0.565137615,0.566972477,0.568807339,0.570642202,
0.572477064,0.574311927,0.576146789,0.577981651,0.579816514,0.581651376,
0.583486239,0.585321101,0.587155963,0.588990826,0.590825688,0.59266055,
0.594495413,0.596330275,0.598165138,0.6,0.601834862,0.603669725,0.605504587,
0.60733945,0.609174312,0.611009174,0.612844037,0.614678899,0.616513761,
0.618348624,0.620183486,0.622018349,0.623853211,0.625688073,0.627522936,
0.629357798,0.631192661,0.633027523,0.634862385,0.636697248,0.63853211,
0.640366972,0.642201835,0.644036697,0.64587156,0.647706422,0.649541284,
0.651376147,0.653211009,0.655045872,0.656880734,0.658715596,0.660550459,
0.662385321,0.664220183,0.666055046,0.667889908,0.669724771,0.671559633,
0.673394495,0.675229358,0.67706422,0.678899083,0.680733945,0.682568807,
0.68440367,0.686238532,0.688073394,0.689908257,0.691743119,0.693577982,
0.695412844,0.697247706,0.699082569,0.700917431,0.702752294,0.704587156,
0.706422018,0.708256881,0.710091743,0.711926606,0.713761468,0.71559633,
0.717431193,0.719266055,0.721100917,0.72293578,0.724770642,0.726605505,
0.728440367,0.730275229,0.732110092,0.733944954,0.735779817,0.737614679,
0.739449541,0.741284404,0.743119266,0.744954128,0.746788991,0.748623853,
0.750458716,0.752293578,0.75412844,0.755963303,0.757798165,0.759633028,
0.76146789,0.763302752,0.765137615,0.766972477,0.768807339,0.770642202,
0.772477064,0.774311927,0.776146789,0.777981651,0.779816514,0.781651376,
0.783486239,0.785321101,0.787155963,0.788990826,0.790825688,0.79266055,
0.794495413,0.796330275,0.798165138,0.8,0.801834862,0.803669725,0.805504587,
0.80733945,0.809174312,0.811009174,0.812844037,0.814678899,0.816513761,
0.818348624,0.820183486,0.822018349,0.823853211,0.825688073,0.827522936,
0.829357798,0.831192661,0.833027523,0.834862385,0.836697248,0.83853211,
0.840366972,0.842201835,0.844036697,0.84587156,0.847706422,0.849541284,
0.851376147,0.853211009,0.855045872,0.856880734,0.858715596,0.860550459,
0.862385321,0.864220183,0.866055046,0.867889908,0.869724771,0.871559633,
0.873394495,0.875229358,0.87706422,0.878899083,0.880733945,0.882568807,
0.88440367,0.886238532,0.888073394,0.889908257,0.891743119,0.893577982,
0.895412844,0.897247706,0.899082569,0.900917431,0.902752294,0.904587156,
0.906422018,0.908256881,0.910091743,0.911926606,0.913761468,0.91559633,
0.917431193,0.919266055,0.921100917,0.92293578,0.924770642,0.926605505,
0.928440367,0.930275229,0.932110092,0.933944954,0.935779817,0.937614679,
0.939449541,0.941284404,0.943119266,0.944954128,0.946788991,0.948623853,
0.950458716,0.952293578,0.95412844,0.955963303,0.957798165,0.959633028,
0.96146789,0.963302752,0.965137615,0.966972477,0.968807339,0.970642202,
0.972477064,0.974311927,0.976146789,0.977981651,0.979816514,0.981651376,
0.983486239,0.985321101,0.987155963,0.988990826,0.990825688,0.99266055,
0.994495413,0.996330275,0.998165138,1.),.UNSPECIFIED.);
#24371=B_SPLINE_CURVE_WITH_KNOTS('',3,(#198907,#198908,#198909,#198910,
#198911,#198912,#198913,#198914,#198915,#198916,#198917,#198918,#198919,
#198920,#198921,#198922,#198923,#198924,#198925,#198926,#198927,#198928,
#198929,#198930,#198931,#198932,#198933,#198934,#198935,#198936,#198937,
#198938,#198939,#198940,#198941,#198942,#198943,#198944,#198945,#198946,
#198947,#198948,#198949,#198950,#198951,#198952,#198953,#198954,#198955,
#198956,#198957,#198958,#198959,#198960,#198961,#198962,#198963,#198964,
#198965,#198966,#198967,#198968,#198969,#198970,#198971,#198972,#198973,
#198974,#198975,#198976,#198977,#198978,#198979,#198980,#198981,#198982,
#198983,#198984,#198985,#198986,#198987,#198988,#198989,#198990,#198991,
#198992,#198993,#198994,#198995,#198996,#198997,#198998,#198999,#199000,
#199001,#199002,#199003,#199004,#199005,#199006,#199007,#199008,#199009,
#199010,#199011,#199012,#199013,#199014,#199015,#199016,#199017,#199018,
#199019,#199020,#199021,#199022,#199023,#199024,#199025,#199026,#199027,
#199028,#199029,#199030,#199031,#199032,#199033,#199034,#199035,#199036,
#199037,#199038,#199039,#199040,#199041,#199042,#199043,#199044,#199045,
#199046,#199047,#199048,#199049,#199050,#199051,#199052,#199053,#199054,
#199055,#199056,#199057,#199058,#199059,#199060,#199061,#199062,#199063,
#199064,#199065,#199066,#199067,#199068,#199069,#199070,#199071,#199072,
#199073,#199074,#199075,#199076,#199077,#199078,#199079,#199080,#199081,
#199082,#199083,#199084,#199085,#199086,#199087,#199088,#199089,#199090,
#199091,#199092,#199093,#199094,#199095,#199096,#199097,#199098,#199099,
#199100,#199101,#199102,#199103,#199104,#199105,#199106,#199107,#199108,
#199109,#199110,#199111,#199112,#199113,#199114,#199115,#199116,#199117,
#199118,#199119,#199120,#199121,#199122,#199123,#199124,#199125,#199126,
#199127,#199128,#199129,#199130,#199131,#199132,#199133,#199134,#199135,
#199136,#199137,#199138,#199139,#199140,#199141,#199142,#199143,#199144,
#199145,#199146,#199147,#199148,#199149,#199150,#199151,#199152,#199153,
#199154,#199155,#199156,#199157,#199158,#199159,#199160,#199161,#199162,
#199163,#199164,#199165,#199166,#199167,#199168,#199169,#199170,#199171,
#199172,#199173,#199174,#199175,#199176,#199177,#199178,#199179,#199180,
#199181,#199182,#199183,#199184,#199185,#199186,#199187,#199188,#199189,
#199190,#199191,#199192,#199193,#199194,#199195,#199196,#199197,#199198,
#199199,#199200,#199201,#199202,#199203,#199204,#199205,#199206,#199207,
#199208,#199209,#199210,#199211,#199212,#199213,#199214,#199215,#199216,
#199217,#199218,#199219),.UNSPECIFIED.,.F.,.F.,(4,3,3,3,3,3,3,3,3,3,3,3,
3,3,3,3,3,3,3,3,3,3,3,3,3,3,3,3,3,3,3,3,3,3,3,3,3,3,3,3,3,3,3,3,3,3,3,3,
3,3,3,3,3,3,3,3,3,3,3,3,3,3,3,3,3,3,3,3,3,3,3,3,3,3,3,3,3,3,3,3,3,3,3,3,
3,3,3,3,3,3,3,3,3,3,3,3,3,3,3,3,3,3,3,3,4),(-1.,-0.990825688,-0.985321101,
-0.979816514,-0.974311927,-0.966972477,-0.959633028,-0.95412844,-0.948623853,
-0.941284404,-0.932110092,-0.926605505,-0.921100917,-0.913761468,-0.908256881,
-0.900917431,-0.895412844,-0.889908257,-0.88440367,-0.878899083,-0.873394495,
-0.867889908,-0.860550459,-0.855045872,-0.849541284,-0.842201835,-0.836697248,
-0.831192661,-0.825688073,-0.820183486,-0.814678899,-0.809174312,-0.801834862,
-0.794495413,-0.781651376,-0.774311927,-0.766972477,-0.759633028,-0.752293578,
-0.743119266,-0.735779817,-0.728440367,-0.721100917,-0.708256881,-0.700917431,
-0.693577982,-0.686238532,-0.678899083,-0.671559633,-0.664220183,-0.656880734,
-0.649541284,-0.642201835,-0.634862385,-0.627522936,-0.620183486,-0.612844037,
-0.605504587,-0.598165138,-0.590825688,-0.583486239,-0.576146789,-0.568807339,
-0.56146789,-0.55412844,-0.546788991,-0.539449541,-0.532110092,-0.52293578,
-0.513761468,-0.504587156,-0.495412844,-0.486238532,-0.47706422,-0.467889908,
-0.458715596,-0.447706422,-0.43853211,-0.429357798,-0.420183486,-0.411009174,
-0.401834862,-0.39266055,-0.381651376,-0.370642202,-0.359633028,-0.346788991,
-0.335779817,-0.324770642,-0.313761468,-0.302752294,-0.291743119,-0.278899083,
-0.267889908,-0.256880734,-0.244036697,-0.233027523,-0.222018349,-0.211009174,
-0.2,-0.188990826,-0.177981651,-0.166972477,-0.155963303,-0.143172102),
 .UNSPECIFIED.);
#24372=B_SPLINE_CURVE_WITH_KNOTS('',3,(#199220,#199221,#199222,#199223,
#199224,#199225,#199226,#199227,#199228,#199229,#199230,#199231,#199232,
#199233,#199234,#199235,#199236,#199237,#199238,#199239,#199240,#199241,
#199242,#199243,#199244,#199245,#199246,#199247,#199248,#199249,#199250,
#199251,#199252,#199253,#199254,#199255,#199256,#199257,#199258,#199259,
#199260,#199261,#199262,#199263,#199264,#199265,#199266,#199267,#199268,
#199269,#199270,#199271,#199272,#199273,#199274,#199275,#199276,#199277,
#199278,#199279,#199280,#199281,#199282,#199283,#199284,#199285,#199286,
#199287,#199288,#199289,#199290,#199291,#199292,#199293,#199294,#199295,
#199296,#199297,#199298,#199299,#199300,#199301,#199302,#199303,#199304,
#199305,#199306,#199307,#199308,#199309,#199310,#199311,#199312,#199313,
#199314,#199315,#199316,#199317,#199318,#199319,#199320,#199321,#199322,
#199323,#199324,#199325,#199326,#199327,#199328,#199329,#199330,#199331,
#199332,#199333,#199334,#199335,#199336,#199337,#199338,#199339,#199340,
#199341,#199342,#199343,#199344,#199345,#199346,#199347,#199348,#199349,
#199350,#199351,#199352,#199353,#199354,#199355,#199356,#199357,#199358,
#199359,#199360,#199361,#199362,#199363,#199364,#199365,#199366,#199367,
#199368,#199369,#199370,#199371,#199372,#199373,#199374,#199375,#199376,
#199377,#199378,#199379,#199380,#199381,#199382,#199383,#199384,#199385,
#199386,#199387,#199388,#199389,#199390,#199391,#199392,#199393,#199394,
#199395,#199396,#199397,#199398,#199399,#199400,#199401,#199402,#199403,
#199404,#199405,#199406,#199407,#199408,#199409,#199410,#199411,#199412,
#199413,#199414,#199415,#199416,#199417,#199418,#199419,#199420,#199421,
#199422,#199423,#199424,#199425,#199426,#199427,#199428,#199429,#199430,
#199431,#199432,#199433,#199434,#199435,#199436,#199437,#199438,#199439,
#199440,#199441,#199442,#199443,#199444,#199445,#199446,#199447,#199448,
#199449,#199450,#199451,#199452,#199453,#199454,#199455,#199456,#199457,
#199458,#199459,#199460,#199461,#199462,#199463,#199464,#199465,#199466,
#199467,#199468,#199469,#199470,#199471,#199472,#199473,#199474,#199475,
#199476,#199477,#199478,#199479,#199480,#199481,#199482,#199483,#199484,
#199485,#199486,#199487,#199488,#199489,#199490,#199491,#199492,#199493,
#199494,#199495,#199496,#199497,#199498,#199499,#199500,#199501,#199502,
#199503,#199504,#199505,#199506,#199507,#199508,#199509,#199510,#199511,
#199512,#199513,#199514,#199515,#199516,#199517),.UNSPECIFIED.,.F.,.F.,
(4,3,3,3,3,3,3,3,3,3,3,3,3,3,3,3,3,3,3,3,3,3,3,3,3,3,3,3,3,3,3,3,3,3,3,
3,3,3,3,3,3,3,3,3,3,3,3,3,3,3,3,3,3,3,3,3,3,3,3,3,3,3,3,3,3,3,3,3,3,3,3,
3,3,3,3,3,3,3,3,3,3,3,3,3,3,3,3,3,3,3,3,3,3,3,3,3,3,3,3,4),(0.143172102,
0.15412844,0.165137615,0.176146789,0.187155963,0.198165138,0.211009174,
0.222018349,0.233027523,0.244036697,0.255045872,0.271559633,0.282568807,
0.293577982,0.304587156,0.317431193,0.328440367,0.339449541,0.352293578,
0.363302752,0.374311927,0.385321101,0.396330275,0.405504587,0.414678899,
0.425688073,0.434862385,0.44587156,0.455045872,0.466055046,0.475229358,
0.48440367,0.493577982,0.502752294,0.511926606,0.521100917,0.530275229,
0.543119266,0.552293578,0.56146789,0.568807339,0.576146789,0.585321101,
0.59266055,0.6,0.60733945,0.614678899,0.623853211,0.633027523,0.640366972,
0.649541284,0.658715596,0.666055046,0.673394495,0.680733945,0.688073394,
0.695412844,0.704587156,0.713761468,0.721100917,0.728440367,0.739449541,
0.748623853,0.755963303,0.763302752,0.770642202,0.777981651,0.785321101,
0.79266055,0.803669725,0.814678899,0.820183486,0.825688073,0.831192661,
0.836697248,0.842201835,0.847706422,0.853211009,0.858715596,0.864220183,
0.873394495,0.878899083,0.88440367,0.889908257,0.897247706,0.906422018,
0.91559633,0.924770642,0.930275229,0.935779817,0.944954128,0.950458716,
0.955963303,0.963302752,0.968807339,0.974311927,0.979816514,0.987155963,
0.99266055,1.),.UNSPECIFIED.);
#24373=B_SPLINE_CURVE_WITH_KNOTS('',3,(#200462,#200463,#200464,#200465,
#200466,#200467,#200468,#200469,#200470,#200471,#200472,#200473,#200474,
#200475,#200476,#200477,#200478,#200479,#200480,#200481,#200482,#200483,
#200484,#200485,#200486,#200487,#200488,#200489,#200490,#200491,#200492,
#200493,#200494,#200495,#200496,#200497,#200498,#200499,#200500,#200501,
#200502,#200503,#200504,#200505,#200506,#200507,#200508,#200509,#200510,
#200511,#200512,#200513,#200514,#200515,#200516,#200517,#200518,#200519,
#200520,#200521,#200522,#200523,#200524,#200525,#200526,#200527,#200528,
#200529,#200530,#200531,#200532,#200533,#200534,#200535,#200536,#200537,
#200538,#200539,#200540,#200541,#200542,#200543,#200544,#200545,#200546,
#200547,#200548,#200549,#200550,#200551,#200552,#200553,#200554,#200555,
#200556,#200557,#200558,#200559,#200560,#200561,#200562,#200563,#200564,
#200565,#200566,#200567,#200568,#200569,#200570,#200571,#200572,#200573,
#200574,#200575,#200576,#200577,#200578,#200579,#200580,#200581,#200582,
#200583,#200584,#200585,#200586,#200587,#200588,#200589,#200590,#200591,
#200592,#200593,#200594,#200595,#200596,#200597,#200598,#200599,#200600,
#200601,#200602,#200603,#200604,#200605,#200606,#200607,#200608,#200609,
#200610,#200611,#200612,#200613,#200614,#200615,#200616,#200617,#200618,
#200619,#200620,#200621,#200622,#200623,#200624,#200625,#200626,#200627,
#200628,#200629,#200630,#200631,#200632,#200633,#200634,#200635,#200636,
#200637,#200638,#200639,#200640,#200641,#200642,#200643,#200644,#200645,
#200646,#200647,#200648,#200649,#200650,#200651,#200652,#200653,#200654,
#200655,#200656,#200657,#200658,#200659,#200660,#200661,#200662,#200663,
#200664,#200665,#200666,#200667,#200668,#200669,#200670,#200671,#200672,
#200673,#200674,#200675,#200676,#200677,#200678,#200679,#200680,#200681,
#200682,#200683,#200684,#200685,#200686,#200687,#200688,#200689,#200690,
#200691,#200692,#200693,#200694,#200695,#200696,#200697,#200698,#200699,
#200700,#200701,#200702,#200703,#200704,#200705,#200706,#200707,#200708,
#200709,#200710,#200711,#200712,#200713,#200714,#200715,#200716,#200717,
#200718,#200719,#200720,#200721,#200722,#200723,#200724,#200725,#200726,
#200727,#200728,#200729,#200730,#200731,#200732,#200733,#200734,#200735,
#200736,#200737,#200738,#200739,#200740,#200741,#200742,#200743,#200744,
#200745,#200746,#200747,#200748,#200749,#200750,#200751,#200752,#200753,
#200754,#200755,#200756,#200757,#200758,#200759,#200760,#200761,#200762,
#200763,#200764,#200765,#200766,#200767,#200768,#200769,#200770,#200771,
#200772,#200773,#200774,#200775,#200776,#200777),.UNSPECIFIED.,.F.,.F.,
(4,3,3,3,3,3,3,3,3,3,3,3,3,3,3,3,3,3,3,3,3,3,3,3,3,3,3,3,3,3,3,3,3,3,3,
3,3,3,3,3,3,3,3,3,3,3,3,3,3,3,3,3,3,3,3,3,3,3,3,3,3,3,3,3,3,3,3,3,3,3,3,
3,3,3,3,3,3,3,3,3,3,3,3,3,3,3,3,3,3,3,3,3,3,3,3,3,3,3,3,3,3,3,3,3,3,4),
(0.143172102,0.15412844,0.165137615,0.176146789,0.187155963,0.198165138,
0.211009174,0.222018349,0.233027523,0.244036697,0.255045872,0.266055046,
0.27706422,0.288073394,0.299082569,0.310091743,0.321100917,0.332110092,
0.343119266,0.355963303,0.366972477,0.377981651,0.388990826,0.398165138,
0.40733945,0.418348624,0.427522936,0.436697248,0.44587156,0.455045872,0.464220183,
0.473394495,0.482568807,0.491743119,0.500917431,0.510091743,0.519266055,
0.528440367,0.535779817,0.543119266,0.550458716,0.557798165,0.565137615,
0.572477064,0.579816514,0.587155963,0.594495413,0.601834862,0.609174312,
0.616513761,0.625688073,0.633027523,0.640366972,0.649541284,0.656880734,
0.666055046,0.673394495,0.680733945,0.689908257,0.697247706,0.704587156,
0.711926606,0.719266055,0.726605505,0.733944954,0.741284404,0.748623853,
0.755963303,0.763302752,0.772477064,0.779816514,0.787155963,0.794495413,
0.803669725,0.811009174,0.816513761,0.822018349,0.827522936,0.833027523,
0.83853211,0.844036697,0.851376147,0.858715596,0.866055046,0.871559633,
0.878899083,0.886238532,0.891743119,0.897247706,0.902752294,0.910091743,
0.91559633,0.921100917,0.926605505,0.932110092,0.937614679,0.943119266,
0.950458716,0.957798165,0.965137615,0.970642202,0.976146789,0.981651376,
0.988990826,0.994495413,1.),.UNSPECIFIED.);
#24374=B_SPLINE_CURVE_WITH_KNOTS('',3,(#200778,#200779,#200780,#200781,
#200782,#200783,#200784,#200785,#200786,#200787,#200788,#200789,#200790,
#200791,#200792,#200793,#200794,#200795,#200796,#200797,#200798,#200799,
#200800,#200801,#200802,#200803,#200804,#200805,#200806,#200807,#200808,
#200809,#200810,#200811,#200812,#200813,#200814,#200815,#200816,#200817,
#200818,#200819,#200820,#200821,#200822,#200823,#200824,#200825,#200826,
#200827,#200828,#200829,#200830,#200831,#200832,#200833,#200834,#200835,
#200836,#200837,#200838,#200839,#200840,#200841,#200842,#200843,#200844,
#200845,#200846,#200847,#200848,#200849,#200850,#200851,#200852,#200853,
#200854,#200855,#200856,#200857,#200858,#200859,#200860,#200861,#200862,
#200863,#200864,#200865,#200866,#200867,#200868,#200869,#200870,#200871,
#200872,#200873,#200874,#200875,#200876,#200877,#200878,#200879,#200880,
#200881,#200882,#200883,#200884,#200885,#200886,#200887,#200888,#200889,
#200890,#200891,#200892,#200893,#200894,#200895,#200896,#200897,#200898,
#200899,#200900,#200901,#200902,#200903,#200904,#200905,#200906,#200907,
#200908,#200909,#200910,#200911,#200912,#200913,#200914,#200915,#200916,
#200917,#200918,#200919,#200920,#200921,#200922,#200923,#200924,#200925,
#200926,#200927,#200928,#200929,#200930,#200931,#200932,#200933,#200934,
#200935,#200936,#200937,#200938,#200939,#200940,#200941,#200942,#200943,
#200944,#200945,#200946,#200947,#200948,#200949,#200950,#200951,#200952,
#200953,#200954,#200955,#200956,#200957,#200958,#200959,#200960,#200961,
#200962,#200963,#200964,#200965,#200966,#200967,#200968,#200969,#200970,
#200971,#200972,#200973,#200974,#200975,#200976,#200977,#200978,#200979,
#200980,#200981,#200982,#200983,#200984,#200985,#200986,#200987,#200988,
#200989,#200990,#200991,#200992,#200993,#200994,#200995,#200996,#200997,
#200998,#200999,#201000,#201001,#201002,#201003,#201004,#201005,#201006,
#201007,#201008,#201009,#201010,#201011,#201012,#201013,#201014,#201015,
#201016,#201017,#201018,#201019,#201020,#201021,#201022,#201023,#201024,
#201025,#201026,#201027,#201028,#201029,#201030,#201031,#201032,#201033,
#201034,#201035,#201036,#201037,#201038,#201039,#201040,#201041,#201042,
#201043,#201044,#201045,#201046,#201047,#201048,#201049,#201050,#201051,
#201052,#201053,#201054,#201055,#201056,#201057,#201058,#201059,#201060,
#201061,#201062,#201063,#201064,#201065,#201066,#201067,#201068,#201069,
#201070,#201071,#201072,#201073,#201074,#201075,#201076,#201077,#201078,
#201079,#201080,#201081,#201082,#201083,#201084,#201085,#201086,#201087,
#201088,#201089,#201090,#201091,#201092,#201093,#201094,#201095,#201096,
#201097,#201098,#201099,#201100,#201101,#201102),.UNSPECIFIED.,.F.,.F.,
(4,3,3,3,3,3,3,3,3,3,3,3,3,3,3,3,3,3,3,3,3,3,3,3,3,3,3,3,3,3,3,3,3,3,3,
3,3,3,3,3,3,3,3,3,3,3,3,3,3,3,3,3,3,3,3,3,3,3,3,3,3,3,3,3,3,3,3,3,3,3,3,
3,3,3,3,3,3,3,3,3,3,3,3,3,3,3,3,3,3,3,3,3,3,3,3,3,3,3,3,3,3,3,3,3,3,3,3,
3,4),(0.143172102,0.15412844,0.165137615,0.176146789,0.187155963,0.198165138,
0.209174312,0.220183486,0.231192661,0.242201835,0.253211009,0.264220183,
0.275229358,0.286238532,0.297247706,0.308256881,0.319266055,0.330275229,
0.341284404,0.352293578,0.363302752,0.374311927,0.385321101,0.396330275,
0.405504587,0.414678899,0.423853211,0.433027523,0.442201835,0.451376147,
0.460550459,0.469724771,0.478899083,0.488073394,0.497247706,0.506422018,
0.51559633,0.524770642,0.533944954,0.541284404,0.548623853,0.555963303,
0.563302752,0.570642202,0.577981651,0.585321101,0.59266055,0.6,0.60733945,
0.614678899,0.622018349,0.629357798,0.636697248,0.644036697,0.651376147,
0.658715596,0.666055046,0.673394495,0.680733945,0.688073394,0.695412844,
0.704587156,0.711926606,0.719266055,0.726605505,0.733944954,0.741284404,
0.748623853,0.755963303,0.763302752,0.772477064,0.779816514,0.787155963,
0.794495413,0.803669725,0.811009174,0.816513761,0.822018349,0.827522936,
0.833027523,0.840366972,0.84587156,0.853211009,0.858715596,0.864220183,
0.869724771,0.875229358,0.880733945,0.886238532,0.891743119,0.897247706,
0.902752294,0.908256881,0.913761468,0.919266055,0.924770642,0.930275229,
0.935779817,0.941284404,0.946788991,0.95412844,0.959633028,0.965137615,
0.970642202,0.976146789,0.981651376,0.987155963,0.99266055,1.),
 .UNSPECIFIED.);
#24375=B_SPLINE_CURVE_WITH_KNOTS('',3,(#202062,#202063,#202064,#202065,
#202066,#202067,#202068,#202069,#202070,#202071,#202072,#202073,#202074,
#202075,#202076,#202077,#202078,#202079,#202080,#202081,#202082,#202083,
#202084,#202085,#202086,#202087,#202088,#202089,#202090,#202091,#202092,
#202093,#202094,#202095,#202096,#202097,#202098,#202099,#202100,#202101,
#202102,#202103,#202104,#202105,#202106,#202107,#202108,#202109,#202110,
#202111,#202112,#202113,#202114,#202115,#202116,#202117,#202118,#202119,
#202120,#202121,#202122,#202123,#202124,#202125,#202126,#202127,#202128,
#202129,#202130,#202131,#202132,#202133,#202134,#202135,#202136,#202137,
#202138,#202139,#202140,#202141,#202142,#202143,#202144,#202145,#202146,
#202147,#202148,#202149,#202150,#202151,#202152,#202153,#202154,#202155,
#202156,#202157,#202158,#202159,#202160,#202161,#202162,#202163,#202164,
#202165,#202166,#202167,#202168,#202169,#202170,#202171,#202172,#202173,
#202174,#202175,#202176,#202177,#202178,#202179,#202180,#202181,#202182,
#202183,#202184,#202185,#202186,#202187,#202188,#202189,#202190,#202191,
#202192,#202193,#202194,#202195,#202196,#202197,#202198,#202199,#202200,
#202201,#202202,#202203,#202204,#202205,#202206,#202207,#202208,#202209,
#202210,#202211,#202212,#202213,#202214,#202215,#202216,#202217,#202218,
#202219,#202220,#202221,#202222,#202223,#202224,#202225,#202226,#202227,
#202228,#202229,#202230,#202231,#202232,#202233,#202234,#202235,#202236,
#202237,#202238,#202239,#202240,#202241,#202242,#202243,#202244,#202245,
#202246,#202247,#202248,#202249,#202250,#202251,#202252,#202253,#202254,
#202255,#202256,#202257,#202258,#202259,#202260,#202261,#202262,#202263,
#202264,#202265,#202266,#202267,#202268,#202269,#202270,#202271,#202272,
#202273,#202274,#202275,#202276,#202277,#202278,#202279,#202280,#202281,
#202282,#202283,#202284,#202285,#202286,#202287,#202288,#202289,#202290,
#202291,#202292,#202293,#202294,#202295,#202296,#202297,#202298,#202299,
#202300,#202301,#202302,#202303,#202304,#202305,#202306,#202307,#202308,
#202309,#202310,#202311,#202312,#202313,#202314,#202315,#202316,#202317,
#202318,#202319,#202320,#202321,#202322,#202323,#202324,#202325,#202326,
#202327,#202328,#202329,#202330,#202331,#202332,#202333,#202334,#202335,
#202336,#202337,#202338,#202339,#202340,#202341,#202342,#202343,#202344,
#202345,#202346,#202347,#202348,#202349,#202350,#202351,#202352,#202353,
#202354,#202355,#202356,#202357,#202358,#202359,#202360,#202361,#202362,
#202363,#202364,#202365,#202366,#202367,#202368,#202369,#202370,#202371),
 .UNSPECIFIED.,.F.,.F.,(4,3,3,3,3,3,3,3,3,3,3,3,3,3,3,3,3,3,3,3,3,3,3,3,
3,3,3,3,3,3,3,3,3,3,3,3,3,3,3,3,3,3,3,3,3,3,3,3,3,3,3,3,3,3,3,3,3,3,3,3,
3,3,3,3,3,3,3,3,3,3,3,3,3,3,3,3,3,3,3,3,3,3,3,3,3,3,3,3,3,3,3,3,3,3,3,3,
3,3,3,3,3,3,3,4),(0.143172102,0.15412844,0.165137615,0.177981651,0.188990826,
0.201834862,0.212844037,0.225688073,0.236697248,0.249541284,0.260550459,
0.271559633,0.282568807,0.293577982,0.304587156,0.317431193,0.328440367,
0.339449541,0.350458716,0.36146789,0.372477064,0.383486239,0.394495413,
0.403669725,0.412844037,0.423853211,0.433027523,0.442201835,0.451376147,
0.460550459,0.469724771,0.478899083,0.488073394,0.497247706,0.506422018,
0.51559633,0.524770642,0.533944954,0.541284404,0.550458716,0.557798165,
0.566972477,0.574311927,0.583486239,0.59266055,0.6,0.60733945,0.614678899,
0.622018349,0.629357798,0.63853211,0.64587156,0.655045872,0.666055046,0.673394495,
0.680733945,0.689908257,0.700917431,0.708256881,0.71559633,0.72293578,0.732110092,
0.739449541,0.746788991,0.757798165,0.766972477,0.774311927,0.781651376,
0.788990826,0.796330275,0.80733945,0.812844037,0.818348624,0.823853211,
0.829357798,0.834862385,0.840366972,0.84587156,0.855045872,0.860550459,
0.866055046,0.871559633,0.87706422,0.882568807,0.888073394,0.893577982,
0.899082569,0.906422018,0.911926606,0.917431193,0.92293578,0.928440367,
0.933944954,0.941284404,0.946788991,0.952293578,0.957798165,0.963302752,
0.970642202,0.976146789,0.981651376,0.987155963,0.99266055,1.),
 .UNSPECIFIED.);
#24376=B_SPLINE_CURVE_WITH_KNOTS('',3,(#202372,#202373,#202374,#202375,
#202376,#202377,#202378,#202379,#202380,#202381,#202382,#202383,#202384,
#202385,#202386,#202387,#202388,#202389,#202390,#202391,#202392,#202393,
#202394,#202395,#202396,#202397,#202398,#202399,#202400,#202401,#202402,
#202403,#202404,#202405,#202406,#202407,#202408,#202409,#202410,#202411,
#202412,#202413,#202414,#202415,#202416,#202417,#202418,#202419,#202420,
#202421,#202422,#202423,#202424,#202425,#202426,#202427,#202428,#202429,
#202430,#202431,#202432,#202433,#202434,#202435,#202436,#202437,#202438,
#202439,#202440,#202441,#202442,#202443,#202444,#202445,#202446,#202447,
#202448,#202449,#202450,#202451,#202452,#202453,#202454,#202455,#202456,
#202457,#202458,#202459,#202460,#202461,#202462,#202463,#202464,#202465,
#202466,#202467,#202468,#202469,#202470,#202471,#202472,#202473,#202474,
#202475,#202476,#202477,#202478,#202479,#202480,#202481,#202482,#202483,
#202484,#202485,#202486,#202487,#202488,#202489,#202490,#202491,#202492,
#202493,#202494,#202495,#202496,#202497,#202498,#202499,#202500,#202501,
#202502,#202503,#202504,#202505,#202506,#202507,#202508,#202509,#202510,
#202511,#202512,#202513,#202514,#202515,#202516,#202517,#202518,#202519,
#202520,#202521,#202522,#202523,#202524,#202525,#202526,#202527,#202528,
#202529,#202530,#202531,#202532,#202533,#202534,#202535,#202536,#202537,
#202538,#202539,#202540,#202541,#202542,#202543,#202544,#202545,#202546,
#202547,#202548,#202549,#202550,#202551,#202552,#202553,#202554,#202555,
#202556,#202557,#202558,#202559,#202560,#202561,#202562,#202563,#202564,
#202565,#202566,#202567,#202568,#202569,#202570,#202571,#202572,#202573,
#202574,#202575,#202576,#202577,#202578,#202579,#202580,#202581,#202582,
#202583,#202584,#202585,#202586,#202587,#202588,#202589,#202590,#202591,
#202592,#202593,#202594,#202595,#202596,#202597,#202598,#202599,#202600,
#202601,#202602,#202603,#202604,#202605,#202606,#202607,#202608,#202609,
#202610,#202611,#202612,#202613,#202614,#202615,#202616,#202617,#202618,
#202619,#202620,#202621,#202622,#202623,#202624,#202625,#202626,#202627,
#202628,#202629,#202630,#202631,#202632,#202633,#202634,#202635,#202636,
#202637,#202638,#202639,#202640,#202641,#202642,#202643,#202644,#202645,
#202646,#202647,#202648,#202649,#202650,#202651,#202652,#202653,#202654,
#202655,#202656,#202657,#202658,#202659,#202660,#202661,#202662,#202663,
#202664,#202665,#202666,#202667,#202668,#202669,#202670,#202671,#202672,
#202673,#202674,#202675,#202676,#202677,#202678,#202679,#202680,#202681,
#202682,#202683,#202684,#202685,#202686,#202687,#202688,#202689,#202690,
#202691,#202692,#202693,#202694,#202695,#202696,#202697,#202698,#202699),
 .UNSPECIFIED.,.F.,.F.,(4,3,3,3,3,3,3,3,3,3,3,3,3,3,3,3,3,3,3,3,3,3,3,3,
3,3,3,3,3,3,3,3,3,3,3,3,3,3,3,3,3,3,3,3,3,3,3,3,3,3,3,3,3,3,3,3,3,3,3,3,
3,3,3,3,3,3,3,3,3,3,3,3,3,3,3,3,3,3,3,3,3,3,3,3,3,3,3,3,3,3,3,3,3,3,3,3,
3,3,3,3,3,3,3,3,3,3,3,3,3,4),(0.143172102,0.15412844,0.165137615,0.177981651,
0.188990826,0.201834862,0.212844037,0.225688073,0.236697248,0.247706422,
0.258715596,0.269724771,0.280733945,0.291743119,0.302752294,0.313761468,
0.324770642,0.335779817,0.346788991,0.357798165,0.368807339,0.379816514,
0.390825688,0.4,0.409174312,0.418348624,0.427522936,0.436697248,0.44587156,
0.455045872,0.464220183,0.473394495,0.482568807,0.491743119,0.500917431,
0.510091743,0.519266055,0.528440367,0.535779817,0.543119266,0.550458716,
0.557798165,0.565137615,0.572477064,0.579816514,0.587155963,0.594495413,
0.601834862,0.609174312,0.616513761,0.623853211,0.631192661,0.63853211,
0.64587156,0.653211009,0.660550459,0.667889908,0.675229358,0.682568807,
0.689908257,0.697247706,0.704587156,0.711926606,0.719266055,0.726605505,
0.733944954,0.741284404,0.748623853,0.755963303,0.763302752,0.772477064,
0.779816514,0.787155963,0.794495413,0.801834862,0.809174312,0.814678899,
0.820183486,0.825688073,0.831192661,0.836697248,0.842201835,0.849541284,
0.855045872,0.860550459,0.866055046,0.871559633,0.87706422,0.882568807,
0.888073394,0.893577982,0.899082569,0.904587156,0.910091743,0.91559633,
0.921100917,0.926605505,0.932110092,0.937614679,0.943119266,0.948623853,
0.95412844,0.959633028,0.965137615,0.970642202,0.976146789,0.981651376,
0.987155963,0.99266055,1.),.UNSPECIFIED.);
#24377=B_SPLINE_CURVE_WITH_KNOTS('',3,(#203647,#203648,#203649,#203650,
#203651,#203652,#203653,#203654,#203655,#203656,#203657,#203658,#203659,
#203660,#203661,#203662,#203663,#203664,#203665,#203666,#203667,#203668,
#203669,#203670,#203671,#203672,#203673,#203674,#203675,#203676,#203677,
#203678,#203679,#203680,#203681,#203682,#203683,#203684,#203685,#203686,
#203687,#203688,#203689,#203690,#203691,#203692,#203693,#203694,#203695,
#203696,#203697,#203698,#203699,#203700,#203701,#203702,#203703,#203704,
#203705,#203706,#203707,#203708,#203709,#203710,#203711,#203712,#203713,
#203714,#203715,#203716,#203717,#203718,#203719,#203720,#203721,#203722,
#203723,#203724,#203725,#203726,#203727,#203728,#203729,#203730,#203731,
#203732,#203733,#203734,#203735,#203736,#203737,#203738,#203739,#203740,
#203741,#203742,#203743,#203744,#203745,#203746,#203747,#203748,#203749,
#203750,#203751,#203752,#203753,#203754,#203755,#203756,#203757,#203758,
#203759,#203760,#203761,#203762,#203763,#203764,#203765,#203766,#203767,
#203768,#203769,#203770,#203771,#203772,#203773,#203774,#203775,#203776,
#203777,#203778,#203779,#203780,#203781,#203782,#203783,#203784,#203785,
#203786,#203787,#203788,#203789,#203790,#203791,#203792,#203793,#203794,
#203795,#203796,#203797,#203798,#203799,#203800,#203801,#203802,#203803,
#203804,#203805,#203806,#203807,#203808,#203809,#203810,#203811,#203812,
#203813,#203814,#203815,#203816,#203817,#203818,#203819,#203820,#203821,
#203822,#203823,#203824,#203825,#203826,#203827,#203828,#203829,#203830,
#203831,#203832,#203833,#203834,#203835,#203836,#203837,#203838,#203839,
#203840,#203841,#203842,#203843,#203844,#203845,#203846,#203847,#203848,
#203849,#203850,#203851,#203852,#203853,#203854,#203855,#203856,#203857,
#203858,#203859,#203860,#203861,#203862,#203863,#203864,#203865,#203866,
#203867,#203868,#203869,#203870,#203871,#203872,#203873,#203874,#203875,
#203876,#203877,#203878,#203879,#203880,#203881,#203882,#203883,#203884,
#203885,#203886,#203887,#203888,#203889,#203890,#203891,#203892,#203893,
#203894,#203895,#203896,#203897,#203898,#203899,#203900,#203901,#203902,
#203903,#203904,#203905,#203906,#203907,#203908,#203909,#203910,#203911,
#203912,#203913,#203914,#203915,#203916,#203917,#203918,#203919,#203920,
#203921,#203922,#203923,#203924,#203925,#203926,#203927,#203928,#203929,
#203930,#203931,#203932,#203933,#203934,#203935,#203936,#203937,#203938,
#203939,#203940,#203941,#203942,#203943,#203944,#203945,#203946,#203947,
#203948,#203949,#203950,#203951,#203952,#203953,#203954,#203955,#203956,
#203957,#203958,#203959,#203960,#203961,#203962,#203963,#203964,#203965,
#203966,#203967,#203968),.UNSPECIFIED.,.F.,.F.,(4,3,3,3,3,3,3,3,3,3,3,3,
3,3,3,3,3,3,3,3,3,3,3,3,3,3,3,3,3,3,3,3,3,3,3,3,3,3,3,3,3,3,3,3,3,3,3,3,
3,3,3,3,3,3,3,3,3,3,3,3,3,3,3,3,3,3,3,3,3,3,3,3,3,3,3,3,3,3,3,3,3,3,3,3,
3,3,3,3,3,3,3,3,3,3,3,3,3,3,3,3,3,3,3,3,3,3,3,4),(-1.,-0.994495413,-0.988990826,
-0.983486239,-0.977981651,-0.972477064,-0.966972477,-0.96146789,-0.955963303,
-0.950458716,-0.944954128,-0.937614679,-0.932110092,-0.926605505,-0.919266055,
-0.913761468,-0.908256881,-0.900917431,-0.895412844,-0.889908257,-0.88440367,
-0.878899083,-0.873394495,-0.867889908,-0.860550459,-0.855045872,-0.849541284,
-0.844036697,-0.83853211,-0.833027523,-0.827522936,-0.822018349,-0.814678899,
-0.809174312,-0.801834862,-0.794495413,-0.787155963,-0.779816514,-0.770642202,
-0.763302752,-0.755963303,-0.748623853,-0.741284404,-0.733944954,-0.726605505,
-0.719266055,-0.710091743,-0.702752294,-0.695412844,-0.688073394,-0.675229358,
-0.667889908,-0.660550459,-0.653211009,-0.64587156,-0.63853211,-0.631192661,
-0.623853211,-0.616513761,-0.609174312,-0.601834862,-0.594495413,-0.587155963,
-0.579816514,-0.572477064,-0.565137615,-0.557798165,-0.550458716,-0.543119266,
-0.535779817,-0.528440367,-0.519266055,-0.510091743,-0.500917431,-0.491743119,
-0.482568807,-0.473394495,-0.464220183,-0.455045872,-0.44587156,-0.436697248,
-0.427522936,-0.418348624,-0.409174312,-0.4,-0.390825688,-0.379816514,-0.368807339,
-0.357798165,-0.346788991,-0.335779817,-0.324770642,-0.313761468,-0.302752294,
-0.291743119,-0.280733945,-0.269724771,-0.258715596,-0.247706422,-0.236697248,
-0.225688073,-0.212844037,-0.201834862,-0.188990826,-0.177981651,-0.165137615,
-0.15412844,-0.143172102),.UNSPECIFIED.);
#24378=B_SPLINE_CURVE_WITH_KNOTS('',3,(#203969,#203970,#203971,#203972,
#203973,#203974,#203975,#203976,#203977,#203978,#203979,#203980,#203981,
#203982,#203983,#203984,#203985,#203986,#203987,#203988,#203989,#203990,
#203991,#203992,#203993,#203994,#203995,#203996,#203997,#203998,#203999,
#204000,#204001,#204002,#204003,#204004,#204005,#204006,#204007,#204008,
#204009,#204010,#204011,#204012,#204013,#204014,#204015,#204016,#204017,
#204018,#204019,#204020,#204021,#204022,#204023,#204024,#204025,#204026,
#204027,#204028,#204029,#204030,#204031,#204032,#204033,#204034,#204035,
#204036,#204037,#204038,#204039,#204040,#204041,#204042,#204043,#204044,
#204045,#204046,#204047,#204048,#204049,#204050,#204051,#204052,#204053,
#204054,#204055,#204056,#204057,#204058,#204059,#204060,#204061,#204062,
#204063,#204064,#204065,#204066,#204067,#204068,#204069,#204070,#204071,
#204072,#204073,#204074,#204075,#204076,#204077,#204078,#204079,#204080,
#204081,#204082,#204083,#204084,#204085,#204086,#204087,#204088,#204089,
#204090,#204091,#204092,#204093,#204094,#204095,#204096,#204097,#204098,
#204099,#204100,#204101,#204102,#204103,#204104,#204105,#204106,#204107,
#204108,#204109,#204110,#204111,#204112,#204113,#204114,#204115,#204116,
#204117,#204118,#204119,#204120,#204121,#204122,#204123,#204124,#204125,
#204126,#204127,#204128,#204129,#204130,#204131,#204132,#204133,#204134,
#204135,#204136,#204137,#204138,#204139,#204140,#204141,#204142,#204143,
#204144,#204145,#204146,#204147,#204148,#204149,#204150,#204151,#204152,
#204153,#204154,#204155,#204156,#204157,#204158,#204159,#204160,#204161,
#204162,#204163,#204164,#204165,#204166,#204167,#204168,#204169,#204170,
#204171,#204172,#204173,#204174,#204175,#204176,#204177,#204178,#204179,
#204180,#204181,#204182,#204183,#204184,#204185,#204186,#204187,#204188,
#204189,#204190,#204191,#204192,#204193,#204194,#204195,#204196,#204197,
#204198,#204199,#204200,#204201,#204202,#204203,#204204,#204205,#204206,
#204207,#204208,#204209,#204210,#204211,#204212,#204213,#204214,#204215,
#204216,#204217,#204218,#204219,#204220,#204221,#204222,#204223,#204224,
#204225,#204226,#204227,#204228,#204229,#204230,#204231,#204232,#204233,
#204234,#204235,#204236,#204237,#204238,#204239,#204240,#204241,#204242,
#204243,#204244,#204245,#204246,#204247,#204248,#204249,#204250,#204251,
#204252,#204253,#204254,#204255,#204256,#204257,#204258,#204259,#204260,
#204261,#204262,#204263,#204264,#204265,#204266,#204267,#204268,#204269,
#204270,#204271,#204272,#204273,#204274,#204275,#204276,#204277,#204278),
 .UNSPECIFIED.,.F.,.F.,(4,3,3,3,3,3,3,3,3,3,3,3,3,3,3,3,3,3,3,3,3,3,3,3,
3,3,3,3,3,3,3,3,3,3,3,3,3,3,3,3,3,3,3,3,3,3,3,3,3,3,3,3,3,3,3,3,3,3,3,3,
3,3,3,3,3,3,3,3,3,3,3,3,3,3,3,3,3,3,3,3,3,3,3,3,3,3,3,3,3,3,3,3,3,3,3,3,
3,3,3,3,3,3,3,4),(0.143172102,0.15412844,0.165137615,0.176146789,0.187155963,
0.198165138,0.209174312,0.222018349,0.233027523,0.244036697,0.255045872,
0.266055046,0.27706422,0.288073394,0.299082569,0.311926606,0.32293578,0.333944954,
0.344954128,0.355963303,0.368807339,0.379816514,0.390825688,0.4,0.409174312,
0.418348624,0.427522936,0.436697248,0.44587156,0.455045872,0.466055046,
0.475229358,0.48440367,0.493577982,0.502752294,0.513761468,0.52293578,0.532110092,
0.539449541,0.546788991,0.55412844,0.56146789,0.568807339,0.577981651,0.585321101,
0.59266055,0.601834862,0.609174312,0.616513761,0.623853211,0.631192661,
0.63853211,0.64587156,0.653211009,0.660550459,0.667889908,0.675229358,0.682568807,
0.689908257,0.697247706,0.704587156,0.713761468,0.721100917,0.730275229,
0.743119266,0.75412844,0.76146789,0.770642202,0.777981651,0.785321101,0.79266055,
0.801834862,0.811009174,0.818348624,0.825688073,0.834862385,0.840366972,
0.84587156,0.853211009,0.858715596,0.864220183,0.869724771,0.875229358,
0.880733945,0.888073394,0.893577982,0.899082569,0.906422018,0.911926606,
0.917431193,0.924770642,0.930275229,0.937614679,0.943119266,0.948623853,
0.95412844,0.96146789,0.966972477,0.972477064,0.977981651,0.983486239,0.988990826,
0.994495413,1.),.UNSPECIFIED.);
#24379=B_SPLINE_CURVE_WITH_KNOTS('',3,(#205241,#205242,#205243,#205244,
#205245,#205246,#205247,#205248,#205249,#205250,#205251,#205252,#205253,
#205254,#205255,#205256,#205257,#205258,#205259,#205260,#205261,#205262,
#205263,#205264,#205265,#205266,#205267,#205268,#205269,#205270,#205271,
#205272,#205273,#205274,#205275,#205276,#205277,#205278,#205279,#205280,
#205281,#205282,#205283,#205284,#205285,#205286,#205287,#205288,#205289,
#205290,#205291,#205292,#205293,#205294,#205295,#205296,#205297,#205298,
#205299,#205300,#205301,#205302,#205303,#205304,#205305,#205306,#205307,
#205308,#205309,#205310,#205311,#205312,#205313,#205314,#205315,#205316,
#205317,#205318,#205319,#205320,#205321,#205322,#205323,#205324,#205325,
#205326,#205327,#205328,#205329,#205330,#205331,#205332,#205333,#205334,
#205335,#205336,#205337,#205338,#205339,#205340,#205341,#205342,#205343,
#205344,#205345,#205346,#205347,#205348,#205349,#205350,#205351,#205352,
#205353,#205354,#205355,#205356,#205357,#205358,#205359,#205360,#205361,
#205362,#205363,#205364,#205365,#205366,#205367,#205368,#205369,#205370,
#205371,#205372,#205373,#205374,#205375,#205376,#205377,#205378,#205379,
#205380,#205381,#205382,#205383,#205384,#205385,#205386,#205387,#205388,
#205389,#205390,#205391,#205392,#205393,#205394,#205395,#205396,#205397,
#205398,#205399,#205400,#205401,#205402,#205403,#205404,#205405,#205406,
#205407,#205408,#205409,#205410,#205411,#205412,#205413,#205414,#205415,
#205416,#205417,#205418,#205419,#205420,#205421,#205422,#205423,#205424,
#205425,#205426,#205427,#205428,#205429,#205430,#205431,#205432,#205433,
#205434,#205435,#205436,#205437,#205438,#205439,#205440,#205441,#205442,
#205443,#205444,#205445,#205446,#205447,#205448,#205449,#205450,#205451,
#205452,#205453,#205454,#205455,#205456,#205457,#205458,#205459,#205460,
#205461,#205462,#205463,#205464,#205465,#205466,#205467,#205468,#205469,
#205470,#205471,#205472,#205473,#205474,#205475,#205476,#205477,#205478,
#205479,#205480,#205481,#205482,#205483,#205484,#205485,#205486,#205487,
#205488,#205489,#205490,#205491,#205492,#205493,#205494,#205495,#205496,
#205497,#205498,#205499,#205500,#205501,#205502,#205503,#205504,#205505,
#205506,#205507,#205508,#205509,#205510,#205511,#205512,#205513,#205514,
#205515,#205516,#205517,#205518,#205519,#205520,#205521,#205522,#205523,
#205524,#205525,#205526,#205527,#205528,#205529,#205530,#205531,#205532,
#205533,#205534,#205535,#205536,#205537,#205538,#205539,#205540,#205541,
#205542,#205543,#205544,#205545,#205546,#205547,#205548,#205549,#205550,
#205551,#205552,#205553,#205554,#205555,#205556,#205557,#205558,#205559,
#205560,#205561,#205562,#205563,#205564,#205565),.UNSPECIFIED.,.F.,.F.,
(4,3,3,3,3,3,3,3,3,3,3,3,3,3,3,3,3,3,3,3,3,3,3,3,3,3,3,3,3,3,3,3,3,3,3,
3,3,3,3,3,3,3,3,3,3,3,3,3,3,3,3,3,3,3,3,3,3,3,3,3,3,3,3,3,3,3,3,3,3,3,3,
3,3,3,3,3,3,3,3,3,3,3,3,3,3,3,3,3,3,3,3,3,3,3,3,3,3,3,3,3,3,3,3,3,3,3,3,
3,4),(-1.,-0.994495413,-0.988990826,-0.983486239,-0.977981651,-0.970642202,
-0.965137615,-0.959633028,-0.95412844,-0.948623853,-0.943119266,-0.937614679,
-0.932110092,-0.926605505,-0.921100917,-0.91559633,-0.910091743,-0.904587156,
-0.899082569,-0.893577982,-0.888073394,-0.882568807,-0.87706422,-0.871559633,
-0.866055046,-0.860550459,-0.855045872,-0.849541284,-0.844036697,-0.83853211,
-0.833027523,-0.827522936,-0.822018349,-0.814678899,-0.809174312,-0.801834862,
-0.794495413,-0.787155963,-0.779816514,-0.772477064,-0.765137615,-0.757798165,
-0.750458716,-0.743119266,-0.735779817,-0.728440367,-0.721100917,-0.710091743,
-0.702752294,-0.695412844,-0.688073394,-0.678899083,-0.671559633,-0.664220183,
-0.656880734,-0.649541284,-0.642201835,-0.634862385,-0.627522936,-0.620183486,
-0.612844037,-0.605504587,-0.598165138,-0.590825688,-0.583486239,-0.576146789,
-0.568807339,-0.559633028,-0.552293578,-0.544954128,-0.537614679,-0.530275229,
-0.521100917,-0.511926606,-0.502752294,-0.493577982,-0.482568807,-0.473394495,
-0.464220183,-0.455045872,-0.44587156,-0.436697248,-0.427522936,-0.418348624,
-0.409174312,-0.4,-0.390825688,-0.379816514,-0.368807339,-0.357798165,-0.346788991,
-0.335779817,-0.324770642,-0.311926606,-0.300917431,-0.289908257,-0.278899083,
-0.267889908,-0.255045872,-0.244036697,-0.233027523,-0.222018349,-0.211009174,
-0.2,-0.188990826,-0.177981651,-0.166972477,-0.155963303,-0.143172102),
 .UNSPECIFIED.);
#24380=B_SPLINE_CURVE_WITH_KNOTS('',3,(#205566,#205567,#205568,#205569,
#205570,#205571,#205572,#205573,#205574,#205575,#205576,#205577,#205578,
#205579,#205580,#205581,#205582,#205583,#205584,#205585,#205586,#205587,
#205588,#205589,#205590,#205591,#205592,#205593,#205594,#205595,#205596,
#205597,#205598,#205599,#205600,#205601,#205602,#205603,#205604,#205605,
#205606,#205607,#205608,#205609,#205610,#205611,#205612,#205613,#205614,
#205615,#205616,#205617,#205618,#205619,#205620,#205621,#205622,#205623,
#205624,#205625,#205626,#205627,#205628,#205629,#205630,#205631,#205632,
#205633,#205634,#205635,#205636,#205637,#205638,#205639,#205640,#205641,
#205642,#205643,#205644,#205645,#205646,#205647,#205648,#205649,#205650,
#205651,#205652,#205653,#205654,#205655,#205656,#205657,#205658,#205659,
#205660,#205661,#205662,#205663,#205664,#205665,#205666,#205667,#205668,
#205669,#205670,#205671,#205672,#205673,#205674,#205675,#205676,#205677,
#205678,#205679,#205680,#205681,#205682,#205683,#205684,#205685,#205686,
#205687,#205688,#205689,#205690,#205691,#205692,#205693,#205694,#205695,
#205696,#205697,#205698,#205699,#205700,#205701,#205702,#205703,#205704,
#205705,#205706,#205707,#205708,#205709,#205710,#205711,#205712,#205713,
#205714,#205715,#205716,#205717,#205718,#205719,#205720,#205721,#205722,
#205723,#205724,#205725,#205726,#205727,#205728,#205729,#205730,#205731,
#205732,#205733,#205734,#205735,#205736,#205737,#205738,#205739,#205740,
#205741,#205742,#205743,#205744,#205745,#205746,#205747,#205748,#205749,
#205750,#205751,#205752,#205753,#205754,#205755,#205756,#205757,#205758,
#205759,#205760,#205761,#205762,#205763,#205764,#205765,#205766,#205767,
#205768,#205769,#205770,#205771,#205772,#205773,#205774,#205775,#205776,
#205777,#205778,#205779,#205780,#205781,#205782,#205783,#205784,#205785,
#205786,#205787,#205788,#205789,#205790,#205791,#205792,#205793,#205794,
#205795,#205796,#205797,#205798,#205799,#205800,#205801,#205802,#205803,
#205804,#205805,#205806,#205807,#205808,#205809,#205810,#205811,#205812,
#205813,#205814,#205815,#205816,#205817,#205818,#205819,#205820,#205821,
#205822,#205823,#205824,#205825,#205826,#205827,#205828,#205829,#205830,
#205831,#205832,#205833,#205834,#205835,#205836,#205837,#205838,#205839,
#205840,#205841,#205842,#205843,#205844,#205845,#205846,#205847,#205848,
#205849,#205850,#205851,#205852,#205853,#205854,#205855,#205856,#205857,
#205858,#205859,#205860,#205861,#205862,#205863,#205864,#205865,#205866),
 .UNSPECIFIED.,.F.,.F.,(4,3,3,3,3,3,3,3,3,3,3,3,3,3,3,3,3,3,3,3,3,3,3,3,
3,3,3,3,3,3,3,3,3,3,3,3,3,3,3,3,3,3,3,3,3,3,3,3,3,3,3,3,3,3,3,3,3,3,3,3,
3,3,3,3,3,3,3,3,3,3,3,3,3,3,3,3,3,3,3,3,3,3,3,3,3,3,3,3,3,3,3,3,3,3,3,3,
3,3,3,3,4),(0.143172102,0.15412844,0.165137615,0.176146789,0.187155963,
0.198165138,0.209174312,0.220183486,0.231192661,0.242201835,0.253211009,
0.266055046,0.27706422,0.288073394,0.299082569,0.310091743,0.321100917,
0.333944954,0.344954128,0.355963303,0.366972477,0.377981651,0.388990826,
0.398165138,0.409174312,0.420183486,0.433027523,0.442201835,0.451376147,
0.460550459,0.471559633,0.482568807,0.491743119,0.500917431,0.513761468,
0.524770642,0.533944954,0.541284404,0.548623853,0.557798165,0.565137615,
0.572477064,0.579816514,0.590825688,0.6,0.611009174,0.618348624,0.625688073,
0.633027523,0.640366972,0.649541284,0.656880734,0.664220183,0.671559633,
0.678899083,0.686238532,0.693577982,0.700917431,0.708256881,0.71559633,
0.72293578,0.732110092,0.739449541,0.748623853,0.757798165,0.765137615,
0.772477064,0.781651376,0.788990826,0.798165138,0.80733945,0.812844037,
0.822018349,0.829357798,0.836697248,0.844036697,0.849541284,0.855045872,
0.860550459,0.866055046,0.871559633,0.87706422,0.882568807,0.889908257,
0.895412844,0.904587156,0.910091743,0.91559633,0.921100917,0.926605505,
0.932110092,0.937614679,0.944954128,0.950458716,0.957798165,0.966972477,
0.972477064,0.977981651,0.983486239,0.99266055,1.),.UNSPECIFIED.);
#24381=B_SPLINE_CURVE_WITH_KNOTS('',3,(#206811,#206812,#206813,#206814,
#206815,#206816,#206817,#206818,#206819,#206820,#206821,#206822,#206823,
#206824,#206825,#206826,#206827,#206828,#206829,#206830,#206831,#206832,
#206833,#206834,#206835,#206836,#206837,#206838,#206839,#206840,#206841,
#206842,#206843,#206844,#206845,#206846,#206847,#206848,#206849,#206850,
#206851,#206852,#206853,#206854,#206855,#206856,#206857,#206858,#206859,
#206860,#206861,#206862,#206863,#206864,#206865,#206866,#206867,#206868,
#206869,#206870,#206871,#206872,#206873,#206874,#206875,#206876,#206877,
#206878,#206879,#206880,#206881,#206882,#206883,#206884,#206885,#206886,
#206887,#206888,#206889,#206890,#206891,#206892,#206893,#206894,#206895,
#206896,#206897,#206898,#206899,#206900,#206901,#206902,#206903,#206904,
#206905,#206906,#206907,#206908,#206909,#206910,#206911,#206912,#206913,
#206914,#206915,#206916,#206917,#206918,#206919,#206920,#206921,#206922,
#206923,#206924,#206925,#206926,#206927,#206928,#206929,#206930,#206931,
#206932,#206933,#206934,#206935,#206936,#206937,#206938,#206939,#206940,
#206941,#206942,#206943,#206944,#206945,#206946,#206947,#206948,#206949,
#206950,#206951,#206952,#206953,#206954,#206955,#206956,#206957,#206958,
#206959,#206960,#206961,#206962,#206963,#206964,#206965,#206966,#206967,
#206968,#206969,#206970,#206971,#206972,#206973,#206974,#206975,#206976,
#206977,#206978,#206979,#206980,#206981,#206982,#206983,#206984,#206985,
#206986,#206987,#206988,#206989,#206990,#206991,#206992,#206993,#206994,
#206995,#206996,#206997,#206998,#206999,#207000,#207001,#207002,#207003,
#207004,#207005,#207006,#207007,#207008,#207009,#207010,#207011,#207012,
#207013,#207014,#207015,#207016,#207017,#207018,#207019,#207020,#207021,
#207022,#207023,#207024,#207025,#207026,#207027,#207028,#207029,#207030,
#207031,#207032,#207033,#207034,#207035,#207036,#207037,#207038,#207039,
#207040,#207041,#207042,#207043,#207044,#207045,#207046,#207047,#207048,
#207049,#207050,#207051,#207052,#207053,#207054,#207055,#207056,#207057,
#207058,#207059,#207060,#207061,#207062,#207063,#207064,#207065,#207066,
#207067,#207068,#207069,#207070,#207071,#207072,#207073,#207074,#207075,
#207076,#207077,#207078,#207079,#207080,#207081,#207082,#207083,#207084,
#207085,#207086,#207087,#207088,#207089,#207090,#207091,#207092,#207093,
#207094,#207095,#207096,#207097,#207098,#207099,#207100,#207101,#207102,
#207103,#207104,#207105,#207106,#207107,#207108,#207109,#207110,#207111),
 .UNSPECIFIED.,.F.,.F.,(4,3,3,3,3,3,3,3,3,3,3,3,3,3,3,3,3,3,3,3,3,3,3,3,
3,3,3,3,3,3,3,3,3,3,3,3,3,3,3,3,3,3,3,3,3,3,3,3,3,3,3,3,3,3,3,3,3,3,3,3,
3,3,3,3,3,3,3,3,3,3,3,3,3,3,3,3,3,3,3,3,3,3,3,3,3,3,3,3,3,3,3,3,3,3,3,3,
3,3,3,3,4),(0.143172102,0.15412844,0.165137615,0.176146789,0.187155963,
0.198165138,0.211009174,0.222018349,0.233027523,0.244036697,0.255045872,
0.266055046,0.27706422,0.288073394,0.299082569,0.310091743,0.321100917,
0.332110092,0.344954128,0.355963303,0.366972477,0.377981651,0.388990826,
0.398165138,0.40733945,0.418348624,0.427522936,0.436697248,0.44587156,0.455045872,
0.464220183,0.475229358,0.48440367,0.495412844,0.504587156,0.51559633,0.524770642,
0.533944954,0.541284404,0.548623853,0.557798165,0.565137615,0.572477064,
0.579816514,0.587155963,0.594495413,0.601834862,0.609174312,0.616513761,
0.623853211,0.631192661,0.644036697,0.651376147,0.658715596,0.667889908,
0.675229358,0.682568807,0.689908257,0.700917431,0.710091743,0.717431193,
0.724770642,0.735779817,0.743119266,0.750458716,0.757798165,0.766972477,
0.774311927,0.781651376,0.788990826,0.796330275,0.803669725,0.811009174,
0.818348624,0.825688073,0.831192661,0.83853211,0.844036697,0.849541284,
0.858715596,0.864220183,0.871559633,0.87706422,0.88440367,0.889908257,0.895412844,
0.900917431,0.908256881,0.913761468,0.919266055,0.924770642,0.932110092,
0.939449541,0.948623853,0.95412844,0.959633028,0.966972477,0.972477064,
0.981651376,0.990825688,1.),.UNSPECIFIED.);
#24382=B_SPLINE_CURVE_WITH_KNOTS('',3,(#207112,#207113,#207114,#207115,
#207116,#207117,#207118,#207119,#207120,#207121,#207122,#207123,#207124,
#207125,#207126,#207127,#207128,#207129,#207130,#207131,#207132,#207133,
#207134,#207135,#207136,#207137,#207138,#207139,#207140,#207141,#207142,
#207143,#207144,#207145,#207146,#207147,#207148,#207149,#207150,#207151,
#207152,#207153,#207154,#207155,#207156,#207157,#207158,#207159,#207160,
#207161,#207162,#207163,#207164,#207165,#207166,#207167,#207168,#207169,
#207170,#207171,#207172,#207173,#207174,#207175,#207176,#207177,#207178,
#207179,#207180,#207181,#207182,#207183,#207184,#207185,#207186,#207187,
#207188,#207189,#207190,#207191,#207192,#207193,#207194,#207195,#207196,
#207197,#207198,#207199,#207200,#207201,#207202,#207203,#207204,#207205,
#207206,#207207,#207208,#207209,#207210,#207211,#207212,#207213,#207214,
#207215,#207216,#207217,#207218,#207219,#207220,#207221,#207222,#207223,
#207224,#207225,#207226,#207227,#207228,#207229,#207230,#207231,#207232,
#207233,#207234,#207235,#207236,#207237,#207238,#207239,#207240,#207241,
#207242,#207243,#207244,#207245,#207246,#207247,#207248,#207249,#207250,
#207251,#207252,#207253,#207254,#207255,#207256,#207257,#207258,#207259,
#207260,#207261,#207262,#207263,#207264,#207265,#207266,#207267,#207268,
#207269,#207270,#207271,#207272,#207273,#207274,#207275,#207276,#207277,
#207278,#207279,#207280,#207281,#207282,#207283,#207284,#207285,#207286,
#207287,#207288,#207289,#207290,#207291,#207292,#207293,#207294,#207295,
#207296,#207297,#207298,#207299,#207300,#207301,#207302,#207303,#207304,
#207305,#207306,#207307,#207308,#207309,#207310,#207311,#207312,#207313,
#207314,#207315,#207316,#207317,#207318,#207319,#207320,#207321,#207322,
#207323,#207324,#207325,#207326,#207327,#207328,#207329,#207330,#207331,
#207332,#207333,#207334,#207335,#207336,#207337,#207338,#207339,#207340,
#207341,#207342,#207343,#207344,#207345,#207346,#207347,#207348,#207349,
#207350,#207351,#207352,#207353,#207354,#207355,#207356,#207357,#207358,
#207359,#207360,#207361,#207362,#207363,#207364,#207365,#207366,#207367,
#207368,#207369,#207370,#207371,#207372,#207373,#207374,#207375,#207376,
#207377,#207378,#207379,#207380,#207381,#207382,#207383,#207384,#207385,
#207386,#207387,#207388,#207389,#207390,#207391,#207392,#207393,#207394,
#207395,#207396,#207397,#207398,#207399,#207400,#207401,#207402,#207403,
#207404,#207405,#207406,#207407,#207408,#207409,#207410,#207411,#207412,
#207413,#207414,#207415,#207416,#207417,#207418,#207419,#207420,#207421,
#207422,#207423,#207424,#207425,#207426,#207427,#207428,#207429,#207430),
 .UNSPECIFIED.,.F.,.F.,(4,3,3,3,3,3,3,3,3,3,3,3,3,3,3,3,3,3,3,3,3,3,3,3,
3,3,3,3,3,3,3,3,3,3,3,3,3,3,3,3,3,3,3,3,3,3,3,3,3,3,3,3,3,3,3,3,3,3,3,3,
3,3,3,3,3,3,3,3,3,3,3,3,3,3,3,3,3,3,3,3,3,3,3,3,3,3,3,3,3,3,3,3,3,3,3,3,
3,3,3,3,3,3,3,3,3,3,4),(0.143172102,0.15412844,0.165137615,0.176146789,
0.187155963,0.198165138,0.211009174,0.222018349,0.233027523,0.244036697,
0.255045872,0.266055046,0.27706422,0.288073394,0.299082569,0.310091743,
0.321100917,0.332110092,0.344954128,0.355963303,0.366972477,0.377981651,
0.388990826,0.398165138,0.40733945,0.418348624,0.427522936,0.436697248,
0.44587156,0.455045872,0.464220183,0.473394495,0.48440367,0.493577982,0.502752294,
0.511926606,0.521100917,0.530275229,0.537614679,0.544954128,0.552293578,
0.559633028,0.566972477,0.574311927,0.581651376,0.588990826,0.596330275,
0.603669725,0.611009174,0.618348624,0.625688073,0.633027523,0.640366972,
0.647706422,0.655045872,0.664220183,0.671559633,0.678899083,0.686238532,
0.693577982,0.700917431,0.710091743,0.717431193,0.724770642,0.733944954,
0.741284404,0.748623853,0.755963303,0.763302752,0.772477064,0.779816514,
0.787155963,0.794495413,0.803669725,0.811009174,0.816513761,0.822018349,
0.827522936,0.834862385,0.840366972,0.84587156,0.851376147,0.856880734,
0.862385321,0.867889908,0.873394495,0.878899083,0.88440367,0.889908257,
0.895412844,0.900917431,0.906422018,0.911926606,0.917431193,0.924770642,
0.930275229,0.937614679,0.943119266,0.948623853,0.95412844,0.959633028,
0.966972477,0.972477064,0.977981651,0.983486239,0.990825688,1.),
 .UNSPECIFIED.);
#24383=B_SPLINE_CURVE_WITH_KNOTS('',3,(#208390,#208391,#208392,#208393,
#208394,#208395,#208396,#208397,#208398,#208399,#208400,#208401,#208402,
#208403,#208404,#208405,#208406,#208407,#208408,#208409,#208410,#208411,
#208412,#208413,#208414,#208415,#208416,#208417,#208418,#208419,#208420,
#208421,#208422,#208423,#208424,#208425,#208426,#208427,#208428,#208429,
#208430,#208431,#208432,#208433,#208434,#208435,#208436,#208437,#208438,
#208439,#208440,#208441,#208442,#208443,#208444,#208445,#208446,#208447,
#208448,#208449,#208450,#208451,#208452,#208453,#208454,#208455,#208456,
#208457,#208458,#208459,#208460,#208461,#208462,#208463,#208464,#208465,
#208466,#208467,#208468,#208469,#208470,#208471,#208472,#208473,#208474,
#208475,#208476,#208477,#208478,#208479,#208480,#208481,#208482,#208483,
#208484,#208485,#208486,#208487,#208488,#208489,#208490,#208491,#208492,
#208493,#208494,#208495,#208496,#208497,#208498,#208499,#208500,#208501,
#208502,#208503,#208504,#208505,#208506,#208507,#208508,#208509,#208510,
#208511,#208512,#208513,#208514,#208515,#208516,#208517,#208518,#208519,
#208520,#208521,#208522,#208523,#208524,#208525,#208526,#208527,#208528,
#208529,#208530,#208531,#208532,#208533,#208534,#208535,#208536,#208537,
#208538,#208539,#208540,#208541,#208542,#208543,#208544,#208545,#208546,
#208547,#208548,#208549,#208550,#208551,#208552,#208553,#208554,#208555,
#208556,#208557,#208558,#208559,#208560,#208561,#208562,#208563,#208564,
#208565,#208566,#208567,#208568,#208569,#208570,#208571,#208572,#208573,
#208574,#208575,#208576,#208577,#208578,#208579,#208580,#208581,#208582,
#208583,#208584,#208585,#208586,#208587,#208588,#208589,#208590,#208591,
#208592,#208593,#208594,#208595,#208596,#208597,#208598,#208599,#208600,
#208601,#208602,#208603,#208604,#208605,#208606,#208607,#208608,#208609,
#208610,#208611,#208612,#208613,#208614,#208615,#208616,#208617,#208618,
#208619,#208620,#208621,#208622,#208623,#208624,#208625,#208626,#208627,
#208628,#208629,#208630,#208631,#208632,#208633,#208634,#208635,#208636,
#208637,#208638,#208639,#208640,#208641,#208642,#208643,#208644,#208645,
#208646,#208647,#208648,#208649,#208650,#208651,#208652,#208653,#208654,
#208655,#208656,#208657,#208658,#208659,#208660,#208661,#208662,#208663,
#208664,#208665,#208666,#208667,#208668,#208669,#208670,#208671,#208672,
#208673,#208674,#208675,#208676,#208677,#208678,#208679,#208680,#208681,
#208682,#208683,#208684,#208685,#208686,#208687,#208688,#208689,#208690,
#208691,#208692,#208693,#208694,#208695,#208696,#208697,#208698,#208699,
#208700,#208701,#208702),.UNSPECIFIED.,.F.,.F.,(4,3,3,3,3,3,3,3,3,3,3,3,
3,3,3,3,3,3,3,3,3,3,3,3,3,3,3,3,3,3,3,3,3,3,3,3,3,3,3,3,3,3,3,3,3,3,3,3,
3,3,3,3,3,3,3,3,3,3,3,3,3,3,3,3,3,3,3,3,3,3,3,3,3,3,3,3,3,3,3,3,3,3,3,3,
3,3,3,3,3,3,3,3,3,3,3,3,3,3,3,3,3,3,3,3,4),(0.143172102,0.15412844,0.165137615,
0.176146789,0.187155963,0.198165138,0.211009174,0.222018349,0.233027523,
0.244036697,0.255045872,0.266055046,0.27706422,0.288073394,0.299082569,
0.310091743,0.321100917,0.332110092,0.343119266,0.35412844,0.365137615,
0.376146789,0.387155963,0.396330275,0.405504587,0.414678899,0.425688073,
0.434862385,0.44587156,0.455045872,0.464220183,0.473394495,0.482568807,
0.491743119,0.500917431,0.511926606,0.521100917,0.530275229,0.537614679,
0.548623853,0.557798165,0.565137615,0.572477064,0.579816514,0.587155963,
0.596330275,0.603669725,0.611009174,0.620183486,0.627522936,0.634862385,
0.642201835,0.649541284,0.656880734,0.664220183,0.673394495,0.680733945,
0.688073394,0.697247706,0.704587156,0.713761468,0.721100917,0.728440367,
0.735779817,0.746788991,0.755963303,0.765137615,0.772477064,0.779816514,
0.790825688,0.798165138,0.805504587,0.811009174,0.818348624,0.823853211,
0.829357798,0.836697248,0.842201835,0.847706422,0.856880734,0.862385321,
0.867889908,0.873394495,0.878899083,0.88440367,0.889908257,0.895412844,
0.902752294,0.908256881,0.913761468,0.921100917,0.926605505,0.932110092,
0.937614679,0.943119266,0.948623853,0.95412844,0.959633028,0.965137615,
0.970642202,0.976146789,0.981651376,0.987155963,0.99266055,1.),
 .UNSPECIFIED.);
#24384=B_SPLINE_CURVE_WITH_KNOTS('',3,(#208703,#208704,#208705,#208706,
#208707,#208708,#208709,#208710,#208711,#208712,#208713,#208714,#208715,
#208716,#208717,#208718,#208719,#208720,#208721,#208722,#208723,#208724,
#208725,#208726,#208727,#208728,#208729,#208730,#208731,#208732,#208733,
#208734,#208735,#208736,#208737,#208738,#208739,#208740,#208741,#208742,
#208743,#208744,#208745,#208746,#208747,#208748,#208749,#208750,#208751,
#208752,#208753,#208754,#208755,#208756,#208757,#208758,#208759,#208760,
#208761,#208762,#208763,#208764,#208765,#208766,#208767,#208768,#208769,
#208770,#208771,#208772,#208773,#208774,#208775,#208776,#208777,#208778,
#208779,#208780,#208781,#208782,#208783,#208784,#208785,#208786,#208787,
#208788,#208789,#208790,#208791,#208792,#208793,#208794,#208795,#208796,
#208797,#208798,#208799,#208800,#208801,#208802,#208803,#208804,#208805,
#208806,#208807,#208808,#208809,#208810,#208811,#208812,#208813,#208814,
#208815,#208816,#208817,#208818,#208819,#208820,#208821,#208822,#208823,
#208824,#208825,#208826,#208827,#208828,#208829,#208830,#208831,#208832,
#208833,#208834,#208835,#208836,#208837,#208838,#208839,#208840,#208841,
#208842,#208843,#208844,#208845,#208846,#208847,#208848,#208849,#208850,
#208851,#208852,#208853,#208854,#208855,#208856,#208857,#208858,#208859,
#208860,#208861,#208862,#208863,#208864,#208865,#208866,#208867,#208868,
#208869,#208870,#208871,#208872,#208873,#208874,#208875,#208876,#208877,
#208878,#208879,#208880,#208881,#208882,#208883,#208884,#208885,#208886,
#208887,#208888,#208889,#208890,#208891,#208892,#208893,#208894,#208895,
#208896,#208897,#208898,#208899,#208900,#208901,#208902,#208903,#208904,
#208905,#208906,#208907,#208908,#208909,#208910,#208911,#208912,#208913,
#208914,#208915,#208916,#208917,#208918,#208919,#208920,#208921,#208922,
#208923,#208924,#208925,#208926,#208927,#208928,#208929,#208930,#208931,
#208932,#208933,#208934,#208935,#208936,#208937,#208938,#208939,#208940,
#208941,#208942,#208943,#208944,#208945,#208946,#208947,#208948,#208949,
#208950,#208951,#208952,#208953,#208954,#208955,#208956,#208957,#208958,
#208959,#208960,#208961,#208962,#208963,#208964,#208965,#208966,#208967,
#208968,#208969,#208970,#208971,#208972,#208973,#208974,#208975,#208976,
#208977,#208978,#208979,#208980,#208981,#208982,#208983,#208984,#208985,
#208986,#208987,#208988,#208989,#208990,#208991,#208992,#208993,#208994,
#208995,#208996,#208997,#208998,#208999,#209000,#209001,#209002,#209003,
#209004,#209005,#209006,#209007,#209008,#209009,#209010,#209011,#209012,
#209013,#209014,#209015,#209016,#209017,#209018,#209019,#209020,#209021,
#209022,#209023,#209024,#209025,#209026,#209027),.UNSPECIFIED.,.F.,.F.,
(4,3,3,3,3,3,3,3,3,3,3,3,3,3,3,3,3,3,3,3,3,3,3,3,3,3,3,3,3,3,3,3,3,3,3,
3,3,3,3,3,3,3,3,3,3,3,3,3,3,3,3,3,3,3,3,3,3,3,3,3,3,3,3,3,3,3,3,3,3,3,3,
3,3,3,3,3,3,3,3,3,3,3,3,3,3,3,3,3,3,3,3,3,3,3,3,3,3,3,3,3,3,3,3,3,3,3,3,
3,4),(0.143172102,0.15412844,0.165137615,0.176146789,0.187155963,0.198165138,
0.211009174,0.222018349,0.233027523,0.244036697,0.255045872,0.266055046,
0.27706422,0.288073394,0.299082569,0.310091743,0.321100917,0.332110092,
0.343119266,0.35412844,0.365137615,0.376146789,0.387155963,0.396330275,
0.405504587,0.414678899,0.423853211,0.433027523,0.442201835,0.451376147,
0.460550459,0.469724771,0.478899083,0.488073394,0.497247706,0.506422018,
0.51559633,0.524770642,0.533944954,0.541284404,0.548623853,0.557798165,
0.565137615,0.572477064,0.579816514,0.587155963,0.596330275,0.603669725,
0.611009174,0.618348624,0.625688073,0.633027523,0.640366972,0.647706422,
0.655045872,0.664220183,0.671559633,0.678899083,0.686238532,0.693577982,
0.700917431,0.708256881,0.71559633,0.72293578,0.730275229,0.737614679,0.744954128,
0.752293578,0.759633028,0.766972477,0.774311927,0.781651376,0.788990826,
0.796330275,0.805504587,0.811009174,0.816513761,0.822018349,0.827522936,
0.833027523,0.83853211,0.844036697,0.849541284,0.855045872,0.860550459,
0.866055046,0.871559633,0.87706422,0.882568807,0.888073394,0.893577982,
0.899082569,0.904587156,0.910091743,0.91559633,0.921100917,0.926605505,
0.933944954,0.939449541,0.944954128,0.950458716,0.955963303,0.96146789,
0.968807339,0.974311927,0.979816514,0.985321101,0.99266055,1.),
 .UNSPECIFIED.);
#24385=B_SPLINE_CURVE_WITH_KNOTS('',3,(#209975,#209976,#209977,#209978,
#209979,#209980,#209981,#209982,#209983,#209984,#209985,#209986,#209987,
#209988,#209989,#209990,#209991,#209992,#209993,#209994,#209995,#209996,
#209997,#209998,#209999,#210000,#210001,#210002,#210003,#210004,#210005,
#210006,#210007,#210008,#210009,#210010,#210011,#210012,#210013,#210014,
#210015,#210016,#210017,#210018,#210019,#210020,#210021,#210022,#210023,
#210024,#210025,#210026,#210027,#210028,#210029,#210030,#210031,#210032,
#210033,#210034,#210035,#210036,#210037,#210038,#210039,#210040,#210041,
#210042,#210043,#210044,#210045,#210046,#210047,#210048,#210049,#210050,
#210051,#210052,#210053,#210054,#210055,#210056,#210057,#210058,#210059,
#210060,#210061,#210062,#210063,#210064,#210065,#210066,#210067,#210068,
#210069,#210070,#210071,#210072,#210073,#210074,#210075,#210076,#210077,
#210078,#210079,#210080,#210081,#210082,#210083,#210084,#210085,#210086,
#210087,#210088,#210089,#210090,#210091,#210092,#210093,#210094,#210095,
#210096,#210097,#210098,#210099,#210100,#210101,#210102,#210103,#210104,
#210105,#210106,#210107,#210108,#210109,#210110,#210111,#210112,#210113,
#210114,#210115,#210116,#210117,#210118,#210119,#210120,#210121,#210122,
#210123,#210124,#210125,#210126,#210127,#210128,#210129,#210130,#210131,
#210132,#210133,#210134,#210135,#210136,#210137,#210138,#210139,#210140,
#210141,#210142,#210143,#210144,#210145,#210146,#210147,#210148,#210149,
#210150,#210151,#210152,#210153,#210154,#210155,#210156,#210157,#210158,
#210159,#210160,#210161,#210162,#210163,#210164,#210165,#210166,#210167,
#210168,#210169,#210170,#210171,#210172,#210173,#210174,#210175,#210176,
#210177,#210178,#210179,#210180,#210181,#210182,#210183,#210184,#210185,
#210186,#210187,#210188,#210189,#210190,#210191,#210192,#210193,#210194,
#210195,#210196,#210197,#210198,#210199,#210200,#210201,#210202,#210203,
#210204,#210205,#210206,#210207,#210208,#210209,#210210,#210211,#210212,
#210213,#210214,#210215,#210216,#210217,#210218,#210219,#210220,#210221,
#210222,#210223,#210224,#210225,#210226,#210227,#210228,#210229,#210230,
#210231,#210232,#210233,#210234,#210235,#210236,#210237,#210238,#210239,
#210240,#210241,#210242,#210243,#210244,#210245,#210246,#210247,#210248,
#210249,#210250,#210251,#210252,#210253,#210254,#210255,#210256,#210257,
#210258,#210259,#210260,#210261,#210262,#210263,#210264,#210265,#210266,
#210267,#210268,#210269,#210270,#210271,#210272,#210273,#210274,#210275,
#210276,#210277,#210278,#210279,#210280,#210281,#210282,#210283,#210284,
#210285,#210286,#210287,#210288,#210289,#210290,#210291,#210292,#210293,
#210294,#210295,#210296,#210297,#210298,#210299),.UNSPECIFIED.,.F.,.F.,
(4,3,3,3,3,3,3,3,3,3,3,3,3,3,3,3,3,3,3,3,3,3,3,3,3,3,3,3,3,3,3,3,3,3,3,
3,3,3,3,3,3,3,3,3,3,3,3,3,3,3,3,3,3,3,3,3,3,3,3,3,3,3,3,3,3,3,3,3,3,3,3,
3,3,3,3,3,3,3,3,3,3,3,3,3,3,3,3,3,3,3,3,3,3,3,3,3,3,3,3,3,3,3,3,3,3,3,3,
3,4),(-1.,-0.994495413,-0.988990826,-0.983486239,-0.977981651,-0.972477064,
-0.966972477,-0.96146789,-0.955963303,-0.950458716,-0.944954128,-0.937614679,
-0.932110092,-0.926605505,-0.919266055,-0.913761468,-0.908256881,-0.902752294,
-0.897247706,-0.889908257,-0.88440367,-0.878899083,-0.873394495,-0.867889908,
-0.862385321,-0.856880734,-0.851376147,-0.84587156,-0.840366972,-0.834862385,
-0.829357798,-0.823853211,-0.818348624,-0.812844037,-0.80733945,-0.8,-0.79266055,
-0.785321101,-0.776146789,-0.768807339,-0.76146789,-0.75412844,-0.746788991,
-0.739449541,-0.732110092,-0.724770642,-0.717431193,-0.708256881,-0.699082569,
-0.691743119,-0.68440367,-0.67706422,-0.669724771,-0.662385321,-0.655045872,
-0.647706422,-0.640366972,-0.633027523,-0.625688073,-0.618348624,-0.611009174,
-0.603669725,-0.594495413,-0.587155963,-0.579816514,-0.572477064,-0.565137615,
-0.557798165,-0.550458716,-0.543119266,-0.535779817,-0.528440367,-0.519266055,
-0.510091743,-0.500917431,-0.491743119,-0.482568807,-0.473394495,-0.464220183,
-0.455045872,-0.44587156,-0.436697248,-0.427522936,-0.418348624,-0.409174312,
-0.398165138,-0.388990826,-0.377981651,-0.366972477,-0.355963303,-0.344954128,
-0.333944954,-0.32293578,-0.311926606,-0.300917431,-0.289908257,-0.278899083,
-0.267889908,-0.256880734,-0.24587156,-0.234862385,-0.223853211,-0.212844037,
-0.201834862,-0.190825688,-0.179816514,-0.168807339,-0.157798165,-0.143172102),
 .UNSPECIFIED.);
#24386=B_SPLINE_CURVE_WITH_KNOTS('',3,(#210300,#210301,#210302,#210303,
#210304,#210305,#210306,#210307,#210308,#210309,#210310,#210311,#210312,
#210313,#210314,#210315,#210316,#210317,#210318,#210319,#210320,#210321,
#210322,#210323,#210324,#210325,#210326,#210327,#210328,#210329,#210330,
#210331,#210332,#210333,#210334,#210335,#210336,#210337,#210338,#210339,
#210340,#210341,#210342,#210343,#210344,#210345,#210346,#210347,#210348,
#210349,#210350,#210351,#210352,#210353,#210354,#210355,#210356,#210357,
#210358,#210359,#210360,#210361,#210362,#210363,#210364,#210365,#210366,
#210367,#210368,#210369,#210370,#210371,#210372,#210373,#210374,#210375,
#210376,#210377,#210378,#210379,#210380,#210381,#210382,#210383,#210384,
#210385,#210386,#210387,#210388,#210389,#210390,#210391,#210392,#210393,
#210394,#210395,#210396,#210397,#210398,#210399,#210400,#210401,#210402,
#210403,#210404,#210405,#210406,#210407,#210408,#210409,#210410,#210411,
#210412,#210413,#210414,#210415,#210416,#210417,#210418,#210419,#210420,
#210421,#210422,#210423,#210424,#210425,#210426,#210427,#210428,#210429,
#210430,#210431,#210432,#210433,#210434,#210435,#210436,#210437,#210438,
#210439,#210440,#210441,#210442,#210443,#210444,#210445,#210446,#210447,
#210448,#210449,#210450,#210451,#210452,#210453,#210454,#210455,#210456,
#210457,#210458,#210459,#210460,#210461,#210462,#210463,#210464,#210465,
#210466,#210467,#210468,#210469,#210470,#210471,#210472,#210473,#210474,
#210475,#210476,#210477,#210478,#210479,#210480,#210481,#210482,#210483,
#210484,#210485,#210486,#210487,#210488,#210489,#210490,#210491,#210492,
#210493,#210494,#210495,#210496,#210497,#210498,#210499,#210500,#210501,
#210502,#210503,#210504,#210505,#210506,#210507,#210508,#210509,#210510,
#210511,#210512,#210513,#210514,#210515,#210516,#210517,#210518,#210519,
#210520,#210521,#210522,#210523,#210524,#210525,#210526,#210527,#210528,
#210529,#210530,#210531,#210532,#210533,#210534,#210535,#210536,#210537,
#210538,#210539,#210540,#210541,#210542,#210543,#210544,#210545,#210546,
#210547,#210548,#210549,#210550,#210551,#210552,#210553,#210554,#210555,
#210556,#210557,#210558,#210559,#210560,#210561,#210562,#210563,#210564,
#210565,#210566,#210567,#210568,#210569,#210570,#210571,#210572,#210573,
#210574,#210575,#210576,#210577,#210578,#210579,#210580,#210581,#210582,
#210583,#210584,#210585,#210586,#210587,#210588,#210589,#210590,#210591,
#210592,#210593,#210594,#210595,#210596,#210597,#210598,#210599,#210600,
#210601,#210602,#210603,#210604,#210605,#210606,#210607,#210608,#210609),
 .UNSPECIFIED.,.F.,.F.,(4,3,3,3,3,3,3,3,3,3,3,3,3,3,3,3,3,3,3,3,3,3,3,3,
3,3,3,3,3,3,3,3,3,3,3,3,3,3,3,3,3,3,3,3,3,3,3,3,3,3,3,3,3,3,3,3,3,3,3,3,
3,3,3,3,3,3,3,3,3,3,3,3,3,3,3,3,3,3,3,3,3,3,3,3,3,3,3,3,3,3,3,3,3,3,3,3,
3,3,3,3,3,3,3,4),(0.143172102,0.15412844,0.165137615,0.176146789,0.187155963,
0.198165138,0.209174312,0.220183486,0.231192661,0.242201835,0.253211009,
0.264220183,0.275229358,0.288073394,0.299082569,0.311926606,0.32293578,
0.333944954,0.344954128,0.355963303,0.366972477,0.377981651,0.388990826,
0.398165138,0.40733945,0.416513761,0.425688073,0.434862385,0.444036697,
0.455045872,0.464220183,0.473394495,0.482568807,0.491743119,0.500917431,
0.510091743,0.519266055,0.528440367,0.535779817,0.543119266,0.550458716,
0.557798165,0.565137615,0.574311927,0.581651376,0.588990826,0.598165138,
0.605504587,0.612844037,0.620183486,0.627522936,0.63853211,0.64587156,0.655045872,
0.662385321,0.671559633,0.678899083,0.686238532,0.693577982,0.706422018,
0.713761468,0.721100917,0.728440367,0.735779817,0.743119266,0.750458716,
0.757798165,0.765137615,0.772477064,0.781651376,0.79266055,0.801834862,
0.809174312,0.814678899,0.820183486,0.825688073,0.831192661,0.840366972,
0.847706422,0.853211009,0.860550459,0.867889908,0.873394495,0.878899083,
0.88440367,0.893577982,0.899082569,0.904587156,0.910091743,0.91559633,0.921100917,
0.930275229,0.935779817,0.943119266,0.948623853,0.955963303,0.96146789,
0.966972477,0.972477064,0.977981651,0.983486239,0.988990826,0.994495413,
1.),.UNSPECIFIED.);
#24387=B_SPLINE_CURVE_WITH_KNOTS('',3,(#211572,#211573,#211574,#211575,
#211576,#211577,#211578,#211579,#211580,#211581,#211582,#211583,#211584,
#211585,#211586,#211587,#211588,#211589,#211590,#211591,#211592,#211593,
#211594,#211595,#211596,#211597,#211598,#211599,#211600,#211601,#211602,
#211603,#211604,#211605,#211606,#211607,#211608,#211609,#211610,#211611,
#211612,#211613,#211614,#211615,#211616,#211617,#211618,#211619,#211620,
#211621,#211622,#211623,#211624,#211625,#211626,#211627,#211628,#211629,
#211630,#211631,#211632,#211633,#211634,#211635,#211636,#211637,#211638,
#211639,#211640,#211641,#211642,#211643,#211644,#211645,#211646,#211647,
#211648,#211649,#211650,#211651,#211652,#211653,#211654,#211655,#211656,
#211657,#211658,#211659,#211660,#211661,#211662,#211663,#211664,#211665,
#211666,#211667,#211668,#211669,#211670,#211671,#211672,#211673,#211674,
#211675,#211676,#211677,#211678,#211679,#211680,#211681,#211682,#211683,
#211684,#211685,#211686,#211687,#211688,#211689,#211690,#211691,#211692,
#211693,#211694,#211695,#211696,#211697,#211698,#211699,#211700,#211701,
#211702,#211703,#211704,#211705,#211706,#211707,#211708,#211709,#211710,
#211711,#211712,#211713,#211714,#211715,#211716,#211717,#211718,#211719,
#211720,#211721,#211722,#211723,#211724,#211725,#211726,#211727,#211728,
#211729,#211730,#211731,#211732,#211733,#211734,#211735,#211736,#211737,
#211738,#211739,#211740,#211741,#211742,#211743,#211744,#211745,#211746,
#211747,#211748,#211749,#211750,#211751,#211752,#211753,#211754,#211755,
#211756,#211757,#211758,#211759,#211760,#211761,#211762,#211763,#211764,
#211765,#211766,#211767,#211768,#211769,#211770,#211771,#211772,#211773,
#211774,#211775,#211776,#211777,#211778,#211779,#211780,#211781,#211782,
#211783,#211784,#211785,#211786,#211787,#211788,#211789,#211790,#211791,
#211792,#211793,#211794,#211795,#211796,#211797,#211798,#211799,#211800,
#211801,#211802,#211803,#211804,#211805,#211806,#211807,#211808,#211809,
#211810,#211811,#211812,#211813,#211814,#211815,#211816,#211817,#211818,
#211819,#211820,#211821,#211822,#211823,#211824,#211825,#211826,#211827,
#211828,#211829,#211830,#211831,#211832,#211833,#211834,#211835,#211836,
#211837,#211838,#211839,#211840,#211841,#211842,#211843,#211844,#211845,
#211846,#211847,#211848,#211849,#211850,#211851,#211852,#211853,#211854,
#211855,#211856,#211857,#211858,#211859,#211860,#211861,#211862,#211863,
#211864,#211865,#211866,#211867,#211868,#211869,#211870,#211871,#211872,
#211873,#211874,#211875,#211876,#211877,#211878,#211879,#211880,#211881,
#211882,#211883,#211884,#211885,#211886,#211887,#211888,#211889,#211890,
#211891,#211892,#211893),.UNSPECIFIED.,.F.,.F.,(4,3,3,3,3,3,3,3,3,3,3,3,
3,3,3,3,3,3,3,3,3,3,3,3,3,3,3,3,3,3,3,3,3,3,3,3,3,3,3,3,3,3,3,3,3,3,3,3,
3,3,3,3,3,3,3,3,3,3,3,3,3,3,3,3,3,3,3,3,3,3,3,3,3,3,3,3,3,3,3,3,3,3,3,3,
3,3,3,3,3,3,3,3,3,3,3,3,3,3,3,3,3,3,3,3,3,3,3,4),(-1.,-0.994495413,-0.988990826,
-0.981651376,-0.976146789,-0.970642202,-0.965137615,-0.959633028,-0.95412844,
-0.948623853,-0.941284404,-0.932110092,-0.926605505,-0.921100917,-0.91559633,
-0.910091743,-0.904587156,-0.899082569,-0.893577982,-0.888073394,-0.882568807,
-0.87706422,-0.871559633,-0.866055046,-0.860550459,-0.855045872,-0.849541284,
-0.842201835,-0.836697248,-0.831192661,-0.825688073,-0.820183486,-0.814678899,
-0.809174312,-0.801834862,-0.794495413,-0.787155963,-0.777981651,-0.770642202,
-0.763302752,-0.755963303,-0.748623853,-0.741284404,-0.732110092,-0.724770642,
-0.717431193,-0.710091743,-0.702752294,-0.695412844,-0.688073394,-0.680733945,
-0.671559633,-0.664220183,-0.656880734,-0.649541284,-0.642201835,-0.634862385,
-0.627522936,-0.620183486,-0.612844037,-0.605504587,-0.598165138,-0.590825688,
-0.583486239,-0.576146789,-0.568807339,-0.56146789,-0.55412844,-0.546788991,
-0.539449541,-0.532110092,-0.52293578,-0.513761468,-0.504587156,-0.495412844,
-0.486238532,-0.47706422,-0.467889908,-0.458715596,-0.449541284,-0.440366972,
-0.431192661,-0.422018349,-0.412844037,-0.403669725,-0.394495413,-0.383486239,
-0.372477064,-0.359633028,-0.348623853,-0.337614679,-0.326605505,-0.31559633,
-0.304587156,-0.293577982,-0.282568807,-0.271559633,-0.260550459,-0.249541284,
-0.23853211,-0.227522936,-0.216513761,-0.205504587,-0.194495413,-0.183486239,
-0.172477064,-0.16146789,-0.143172102),.UNSPECIFIED.);
#24388=B_SPLINE_CURVE_WITH_KNOTS('',3,(#211894,#211895,#211896,#211897,
#211898,#211899,#211900,#211901,#211902,#211903,#211904,#211905,#211906,
#211907,#211908,#211909,#211910,#211911,#211912,#211913,#211914,#211915,
#211916,#211917,#211918,#211919,#211920,#211921,#211922,#211923,#211924,
#211925,#211926,#211927,#211928,#211929,#211930,#211931,#211932,#211933,
#211934,#211935,#211936,#211937,#211938,#211939,#211940,#211941,#211942,
#211943,#211944,#211945,#211946,#211947,#211948,#211949,#211950,#211951,
#211952,#211953,#211954,#211955,#211956,#211957,#211958,#211959,#211960,
#211961,#211962,#211963,#211964,#211965,#211966,#211967,#211968,#211969,
#211970,#211971,#211972,#211973,#211974,#211975,#211976,#211977,#211978,
#211979,#211980,#211981,#211982,#211983,#211984,#211985,#211986,#211987,
#211988,#211989,#211990,#211991,#211992,#211993,#211994,#211995,#211996,
#211997,#211998,#211999,#212000,#212001,#212002,#212003,#212004,#212005,
#212006,#212007,#212008,#212009,#212010,#212011,#212012,#212013,#212014,
#212015,#212016,#212017,#212018,#212019,#212020,#212021,#212022,#212023,
#212024,#212025,#212026,#212027,#212028,#212029,#212030,#212031,#212032,
#212033,#212034,#212035,#212036,#212037,#212038,#212039,#212040,#212041,
#212042,#212043,#212044,#212045,#212046,#212047,#212048,#212049,#212050,
#212051,#212052,#212053,#212054,#212055,#212056,#212057,#212058,#212059,
#212060,#212061,#212062,#212063,#212064,#212065,#212066,#212067,#212068,
#212069,#212070,#212071,#212072,#212073,#212074,#212075,#212076,#212077,
#212078,#212079,#212080,#212081,#212082,#212083,#212084,#212085,#212086,
#212087,#212088,#212089,#212090,#212091,#212092,#212093,#212094,#212095,
#212096,#212097,#212098,#212099,#212100,#212101,#212102,#212103,#212104,
#212105,#212106,#212107,#212108,#212109,#212110,#212111,#212112,#212113,
#212114,#212115,#212116,#212117,#212118,#212119,#212120,#212121,#212122,
#212123,#212124,#212125,#212126,#212127,#212128,#212129,#212130,#212131,
#212132,#212133,#212134,#212135,#212136,#212137,#212138,#212139,#212140,
#212141,#212142,#212143,#212144,#212145,#212146,#212147,#212148,#212149,
#212150,#212151,#212152,#212153,#212154,#212155,#212156,#212157,#212158,
#212159,#212160,#212161,#212162,#212163,#212164,#212165,#212166,#212167,
#212168,#212169,#212170,#212171,#212172,#212173,#212174,#212175,#212176,
#212177,#212178,#212179,#212180,#212181,#212182,#212183,#212184,#212185,
#212186,#212187,#212188,#212189,#212190,#212191,#212192,#212193,#212194),
 .UNSPECIFIED.,.F.,.F.,(4,3,3,3,3,3,3,3,3,3,3,3,3,3,3,3,3,3,3,3,3,3,3,3,
3,3,3,3,3,3,3,3,3,3,3,3,3,3,3,3,3,3,3,3,3,3,3,3,3,3,3,3,3,3,3,3,3,3,3,3,
3,3,3,3,3,3,3,3,3,3,3,3,3,3,3,3,3,3,3,3,3,3,3,3,3,3,3,3,3,3,3,3,3,3,3,3,
3,3,3,3,4),(0.143172102,0.15412844,0.165137615,0.176146789,0.187155963,
0.198165138,0.209174312,0.220183486,0.231192661,0.242201835,0.253211009,
0.264220183,0.275229358,0.288073394,0.299082569,0.310091743,0.326605505,
0.337614679,0.348623853,0.359633028,0.370642202,0.381651376,0.39266055,
0.401834862,0.411009174,0.420183486,0.429357798,0.43853211,0.449541284,
0.458715596,0.467889908,0.47706422,0.488073394,0.499082569,0.508256881,
0.517431193,0.526605505,0.533944954,0.541284404,0.548623853,0.555963303,
0.563302752,0.572477064,0.579816514,0.590825688,0.598165138,0.60733945,
0.614678899,0.622018349,0.631192661,0.640366972,0.647706422,0.656880734,
0.669724771,0.67706422,0.686238532,0.693577982,0.704587156,0.713761468,
0.721100917,0.728440367,0.737614679,0.744954128,0.752293578,0.76146789,
0.768807339,0.776146789,0.785321101,0.79266055,0.8,0.80733945,0.814678899,
0.820183486,0.825688073,0.833027523,0.83853211,0.844036697,0.853211009,
0.858715596,0.864220183,0.873394495,0.878899083,0.886238532,0.891743119,
0.897247706,0.902752294,0.908256881,0.917431193,0.92293578,0.930275229,
0.937614679,0.944954128,0.952293578,0.957798165,0.963302752,0.968807339,
0.974311927,0.979816514,0.988990826,0.994495413,1.),.UNSPECIFIED.);
#24389=B_SPLINE_CURVE_WITH_KNOTS('',3,(#213139,#213140,#213141,#213142,
#213143,#213144,#213145,#213146,#213147,#213148,#213149,#213150,#213151,
#213152,#213153,#213154,#213155,#213156,#213157,#213158,#213159,#213160,
#213161,#213162,#213163,#213164,#213165,#213166,#213167,#213168,#213169,
#213170,#213171,#213172,#213173,#213174,#213175,#213176,#213177,#213178,
#213179,#213180,#213181,#213182,#213183,#213184,#213185,#213186,#213187,
#213188,#213189,#213190,#213191,#213192,#213193,#213194,#213195,#213196,
#213197,#213198,#213199,#213200,#213201,#213202,#213203,#213204,#213205,
#213206,#213207,#213208,#213209,#213210,#213211,#213212,#213213,#213214,
#213215,#213216,#213217,#213218,#213219,#213220,#213221,#213222,#213223,
#213224,#213225,#213226,#213227,#213228,#213229,#213230,#213231,#213232,
#213233,#213234,#213235,#213236,#213237,#213238,#213239,#213240,#213241,
#213242,#213243,#213244,#213245,#213246,#213247,#213248,#213249,#213250,
#213251,#213252,#213253,#213254,#213255,#213256,#213257,#213258,#213259,
#213260,#213261,#213262,#213263,#213264,#213265,#213266,#213267,#213268,
#213269,#213270,#213271,#213272,#213273,#213274,#213275,#213276,#213277,
#213278,#213279,#213280,#213281,#213282,#213283,#213284,#213285,#213286,
#213287,#213288,#213289,#213290,#213291,#213292,#213293,#213294,#213295,
#213296,#213297,#213298,#213299,#213300,#213301,#213302,#213303,#213304,
#213305,#213306,#213307,#213308,#213309,#213310,#213311,#213312,#213313,
#213314,#213315,#213316,#213317,#213318,#213319,#213320,#213321,#213322,
#213323,#213324,#213325,#213326,#213327,#213328,#213329,#213330,#213331,
#213332,#213333,#213334,#213335,#213336,#213337,#213338,#213339,#213340,
#213341,#213342,#213343,#213344,#213345,#213346,#213347,#213348,#213349,
#213350,#213351,#213352,#213353,#213354,#213355,#213356,#213357,#213358,
#213359,#213360,#213361,#213362,#213363,#213364,#213365,#213366,#213367,
#213368,#213369,#213370,#213371,#213372,#213373,#213374,#213375,#213376,
#213377,#213378,#213379,#213380,#213381,#213382,#213383,#213384,#213385,
#213386,#213387,#213388,#213389,#213390,#213391,#213392,#213393,#213394,
#213395,#213396,#213397,#213398,#213399,#213400,#213401,#213402,#213403,
#213404,#213405,#213406,#213407,#213408,#213409,#213410,#213411,#213412,
#213413,#213414,#213415,#213416,#213417,#213418,#213419,#213420,#213421,
#213422,#213423,#213424,#213425,#213426,#213427,#213428,#213429,#213430,
#213431,#213432,#213433,#213434,#213435,#213436,#213437,#213438,#213439,
#213440,#213441,#213442,#213443,#213444,#213445,#213446,#213447,#213448),
 .UNSPECIFIED.,.F.,.F.,(4,3,3,3,3,3,3,3,3,3,3,3,3,3,3,3,3,3,3,3,3,3,3,3,
3,3,3,3,3,3,3,3,3,3,3,3,3,3,3,3,3,3,3,3,3,3,3,3,3,3,3,3,3,3,3,3,3,3,3,3,
3,3,3,3,3,3,3,3,3,3,3,3,3,3,3,3,3,3,3,3,3,3,3,3,3,3,3,3,3,3,3,3,3,3,3,3,
3,3,3,3,3,3,3,4),(0.143172102,0.15412844,0.165137615,0.177981651,0.188990826,
0.2,0.211009174,0.222018349,0.233027523,0.244036697,0.255045872,0.266055046,
0.27706422,0.288073394,0.302752294,0.313761468,0.324770642,0.335779817,
0.346788991,0.357798165,0.368807339,0.379816514,0.390825688,0.4,0.409174312,
0.418348624,0.429357798,0.43853211,0.447706422,0.456880734,0.467889908,
0.47706422,0.486238532,0.495412844,0.504587156,0.513761468,0.52293578,0.532110092,
0.539449541,0.546788991,0.55412844,0.56146789,0.568807339,0.576146789,0.583486239,
0.590825688,0.601834862,0.611009174,0.618348624,0.625688073,0.634862385,
0.644036697,0.653211009,0.660550459,0.667889908,0.675229358,0.68440367,
0.691743119,0.699082569,0.706422018,0.713761468,0.721100917,0.730275229,
0.739449541,0.746788991,0.755963303,0.763302752,0.772477064,0.779816514,
0.787155963,0.794495413,0.801834862,0.809174312,0.814678899,0.823853211,
0.829357798,0.834862385,0.840366972,0.84587156,0.851376147,0.856880734,
0.864220183,0.869724771,0.875229358,0.88440367,0.889908257,0.895412844,
0.900917431,0.906422018,0.911926606,0.917431193,0.92293578,0.928440367,
0.933944954,0.941284404,0.946788991,0.955963303,0.96146789,0.966972477,
0.974311927,0.981651376,0.987155963,0.99266055,1.),.UNSPECIFIED.);
#24390=B_SPLINE_CURVE_WITH_KNOTS('',3,(#213449,#213450,#213451,#213452,
#213453,#213454,#213455,#213456,#213457,#213458,#213459,#213460,#213461,
#213462,#213463,#213464,#213465,#213466,#213467,#213468,#213469,#213470,
#213471,#213472,#213473,#213474,#213475,#213476,#213477,#213478,#213479,
#213480,#213481,#213482,#213483,#213484,#213485,#213486,#213487,#213488,
#213489,#213490,#213491,#213492,#213493,#213494,#213495,#213496,#213497,
#213498,#213499,#213500,#213501,#213502,#213503,#213504,#213505,#213506,
#213507,#213508,#213509,#213510,#213511,#213512,#213513,#213514,#213515,
#213516,#213517,#213518,#213519,#213520,#213521,#213522,#213523,#213524,
#213525,#213526,#213527,#213528,#213529,#213530,#213531,#213532,#213533,
#213534,#213535,#213536,#213537,#213538,#213539,#213540,#213541,#213542,
#213543,#213544,#213545,#213546,#213547,#213548,#213549,#213550,#213551,
#213552,#213553,#213554,#213555,#213556,#213557,#213558,#213559,#213560,
#213561,#213562,#213563,#213564,#213565,#213566,#213567,#213568,#213569,
#213570,#213571,#213572,#213573,#213574,#213575,#213576,#213577,#213578,
#213579,#213580,#213581,#213582,#213583,#213584,#213585,#213586,#213587,
#213588,#213589,#213590,#213591,#213592,#213593,#213594,#213595,#213596,
#213597,#213598,#213599,#213600,#213601,#213602,#213603,#213604,#213605,
#213606,#213607,#213608,#213609,#213610,#213611,#213612,#213613,#213614,
#213615,#213616,#213617,#213618,#213619,#213620,#213621,#213622,#213623,
#213624,#213625,#213626,#213627,#213628,#213629,#213630,#213631,#213632,
#213633,#213634,#213635,#213636,#213637,#213638,#213639,#213640,#213641,
#213642,#213643,#213644,#213645,#213646,#213647,#213648,#213649,#213650,
#213651,#213652,#213653,#213654,#213655,#213656,#213657,#213658,#213659,
#213660,#213661,#213662,#213663,#213664,#213665,#213666,#213667,#213668,
#213669,#213670,#213671,#213672,#213673,#213674,#213675,#213676,#213677,
#213678,#213679,#213680,#213681,#213682,#213683,#213684,#213685,#213686,
#213687,#213688,#213689,#213690,#213691,#213692,#213693,#213694,#213695,
#213696,#213697,#213698,#213699,#213700,#213701,#213702,#213703,#213704,
#213705,#213706,#213707,#213708,#213709,#213710,#213711,#213712,#213713,
#213714,#213715,#213716,#213717,#213718,#213719,#213720,#213721,#213722,
#213723,#213724,#213725,#213726,#213727,#213728,#213729,#213730,#213731,
#213732,#213733,#213734,#213735,#213736,#213737,#213738,#213739,#213740,
#213741,#213742,#213743,#213744,#213745,#213746,#213747,#213748,#213749,
#213750,#213751,#213752,#213753,#213754,#213755,#213756,#213757,#213758,
#213759,#213760,#213761,#213762,#213763,#213764,#213765,#213766,#213767,
#213768,#213769,#213770,#213771,#213772,#213773),.UNSPECIFIED.,.F.,.F.,
(4,3,3,3,3,3,3,3,3,3,3,3,3,3,3,3,3,3,3,3,3,3,3,3,3,3,3,3,3,3,3,3,3,3,3,
3,3,3,3,3,3,3,3,3,3,3,3,3,3,3,3,3,3,3,3,3,3,3,3,3,3,3,3,3,3,3,3,3,3,3,3,
3,3,3,3,3,3,3,3,3,3,3,3,3,3,3,3,3,3,3,3,3,3,3,3,3,3,3,3,3,3,3,3,3,3,3,3,
3,4),(0.143172102,0.15412844,0.165137615,0.177981651,0.188990826,0.2,0.211009174,
0.222018349,0.233027523,0.244036697,0.255045872,0.266055046,0.27706422,
0.288073394,0.300917431,0.311926606,0.32293578,0.333944954,0.344954128,
0.355963303,0.366972477,0.377981651,0.388990826,0.398165138,0.40733945,
0.416513761,0.429357798,0.43853211,0.447706422,0.456880734,0.466055046,
0.475229358,0.486238532,0.495412844,0.504587156,0.513761468,0.52293578,
0.532110092,0.539449541,0.546788991,0.55412844,0.56146789,0.568807339,0.576146789,
0.583486239,0.590825688,0.598165138,0.605504587,0.612844037,0.620183486,
0.627522936,0.634862385,0.644036697,0.651376147,0.658715596,0.666055046,
0.673394495,0.680733945,0.688073394,0.695412844,0.702752294,0.710091743,
0.717431193,0.724770642,0.732110092,0.739449541,0.746788991,0.75412844,
0.76146789,0.768807339,0.776146789,0.783486239,0.790825688,0.798165138,
0.805504587,0.811009174,0.816513761,0.822018349,0.827522936,0.833027523,
0.83853211,0.844036697,0.849541284,0.855045872,0.860550459,0.866055046,
0.871559633,0.87706422,0.882568807,0.888073394,0.893577982,0.899082569,
0.904587156,0.910091743,0.91559633,0.921100917,0.928440367,0.933944954,
0.939449541,0.944954128,0.950458716,0.955963303,0.96146789,0.966972477,
0.974311927,0.979816514,0.987155963,0.99266055,1.),.UNSPECIFIED.);
#24391=B_SPLINE_CURVE_WITH_KNOTS('',3,(#214733,#214734,#214735,#214736,
#214737,#214738,#214739,#214740,#214741,#214742,#214743,#214744,#214745,
#214746,#214747,#214748,#214749,#214750,#214751,#214752,#214753,#214754,
#214755,#214756,#214757,#214758,#214759,#214760,#214761,#214762,#214763,
#214764,#214765,#214766,#214767,#214768,#214769,#214770,#214771,#214772,
#214773,#214774,#214775,#214776,#214777,#214778,#214779,#214780,#214781,
#214782,#214783,#214784,#214785,#214786,#214787,#214788,#214789,#214790,
#214791,#214792,#214793,#214794,#214795,#214796,#214797,#214798,#214799,
#214800,#214801,#214802,#214803,#214804,#214805,#214806,#214807,#214808,
#214809,#214810,#214811,#214812,#214813,#214814,#214815,#214816,#214817,
#214818,#214819,#214820,#214821,#214822,#214823,#214824,#214825,#214826,
#214827,#214828,#214829,#214830,#214831,#214832,#214833,#214834,#214835,
#214836,#214837,#214838,#214839,#214840,#214841,#214842,#214843,#214844,
#214845,#214846,#214847,#214848,#214849,#214850,#214851,#214852,#214853,
#214854,#214855,#214856,#214857,#214858,#214859,#214860,#214861,#214862,
#214863,#214864,#214865,#214866,#214867,#214868,#214869,#214870,#214871,
#214872,#214873,#214874,#214875,#214876,#214877,#214878,#214879,#214880,
#214881,#214882,#214883,#214884,#214885,#214886,#214887,#214888,#214889,
#214890,#214891,#214892,#214893,#214894,#214895,#214896,#214897,#214898,
#214899,#214900,#214901,#214902,#214903,#214904,#214905,#214906,#214907,
#214908,#214909,#214910,#214911,#214912,#214913,#214914,#214915,#214916,
#214917,#214918,#214919,#214920,#214921,#214922,#214923,#214924,#214925,
#214926,#214927,#214928,#214929,#214930,#214931,#214932,#214933,#214934,
#214935,#214936,#214937,#214938,#214939,#214940,#214941,#214942,#214943,
#214944,#214945,#214946,#214947,#214948,#214949,#214950,#214951,#214952,
#214953,#214954,#214955,#214956,#214957,#214958,#214959,#214960,#214961,
#214962,#214963,#214964,#214965,#214966,#214967,#214968,#214969,#214970,
#214971,#214972,#214973,#214974,#214975,#214976,#214977,#214978,#214979,
#214980,#214981,#214982,#214983,#214984,#214985,#214986,#214987,#214988,
#214989,#214990,#214991,#214992,#214993,#214994,#214995,#214996,#214997,
#214998,#214999,#215000,#215001,#215002,#215003,#215004,#215005,#215006,
#215007,#215008,#215009,#215010,#215011,#215012,#215013,#215014,#215015,
#215016,#215017,#215018,#215019,#215020,#215021,#215022,#215023,#215024,
#215025,#215026,#215027,#215028,#215029,#215030,#215031,#215032,#215033,
#215034,#215035,#215036,#215037,#215038,#215039),.UNSPECIFIED.,.F.,.F.,
(4,3,3,3,3,3,3,3,3,3,3,3,3,3,3,3,3,3,3,3,3,3,3,3,3,3,3,3,3,3,3,3,3,3,3,
3,3,3,3,3,3,3,3,3,3,3,3,3,3,3,3,3,3,3,3,3,3,3,3,3,3,3,3,3,3,3,3,3,3,3,3,
3,3,3,3,3,3,3,3,3,3,3,3,3,3,3,3,3,3,3,3,3,3,3,3,3,3,3,3,3,3,3,4),(0.143172102,
0.15412844,0.165137615,0.176146789,0.187155963,0.198165138,0.211009174,
0.222018349,0.233027523,0.244036697,0.255045872,0.266055046,0.27706422,
0.288073394,0.299082569,0.310091743,0.321100917,0.332110092,0.343119266,
0.35412844,0.365137615,0.376146789,0.387155963,0.396330275,0.405504587,
0.414678899,0.423853211,0.434862385,0.444036697,0.455045872,0.464220183,
0.473394495,0.482568807,0.491743119,0.500917431,0.510091743,0.519266055,
0.530275229,0.537614679,0.544954128,0.552293578,0.559633028,0.566972477,
0.574311927,0.581651376,0.59266055,0.6,0.60733945,0.614678899,0.622018349,
0.629357798,0.636697248,0.644036697,0.651376147,0.658715596,0.666055046,
0.673394495,0.680733945,0.693577982,0.704587156,0.711926606,0.719266055,
0.726605505,0.733944954,0.741284404,0.748623853,0.755963303,0.763302752,
0.772477064,0.781651376,0.790825688,0.798165138,0.80733945,0.814678899,
0.822018349,0.831192661,0.836697248,0.84587156,0.853211009,0.858715596,
0.864220183,0.869724771,0.875229358,0.88440367,0.893577982,0.899082569,
0.904587156,0.910091743,0.919266055,0.924770642,0.930275229,0.935779817,
0.943119266,0.948623853,0.95412844,0.959633028,0.966972477,0.972477064,
0.977981651,0.983486239,0.988990826,0.994495413,1.),.UNSPECIFIED.);
#24392=B_SPLINE_CURVE_WITH_KNOTS('',3,(#215040,#215041,#215042,#215043,
#215044,#215045,#215046,#215047,#215048,#215049,#215050,#215051,#215052,
#215053,#215054,#215055,#215056,#215057,#215058,#215059,#215060,#215061,
#215062,#215063,#215064,#215065,#215066,#215067,#215068,#215069,#215070,
#215071,#215072,#215073,#215074,#215075,#215076,#215077,#215078,#215079,
#215080,#215081,#215082,#215083,#215084,#215085,#215086,#215087,#215088,
#215089,#215090,#215091,#215092,#215093,#215094,#215095,#215096,#215097,
#215098,#215099,#215100,#215101,#215102,#215103,#215104,#215105,#215106,
#215107,#215108,#215109,#215110,#215111,#215112,#215113,#215114,#215115,
#215116,#215117,#215118,#215119,#215120,#215121,#215122,#215123,#215124,
#215125,#215126,#215127,#215128,#215129,#215130,#215131,#215132,#215133,
#215134,#215135,#215136,#215137,#215138,#215139,#215140,#215141,#215142,
#215143,#215144,#215145,#215146,#215147,#215148,#215149,#215150,#215151,
#215152,#215153,#215154,#215155,#215156,#215157,#215158,#215159,#215160,
#215161,#215162,#215163,#215164,#215165,#215166,#215167,#215168,#215169,
#215170,#215171,#215172,#215173,#215174,#215175,#215176,#215177,#215178,
#215179,#215180,#215181,#215182,#215183,#215184,#215185,#215186,#215187,
#215188,#215189,#215190,#215191,#215192,#215193,#215194,#215195,#215196,
#215197,#215198,#215199,#215200,#215201,#215202,#215203,#215204,#215205,
#215206,#215207,#215208,#215209,#215210,#215211,#215212,#215213,#215214,
#215215,#215216,#215217,#215218,#215219,#215220,#215221,#215222,#215223,
#215224,#215225,#215226,#215227,#215228,#215229,#215230,#215231,#215232,
#215233,#215234,#215235,#215236,#215237,#215238,#215239,#215240,#215241,
#215242,#215243,#215244,#215245,#215246,#215247,#215248,#215249,#215250,
#215251,#215252,#215253,#215254,#215255,#215256,#215257,#215258,#215259,
#215260,#215261,#215262,#215263,#215264,#215265,#215266,#215267,#215268,
#215269,#215270,#215271,#215272,#215273,#215274,#215275,#215276,#215277,
#215278,#215279,#215280,#215281,#215282,#215283,#215284,#215285,#215286,
#215287,#215288,#215289,#215290,#215291,#215292,#215293,#215294,#215295,
#215296,#215297,#215298,#215299,#215300,#215301,#215302,#215303,#215304,
#215305,#215306,#215307,#215308,#215309,#215310,#215311,#215312,#215313,
#215314,#215315,#215316,#215317,#215318,#215319,#215320,#215321,#215322,
#215323,#215324,#215325,#215326,#215327,#215328,#215329,#215330,#215331,
#215332,#215333,#215334,#215335,#215336,#215337,#215338,#215339,#215340,
#215341,#215342,#215343,#215344,#215345,#215346,#215347,#215348,#215349,
#215350,#215351,#215352,#215353,#215354,#215355,#215356,#215357,#215358,
#215359,#215360,#215361,#215362,#215363,#215364),.UNSPECIFIED.,.F.,.F.,
(4,3,3,3,3,3,3,3,3,3,3,3,3,3,3,3,3,3,3,3,3,3,3,3,3,3,3,3,3,3,3,3,3,3,3,
3,3,3,3,3,3,3,3,3,3,3,3,3,3,3,3,3,3,3,3,3,3,3,3,3,3,3,3,3,3,3,3,3,3,3,3,
3,3,3,3,3,3,3,3,3,3,3,3,3,3,3,3,3,3,3,3,3,3,3,3,3,3,3,3,3,3,3,3,3,3,3,3,
3,4),(0.143172102,0.15412844,0.165137615,0.176146789,0.187155963,0.198165138,
0.211009174,0.222018349,0.233027523,0.244036697,0.255045872,0.266055046,
0.27706422,0.288073394,0.299082569,0.310091743,0.321100917,0.332110092,
0.343119266,0.35412844,0.365137615,0.376146789,0.387155963,0.396330275,
0.405504587,0.414678899,0.423853211,0.433027523,0.442201835,0.451376147,
0.460550459,0.469724771,0.478899083,0.488073394,0.497247706,0.506422018,
0.51559633,0.524770642,0.533944954,0.541284404,0.548623853,0.555963303,
0.563302752,0.570642202,0.577981651,0.585321101,0.59266055,0.6,0.60733945,
0.614678899,0.622018349,0.629357798,0.636697248,0.644036697,0.651376147,
0.658715596,0.666055046,0.673394495,0.680733945,0.688073394,0.695412844,
0.704587156,0.711926606,0.719266055,0.726605505,0.733944954,0.741284404,
0.748623853,0.755963303,0.763302752,0.772477064,0.779816514,0.787155963,
0.794495413,0.801834862,0.809174312,0.814678899,0.820183486,0.825688073,
0.831192661,0.836697248,0.842201835,0.847706422,0.853211009,0.858715596,
0.864220183,0.869724771,0.875229358,0.882568807,0.888073394,0.893577982,
0.899082569,0.904587156,0.910091743,0.91559633,0.921100917,0.928440367,
0.933944954,0.939449541,0.944954128,0.950458716,0.957798165,0.963302752,
0.968807339,0.974311927,0.979816514,0.985321101,0.990825688,1.),
 .UNSPECIFIED.);
#24393=B_SPLINE_CURVE_WITH_KNOTS('',3,(#216312,#216313,#216314,#216315,
#216316,#216317,#216318,#216319,#216320,#216321,#216322,#216323,#216324,
#216325,#216326,#216327,#216328,#216329,#216330,#216331,#216332,#216333,
#216334,#216335,#216336,#216337,#216338,#216339,#216340,#216341,#216342,
#216343,#216344,#216345,#216346,#216347,#216348,#216349,#216350,#216351,
#216352,#216353,#216354,#216355,#216356,#216357,#216358,#216359,#216360,
#216361,#216362,#216363,#216364,#216365,#216366,#216367,#216368,#216369,
#216370,#216371,#216372,#216373,#216374,#216375,#216376,#216377,#216378,
#216379,#216380,#216381,#216382,#216383,#216384,#216385,#216386,#216387,
#216388,#216389,#216390,#216391,#216392,#216393,#216394,#216395,#216396,
#216397,#216398,#216399,#216400,#216401,#216402,#216403,#216404,#216405,
#216406,#216407,#216408,#216409,#216410,#216411,#216412,#216413,#216414,
#216415,#216416,#216417,#216418,#216419,#216420,#216421,#216422,#216423,
#216424,#216425,#216426,#216427,#216428,#216429,#216430,#216431,#216432,
#216433,#216434,#216435,#216436,#216437,#216438,#216439,#216440,#216441,
#216442,#216443,#216444,#216445,#216446,#216447,#216448,#216449,#216450,
#216451,#216452,#216453,#216454,#216455,#216456,#216457,#216458,#216459,
#216460,#216461,#216462,#216463,#216464,#216465,#216466,#216467,#216468,
#216469,#216470,#216471,#216472,#216473,#216474,#216475,#216476,#216477,
#216478,#216479,#216480,#216481,#216482,#216483,#216484,#216485,#216486,
#216487,#216488,#216489,#216490,#216491,#216492,#216493,#216494,#216495,
#216496,#216497,#216498,#216499,#216500,#216501,#216502,#216503,#216504,
#216505,#216506,#216507,#216508,#216509,#216510,#216511,#216512,#216513,
#216514,#216515,#216516,#216517,#216518,#216519,#216520,#216521,#216522,
#216523,#216524,#216525,#216526,#216527,#216528,#216529,#216530,#216531,
#216532,#216533,#216534,#216535,#216536,#216537,#216538,#216539,#216540,
#216541,#216542,#216543,#216544,#216545,#216546,#216547,#216548,#216549,
#216550,#216551,#216552,#216553,#216554,#216555,#216556,#216557,#216558,
#216559,#216560,#216561,#216562,#216563,#216564,#216565,#216566,#216567,
#216568,#216569,#216570,#216571,#216572,#216573,#216574,#216575,#216576,
#216577,#216578,#216579,#216580,#216581,#216582,#216583,#216584,#216585,
#216586,#216587,#216588,#216589,#216590,#216591,#216592,#216593,#216594,
#216595,#216596,#216597,#216598,#216599,#216600,#216601,#216602,#216603,
#216604,#216605,#216606,#216607,#216608,#216609,#216610,#216611,#216612,
#216613,#216614,#216615,#216616,#216617,#216618,#216619,#216620,#216621,
#216622,#216623,#216624,#216625,#216626,#216627,#216628,#216629,#216630,
#216631,#216632,#216633),.UNSPECIFIED.,.F.,.F.,(4,3,3,3,3,3,3,3,3,3,3,3,
3,3,3,3,3,3,3,3,3,3,3,3,3,3,3,3,3,3,3,3,3,3,3,3,3,3,3,3,3,3,3,3,3,3,3,3,
3,3,3,3,3,3,3,3,3,3,3,3,3,3,3,3,3,3,3,3,3,3,3,3,3,3,3,3,3,3,3,3,3,3,3,3,
3,3,3,3,3,3,3,3,3,3,3,3,3,3,3,3,3,3,3,3,3,3,3,4),(-1.,-0.99266055,-0.985321101,
-0.979816514,-0.974311927,-0.968807339,-0.963302752,-0.957798165,-0.952293578,
-0.946788991,-0.941284404,-0.933944954,-0.928440367,-0.92293578,-0.917431193,
-0.911926606,-0.906422018,-0.900917431,-0.895412844,-0.889908257,-0.88440367,
-0.878899083,-0.873394495,-0.867889908,-0.862385321,-0.856880734,-0.851376147,
-0.84587156,-0.840366972,-0.833027523,-0.827522936,-0.822018349,-0.816513761,
-0.809174312,-0.801834862,-0.794495413,-0.787155963,-0.779816514,-0.772477064,
-0.765137615,-0.757798165,-0.750458716,-0.743119266,-0.735779817,-0.728440367,
-0.721100917,-0.710091743,-0.702752294,-0.695412844,-0.688073394,-0.680733945,
-0.673394495,-0.666055046,-0.658715596,-0.651376147,-0.644036697,-0.636697248,
-0.627522936,-0.620183486,-0.612844037,-0.605504587,-0.598165138,-0.590825688,
-0.583486239,-0.576146789,-0.568807339,-0.56146789,-0.55412844,-0.546788991,
-0.539449541,-0.532110092,-0.52293578,-0.513761468,-0.504587156,-0.495412844,
-0.486238532,-0.47706422,-0.467889908,-0.458715596,-0.447706422,-0.43853211,
-0.429357798,-0.420183486,-0.411009174,-0.401834862,-0.39266055,-0.381651376,
-0.370642202,-0.359633028,-0.346788991,-0.335779817,-0.324770642,-0.313761468,
-0.302752294,-0.291743119,-0.280733945,-0.269724771,-0.258715596,-0.247706422,
-0.236697248,-0.225688073,-0.214678899,-0.203669725,-0.19266055,-0.181651376,
-0.170642202,-0.159633028,-0.143172102),.UNSPECIFIED.);
#24394=B_SPLINE_CURVE_WITH_KNOTS('',3,(#216634,#216635,#216636,#216637,
#216638,#216639,#216640,#216641,#216642,#216643,#216644,#216645,#216646,
#216647,#216648,#216649,#216650,#216651,#216652,#216653,#216654,#216655,
#216656,#216657,#216658,#216659,#216660,#216661,#216662,#216663,#216664,
#216665,#216666,#216667,#216668,#216669,#216670,#216671,#216672,#216673,
#216674,#216675,#216676,#216677,#216678,#216679,#216680,#216681,#216682,
#216683,#216684,#216685,#216686,#216687,#216688,#216689,#216690,#216691,
#216692,#216693,#216694,#216695,#216696,#216697,#216698,#216699,#216700,
#216701,#216702,#216703,#216704,#216705,#216706,#216707,#216708,#216709,
#216710,#216711,#216712,#216713,#216714,#216715,#216716,#216717,#216718,
#216719,#216720,#216721,#216722,#216723,#216724,#216725,#216726,#216727,
#216728,#216729,#216730,#216731,#216732,#216733,#216734,#216735,#216736,
#216737,#216738,#216739,#216740,#216741,#216742,#216743,#216744,#216745,
#216746,#216747,#216748,#216749,#216750,#216751,#216752,#216753,#216754,
#216755,#216756,#216757,#216758,#216759,#216760,#216761,#216762,#216763,
#216764,#216765,#216766,#216767,#216768,#216769,#216770,#216771,#216772,
#216773,#216774,#216775,#216776,#216777,#216778,#216779,#216780,#216781,
#216782,#216783,#216784,#216785,#216786,#216787,#216788,#216789,#216790,
#216791,#216792,#216793,#216794,#216795,#216796,#216797,#216798,#216799,
#216800,#216801,#216802,#216803,#216804,#216805,#216806,#216807,#216808,
#216809,#216810,#216811,#216812,#216813,#216814,#216815,#216816,#216817,
#216818,#216819,#216820,#216821,#216822,#216823,#216824,#216825,#216826,
#216827,#216828,#216829,#216830,#216831,#216832,#216833,#216834,#216835,
#216836,#216837,#216838,#216839,#216840,#216841,#216842,#216843,#216844,
#216845,#216846,#216847,#216848,#216849,#216850,#216851,#216852,#216853,
#216854,#216855,#216856,#216857,#216858,#216859,#216860,#216861,#216862,
#216863,#216864,#216865,#216866,#216867,#216868,#216869,#216870,#216871,
#216872,#216873,#216874,#216875,#216876,#216877,#216878,#216879,#216880,
#216881,#216882,#216883,#216884,#216885,#216886,#216887,#216888,#216889,
#216890,#216891,#216892,#216893,#216894,#216895,#216896,#216897,#216898,
#216899,#216900,#216901,#216902,#216903,#216904,#216905,#216906,#216907,
#216908,#216909,#216910,#216911,#216912,#216913,#216914,#216915,#216916,
#216917,#216918,#216919,#216920,#216921,#216922,#216923,#216924,#216925,
#216926,#216927,#216928,#216929,#216930,#216931,#216932,#216933,#216934,
#216935,#216936,#216937,#216938,#216939,#216940),.UNSPECIFIED.,.F.,.F.,
(4,3,3,3,3,3,3,3,3,3,3,3,3,3,3,3,3,3,3,3,3,3,3,3,3,3,3,3,3,3,3,3,3,3,3,
3,3,3,3,3,3,3,3,3,3,3,3,3,3,3,3,3,3,3,3,3,3,3,3,3,3,3,3,3,3,3,3,3,3,3,3,
3,3,3,3,3,3,3,3,3,3,3,3,3,3,3,3,3,3,3,3,3,3,3,3,3,3,3,3,3,3,3,4),(0.143172102,
0.15412844,0.165137615,0.176146789,0.187155963,0.198165138,0.209174312,
0.220183486,0.231192661,0.242201835,0.253211009,0.264220183,0.275229358,
0.286238532,0.297247706,0.308256881,0.319266055,0.330275229,0.341284404,
0.352293578,0.363302752,0.376146789,0.387155963,0.396330275,0.405504587,
0.416513761,0.425688073,0.434862385,0.444036697,0.453211009,0.462385321,
0.471559633,0.48440367,0.493577982,0.502752294,0.511926606,0.521100917,
0.530275229,0.537614679,0.544954128,0.552293578,0.56146789,0.568807339,
0.576146789,0.585321101,0.594495413,0.601834862,0.609174312,0.616513761,
0.623853211,0.631192661,0.63853211,0.64587156,0.653211009,0.662385321,0.669724771,
0.678899083,0.688073394,0.695412844,0.702752294,0.710091743,0.721100917,
0.730275229,0.739449541,0.746788991,0.75412844,0.763302752,0.770642202,
0.777981651,0.785321101,0.79266055,0.801834862,0.809174312,0.816513761,
0.822018349,0.827522936,0.836697248,0.844036697,0.851376147,0.856880734,
0.862385321,0.867889908,0.873394495,0.882568807,0.888073394,0.893577982,
0.900917431,0.906422018,0.913761468,0.919266055,0.924770642,0.930275229,
0.937614679,0.944954128,0.952293578,0.957798165,0.963302752,0.968807339,
0.974311927,0.979816514,0.988990826,0.994495413,1.),.UNSPECIFIED.);
#24395=B_SPLINE_CURVE_WITH_KNOTS('',5,(#217903,#217904,#217905,#217906,
#217907,#217908,#217909,#217910,#217911,#217912,#217913,#217914,#217915,
#217916,#217917,#217918,#217919,#217920,#217921,#217922,#217923,#217924,
#217925,#217926,#217927,#217928,#217929,#217930,#217931,#217932,#217933,
#217934,#217935,#217936,#217937,#217938,#217939,#217940,#217941,#217942,
#217943,#217944,#217945,#217946,#217947,#217948,#217949,#217950,#217951,
#217952,#217953,#217954,#217955,#217956,#217957,#217958,#217959,#217960,
#217961,#217962,#217963,#217964,#217965,#217966,#217967,#217968,#217969,
#217970,#217971,#217972,#217973,#217974,#217975,#217976,#217977,#217978,
#217979,#217980,#217981,#217982,#217983,#217984,#217985,#217986,#217987,
#217988,#217989,#217990,#217991,#217992,#217993,#217994,#217995,#217996,
#217997,#217998,#217999,#218000,#218001,#218002,#218003,#218004,#218005,
#218006,#218007,#218008,#218009,#218010,#218011,#218012,#218013,#218014,
#218015,#218016,#218017,#218018,#218019,#218020,#218021,#218022,#218023,
#218024,#218025,#218026,#218027,#218028,#218029,#218030,#218031,#218032,
#218033,#218034,#218035,#218036,#218037,#218038,#218039,#218040,#218041,
#218042,#218043,#218044,#218045,#218046,#218047,#218048,#218049,#218050,
#218051,#218052,#218053,#218054,#218055,#218056,#218057,#218058,#218059,
#218060,#218061,#218062,#218063,#218064,#218065,#218066,#218067,#218068,
#218069,#218070,#218071,#218072,#218073,#218074,#218075,#218076,#218077,
#218078,#218079,#218080,#218081,#218082,#218083,#218084,#218085,#218086,
#218087,#218088,#218089,#218090,#218091,#218092,#218093,#218094,#218095,
#218096,#218097,#218098,#218099,#218100,#218101,#218102,#218103,#218104,
#218105,#218106,#218107,#218108,#218109,#218110,#218111,#218112,#218113,
#218114,#218115,#218116,#218117,#218118,#218119,#218120,#218121,#218122,
#218123,#218124,#218125,#218126,#218127,#218128,#218129,#218130,#218131,
#218132,#218133,#218134,#218135,#218136,#218137,#218138,#218139,#218140,
#218141,#218142,#218143,#218144,#218145,#218146,#218147,#218148,#218149,
#218150,#218151,#218152,#218153,#218154,#218155,#218156,#218157,#218158,
#218159,#218160,#218161,#218162,#218163,#218164,#218165,#218166,#218167,
#218168,#218169,#218170,#218171,#218172,#218173,#218174,#218175,#218176,
#218177,#218178,#218179,#218180,#218181,#218182,#218183,#218184,#218185,
#218186,#218187,#218188,#218189,#218190,#218191,#218192,#218193,#218194,
#218195,#218196,#218197,#218198,#218199,#218200,#218201,#218202,#218203,
#218204,#218205,#218206,#218207,#218208,#218209,#218210,#218211,#218212,
#218213,#218214,#218215,#218216,#218217,#218218,#218219,#218220,#218221,
#218222,#218223,#218224,#218225,#218226,#218227,#218228,#218229,#218230,
#218231,#218232,#218233,#218234,#218235,#218236,#218237,#218238,#218239,
#218240,#218241,#218242,#218243,#218244,#218245,#218246,#218247,#218248,
#218249,#218250,#218251,#218252,#218253,#218254,#218255,#218256,#218257,
#218258,#218259,#218260,#218261,#218262,#218263,#218264,#218265,#218266,
#218267,#218268,#218269,#218270,#218271,#218272,#218273,#218274,#218275,
#218276,#218277,#218278,#218279,#218280,#218281,#218282,#218283,#218284,
#218285,#218286,#218287,#218288,#218289,#218290,#218291,#218292,#218293,
#218294,#218295,#218296,#218297,#218298,#218299,#218300,#218301,#218302,
#218303,#218304,#218305,#218306,#218307,#218308,#218309,#218310,#218311,
#218312,#218313,#218314,#218315,#218316,#218317,#218318,#218319,#218320,
#218321,#218322,#218323,#218324,#218325,#218326,#218327,#218328,#218329,
#218330,#218331,#218332,#218333,#218334,#218335,#218336,#218337,#218338,
#218339,#218340,#218341,#218342,#218343,#218344,#218345,#218346,#218347,
#218348,#218349,#218350,#218351,#218352,#218353,#218354,#218355,#218356,
#218357,#218358,#218359,#218360,#218361,#218362,#218363,#218364,#218365,
#218366,#218367,#218368,#218369,#218370,#218371,#218372,#218373),
 .UNSPECIFIED.,.F.,.F.,(6,1,1,1,1,1,1,1,1,1,1,1,1,1,1,1,1,1,1,1,1,1,1,1,
1,1,1,1,1,1,1,1,1,1,1,1,1,1,1,1,1,1,1,1,1,1,1,1,1,1,1,1,1,1,1,1,1,1,1,1,
1,1,1,1,1,1,1,1,1,1,1,1,1,1,1,1,1,1,1,1,1,1,1,1,1,1,1,1,1,1,1,1,1,1,1,1,
1,1,1,1,1,1,1,1,1,1,1,1,1,1,1,1,1,1,1,1,1,1,1,1,1,1,1,1,1,1,1,1,1,1,1,1,
1,1,1,1,1,1,1,1,1,1,1,1,1,1,1,1,1,1,1,1,1,1,1,1,1,1,1,1,1,1,1,1,1,1,1,1,
1,1,1,1,1,1,1,1,1,1,1,1,1,1,1,1,1,1,1,1,1,1,1,1,1,1,1,1,1,1,1,1,1,1,1,1,
1,1,1,1,1,1,1,1,1,1,1,1,1,1,1,1,1,1,1,1,1,1,1,1,1,1,1,1,1,1,1,1,1,1,1,1,
1,1,1,1,1,1,1,1,1,1,1,1,1,1,1,1,1,1,1,1,1,1,1,1,1,1,1,1,1,1,1,1,1,1,1,1,
1,1,1,1,1,1,1,1,1,1,1,1,1,1,1,1,1,1,1,1,1,1,1,1,1,1,1,1,1,1,1,1,1,1,1,1,
1,1,1,1,1,1,1,1,1,1,1,1,1,1,1,1,1,1,1,1,1,1,1,1,1,1,1,1,1,1,1,1,1,1,1,1,
1,1,1,1,1,1,1,1,1,1,1,1,1,1,1,1,1,1,1,1,1,1,1,1,1,1,1,1,1,1,1,1,1,1,1,1,
1,1,1,1,1,1,1,1,1,1,1,1,1,1,1,1,1,1,1,1,1,1,1,1,1,1,1,1,1,1,1,1,1,1,1,1,
1,1,1,1,1,1,1,1,1,1,1,1,1,1,1,1,1,1,1,1,1,1,1,1,1,1,1,1,1,1,1,1,1,1,1,1,
1,1,1,1,1,1,1,1,1,1,6),(-1.,-0.998165138,-0.996330275,-0.994495413,-0.99266055,
-0.990825688,-0.988990826,-0.987155963,-0.985321101,-0.983486239,-0.981651376,
-0.979816514,-0.977981651,-0.976146789,-0.974311927,-0.972477064,-0.970642202,
-0.968807339,-0.966972477,-0.965137615,-0.963302752,-0.96146789,-0.959633028,
-0.957798165,-0.955963303,-0.95412844,-0.952293578,-0.950458716,-0.948623853,
-0.946788991,-0.944954128,-0.943119266,-0.941284404,-0.939449541,-0.937614679,
-0.935779817,-0.933944954,-0.932110092,-0.930275229,-0.928440367,-0.926605505,
-0.924770642,-0.92293578,-0.921100917,-0.919266055,-0.917431193,-0.91559633,
-0.913761468,-0.911926606,-0.910091743,-0.908256881,-0.906422018,-0.904587156,
-0.902752294,-0.900917431,-0.899082569,-0.897247706,-0.895412844,-0.893577982,
-0.891743119,-0.889908257,-0.888073394,-0.886238532,-0.88440367,-0.882568807,
-0.880733945,-0.878899083,-0.87706422,-0.875229358,-0.873394495,-0.871559633,
-0.869724771,-0.867889908,-0.866055046,-0.864220183,-0.862385321,-0.860550459,
-0.858715596,-0.856880734,-0.855045872,-0.853211009,-0.851376147,-0.849541284,
-0.847706422,-0.84587156,-0.844036697,-0.842201835,-0.840366972,-0.83853211,
-0.836697248,-0.834862385,-0.833027523,-0.831192661,-0.829357798,-0.827522936,
-0.825688073,-0.823853211,-0.822018349,-0.820183486,-0.818348624,-0.816513761,
-0.814678899,-0.812844037,-0.811009174,-0.809174312,-0.80733945,-0.805504587,
-0.803669725,-0.801834862,-0.8,-0.798165138,-0.796330275,-0.794495413,-0.79266055,
-0.790825688,-0.788990826,-0.787155963,-0.785321101,-0.783486239,-0.781651376,
-0.779816514,-0.777981651,-0.776146789,-0.774311927,-0.772477064,-0.770642202,
-0.768807339,-0.766972477,-0.765137615,-0.763302752,-0.76146789,-0.759633028,
-0.757798165,-0.755963303,-0.75412844,-0.752293578,-0.750458716,-0.748623853,
-0.746788991,-0.744954128,-0.743119266,-0.741284404,-0.739449541,-0.737614679,
-0.735779817,-0.733944954,-0.732110092,-0.730275229,-0.728440367,-0.726605505,
-0.724770642,-0.72293578,-0.721100917,-0.719266055,-0.717431193,-0.71559633,
-0.713761468,-0.711926606,-0.710091743,-0.708256881,-0.706422018,-0.704587156,
-0.702752294,-0.700917431,-0.699082569,-0.697247706,-0.695412844,-0.693577982,
-0.691743119,-0.689908257,-0.688073394,-0.686238532,-0.68440367,-0.682568807,
-0.680733945,-0.678899083,-0.67706422,-0.675229358,-0.673394495,-0.671559633,
-0.669724771,-0.667889908,-0.666055046,-0.664220183,-0.662385321,-0.660550459,
-0.658715596,-0.656880734,-0.655045872,-0.653211009,-0.651376147,-0.649541284,
-0.647706422,-0.64587156,-0.644036697,-0.642201835,-0.640366972,-0.63853211,
-0.636697248,-0.634862385,-0.633027523,-0.631192661,-0.629357798,-0.627522936,
-0.625688073,-0.623853211,-0.622018349,-0.618348624,-0.616513761,-0.614678899,
-0.612844037,-0.611009174,-0.609174312,-0.60733945,-0.605504587,-0.603669725,
-0.601834862,-0.6,-0.598165138,-0.596330275,-0.594495413,-0.59266055,-0.590825688,
-0.588990826,-0.587155963,-0.585321101,-0.583486239,-0.581651376,-0.579816514,
-0.577981651,-0.576146789,-0.574311927,-0.572477064,-0.570642202,-0.568807339,
-0.566972477,-0.565137615,-0.563302752,-0.56146789,-0.559633028,-0.557798165,
-0.555963303,-0.55412844,-0.552293578,-0.550458716,-0.548623853,-0.546788991,
-0.544954128,-0.543119266,-0.541284404,-0.539449541,-0.537614679,-0.535779817,
-0.533944954,-0.532110092,-0.530275229,-0.528440367,-0.526605505,-0.524770642,
-0.52293578,-0.521100917,-0.519266055,-0.517431193,-0.51559633,-0.513761468,
-0.511926606,-0.510091743,-0.508256881,-0.506422018,-0.504587156,-0.502752294,
-0.500917431,-0.499082569,-0.497247706,-0.495412844,-0.493577982,-0.491743119,
-0.489908257,-0.488073394,-0.486238532,-0.48440367,-0.482568807,-0.480733945,
-0.478899083,-0.47706422,-0.475229358,-0.473394495,-0.471559633,-0.469724771,
-0.467889908,-0.466055046,-0.464220183,-0.462385321,-0.460550459,-0.458715596,
-0.456880734,-0.455045872,-0.453211009,-0.451376147,-0.449541284,-0.447706422,
-0.44587156,-0.444036697,-0.442201835,-0.440366972,-0.43853211,-0.436697248,
-0.434862385,-0.433027523,-0.431192661,-0.429357798,-0.427522936,-0.425688073,
-0.423853211,-0.422018349,-0.420183486,-0.418348624,-0.416513761,-0.414678899,
-0.412844037,-0.411009174,-0.409174312,-0.40733945,-0.405504587,-0.403669725,
-0.401834862,-0.4,-0.398165138,-0.396330275,-0.394495413,-0.39266055,-0.390825688,
-0.388990826,-0.387155963,-0.385321101,-0.383486239,-0.381651376,-0.379816514,
-0.377981651,-0.376146789,-0.374311927,-0.372477064,-0.370642202,-0.368807339,
-0.366972477,-0.365137615,-0.363302752,-0.36146789,-0.359633028,-0.357798165,
-0.355963303,-0.35412844,-0.352293578,-0.350458716,-0.348623853,-0.346788991,
-0.344954128,-0.343119266,-0.341284404,-0.339449541,-0.337614679,-0.335779817,
-0.333944954,-0.332110092,-0.330275229,-0.328440367,-0.326605505,-0.324770642,
-0.32293578,-0.321100917,-0.319266055,-0.317431193,-0.31559633,-0.313761468,
-0.311926606,-0.310091743,-0.308256881,-0.306422018,-0.304587156,-0.302752294,
-0.300917431,-0.299082569,-0.297247706,-0.295412844,-0.293577982,-0.291743119,
-0.289908257,-0.288073394,-0.286238532,-0.28440367,-0.282568807,-0.280733945,
-0.278899083,-0.27706422,-0.275229358,-0.273394495,-0.271559633,-0.269724771,
-0.267889908,-0.266055046,-0.264220183,-0.262385321,-0.260550459,-0.258715596,
-0.256880734,-0.255045872,-0.253211009,-0.251376147,-0.249541284,-0.247706422,
-0.24587156,-0.244036697,-0.242201835,-0.240366972,-0.23853211,-0.236697248,
-0.234862385,-0.233027523,-0.231192661,-0.229357798,-0.227522936,-0.225688073,
-0.223853211,-0.222018349,-0.220183486,-0.218348624,-0.216513761,-0.214678899,
-0.212844037,-0.211009174,-0.209174312,-0.20733945,-0.205504587,-0.203669725,
-0.201834862,-0.2,-0.198165138,-0.196330275,-0.194495413,-0.19266055,-0.190825688,
-0.188990826,-0.187155963,-0.185321101,-0.183486239,-0.181651376,-0.179816514,
-0.177981651,-0.176146789,-0.174311927,-0.172477064,-0.170642202,-0.168807339,
-0.166972477,-0.165137615,-0.163302752,-0.16146789,-0.159633028,-0.157798165,
-0.155963303,-0.15412844,-0.152293578,-0.150458716,-0.148623853,-0.146788991,
-0.144954128,-0.143172102),.UNSPECIFIED.);
#24396=B_SPLINE_CURVE_WITH_KNOTS('',5,(#218374,#218375,#218376,#218377,
#218378,#218379,#218380,#218381,#218382,#218383,#218384,#218385,#218386,
#218387,#218388,#218389,#218390,#218391,#218392,#218393,#218394,#218395,
#218396,#218397,#218398,#218399,#218400,#218401,#218402,#218403,#218404,
#218405,#218406,#218407,#218408,#218409,#218410,#218411,#218412,#218413,
#218414,#218415,#218416,#218417,#218418,#218419,#218420,#218421,#218422,
#218423,#218424,#218425,#218426,#218427,#218428,#218429,#218430,#218431,
#218432,#218433,#218434,#218435,#218436,#218437,#218438,#218439,#218440,
#218441,#218442,#218443,#218444,#218445,#218446,#218447,#218448,#218449,
#218450,#218451,#218452,#218453,#218454,#218455,#218456,#218457,#218458,
#218459,#218460,#218461,#218462,#218463,#218464,#218465,#218466,#218467,
#218468,#218469,#218470,#218471,#218472,#218473,#218474,#218475,#218476,
#218477,#218478,#218479,#218480,#218481,#218482,#218483,#218484,#218485,
#218486,#218487,#218488,#218489,#218490,#218491,#218492,#218493,#218494,
#218495,#218496,#218497,#218498,#218499,#218500,#218501,#218502,#218503,
#218504,#218505,#218506,#218507,#218508,#218509,#218510,#218511,#218512,
#218513,#218514,#218515,#218516,#218517,#218518,#218519,#218520,#218521,
#218522,#218523,#218524,#218525,#218526,#218527,#218528,#218529,#218530,
#218531,#218532,#218533,#218534,#218535,#218536,#218537,#218538,#218539,
#218540,#218541,#218542,#218543,#218544,#218545,#218546,#218547,#218548,
#218549,#218550,#218551,#218552,#218553,#218554,#218555,#218556,#218557,
#218558,#218559,#218560,#218561,#218562,#218563,#218564,#218565,#218566,
#218567,#218568,#218569,#218570,#218571,#218572,#218573,#218574,#218575,
#218576,#218577,#218578,#218579,#218580,#218581,#218582,#218583,#218584,
#218585,#218586,#218587,#218588,#218589,#218590,#218591,#218592,#218593,
#218594,#218595,#218596,#218597,#218598,#218599,#218600,#218601,#218602,
#218603,#218604,#218605,#218606,#218607,#218608,#218609,#218610,#218611,
#218612,#218613,#218614,#218615,#218616,#218617,#218618,#218619,#218620,
#218621,#218622,#218623,#218624,#218625,#218626,#218627,#218628,#218629,
#218630,#218631,#218632,#218633,#218634,#218635,#218636,#218637,#218638,
#218639,#218640,#218641,#218642,#218643,#218644,#218645,#218646,#218647,
#218648,#218649,#218650,#218651,#218652,#218653,#218654,#218655,#218656,
#218657,#218658,#218659,#218660,#218661,#218662,#218663,#218664,#218665,
#218666,#218667,#218668,#218669,#218670,#218671,#218672,#218673,#218674,
#218675,#218676,#218677,#218678,#218679,#218680,#218681,#218682,#218683,
#218684,#218685,#218686,#218687,#218688,#218689,#218690,#218691,#218692,
#218693,#218694,#218695,#218696,#218697,#218698,#218699,#218700,#218701,
#218702,#218703,#218704,#218705,#218706,#218707,#218708,#218709,#218710,
#218711,#218712,#218713,#218714,#218715,#218716,#218717,#218718,#218719,
#218720,#218721,#218722,#218723,#218724,#218725,#218726,#218727,#218728,
#218729,#218730,#218731,#218732,#218733,#218734,#218735,#218736,#218737,
#218738,#218739,#218740,#218741,#218742,#218743,#218744,#218745,#218746,
#218747,#218748,#218749,#218750,#218751,#218752,#218753,#218754,#218755,
#218756,#218757,#218758,#218759,#218760,#218761,#218762,#218763,#218764,
#218765,#218766,#218767,#218768,#218769,#218770,#218771,#218772,#218773,
#218774,#218775,#218776,#218777,#218778,#218779,#218780,#218781,#218782,
#218783,#218784,#218785,#218786,#218787,#218788,#218789,#218790,#218791,
#218792,#218793,#218794,#218795,#218796,#218797,#218798,#218799,#218800,
#218801,#218802,#218803,#218804,#218805,#218806,#218807,#218808,#218809,
#218810,#218811,#218812,#218813,#218814,#218815,#218816,#218817,#218818,
#218819,#218820,#218821,#218822,#218823,#218824,#218825,#218826,#218827,
#218828,#218829,#218830,#218831,#218832,#218833,#218834,#218835,#218836,
#218837,#218838,#218839,#218840,#218841,#218842,#218843,#218844),
 .UNSPECIFIED.,.F.,.F.,(6,1,1,1,1,1,1,1,1,1,1,1,1,1,1,1,1,1,1,1,1,1,1,1,
1,1,1,1,1,1,1,1,1,1,1,1,1,1,1,1,1,1,1,1,1,1,1,1,1,1,1,1,1,1,1,1,1,1,1,1,
1,1,1,1,1,1,1,1,1,1,1,1,1,1,1,1,1,1,1,1,1,1,1,1,1,1,1,1,1,1,1,1,1,1,1,1,
1,1,1,1,1,1,1,1,1,1,1,1,1,1,1,1,1,1,1,1,1,1,1,1,1,1,1,1,1,1,1,1,1,1,1,1,
1,1,1,1,1,1,1,1,1,1,1,1,1,1,1,1,1,1,1,1,1,1,1,1,1,1,1,1,1,1,1,1,1,1,1,1,
1,1,1,1,1,1,1,1,1,1,1,1,1,1,1,1,1,1,1,1,1,1,1,1,1,1,1,1,1,1,1,1,1,1,1,1,
1,1,1,1,1,1,1,1,1,1,1,1,1,1,1,1,1,1,1,1,1,1,1,1,1,1,1,1,1,1,1,1,1,1,1,1,
1,1,1,1,1,1,1,1,1,1,1,1,1,1,1,1,1,1,1,1,1,1,1,1,1,1,1,1,1,1,1,1,1,1,1,1,
1,1,1,1,1,1,1,1,1,1,1,1,1,1,1,1,1,1,1,1,1,1,1,1,1,1,1,1,1,1,1,1,1,1,1,1,
1,1,1,1,1,1,1,1,1,1,1,1,1,1,1,1,1,1,1,1,1,1,1,1,1,1,1,1,1,1,1,1,1,1,1,1,
1,1,1,1,1,1,1,1,1,1,1,1,1,1,1,1,1,1,1,1,1,1,1,1,1,1,1,1,1,1,1,1,1,1,1,1,
1,1,1,1,1,1,1,1,1,1,1,1,1,1,1,1,1,1,1,1,1,1,1,1,1,1,1,1,1,1,1,1,1,1,1,1,
1,1,1,1,1,1,1,1,1,1,1,1,1,1,1,1,1,1,1,1,1,1,1,1,1,1,1,1,1,1,1,1,1,1,1,1,
1,1,1,1,1,1,1,1,1,1,6),(0.143172102,0.144954128,0.146788991,0.148623853,
0.150458716,0.152293578,0.15412844,0.155963303,0.157798165,0.159633028,
0.16146789,0.163302752,0.165137615,0.166972477,0.168807339,0.170642202,
0.172477064,0.174311927,0.176146789,0.177981651,0.179816514,0.181651376,
0.183486239,0.185321101,0.187155963,0.188990826,0.190825688,0.19266055,
0.194495413,0.196330275,0.198165138,0.2,0.201834862,0.203669725,0.205504587,
0.20733945,0.209174312,0.211009174,0.212844037,0.214678899,0.216513761,
0.218348624,0.220183486,0.222018349,0.223853211,0.225688073,0.227522936,
0.229357798,0.231192661,0.233027523,0.234862385,0.236697248,0.23853211,
0.240366972,0.242201835,0.244036697,0.24587156,0.247706422,0.249541284,
0.251376147,0.253211009,0.255045872,0.256880734,0.258715596,0.260550459,
0.262385321,0.264220183,0.266055046,0.267889908,0.269724771,0.271559633,
0.273394495,0.275229358,0.27706422,0.278899083,0.280733945,0.282568807,
0.28440367,0.286238532,0.288073394,0.289908257,0.291743119,0.293577982,
0.295412844,0.297247706,0.299082569,0.300917431,0.302752294,0.304587156,
0.306422018,0.308256881,0.310091743,0.311926606,0.313761468,0.31559633,
0.317431193,0.319266055,0.321100917,0.32293578,0.324770642,0.326605505,
0.328440367,0.330275229,0.332110092,0.333944954,0.335779817,0.337614679,
0.339449541,0.341284404,0.343119266,0.344954128,0.346788991,0.348623853,
0.350458716,0.352293578,0.35412844,0.355963303,0.357798165,0.359633028,
0.36146789,0.363302752,0.365137615,0.366972477,0.368807339,0.370642202,
0.372477064,0.374311927,0.376146789,0.377981651,0.379816514,0.381651376,
0.383486239,0.385321101,0.387155963,0.388990826,0.390825688,0.39266055,
0.394495413,0.396330275,0.398165138,0.4,0.401834862,0.403669725,0.405504587,
0.40733945,0.409174312,0.411009174,0.412844037,0.414678899,0.416513761,
0.418348624,0.420183486,0.422018349,0.423853211,0.425688073,0.427522936,
0.429357798,0.431192661,0.433027523,0.434862385,0.436697248,0.43853211,
0.440366972,0.442201835,0.444036697,0.44587156,0.447706422,0.449541284,
0.451376147,0.453211009,0.455045872,0.456880734,0.458715596,0.460550459,
0.462385321,0.464220183,0.466055046,0.467889908,0.469724771,0.471559633,
0.473394495,0.475229358,0.47706422,0.478899083,0.480733945,0.482568807,
0.48440367,0.486238532,0.488073394,0.489908257,0.491743119,0.493577982,
0.495412844,0.497247706,0.499082569,0.500917431,0.502752294,0.504587156,
0.506422018,0.508256881,0.510091743,0.511926606,0.513761468,0.51559633,
0.517431193,0.519266055,0.521100917,0.52293578,0.524770642,0.526605505,
0.528440367,0.530275229,0.532110092,0.533944954,0.535779817,0.537614679,
0.539449541,0.541284404,0.543119266,0.544954128,0.546788991,0.548623853,
0.550458716,0.552293578,0.55412844,0.555963303,0.557798165,0.559633028,
0.56146789,0.563302752,0.565137615,0.566972477,0.568807339,0.570642202,
0.572477064,0.574311927,0.576146789,0.577981651,0.579816514,0.581651376,
0.583486239,0.585321101,0.587155963,0.588990826,0.590825688,0.59266055,
0.594495413,0.596330275,0.598165138,0.6,0.601834862,0.603669725,0.605504587,
0.60733945,0.609174312,0.611009174,0.612844037,0.614678899,0.616513761,
0.618348624,0.622018349,0.623853211,0.625688073,0.627522936,0.629357798,
0.631192661,0.633027523,0.634862385,0.636697248,0.63853211,0.640366972,
0.642201835,0.644036697,0.64587156,0.647706422,0.649541284,0.651376147,
0.653211009,0.655045872,0.656880734,0.658715596,0.660550459,0.662385321,
0.664220183,0.666055046,0.667889908,0.669724771,0.671559633,0.673394495,
0.675229358,0.67706422,0.678899083,0.680733945,0.682568807,0.68440367,0.686238532,
0.688073394,0.689908257,0.691743119,0.693577982,0.695412844,0.697247706,
0.699082569,0.700917431,0.702752294,0.704587156,0.706422018,0.708256881,
0.710091743,0.711926606,0.713761468,0.71559633,0.717431193,0.719266055,
0.721100917,0.72293578,0.724770642,0.726605505,0.728440367,0.730275229,
0.732110092,0.733944954,0.735779817,0.737614679,0.739449541,0.741284404,
0.743119266,0.744954128,0.746788991,0.748623853,0.750458716,0.752293578,
0.75412844,0.755963303,0.757798165,0.759633028,0.76146789,0.763302752,0.765137615,
0.766972477,0.768807339,0.770642202,0.772477064,0.774311927,0.776146789,
0.777981651,0.779816514,0.781651376,0.783486239,0.785321101,0.787155963,
0.788990826,0.790825688,0.79266055,0.794495413,0.796330275,0.798165138,
0.8,0.801834862,0.803669725,0.805504587,0.80733945,0.809174312,0.811009174,
0.812844037,0.814678899,0.816513761,0.818348624,0.820183486,0.822018349,
0.823853211,0.825688073,0.827522936,0.829357798,0.831192661,0.833027523,
0.834862385,0.836697248,0.83853211,0.840366972,0.842201835,0.844036697,
0.84587156,0.847706422,0.849541284,0.851376147,0.853211009,0.855045872,
0.856880734,0.858715596,0.860550459,0.862385321,0.864220183,0.866055046,
0.867889908,0.869724771,0.871559633,0.873394495,0.875229358,0.87706422,
0.878899083,0.880733945,0.882568807,0.88440367,0.886238532,0.888073394,
0.889908257,0.891743119,0.893577982,0.895412844,0.897247706,0.899082569,
0.900917431,0.902752294,0.904587156,0.906422018,0.908256881,0.910091743,
0.911926606,0.913761468,0.91559633,0.917431193,0.919266055,0.921100917,
0.92293578,0.924770642,0.926605505,0.928440367,0.930275229,0.932110092,
0.933944954,0.935779817,0.937614679,0.939449541,0.941284404,0.943119266,
0.944954128,0.946788991,0.948623853,0.950458716,0.952293578,0.95412844,
0.955963303,0.957798165,0.959633028,0.96146789,0.963302752,0.965137615,
0.966972477,0.968807339,0.970642202,0.972477064,0.974311927,0.976146789,
0.977981651,0.979816514,0.981651376,0.983486239,0.985321101,0.987155963,
0.988990826,0.990825688,0.99266055,0.994495413,0.996330275,0.998165138,
1.),.UNSPECIFIED.);
#24397=B_SPLINE_CURVE_WITH_KNOTS('',3,(#219789,#219790,#219791,#219792,
#219793,#219794,#219795,#219796,#219797,#219798,#219799,#219800,#219801,
#219802,#219803,#219804,#219805,#219806,#219807,#219808,#219809,#219810,
#219811,#219812,#219813,#219814,#219815,#219816,#219817,#219818,#219819,
#219820,#219821,#219822,#219823,#219824,#219825,#219826,#219827,#219828,
#219829,#219830,#219831,#219832,#219833,#219834,#219835,#219836,#219837,
#219838,#219839,#219840,#219841,#219842,#219843,#219844,#219845,#219846,
#219847,#219848,#219849,#219850,#219851,#219852,#219853,#219854,#219855,
#219856,#219857,#219858,#219859,#219860,#219861,#219862,#219863,#219864,
#219865,#219866,#219867,#219868,#219869,#219870,#219871,#219872,#219873,
#219874,#219875,#219876,#219877,#219878,#219879,#219880,#219881,#219882,
#219883,#219884,#219885,#219886,#219887,#219888,#219889,#219890,#219891,
#219892,#219893,#219894,#219895,#219896,#219897,#219898,#219899,#219900,
#219901,#219902,#219903,#219904,#219905,#219906,#219907,#219908,#219909,
#219910,#219911,#219912,#219913,#219914,#219915,#219916,#219917,#219918,
#219919,#219920,#219921,#219922,#219923,#219924,#219925,#219926,#219927,
#219928,#219929,#219930,#219931,#219932,#219933,#219934,#219935,#219936,
#219937,#219938,#219939,#219940,#219941,#219942,#219943,#219944,#219945,
#219946,#219947,#219948,#219949,#219950,#219951,#219952,#219953,#219954,
#219955,#219956,#219957,#219958,#219959,#219960,#219961,#219962,#219963,
#219964,#219965,#219966,#219967,#219968,#219969,#219970,#219971,#219972,
#219973,#219974,#219975,#219976,#219977,#219978,#219979,#219980,#219981,
#219982,#219983,#219984,#219985,#219986,#219987,#219988,#219989,#219990,
#219991,#219992,#219993,#219994,#219995,#219996,#219997,#219998,#219999,
#220000,#220001,#220002,#220003,#220004,#220005,#220006,#220007,#220008,
#220009,#220010,#220011,#220012,#220013,#220014,#220015,#220016,#220017,
#220018,#220019,#220020,#220021,#220022,#220023,#220024,#220025,#220026,
#220027,#220028,#220029,#220030,#220031,#220032,#220033,#220034,#220035,
#220036,#220037,#220038,#220039,#220040,#220041,#220042,#220043,#220044,
#220045,#220046,#220047,#220048,#220049,#220050,#220051,#220052,#220053,
#220054,#220055,#220056,#220057,#220058,#220059,#220060,#220061,#220062,
#220063,#220064,#220065,#220066,#220067,#220068,#220069,#220070,#220071,
#220072,#220073,#220074,#220075,#220076,#220077,#220078,#220079,#220080,
#220081,#220082,#220083,#220084,#220085,#220086,#220087,#220088,#220089),
 .UNSPECIFIED.,.F.,.F.,(4,3,3,3,3,3,3,3,3,3,3,3,3,3,3,3,3,3,3,3,3,3,3,3,
3,3,3,3,3,3,3,3,3,3,3,3,3,3,3,3,3,3,3,3,3,3,3,3,3,3,3,3,3,3,3,3,3,3,3,3,
3,3,3,3,3,3,3,3,3,3,3,3,3,3,3,3,3,3,3,3,3,3,3,3,3,3,3,3,3,3,3,3,3,3,3,3,
3,3,3,3,4),(0.143172102,0.15412844,0.165137615,0.176146789,0.187155963,
0.198165138,0.209174312,0.220183486,0.231192661,0.242201835,0.253211009,
0.264220183,0.275229358,0.286238532,0.297247706,0.308256881,0.319266055,
0.330275229,0.343119266,0.35412844,0.365137615,0.376146789,0.387155963,
0.396330275,0.405504587,0.416513761,0.425688073,0.436697248,0.44587156,
0.455045872,0.464220183,0.473394495,0.48440367,0.499082569,0.511926606,
0.521100917,0.530275229,0.539449541,0.548623853,0.555963303,0.565137615,
0.572477064,0.581651376,0.590825688,0.598165138,0.605504587,0.614678899,
0.622018349,0.629357798,0.63853211,0.647706422,0.655045872,0.667889908,
0.678899083,0.686238532,0.693577982,0.700917431,0.710091743,0.717431193,
0.726605505,0.733944954,0.741284404,0.748623853,0.757798165,0.770642202,
0.779816514,0.79266055,0.8,0.80733945,0.812844037,0.818348624,0.823853211,
0.831192661,0.836697248,0.844036697,0.849541284,0.855045872,0.862385321,
0.867889908,0.873394495,0.878899083,0.88440367,0.889908257,0.895412844,
0.900917431,0.906422018,0.911926606,0.917431193,0.924770642,0.930275229,
0.935779817,0.941284404,0.950458716,0.955963303,0.96146789,0.966972477,
0.972477064,0.979816514,0.985321101,0.994495413,1.),.UNSPECIFIED.);
#24398=B_SPLINE_CURVE_WITH_KNOTS('',3,(#220090,#220091,#220092,#220093,
#220094,#220095,#220096,#220097,#220098,#220099,#220100,#220101,#220102,
#220103,#220104,#220105,#220106,#220107,#220108,#220109,#220110,#220111,
#220112,#220113,#220114,#220115,#220116,#220117,#220118,#220119,#220120,
#220121,#220122,#220123,#220124,#220125,#220126,#220127,#220128,#220129,
#220130,#220131,#220132,#220133,#220134,#220135,#220136,#220137,#220138,
#220139,#220140,#220141,#220142,#220143,#220144,#220145,#220146,#220147,
#220148,#220149,#220150,#220151,#220152,#220153,#220154,#220155,#220156,
#220157,#220158,#220159,#220160,#220161,#220162,#220163,#220164,#220165,
#220166,#220167,#220168,#220169,#220170,#220171,#220172,#220173,#220174,
#220175,#220176,#220177,#220178,#220179,#220180,#220181,#220182,#220183,
#220184,#220185,#220186,#220187,#220188,#220189,#220190,#220191,#220192,
#220193,#220194,#220195,#220196,#220197,#220198,#220199,#220200,#220201,
#220202,#220203,#220204,#220205,#220206,#220207,#220208,#220209,#220210,
#220211,#220212,#220213,#220214,#220215,#220216,#220217,#220218,#220219,
#220220,#220221,#220222,#220223,#220224,#220225,#220226,#220227,#220228,
#220229,#220230,#220231,#220232,#220233,#220234,#220235,#220236,#220237,
#220238,#220239,#220240,#220241,#220242,#220243,#220244,#220245,#220246,
#220247,#220248,#220249,#220250,#220251,#220252,#220253,#220254,#220255,
#220256,#220257,#220258,#220259,#220260,#220261,#220262,#220263,#220264,
#220265,#220266,#220267,#220268,#220269,#220270,#220271,#220272,#220273,
#220274,#220275,#220276,#220277,#220278,#220279,#220280,#220281,#220282,
#220283,#220284,#220285,#220286,#220287,#220288,#220289,#220290,#220291,
#220292,#220293,#220294,#220295,#220296,#220297,#220298,#220299,#220300,
#220301,#220302,#220303,#220304,#220305,#220306,#220307,#220308,#220309,
#220310,#220311,#220312,#220313,#220314,#220315,#220316,#220317,#220318,
#220319,#220320,#220321,#220322,#220323,#220324,#220325,#220326,#220327,
#220328,#220329,#220330,#220331,#220332,#220333,#220334,#220335,#220336,
#220337,#220338,#220339,#220340,#220341,#220342,#220343,#220344,#220345,
#220346,#220347,#220348,#220349,#220350,#220351,#220352,#220353,#220354,
#220355,#220356,#220357,#220358,#220359,#220360,#220361,#220362,#220363,
#220364,#220365,#220366,#220367,#220368,#220369,#220370,#220371,#220372,
#220373,#220374,#220375,#220376,#220377,#220378,#220379,#220380,#220381,
#220382,#220383,#220384,#220385,#220386,#220387,#220388,#220389,#220390,
#220391,#220392,#220393,#220394,#220395,#220396,#220397,#220398,#220399,
#220400,#220401,#220402,#220403,#220404,#220405),.UNSPECIFIED.,.F.,.F.,
(4,3,3,3,3,3,3,3,3,3,3,3,3,3,3,3,3,3,3,3,3,3,3,3,3,3,3,3,3,3,3,3,3,3,3,
3,3,3,3,3,3,3,3,3,3,3,3,3,3,3,3,3,3,3,3,3,3,3,3,3,3,3,3,3,3,3,3,3,3,3,3,
3,3,3,3,3,3,3,3,3,3,3,3,3,3,3,3,3,3,3,3,3,3,3,3,3,3,3,3,3,3,3,3,3,3,4),
(0.143172102,0.15412844,0.165137615,0.176146789,0.187155963,0.198165138,
0.209174312,0.220183486,0.231192661,0.242201835,0.253211009,0.264220183,
0.275229358,0.286238532,0.297247706,0.308256881,0.319266055,0.330275229,
0.341284404,0.352293578,0.363302752,0.374311927,0.385321101,0.396330275,
0.405504587,0.416513761,0.425688073,0.434862385,0.444036697,0.453211009,
0.462385321,0.471559633,0.480733945,0.489908257,0.499082569,0.510091743,
0.519266055,0.528440367,0.535779817,0.543119266,0.550458716,0.557798165,
0.565137615,0.572477064,0.581651376,0.588990826,0.596330275,0.603669725,
0.611009174,0.618348624,0.625688073,0.633027523,0.640366972,0.647706422,
0.655045872,0.662385321,0.669724771,0.67706422,0.68440367,0.691743119,0.700917431,
0.710091743,0.717431193,0.724770642,0.733944954,0.741284404,0.748623853,
0.755963303,0.763302752,0.770642202,0.777981651,0.785321101,0.79266055,
0.8,0.809174312,0.816513761,0.822018349,0.827522936,0.834862385,0.842201835,
0.847706422,0.853211009,0.858715596,0.864220183,0.869724771,0.875229358,
0.880733945,0.888073394,0.893577982,0.900917431,0.906422018,0.911926606,
0.917431193,0.924770642,0.930275229,0.937614679,0.943119266,0.948623853,
0.95412844,0.96146789,0.968807339,0.974311927,0.979816514,0.987155963,0.994495413,
1.),.UNSPECIFIED.);
#24399=B_SPLINE_CURVE_WITH_KNOTS('',3,(#221365,#221366,#221367,#221368,
#221369,#221370,#221371,#221372,#221373,#221374,#221375,#221376,#221377,
#221378,#221379,#221380,#221381,#221382,#221383,#221384,#221385,#221386,
#221387,#221388,#221389,#221390,#221391,#221392,#221393,#221394,#221395,
#221396,#221397,#221398,#221399,#221400,#221401,#221402,#221403,#221404,
#221405,#221406,#221407,#221408,#221409,#221410,#221411,#221412,#221413,
#221414,#221415,#221416,#221417,#221418,#221419,#221420,#221421,#221422,
#221423,#221424,#221425,#221426,#221427,#221428,#221429,#221430,#221431,
#221432,#221433,#221434,#221435,#221436,#221437,#221438,#221439,#221440,
#221441,#221442,#221443,#221444,#221445,#221446,#221447,#221448,#221449,
#221450,#221451,#221452,#221453,#221454,#221455,#221456,#221457,#221458,
#221459,#221460,#221461,#221462,#221463,#221464,#221465,#221466,#221467,
#221468,#221469,#221470,#221471,#221472,#221473,#221474,#221475,#221476,
#221477,#221478,#221479,#221480,#221481,#221482,#221483,#221484,#221485,
#221486,#221487,#221488,#221489,#221490,#221491,#221492,#221493,#221494,
#221495,#221496,#221497,#221498,#221499,#221500,#221501,#221502,#221503,
#221504,#221505,#221506,#221507,#221508,#221509,#221510,#221511,#221512,
#221513,#221514,#221515,#221516,#221517,#221518,#221519,#221520,#221521,
#221522,#221523,#221524,#221525,#221526,#221527,#221528,#221529,#221530,
#221531,#221532,#221533,#221534,#221535,#221536,#221537,#221538,#221539,
#221540,#221541,#221542,#221543,#221544,#221545,#221546,#221547,#221548,
#221549,#221550,#221551,#221552,#221553,#221554,#221555,#221556,#221557,
#221558,#221559,#221560,#221561,#221562,#221563,#221564,#221565,#221566,
#221567,#221568,#221569,#221570,#221571,#221572,#221573,#221574,#221575,
#221576,#221577,#221578,#221579,#221580,#221581,#221582,#221583,#221584,
#221585,#221586,#221587,#221588,#221589,#221590,#221591,#221592,#221593,
#221594,#221595,#221596,#221597,#221598,#221599,#221600,#221601,#221602,
#221603,#221604,#221605,#221606,#221607,#221608,#221609,#221610,#221611,
#221612,#221613,#221614,#221615,#221616,#221617,#221618,#221619,#221620,
#221621,#221622,#221623,#221624,#221625,#221626,#221627,#221628,#221629,
#221630,#221631,#221632,#221633,#221634,#221635,#221636,#221637,#221638,
#221639,#221640,#221641,#221642,#221643,#221644,#221645,#221646,#221647,
#221648,#221649,#221650,#221651,#221652,#221653,#221654,#221655,#221656),
 .UNSPECIFIED.,.F.,.F.,(4,3,3,3,3,3,3,3,3,3,3,3,3,3,3,3,3,3,3,3,3,3,3,3,
3,3,3,3,3,3,3,3,3,3,3,3,3,3,3,3,3,3,3,3,3,3,3,3,3,3,3,3,3,3,3,3,3,3,3,3,
3,3,3,3,3,3,3,3,3,3,3,3,3,3,3,3,3,3,3,3,3,3,3,3,3,3,3,3,3,3,3,3,3,3,3,3,
3,4),(0.143172102,0.15412844,0.165137615,0.176146789,0.187155963,0.198165138,
0.209174312,0.220183486,0.231192661,0.242201835,0.253211009,0.264220183,
0.275229358,0.288073394,0.300917431,0.311926606,0.32293578,0.333944954,
0.344954128,0.357798165,0.368807339,0.379816514,0.39266055,0.401834862,
0.412844037,0.422018349,0.431192661,0.440366972,0.449541284,0.458715596,
0.469724771,0.478899083,0.488073394,0.497247706,0.508256881,0.519266055,
0.530275229,0.537614679,0.550458716,0.56146789,0.572477064,0.581651376,
0.588990826,0.598165138,0.605504587,0.612844037,0.622018349,0.629357798,
0.636697248,0.644036697,0.653211009,0.660550459,0.669724771,0.67706422,
0.68440367,0.691743119,0.699082569,0.706422018,0.71559633,0.72293578,0.730275229,
0.743119266,0.755963303,0.768807339,0.781651376,0.79266055,0.803669725,
0.811009174,0.816513761,0.822018349,0.831192661,0.836697248,0.842201835,
0.847706422,0.855045872,0.860550459,0.866055046,0.873394495,0.878899083,
0.88440367,0.889908257,0.897247706,0.904587156,0.910091743,0.917431193,
0.92293578,0.928440367,0.933944954,0.939449541,0.946788991,0.952293578,
0.96146789,0.966972477,0.972477064,0.979816514,0.985321101,0.990825688,
1.),.UNSPECIFIED.);
#24400=B_SPLINE_CURVE_WITH_KNOTS('',3,(#221657,#221658,#221659,#221660,
#221661,#221662,#221663,#221664,#221665,#221666,#221667,#221668,#221669,
#221670,#221671,#221672,#221673,#221674,#221675,#221676,#221677,#221678,
#221679,#221680,#221681,#221682,#221683,#221684,#221685,#221686,#221687,
#221688,#221689,#221690,#221691,#221692,#221693,#221694,#221695,#221696,
#221697,#221698,#221699,#221700,#221701,#221702,#221703,#221704,#221705,
#221706,#221707,#221708,#221709,#221710,#221711,#221712,#221713,#221714,
#221715,#221716,#221717,#221718,#221719,#221720,#221721,#221722,#221723,
#221724,#221725,#221726,#221727,#221728,#221729,#221730,#221731,#221732,
#221733,#221734,#221735,#221736,#221737,#221738,#221739,#221740,#221741,
#221742,#221743,#221744,#221745,#221746,#221747,#221748,#221749,#221750,
#221751,#221752,#221753,#221754,#221755,#221756,#221757,#221758,#221759,
#221760,#221761,#221762,#221763,#221764,#221765,#221766,#221767,#221768,
#221769,#221770,#221771,#221772,#221773,#221774,#221775,#221776,#221777,
#221778,#221779,#221780,#221781,#221782,#221783,#221784,#221785,#221786,
#221787,#221788,#221789,#221790,#221791,#221792,#221793,#221794,#221795,
#221796,#221797,#221798,#221799,#221800,#221801,#221802,#221803,#221804,
#221805,#221806,#221807,#221808,#221809,#221810,#221811,#221812,#221813,
#221814,#221815,#221816,#221817,#221818,#221819,#221820,#221821,#221822,
#221823,#221824,#221825,#221826,#221827,#221828,#221829,#221830,#221831,
#221832,#221833,#221834,#221835,#221836,#221837,#221838,#221839,#221840,
#221841,#221842,#221843,#221844,#221845,#221846,#221847,#221848,#221849,
#221850,#221851,#221852,#221853,#221854,#221855,#221856,#221857,#221858,
#221859,#221860,#221861,#221862,#221863,#221864,#221865,#221866,#221867,
#221868,#221869,#221870,#221871,#221872,#221873,#221874,#221875,#221876,
#221877,#221878,#221879,#221880,#221881,#221882,#221883,#221884,#221885,
#221886,#221887,#221888,#221889,#221890,#221891,#221892,#221893,#221894,
#221895,#221896,#221897,#221898,#221899,#221900,#221901,#221902,#221903,
#221904,#221905,#221906,#221907,#221908,#221909,#221910,#221911,#221912,
#221913,#221914,#221915,#221916,#221917,#221918,#221919,#221920,#221921,
#221922,#221923,#221924,#221925,#221926,#221927,#221928,#221929,#221930,
#221931,#221932,#221933,#221934,#221935,#221936,#221937,#221938,#221939,
#221940,#221941,#221942,#221943,#221944,#221945,#221946,#221947,#221948,
#221949,#221950,#221951,#221952,#221953,#221954,#221955,#221956,#221957,
#221958,#221959,#221960,#221961,#221962,#221963,#221964,#221965,#221966,
#221967,#221968,#221969,#221970,#221971,#221972,#221973,#221974,#221975),
 .UNSPECIFIED.,.F.,.F.,(4,3,3,3,3,3,3,3,3,3,3,3,3,3,3,3,3,3,3,3,3,3,3,3,
3,3,3,3,3,3,3,3,3,3,3,3,3,3,3,3,3,3,3,3,3,3,3,3,3,3,3,3,3,3,3,3,3,3,3,3,
3,3,3,3,3,3,3,3,3,3,3,3,3,3,3,3,3,3,3,3,3,3,3,3,3,3,3,3,3,3,3,3,3,3,3,3,
3,3,3,3,3,3,3,3,3,3,4),(0.143172102,0.15412844,0.165137615,0.176146789,
0.187155963,0.198165138,0.209174312,0.220183486,0.231192661,0.242201835,
0.253211009,0.264220183,0.275229358,0.288073394,0.300917431,0.311926606,
0.32293578,0.333944954,0.344954128,0.355963303,0.366972477,0.377981651,
0.388990826,0.398165138,0.40733945,0.418348624,0.427522936,0.436697248,
0.44587156,0.456880734,0.466055046,0.475229358,0.488073394,0.497247706,
0.508256881,0.519266055,0.528440367,0.535779817,0.543119266,0.550458716,
0.557798165,0.566972477,0.574311927,0.581651376,0.588990826,0.596330275,
0.603669725,0.611009174,0.618348624,0.625688073,0.633027523,0.640366972,
0.647706422,0.655045872,0.664220183,0.671559633,0.678899083,0.686238532,
0.693577982,0.700917431,0.708256881,0.71559633,0.72293578,0.730275229,0.737614679,
0.744954128,0.752293578,0.759633028,0.768807339,0.776146789,0.783486239,
0.790825688,0.798165138,0.805504587,0.811009174,0.816513761,0.822018349,
0.827522936,0.833027523,0.840366972,0.84587156,0.853211009,0.858715596,
0.864220183,0.869724771,0.875229358,0.882568807,0.888073394,0.893577982,
0.900917431,0.906422018,0.911926606,0.917431193,0.924770642,0.930275229,
0.935779817,0.943119266,0.948623853,0.95412844,0.96146789,0.966972477,0.972477064,
0.977981651,0.983486239,0.988990826,0.994495413,1.),.UNSPECIFIED.);
#24401=B_SPLINE_CURVE_WITH_KNOTS('',3,(#222923,#222924,#222925,#222926,
#222927,#222928,#222929,#222930,#222931,#222932,#222933,#222934,#222935,
#222936,#222937,#222938,#222939,#222940,#222941,#222942,#222943,#222944,
#222945,#222946,#222947,#222948,#222949,#222950,#222951,#222952,#222953,
#222954,#222955,#222956,#222957,#222958,#222959,#222960,#222961,#222962,
#222963,#222964,#222965,#222966,#222967,#222968,#222969,#222970,#222971,
#222972,#222973,#222974,#222975,#222976,#222977,#222978,#222979,#222980,
#222981,#222982,#222983,#222984,#222985,#222986,#222987,#222988,#222989,
#222990,#222991,#222992,#222993,#222994,#222995,#222996,#222997,#222998,
#222999,#223000,#223001,#223002,#223003,#223004,#223005,#223006,#223007,
#223008,#223009,#223010,#223011,#223012,#223013,#223014,#223015,#223016,
#223017,#223018,#223019,#223020,#223021,#223022,#223023,#223024,#223025,
#223026,#223027,#223028,#223029,#223030,#223031,#223032,#223033,#223034,
#223035,#223036,#223037,#223038,#223039,#223040,#223041,#223042,#223043,
#223044,#223045,#223046,#223047,#223048,#223049,#223050,#223051,#223052,
#223053,#223054,#223055,#223056,#223057,#223058,#223059,#223060,#223061,
#223062,#223063,#223064,#223065,#223066,#223067,#223068,#223069,#223070,
#223071,#223072,#223073,#223074,#223075,#223076,#223077,#223078,#223079,
#223080,#223081,#223082,#223083,#223084,#223085,#223086,#223087,#223088,
#223089,#223090,#223091,#223092,#223093,#223094,#223095,#223096,#223097,
#223098,#223099,#223100,#223101,#223102,#223103,#223104,#223105,#223106,
#223107,#223108,#223109,#223110,#223111,#223112,#223113,#223114,#223115,
#223116,#223117,#223118,#223119,#223120,#223121,#223122,#223123,#223124,
#223125,#223126,#223127,#223128,#223129,#223130,#223131,#223132,#223133,
#223134,#223135,#223136,#223137,#223138,#223139,#223140,#223141,#223142,
#223143,#223144,#223145,#223146,#223147,#223148,#223149,#223150,#223151,
#223152,#223153,#223154,#223155,#223156,#223157,#223158,#223159,#223160,
#223161,#223162,#223163,#223164,#223165,#223166,#223167,#223168,#223169,
#223170,#223171,#223172,#223173,#223174,#223175,#223176,#223177,#223178,
#223179,#223180,#223181,#223182,#223183,#223184,#223185,#223186,#223187,
#223188,#223189,#223190,#223191,#223192,#223193,#223194,#223195,#223196,
#223197,#223198,#223199,#223200,#223201,#223202,#223203,#223204,#223205,
#223206,#223207,#223208,#223209,#223210,#223211,#223212,#223213,#223214,
#223215,#223216,#223217,#223218,#223219,#223220,#223221,#223222,#223223,
#223224,#223225,#223226,#223227,#223228,#223229,#223230,#223231,#223232,
#223233,#223234,#223235,#223236,#223237,#223238,#223239,#223240,#223241,
#223242,#223243,#223244,#223245,#223246,#223247),.UNSPECIFIED.,.F.,.F.,
(4,3,3,3,3,3,3,3,3,3,3,3,3,3,3,3,3,3,3,3,3,3,3,3,3,3,3,3,3,3,3,3,3,3,3,
3,3,3,3,3,3,3,3,3,3,3,3,3,3,3,3,3,3,3,3,3,3,3,3,3,3,3,3,3,3,3,3,3,3,3,3,
3,3,3,3,3,3,3,3,3,3,3,3,3,3,3,3,3,3,3,3,3,3,3,3,3,3,3,3,3,3,3,3,3,3,3,3,
3,4),(-1.,-0.99266055,-0.987155963,-0.981651376,-0.976146789,-0.970642202,
-0.965137615,-0.959633028,-0.95412844,-0.948623853,-0.943119266,-0.937614679,
-0.932110092,-0.926605505,-0.921100917,-0.91559633,-0.910091743,-0.904587156,
-0.899082569,-0.893577982,-0.888073394,-0.882568807,-0.87706422,-0.871559633,
-0.866055046,-0.860550459,-0.855045872,-0.849541284,-0.842201835,-0.836697248,
-0.831192661,-0.825688073,-0.818348624,-0.812844037,-0.80733945,-0.8,-0.79266055,
-0.781651376,-0.774311927,-0.766972477,-0.759633028,-0.752293578,-0.744954128,
-0.737614679,-0.730275229,-0.72293578,-0.71559633,-0.708256881,-0.700917431,
-0.693577982,-0.686238532,-0.678899083,-0.671559633,-0.664220183,-0.656880734,
-0.649541284,-0.642201835,-0.634862385,-0.627522936,-0.620183486,-0.612844037,
-0.605504587,-0.598165138,-0.590825688,-0.583486239,-0.576146789,-0.568807339,
-0.56146789,-0.55412844,-0.546788991,-0.539449541,-0.532110092,-0.52293578,
-0.513761468,-0.504587156,-0.495412844,-0.486238532,-0.47706422,-0.467889908,
-0.458715596,-0.449541284,-0.440366972,-0.431192661,-0.422018349,-0.412844037,
-0.403669725,-0.394495413,-0.383486239,-0.372477064,-0.36146789,-0.350458716,
-0.339449541,-0.328440367,-0.317431193,-0.306422018,-0.295412844,-0.28440367,
-0.273394495,-0.262385321,-0.251376147,-0.240366972,-0.229357798,-0.218348624,
-0.20733945,-0.196330275,-0.183486239,-0.172477064,-0.16146789,-0.143172102),
 .UNSPECIFIED.);
#24402=B_SPLINE_CURVE_WITH_KNOTS('',3,(#223248,#223249,#223250,#223251,
#223252,#223253,#223254,#223255,#223256,#223257,#223258,#223259,#223260,
#223261,#223262,#223263,#223264,#223265,#223266,#223267,#223268,#223269,
#223270,#223271,#223272,#223273,#223274,#223275,#223276,#223277,#223278,
#223279,#223280,#223281,#223282,#223283,#223284,#223285,#223286,#223287,
#223288,#223289,#223290,#223291,#223292,#223293,#223294,#223295,#223296,
#223297,#223298,#223299,#223300,#223301,#223302,#223303,#223304,#223305,
#223306,#223307,#223308,#223309,#223310,#223311,#223312,#223313,#223314,
#223315,#223316,#223317,#223318,#223319,#223320,#223321,#223322,#223323,
#223324,#223325,#223326,#223327,#223328,#223329,#223330,#223331,#223332,
#223333,#223334,#223335,#223336,#223337,#223338,#223339,#223340,#223341,
#223342,#223343,#223344,#223345,#223346,#223347,#223348,#223349,#223350,
#223351,#223352,#223353,#223354,#223355,#223356,#223357,#223358,#223359,
#223360,#223361,#223362,#223363,#223364,#223365,#223366,#223367,#223368,
#223369,#223370,#223371,#223372,#223373,#223374,#223375,#223376,#223377,
#223378,#223379,#223380,#223381,#223382,#223383,#223384,#223385,#223386,
#223387,#223388,#223389,#223390,#223391,#223392,#223393,#223394,#223395,
#223396,#223397,#223398,#223399,#223400,#223401,#223402,#223403,#223404,
#223405,#223406,#223407,#223408,#223409,#223410,#223411,#223412,#223413,
#223414,#223415,#223416,#223417,#223418,#223419,#223420,#223421,#223422,
#223423,#223424,#223425,#223426,#223427,#223428,#223429,#223430,#223431,
#223432,#223433,#223434,#223435,#223436,#223437,#223438,#223439,#223440,
#223441,#223442,#223443,#223444,#223445,#223446,#223447,#223448,#223449,
#223450,#223451,#223452,#223453,#223454,#223455,#223456,#223457,#223458,
#223459,#223460,#223461,#223462,#223463,#223464,#223465,#223466,#223467,
#223468,#223469,#223470,#223471,#223472,#223473,#223474,#223475,#223476,
#223477,#223478,#223479,#223480,#223481,#223482,#223483,#223484,#223485,
#223486,#223487,#223488,#223489,#223490,#223491,#223492,#223493,#223494,
#223495,#223496,#223497,#223498,#223499,#223500,#223501,#223502,#223503,
#223504,#223505,#223506,#223507,#223508,#223509,#223510,#223511,#223512,
#223513,#223514,#223515,#223516,#223517,#223518,#223519,#223520,#223521,
#223522,#223523,#223524,#223525,#223526,#223527,#223528,#223529,#223530,
#223531,#223532,#223533,#223534,#223535,#223536,#223537,#223538,#223539,
#223540,#223541,#223542,#223543,#223544,#223545,#223546,#223547,#223548),
 .UNSPECIFIED.,.F.,.F.,(4,3,3,3,3,3,3,3,3,3,3,3,3,3,3,3,3,3,3,3,3,3,3,3,
3,3,3,3,3,3,3,3,3,3,3,3,3,3,3,3,3,3,3,3,3,3,3,3,3,3,3,3,3,3,3,3,3,3,3,3,
3,3,3,3,3,3,3,3,3,3,3,3,3,3,3,3,3,3,3,3,3,3,3,3,3,3,3,3,3,3,3,3,3,3,3,3,
3,3,3,3,4),(0.143172102,0.15412844,0.165137615,0.176146789,0.187155963,
0.198165138,0.209174312,0.220183486,0.231192661,0.242201835,0.255045872,
0.266055046,0.280733945,0.291743119,0.302752294,0.313761468,0.326605505,
0.337614679,0.348623853,0.359633028,0.370642202,0.381651376,0.39266055,
0.401834862,0.411009174,0.420183486,0.429357798,0.440366972,0.449541284,
0.458715596,0.467889908,0.47706422,0.488073394,0.497247706,0.506422018,
0.51559633,0.526605505,0.533944954,0.541284404,0.548623853,0.555963303,
0.565137615,0.572477064,0.579816514,0.588990826,0.596330275,0.603669725,
0.616513761,0.625688073,0.633027523,0.640366972,0.649541284,0.658715596,
0.667889908,0.67706422,0.68440367,0.691743119,0.702752294,0.710091743,0.719266055,
0.726605505,0.735779817,0.743119266,0.750458716,0.757798165,0.766972477,
0.776146789,0.787155963,0.794495413,0.803669725,0.811009174,0.816513761,
0.823853211,0.829357798,0.834862385,0.840366972,0.847706422,0.853211009,
0.858715596,0.864220183,0.869724771,0.875229358,0.880733945,0.888073394,
0.893577982,0.902752294,0.908256881,0.913761468,0.921100917,0.928440367,
0.933944954,0.941284404,0.950458716,0.955963303,0.96146789,0.968807339,
0.974311927,0.979816514,0.985321101,0.990825688,1.),.UNSPECIFIED.);
#24403=B_SPLINE_CURVE_WITH_KNOTS('',5,(#224511,#224512,#224513,#224514,
#224515,#224516,#224517,#224518,#224519,#224520,#224521,#224522,#224523,
#224524,#224525,#224526,#224527,#224528,#224529,#224530,#224531,#224532,
#224533,#224534,#224535,#224536,#224537,#224538,#224539,#224540,#224541,
#224542,#224543,#224544,#224545,#224546,#224547,#224548,#224549,#224550,
#224551,#224552,#224553,#224554,#224555,#224556,#224557,#224558,#224559,
#224560,#224561,#224562,#224563,#224564,#224565,#224566,#224567,#224568,
#224569,#224570,#224571,#224572,#224573,#224574,#224575,#224576,#224577,
#224578,#224579,#224580,#224581,#224582,#224583,#224584,#224585,#224586,
#224587,#224588,#224589,#224590,#224591,#224592,#224593,#224594,#224595,
#224596,#224597,#224598,#224599,#224600,#224601,#224602,#224603,#224604,
#224605,#224606,#224607,#224608,#224609,#224610,#224611,#224612,#224613,
#224614,#224615,#224616,#224617,#224618,#224619,#224620,#224621,#224622,
#224623,#224624,#224625,#224626,#224627,#224628,#224629,#224630,#224631,
#224632,#224633,#224634,#224635,#224636,#224637,#224638,#224639,#224640,
#224641,#224642,#224643,#224644,#224645,#224646,#224647,#224648,#224649,
#224650,#224651,#224652,#224653,#224654,#224655,#224656,#224657,#224658,
#224659,#224660,#224661,#224662,#224663,#224664,#224665,#224666,#224667,
#224668,#224669,#224670,#224671,#224672,#224673,#224674,#224675,#224676,
#224677,#224678,#224679,#224680,#224681,#224682,#224683,#224684,#224685,
#224686,#224687,#224688,#224689,#224690,#224691,#224692,#224693,#224694,
#224695,#224696,#224697,#224698,#224699,#224700,#224701,#224702,#224703,
#224704,#224705,#224706,#224707,#224708,#224709,#224710,#224711,#224712,
#224713,#224714,#224715,#224716,#224717,#224718,#224719,#224720,#224721,
#224722,#224723,#224724,#224725,#224726,#224727,#224728,#224729,#224730,
#224731,#224732,#224733,#224734,#224735,#224736,#224737,#224738,#224739,
#224740,#224741,#224742,#224743,#224744,#224745,#224746,#224747,#224748,
#224749,#224750,#224751,#224752,#224753,#224754,#224755,#224756,#224757,
#224758,#224759,#224760,#224761,#224762,#224763,#224764,#224765,#224766,
#224767,#224768,#224769,#224770,#224771,#224772,#224773,#224774,#224775,
#224776,#224777,#224778,#224779,#224780,#224781,#224782,#224783,#224784,
#224785,#224786,#224787,#224788,#224789,#224790,#224791,#224792,#224793,
#224794,#224795,#224796,#224797,#224798,#224799,#224800,#224801,#224802,
#224803,#224804,#224805,#224806,#224807,#224808,#224809,#224810,#224811,
#224812,#224813,#224814,#224815,#224816,#224817,#224818,#224819,#224820,
#224821,#224822,#224823,#224824,#224825,#224826,#224827,#224828,#224829,
#224830,#224831,#224832,#224833,#224834,#224835,#224836,#224837,#224838,
#224839,#224840,#224841,#224842,#224843,#224844,#224845,#224846,#224847,
#224848,#224849,#224850,#224851,#224852,#224853,#224854,#224855,#224856,
#224857,#224858,#224859,#224860,#224861,#224862,#224863,#224864,#224865,
#224866,#224867,#224868,#224869,#224870,#224871,#224872,#224873,#224874,
#224875,#224876,#224877,#224878,#224879,#224880,#224881,#224882,#224883,
#224884,#224885,#224886,#224887,#224888,#224889,#224890,#224891,#224892,
#224893,#224894,#224895,#224896,#224897,#224898,#224899,#224900,#224901,
#224902,#224903,#224904,#224905,#224906,#224907,#224908,#224909,#224910,
#224911,#224912,#224913,#224914,#224915,#224916,#224917,#224918,#224919,
#224920,#224921,#224922,#224923,#224924,#224925,#224926,#224927,#224928,
#224929,#224930,#224931,#224932,#224933,#224934,#224935,#224936,#224937,
#224938,#224939,#224940,#224941,#224942,#224943,#224944,#224945,#224946,
#224947,#224948,#224949,#224950,#224951,#224952,#224953,#224954,#224955,
#224956,#224957,#224958,#224959,#224960,#224961,#224962,#224963,#224964,
#224965,#224966,#224967,#224968,#224969,#224970,#224971,#224972,#224973,
#224974,#224975,#224976,#224977,#224978,#224979,#224980,#224981),
 .UNSPECIFIED.,.F.,.F.,(6,1,1,1,1,1,1,1,1,1,1,1,1,1,1,1,1,1,1,1,1,1,1,1,
1,1,1,1,1,1,1,1,1,1,1,1,1,1,1,1,1,1,1,1,1,1,1,1,1,1,1,1,1,1,1,1,1,1,1,1,
1,1,1,1,1,1,1,1,1,1,1,1,1,1,1,1,1,1,1,1,1,1,1,1,1,1,1,1,1,1,1,1,1,1,1,1,
1,1,1,1,1,1,1,1,1,1,1,1,1,1,1,1,1,1,1,1,1,1,1,1,1,1,1,1,1,1,1,1,1,1,1,1,
1,1,1,1,1,1,1,1,1,1,1,1,1,1,1,1,1,1,1,1,1,1,1,1,1,1,1,1,1,1,1,1,1,1,1,1,
1,1,1,1,1,1,1,1,1,1,1,1,1,1,1,1,1,1,1,1,1,1,1,1,1,1,1,1,1,1,1,1,1,1,1,1,
1,1,1,1,1,1,1,1,1,1,1,1,1,1,1,1,1,1,1,1,1,1,1,1,1,1,1,1,1,1,1,1,1,1,1,1,
1,1,1,1,1,1,1,1,1,1,1,1,1,1,1,1,1,1,1,1,1,1,1,1,1,1,1,1,1,1,1,1,1,1,1,1,
1,1,1,1,1,1,1,1,1,1,1,1,1,1,1,1,1,1,1,1,1,1,1,1,1,1,1,1,1,1,1,1,1,1,1,1,
1,1,1,1,1,1,1,1,1,1,1,1,1,1,1,1,1,1,1,1,1,1,1,1,1,1,1,1,1,1,1,1,1,1,1,1,
1,1,1,1,1,1,1,1,1,1,1,1,1,1,1,1,1,1,1,1,1,1,1,1,1,1,1,1,1,1,1,1,1,1,1,1,
1,1,1,1,1,1,1,1,1,1,1,1,1,1,1,1,1,1,1,1,1,1,1,1,1,1,1,1,1,1,1,1,1,1,1,1,
1,1,1,1,1,1,1,1,1,1,1,1,1,1,1,1,1,1,1,1,1,1,1,1,1,1,1,1,1,1,1,1,1,1,1,1,
1,1,1,1,1,1,1,1,1,1,6),(-1.,-0.998165138,-0.996330275,-0.994495413,-0.99266055,
-0.990825688,-0.988990826,-0.987155963,-0.985321101,-0.983486239,-0.981651376,
-0.979816514,-0.977981651,-0.976146789,-0.974311927,-0.972477064,-0.970642202,
-0.968807339,-0.966972477,-0.965137615,-0.963302752,-0.96146789,-0.959633028,
-0.957798165,-0.955963303,-0.95412844,-0.952293578,-0.950458716,-0.948623853,
-0.946788991,-0.944954128,-0.943119266,-0.941284404,-0.939449541,-0.937614679,
-0.935779817,-0.933944954,-0.932110092,-0.930275229,-0.928440367,-0.926605505,
-0.924770642,-0.92293578,-0.921100917,-0.919266055,-0.917431193,-0.91559633,
-0.913761468,-0.911926606,-0.910091743,-0.908256881,-0.906422018,-0.904587156,
-0.902752294,-0.900917431,-0.899082569,-0.897247706,-0.895412844,-0.893577982,
-0.891743119,-0.889908257,-0.888073394,-0.886238532,-0.88440367,-0.882568807,
-0.880733945,-0.878899083,-0.87706422,-0.875229358,-0.873394495,-0.869724771,
-0.867889908,-0.866055046,-0.864220183,-0.862385321,-0.860550459,-0.858715596,
-0.856880734,-0.855045872,-0.853211009,-0.851376147,-0.849541284,-0.847706422,
-0.84587156,-0.844036697,-0.842201835,-0.840366972,-0.83853211,-0.836697248,
-0.834862385,-0.833027523,-0.831192661,-0.829357798,-0.827522936,-0.825688073,
-0.823853211,-0.822018349,-0.820183486,-0.818348624,-0.816513761,-0.814678899,
-0.812844037,-0.811009174,-0.809174312,-0.80733945,-0.805504587,-0.803669725,
-0.801834862,-0.8,-0.798165138,-0.796330275,-0.794495413,-0.79266055,-0.790825688,
-0.788990826,-0.787155963,-0.785321101,-0.783486239,-0.781651376,-0.779816514,
-0.777981651,-0.776146789,-0.774311927,-0.772477064,-0.770642202,-0.768807339,
-0.766972477,-0.765137615,-0.763302752,-0.76146789,-0.759633028,-0.757798165,
-0.755963303,-0.75412844,-0.752293578,-0.750458716,-0.748623853,-0.746788991,
-0.744954128,-0.743119266,-0.741284404,-0.739449541,-0.737614679,-0.735779817,
-0.733944954,-0.732110092,-0.730275229,-0.728440367,-0.726605505,-0.724770642,
-0.72293578,-0.721100917,-0.719266055,-0.717431193,-0.71559633,-0.713761468,
-0.711926606,-0.710091743,-0.708256881,-0.706422018,-0.704587156,-0.702752294,
-0.700917431,-0.699082569,-0.697247706,-0.695412844,-0.693577982,-0.691743119,
-0.689908257,-0.688073394,-0.686238532,-0.68440367,-0.682568807,-0.680733945,
-0.678899083,-0.67706422,-0.675229358,-0.673394495,-0.671559633,-0.669724771,
-0.667889908,-0.666055046,-0.664220183,-0.662385321,-0.660550459,-0.658715596,
-0.656880734,-0.655045872,-0.653211009,-0.651376147,-0.649541284,-0.647706422,
-0.64587156,-0.644036697,-0.642201835,-0.640366972,-0.63853211,-0.636697248,
-0.634862385,-0.633027523,-0.631192661,-0.629357798,-0.627522936,-0.625688073,
-0.623853211,-0.622018349,-0.620183486,-0.618348624,-0.616513761,-0.614678899,
-0.612844037,-0.611009174,-0.609174312,-0.60733945,-0.605504587,-0.603669725,
-0.601834862,-0.6,-0.598165138,-0.596330275,-0.594495413,-0.59266055,-0.590825688,
-0.588990826,-0.587155963,-0.585321101,-0.583486239,-0.581651376,-0.579816514,
-0.577981651,-0.576146789,-0.574311927,-0.572477064,-0.570642202,-0.568807339,
-0.566972477,-0.565137615,-0.563302752,-0.56146789,-0.559633028,-0.557798165,
-0.555963303,-0.55412844,-0.552293578,-0.550458716,-0.548623853,-0.546788991,
-0.544954128,-0.543119266,-0.541284404,-0.539449541,-0.537614679,-0.535779817,
-0.533944954,-0.532110092,-0.530275229,-0.528440367,-0.526605505,-0.524770642,
-0.52293578,-0.521100917,-0.519266055,-0.517431193,-0.51559633,-0.513761468,
-0.511926606,-0.510091743,-0.508256881,-0.506422018,-0.504587156,-0.502752294,
-0.500917431,-0.499082569,-0.497247706,-0.495412844,-0.493577982,-0.491743119,
-0.489908257,-0.488073394,-0.486238532,-0.48440367,-0.482568807,-0.480733945,
-0.478899083,-0.47706422,-0.475229358,-0.473394495,-0.471559633,-0.469724771,
-0.467889908,-0.466055046,-0.464220183,-0.462385321,-0.460550459,-0.458715596,
-0.456880734,-0.455045872,-0.453211009,-0.451376147,-0.449541284,-0.447706422,
-0.44587156,-0.444036697,-0.442201835,-0.440366972,-0.43853211,-0.436697248,
-0.434862385,-0.433027523,-0.431192661,-0.429357798,-0.427522936,-0.425688073,
-0.423853211,-0.422018349,-0.420183486,-0.418348624,-0.416513761,-0.414678899,
-0.412844037,-0.411009174,-0.409174312,-0.40733945,-0.405504587,-0.403669725,
-0.401834862,-0.4,-0.398165138,-0.396330275,-0.394495413,-0.39266055,-0.390825688,
-0.388990826,-0.387155963,-0.385321101,-0.383486239,-0.381651376,-0.379816514,
-0.377981651,-0.376146789,-0.374311927,-0.372477064,-0.370642202,-0.368807339,
-0.366972477,-0.365137615,-0.363302752,-0.36146789,-0.359633028,-0.357798165,
-0.355963303,-0.35412844,-0.352293578,-0.350458716,-0.348623853,-0.346788991,
-0.344954128,-0.343119266,-0.341284404,-0.339449541,-0.337614679,-0.335779817,
-0.333944954,-0.332110092,-0.330275229,-0.328440367,-0.326605505,-0.324770642,
-0.32293578,-0.321100917,-0.319266055,-0.317431193,-0.31559633,-0.313761468,
-0.311926606,-0.310091743,-0.308256881,-0.306422018,-0.304587156,-0.302752294,
-0.300917431,-0.299082569,-0.297247706,-0.295412844,-0.293577982,-0.291743119,
-0.289908257,-0.288073394,-0.286238532,-0.28440367,-0.282568807,-0.280733945,
-0.278899083,-0.27706422,-0.275229358,-0.273394495,-0.271559633,-0.269724771,
-0.267889908,-0.266055046,-0.264220183,-0.262385321,-0.260550459,-0.258715596,
-0.256880734,-0.255045872,-0.253211009,-0.251376147,-0.249541284,-0.247706422,
-0.24587156,-0.244036697,-0.242201835,-0.240366972,-0.23853211,-0.236697248,
-0.234862385,-0.233027523,-0.231192661,-0.229357798,-0.227522936,-0.225688073,
-0.223853211,-0.222018349,-0.220183486,-0.218348624,-0.216513761,-0.214678899,
-0.212844037,-0.211009174,-0.209174312,-0.20733945,-0.205504587,-0.203669725,
-0.201834862,-0.2,-0.198165138,-0.196330275,-0.194495413,-0.19266055,-0.190825688,
-0.188990826,-0.187155963,-0.185321101,-0.183486239,-0.181651376,-0.179816514,
-0.177981651,-0.176146789,-0.174311927,-0.172477064,-0.170642202,-0.168807339,
-0.166972477,-0.165137615,-0.163302752,-0.16146789,-0.159633028,-0.157798165,
-0.155963303,-0.15412844,-0.152293578,-0.150458716,-0.148623853,-0.146788991,
-0.144954128,-0.143172102),.UNSPECIFIED.);
#24404=B_SPLINE_CURVE_WITH_KNOTS('',5,(#224982,#224983,#224984,#224985,
#224986,#224987,#224988,#224989,#224990,#224991,#224992,#224993,#224994,
#224995,#224996,#224997,#224998,#224999,#225000,#225001,#225002,#225003,
#225004,#225005,#225006,#225007,#225008,#225009,#225010,#225011,#225012,
#225013,#225014,#225015,#225016,#225017,#225018,#225019,#225020,#225021,
#225022,#225023,#225024,#225025,#225026,#225027,#225028,#225029,#225030,
#225031,#225032,#225033,#225034,#225035,#225036,#225037,#225038,#225039,
#225040,#225041,#225042,#225043,#225044,#225045,#225046,#225047,#225048,
#225049,#225050,#225051,#225052,#225053,#225054,#225055,#225056,#225057,
#225058,#225059,#225060,#225061,#225062,#225063,#225064,#225065,#225066,
#225067,#225068,#225069,#225070,#225071,#225072,#225073,#225074,#225075,
#225076,#225077,#225078,#225079,#225080,#225081,#225082,#225083,#225084,
#225085,#225086,#225087,#225088,#225089,#225090,#225091,#225092,#225093,
#225094,#225095,#225096,#225097,#225098,#225099,#225100,#225101,#225102,
#225103,#225104,#225105,#225106,#225107,#225108,#225109,#225110,#225111,
#225112,#225113,#225114,#225115,#225116,#225117,#225118,#225119,#225120,
#225121,#225122,#225123,#225124,#225125,#225126,#225127,#225128,#225129,
#225130,#225131,#225132,#225133,#225134,#225135,#225136,#225137,#225138,
#225139,#225140,#225141,#225142,#225143,#225144,#225145,#225146,#225147,
#225148,#225149,#225150,#225151,#225152,#225153,#225154,#225155,#225156,
#225157,#225158,#225159,#225160,#225161,#225162,#225163,#225164,#225165,
#225166,#225167,#225168,#225169,#225170,#225171,#225172,#225173,#225174,
#225175,#225176,#225177,#225178,#225179,#225180,#225181,#225182,#225183,
#225184,#225185,#225186,#225187,#225188,#225189,#225190,#225191,#225192,
#225193,#225194,#225195,#225196,#225197,#225198,#225199,#225200,#225201,
#225202,#225203,#225204,#225205,#225206,#225207,#225208,#225209,#225210,
#225211,#225212,#225213,#225214,#225215,#225216,#225217,#225218,#225219,
#225220,#225221,#225222,#225223,#225224,#225225,#225226,#225227,#225228,
#225229,#225230,#225231,#225232,#225233,#225234,#225235,#225236,#225237,
#225238,#225239,#225240,#225241,#225242,#225243,#225244,#225245,#225246,
#225247,#225248,#225249,#225250,#225251,#225252,#225253,#225254,#225255,
#225256,#225257,#225258,#225259,#225260,#225261,#225262,#225263,#225264,
#225265,#225266,#225267,#225268,#225269,#225270,#225271,#225272,#225273,
#225274,#225275,#225276,#225277,#225278,#225279,#225280,#225281,#225282,
#225283,#225284,#225285,#225286,#225287,#225288,#225289,#225290,#225291,
#225292,#225293,#225294,#225295,#225296,#225297,#225298,#225299,#225300,
#225301,#225302,#225303,#225304,#225305,#225306,#225307,#225308,#225309,
#225310,#225311,#225312,#225313,#225314,#225315,#225316,#225317,#225318,
#225319,#225320,#225321,#225322,#225323,#225324,#225325,#225326,#225327,
#225328,#225329,#225330,#225331,#225332,#225333,#225334,#225335,#225336,
#225337,#225338,#225339,#225340,#225341,#225342,#225343,#225344,#225345,
#225346,#225347,#225348,#225349,#225350,#225351,#225352,#225353,#225354,
#225355,#225356,#225357,#225358,#225359,#225360,#225361,#225362,#225363,
#225364,#225365,#225366,#225367,#225368,#225369,#225370,#225371,#225372,
#225373,#225374,#225375,#225376,#225377,#225378,#225379,#225380,#225381,
#225382,#225383,#225384,#225385,#225386,#225387,#225388,#225389,#225390,
#225391,#225392,#225393,#225394,#225395,#225396,#225397,#225398,#225399,
#225400,#225401,#225402,#225403,#225404,#225405,#225406,#225407,#225408,
#225409,#225410,#225411,#225412,#225413,#225414,#225415,#225416,#225417,
#225418,#225419,#225420,#225421,#225422,#225423,#225424,#225425,#225426,
#225427,#225428,#225429,#225430,#225431,#225432,#225433,#225434,#225435,
#225436,#225437,#225438,#225439,#225440,#225441,#225442,#225443,#225444,
#225445,#225446,#225447,#225448,#225449,#225450,#225451,#225452),
 .UNSPECIFIED.,.F.,.F.,(6,1,1,1,1,1,1,1,1,1,1,1,1,1,1,1,1,1,1,1,1,1,1,1,
1,1,1,1,1,1,1,1,1,1,1,1,1,1,1,1,1,1,1,1,1,1,1,1,1,1,1,1,1,1,1,1,1,1,1,1,
1,1,1,1,1,1,1,1,1,1,1,1,1,1,1,1,1,1,1,1,1,1,1,1,1,1,1,1,1,1,1,1,1,1,1,1,
1,1,1,1,1,1,1,1,1,1,1,1,1,1,1,1,1,1,1,1,1,1,1,1,1,1,1,1,1,1,1,1,1,1,1,1,
1,1,1,1,1,1,1,1,1,1,1,1,1,1,1,1,1,1,1,1,1,1,1,1,1,1,1,1,1,1,1,1,1,1,1,1,
1,1,1,1,1,1,1,1,1,1,1,1,1,1,1,1,1,1,1,1,1,1,1,1,1,1,1,1,1,1,1,1,1,1,1,1,
1,1,1,1,1,1,1,1,1,1,1,1,1,1,1,1,1,1,1,1,1,1,1,1,1,1,1,1,1,1,1,1,1,1,1,1,
1,1,1,1,1,1,1,1,1,1,1,1,1,1,1,1,1,1,1,1,1,1,1,1,1,1,1,1,1,1,1,1,1,1,1,1,
1,1,1,1,1,1,1,1,1,1,1,1,1,1,1,1,1,1,1,1,1,1,1,1,1,1,1,1,1,1,1,1,1,1,1,1,
1,1,1,1,1,1,1,1,1,1,1,1,1,1,1,1,1,1,1,1,1,1,1,1,1,1,1,1,1,1,1,1,1,1,1,1,
1,1,1,1,1,1,1,1,1,1,1,1,1,1,1,1,1,1,1,1,1,1,1,1,1,1,1,1,1,1,1,1,1,1,1,1,
1,1,1,1,1,1,1,1,1,1,1,1,1,1,1,1,1,1,1,1,1,1,1,1,1,1,1,1,1,1,1,1,1,1,1,1,
1,1,1,1,1,1,1,1,1,1,1,1,1,1,1,1,1,1,1,1,1,1,1,1,1,1,1,1,1,1,1,1,1,1,1,1,
1,1,1,1,1,1,1,1,1,1,6),(0.143172102,0.144954128,0.146788991,0.148623853,
0.150458716,0.152293578,0.15412844,0.155963303,0.157798165,0.159633028,
0.16146789,0.163302752,0.165137615,0.166972477,0.168807339,0.170642202,
0.172477064,0.174311927,0.176146789,0.177981651,0.179816514,0.181651376,
0.183486239,0.185321101,0.187155963,0.188990826,0.190825688,0.19266055,
0.194495413,0.196330275,0.198165138,0.2,0.201834862,0.203669725,0.205504587,
0.20733945,0.209174312,0.211009174,0.212844037,0.214678899,0.216513761,
0.218348624,0.220183486,0.222018349,0.223853211,0.225688073,0.227522936,
0.229357798,0.231192661,0.233027523,0.234862385,0.236697248,0.23853211,
0.240366972,0.242201835,0.244036697,0.24587156,0.247706422,0.249541284,
0.251376147,0.253211009,0.255045872,0.256880734,0.258715596,0.260550459,
0.262385321,0.264220183,0.266055046,0.267889908,0.269724771,0.271559633,
0.273394495,0.275229358,0.27706422,0.278899083,0.280733945,0.282568807,
0.28440367,0.286238532,0.288073394,0.289908257,0.291743119,0.293577982,
0.295412844,0.297247706,0.299082569,0.300917431,0.302752294,0.304587156,
0.306422018,0.308256881,0.310091743,0.311926606,0.313761468,0.31559633,
0.317431193,0.319266055,0.321100917,0.32293578,0.324770642,0.326605505,
0.328440367,0.330275229,0.332110092,0.333944954,0.335779817,0.337614679,
0.339449541,0.341284404,0.343119266,0.344954128,0.346788991,0.348623853,
0.350458716,0.352293578,0.35412844,0.355963303,0.357798165,0.359633028,
0.36146789,0.363302752,0.365137615,0.366972477,0.368807339,0.370642202,
0.372477064,0.374311927,0.376146789,0.377981651,0.379816514,0.381651376,
0.383486239,0.385321101,0.387155963,0.388990826,0.390825688,0.39266055,
0.394495413,0.396330275,0.398165138,0.4,0.401834862,0.403669725,0.405504587,
0.40733945,0.409174312,0.411009174,0.412844037,0.414678899,0.416513761,
0.418348624,0.420183486,0.422018349,0.423853211,0.425688073,0.427522936,
0.429357798,0.431192661,0.433027523,0.434862385,0.436697248,0.43853211,
0.440366972,0.442201835,0.444036697,0.44587156,0.447706422,0.449541284,
0.451376147,0.453211009,0.455045872,0.456880734,0.458715596,0.460550459,
0.462385321,0.464220183,0.466055046,0.467889908,0.469724771,0.471559633,
0.473394495,0.475229358,0.47706422,0.478899083,0.480733945,0.482568807,
0.48440367,0.486238532,0.488073394,0.489908257,0.491743119,0.493577982,
0.495412844,0.497247706,0.499082569,0.500917431,0.502752294,0.504587156,
0.506422018,0.508256881,0.510091743,0.511926606,0.513761468,0.51559633,
0.517431193,0.519266055,0.521100917,0.52293578,0.524770642,0.526605505,
0.528440367,0.530275229,0.532110092,0.533944954,0.535779817,0.537614679,
0.539449541,0.541284404,0.543119266,0.544954128,0.546788991,0.548623853,
0.550458716,0.552293578,0.55412844,0.555963303,0.557798165,0.559633028,
0.56146789,0.563302752,0.565137615,0.566972477,0.568807339,0.570642202,
0.572477064,0.574311927,0.576146789,0.577981651,0.579816514,0.581651376,
0.583486239,0.585321101,0.587155963,0.588990826,0.590825688,0.59266055,
0.594495413,0.596330275,0.598165138,0.6,0.601834862,0.603669725,0.605504587,
0.60733945,0.609174312,0.611009174,0.612844037,0.614678899,0.616513761,
0.618348624,0.620183486,0.622018349,0.623853211,0.625688073,0.627522936,
0.629357798,0.631192661,0.633027523,0.634862385,0.636697248,0.63853211,
0.640366972,0.642201835,0.644036697,0.64587156,0.647706422,0.649541284,
0.651376147,0.653211009,0.655045872,0.656880734,0.658715596,0.660550459,
0.662385321,0.664220183,0.666055046,0.667889908,0.669724771,0.671559633,
0.673394495,0.675229358,0.67706422,0.678899083,0.680733945,0.682568807,
0.68440367,0.686238532,0.688073394,0.689908257,0.691743119,0.693577982,
0.695412844,0.697247706,0.699082569,0.700917431,0.702752294,0.704587156,
0.706422018,0.708256881,0.710091743,0.711926606,0.713761468,0.71559633,
0.717431193,0.719266055,0.721100917,0.72293578,0.724770642,0.726605505,
0.728440367,0.730275229,0.732110092,0.733944954,0.735779817,0.737614679,
0.739449541,0.741284404,0.743119266,0.744954128,0.746788991,0.748623853,
0.750458716,0.752293578,0.75412844,0.755963303,0.757798165,0.759633028,
0.76146789,0.763302752,0.765137615,0.766972477,0.768807339,0.770642202,
0.772477064,0.774311927,0.776146789,0.777981651,0.779816514,0.781651376,
0.783486239,0.785321101,0.787155963,0.788990826,0.790825688,0.79266055,
0.794495413,0.796330275,0.798165138,0.8,0.801834862,0.803669725,0.805504587,
0.80733945,0.809174312,0.811009174,0.812844037,0.814678899,0.816513761,
0.818348624,0.820183486,0.822018349,0.823853211,0.825688073,0.827522936,
0.829357798,0.831192661,0.833027523,0.834862385,0.836697248,0.83853211,
0.840366972,0.842201835,0.844036697,0.84587156,0.847706422,0.849541284,
0.851376147,0.853211009,0.855045872,0.856880734,0.858715596,0.860550459,
0.862385321,0.864220183,0.866055046,0.867889908,0.869724771,0.873394495,
0.875229358,0.87706422,0.878899083,0.880733945,0.882568807,0.88440367,0.886238532,
0.888073394,0.889908257,0.891743119,0.893577982,0.895412844,0.897247706,
0.899082569,0.900917431,0.902752294,0.904587156,0.906422018,0.908256881,
0.910091743,0.911926606,0.913761468,0.91559633,0.917431193,0.919266055,
0.921100917,0.92293578,0.924770642,0.926605505,0.928440367,0.930275229,
0.932110092,0.933944954,0.935779817,0.937614679,0.939449541,0.941284404,
0.943119266,0.944954128,0.946788991,0.948623853,0.950458716,0.952293578,
0.95412844,0.955963303,0.957798165,0.959633028,0.96146789,0.963302752,0.965137615,
0.966972477,0.968807339,0.970642202,0.972477064,0.974311927,0.976146789,
0.977981651,0.979816514,0.981651376,0.983486239,0.985321101,0.987155963,
0.988990826,0.990825688,0.99266055,0.994495413,0.996330275,0.998165138,
1.),.UNSPECIFIED.);
#24405=B_SPLINE_CURVE_WITH_KNOTS('',3,(#226397,#226398,#226399,#226400,
#226401,#226402,#226403,#226404,#226405,#226406,#226407,#226408,#226409,
#226410,#226411,#226412,#226413,#226414,#226415,#226416,#226417,#226418,
#226419,#226420,#226421,#226422,#226423,#226424,#226425,#226426,#226427,
#226428,#226429,#226430,#226431,#226432,#226433,#226434,#226435,#226436,
#226437,#226438,#226439,#226440,#226441,#226442,#226443,#226444,#226445,
#226446,#226447,#226448,#226449,#226450,#226451,#226452,#226453,#226454,
#226455,#226456,#226457,#226458,#226459,#226460,#226461,#226462,#226463,
#226464,#226465,#226466,#226467,#226468,#226469,#226470,#226471,#226472,
#226473,#226474,#226475,#226476,#226477,#226478,#226479,#226480,#226481,
#226482,#226483,#226484,#226485,#226486,#226487,#226488,#226489,#226490,
#226491,#226492,#226493,#226494,#226495,#226496,#226497,#226498,#226499,
#226500,#226501,#226502,#226503,#226504,#226505,#226506,#226507,#226508,
#226509,#226510,#226511,#226512,#226513,#226514,#226515,#226516,#226517,
#226518,#226519,#226520,#226521,#226522,#226523,#226524,#226525,#226526,
#226527,#226528,#226529,#226530,#226531,#226532,#226533,#226534,#226535,
#226536,#226537,#226538,#226539,#226540,#226541,#226542,#226543,#226544,
#226545,#226546,#226547,#226548,#226549,#226550,#226551,#226552,#226553,
#226554,#226555,#226556,#226557,#226558,#226559,#226560,#226561,#226562,
#226563,#226564,#226565,#226566,#226567,#226568,#226569,#226570,#226571,
#226572,#226573,#226574,#226575,#226576,#226577,#226578,#226579,#226580,
#226581,#226582,#226583,#226584,#226585,#226586,#226587,#226588,#226589,
#226590,#226591,#226592,#226593,#226594,#226595,#226596,#226597,#226598,
#226599,#226600,#226601,#226602,#226603,#226604,#226605,#226606,#226607,
#226608,#226609,#226610,#226611,#226612,#226613,#226614,#226615,#226616,
#226617,#226618,#226619,#226620,#226621,#226622,#226623,#226624,#226625,
#226626,#226627,#226628,#226629,#226630,#226631,#226632,#226633,#226634,
#226635,#226636,#226637,#226638,#226639,#226640,#226641,#226642,#226643,
#226644,#226645,#226646,#226647,#226648,#226649,#226650,#226651,#226652,
#226653,#226654,#226655,#226656,#226657,#226658,#226659,#226660,#226661,
#226662,#226663,#226664,#226665,#226666,#226667,#226668,#226669,#226670,
#226671,#226672,#226673,#226674,#226675,#226676),.UNSPECIFIED.,.F.,.F.,
(4,3,3,3,3,3,3,3,3,3,3,3,3,3,3,3,3,3,3,3,3,3,3,3,3,3,3,3,3,3,3,3,3,3,3,
3,3,3,3,3,3,3,3,3,3,3,3,3,3,3,3,3,3,3,3,3,3,3,3,3,3,3,3,3,3,3,3,3,3,3,3,
3,3,3,3,3,3,3,3,3,3,3,3,3,3,3,3,3,3,3,3,3,3,4),(0.143172102,0.15412844,
0.165137615,0.181651376,0.19266055,0.203669725,0.214678899,0.231192661,
0.242201835,0.253211009,0.266055046,0.27706422,0.291743119,0.302752294,
0.32293578,0.335779817,0.346788991,0.359633028,0.370642202,0.383486239,
0.394495413,0.405504587,0.414678899,0.423853211,0.433027523,0.444036697,
0.455045872,0.464220183,0.47706422,0.486238532,0.497247706,0.508256881,
0.517431193,0.526605505,0.533944954,0.541284404,0.550458716,0.56146789,
0.568807339,0.581651376,0.588990826,0.6,0.60733945,0.616513761,0.623853211,
0.634862385,0.64587156,0.655045872,0.664220183,0.671559633,0.682568807,
0.691743119,0.700917431,0.713761468,0.724770642,0.732110092,0.739449541,
0.752293578,0.759633028,0.766972477,0.774311927,0.781651376,0.790825688,
0.798165138,0.80733945,0.814678899,0.823853211,0.829357798,0.836697248,
0.844036697,0.853211009,0.862385321,0.867889908,0.873394495,0.878899083,
0.886238532,0.891743119,0.899082569,0.904587156,0.910091743,0.91559633,
0.921100917,0.926605505,0.932110092,0.941284404,0.950458716,0.955963303,
0.96146789,0.966972477,0.976146789,0.983486239,0.988990826,0.994495413,
1.),.UNSPECIFIED.);
#24406=B_SPLINE_CURVE_WITH_KNOTS('',3,(#226677,#226678,#226679,#226680,
#226681,#226682,#226683,#226684,#226685,#226686,#226687,#226688,#226689,
#226690,#226691,#226692,#226693,#226694,#226695,#226696,#226697,#226698,
#226699,#226700,#226701,#226702,#226703,#226704,#226705,#226706,#226707,
#226708,#226709,#226710,#226711,#226712,#226713,#226714,#226715,#226716,
#226717,#226718,#226719,#226720,#226721,#226722,#226723,#226724,#226725,
#226726,#226727,#226728,#226729,#226730,#226731,#226732,#226733,#226734,
#226735,#226736,#226737,#226738,#226739,#226740,#226741,#226742,#226743,
#226744,#226745,#226746,#226747,#226748,#226749,#226750,#226751,#226752,
#226753,#226754,#226755,#226756,#226757,#226758,#226759,#226760,#226761,
#226762,#226763,#226764,#226765,#226766,#226767,#226768,#226769,#226770,
#226771,#226772,#226773,#226774,#226775,#226776,#226777,#226778,#226779,
#226780,#226781,#226782,#226783,#226784,#226785,#226786,#226787,#226788,
#226789,#226790,#226791,#226792,#226793,#226794,#226795,#226796,#226797,
#226798,#226799,#226800,#226801,#226802,#226803,#226804,#226805,#226806,
#226807,#226808,#226809,#226810,#226811,#226812,#226813,#226814,#226815,
#226816,#226817,#226818,#226819,#226820,#226821,#226822,#226823,#226824,
#226825,#226826,#226827,#226828,#226829,#226830,#226831,#226832,#226833,
#226834,#226835,#226836,#226837,#226838,#226839,#226840,#226841,#226842,
#226843,#226844,#226845,#226846,#226847,#226848,#226849,#226850,#226851,
#226852,#226853,#226854,#226855,#226856,#226857,#226858,#226859,#226860,
#226861,#226862,#226863,#226864,#226865,#226866,#226867,#226868,#226869,
#226870,#226871,#226872,#226873,#226874,#226875,#226876,#226877,#226878,
#226879,#226880,#226881,#226882,#226883,#226884,#226885,#226886,#226887,
#226888,#226889,#226890,#226891,#226892,#226893,#226894,#226895,#226896,
#226897,#226898,#226899,#226900,#226901,#226902,#226903,#226904,#226905,
#226906,#226907,#226908,#226909,#226910,#226911,#226912,#226913,#226914,
#226915,#226916,#226917,#226918,#226919,#226920,#226921,#226922,#226923,
#226924,#226925,#226926,#226927,#226928,#226929,#226930,#226931,#226932,
#226933,#226934,#226935,#226936,#226937,#226938,#226939,#226940,#226941,
#226942,#226943,#226944,#226945,#226946,#226947,#226948,#226949,#226950,
#226951,#226952,#226953,#226954,#226955,#226956,#226957,#226958,#226959,
#226960,#226961,#226962,#226963,#226964,#226965,#226966,#226967,#226968,
#226969,#226970,#226971,#226972,#226973,#226974,#226975,#226976,#226977,
#226978,#226979,#226980,#226981,#226982,#226983,#226984,#226985,#226986,
#226987,#226988,#226989,#226990,#226991,#226992),.UNSPECIFIED.,.F.,.F.,
(4,3,3,3,3,3,3,3,3,3,3,3,3,3,3,3,3,3,3,3,3,3,3,3,3,3,3,3,3,3,3,3,3,3,3,
3,3,3,3,3,3,3,3,3,3,3,3,3,3,3,3,3,3,3,3,3,3,3,3,3,3,3,3,3,3,3,3,3,3,3,3,
3,3,3,3,3,3,3,3,3,3,3,3,3,3,3,3,3,3,3,3,3,3,3,3,3,3,3,3,3,3,3,3,3,3,4),
(0.143172102,0.15412844,0.165137615,0.177981651,0.188990826,0.2,0.211009174,
0.222018349,0.234862385,0.24587156,0.256880734,0.267889908,0.278899083,
0.289908257,0.300917431,0.311926606,0.32293578,0.333944954,0.344954128,
0.355963303,0.368807339,0.379816514,0.39266055,0.401834862,0.411009174,
0.420183486,0.429357798,0.43853211,0.447706422,0.456880734,0.466055046,
0.47706422,0.489908257,0.500917431,0.510091743,0.519266055,0.528440367,
0.535779817,0.543119266,0.550458716,0.557798165,0.565137615,0.572477064,
0.581651376,0.588990826,0.596330275,0.603669725,0.611009174,0.618348624,
0.625688073,0.633027523,0.640366972,0.647706422,0.655045872,0.664220183,
0.671559633,0.678899083,0.686238532,0.693577982,0.700917431,0.710091743,
0.717431193,0.724770642,0.732110092,0.739449541,0.748623853,0.755963303,
0.763302752,0.774311927,0.781651376,0.788990826,0.796330275,0.803669725,
0.811009174,0.816513761,0.822018349,0.827522936,0.833027523,0.83853211,
0.844036697,0.849541284,0.855045872,0.860550459,0.867889908,0.873394495,
0.878899083,0.88440367,0.891743119,0.897247706,0.902752294,0.908256881,
0.913761468,0.921100917,0.926605505,0.933944954,0.939449541,0.944954128,
0.950458716,0.957798165,0.963302752,0.968807339,0.974311927,0.979816514,
0.985321101,0.994495413,1.),.UNSPECIFIED.);
#24407=B_SPLINE_CURVE_WITH_KNOTS('',3,(#227952,#227953,#227954,#227955,
#227956,#227957,#227958,#227959,#227960,#227961,#227962,#227963,#227964,
#227965,#227966,#227967,#227968,#227969,#227970,#227971,#227972,#227973,
#227974,#227975,#227976,#227977,#227978,#227979,#227980,#227981,#227982,
#227983,#227984,#227985,#227986,#227987,#227988,#227989,#227990,#227991,
#227992,#227993,#227994,#227995,#227996,#227997,#227998,#227999,#228000,
#228001,#228002,#228003,#228004,#228005,#228006,#228007,#228008,#228009,
#228010,#228011,#228012,#228013,#228014,#228015,#228016,#228017,#228018,
#228019,#228020,#228021,#228022,#228023,#228024,#228025,#228026,#228027,
#228028,#228029,#228030,#228031,#228032,#228033,#228034,#228035,#228036,
#228037,#228038,#228039,#228040,#228041,#228042,#228043,#228044,#228045,
#228046,#228047,#228048,#228049,#228050,#228051,#228052,#228053,#228054,
#228055,#228056,#228057,#228058,#228059,#228060,#228061,#228062,#228063,
#228064,#228065,#228066,#228067,#228068,#228069,#228070,#228071,#228072,
#228073,#228074,#228075,#228076,#228077,#228078,#228079,#228080,#228081,
#228082,#228083,#228084,#228085,#228086,#228087,#228088,#228089,#228090,
#228091,#228092,#228093,#228094,#228095,#228096,#228097,#228098,#228099,
#228100,#228101,#228102,#228103,#228104,#228105,#228106,#228107,#228108,
#228109,#228110,#228111,#228112,#228113,#228114,#228115,#228116,#228117,
#228118,#228119,#228120,#228121,#228122,#228123,#228124,#228125,#228126,
#228127,#228128,#228129,#228130,#228131,#228132,#228133,#228134,#228135,
#228136,#228137,#228138,#228139,#228140,#228141,#228142,#228143,#228144,
#228145,#228146,#228147,#228148,#228149,#228150,#228151,#228152,#228153,
#228154,#228155,#228156,#228157,#228158,#228159,#228160,#228161,#228162,
#228163,#228164,#228165,#228166,#228167,#228168,#228169,#228170,#228171,
#228172,#228173,#228174,#228175,#228176,#228177,#228178,#228179,#228180,
#228181,#228182,#228183,#228184,#228185,#228186,#228187,#228188,#228189,
#228190,#228191,#228192,#228193,#228194,#228195,#228196,#228197,#228198,
#228199,#228200,#228201,#228202,#228203,#228204,#228205,#228206,#228207,
#228208,#228209,#228210,#228211,#228212,#228213,#228214,#228215,#228216,
#228217,#228218,#228219,#228220,#228221,#228222,#228223,#228224,#228225,
#228226,#228227,#228228,#228229,#228230,#228231,#228232,#228233,#228234,
#228235,#228236,#228237,#228238,#228239,#228240,#228241,#228242,#228243,
#228244,#228245,#228246,#228247,#228248,#228249,#228250,#228251,#228252),
 .UNSPECIFIED.,.F.,.F.,(4,3,3,3,3,3,3,3,3,3,3,3,3,3,3,3,3,3,3,3,3,3,3,3,
3,3,3,3,3,3,3,3,3,3,3,3,3,3,3,3,3,3,3,3,3,3,3,3,3,3,3,3,3,3,3,3,3,3,3,3,
3,3,3,3,3,3,3,3,3,3,3,3,3,3,3,3,3,3,3,3,3,3,3,3,3,3,3,3,3,3,3,3,3,3,3,3,
3,3,3,3,4),(0.143172102,0.15412844,0.165137615,0.179816514,0.190825688,
0.201834862,0.212844037,0.225688073,0.236697248,0.247706422,0.258715596,
0.269724771,0.282568807,0.293577982,0.304587156,0.31559633,0.326605505,
0.344954128,0.355963303,0.366972477,0.377981651,0.388990826,0.398165138,
0.40733945,0.416513761,0.427522936,0.43853211,0.449541284,0.460550459,0.473394495,
0.48440367,0.493577982,0.502752294,0.511926606,0.521100917,0.530275229,
0.537614679,0.544954128,0.552293578,0.559633028,0.568807339,0.576146789,
0.583486239,0.590825688,0.598165138,0.605504587,0.616513761,0.623853211,
0.633027523,0.640366972,0.647706422,0.655045872,0.664220183,0.671559633,
0.682568807,0.689908257,0.700917431,0.711926606,0.719266055,0.726605505,
0.733944954,0.741284404,0.750458716,0.757798165,0.766972477,0.774311927,
0.781651376,0.790825688,0.798165138,0.80733945,0.812844037,0.822018349,
0.827522936,0.833027523,0.83853211,0.844036697,0.851376147,0.856880734,
0.862385321,0.867889908,0.875229358,0.880733945,0.886238532,0.895412844,
0.900917431,0.906422018,0.911926606,0.919266055,0.924770642,0.930275229,
0.935779817,0.943119266,0.950458716,0.955963303,0.963302752,0.968807339,
0.974311927,0.981651376,0.987155963,0.99266055,1.),.UNSPECIFIED.);
#24408=B_SPLINE_CURVE_WITH_KNOTS('',3,(#228253,#228254,#228255,#228256,
#228257,#228258,#228259,#228260,#228261,#228262,#228263,#228264,#228265,
#228266,#228267,#228268,#228269,#228270,#228271,#228272,#228273,#228274,
#228275,#228276,#228277,#228278,#228279,#228280,#228281,#228282,#228283,
#228284,#228285,#228286,#228287,#228288,#228289,#228290,#228291,#228292,
#228293,#228294,#228295,#228296,#228297,#228298,#228299,#228300,#228301,
#228302,#228303,#228304,#228305,#228306,#228307,#228308,#228309,#228310,
#228311,#228312,#228313,#228314,#228315,#228316,#228317,#228318,#228319,
#228320,#228321,#228322,#228323,#228324,#228325,#228326,#228327,#228328,
#228329,#228330,#228331,#228332,#228333,#228334,#228335,#228336,#228337,
#228338,#228339,#228340,#228341,#228342,#228343,#228344,#228345,#228346,
#228347,#228348,#228349,#228350,#228351,#228352,#228353,#228354,#228355,
#228356,#228357,#228358,#228359,#228360,#228361,#228362,#228363,#228364,
#228365,#228366,#228367,#228368,#228369,#228370,#228371,#228372,#228373,
#228374,#228375,#228376,#228377,#228378,#228379,#228380,#228381,#228382,
#228383,#228384,#228385,#228386,#228387,#228388,#228389,#228390,#228391,
#228392,#228393,#228394,#228395,#228396,#228397,#228398,#228399,#228400,
#228401,#228402,#228403,#228404,#228405,#228406,#228407,#228408,#228409,
#228410,#228411,#228412,#228413,#228414,#228415,#228416,#228417,#228418,
#228419,#228420,#228421,#228422,#228423,#228424,#228425,#228426,#228427,
#228428,#228429,#228430,#228431,#228432,#228433,#228434,#228435,#228436,
#228437,#228438,#228439,#228440,#228441,#228442,#228443,#228444,#228445,
#228446,#228447,#228448,#228449,#228450,#228451,#228452,#228453,#228454,
#228455,#228456,#228457,#228458,#228459,#228460,#228461,#228462,#228463,
#228464,#228465,#228466,#228467,#228468,#228469,#228470,#228471,#228472,
#228473,#228474,#228475,#228476,#228477,#228478,#228479,#228480,#228481,
#228482,#228483,#228484,#228485,#228486,#228487,#228488,#228489,#228490,
#228491,#228492,#228493,#228494,#228495,#228496,#228497,#228498,#228499,
#228500,#228501,#228502,#228503,#228504,#228505,#228506,#228507,#228508,
#228509,#228510,#228511,#228512,#228513,#228514,#228515,#228516,#228517,
#228518,#228519,#228520,#228521,#228522,#228523,#228524,#228525,#228526,
#228527,#228528,#228529,#228530,#228531,#228532,#228533,#228534,#228535,
#228536,#228537,#228538,#228539,#228540,#228541,#228542,#228543,#228544,
#228545,#228546,#228547,#228548,#228549,#228550,#228551,#228552,#228553,
#228554,#228555,#228556,#228557,#228558,#228559,#228560,#228561,#228562,
#228563,#228564,#228565,#228566,#228567,#228568,#228569,#228570,#228571,
#228572,#228573,#228574),.UNSPECIFIED.,.F.,.F.,(4,3,3,3,3,3,3,3,3,3,3,3,
3,3,3,3,3,3,3,3,3,3,3,3,3,3,3,3,3,3,3,3,3,3,3,3,3,3,3,3,3,3,3,3,3,3,3,3,
3,3,3,3,3,3,3,3,3,3,3,3,3,3,3,3,3,3,3,3,3,3,3,3,3,3,3,3,3,3,3,3,3,3,3,3,
3,3,3,3,3,3,3,3,3,3,3,3,3,3,3,3,3,3,3,3,3,3,3,4),(0.143172102,0.15412844,
0.165137615,0.176146789,0.187155963,0.198165138,0.211009174,0.222018349,
0.233027523,0.244036697,0.255045872,0.267889908,0.278899083,0.289908257,
0.300917431,0.311926606,0.32293578,0.333944954,0.344954128,0.355963303,
0.366972477,0.377981651,0.388990826,0.398165138,0.40733945,0.416513761,
0.427522936,0.436697248,0.44587156,0.455045872,0.464220183,0.473394495,
0.48440367,0.493577982,0.502752294,0.511926606,0.521100917,0.530275229,
0.537614679,0.544954128,0.552293578,0.559633028,0.566972477,0.574311927,
0.581651376,0.588990826,0.596330275,0.603669725,0.611009174,0.618348624,
0.625688073,0.633027523,0.640366972,0.647706422,0.655045872,0.664220183,
0.671559633,0.678899083,0.686238532,0.693577982,0.700917431,0.710091743,
0.717431193,0.724770642,0.733944954,0.741284404,0.748623853,0.755963303,
0.763302752,0.772477064,0.779816514,0.787155963,0.794495413,0.803669725,
0.811009174,0.816513761,0.822018349,0.827522936,0.833027523,0.83853211,
0.844036697,0.849541284,0.855045872,0.860550459,0.867889908,0.873394495,
0.878899083,0.88440367,0.889908257,0.895412844,0.900917431,0.906422018,
0.911926606,0.917431193,0.924770642,0.930275229,0.935779817,0.941284404,
0.946788991,0.95412844,0.96146789,0.966972477,0.972477064,0.977981651,0.983486239,
0.988990826,0.994495413,1.),.UNSPECIFIED.);
#24409=B_SPLINE_CURVE_WITH_KNOTS('',3,(#229522,#229523,#229524,#229525,
#229526,#229527,#229528,#229529,#229530,#229531,#229532,#229533,#229534,
#229535,#229536,#229537,#229538,#229539,#229540,#229541,#229542,#229543,
#229544,#229545,#229546,#229547,#229548,#229549,#229550,#229551,#229552,
#229553,#229554,#229555,#229556,#229557,#229558,#229559,#229560,#229561,
#229562,#229563,#229564,#229565,#229566,#229567,#229568,#229569,#229570,
#229571,#229572,#229573,#229574,#229575,#229576,#229577,#229578,#229579,
#229580,#229581,#229582,#229583,#229584,#229585,#229586,#229587,#229588,
#229589,#229590,#229591,#229592,#229593,#229594,#229595,#229596,#229597,
#229598,#229599,#229600,#229601,#229602,#229603,#229604,#229605,#229606,
#229607,#229608,#229609,#229610,#229611,#229612,#229613,#229614,#229615,
#229616,#229617,#229618,#229619,#229620,#229621,#229622,#229623,#229624,
#229625,#229626,#229627,#229628,#229629,#229630,#229631,#229632,#229633,
#229634,#229635,#229636,#229637,#229638,#229639,#229640,#229641,#229642,
#229643,#229644,#229645,#229646,#229647,#229648,#229649,#229650,#229651,
#229652,#229653,#229654,#229655,#229656,#229657,#229658,#229659,#229660,
#229661,#229662,#229663,#229664,#229665,#229666,#229667,#229668,#229669,
#229670,#229671,#229672,#229673,#229674,#229675,#229676,#229677,#229678,
#229679,#229680,#229681,#229682,#229683,#229684,#229685,#229686,#229687,
#229688,#229689,#229690,#229691,#229692,#229693,#229694,#229695,#229696,
#229697,#229698,#229699,#229700,#229701,#229702,#229703,#229704,#229705,
#229706,#229707,#229708,#229709,#229710,#229711,#229712,#229713,#229714,
#229715,#229716,#229717,#229718,#229719,#229720,#229721,#229722,#229723,
#229724,#229725,#229726,#229727,#229728,#229729,#229730,#229731,#229732,
#229733,#229734,#229735,#229736,#229737,#229738,#229739,#229740,#229741,
#229742,#229743,#229744,#229745,#229746,#229747,#229748,#229749,#229750,
#229751,#229752,#229753,#229754,#229755,#229756,#229757,#229758,#229759,
#229760,#229761,#229762,#229763,#229764,#229765,#229766,#229767,#229768,
#229769,#229770,#229771,#229772,#229773,#229774,#229775,#229776,#229777,
#229778,#229779,#229780,#229781,#229782,#229783,#229784,#229785,#229786,
#229787,#229788,#229789,#229790,#229791,#229792,#229793,#229794,#229795,
#229796,#229797,#229798,#229799,#229800,#229801,#229802,#229803,#229804,
#229805,#229806,#229807,#229808,#229809,#229810,#229811,#229812,#229813,
#229814,#229815,#229816,#229817,#229818,#229819,#229820,#229821,#229822,
#229823,#229824,#229825,#229826,#229827,#229828,#229829,#229830,#229831,
#229832,#229833,#229834,#229835,#229836,#229837,#229838,#229839,#229840,
#229841,#229842,#229843),.UNSPECIFIED.,.F.,.F.,(4,3,3,3,3,3,3,3,3,3,3,3,
3,3,3,3,3,3,3,3,3,3,3,3,3,3,3,3,3,3,3,3,3,3,3,3,3,3,3,3,3,3,3,3,3,3,3,3,
3,3,3,3,3,3,3,3,3,3,3,3,3,3,3,3,3,3,3,3,3,3,3,3,3,3,3,3,3,3,3,3,3,3,3,3,
3,3,3,3,3,3,3,3,3,3,3,3,3,3,3,3,3,3,3,3,3,3,3,4),(-1.,-0.994495413,-0.988990826,
-0.983486239,-0.977981651,-0.970642202,-0.965137615,-0.959633028,-0.95412844,
-0.948623853,-0.943119266,-0.937614679,-0.932110092,-0.926605505,-0.921100917,
-0.91559633,-0.910091743,-0.904587156,-0.899082569,-0.893577982,-0.888073394,
-0.882568807,-0.87706422,-0.871559633,-0.866055046,-0.860550459,-0.855045872,
-0.849541284,-0.842201835,-0.836697248,-0.831192661,-0.825688073,-0.820183486,
-0.814678899,-0.809174312,-0.801834862,-0.794495413,-0.787155963,-0.779816514,
-0.770642202,-0.763302752,-0.755963303,-0.746788991,-0.737614679,-0.730275229,
-0.72293578,-0.71559633,-0.706422018,-0.699082569,-0.691743119,-0.68440367,
-0.675229358,-0.666055046,-0.658715596,-0.651376147,-0.644036697,-0.636697248,
-0.629357798,-0.622018349,-0.614678899,-0.60733945,-0.6,-0.59266055,-0.585321101,
-0.577981651,-0.570642202,-0.563302752,-0.555963303,-0.546788991,-0.537614679,
-0.530275229,-0.521100917,-0.511926606,-0.502752294,-0.493577982,-0.48440367,
-0.475229358,-0.466055046,-0.453211009,-0.444036697,-0.434862385,-0.425688073,
-0.414678899,-0.405504587,-0.396330275,-0.387155963,-0.376146789,-0.365137615,
-0.35412844,-0.343119266,-0.332110092,-0.321100917,-0.308256881,-0.297247706,
-0.286238532,-0.275229358,-0.264220183,-0.253211009,-0.242201835,-0.231192661,
-0.220183486,-0.209174312,-0.198165138,-0.187155963,-0.176146789,-0.165137615,
-0.15412844,-0.143172102),.UNSPECIFIED.);
#24410=B_SPLINE_CURVE_WITH_KNOTS('',3,(#229844,#229845,#229846,#229847,
#229848,#229849,#229850,#229851,#229852,#229853,#229854,#229855,#229856,
#229857,#229858,#229859,#229860,#229861,#229862,#229863,#229864,#229865,
#229866,#229867,#229868,#229869,#229870,#229871,#229872,#229873,#229874,
#229875,#229876,#229877,#229878,#229879,#229880,#229881,#229882,#229883,
#229884,#229885,#229886,#229887,#229888,#229889,#229890,#229891,#229892,
#229893,#229894,#229895,#229896,#229897,#229898,#229899,#229900,#229901,
#229902,#229903,#229904,#229905,#229906,#229907,#229908,#229909,#229910,
#229911,#229912,#229913,#229914,#229915,#229916,#229917,#229918,#229919,
#229920,#229921,#229922,#229923,#229924,#229925,#229926,#229927,#229928,
#229929,#229930,#229931,#229932,#229933,#229934,#229935,#229936,#229937,
#229938,#229939,#229940,#229941,#229942,#229943,#229944,#229945,#229946,
#229947,#229948,#229949,#229950,#229951,#229952,#229953,#229954,#229955,
#229956,#229957,#229958,#229959,#229960,#229961,#229962,#229963,#229964,
#229965,#229966,#229967,#229968,#229969,#229970,#229971,#229972,#229973,
#229974,#229975,#229976,#229977,#229978,#229979,#229980,#229981,#229982,
#229983,#229984,#229985,#229986,#229987,#229988,#229989,#229990,#229991,
#229992,#229993,#229994,#229995,#229996,#229997,#229998,#229999,#230000,
#230001,#230002,#230003,#230004,#230005,#230006,#230007,#230008,#230009,
#230010,#230011,#230012,#230013,#230014,#230015,#230016,#230017,#230018,
#230019,#230020,#230021,#230022,#230023,#230024,#230025,#230026,#230027,
#230028,#230029,#230030,#230031,#230032,#230033,#230034,#230035,#230036,
#230037,#230038,#230039,#230040,#230041,#230042,#230043,#230044,#230045,
#230046,#230047,#230048,#230049,#230050,#230051,#230052,#230053,#230054,
#230055,#230056,#230057,#230058,#230059,#230060,#230061,#230062,#230063,
#230064,#230065,#230066,#230067,#230068,#230069,#230070,#230071,#230072,
#230073,#230074,#230075,#230076,#230077,#230078,#230079,#230080,#230081,
#230082,#230083,#230084,#230085,#230086,#230087,#230088,#230089,#230090,
#230091,#230092,#230093,#230094,#230095,#230096,#230097,#230098,#230099,
#230100,#230101,#230102,#230103,#230104,#230105,#230106,#230107,#230108,
#230109,#230110,#230111,#230112,#230113,#230114,#230115,#230116,#230117,
#230118,#230119,#230120,#230121,#230122,#230123,#230124,#230125,#230126,
#230127,#230128,#230129,#230130,#230131,#230132),.UNSPECIFIED.,.F.,.F.,
(4,3,3,3,3,3,3,3,3,3,3,3,3,3,3,3,3,3,3,3,3,3,3,3,3,3,3,3,3,3,3,3,3,3,3,
3,3,3,3,3,3,3,3,3,3,3,3,3,3,3,3,3,3,3,3,3,3,3,3,3,3,3,3,3,3,3,3,3,3,3,3,
3,3,3,3,3,3,3,3,3,3,3,3,3,3,3,3,3,3,3,3,3,3,3,3,3,4),(0.143172102,0.15412844,
0.165137615,0.176146789,0.187155963,0.198165138,0.209174312,0.220183486,
0.231192661,0.242201835,0.253211009,0.264220183,0.278899083,0.291743119,
0.302752294,0.31559633,0.326605505,0.337614679,0.350458716,0.363302752,
0.374311927,0.385321101,0.403669725,0.412844037,0.425688073,0.434862385,
0.444036697,0.453211009,0.466055046,0.475229358,0.48440367,0.493577982,
0.506422018,0.517431193,0.526605505,0.533944954,0.541284404,0.55412844,
0.565137615,0.572477064,0.585321101,0.594495413,0.601834862,0.611009174,
0.618348624,0.629357798,0.636697248,0.649541284,0.656880734,0.664220183,
0.671559633,0.678899083,0.688073394,0.697247706,0.704587156,0.711926606,
0.719266055,0.728440367,0.735779817,0.744954128,0.75412844,0.763302752,
0.770642202,0.777981651,0.785321101,0.79266055,0.803669725,0.811009174,
0.816513761,0.825688073,0.833027523,0.83853211,0.84587156,0.851376147,0.858715596,
0.864220183,0.871559633,0.87706422,0.882568807,0.888073394,0.893577982,
0.899082569,0.906422018,0.911926606,0.917431193,0.926605505,0.932110092,
0.939449541,0.944954128,0.95412844,0.959633028,0.968807339,0.974311927,
0.979816514,0.985321101,0.994495413,1.),.UNSPECIFIED.);
#24411=B_SPLINE_CURVE_WITH_KNOTS('',3,(#231095,#231096,#231097,#231098,
#231099,#231100,#231101,#231102,#231103,#231104,#231105,#231106,#231107,
#231108,#231109,#231110,#231111,#231112,#231113,#231114,#231115,#231116,
#231117,#231118,#231119,#231120,#231121,#231122,#231123,#231124,#231125,
#231126,#231127,#231128,#231129,#231130,#231131,#231132,#231133,#231134,
#231135,#231136,#231137,#231138,#231139,#231140,#231141,#231142,#231143,
#231144,#231145,#231146,#231147,#231148,#231149,#231150,#231151,#231152,
#231153,#231154,#231155,#231156,#231157,#231158,#231159,#231160,#231161,
#231162,#231163,#231164,#231165,#231166,#231167,#231168,#231169,#231170,
#231171,#231172,#231173,#231174,#231175,#231176,#231177,#231178,#231179,
#231180,#231181,#231182,#231183,#231184,#231185,#231186,#231187,#231188,
#231189,#231190,#231191,#231192,#231193,#231194,#231195,#231196,#231197,
#231198,#231199,#231200,#231201,#231202,#231203,#231204,#231205,#231206,
#231207,#231208,#231209,#231210,#231211,#231212,#231213,#231214,#231215,
#231216,#231217,#231218,#231219,#231220,#231221,#231222,#231223,#231224,
#231225,#231226,#231227,#231228,#231229,#231230,#231231,#231232,#231233,
#231234,#231235,#231236,#231237,#231238,#231239,#231240,#231241,#231242,
#231243,#231244,#231245,#231246,#231247,#231248,#231249,#231250,#231251,
#231252,#231253,#231254,#231255,#231256,#231257,#231258,#231259,#231260,
#231261,#231262,#231263,#231264,#231265,#231266,#231267,#231268,#231269,
#231270,#231271,#231272,#231273,#231274,#231275,#231276,#231277,#231278,
#231279,#231280,#231281,#231282,#231283,#231284,#231285,#231286,#231287,
#231288,#231289,#231290,#231291,#231292,#231293,#231294,#231295,#231296,
#231297,#231298,#231299,#231300,#231301,#231302,#231303,#231304,#231305,
#231306,#231307,#231308,#231309,#231310,#231311,#231312,#231313,#231314,
#231315,#231316,#231317,#231318,#231319,#231320,#231321,#231322,#231323,
#231324,#231325,#231326,#231327,#231328,#231329,#231330,#231331,#231332,
#231333,#231334,#231335,#231336,#231337,#231338,#231339,#231340,#231341,
#231342,#231343,#231344,#231345,#231346,#231347,#231348,#231349,#231350,
#231351,#231352,#231353,#231354,#231355,#231356,#231357,#231358,#231359,
#231360,#231361,#231362,#231363,#231364,#231365,#231366,#231367,#231368,
#231369,#231370,#231371,#231372,#231373,#231374,#231375,#231376,#231377,
#231378,#231379,#231380,#231381,#231382,#231383,#231384,#231385,#231386,
#231387,#231388,#231389,#231390,#231391,#231392,#231393,#231394,#231395,
#231396,#231397,#231398,#231399,#231400,#231401,#231402,#231403,#231404,
#231405,#231406,#231407,#231408,#231409,#231410,#231411,#231412,#231413),
 .UNSPECIFIED.,.F.,.F.,(4,3,3,3,3,3,3,3,3,3,3,3,3,3,3,3,3,3,3,3,3,3,3,3,
3,3,3,3,3,3,3,3,3,3,3,3,3,3,3,3,3,3,3,3,3,3,3,3,3,3,3,3,3,3,3,3,3,3,3,3,
3,3,3,3,3,3,3,3,3,3,3,3,3,3,3,3,3,3,3,3,3,3,3,3,3,3,3,3,3,3,3,3,3,3,3,3,
3,3,3,3,3,3,3,3,3,3,4),(-1.,-0.990825688,-0.985321101,-0.979816514,-0.974311927,
-0.965137615,-0.959633028,-0.95412844,-0.948623853,-0.943119266,-0.937614679,
-0.932110092,-0.926605505,-0.921100917,-0.91559633,-0.910091743,-0.904587156,
-0.899082569,-0.893577982,-0.888073394,-0.882568807,-0.87706422,-0.871559633,
-0.866055046,-0.860550459,-0.855045872,-0.849541284,-0.844036697,-0.83853211,
-0.833027523,-0.827522936,-0.822018349,-0.814678899,-0.809174312,-0.801834862,
-0.794495413,-0.787155963,-0.779816514,-0.772477064,-0.765137615,-0.757798165,
-0.750458716,-0.743119266,-0.735779817,-0.728440367,-0.721100917,-0.711926606,
-0.704587156,-0.697247706,-0.689908257,-0.682568807,-0.675229358,-0.666055046,
-0.658715596,-0.651376147,-0.644036697,-0.636697248,-0.627522936,-0.620183486,
-0.612844037,-0.605504587,-0.598165138,-0.590825688,-0.583486239,-0.576146789,
-0.568807339,-0.559633028,-0.550458716,-0.543119266,-0.535779817,-0.528440367,
-0.519266055,-0.508256881,-0.499082569,-0.489908257,-0.480733945,-0.471559633,
-0.462385321,-0.453211009,-0.444036697,-0.434862385,-0.425688073,-0.414678899,
-0.405504587,-0.396330275,-0.383486239,-0.372477064,-0.36146789,-0.350458716,
-0.339449541,-0.328440367,-0.317431193,-0.306422018,-0.293577982,-0.282568807,
-0.271559633,-0.260550459,-0.249541284,-0.23853211,-0.227522936,-0.216513761,
-0.205504587,-0.194495413,-0.183486239,-0.172477064,-0.16146789,-0.143172102),
 .UNSPECIFIED.);
#24412=B_SPLINE_CURVE_WITH_KNOTS('',3,(#231414,#231415,#231416,#231417,
#231418,#231419,#231420,#231421,#231422,#231423,#231424,#231425,#231426,
#231427,#231428,#231429,#231430,#231431,#231432,#231433,#231434,#231435,
#231436,#231437,#231438,#231439,#231440,#231441,#231442,#231443,#231444,
#231445,#231446,#231447,#231448,#231449,#231450,#231451,#231452,#231453,
#231454,#231455,#231456,#231457,#231458,#231459,#231460,#231461,#231462,
#231463,#231464,#231465,#231466,#231467,#231468,#231469,#231470,#231471,
#231472,#231473,#231474,#231475,#231476,#231477,#231478,#231479,#231480,
#231481,#231482,#231483,#231484,#231485,#231486,#231487,#231488,#231489,
#231490,#231491,#231492,#231493,#231494,#231495,#231496,#231497,#231498,
#231499,#231500,#231501,#231502,#231503,#231504,#231505,#231506,#231507,
#231508,#231509,#231510,#231511,#231512,#231513,#231514,#231515,#231516,
#231517,#231518,#231519,#231520,#231521,#231522,#231523,#231524,#231525,
#231526,#231527,#231528,#231529,#231530,#231531,#231532,#231533,#231534,
#231535,#231536,#231537,#231538,#231539,#231540,#231541,#231542,#231543,
#231544,#231545,#231546,#231547,#231548,#231549,#231550,#231551,#231552,
#231553,#231554,#231555,#231556,#231557,#231558,#231559,#231560,#231561,
#231562,#231563,#231564,#231565,#231566,#231567,#231568,#231569,#231570,
#231571,#231572,#231573,#231574,#231575,#231576,#231577,#231578,#231579,
#231580,#231581,#231582,#231583,#231584,#231585,#231586,#231587,#231588,
#231589,#231590,#231591,#231592,#231593,#231594,#231595,#231596,#231597,
#231598,#231599,#231600,#231601,#231602,#231603,#231604,#231605,#231606,
#231607,#231608,#231609,#231610,#231611,#231612,#231613,#231614,#231615,
#231616,#231617,#231618,#231619,#231620,#231621,#231622,#231623,#231624,
#231625,#231626,#231627,#231628,#231629,#231630,#231631,#231632,#231633,
#231634,#231635,#231636,#231637,#231638,#231639,#231640,#231641,#231642,
#231643,#231644,#231645,#231646,#231647,#231648,#231649,#231650,#231651,
#231652,#231653,#231654,#231655,#231656,#231657,#231658,#231659,#231660,
#231661,#231662,#231663,#231664,#231665,#231666,#231667,#231668,#231669,
#231670,#231671,#231672,#231673,#231674,#231675,#231676,#231677,#231678,
#231679,#231680,#231681,#231682,#231683,#231684,#231685,#231686,#231687,
#231688,#231689,#231690,#231691,#231692,#231693,#231694,#231695,#231696,
#231697,#231698,#231699,#231700,#231701,#231702,#231703,#231704,#231705),
 .UNSPECIFIED.,.F.,.F.,(4,3,3,3,3,3,3,3,3,3,3,3,3,3,3,3,3,3,3,3,3,3,3,3,
3,3,3,3,3,3,3,3,3,3,3,3,3,3,3,3,3,3,3,3,3,3,3,3,3,3,3,3,3,3,3,3,3,3,3,3,
3,3,3,3,3,3,3,3,3,3,3,3,3,3,3,3,3,3,3,3,3,3,3,3,3,3,3,3,3,3,3,3,3,3,3,3,
3,4),(0.143172102,0.15412844,0.165137615,0.176146789,0.187155963,0.198165138,
0.209174312,0.220183486,0.231192661,0.242201835,0.253211009,0.264220183,
0.275229358,0.286238532,0.299082569,0.310091743,0.321100917,0.332110092,
0.343119266,0.35412844,0.366972477,0.379816514,0.39266055,0.401834862,0.412844037,
0.422018349,0.431192661,0.440366972,0.453211009,0.462385321,0.471559633,
0.480733945,0.489908257,0.500917431,0.513761468,0.52293578,0.532110092,
0.539449541,0.546788991,0.55412844,0.563302752,0.570642202,0.579816514,
0.587155963,0.596330275,0.603669725,0.611009174,0.620183486,0.631192661,
0.640366972,0.649541284,0.658715596,0.666055046,0.673394495,0.680733945,
0.688073394,0.695412844,0.706422018,0.71559633,0.72293578,0.733944954,0.743119266,
0.750458716,0.76146789,0.768807339,0.776146789,0.783486239,0.79266055,0.801834862,
0.809174312,0.818348624,0.825688073,0.831192661,0.836697248,0.842201835,
0.849541284,0.858715596,0.864220183,0.869724771,0.87706422,0.886238532,
0.893577982,0.899082569,0.906422018,0.913761468,0.919266055,0.924770642,
0.930275229,0.935779817,0.944954128,0.95412844,0.959633028,0.968807339,
0.974311927,0.979816514,0.985321101,0.990825688,1.),.UNSPECIFIED.);
#24413=B_SPLINE_CURVE_WITH_KNOTS('',3,(#232650,#232651,#232652,#232653,
#232654,#232655,#232656,#232657,#232658,#232659,#232660,#232661,#232662,
#232663,#232664,#232665,#232666,#232667,#232668,#232669,#232670,#232671,
#232672,#232673,#232674,#232675,#232676,#232677,#232678,#232679,#232680,
#232681,#232682,#232683,#232684,#232685,#232686,#232687,#232688,#232689,
#232690,#232691,#232692,#232693,#232694,#232695,#232696,#232697,#232698,
#232699,#232700,#232701,#232702,#232703,#232704,#232705,#232706,#232707,
#232708,#232709,#232710,#232711,#232712,#232713,#232714,#232715,#232716,
#232717,#232718,#232719,#232720,#232721,#232722,#232723,#232724,#232725,
#232726,#232727,#232728,#232729,#232730,#232731,#232732,#232733,#232734,
#232735,#232736,#232737,#232738,#232739,#232740,#232741,#232742,#232743,
#232744,#232745,#232746,#232747,#232748,#232749,#232750,#232751,#232752,
#232753,#232754,#232755,#232756,#232757,#232758,#232759,#232760,#232761,
#232762,#232763,#232764,#232765,#232766,#232767,#232768,#232769,#232770,
#232771,#232772,#232773,#232774,#232775,#232776,#232777,#232778,#232779,
#232780,#232781,#232782,#232783,#232784,#232785,#232786,#232787,#232788,
#232789,#232790,#232791,#232792,#232793,#232794,#232795,#232796,#232797,
#232798,#232799,#232800,#232801,#232802,#232803,#232804,#232805,#232806,
#232807,#232808,#232809,#232810,#232811,#232812,#232813,#232814,#232815,
#232816,#232817,#232818,#232819,#232820,#232821,#232822,#232823,#232824,
#232825,#232826,#232827,#232828,#232829,#232830,#232831,#232832,#232833,
#232834,#232835,#232836,#232837,#232838,#232839,#232840,#232841,#232842,
#232843,#232844,#232845,#232846,#232847,#232848,#232849,#232850,#232851,
#232852,#232853,#232854,#232855,#232856,#232857,#232858,#232859,#232860,
#232861,#232862,#232863,#232864,#232865,#232866,#232867,#232868,#232869,
#232870,#232871,#232872,#232873,#232874,#232875,#232876,#232877,#232878,
#232879,#232880,#232881,#232882,#232883,#232884,#232885,#232886,#232887,
#232888,#232889,#232890,#232891,#232892,#232893,#232894,#232895,#232896,
#232897,#232898,#232899,#232900,#232901,#232902,#232903,#232904,#232905,
#232906,#232907,#232908,#232909,#232910,#232911,#232912,#232913,#232914,
#232915,#232916,#232917,#232918,#232919,#232920,#232921,#232922,#232923,
#232924,#232925,#232926,#232927,#232928,#232929,#232930,#232931,#232932,
#232933,#232934,#232935,#232936,#232937,#232938,#232939,#232940,#232941,
#232942,#232943,#232944,#232945,#232946,#232947,#232948,#232949,#232950,
#232951,#232952,#232953),.UNSPECIFIED.,.F.,.F.,(4,3,3,3,3,3,3,3,3,3,3,3,
3,3,3,3,3,3,3,3,3,3,3,3,3,3,3,3,3,3,3,3,3,3,3,3,3,3,3,3,3,3,3,3,3,3,3,3,
3,3,3,3,3,3,3,3,3,3,3,3,3,3,3,3,3,3,3,3,3,3,3,3,3,3,3,3,3,3,3,3,3,3,3,3,
3,3,3,3,3,3,3,3,3,3,3,3,3,3,3,3,3,4),(0.143172102,0.15412844,0.165137615,
0.176146789,0.187155963,0.198165138,0.209174312,0.220183486,0.231192661,
0.242201835,0.253211009,0.264220183,0.27706422,0.289908257,0.300917431,
0.313761468,0.324770642,0.335779817,0.348623853,0.359633028,0.370642202,
0.383486239,0.394495413,0.403669725,0.412844037,0.423853211,0.433027523,
0.442201835,0.451376147,0.460550459,0.473394495,0.482568807,0.491743119,
0.500917431,0.510091743,0.519266055,0.528440367,0.535779817,0.543119266,
0.550458716,0.557798165,0.565137615,0.574311927,0.583486239,0.590825688,
0.598165138,0.605504587,0.612844037,0.622018349,0.629357798,0.636697248,
0.644036697,0.651376147,0.664220183,0.673394495,0.680733945,0.689908257,
0.699082569,0.710091743,0.719266055,0.726605505,0.735779817,0.743119266,
0.750458716,0.757798165,0.765137615,0.774311927,0.781651376,0.788990826,
0.796330275,0.803669725,0.812844037,0.820183486,0.825688073,0.831192661,
0.83853211,0.844036697,0.851376147,0.856880734,0.862385321,0.867889908,
0.873394495,0.878899083,0.88440367,0.891743119,0.897247706,0.904587156,
0.910091743,0.91559633,0.921100917,0.928440367,0.933944954,0.939449541,
0.948623853,0.955963303,0.96146789,0.966972477,0.974311927,0.979816514,
0.985321101,0.990825688,1.),.UNSPECIFIED.);
#24414=B_SPLINE_CURVE_WITH_KNOTS('',3,(#232954,#232955,#232956,#232957,
#232958,#232959,#232960,#232961,#232962,#232963,#232964,#232965,#232966,
#232967,#232968,#232969,#232970,#232971,#232972,#232973,#232974,#232975,
#232976,#232977,#232978,#232979,#232980,#232981,#232982,#232983,#232984,
#232985,#232986,#232987,#232988,#232989,#232990,#232991,#232992,#232993,
#232994,#232995,#232996,#232997,#232998,#232999,#233000,#233001,#233002,
#233003,#233004,#233005,#233006,#233007,#233008,#233009,#233010,#233011,
#233012,#233013,#233014,#233015,#233016,#233017,#233018,#233019,#233020,
#233021,#233022,#233023,#233024,#233025,#233026,#233027,#233028,#233029,
#233030,#233031,#233032,#233033,#233034,#233035,#233036,#233037,#233038,
#233039,#233040,#233041,#233042,#233043,#233044,#233045,#233046,#233047,
#233048,#233049,#233050,#233051,#233052,#233053,#233054,#233055,#233056,
#233057,#233058,#233059,#233060,#233061,#233062,#233063,#233064,#233065,
#233066,#233067,#233068,#233069,#233070,#233071,#233072,#233073,#233074,
#233075,#233076,#233077,#233078,#233079,#233080,#233081,#233082,#233083,
#233084,#233085,#233086,#233087,#233088,#233089,#233090,#233091,#233092,
#233093,#233094,#233095,#233096,#233097,#233098,#233099,#233100,#233101,
#233102,#233103,#233104,#233105,#233106,#233107,#233108,#233109,#233110,
#233111,#233112,#233113,#233114,#233115,#233116,#233117,#233118,#233119,
#233120,#233121,#233122,#233123,#233124,#233125,#233126,#233127,#233128,
#233129,#233130,#233131,#233132,#233133,#233134,#233135,#233136,#233137,
#233138,#233139,#233140,#233141,#233142,#233143,#233144,#233145,#233146,
#233147,#233148,#233149,#233150,#233151,#233152,#233153,#233154,#233155,
#233156,#233157,#233158,#233159,#233160,#233161,#233162,#233163,#233164,
#233165,#233166,#233167,#233168,#233169,#233170,#233171,#233172,#233173,
#233174,#233175,#233176,#233177,#233178,#233179,#233180,#233181,#233182,
#233183,#233184,#233185,#233186,#233187,#233188,#233189,#233190,#233191,
#233192,#233193,#233194,#233195,#233196,#233197,#233198,#233199,#233200,
#233201,#233202,#233203,#233204,#233205,#233206,#233207,#233208,#233209,
#233210,#233211,#233212,#233213,#233214,#233215,#233216,#233217,#233218,
#233219,#233220,#233221,#233222,#233223,#233224,#233225,#233226,#233227,
#233228,#233229,#233230,#233231,#233232,#233233,#233234,#233235,#233236,
#233237,#233238,#233239,#233240,#233241,#233242,#233243,#233244,#233245,
#233246,#233247,#233248,#233249,#233250,#233251,#233252,#233253,#233254,
#233255,#233256,#233257,#233258,#233259,#233260,#233261,#233262,#233263,
#233264,#233265,#233266,#233267,#233268,#233269,#233270,#233271,#233272),
 .UNSPECIFIED.,.F.,.F.,(4,3,3,3,3,3,3,3,3,3,3,3,3,3,3,3,3,3,3,3,3,3,3,3,
3,3,3,3,3,3,3,3,3,3,3,3,3,3,3,3,3,3,3,3,3,3,3,3,3,3,3,3,3,3,3,3,3,3,3,3,
3,3,3,3,3,3,3,3,3,3,3,3,3,3,3,3,3,3,3,3,3,3,3,3,3,3,3,3,3,3,3,3,3,3,3,3,
3,3,3,3,3,3,3,3,3,3,4),(0.143172102,0.15412844,0.165137615,0.176146789,
0.187155963,0.198165138,0.209174312,0.220183486,0.231192661,0.242201835,
0.253211009,0.264220183,0.27706422,0.289908257,0.300917431,0.311926606,
0.32293578,0.333944954,0.344954128,0.355963303,0.366972477,0.377981651,
0.388990826,0.398165138,0.40733945,0.416513761,0.425688073,0.434862385,
0.44587156,0.455045872,0.464220183,0.473394495,0.482568807,0.491743119,
0.500917431,0.510091743,0.519266055,0.528440367,0.535779817,0.543119266,
0.550458716,0.557798165,0.565137615,0.572477064,0.579816514,0.587155963,
0.598165138,0.605504587,0.612844037,0.620183486,0.629357798,0.636697248,
0.644036697,0.651376147,0.658715596,0.666055046,0.673394495,0.680733945,
0.688073394,0.695412844,0.702752294,0.710091743,0.717431193,0.724770642,
0.732110092,0.739449541,0.746788991,0.75412844,0.76146789,0.770642202,0.777981651,
0.785321101,0.79266055,0.8,0.80733945,0.812844037,0.820183486,0.825688073,
0.831192661,0.83853211,0.844036697,0.849541284,0.855045872,0.860550459,
0.867889908,0.873394495,0.878899083,0.88440367,0.891743119,0.897247706,
0.902752294,0.908256881,0.913761468,0.921100917,0.926605505,0.933944954,
0.939449541,0.944954128,0.950458716,0.955963303,0.96146789,0.966972477,
0.972477064,0.977981651,0.983486239,0.990825688,1.),.UNSPECIFIED.);
#24415=B_SPLINE_CURVE_WITH_KNOTS('',3,(#234232,#234233,#234234,#234235,
#234236,#234237,#234238,#234239,#234240,#234241,#234242,#234243,#234244,
#234245,#234246,#234247,#234248,#234249,#234250,#234251,#234252,#234253,
#234254,#234255,#234256,#234257,#234258,#234259,#234260,#234261,#234262,
#234263,#234264,#234265,#234266,#234267,#234268,#234269,#234270,#234271,
#234272,#234273,#234274,#234275,#234276,#234277,#234278,#234279,#234280,
#234281,#234282,#234283,#234284,#234285,#234286,#234287,#234288,#234289,
#234290,#234291,#234292,#234293,#234294,#234295,#234296,#234297,#234298,
#234299,#234300,#234301,#234302,#234303,#234304,#234305,#234306,#234307,
#234308,#234309,#234310,#234311,#234312,#234313,#234314,#234315,#234316,
#234317,#234318,#234319,#234320,#234321,#234322,#234323,#234324,#234325,
#234326,#234327,#234328,#234329,#234330,#234331,#234332,#234333,#234334,
#234335,#234336,#234337,#234338,#234339,#234340,#234341,#234342,#234343,
#234344,#234345,#234346,#234347,#234348,#234349,#234350,#234351,#234352,
#234353,#234354,#234355,#234356,#234357,#234358,#234359,#234360,#234361,
#234362,#234363,#234364,#234365,#234366,#234367,#234368,#234369,#234370,
#234371,#234372,#234373,#234374,#234375,#234376,#234377,#234378,#234379,
#234380,#234381,#234382,#234383,#234384,#234385,#234386,#234387,#234388,
#234389,#234390,#234391,#234392,#234393,#234394,#234395,#234396,#234397,
#234398,#234399,#234400,#234401,#234402,#234403,#234404,#234405,#234406,
#234407,#234408,#234409,#234410,#234411,#234412,#234413,#234414,#234415,
#234416,#234417,#234418,#234419,#234420,#234421,#234422,#234423,#234424,
#234425,#234426,#234427,#234428,#234429,#234430,#234431,#234432,#234433,
#234434,#234435,#234436,#234437,#234438,#234439,#234440,#234441,#234442,
#234443,#234444,#234445,#234446,#234447,#234448,#234449,#234450,#234451,
#234452,#234453,#234454,#234455,#234456,#234457,#234458,#234459,#234460,
#234461,#234462,#234463,#234464,#234465,#234466,#234467,#234468,#234469,
#234470,#234471,#234472,#234473,#234474,#234475,#234476,#234477,#234478,
#234479,#234480,#234481,#234482,#234483,#234484,#234485,#234486,#234487,
#234488,#234489,#234490,#234491,#234492,#234493,#234494,#234495,#234496,
#234497,#234498,#234499,#234500,#234501,#234502,#234503,#234504,#234505,
#234506,#234507,#234508,#234509,#234510,#234511,#234512,#234513,#234514,
#234515,#234516,#234517,#234518,#234519,#234520,#234521,#234522,#234523,
#234524,#234525,#234526,#234527,#234528,#234529,#234530,#234531,#234532,
#234533,#234534,#234535,#234536,#234537,#234538,#234539,#234540,#234541),
 .UNSPECIFIED.,.F.,.F.,(4,3,3,3,3,3,3,3,3,3,3,3,3,3,3,3,3,3,3,3,3,3,3,3,
3,3,3,3,3,3,3,3,3,3,3,3,3,3,3,3,3,3,3,3,3,3,3,3,3,3,3,3,3,3,3,3,3,3,3,3,
3,3,3,3,3,3,3,3,3,3,3,3,3,3,3,3,3,3,3,3,3,3,3,3,3,3,3,3,3,3,3,3,3,3,3,3,
3,3,3,3,3,3,3,4),(0.143172102,0.15412844,0.165137615,0.176146789,0.187155963,
0.198165138,0.209174312,0.220183486,0.231192661,0.242201835,0.253211009,
0.264220183,0.275229358,0.286238532,0.297247706,0.308256881,0.319266055,
0.332110092,0.343119266,0.35412844,0.365137615,0.376146789,0.387155963,
0.396330275,0.405504587,0.414678899,0.423853211,0.433027523,0.442201835,
0.451376147,0.460550459,0.469724771,0.478899083,0.488073394,0.497247706,
0.506422018,0.51559633,0.524770642,0.533944954,0.541284404,0.550458716,
0.557798165,0.565137615,0.572477064,0.579816514,0.587155963,0.594495413,
0.601834862,0.609174312,0.622018349,0.629357798,0.642201835,0.649541284,
0.656880734,0.666055046,0.673394495,0.680733945,0.688073394,0.697247706,
0.706422018,0.71559633,0.724770642,0.732110092,0.739449541,0.746788991,
0.75412844,0.76146789,0.768807339,0.777981651,0.785321101,0.794495413,0.801834862,
0.812844037,0.818348624,0.823853211,0.829357798,0.834862385,0.840366972,
0.84587156,0.851376147,0.856880734,0.866055046,0.871559633,0.87706422,0.882568807,
0.888073394,0.895412844,0.900917431,0.908256881,0.913761468,0.92293578,
0.928440367,0.933944954,0.939449541,0.944954128,0.950458716,0.955963303,
0.96146789,0.968807339,0.974311927,0.979816514,0.988990826,0.994495413,
1.),.UNSPECIFIED.);
#24416=B_SPLINE_CURVE_WITH_KNOTS('',3,(#234542,#234543,#234544,#234545,
#234546,#234547,#234548,#234549,#234550,#234551,#234552,#234553,#234554,
#234555,#234556,#234557,#234558,#234559,#234560,#234561,#234562,#234563,
#234564,#234565,#234566,#234567,#234568,#234569,#234570,#234571,#234572,
#234573,#234574,#234575,#234576,#234577,#234578,#234579,#234580,#234581,
#234582,#234583,#234584,#234585,#234586,#234587,#234588,#234589,#234590,
#234591,#234592,#234593,#234594,#234595,#234596,#234597,#234598,#234599,
#234600,#234601,#234602,#234603,#234604,#234605,#234606,#234607,#234608,
#234609,#234610,#234611,#234612,#234613,#234614,#234615,#234616,#234617,
#234618,#234619,#234620,#234621,#234622,#234623,#234624,#234625,#234626,
#234627,#234628,#234629,#234630,#234631,#234632,#234633,#234634,#234635,
#234636,#234637,#234638,#234639,#234640,#234641,#234642,#234643,#234644,
#234645,#234646,#234647,#234648,#234649,#234650,#234651,#234652,#234653,
#234654,#234655,#234656,#234657,#234658,#234659,#234660,#234661,#234662,
#234663,#234664,#234665,#234666,#234667,#234668,#234669,#234670,#234671,
#234672,#234673,#234674,#234675,#234676,#234677,#234678,#234679,#234680,
#234681,#234682,#234683,#234684,#234685,#234686,#234687,#234688,#234689,
#234690,#234691,#234692,#234693,#234694,#234695,#234696,#234697,#234698,
#234699,#234700,#234701,#234702,#234703,#234704,#234705,#234706,#234707,
#234708,#234709,#234710,#234711,#234712,#234713,#234714,#234715,#234716,
#234717,#234718,#234719,#234720,#234721,#234722,#234723,#234724,#234725,
#234726,#234727,#234728,#234729,#234730,#234731,#234732,#234733,#234734,
#234735,#234736,#234737,#234738,#234739,#234740,#234741,#234742,#234743,
#234744,#234745,#234746,#234747,#234748,#234749,#234750,#234751,#234752,
#234753,#234754,#234755,#234756,#234757,#234758,#234759,#234760,#234761,
#234762,#234763,#234764,#234765,#234766,#234767,#234768,#234769,#234770,
#234771,#234772,#234773,#234774,#234775,#234776,#234777,#234778,#234779,
#234780,#234781,#234782,#234783,#234784,#234785,#234786,#234787,#234788,
#234789,#234790,#234791,#234792,#234793,#234794,#234795,#234796,#234797,
#234798,#234799,#234800,#234801,#234802,#234803,#234804,#234805,#234806,
#234807,#234808,#234809,#234810,#234811,#234812,#234813,#234814,#234815,
#234816,#234817,#234818,#234819,#234820,#234821,#234822,#234823,#234824,
#234825,#234826,#234827,#234828,#234829,#234830,#234831,#234832,#234833,
#234834,#234835,#234836,#234837,#234838,#234839,#234840,#234841,#234842,
#234843,#234844,#234845,#234846,#234847,#234848,#234849,#234850,#234851,
#234852,#234853,#234854,#234855,#234856,#234857,#234858,#234859,#234860,
#234861,#234862,#234863,#234864,#234865,#234866,#234867,#234868,#234869),
 .UNSPECIFIED.,.F.,.F.,(4,3,3,3,3,3,3,3,3,3,3,3,3,3,3,3,3,3,3,3,3,3,3,3,
3,3,3,3,3,3,3,3,3,3,3,3,3,3,3,3,3,3,3,3,3,3,3,3,3,3,3,3,3,3,3,3,3,3,3,3,
3,3,3,3,3,3,3,3,3,3,3,3,3,3,3,3,3,3,3,3,3,3,3,3,3,3,3,3,3,3,3,3,3,3,3,3,
3,3,3,3,3,3,3,3,3,3,3,3,3,4),(0.143172102,0.15412844,0.165137615,0.176146789,
0.187155963,0.198165138,0.209174312,0.220183486,0.231192661,0.242201835,
0.253211009,0.264220183,0.275229358,0.286238532,0.297247706,0.308256881,
0.319266055,0.332110092,0.343119266,0.35412844,0.365137615,0.376146789,
0.387155963,0.396330275,0.405504587,0.414678899,0.423853211,0.433027523,
0.442201835,0.451376147,0.460550459,0.469724771,0.478899083,0.488073394,
0.497247706,0.506422018,0.51559633,0.524770642,0.533944954,0.541284404,
0.548623853,0.555963303,0.563302752,0.570642202,0.577981651,0.585321101,
0.59266055,0.6,0.60733945,0.614678899,0.622018349,0.629357798,0.636697248,
0.644036697,0.651376147,0.658715596,0.666055046,0.673394495,0.680733945,
0.688073394,0.695412844,0.702752294,0.710091743,0.717431193,0.724770642,
0.732110092,0.739449541,0.746788991,0.75412844,0.76146789,0.768807339,0.776146789,
0.785321101,0.79266055,0.8,0.80733945,0.812844037,0.818348624,0.823853211,
0.829357798,0.834862385,0.840366972,0.84587156,0.851376147,0.856880734,
0.862385321,0.867889908,0.873394495,0.878899083,0.88440367,0.889908257,
0.895412844,0.900917431,0.906422018,0.911926606,0.917431193,0.92293578,
0.928440367,0.933944954,0.939449541,0.944954128,0.950458716,0.955963303,
0.96146789,0.968807339,0.974311927,0.979816514,0.987155963,0.994495413,
1.),.UNSPECIFIED.);
#24417=B_SPLINE_CURVE_WITH_KNOTS('',3,(#235817,#235818,#235819,#235820,
#235821,#235822,#235823,#235824,#235825,#235826,#235827,#235828,#235829,
#235830,#235831,#235832,#235833,#235834,#235835,#235836,#235837,#235838,
#235839,#235840,#235841,#235842,#235843,#235844,#235845,#235846,#235847,
#235848,#235849,#235850,#235851,#235852,#235853,#235854,#235855,#235856,
#235857,#235858,#235859,#235860,#235861,#235862,#235863,#235864,#235865,
#235866,#235867,#235868,#235869,#235870,#235871,#235872,#235873,#235874,
#235875,#235876,#235877,#235878,#235879,#235880,#235881,#235882,#235883,
#235884,#235885,#235886,#235887,#235888,#235889,#235890,#235891,#235892,
#235893,#235894,#235895,#235896,#235897,#235898,#235899,#235900,#235901,
#235902,#235903,#235904,#235905,#235906,#235907,#235908,#235909,#235910,
#235911,#235912,#235913,#235914,#235915,#235916,#235917,#235918,#235919,
#235920,#235921,#235922,#235923,#235924,#235925,#235926,#235927,#235928,
#235929,#235930,#235931,#235932,#235933,#235934,#235935,#235936,#235937,
#235938,#235939,#235940,#235941,#235942,#235943,#235944,#235945,#235946,
#235947,#235948,#235949,#235950,#235951,#235952,#235953,#235954,#235955,
#235956,#235957,#235958,#235959,#235960,#235961,#235962,#235963,#235964,
#235965,#235966,#235967,#235968,#235969,#235970,#235971,#235972,#235973,
#235974,#235975,#235976,#235977,#235978,#235979,#235980,#235981,#235982,
#235983,#235984,#235985,#235986,#235987,#235988,#235989,#235990,#235991,
#235992,#235993,#235994,#235995,#235996,#235997,#235998,#235999,#236000,
#236001,#236002,#236003,#236004,#236005,#236006,#236007,#236008,#236009,
#236010,#236011,#236012,#236013,#236014,#236015,#236016,#236017,#236018,
#236019,#236020,#236021,#236022,#236023,#236024,#236025,#236026,#236027,
#236028,#236029,#236030,#236031,#236032,#236033,#236034,#236035,#236036,
#236037,#236038,#236039,#236040,#236041,#236042,#236043,#236044,#236045,
#236046,#236047,#236048,#236049,#236050,#236051,#236052,#236053,#236054,
#236055,#236056,#236057,#236058,#236059,#236060,#236061,#236062,#236063,
#236064,#236065,#236066,#236067,#236068,#236069,#236070,#236071,#236072,
#236073,#236074,#236075,#236076,#236077,#236078,#236079,#236080,#236081,
#236082,#236083,#236084,#236085,#236086,#236087,#236088,#236089,#236090,
#236091,#236092,#236093,#236094,#236095,#236096,#236097,#236098,#236099,
#236100,#236101,#236102,#236103,#236104,#236105,#236106,#236107,#236108,
#236109,#236110,#236111,#236112,#236113,#236114,#236115,#236116,#236117,
#236118,#236119,#236120,#236121,#236122,#236123,#236124,#236125,#236126,
#236127,#236128,#236129,#236130,#236131,#236132,#236133,#236134,#236135,
#236136,#236137,#236138),.UNSPECIFIED.,.F.,.F.,(4,3,3,3,3,3,3,3,3,3,3,3,
3,3,3,3,3,3,3,3,3,3,3,3,3,3,3,3,3,3,3,3,3,3,3,3,3,3,3,3,3,3,3,3,3,3,3,3,
3,3,3,3,3,3,3,3,3,3,3,3,3,3,3,3,3,3,3,3,3,3,3,3,3,3,3,3,3,3,3,3,3,3,3,3,
3,3,3,3,3,3,3,3,3,3,3,3,3,3,3,3,3,3,3,3,3,3,3,4),(-1.,-0.99266055,-0.987155963,
-0.981651376,-0.972477064,-0.966972477,-0.96146789,-0.955963303,-0.950458716,
-0.944954128,-0.937614679,-0.932110092,-0.926605505,-0.921100917,-0.91559633,
-0.910091743,-0.904587156,-0.899082569,-0.893577982,-0.888073394,-0.882568807,
-0.87706422,-0.871559633,-0.866055046,-0.860550459,-0.855045872,-0.849541284,
-0.842201835,-0.836697248,-0.831192661,-0.825688073,-0.820183486,-0.814678899,
-0.809174312,-0.801834862,-0.794495413,-0.787155963,-0.779816514,-0.772477064,
-0.765137615,-0.757798165,-0.748623853,-0.741284404,-0.733944954,-0.726605505,
-0.719266055,-0.708256881,-0.700917431,-0.693577982,-0.686238532,-0.678899083,
-0.671559633,-0.664220183,-0.656880734,-0.649541284,-0.642201835,-0.634862385,
-0.627522936,-0.620183486,-0.612844037,-0.605504587,-0.598165138,-0.590825688,
-0.583486239,-0.576146789,-0.568807339,-0.56146789,-0.55412844,-0.546788991,
-0.539449541,-0.532110092,-0.52293578,-0.513761468,-0.504587156,-0.495412844,
-0.486238532,-0.475229358,-0.466055046,-0.453211009,-0.444036697,-0.434862385,
-0.425688073,-0.416513761,-0.40733945,-0.398165138,-0.388990826,-0.377981651,
-0.366972477,-0.355963303,-0.344954128,-0.333944954,-0.32293578,-0.311926606,
-0.300917431,-0.289908257,-0.278899083,-0.267889908,-0.255045872,-0.244036697,
-0.233027523,-0.222018349,-0.211009174,-0.2,-0.188990826,-0.177981651,-0.166972477,
-0.155963303,-0.143172102),.UNSPECIFIED.);
#24418=B_SPLINE_CURVE_WITH_KNOTS('',3,(#236139,#236140,#236141,#236142,
#236143,#236144,#236145,#236146,#236147,#236148,#236149,#236150,#236151,
#236152,#236153,#236154,#236155,#236156,#236157,#236158,#236159,#236160,
#236161,#236162,#236163,#236164,#236165,#236166,#236167,#236168,#236169,
#236170,#236171,#236172,#236173,#236174,#236175,#236176,#236177,#236178,
#236179,#236180,#236181,#236182,#236183,#236184,#236185,#236186,#236187,
#236188,#236189,#236190,#236191,#236192,#236193,#236194,#236195,#236196,
#236197,#236198,#236199,#236200,#236201,#236202,#236203,#236204,#236205,
#236206,#236207,#236208,#236209,#236210,#236211,#236212,#236213,#236214,
#236215,#236216,#236217,#236218,#236219,#236220,#236221,#236222,#236223,
#236224,#236225,#236226,#236227,#236228,#236229,#236230,#236231,#236232,
#236233,#236234,#236235,#236236,#236237,#236238,#236239,#236240,#236241,
#236242,#236243,#236244,#236245,#236246,#236247,#236248,#236249,#236250,
#236251,#236252,#236253,#236254,#236255,#236256,#236257,#236258,#236259,
#236260,#236261,#236262,#236263,#236264,#236265,#236266,#236267,#236268,
#236269,#236270,#236271,#236272,#236273,#236274,#236275,#236276,#236277,
#236278,#236279,#236280,#236281,#236282,#236283,#236284,#236285,#236286,
#236287,#236288,#236289,#236290,#236291,#236292,#236293,#236294,#236295,
#236296,#236297,#236298,#236299,#236300,#236301,#236302,#236303,#236304,
#236305,#236306,#236307,#236308,#236309,#236310,#236311,#236312,#236313,
#236314,#236315,#236316,#236317,#236318,#236319,#236320,#236321,#236322,
#236323,#236324,#236325,#236326,#236327,#236328,#236329,#236330,#236331,
#236332,#236333,#236334,#236335,#236336,#236337,#236338,#236339,#236340,
#236341,#236342,#236343,#236344,#236345,#236346,#236347,#236348,#236349,
#236350,#236351,#236352,#236353,#236354,#236355,#236356,#236357,#236358,
#236359,#236360,#236361,#236362,#236363,#236364,#236365,#236366,#236367,
#236368,#236369,#236370,#236371,#236372,#236373,#236374,#236375,#236376,
#236377,#236378,#236379,#236380,#236381,#236382,#236383,#236384,#236385,
#236386,#236387,#236388,#236389,#236390,#236391,#236392,#236393,#236394,
#236395,#236396,#236397,#236398,#236399,#236400,#236401,#236402,#236403,
#236404,#236405,#236406,#236407,#236408,#236409,#236410,#236411,#236412,
#236413,#236414,#236415,#236416,#236417,#236418,#236419,#236420,#236421,
#236422,#236423,#236424,#236425,#236426,#236427,#236428,#236429,#236430),
 .UNSPECIFIED.,.F.,.F.,(4,3,3,3,3,3,3,3,3,3,3,3,3,3,3,3,3,3,3,3,3,3,3,3,
3,3,3,3,3,3,3,3,3,3,3,3,3,3,3,3,3,3,3,3,3,3,3,3,3,3,3,3,3,3,3,3,3,3,3,3,
3,3,3,3,3,3,3,3,3,3,3,3,3,3,3,3,3,3,3,3,3,3,3,3,3,3,3,3,3,3,3,3,3,3,3,3,
3,4),(0.143172102,0.15412844,0.165137615,0.176146789,0.187155963,0.198165138,
0.209174312,0.220183486,0.231192661,0.242201835,0.255045872,0.267889908,
0.278899083,0.291743119,0.306422018,0.317431193,0.330275229,0.343119266,
0.35412844,0.365137615,0.376146789,0.387155963,0.396330275,0.40733945,0.416513761,
0.425688073,0.43853211,0.449541284,0.458715596,0.469724771,0.482568807,
0.491743119,0.506422018,0.517431193,0.530275229,0.537614679,0.544954128,
0.55412844,0.56146789,0.568807339,0.576146789,0.585321101,0.59266055,0.6,
0.60733945,0.614678899,0.622018349,0.634862385,0.642201835,0.649541284,
0.656880734,0.666055046,0.673394495,0.682568807,0.689908257,0.700917431,
0.708256881,0.717431193,0.726605505,0.733944954,0.741284404,0.748623853,
0.755963303,0.763302752,0.770642202,0.777981651,0.787155963,0.798165138,
0.805504587,0.812844037,0.823853211,0.829357798,0.834862385,0.842201835,
0.849541284,0.855045872,0.860550459,0.867889908,0.873394495,0.878899083,
0.88440367,0.889908257,0.897247706,0.904587156,0.910091743,0.917431193,
0.92293578,0.928440367,0.937614679,0.944954128,0.95412844,0.963302752,0.968807339,
0.977981651,0.983486239,0.988990826,0.994495413,1.),.UNSPECIFIED.);
#24419=B_SPLINE_CURVE_WITH_KNOTS('',3,(#237393,#237394,#237395,#237396,
#237397,#237398,#237399,#237400,#237401,#237402,#237403,#237404,#237405,
#237406,#237407,#237408,#237409,#237410,#237411,#237412,#237413,#237414,
#237415,#237416,#237417,#237418,#237419,#237420,#237421,#237422,#237423,
#237424,#237425,#237426,#237427,#237428,#237429,#237430,#237431,#237432,
#237433,#237434,#237435,#237436,#237437,#237438,#237439,#237440,#237441,
#237442,#237443,#237444,#237445,#237446,#237447,#237448,#237449,#237450,
#237451,#237452,#237453,#237454,#237455,#237456,#237457,#237458,#237459,
#237460,#237461,#237462,#237463,#237464,#237465,#237466,#237467,#237468,
#237469,#237470,#237471,#237472,#237473,#237474,#237475,#237476,#237477,
#237478,#237479,#237480,#237481,#237482,#237483,#237484,#237485,#237486,
#237487,#237488,#237489,#237490,#237491,#237492,#237493,#237494,#237495,
#237496,#237497,#237498,#237499,#237500,#237501,#237502,#237503,#237504,
#237505,#237506,#237507,#237508,#237509,#237510,#237511,#237512,#237513,
#237514,#237515,#237516,#237517,#237518,#237519,#237520,#237521,#237522,
#237523,#237524,#237525,#237526,#237527,#237528,#237529,#237530,#237531,
#237532,#237533,#237534,#237535,#237536,#237537,#237538,#237539,#237540,
#237541,#237542,#237543,#237544,#237545,#237546,#237547,#237548,#237549,
#237550,#237551,#237552,#237553,#237554,#237555,#237556,#237557,#237558,
#237559,#237560,#237561,#237562,#237563,#237564,#237565,#237566,#237567,
#237568,#237569,#237570,#237571,#237572,#237573,#237574,#237575,#237576,
#237577,#237578,#237579,#237580,#237581,#237582,#237583,#237584,#237585,
#237586,#237587,#237588,#237589,#237590,#237591,#237592,#237593,#237594,
#237595,#237596,#237597,#237598,#237599,#237600,#237601,#237602,#237603,
#237604,#237605,#237606,#237607,#237608,#237609,#237610,#237611,#237612,
#237613,#237614,#237615,#237616,#237617,#237618,#237619,#237620,#237621,
#237622,#237623,#237624,#237625,#237626,#237627,#237628,#237629,#237630,
#237631,#237632,#237633,#237634,#237635,#237636,#237637,#237638,#237639,
#237640,#237641,#237642,#237643,#237644,#237645,#237646,#237647,#237648,
#237649,#237650,#237651,#237652,#237653,#237654,#237655,#237656,#237657,
#237658,#237659,#237660,#237661,#237662,#237663,#237664,#237665,#237666,
#237667,#237668,#237669,#237670,#237671,#237672,#237673,#237674,#237675,
#237676,#237677,#237678,#237679,#237680,#237681,#237682,#237683,#237684,
#237685,#237686,#237687,#237688,#237689,#237690,#237691,#237692,#237693,
#237694,#237695,#237696,#237697,#237698,#237699,#237700,#237701,#237702,
#237703,#237704,#237705,#237706,#237707,#237708,#237709,#237710,#237711),
 .UNSPECIFIED.,.F.,.F.,(4,3,3,3,3,3,3,3,3,3,3,3,3,3,3,3,3,3,3,3,3,3,3,3,
3,3,3,3,3,3,3,3,3,3,3,3,3,3,3,3,3,3,3,3,3,3,3,3,3,3,3,3,3,3,3,3,3,3,3,3,
3,3,3,3,3,3,3,3,3,3,3,3,3,3,3,3,3,3,3,3,3,3,3,3,3,3,3,3,3,3,3,3,3,3,3,3,
3,3,3,3,3,3,3,3,3,3,4),(-1.,-0.994495413,-0.988990826,-0.983486239,-0.977981651,
-0.970642202,-0.965137615,-0.959633028,-0.95412844,-0.948623853,-0.943119266,
-0.935779817,-0.928440367,-0.92293578,-0.917431193,-0.911926606,-0.906422018,
-0.900917431,-0.895412844,-0.889908257,-0.88440367,-0.878899083,-0.873394495,
-0.867889908,-0.860550459,-0.855045872,-0.849541284,-0.844036697,-0.83853211,
-0.833027523,-0.827522936,-0.822018349,-0.814678899,-0.80733945,-0.8,-0.79266055,
-0.783486239,-0.776146789,-0.768807339,-0.76146789,-0.75412844,-0.746788991,
-0.739449541,-0.732110092,-0.724770642,-0.717431193,-0.708256881,-0.700917431,
-0.693577982,-0.686238532,-0.678899083,-0.671559633,-0.664220183,-0.656880734,
-0.649541284,-0.642201835,-0.634862385,-0.627522936,-0.620183486,-0.612844037,
-0.605504587,-0.598165138,-0.590825688,-0.583486239,-0.576146789,-0.568807339,
-0.559633028,-0.552293578,-0.543119266,-0.535779817,-0.528440367,-0.519266055,
-0.508256881,-0.499082569,-0.489908257,-0.480733945,-0.471559633,-0.462385321,
-0.453211009,-0.442201835,-0.433027523,-0.423853211,-0.414678899,-0.405504587,
-0.394495413,-0.381651376,-0.370642202,-0.359633028,-0.348623853,-0.337614679,
-0.324770642,-0.311926606,-0.300917431,-0.289908257,-0.278899083,-0.267889908,
-0.255045872,-0.244036697,-0.233027523,-0.222018349,-0.211009174,-0.2,-0.188990826,
-0.177981651,-0.165137615,-0.15412844,-0.143172102),.UNSPECIFIED.);
#24420=B_SPLINE_CURVE_WITH_KNOTS('',3,(#237712,#237713,#237714,#237715,
#237716,#237717,#237718,#237719,#237720,#237721,#237722,#237723,#237724,
#237725,#237726,#237727,#237728,#237729,#237730,#237731,#237732,#237733,
#237734,#237735,#237736,#237737,#237738,#237739,#237740,#237741,#237742,
#237743,#237744,#237745,#237746,#237747,#237748,#237749,#237750,#237751,
#237752,#237753,#237754,#237755,#237756,#237757,#237758,#237759,#237760,
#237761,#237762,#237763,#237764,#237765,#237766,#237767,#237768,#237769,
#237770,#237771,#237772,#237773,#237774,#237775,#237776,#237777,#237778,
#237779,#237780,#237781,#237782,#237783,#237784,#237785,#237786,#237787,
#237788,#237789,#237790,#237791,#237792,#237793,#237794,#237795,#237796,
#237797,#237798,#237799,#237800,#237801,#237802,#237803,#237804,#237805,
#237806,#237807,#237808,#237809,#237810,#237811,#237812,#237813,#237814,
#237815,#237816,#237817,#237818,#237819,#237820,#237821,#237822,#237823,
#237824,#237825,#237826,#237827,#237828,#237829,#237830,#237831,#237832,
#237833,#237834,#237835,#237836,#237837,#237838,#237839,#237840,#237841,
#237842,#237843,#237844,#237845,#237846,#237847,#237848,#237849,#237850,
#237851,#237852,#237853,#237854,#237855,#237856,#237857,#237858,#237859,
#237860,#237861,#237862,#237863,#237864,#237865,#237866,#237867,#237868,
#237869,#237870,#237871,#237872,#237873,#237874,#237875,#237876,#237877,
#237878,#237879,#237880,#237881,#237882,#237883,#237884,#237885,#237886,
#237887,#237888,#237889,#237890,#237891,#237892,#237893,#237894,#237895,
#237896,#237897,#237898,#237899,#237900,#237901,#237902,#237903,#237904,
#237905,#237906,#237907,#237908,#237909,#237910,#237911,#237912,#237913,
#237914,#237915,#237916,#237917,#237918,#237919,#237920,#237921,#237922,
#237923,#237924,#237925,#237926,#237927,#237928,#237929,#237930,#237931,
#237932,#237933,#237934,#237935,#237936,#237937,#237938,#237939,#237940,
#237941,#237942,#237943,#237944,#237945,#237946,#237947,#237948,#237949,
#237950,#237951,#237952,#237953,#237954,#237955,#237956,#237957,#237958,
#237959,#237960,#237961,#237962,#237963,#237964,#237965,#237966,#237967,
#237968,#237969,#237970,#237971,#237972,#237973,#237974,#237975,#237976,
#237977,#237978,#237979,#237980,#237981,#237982,#237983,#237984,#237985,
#237986,#237987,#237988,#237989,#237990,#237991,#237992,#237993,#237994,
#237995,#237996,#237997,#237998,#237999,#238000,#238001,#238002,#238003,
#238004,#238005,#238006,#238007,#238008,#238009,#238010,#238011,#238012,
#238013,#238014,#238015,#238016,#238017,#238018,#238019,#238020,#238021),
 .UNSPECIFIED.,.F.,.F.,(4,3,3,3,3,3,3,3,3,3,3,3,3,3,3,3,3,3,3,3,3,3,3,3,
3,3,3,3,3,3,3,3,3,3,3,3,3,3,3,3,3,3,3,3,3,3,3,3,3,3,3,3,3,3,3,3,3,3,3,3,
3,3,3,3,3,3,3,3,3,3,3,3,3,3,3,3,3,3,3,3,3,3,3,3,3,3,3,3,3,3,3,3,3,3,3,3,
3,3,3,3,3,3,3,4),(0.143172102,0.15412844,0.165137615,0.176146789,0.187155963,
0.198165138,0.209174312,0.220183486,0.231192661,0.242201835,0.253211009,
0.264220183,0.275229358,0.286238532,0.297247706,0.308256881,0.32293578,
0.333944954,0.344954128,0.355963303,0.368807339,0.379816514,0.390825688,
0.4,0.409174312,0.418348624,0.427522936,0.436697248,0.44587156,0.455045872,
0.464220183,0.473394495,0.48440367,0.495412844,0.504587156,0.513761468,
0.52293578,0.532110092,0.539449541,0.550458716,0.559633028,0.566972477,
0.574311927,0.581651376,0.588990826,0.596330275,0.603669725,0.611009174,
0.618348624,0.625688073,0.633027523,0.640366972,0.647706422,0.656880734,
0.664220183,0.673394495,0.682568807,0.689908257,0.697247706,0.706422018,
0.71559633,0.72293578,0.730275229,0.737614679,0.744954128,0.75412844,0.76146789,
0.768807339,0.776146789,0.783486239,0.79266055,0.8,0.80733945,0.812844037,
0.818348624,0.823853211,0.829357798,0.836697248,0.84587156,0.851376147,
0.856880734,0.864220183,0.871559633,0.87706422,0.882568807,0.888073394,
0.893577982,0.900917431,0.906422018,0.913761468,0.919266055,0.924770642,
0.930275229,0.935779817,0.941284404,0.950458716,0.955963303,0.96146789,
0.968807339,0.974311927,0.979816514,0.985321101,0.99266055,1.),
 .UNSPECIFIED.);
#24421=B_SPLINE_CURVE_WITH_KNOTS('',3,(#238966,#238967,#238968,#238969,
#238970,#238971,#238972,#238973,#238974,#238975,#238976,#238977,#238978,
#238979,#238980,#238981,#238982,#238983,#238984,#238985,#238986,#238987,
#238988,#238989,#238990,#238991,#238992,#238993,#238994,#238995,#238996,
#238997,#238998,#238999,#239000,#239001,#239002,#239003,#239004,#239005,
#239006,#239007,#239008,#239009,#239010,#239011,#239012,#239013,#239014,
#239015,#239016,#239017,#239018,#239019,#239020,#239021,#239022,#239023,
#239024,#239025,#239026,#239027,#239028,#239029,#239030,#239031,#239032,
#239033,#239034,#239035,#239036,#239037,#239038,#239039,#239040,#239041,
#239042,#239043,#239044,#239045,#239046,#239047,#239048,#239049,#239050,
#239051,#239052,#239053,#239054,#239055,#239056,#239057,#239058,#239059,
#239060,#239061,#239062,#239063,#239064,#239065,#239066,#239067,#239068,
#239069,#239070,#239071,#239072,#239073,#239074,#239075,#239076,#239077,
#239078,#239079,#239080,#239081,#239082,#239083,#239084,#239085,#239086,
#239087,#239088,#239089,#239090,#239091,#239092,#239093,#239094,#239095,
#239096,#239097,#239098,#239099,#239100,#239101,#239102,#239103,#239104,
#239105,#239106,#239107,#239108,#239109,#239110,#239111,#239112,#239113,
#239114,#239115,#239116,#239117,#239118,#239119,#239120,#239121,#239122,
#239123,#239124,#239125,#239126,#239127,#239128,#239129,#239130,#239131,
#239132,#239133,#239134,#239135,#239136,#239137,#239138,#239139,#239140,
#239141,#239142,#239143,#239144,#239145,#239146,#239147,#239148,#239149,
#239150,#239151,#239152,#239153,#239154,#239155,#239156,#239157,#239158,
#239159,#239160,#239161,#239162,#239163,#239164,#239165,#239166,#239167,
#239168,#239169,#239170,#239171,#239172,#239173,#239174,#239175,#239176,
#239177,#239178,#239179,#239180,#239181,#239182,#239183,#239184,#239185,
#239186,#239187,#239188,#239189,#239190,#239191,#239192,#239193,#239194,
#239195,#239196,#239197,#239198,#239199,#239200,#239201,#239202,#239203,
#239204,#239205,#239206,#239207,#239208,#239209,#239210,#239211,#239212,
#239213,#239214,#239215,#239216,#239217,#239218,#239219,#239220,#239221,
#239222,#239223,#239224,#239225,#239226,#239227,#239228,#239229,#239230,
#239231,#239232,#239233,#239234,#239235,#239236,#239237,#239238,#239239,
#239240,#239241,#239242,#239243,#239244,#239245,#239246,#239247,#239248,
#239249,#239250,#239251,#239252,#239253,#239254,#239255,#239256,#239257,
#239258,#239259,#239260,#239261,#239262,#239263,#239264,#239265,#239266,
#239267,#239268,#239269,#239270,#239271,#239272,#239273,#239274,#239275),
 .UNSPECIFIED.,.F.,.F.,(4,3,3,3,3,3,3,3,3,3,3,3,3,3,3,3,3,3,3,3,3,3,3,3,
3,3,3,3,3,3,3,3,3,3,3,3,3,3,3,3,3,3,3,3,3,3,3,3,3,3,3,3,3,3,3,3,3,3,3,3,
3,3,3,3,3,3,3,3,3,3,3,3,3,3,3,3,3,3,3,3,3,3,3,3,3,3,3,3,3,3,3,3,3,3,3,3,
3,3,3,3,3,3,3,4),(0.143172102,0.15412844,0.165137615,0.176146789,0.187155963,
0.198165138,0.209174312,0.220183486,0.231192661,0.242201835,0.253211009,
0.264220183,0.275229358,0.286238532,0.297247706,0.308256881,0.319266055,
0.330275229,0.343119266,0.35412844,0.365137615,0.376146789,0.387155963,
0.396330275,0.405504587,0.414678899,0.427522936,0.436697248,0.44587156,
0.456880734,0.466055046,0.47706422,0.486238532,0.495412844,0.504587156,
0.513761468,0.52293578,0.532110092,0.539449541,0.546788991,0.55412844,0.56146789,
0.570642202,0.577981651,0.585321101,0.59266055,0.6,0.60733945,0.616513761,
0.625688073,0.633027523,0.640366972,0.647706422,0.655045872,0.664220183,
0.671559633,0.680733945,0.688073394,0.695412844,0.702752294,0.710091743,
0.717431193,0.724770642,0.733944954,0.741284404,0.748623853,0.755963303,
0.763302752,0.770642202,0.777981651,0.785321101,0.794495413,0.801834862,
0.811009174,0.820183486,0.827522936,0.833027523,0.840366972,0.84587156,
0.851376147,0.856880734,0.862385321,0.871559633,0.87706422,0.886238532,
0.891743119,0.897247706,0.902752294,0.911926606,0.917431193,0.92293578,
0.928440367,0.933944954,0.939449541,0.944954128,0.950458716,0.955963303,
0.96146789,0.966972477,0.972477064,0.977981651,0.983486239,0.990825688,
1.),.UNSPECIFIED.);
#24422=B_SPLINE_CURVE_WITH_KNOTS('',3,(#239276,#239277,#239278,#239279,
#239280,#239281,#239282,#239283,#239284,#239285,#239286,#239287,#239288,
#239289,#239290,#239291,#239292,#239293,#239294,#239295,#239296,#239297,
#239298,#239299,#239300,#239301,#239302,#239303,#239304,#239305,#239306,
#239307,#239308,#239309,#239310,#239311,#239312,#239313,#239314,#239315,
#239316,#239317,#239318,#239319,#239320,#239321,#239322,#239323,#239324,
#239325,#239326,#239327,#239328,#239329,#239330,#239331,#239332,#239333,
#239334,#239335,#239336,#239337,#239338,#239339,#239340,#239341,#239342,
#239343,#239344,#239345,#239346,#239347,#239348,#239349,#239350,#239351,
#239352,#239353,#239354,#239355,#239356,#239357,#239358,#239359,#239360,
#239361,#239362,#239363,#239364,#239365,#239366,#239367,#239368,#239369,
#239370,#239371,#239372,#239373,#239374,#239375,#239376,#239377,#239378,
#239379,#239380,#239381,#239382,#239383,#239384,#239385,#239386,#239387,
#239388,#239389,#239390,#239391,#239392,#239393,#239394,#239395,#239396,
#239397,#239398,#239399,#239400,#239401,#239402,#239403,#239404,#239405,
#239406,#239407,#239408,#239409,#239410,#239411,#239412,#239413,#239414,
#239415,#239416,#239417,#239418,#239419,#239420,#239421,#239422,#239423,
#239424,#239425,#239426,#239427,#239428,#239429,#239430,#239431,#239432,
#239433,#239434,#239435,#239436,#239437,#239438,#239439,#239440,#239441,
#239442,#239443,#239444,#239445,#239446,#239447,#239448,#239449,#239450,
#239451,#239452,#239453,#239454,#239455,#239456,#239457,#239458,#239459,
#239460,#239461,#239462,#239463,#239464,#239465,#239466,#239467,#239468,
#239469,#239470,#239471,#239472,#239473,#239474,#239475,#239476,#239477,
#239478,#239479,#239480,#239481,#239482,#239483,#239484,#239485,#239486,
#239487,#239488,#239489,#239490,#239491,#239492,#239493,#239494,#239495,
#239496,#239497,#239498,#239499,#239500,#239501,#239502,#239503,#239504,
#239505,#239506,#239507,#239508,#239509,#239510,#239511,#239512,#239513,
#239514,#239515,#239516,#239517,#239518,#239519,#239520,#239521,#239522,
#239523,#239524,#239525,#239526,#239527,#239528,#239529,#239530,#239531,
#239532,#239533,#239534,#239535,#239536,#239537,#239538,#239539,#239540,
#239541,#239542,#239543,#239544,#239545,#239546,#239547,#239548,#239549,
#239550,#239551,#239552,#239553,#239554,#239555,#239556,#239557,#239558,
#239559,#239560,#239561,#239562,#239563,#239564,#239565,#239566,#239567,
#239568,#239569,#239570,#239571,#239572,#239573,#239574,#239575,#239576,
#239577,#239578,#239579,#239580,#239581,#239582,#239583,#239584,#239585,
#239586,#239587,#239588,#239589,#239590,#239591,#239592,#239593,#239594,
#239595,#239596,#239597,#239598,#239599,#239600),.UNSPECIFIED.,.F.,.F.,
(4,3,3,3,3,3,3,3,3,3,3,3,3,3,3,3,3,3,3,3,3,3,3,3,3,3,3,3,3,3,3,3,3,3,3,
3,3,3,3,3,3,3,3,3,3,3,3,3,3,3,3,3,3,3,3,3,3,3,3,3,3,3,3,3,3,3,3,3,3,3,3,
3,3,3,3,3,3,3,3,3,3,3,3,3,3,3,3,3,3,3,3,3,3,3,3,3,3,3,3,3,3,3,3,3,3,3,3,
3,4),(0.143172102,0.15412844,0.165137615,0.176146789,0.187155963,0.198165138,
0.209174312,0.220183486,0.231192661,0.244036697,0.255045872,0.266055046,
0.27706422,0.288073394,0.299082569,0.310091743,0.321100917,0.332110092,
0.343119266,0.35412844,0.365137615,0.376146789,0.387155963,0.396330275,
0.405504587,0.414678899,0.423853211,0.433027523,0.444036697,0.453211009,
0.462385321,0.475229358,0.48440367,0.493577982,0.502752294,0.511926606,
0.521100917,0.530275229,0.537614679,0.544954128,0.552293578,0.559633028,
0.566972477,0.574311927,0.581651376,0.588990826,0.596330275,0.603669725,
0.611009174,0.618348624,0.625688073,0.633027523,0.640366972,0.647706422,
0.655045872,0.664220183,0.671559633,0.678899083,0.686238532,0.693577982,
0.700917431,0.708256881,0.71559633,0.72293578,0.730275229,0.739449541,0.746788991,
0.75412844,0.76146789,0.768807339,0.776146789,0.783486239,0.790825688,0.798165138,
0.805504587,0.811009174,0.816513761,0.823853211,0.829357798,0.834862385,
0.840366972,0.84587156,0.851376147,0.856880734,0.862385321,0.867889908,
0.873394495,0.878899083,0.886238532,0.891743119,0.897247706,0.902752294,
0.908256881,0.913761468,0.921100917,0.926605505,0.932110092,0.937614679,
0.943119266,0.948623853,0.95412844,0.959633028,0.965137615,0.970642202,
0.976146789,0.981651376,0.987155963,0.994495413,1.),.UNSPECIFIED.);
#24423=B_SPLINE_CURVE_WITH_KNOTS('',3,(#240560,#240561,#240562,#240563,
#240564,#240565,#240566,#240567,#240568,#240569,#240570,#240571,#240572,
#240573,#240574,#240575,#240576,#240577,#240578,#240579,#240580,#240581,
#240582,#240583,#240584,#240585,#240586,#240587,#240588,#240589,#240590,
#240591,#240592,#240593,#240594,#240595,#240596,#240597,#240598,#240599,
#240600,#240601,#240602,#240603,#240604,#240605,#240606,#240607,#240608,
#240609,#240610,#240611,#240612,#240613,#240614,#240615,#240616,#240617,
#240618,#240619,#240620,#240621,#240622,#240623,#240624,#240625,#240626,
#240627,#240628,#240629,#240630,#240631,#240632,#240633,#240634,#240635,
#240636,#240637,#240638,#240639,#240640,#240641,#240642,#240643,#240644,
#240645,#240646,#240647,#240648,#240649,#240650,#240651,#240652,#240653,
#240654,#240655,#240656,#240657,#240658,#240659,#240660,#240661,#240662,
#240663,#240664,#240665,#240666,#240667,#240668,#240669,#240670,#240671,
#240672,#240673,#240674,#240675,#240676,#240677,#240678,#240679,#240680,
#240681,#240682,#240683,#240684,#240685,#240686,#240687,#240688,#240689,
#240690,#240691,#240692,#240693,#240694,#240695,#240696,#240697,#240698,
#240699,#240700,#240701,#240702,#240703,#240704,#240705,#240706,#240707,
#240708,#240709,#240710,#240711,#240712,#240713,#240714,#240715,#240716,
#240717,#240718,#240719,#240720,#240721,#240722,#240723,#240724,#240725,
#240726,#240727,#240728,#240729,#240730,#240731,#240732,#240733,#240734,
#240735,#240736,#240737,#240738,#240739,#240740,#240741,#240742,#240743,
#240744,#240745,#240746,#240747,#240748,#240749,#240750,#240751,#240752,
#240753,#240754,#240755,#240756,#240757,#240758,#240759,#240760,#240761,
#240762,#240763,#240764,#240765,#240766,#240767,#240768,#240769,#240770,
#240771,#240772,#240773,#240774,#240775,#240776,#240777,#240778,#240779,
#240780,#240781,#240782,#240783,#240784,#240785,#240786,#240787,#240788,
#240789,#240790,#240791,#240792,#240793,#240794,#240795,#240796,#240797,
#240798,#240799,#240800,#240801,#240802,#240803,#240804,#240805,#240806,
#240807,#240808,#240809,#240810,#240811,#240812,#240813,#240814,#240815,
#240816,#240817,#240818,#240819,#240820,#240821,#240822,#240823,#240824,
#240825,#240826,#240827,#240828,#240829,#240830,#240831,#240832,#240833,
#240834,#240835,#240836,#240837,#240838,#240839,#240840,#240841,#240842,
#240843,#240844,#240845,#240846,#240847,#240848,#240849,#240850,#240851,
#240852,#240853,#240854,#240855,#240856,#240857,#240858,#240859,#240860,
#240861,#240862,#240863,#240864,#240865,#240866,#240867,#240868,#240869),
 .UNSPECIFIED.,.F.,.F.,(4,3,3,3,3,3,3,3,3,3,3,3,3,3,3,3,3,3,3,3,3,3,3,3,
3,3,3,3,3,3,3,3,3,3,3,3,3,3,3,3,3,3,3,3,3,3,3,3,3,3,3,3,3,3,3,3,3,3,3,3,
3,3,3,3,3,3,3,3,3,3,3,3,3,3,3,3,3,3,3,3,3,3,3,3,3,3,3,3,3,3,3,3,3,3,3,3,
3,3,3,3,3,3,3,4),(0.143172102,0.15412844,0.165137615,0.176146789,0.187155963,
0.198165138,0.209174312,0.222018349,0.233027523,0.244036697,0.255045872,
0.266055046,0.27706422,0.288073394,0.299082569,0.310091743,0.321100917,
0.332110092,0.343119266,0.35412844,0.365137615,0.377981651,0.388990826,
0.398165138,0.409174312,0.418348624,0.427522936,0.436697248,0.44587156,
0.455045872,0.464220183,0.473394495,0.482568807,0.491743119,0.500917431,
0.510091743,0.519266055,0.528440367,0.535779817,0.546788991,0.55412844,
0.56146789,0.568807339,0.576146789,0.583486239,0.590825688,0.598165138,
0.605504587,0.612844037,0.620183486,0.627522936,0.634862385,0.642201835,
0.649541284,0.656880734,0.664220183,0.671559633,0.680733945,0.688073394,
0.699082569,0.710091743,0.717431193,0.724770642,0.732110092,0.739449541,
0.748623853,0.755963303,0.763302752,0.774311927,0.781651376,0.79266055,
0.8,0.80733945,0.812844037,0.818348624,0.825688073,0.831192661,0.836697248,
0.844036697,0.849541284,0.856880734,0.862385321,0.869724771,0.87706422,
0.88440367,0.889908257,0.895412844,0.900917431,0.910091743,0.91559633,0.921100917,
0.926605505,0.932110092,0.937614679,0.944954128,0.950458716,0.957798165,
0.963302752,0.968807339,0.974311927,0.979816514,0.985321101,0.990825688,
1.),.UNSPECIFIED.);
#24424=B_SPLINE_CURVE_WITH_KNOTS('',3,(#240870,#240871,#240872,#240873,
#240874,#240875,#240876,#240877,#240878,#240879,#240880,#240881,#240882,
#240883,#240884,#240885,#240886,#240887,#240888,#240889,#240890,#240891,
#240892,#240893,#240894,#240895,#240896,#240897,#240898,#240899,#240900,
#240901,#240902,#240903,#240904,#240905,#240906,#240907,#240908,#240909,
#240910,#240911,#240912,#240913,#240914,#240915,#240916,#240917,#240918,
#240919,#240920,#240921,#240922,#240923,#240924,#240925,#240926,#240927,
#240928,#240929,#240930,#240931,#240932,#240933,#240934,#240935,#240936,
#240937,#240938,#240939,#240940,#240941,#240942,#240943,#240944,#240945,
#240946,#240947,#240948,#240949,#240950,#240951,#240952,#240953,#240954,
#240955,#240956,#240957,#240958,#240959,#240960,#240961,#240962,#240963,
#240964,#240965,#240966,#240967,#240968,#240969,#240970,#240971,#240972,
#240973,#240974,#240975,#240976,#240977,#240978,#240979,#240980,#240981,
#240982,#240983,#240984,#240985,#240986,#240987,#240988,#240989,#240990,
#240991,#240992,#240993,#240994,#240995,#240996,#240997,#240998,#240999,
#241000,#241001,#241002,#241003,#241004,#241005,#241006,#241007,#241008,
#241009,#241010,#241011,#241012,#241013,#241014,#241015,#241016,#241017,
#241018,#241019,#241020,#241021,#241022,#241023,#241024,#241025,#241026,
#241027,#241028,#241029,#241030,#241031,#241032,#241033,#241034,#241035,
#241036,#241037,#241038,#241039,#241040,#241041,#241042,#241043,#241044,
#241045,#241046,#241047,#241048,#241049,#241050,#241051,#241052,#241053,
#241054,#241055,#241056,#241057,#241058,#241059,#241060,#241061,#241062,
#241063,#241064,#241065,#241066,#241067,#241068,#241069,#241070,#241071,
#241072,#241073,#241074,#241075,#241076,#241077,#241078,#241079,#241080,
#241081,#241082,#241083,#241084,#241085,#241086,#241087,#241088,#241089,
#241090,#241091,#241092,#241093,#241094,#241095,#241096,#241097,#241098,
#241099,#241100,#241101,#241102,#241103,#241104,#241105,#241106,#241107,
#241108,#241109,#241110,#241111,#241112,#241113,#241114,#241115,#241116,
#241117,#241118,#241119,#241120,#241121,#241122,#241123,#241124,#241125,
#241126,#241127,#241128,#241129,#241130,#241131,#241132,#241133,#241134,
#241135,#241136,#241137,#241138,#241139,#241140,#241141,#241142,#241143,
#241144,#241145,#241146,#241147,#241148,#241149,#241150,#241151,#241152,
#241153,#241154,#241155,#241156,#241157,#241158,#241159,#241160,#241161,
#241162,#241163,#241164,#241165,#241166,#241167,#241168,#241169,#241170,
#241171,#241172,#241173,#241174,#241175,#241176,#241177,#241178,#241179,
#241180,#241181,#241182,#241183,#241184,#241185,#241186,#241187,#241188,
#241189,#241190,#241191),.UNSPECIFIED.,.F.,.F.,(4,3,3,3,3,3,3,3,3,3,3,3,
3,3,3,3,3,3,3,3,3,3,3,3,3,3,3,3,3,3,3,3,3,3,3,3,3,3,3,3,3,3,3,3,3,3,3,3,
3,3,3,3,3,3,3,3,3,3,3,3,3,3,3,3,3,3,3,3,3,3,3,3,3,3,3,3,3,3,3,3,3,3,3,3,
3,3,3,3,3,3,3,3,3,3,3,3,3,3,3,3,3,3,3,3,3,3,3,4),(0.143172102,0.15412844,
0.165137615,0.176146789,0.187155963,0.198165138,0.209174312,0.220183486,
0.231192661,0.242201835,0.253211009,0.264220183,0.275229358,0.286238532,
0.297247706,0.308256881,0.319266055,0.330275229,0.341284404,0.352293578,
0.363302752,0.374311927,0.385321101,0.396330275,0.405504587,0.414678899,
0.423853211,0.433027523,0.442201835,0.451376147,0.460550459,0.469724771,
0.478899083,0.488073394,0.497247706,0.506422018,0.51559633,0.524770642,
0.533944954,0.541284404,0.548623853,0.557798165,0.565137615,0.572477064,
0.579816514,0.587155963,0.596330275,0.603669725,0.611009174,0.618348624,
0.625688073,0.633027523,0.640366972,0.647706422,0.655045872,0.662385321,
0.671559633,0.678899083,0.686238532,0.693577982,0.700917431,0.710091743,
0.717431193,0.724770642,0.732110092,0.739449541,0.748623853,0.755963303,
0.763302752,0.772477064,0.779816514,0.787155963,0.794495413,0.801834862,
0.809174312,0.814678899,0.820183486,0.825688073,0.831192661,0.836697248,
0.842201835,0.847706422,0.853211009,0.858715596,0.864220183,0.869724771,
0.875229358,0.880733945,0.888073394,0.893577982,0.899082569,0.904587156,
0.910091743,0.91559633,0.921100917,0.926605505,0.932110092,0.937614679,
0.943119266,0.948623853,0.95412844,0.96146789,0.966972477,0.972477064,0.977981651,
0.983486239,0.990825688,1.),.UNSPECIFIED.);
#24425=B_SPLINE_CURVE_WITH_KNOTS('',3,(#242139,#242140,#242141,#242142,
#242143,#242144,#242145,#242146,#242147,#242148,#242149,#242150,#242151,
#242152,#242153,#242154,#242155,#242156,#242157,#242158,#242159,#242160,
#242161,#242162,#242163,#242164,#242165,#242166,#242167,#242168,#242169,
#242170,#242171,#242172,#242173,#242174,#242175,#242176,#242177,#242178,
#242179,#242180,#242181,#242182,#242183,#242184,#242185,#242186,#242187,
#242188,#242189,#242190,#242191,#242192,#242193,#242194,#242195,#242196,
#242197,#242198,#242199,#242200,#242201,#242202,#242203,#242204,#242205,
#242206,#242207,#242208,#242209,#242210,#242211,#242212,#242213,#242214,
#242215,#242216,#242217,#242218,#242219,#242220,#242221,#242222,#242223,
#242224,#242225,#242226,#242227,#242228,#242229,#242230,#242231,#242232,
#242233,#242234,#242235,#242236,#242237,#242238,#242239,#242240,#242241,
#242242,#242243,#242244,#242245,#242246,#242247,#242248,#242249,#242250,
#242251,#242252,#242253,#242254,#242255,#242256,#242257,#242258,#242259,
#242260,#242261,#242262,#242263,#242264,#242265,#242266,#242267,#242268,
#242269,#242270,#242271,#242272,#242273,#242274,#242275,#242276,#242277,
#242278,#242279,#242280,#242281,#242282,#242283,#242284,#242285,#242286,
#242287,#242288,#242289,#242290,#242291,#242292,#242293,#242294,#242295,
#242296,#242297,#242298,#242299,#242300,#242301,#242302,#242303,#242304,
#242305,#242306,#242307,#242308,#242309,#242310,#242311,#242312,#242313,
#242314,#242315,#242316,#242317,#242318,#242319,#242320,#242321,#242322,
#242323,#242324,#242325,#242326,#242327,#242328,#242329,#242330,#242331,
#242332,#242333,#242334,#242335,#242336,#242337,#242338,#242339,#242340,
#242341,#242342,#242343,#242344,#242345,#242346,#242347,#242348,#242349,
#242350,#242351,#242352,#242353,#242354,#242355,#242356,#242357,#242358,
#242359,#242360,#242361,#242362,#242363,#242364,#242365,#242366,#242367,
#242368,#242369,#242370,#242371,#242372,#242373,#242374,#242375,#242376,
#242377,#242378,#242379,#242380,#242381,#242382,#242383,#242384,#242385,
#242386,#242387,#242388,#242389,#242390,#242391,#242392,#242393,#242394,
#242395,#242396,#242397,#242398,#242399,#242400,#242401,#242402,#242403,
#242404,#242405,#242406,#242407,#242408,#242409,#242410,#242411,#242412,
#242413,#242414,#242415,#242416,#242417,#242418,#242419,#242420,#242421,
#242422,#242423,#242424,#242425,#242426,#242427,#242428,#242429,#242430,
#242431,#242432,#242433,#242434,#242435,#242436,#242437,#242438,#242439,
#242440,#242441,#242442,#242443,#242444,#242445,#242446,#242447,#242448,
#242449,#242450,#242451,#242452,#242453,#242454,#242455,#242456,#242457,
#242458,#242459,#242460),.UNSPECIFIED.,.F.,.F.,(4,3,3,3,3,3,3,3,3,3,3,3,
3,3,3,3,3,3,3,3,3,3,3,3,3,3,3,3,3,3,3,3,3,3,3,3,3,3,3,3,3,3,3,3,3,3,3,3,
3,3,3,3,3,3,3,3,3,3,3,3,3,3,3,3,3,3,3,3,3,3,3,3,3,3,3,3,3,3,3,3,3,3,3,3,
3,3,3,3,3,3,3,3,3,3,3,3,3,3,3,3,3,3,3,3,3,3,3,4),(-1.,-0.994495413,-0.988990826,
-0.983486239,-0.977981651,-0.968807339,-0.959633028,-0.95412844,-0.948623853,
-0.941284404,-0.935779817,-0.930275229,-0.924770642,-0.919266055,-0.913761468,
-0.908256881,-0.902752294,-0.897247706,-0.891743119,-0.886238532,-0.880733945,
-0.875229358,-0.867889908,-0.862385321,-0.855045872,-0.849541284,-0.844036697,
-0.83853211,-0.833027523,-0.827522936,-0.822018349,-0.816513761,-0.811009174,
-0.803669725,-0.796330275,-0.788990826,-0.781651376,-0.774311927,-0.766972477,
-0.759633028,-0.752293578,-0.743119266,-0.735779817,-0.728440367,-0.721100917,
-0.713761468,-0.706422018,-0.699082569,-0.691743119,-0.68440367,-0.67706422,
-0.669724771,-0.662385321,-0.655045872,-0.647706422,-0.640366972,-0.633027523,
-0.625688073,-0.618348624,-0.611009174,-0.603669725,-0.594495413,-0.587155963,
-0.579816514,-0.572477064,-0.565137615,-0.557798165,-0.550458716,-0.543119266,
-0.535779817,-0.528440367,-0.519266055,-0.510091743,-0.500917431,-0.491743119,
-0.480733945,-0.471559633,-0.462385321,-0.453211009,-0.444036697,-0.434862385,
-0.425688073,-0.416513761,-0.40733945,-0.398165138,-0.388990826,-0.377981651,
-0.366972477,-0.355963303,-0.344954128,-0.333944954,-0.32293578,-0.310091743,
-0.299082569,-0.288073394,-0.27706422,-0.266055046,-0.255045872,-0.244036697,
-0.233027523,-0.222018349,-0.211009174,-0.198165138,-0.187155963,-0.176146789,
-0.165137615,-0.15412844,-0.143172102),.UNSPECIFIED.);
#24426=B_SPLINE_CURVE_WITH_KNOTS('',3,(#242461,#242462,#242463,#242464,
#242465,#242466,#242467,#242468,#242469,#242470,#242471,#242472,#242473,
#242474,#242475,#242476,#242477,#242478,#242479,#242480,#242481,#242482,
#242483,#242484,#242485,#242486,#242487,#242488,#242489,#242490,#242491,
#242492,#242493,#242494,#242495,#242496,#242497,#242498,#242499,#242500,
#242501,#242502,#242503,#242504,#242505,#242506,#242507,#242508,#242509,
#242510,#242511,#242512,#242513,#242514,#242515,#242516,#242517,#242518,
#242519,#242520,#242521,#242522,#242523,#242524,#242525,#242526,#242527,
#242528,#242529,#242530,#242531,#242532,#242533,#242534,#242535,#242536,
#242537,#242538,#242539,#242540,#242541,#242542,#242543,#242544,#242545,
#242546,#242547,#242548,#242549,#242550,#242551,#242552,#242553,#242554,
#242555,#242556,#242557,#242558,#242559,#242560,#242561,#242562,#242563,
#242564,#242565,#242566,#242567,#242568,#242569,#242570,#242571,#242572,
#242573,#242574,#242575,#242576,#242577,#242578,#242579,#242580,#242581,
#242582,#242583,#242584,#242585,#242586,#242587,#242588,#242589,#242590,
#242591,#242592,#242593,#242594,#242595,#242596,#242597,#242598,#242599,
#242600,#242601,#242602,#242603,#242604,#242605,#242606,#242607,#242608,
#242609,#242610,#242611,#242612,#242613,#242614,#242615,#242616,#242617,
#242618,#242619,#242620,#242621,#242622,#242623,#242624,#242625,#242626,
#242627,#242628,#242629,#242630,#242631,#242632,#242633,#242634,#242635,
#242636,#242637,#242638,#242639,#242640,#242641,#242642,#242643,#242644,
#242645,#242646,#242647,#242648,#242649,#242650,#242651,#242652,#242653,
#242654,#242655,#242656,#242657,#242658,#242659,#242660,#242661,#242662,
#242663,#242664,#242665,#242666,#242667,#242668,#242669,#242670,#242671,
#242672,#242673,#242674,#242675,#242676,#242677,#242678,#242679,#242680,
#242681,#242682,#242683,#242684,#242685,#242686,#242687,#242688,#242689,
#242690,#242691,#242692,#242693,#242694,#242695,#242696,#242697,#242698,
#242699,#242700,#242701,#242702,#242703,#242704,#242705,#242706,#242707,
#242708,#242709,#242710,#242711,#242712,#242713,#242714,#242715,#242716,
#242717,#242718,#242719,#242720,#242721,#242722,#242723,#242724,#242725,
#242726,#242727,#242728,#242729,#242730,#242731,#242732,#242733,#242734,
#242735,#242736,#242737,#242738,#242739,#242740,#242741,#242742,#242743,
#242744,#242745,#242746,#242747,#242748,#242749,#242750,#242751,#242752,
#242753,#242754,#242755,#242756,#242757,#242758,#242759,#242760,#242761,
#242762,#242763,#242764,#242765,#242766,#242767),.UNSPECIFIED.,.F.,.F.,
(4,3,3,3,3,3,3,3,3,3,3,3,3,3,3,3,3,3,3,3,3,3,3,3,3,3,3,3,3,3,3,3,3,3,3,
3,3,3,3,3,3,3,3,3,3,3,3,3,3,3,3,3,3,3,3,3,3,3,3,3,3,3,3,3,3,3,3,3,3,3,3,
3,3,3,3,3,3,3,3,3,3,3,3,3,3,3,3,3,3,3,3,3,3,3,3,3,3,3,3,3,3,3,4),(0.143172102,
0.15412844,0.165137615,0.176146789,0.187155963,0.198165138,0.209174312,
0.220183486,0.231192661,0.242201835,0.253211009,0.264220183,0.275229358,
0.286238532,0.297247706,0.308256881,0.319266055,0.330275229,0.341284404,
0.352293578,0.363302752,0.374311927,0.385321101,0.396330275,0.405504587,
0.414678899,0.425688073,0.434862385,0.444036697,0.455045872,0.464220183,
0.473394495,0.48440367,0.495412844,0.506422018,0.51559633,0.524770642,0.533944954,
0.541284404,0.548623853,0.555963303,0.563302752,0.572477064,0.579816514,
0.587155963,0.594495413,0.601834862,0.609174312,0.616513761,0.623853211,
0.631192661,0.640366972,0.647706422,0.658715596,0.669724771,0.67706422,
0.68440367,0.693577982,0.700917431,0.708256881,0.71559633,0.72293578,0.730275229,
0.737614679,0.744954128,0.752293578,0.759633028,0.766972477,0.774311927,
0.781651376,0.788990826,0.796330275,0.80733945,0.814678899,0.820183486,
0.825688073,0.831192661,0.840366972,0.84587156,0.851376147,0.858715596,
0.864220183,0.871559633,0.87706422,0.882568807,0.891743119,0.897247706,
0.902752294,0.908256881,0.91559633,0.921100917,0.928440367,0.933944954,
0.939449541,0.944954128,0.952293578,0.957798165,0.963302752,0.968807339,
0.974311927,0.981651376,0.990825688,1.),.UNSPECIFIED.);
#24427=B_SPLINE_CURVE_WITH_KNOTS('',3,(#243730,#243731,#243732,#243733,
#243734,#243735,#243736,#243737,#243738,#243739,#243740,#243741,#243742,
#243743,#243744,#243745,#243746,#243747,#243748,#243749,#243750,#243751,
#243752,#243753,#243754,#243755,#243756,#243757,#243758,#243759,#243760,
#243761,#243762,#243763,#243764,#243765,#243766,#243767,#243768,#243769,
#243770,#243771,#243772,#243773,#243774,#243775,#243776,#243777,#243778,
#243779,#243780,#243781,#243782,#243783,#243784,#243785,#243786,#243787,
#243788,#243789,#243790,#243791,#243792,#243793,#243794,#243795,#243796,
#243797,#243798,#243799,#243800,#243801,#243802,#243803,#243804,#243805,
#243806,#243807,#243808,#243809,#243810,#243811,#243812,#243813,#243814,
#243815,#243816,#243817,#243818,#243819,#243820,#243821,#243822,#243823,
#243824,#243825,#243826,#243827,#243828,#243829,#243830,#243831,#243832,
#243833,#243834,#243835,#243836,#243837,#243838,#243839,#243840,#243841,
#243842,#243843,#243844,#243845,#243846,#243847,#243848,#243849,#243850,
#243851,#243852,#243853,#243854,#243855,#243856,#243857,#243858,#243859,
#243860,#243861,#243862,#243863,#243864,#243865,#243866,#243867,#243868,
#243869,#243870,#243871,#243872,#243873,#243874,#243875,#243876,#243877,
#243878,#243879,#243880,#243881,#243882,#243883,#243884,#243885,#243886,
#243887,#243888,#243889,#243890,#243891,#243892,#243893,#243894,#243895,
#243896,#243897,#243898,#243899,#243900,#243901,#243902,#243903,#243904,
#243905,#243906,#243907,#243908,#243909,#243910,#243911,#243912,#243913,
#243914,#243915,#243916,#243917,#243918,#243919,#243920,#243921,#243922,
#243923,#243924,#243925,#243926,#243927,#243928,#243929,#243930,#243931,
#243932,#243933,#243934,#243935,#243936,#243937,#243938,#243939,#243940,
#243941,#243942,#243943,#243944,#243945,#243946,#243947,#243948,#243949,
#243950,#243951,#243952,#243953,#243954,#243955,#243956,#243957,#243958,
#243959,#243960,#243961,#243962,#243963,#243964,#243965,#243966,#243967,
#243968,#243969,#243970,#243971,#243972,#243973,#243974,#243975,#243976,
#243977,#243978,#243979,#243980,#243981,#243982,#243983,#243984,#243985,
#243986,#243987,#243988,#243989,#243990,#243991,#243992,#243993,#243994,
#243995,#243996,#243997,#243998,#243999,#244000,#244001,#244002,#244003,
#244004,#244005,#244006,#244007,#244008,#244009,#244010,#244011,#244012,
#244013,#244014,#244015,#244016,#244017,#244018,#244019,#244020,#244021,
#244022,#244023,#244024,#244025,#244026,#244027,#244028,#244029,#244030,
#244031,#244032,#244033,#244034,#244035,#244036,#244037,#244038,#244039,
#244040,#244041,#244042,#244043,#244044,#244045,#244046,#244047,#244048,
#244049,#244050,#244051,#244052,#244053,#244054),.UNSPECIFIED.,.F.,.F.,
(4,3,3,3,3,3,3,3,3,3,3,3,3,3,3,3,3,3,3,3,3,3,3,3,3,3,3,3,3,3,3,3,3,3,3,
3,3,3,3,3,3,3,3,3,3,3,3,3,3,3,3,3,3,3,3,3,3,3,3,3,3,3,3,3,3,3,3,3,3,3,3,
3,3,3,3,3,3,3,3,3,3,3,3,3,3,3,3,3,3,3,3,3,3,3,3,3,3,3,3,3,3,3,3,3,3,3,3,
3,4),(-1.,-0.994495413,-0.988990826,-0.983486239,-0.977981651,-0.972477064,
-0.966972477,-0.96146789,-0.955963303,-0.950458716,-0.944954128,-0.939449541,
-0.933944954,-0.926605505,-0.919266055,-0.913761468,-0.908256881,-0.902752294,
-0.897247706,-0.891743119,-0.886238532,-0.880733945,-0.875229358,-0.869724771,
-0.864220183,-0.858715596,-0.851376147,-0.84587156,-0.840366972,-0.834862385,
-0.829357798,-0.823853211,-0.818348624,-0.812844037,-0.80733945,-0.8,-0.79266055,
-0.785321101,-0.777981651,-0.770642202,-0.763302752,-0.755963303,-0.748623853,
-0.741284404,-0.732110092,-0.724770642,-0.717431193,-0.708256881,-0.700917431,
-0.693577982,-0.686238532,-0.67706422,-0.669724771,-0.662385321,-0.655045872,
-0.647706422,-0.640366972,-0.633027523,-0.625688073,-0.618348624,-0.611009174,
-0.603669725,-0.596330275,-0.588990826,-0.581651376,-0.574311927,-0.566972477,
-0.559633028,-0.552293578,-0.544954128,-0.537614679,-0.530275229,-0.521100917,
-0.511926606,-0.502752294,-0.493577982,-0.478899083,-0.469724771,-0.460550459,
-0.451376147,-0.442201835,-0.433027523,-0.423853211,-0.414678899,-0.405504587,
-0.396330275,-0.387155963,-0.376146789,-0.365137615,-0.35412844,-0.343119266,
-0.332110092,-0.321100917,-0.310091743,-0.299082569,-0.288073394,-0.27706422,
-0.266055046,-0.255045872,-0.244036697,-0.233027523,-0.222018349,-0.211009174,
-0.2,-0.188990826,-0.177981651,-0.166972477,-0.155963303,-0.143172102),
 .UNSPECIFIED.);
#24428=B_SPLINE_CURVE_WITH_KNOTS('',3,(#244055,#244056,#244057,#244058,
#244059,#244060,#244061,#244062,#244063,#244064,#244065,#244066,#244067,
#244068,#244069,#244070,#244071,#244072,#244073,#244074,#244075,#244076,
#244077,#244078,#244079,#244080,#244081,#244082,#244083,#244084,#244085,
#244086,#244087,#244088,#244089,#244090,#244091,#244092,#244093,#244094,
#244095,#244096,#244097,#244098,#244099,#244100,#244101,#244102,#244103,
#244104,#244105,#244106,#244107,#244108,#244109,#244110,#244111,#244112,
#244113,#244114,#244115,#244116,#244117,#244118,#244119,#244120,#244121,
#244122,#244123,#244124,#244125,#244126,#244127,#244128,#244129,#244130,
#244131,#244132,#244133,#244134,#244135,#244136,#244137,#244138,#244139,
#244140,#244141,#244142,#244143,#244144,#244145,#244146,#244147,#244148,
#244149,#244150,#244151,#244152,#244153,#244154,#244155,#244156,#244157,
#244158,#244159,#244160,#244161,#244162,#244163,#244164,#244165,#244166,
#244167,#244168,#244169,#244170,#244171,#244172,#244173,#244174,#244175,
#244176,#244177,#244178,#244179,#244180,#244181,#244182,#244183,#244184,
#244185,#244186,#244187,#244188,#244189,#244190,#244191,#244192,#244193,
#244194,#244195,#244196,#244197,#244198,#244199,#244200,#244201,#244202,
#244203,#244204,#244205,#244206,#244207,#244208,#244209,#244210,#244211,
#244212,#244213,#244214,#244215,#244216,#244217,#244218,#244219,#244220,
#244221,#244222,#244223,#244224,#244225,#244226,#244227,#244228,#244229,
#244230,#244231,#244232,#244233,#244234,#244235,#244236,#244237,#244238,
#244239,#244240,#244241,#244242,#244243,#244244,#244245,#244246,#244247,
#244248,#244249,#244250,#244251,#244252,#244253,#244254,#244255,#244256,
#244257,#244258,#244259,#244260,#244261,#244262,#244263,#244264,#244265,
#244266,#244267,#244268,#244269,#244270,#244271,#244272,#244273,#244274,
#244275,#244276,#244277,#244278,#244279,#244280,#244281,#244282,#244283,
#244284,#244285,#244286,#244287,#244288,#244289,#244290,#244291,#244292,
#244293,#244294,#244295,#244296,#244297,#244298,#244299,#244300,#244301,
#244302,#244303,#244304,#244305,#244306,#244307,#244308,#244309,#244310,
#244311,#244312,#244313,#244314,#244315,#244316,#244317,#244318,#244319,
#244320,#244321,#244322,#244323,#244324,#244325,#244326,#244327,#244328,
#244329,#244330,#244331,#244332,#244333,#244334,#244335,#244336,#244337,
#244338,#244339,#244340,#244341,#244342,#244343,#244344,#244345,#244346,
#244347,#244348,#244349,#244350,#244351,#244352,#244353,#244354,#244355,
#244356,#244357,#244358,#244359,#244360,#244361),.UNSPECIFIED.,.F.,.F.,
(4,3,3,3,3,3,3,3,3,3,3,3,3,3,3,3,3,3,3,3,3,3,3,3,3,3,3,3,3,3,3,3,3,3,3,
3,3,3,3,3,3,3,3,3,3,3,3,3,3,3,3,3,3,3,3,3,3,3,3,3,3,3,3,3,3,3,3,3,3,3,3,
3,3,3,3,3,3,3,3,3,3,3,3,3,3,3,3,3,3,3,3,3,3,3,3,3,3,3,3,3,3,3,4),(0.143172102,
0.15412844,0.165137615,0.177981651,0.188990826,0.2,0.211009174,0.222018349,
0.233027523,0.244036697,0.255045872,0.266055046,0.27706422,0.288073394,
0.299082569,0.310091743,0.321100917,0.332110092,0.343119266,0.35412844,
0.365137615,0.376146789,0.387155963,0.396330275,0.405504587,0.418348624,
0.429357798,0.43853211,0.449541284,0.460550459,0.473394495,0.486238532,
0.495412844,0.506422018,0.51559633,0.524770642,0.535779817,0.543119266,
0.550458716,0.557798165,0.565137615,0.572477064,0.581651376,0.588990826,
0.596330275,0.603669725,0.611009174,0.618348624,0.625688073,0.633027523,
0.640366972,0.647706422,0.655045872,0.662385321,0.669724771,0.67706422,
0.68440367,0.693577982,0.700917431,0.708256881,0.71559633,0.72293578,0.730275229,
0.737614679,0.744954128,0.752293578,0.763302752,0.770642202,0.777981651,
0.785321101,0.79266055,0.8,0.80733945,0.812844037,0.820183486,0.825688073,
0.831192661,0.836697248,0.842201835,0.851376147,0.856880734,0.864220183,
0.869724771,0.875229358,0.882568807,0.888073394,0.897247706,0.902752294,
0.908256881,0.91559633,0.92293578,0.930275229,0.937614679,0.943119266,0.950458716,
0.955963303,0.96146789,0.966972477,0.972477064,0.977981651,0.983486239,
0.99266055,1.),.UNSPECIFIED.);
#24429=B_SPLINE_CURVE_WITH_KNOTS('',5,(#245306,#245307,#245308,#245309,
#245310,#245311,#245312,#245313,#245314,#245315,#245316,#245317,#245318,
#245319,#245320,#245321,#245322,#245323,#245324,#245325,#245326,#245327,
#245328,#245329,#245330,#245331,#245332,#245333,#245334,#245335,#245336,
#245337,#245338,#245339,#245340,#245341,#245342,#245343,#245344,#245345,
#245346,#245347,#245348,#245349,#245350,#245351,#245352,#245353,#245354,
#245355,#245356,#245357,#245358,#245359,#245360,#245361,#245362,#245363,
#245364,#245365,#245366,#245367,#245368,#245369,#245370,#245371,#245372,
#245373,#245374,#245375,#245376,#245377,#245378,#245379,#245380,#245381,
#245382,#245383,#245384,#245385,#245386,#245387,#245388,#245389,#245390,
#245391,#245392,#245393,#245394,#245395,#245396,#245397,#245398,#245399,
#245400,#245401,#245402,#245403,#245404,#245405,#245406,#245407,#245408,
#245409,#245410,#245411,#245412,#245413,#245414,#245415,#245416,#245417,
#245418,#245419,#245420,#245421,#245422,#245423,#245424,#245425,#245426,
#245427,#245428,#245429,#245430,#245431,#245432,#245433,#245434,#245435,
#245436,#245437,#245438,#245439,#245440,#245441,#245442,#245443,#245444,
#245445,#245446,#245447,#245448,#245449,#245450,#245451,#245452,#245453,
#245454,#245455,#245456,#245457,#245458,#245459,#245460,#245461,#245462,
#245463,#245464,#245465,#245466,#245467,#245468,#245469,#245470,#245471,
#245472,#245473,#245474,#245475,#245476,#245477,#245478,#245479,#245480,
#245481,#245482,#245483,#245484,#245485,#245486,#245487,#245488,#245489,
#245490,#245491,#245492,#245493,#245494,#245495,#245496,#245497,#245498,
#245499,#245500,#245501,#245502,#245503,#245504,#245505,#245506,#245507,
#245508,#245509,#245510,#245511,#245512,#245513,#245514,#245515,#245516,
#245517,#245518,#245519,#245520,#245521,#245522,#245523,#245524,#245525,
#245526,#245527,#245528,#245529,#245530,#245531,#245532,#245533,#245534,
#245535,#245536,#245537,#245538,#245539,#245540,#245541,#245542,#245543,
#245544,#245545,#245546,#245547,#245548,#245549,#245550,#245551,#245552,
#245553,#245554,#245555,#245556,#245557,#245558,#245559,#245560,#245561,
#245562,#245563,#245564,#245565,#245566,#245567,#245568,#245569,#245570,
#245571,#245572,#245573,#245574,#245575,#245576,#245577,#245578,#245579,
#245580,#245581,#245582,#245583,#245584,#245585,#245586,#245587,#245588,
#245589,#245590,#245591,#245592,#245593,#245594,#245595,#245596,#245597,
#245598,#245599,#245600,#245601,#245602,#245603,#245604,#245605,#245606,
#245607,#245608,#245609,#245610,#245611,#245612,#245613,#245614,#245615,
#245616,#245617,#245618,#245619,#245620,#245621,#245622,#245623,#245624,
#245625,#245626,#245627,#245628,#245629,#245630,#245631,#245632,#245633,
#245634,#245635,#245636,#245637,#245638,#245639,#245640,#245641,#245642,
#245643,#245644,#245645,#245646,#245647,#245648,#245649,#245650,#245651,
#245652,#245653,#245654,#245655,#245656,#245657,#245658,#245659,#245660,
#245661,#245662,#245663,#245664,#245665,#245666,#245667,#245668,#245669,
#245670,#245671,#245672,#245673,#245674,#245675,#245676,#245677,#245678,
#245679,#245680,#245681,#245682,#245683,#245684,#245685,#245686,#245687,
#245688,#245689,#245690,#245691,#245692,#245693,#245694,#245695,#245696,
#245697,#245698,#245699,#245700,#245701,#245702,#245703,#245704,#245705,
#245706,#245707,#245708,#245709,#245710,#245711,#245712,#245713,#245714,
#245715,#245716,#245717,#245718,#245719,#245720,#245721,#245722,#245723,
#245724,#245725,#245726,#245727,#245728,#245729,#245730,#245731,#245732,
#245733,#245734,#245735,#245736,#245737,#245738,#245739,#245740,#245741,
#245742,#245743,#245744,#245745,#245746,#245747,#245748,#245749,#245750,
#245751,#245752,#245753,#245754,#245755,#245756,#245757,#245758,#245759,
#245760,#245761,#245762,#245763,#245764,#245765,#245766,#245767,#245768,
#245769,#245770,#245771,#245772,#245773,#245774,#245775,#245776,#245777),
 .UNSPECIFIED.,.F.,.F.,(6,1,1,1,1,1,1,1,1,1,1,1,1,1,1,1,1,1,1,1,1,1,1,1,
1,1,1,1,1,1,1,1,1,1,1,1,1,1,1,1,1,1,1,1,1,1,1,1,1,1,1,1,1,1,1,1,1,1,1,1,
1,1,1,1,1,1,1,1,1,1,1,1,1,1,1,1,1,1,1,1,1,1,1,1,1,1,1,1,1,1,1,1,1,1,1,1,
1,1,1,1,1,1,1,1,1,1,1,1,1,1,1,1,1,1,1,1,1,1,1,1,1,1,1,1,1,1,1,1,1,1,1,1,
1,1,1,1,1,1,1,1,1,1,1,1,1,1,1,1,1,1,1,1,1,1,1,1,1,1,1,1,1,1,1,1,1,1,1,1,
1,1,1,1,1,1,1,1,1,1,1,1,1,1,1,1,1,1,1,1,1,1,1,1,1,1,1,1,1,1,1,1,1,1,1,1,
1,1,1,1,1,1,1,1,1,1,1,1,1,1,1,1,1,1,1,1,1,1,1,1,1,1,1,1,1,1,1,1,1,1,1,1,
1,1,1,1,1,1,1,1,1,1,1,1,1,1,1,1,1,1,1,1,1,1,1,1,1,1,1,1,1,1,1,1,1,1,1,1,
1,1,1,1,1,1,1,1,1,1,1,1,1,1,1,1,1,1,1,1,1,1,1,1,1,1,1,1,1,1,1,1,1,1,1,1,
1,1,1,1,1,1,1,1,1,1,1,1,1,1,1,1,1,1,1,1,1,1,1,1,1,1,1,1,1,1,1,1,1,1,1,1,
1,1,1,1,1,1,1,1,1,1,1,1,1,1,1,1,1,1,1,1,1,1,1,1,1,1,1,1,1,1,1,1,1,1,1,1,
1,1,1,1,1,1,1,1,1,1,1,1,1,1,1,1,1,1,1,1,1,1,1,1,1,1,1,1,1,1,1,1,1,1,1,1,
1,1,1,1,1,1,1,1,1,1,1,1,1,1,1,1,1,1,1,1,1,1,1,1,1,1,1,1,1,1,1,1,1,1,1,1,
1,1,1,1,1,1,1,1,1,1,1,6),(0.143172102,0.144954128,0.146788991,0.148623853,
0.150458716,0.152293578,0.15412844,0.155963303,0.157798165,0.159633028,
0.16146789,0.163302752,0.165137615,0.166972477,0.168807339,0.170642202,
0.172477064,0.174311927,0.176146789,0.177981651,0.179816514,0.181651376,
0.183486239,0.185321101,0.187155963,0.188990826,0.190825688,0.19266055,
0.194495413,0.196330275,0.198165138,0.2,0.201834862,0.203669725,0.205504587,
0.20733945,0.209174312,0.211009174,0.212844037,0.214678899,0.216513761,
0.218348624,0.220183486,0.222018349,0.223853211,0.225688073,0.227522936,
0.229357798,0.231192661,0.233027523,0.234862385,0.236697248,0.23853211,
0.240366972,0.242201835,0.244036697,0.24587156,0.247706422,0.249541284,
0.251376147,0.253211009,0.255045872,0.256880734,0.258715596,0.260550459,
0.262385321,0.264220183,0.266055046,0.267889908,0.269724771,0.271559633,
0.273394495,0.275229358,0.27706422,0.278899083,0.280733945,0.282568807,
0.28440367,0.286238532,0.288073394,0.289908257,0.291743119,0.293577982,
0.295412844,0.297247706,0.299082569,0.300917431,0.302752294,0.304587156,
0.306422018,0.308256881,0.310091743,0.311926606,0.313761468,0.31559633,
0.317431193,0.319266055,0.321100917,0.32293578,0.324770642,0.326605505,
0.328440367,0.330275229,0.332110092,0.333944954,0.335779817,0.337614679,
0.339449541,0.341284404,0.343119266,0.344954128,0.346788991,0.348623853,
0.350458716,0.352293578,0.35412844,0.355963303,0.357798165,0.359633028,
0.36146789,0.363302752,0.365137615,0.366972477,0.368807339,0.370642202,
0.372477064,0.374311927,0.376146789,0.377981651,0.379816514,0.381651376,
0.383486239,0.385321101,0.387155963,0.388990826,0.390825688,0.39266055,
0.394495413,0.396330275,0.398165138,0.4,0.401834862,0.403669725,0.405504587,
0.40733945,0.409174312,0.411009174,0.412844037,0.414678899,0.416513761,
0.418348624,0.420183486,0.422018349,0.423853211,0.425688073,0.427522936,
0.429357798,0.431192661,0.433027523,0.434862385,0.436697248,0.43853211,
0.440366972,0.442201835,0.444036697,0.44587156,0.447706422,0.449541284,
0.451376147,0.453211009,0.455045872,0.456880734,0.458715596,0.460550459,
0.462385321,0.464220183,0.466055046,0.467889908,0.469724771,0.471559633,
0.473394495,0.475229358,0.47706422,0.478899083,0.480733945,0.482568807,
0.48440367,0.486238532,0.488073394,0.489908257,0.491743119,0.493577982,
0.495412844,0.497247706,0.499082569,0.500917431,0.502752294,0.504587156,
0.506422018,0.508256881,0.510091743,0.511926606,0.513761468,0.51559633,
0.517431193,0.519266055,0.521100917,0.52293578,0.524770642,0.526605505,
0.528440367,0.530275229,0.532110092,0.533944954,0.535779817,0.537614679,
0.539449541,0.541284404,0.543119266,0.544954128,0.546788991,0.548623853,
0.550458716,0.552293578,0.55412844,0.555963303,0.557798165,0.559633028,
0.56146789,0.563302752,0.565137615,0.566972477,0.568807339,0.570642202,
0.572477064,0.574311927,0.576146789,0.577981651,0.579816514,0.581651376,
0.583486239,0.585321101,0.587155963,0.588990826,0.590825688,0.59266055,
0.594495413,0.596330275,0.598165138,0.6,0.601834862,0.603669725,0.605504587,
0.60733945,0.609174312,0.611009174,0.612844037,0.614678899,0.616513761,
0.618348624,0.620183486,0.622018349,0.623853211,0.625688073,0.627522936,
0.629357798,0.631192661,0.633027523,0.634862385,0.636697248,0.63853211,
0.640366972,0.642201835,0.644036697,0.64587156,0.647706422,0.649541284,
0.651376147,0.653211009,0.655045872,0.656880734,0.658715596,0.660550459,
0.662385321,0.664220183,0.666055046,0.667889908,0.669724771,0.671559633,
0.673394495,0.675229358,0.67706422,0.678899083,0.680733945,0.682568807,
0.68440367,0.686238532,0.688073394,0.689908257,0.691743119,0.693577982,
0.695412844,0.697247706,0.699082569,0.700917431,0.702752294,0.704587156,
0.706422018,0.708256881,0.710091743,0.711926606,0.713761468,0.71559633,
0.717431193,0.719266055,0.721100917,0.72293578,0.724770642,0.726605505,
0.728440367,0.730275229,0.732110092,0.733944954,0.735779817,0.737614679,
0.739449541,0.741284404,0.743119266,0.744954128,0.746788991,0.748623853,
0.750458716,0.752293578,0.75412844,0.755963303,0.757798165,0.759633028,
0.76146789,0.763302752,0.765137615,0.766972477,0.768807339,0.770642202,
0.772477064,0.774311927,0.776146789,0.777981651,0.779816514,0.781651376,
0.783486239,0.785321101,0.787155963,0.788990826,0.790825688,0.79266055,
0.794495413,0.796330275,0.798165138,0.8,0.801834862,0.803669725,0.805504587,
0.80733945,0.809174312,0.811009174,0.812844037,0.814678899,0.816513761,
0.818348624,0.820183486,0.822018349,0.823853211,0.825688073,0.827522936,
0.829357798,0.831192661,0.833027523,0.834862385,0.836697248,0.83853211,
0.840366972,0.842201835,0.844036697,0.84587156,0.847706422,0.849541284,
0.851376147,0.853211009,0.855045872,0.856880734,0.858715596,0.860550459,
0.862385321,0.864220183,0.866055046,0.867889908,0.869724771,0.871559633,
0.873394495,0.875229358,0.87706422,0.878899083,0.880733945,0.882568807,
0.88440367,0.886238532,0.888073394,0.889908257,0.891743119,0.893577982,
0.895412844,0.897247706,0.899082569,0.900917431,0.902752294,0.904587156,
0.906422018,0.908256881,0.910091743,0.911926606,0.913761468,0.91559633,
0.917431193,0.919266055,0.921100917,0.92293578,0.924770642,0.926605505,
0.928440367,0.930275229,0.932110092,0.933944954,0.935779817,0.937614679,
0.939449541,0.941284404,0.943119266,0.944954128,0.946788991,0.948623853,
0.950458716,0.952293578,0.95412844,0.955963303,0.957798165,0.959633028,
0.96146789,0.963302752,0.965137615,0.966972477,0.968807339,0.970642202,
0.972477064,0.974311927,0.976146789,0.977981651,0.979816514,0.981651376,
0.983486239,0.985321101,0.987155963,0.988990826,0.990825688,0.99266055,
0.994495413,0.996330275,0.998165138,1.),.UNSPECIFIED.);
#24430=B_SPLINE_CURVE_WITH_KNOTS('',5,(#245778,#245779,#245780,#245781,
#245782,#245783,#245784,#245785,#245786,#245787,#245788,#245789,#245790,
#245791,#245792,#245793,#245794,#245795,#245796,#245797,#245798,#245799,
#245800,#245801,#245802,#245803,#245804,#245805,#245806,#245807,#245808,
#245809,#245810,#245811,#245812,#245813,#245814,#245815,#245816,#245817,
#245818,#245819,#245820,#245821,#245822,#245823,#245824,#245825,#245826,
#245827,#245828,#245829,#245830,#245831,#245832,#245833,#245834,#245835,
#245836,#245837,#245838,#245839,#245840,#245841,#245842,#245843,#245844,
#245845,#245846,#245847,#245848,#245849,#245850,#245851,#245852,#245853,
#245854,#245855,#245856,#245857,#245858,#245859,#245860,#245861,#245862,
#245863,#245864,#245865,#245866,#245867,#245868,#245869,#245870,#245871,
#245872,#245873,#245874,#245875,#245876,#245877,#245878,#245879,#245880,
#245881,#245882,#245883,#245884,#245885,#245886,#245887,#245888,#245889,
#245890,#245891,#245892,#245893,#245894,#245895,#245896,#245897,#245898,
#245899,#245900,#245901,#245902,#245903,#245904,#245905,#245906,#245907,
#245908,#245909,#245910,#245911,#245912,#245913,#245914,#245915,#245916,
#245917,#245918,#245919,#245920,#245921,#245922,#245923,#245924,#245925,
#245926,#245927,#245928,#245929,#245930,#245931,#245932,#245933,#245934,
#245935,#245936,#245937,#245938,#245939,#245940,#245941,#245942,#245943,
#245944,#245945,#245946,#245947,#245948,#245949,#245950,#245951,#245952,
#245953,#245954,#245955,#245956,#245957,#245958,#245959,#245960,#245961,
#245962,#245963,#245964,#245965,#245966,#245967,#245968,#245969,#245970,
#245971,#245972,#245973,#245974,#245975,#245976,#245977,#245978,#245979,
#245980,#245981,#245982,#245983,#245984,#245985,#245986,#245987,#245988,
#245989,#245990,#245991,#245992,#245993,#245994,#245995,#245996,#245997,
#245998,#245999,#246000,#246001,#246002,#246003,#246004,#246005,#246006,
#246007,#246008,#246009,#246010,#246011,#246012,#246013,#246014,#246015,
#246016,#246017,#246018,#246019,#246020,#246021,#246022,#246023,#246024,
#246025,#246026,#246027,#246028,#246029,#246030,#246031,#246032,#246033,
#246034,#246035,#246036,#246037,#246038,#246039,#246040,#246041,#246042,
#246043,#246044,#246045,#246046,#246047,#246048,#246049,#246050,#246051,
#246052,#246053,#246054,#246055,#246056,#246057,#246058,#246059,#246060,
#246061,#246062,#246063,#246064,#246065,#246066,#246067,#246068,#246069,
#246070,#246071,#246072,#246073,#246074,#246075,#246076,#246077,#246078,
#246079,#246080,#246081,#246082,#246083,#246084,#246085,#246086,#246087,
#246088,#246089,#246090,#246091,#246092,#246093,#246094,#246095,#246096,
#246097,#246098,#246099,#246100,#246101,#246102,#246103,#246104,#246105,
#246106,#246107,#246108,#246109,#246110,#246111,#246112,#246113,#246114,
#246115,#246116,#246117,#246118,#246119,#246120,#246121,#246122,#246123,
#246124,#246125,#246126,#246127,#246128,#246129,#246130,#246131,#246132,
#246133,#246134,#246135,#246136,#246137,#246138,#246139,#246140,#246141,
#246142,#246143,#246144,#246145,#246146,#246147,#246148,#246149,#246150,
#246151,#246152,#246153,#246154,#246155,#246156,#246157,#246158,#246159,
#246160,#246161,#246162,#246163,#246164,#246165,#246166,#246167,#246168,
#246169,#246170,#246171,#246172,#246173,#246174,#246175,#246176,#246177,
#246178,#246179,#246180,#246181,#246182,#246183,#246184,#246185,#246186,
#246187,#246188,#246189,#246190,#246191,#246192,#246193,#246194,#246195,
#246196,#246197,#246198,#246199,#246200,#246201,#246202,#246203,#246204,
#246205,#246206,#246207,#246208,#246209,#246210,#246211,#246212,#246213,
#246214,#246215,#246216,#246217,#246218,#246219,#246220,#246221,#246222,
#246223,#246224,#246225,#246226,#246227,#246228,#246229,#246230,#246231,
#246232,#246233,#246234,#246235,#246236,#246237,#246238,#246239,#246240,
#246241,#246242,#246243,#246244,#246245,#246246,#246247,#246248,#246249),
 .UNSPECIFIED.,.F.,.F.,(6,1,1,1,1,1,1,1,1,1,1,1,1,1,1,1,1,1,1,1,1,1,1,1,
1,1,1,1,1,1,1,1,1,1,1,1,1,1,1,1,1,1,1,1,1,1,1,1,1,1,1,1,1,1,1,1,1,1,1,1,
1,1,1,1,1,1,1,1,1,1,1,1,1,1,1,1,1,1,1,1,1,1,1,1,1,1,1,1,1,1,1,1,1,1,1,1,
1,1,1,1,1,1,1,1,1,1,1,1,1,1,1,1,1,1,1,1,1,1,1,1,1,1,1,1,1,1,1,1,1,1,1,1,
1,1,1,1,1,1,1,1,1,1,1,1,1,1,1,1,1,1,1,1,1,1,1,1,1,1,1,1,1,1,1,1,1,1,1,1,
1,1,1,1,1,1,1,1,1,1,1,1,1,1,1,1,1,1,1,1,1,1,1,1,1,1,1,1,1,1,1,1,1,1,1,1,
1,1,1,1,1,1,1,1,1,1,1,1,1,1,1,1,1,1,1,1,1,1,1,1,1,1,1,1,1,1,1,1,1,1,1,1,
1,1,1,1,1,1,1,1,1,1,1,1,1,1,1,1,1,1,1,1,1,1,1,1,1,1,1,1,1,1,1,1,1,1,1,1,
1,1,1,1,1,1,1,1,1,1,1,1,1,1,1,1,1,1,1,1,1,1,1,1,1,1,1,1,1,1,1,1,1,1,1,1,
1,1,1,1,1,1,1,1,1,1,1,1,1,1,1,1,1,1,1,1,1,1,1,1,1,1,1,1,1,1,1,1,1,1,1,1,
1,1,1,1,1,1,1,1,1,1,1,1,1,1,1,1,1,1,1,1,1,1,1,1,1,1,1,1,1,1,1,1,1,1,1,1,
1,1,1,1,1,1,1,1,1,1,1,1,1,1,1,1,1,1,1,1,1,1,1,1,1,1,1,1,1,1,1,1,1,1,1,1,
1,1,1,1,1,1,1,1,1,1,1,1,1,1,1,1,1,1,1,1,1,1,1,1,1,1,1,1,1,1,1,1,1,1,1,1,
1,1,1,1,1,1,1,1,1,1,1,6),(0.143172102,0.144954128,0.146788991,0.148623853,
0.150458716,0.152293578,0.15412844,0.155963303,0.157798165,0.159633028,
0.16146789,0.163302752,0.165137615,0.166972477,0.168807339,0.170642202,
0.172477064,0.174311927,0.176146789,0.177981651,0.179816514,0.181651376,
0.183486239,0.185321101,0.187155963,0.188990826,0.190825688,0.19266055,
0.194495413,0.196330275,0.198165138,0.2,0.201834862,0.203669725,0.205504587,
0.20733945,0.209174312,0.211009174,0.212844037,0.214678899,0.216513761,
0.218348624,0.220183486,0.222018349,0.223853211,0.225688073,0.227522936,
0.229357798,0.231192661,0.233027523,0.234862385,0.236697248,0.23853211,
0.240366972,0.242201835,0.244036697,0.24587156,0.247706422,0.249541284,
0.251376147,0.253211009,0.255045872,0.256880734,0.258715596,0.260550459,
0.262385321,0.264220183,0.266055046,0.267889908,0.269724771,0.271559633,
0.273394495,0.275229358,0.27706422,0.278899083,0.280733945,0.282568807,
0.28440367,0.286238532,0.288073394,0.289908257,0.291743119,0.293577982,
0.295412844,0.297247706,0.299082569,0.300917431,0.302752294,0.304587156,
0.306422018,0.308256881,0.310091743,0.311926606,0.313761468,0.31559633,
0.317431193,0.319266055,0.321100917,0.32293578,0.324770642,0.326605505,
0.328440367,0.330275229,0.332110092,0.333944954,0.335779817,0.337614679,
0.339449541,0.341284404,0.343119266,0.344954128,0.346788991,0.348623853,
0.350458716,0.352293578,0.35412844,0.355963303,0.357798165,0.359633028,
0.36146789,0.363302752,0.365137615,0.366972477,0.368807339,0.370642202,
0.372477064,0.374311927,0.376146789,0.377981651,0.379816514,0.381651376,
0.383486239,0.385321101,0.387155963,0.388990826,0.390825688,0.39266055,
0.394495413,0.396330275,0.398165138,0.4,0.401834862,0.403669725,0.405504587,
0.40733945,0.409174312,0.411009174,0.412844037,0.414678899,0.416513761,
0.418348624,0.420183486,0.422018349,0.423853211,0.425688073,0.427522936,
0.429357798,0.431192661,0.433027523,0.434862385,0.436697248,0.43853211,
0.440366972,0.442201835,0.444036697,0.44587156,0.447706422,0.449541284,
0.451376147,0.453211009,0.455045872,0.456880734,0.458715596,0.460550459,
0.462385321,0.464220183,0.466055046,0.467889908,0.469724771,0.471559633,
0.473394495,0.475229358,0.47706422,0.478899083,0.480733945,0.482568807,
0.48440367,0.486238532,0.488073394,0.489908257,0.491743119,0.493577982,
0.495412844,0.497247706,0.499082569,0.500917431,0.502752294,0.504587156,
0.506422018,0.508256881,0.510091743,0.511926606,0.513761468,0.51559633,
0.517431193,0.519266055,0.521100917,0.52293578,0.524770642,0.526605505,
0.528440367,0.530275229,0.532110092,0.533944954,0.535779817,0.537614679,
0.539449541,0.541284404,0.543119266,0.544954128,0.546788991,0.548623853,
0.550458716,0.552293578,0.55412844,0.555963303,0.557798165,0.559633028,
0.56146789,0.563302752,0.565137615,0.566972477,0.568807339,0.570642202,
0.572477064,0.574311927,0.576146789,0.577981651,0.579816514,0.581651376,
0.583486239,0.585321101,0.587155963,0.588990826,0.590825688,0.59266055,
0.594495413,0.596330275,0.598165138,0.6,0.601834862,0.603669725,0.605504587,
0.60733945,0.609174312,0.611009174,0.612844037,0.614678899,0.616513761,
0.618348624,0.620183486,0.622018349,0.623853211,0.625688073,0.627522936,
0.629357798,0.631192661,0.633027523,0.634862385,0.636697248,0.63853211,
0.640366972,0.642201835,0.644036697,0.64587156,0.647706422,0.649541284,
0.651376147,0.653211009,0.655045872,0.656880734,0.658715596,0.660550459,
0.662385321,0.664220183,0.666055046,0.667889908,0.669724771,0.671559633,
0.673394495,0.675229358,0.67706422,0.678899083,0.680733945,0.682568807,
0.68440367,0.686238532,0.688073394,0.689908257,0.691743119,0.693577982,
0.695412844,0.697247706,0.699082569,0.700917431,0.702752294,0.704587156,
0.706422018,0.708256881,0.710091743,0.711926606,0.713761468,0.71559633,
0.717431193,0.719266055,0.721100917,0.72293578,0.724770642,0.726605505,
0.728440367,0.730275229,0.732110092,0.733944954,0.735779817,0.737614679,
0.739449541,0.741284404,0.743119266,0.744954128,0.746788991,0.748623853,
0.750458716,0.752293578,0.75412844,0.755963303,0.757798165,0.759633028,
0.76146789,0.763302752,0.765137615,0.766972477,0.768807339,0.770642202,
0.772477064,0.774311927,0.776146789,0.777981651,0.779816514,0.781651376,
0.783486239,0.785321101,0.787155963,0.788990826,0.790825688,0.79266055,
0.794495413,0.796330275,0.798165138,0.8,0.801834862,0.803669725,0.805504587,
0.80733945,0.809174312,0.811009174,0.812844037,0.814678899,0.816513761,
0.818348624,0.820183486,0.822018349,0.823853211,0.825688073,0.827522936,
0.829357798,0.831192661,0.833027523,0.834862385,0.836697248,0.83853211,
0.840366972,0.842201835,0.844036697,0.84587156,0.847706422,0.849541284,
0.851376147,0.853211009,0.855045872,0.856880734,0.858715596,0.860550459,
0.862385321,0.864220183,0.866055046,0.867889908,0.869724771,0.871559633,
0.873394495,0.875229358,0.87706422,0.878899083,0.880733945,0.882568807,
0.88440367,0.886238532,0.888073394,0.889908257,0.891743119,0.893577982,
0.895412844,0.897247706,0.899082569,0.900917431,0.902752294,0.904587156,
0.906422018,0.908256881,0.910091743,0.911926606,0.913761468,0.91559633,
0.917431193,0.919266055,0.921100917,0.92293578,0.924770642,0.926605505,
0.928440367,0.930275229,0.932110092,0.933944954,0.935779817,0.937614679,
0.939449541,0.941284404,0.943119266,0.944954128,0.946788991,0.948623853,
0.950458716,0.952293578,0.95412844,0.955963303,0.957798165,0.959633028,
0.96146789,0.963302752,0.965137615,0.966972477,0.968807339,0.970642202,
0.972477064,0.974311927,0.976146789,0.977981651,0.979816514,0.981651376,
0.983486239,0.985321101,0.987155963,0.988990826,0.990825688,0.99266055,
0.994495413,0.996330275,0.998165138,1.),.UNSPECIFIED.);
#24431=B_SPLINE_CURVE_WITH_KNOTS('',3,(#247209,#247210,#247211,#247212,
#247213,#247214,#247215,#247216,#247217,#247218,#247219,#247220,#247221,
#247222,#247223,#247224,#247225,#247226,#247227,#247228,#247229,#247230,
#247231,#247232,#247233,#247234,#247235,#247236,#247237,#247238,#247239,
#247240,#247241,#247242,#247243,#247244,#247245,#247246,#247247,#247248,
#247249,#247250,#247251,#247252,#247253,#247254,#247255,#247256,#247257,
#247258,#247259,#247260,#247261,#247262,#247263,#247264,#247265,#247266,
#247267,#247268,#247269,#247270,#247271,#247272,#247273,#247274,#247275,
#247276,#247277,#247278,#247279,#247280,#247281,#247282,#247283,#247284,
#247285,#247286,#247287,#247288,#247289,#247290,#247291,#247292,#247293,
#247294,#247295,#247296,#247297,#247298,#247299,#247300,#247301,#247302,
#247303,#247304,#247305,#247306,#247307,#247308,#247309,#247310,#247311,
#247312,#247313,#247314,#247315,#247316,#247317,#247318,#247319,#247320,
#247321,#247322,#247323,#247324,#247325,#247326,#247327,#247328,#247329,
#247330,#247331,#247332,#247333,#247334,#247335,#247336,#247337,#247338,
#247339,#247340,#247341,#247342,#247343,#247344,#247345,#247346,#247347,
#247348,#247349,#247350,#247351,#247352,#247353,#247354,#247355,#247356,
#247357,#247358,#247359,#247360,#247361,#247362,#247363,#247364,#247365,
#247366,#247367,#247368,#247369,#247370,#247371,#247372,#247373,#247374,
#247375,#247376,#247377,#247378,#247379,#247380,#247381,#247382,#247383,
#247384,#247385,#247386,#247387,#247388,#247389,#247390,#247391,#247392,
#247393,#247394,#247395,#247396,#247397,#247398,#247399,#247400,#247401,
#247402,#247403,#247404,#247405,#247406,#247407,#247408,#247409,#247410,
#247411,#247412,#247413,#247414,#247415,#247416,#247417,#247418,#247419,
#247420,#247421,#247422,#247423,#247424,#247425,#247426,#247427,#247428,
#247429,#247430,#247431,#247432,#247433,#247434,#247435,#247436,#247437,
#247438,#247439,#247440,#247441,#247442,#247443,#247444,#247445,#247446,
#247447,#247448,#247449,#247450,#247451,#247452,#247453,#247454,#247455,
#247456,#247457,#247458,#247459,#247460,#247461,#247462,#247463,#247464,
#247465,#247466,#247467,#247468,#247469,#247470,#247471,#247472,#247473,
#247474,#247475,#247476,#247477,#247478,#247479,#247480,#247481,#247482,
#247483,#247484,#247485,#247486,#247487,#247488,#247489,#247490,#247491,
#247492,#247493,#247494,#247495,#247496,#247497,#247498,#247499,#247500,
#247501,#247502,#247503,#247504,#247505,#247506,#247507,#247508,#247509,
#247510,#247511,#247512,#247513,#247514,#247515,#247516,#247517,#247518,
#247519,#247520,#247521),.UNSPECIFIED.,.F.,.F.,(4,3,3,3,3,3,3,3,3,3,3,3,
3,3,3,3,3,3,3,3,3,3,3,3,3,3,3,3,3,3,3,3,3,3,3,3,3,3,3,3,3,3,3,3,3,3,3,3,
3,3,3,3,3,3,3,3,3,3,3,3,3,3,3,3,3,3,3,3,3,3,3,3,3,3,3,3,3,3,3,3,3,3,3,3,
3,3,3,3,3,3,3,3,3,3,3,3,3,3,3,3,3,3,3,3,4),(0.143172102,0.15412844,0.165137615,
0.176146789,0.187155963,0.198165138,0.209174312,0.220183486,0.231192661,
0.242201835,0.253211009,0.264220183,0.275229358,0.286238532,0.297247706,
0.308256881,0.319266055,0.330275229,0.341284404,0.352293578,0.363302752,
0.374311927,0.385321101,0.396330275,0.405504587,0.414678899,0.423853211,
0.434862385,0.444036697,0.453211009,0.462385321,0.471559633,0.480733945,
0.489908257,0.499082569,0.508256881,0.517431193,0.526605505,0.535779817,
0.543119266,0.550458716,0.557798165,0.565137615,0.572477064,0.579816514,
0.587155963,0.594495413,0.603669725,0.611009174,0.618348624,0.625688073,
0.634862385,0.644036697,0.653211009,0.662385321,0.669724771,0.67706422,
0.68440367,0.691743119,0.702752294,0.710091743,0.717431193,0.726605505,
0.733944954,0.741284404,0.752293578,0.759633028,0.768807339,0.779816514,
0.787155963,0.794495413,0.801834862,0.809174312,0.814678899,0.820183486,
0.827522936,0.833027523,0.840366972,0.84587156,0.851376147,0.856880734,
0.862385321,0.867889908,0.873394495,0.878899083,0.888073394,0.895412844,
0.900917431,0.908256881,0.91559633,0.921100917,0.926605505,0.933944954,
0.939449541,0.944954128,0.950458716,0.955963303,0.96146789,0.966972477,
0.972477064,0.977981651,0.983486239,0.988990826,0.994495413,1.),
 .UNSPECIFIED.);
#24432=B_SPLINE_CURVE_WITH_KNOTS('',3,(#247522,#247523,#247524,#247525,
#247526,#247527,#247528,#247529,#247530,#247531,#247532,#247533,#247534,
#247535,#247536,#247537,#247538,#247539,#247540,#247541,#247542,#247543,
#247544,#247545,#247546,#247547,#247548,#247549,#247550,#247551,#247552,
#247553,#247554,#247555,#247556,#247557,#247558,#247559,#247560,#247561,
#247562,#247563,#247564,#247565,#247566,#247567,#247568,#247569,#247570,
#247571,#247572,#247573,#247574,#247575,#247576,#247577,#247578,#247579,
#247580,#247581,#247582,#247583,#247584,#247585,#247586,#247587,#247588,
#247589,#247590,#247591,#247592,#247593,#247594,#247595,#247596,#247597,
#247598,#247599,#247600,#247601,#247602,#247603,#247604,#247605,#247606,
#247607,#247608,#247609,#247610,#247611,#247612,#247613,#247614,#247615,
#247616,#247617,#247618,#247619,#247620,#247621,#247622,#247623,#247624,
#247625,#247626,#247627,#247628,#247629,#247630,#247631,#247632,#247633,
#247634,#247635,#247636,#247637,#247638,#247639,#247640,#247641,#247642,
#247643,#247644,#247645,#247646,#247647,#247648,#247649,#247650,#247651,
#247652,#247653,#247654,#247655,#247656,#247657,#247658,#247659,#247660,
#247661,#247662,#247663,#247664,#247665,#247666,#247667,#247668,#247669,
#247670,#247671,#247672,#247673,#247674,#247675,#247676,#247677,#247678,
#247679,#247680,#247681,#247682,#247683,#247684,#247685,#247686,#247687,
#247688,#247689,#247690,#247691,#247692,#247693,#247694,#247695,#247696,
#247697,#247698,#247699,#247700,#247701,#247702,#247703,#247704,#247705,
#247706,#247707,#247708,#247709,#247710,#247711,#247712,#247713,#247714,
#247715,#247716,#247717,#247718,#247719,#247720,#247721,#247722,#247723,
#247724,#247725,#247726,#247727,#247728,#247729,#247730,#247731,#247732,
#247733,#247734,#247735,#247736,#247737,#247738,#247739,#247740,#247741,
#247742,#247743,#247744,#247745,#247746,#247747,#247748,#247749,#247750,
#247751,#247752,#247753,#247754,#247755,#247756,#247757,#247758,#247759,
#247760,#247761,#247762,#247763,#247764,#247765,#247766,#247767,#247768,
#247769,#247770,#247771,#247772,#247773,#247774,#247775,#247776,#247777,
#247778,#247779,#247780,#247781,#247782,#247783,#247784,#247785,#247786,
#247787,#247788,#247789,#247790,#247791,#247792,#247793,#247794,#247795,
#247796,#247797,#247798,#247799,#247800,#247801,#247802,#247803,#247804,
#247805,#247806,#247807,#247808,#247809,#247810,#247811,#247812,#247813,
#247814,#247815,#247816,#247817,#247818,#247819,#247820,#247821,#247822,
#247823,#247824,#247825,#247826,#247827,#247828,#247829,#247830,#247831,
#247832,#247833,#247834,#247835,#247836,#247837,#247838,#247839,#247840,
#247841,#247842,#247843),.UNSPECIFIED.,.F.,.F.,(4,3,3,3,3,3,3,3,3,3,3,3,
3,3,3,3,3,3,3,3,3,3,3,3,3,3,3,3,3,3,3,3,3,3,3,3,3,3,3,3,3,3,3,3,3,3,3,3,
3,3,3,3,3,3,3,3,3,3,3,3,3,3,3,3,3,3,3,3,3,3,3,3,3,3,3,3,3,3,3,3,3,3,3,3,
3,3,3,3,3,3,3,3,3,3,3,3,3,3,3,3,3,3,3,3,3,3,3,4),(0.143172102,0.15412844,
0.165137615,0.176146789,0.187155963,0.198165138,0.209174312,0.220183486,
0.231192661,0.242201835,0.253211009,0.264220183,0.275229358,0.286238532,
0.297247706,0.308256881,0.319266055,0.330275229,0.341284404,0.352293578,
0.363302752,0.374311927,0.385321101,0.396330275,0.405504587,0.414678899,
0.423853211,0.433027523,0.442201835,0.451376147,0.460550459,0.469724771,
0.478899083,0.488073394,0.497247706,0.508256881,0.517431193,0.526605505,
0.533944954,0.541284404,0.548623853,0.555963303,0.563302752,0.570642202,
0.577981651,0.585321101,0.59266055,0.6,0.60733945,0.614678899,0.622018349,
0.629357798,0.636697248,0.644036697,0.651376147,0.658715596,0.667889908,
0.675229358,0.682568807,0.689908257,0.697247706,0.704587156,0.711926606,
0.719266055,0.726605505,0.733944954,0.744954128,0.752293578,0.759633028,
0.768807339,0.776146789,0.783486239,0.790825688,0.798165138,0.805504587,
0.811009174,0.816513761,0.822018349,0.827522936,0.834862385,0.840366972,
0.84587156,0.851376147,0.856880734,0.862385321,0.867889908,0.873394495,
0.878899083,0.888073394,0.895412844,0.900917431,0.906422018,0.911926606,
0.917431193,0.924770642,0.930275229,0.935779817,0.941284404,0.946788991,
0.952293578,0.957798165,0.963302752,0.968807339,0.974311927,0.979816514,
0.985321101,0.994495413,1.),.UNSPECIFIED.);
#24433=B_SPLINE_CURVE_WITH_KNOTS('',3,(#248791,#248792,#248793,#248794,
#248795,#248796,#248797,#248798,#248799,#248800,#248801,#248802,#248803,
#248804,#248805,#248806,#248807,#248808,#248809,#248810,#248811,#248812,
#248813,#248814,#248815,#248816,#248817,#248818,#248819,#248820,#248821,
#248822,#248823,#248824,#248825,#248826,#248827,#248828,#248829,#248830,
#248831,#248832,#248833,#248834,#248835,#248836,#248837,#248838,#248839,
#248840,#248841,#248842,#248843,#248844,#248845,#248846,#248847,#248848,
#248849,#248850,#248851,#248852,#248853,#248854,#248855,#248856,#248857,
#248858,#248859,#248860,#248861,#248862,#248863,#248864,#248865,#248866,
#248867,#248868,#248869,#248870,#248871,#248872,#248873,#248874,#248875,
#248876,#248877,#248878,#248879,#248880,#248881,#248882,#248883,#248884,
#248885,#248886,#248887,#248888,#248889,#248890,#248891,#248892,#248893,
#248894,#248895,#248896,#248897,#248898,#248899,#248900,#248901,#248902,
#248903,#248904,#248905,#248906,#248907,#248908,#248909,#248910,#248911,
#248912,#248913,#248914,#248915,#248916,#248917,#248918,#248919,#248920,
#248921,#248922,#248923,#248924,#248925,#248926,#248927,#248928,#248929,
#248930,#248931,#248932,#248933,#248934,#248935,#248936,#248937,#248938,
#248939,#248940,#248941,#248942,#248943,#248944,#248945,#248946,#248947,
#248948,#248949,#248950,#248951,#248952,#248953,#248954,#248955,#248956,
#248957,#248958,#248959,#248960,#248961,#248962,#248963,#248964,#248965,
#248966,#248967,#248968,#248969,#248970,#248971,#248972,#248973,#248974,
#248975,#248976,#248977,#248978,#248979,#248980,#248981,#248982,#248983,
#248984,#248985,#248986,#248987,#248988,#248989,#248990,#248991,#248992,
#248993,#248994,#248995,#248996,#248997,#248998,#248999,#249000,#249001,
#249002,#249003,#249004,#249005,#249006,#249007,#249008,#249009,#249010,
#249011,#249012,#249013,#249014,#249015,#249016,#249017,#249018,#249019,
#249020,#249021,#249022,#249023,#249024,#249025,#249026,#249027,#249028,
#249029,#249030,#249031,#249032,#249033,#249034,#249035,#249036,#249037,
#249038,#249039,#249040,#249041,#249042,#249043,#249044,#249045,#249046,
#249047,#249048,#249049,#249050,#249051,#249052,#249053,#249054,#249055,
#249056,#249057,#249058,#249059,#249060,#249061,#249062,#249063,#249064,
#249065,#249066,#249067,#249068,#249069,#249070,#249071,#249072,#249073,
#249074,#249075,#249076,#249077,#249078,#249079,#249080,#249081,#249082,
#249083,#249084,#249085,#249086,#249087,#249088,#249089,#249090,#249091,
#249092,#249093,#249094,#249095,#249096,#249097,#249098,#249099,#249100,
#249101,#249102,#249103,#249104,#249105,#249106,#249107,#249108,#249109,
#249110,#249111,#249112,#249113,#249114,#249115),.UNSPECIFIED.,.F.,.F.,
(4,3,3,3,3,3,3,3,3,3,3,3,3,3,3,3,3,3,3,3,3,3,3,3,3,3,3,3,3,3,3,3,3,3,3,
3,3,3,3,3,3,3,3,3,3,3,3,3,3,3,3,3,3,3,3,3,3,3,3,3,3,3,3,3,3,3,3,3,3,3,3,
3,3,3,3,3,3,3,3,3,3,3,3,3,3,3,3,3,3,3,3,3,3,3,3,3,3,3,3,3,3,3,3,3,3,3,3,
3,4),(-1.,-0.994495413,-0.988990826,-0.983486239,-0.977981651,-0.970642202,
-0.965137615,-0.959633028,-0.95412844,-0.948623853,-0.943119266,-0.937614679,
-0.932110092,-0.926605505,-0.921100917,-0.91559633,-0.910091743,-0.904587156,
-0.899082569,-0.893577982,-0.886238532,-0.880733945,-0.875229358,-0.869724771,
-0.864220183,-0.858715596,-0.853211009,-0.847706422,-0.842201835,-0.836697248,
-0.831192661,-0.825688073,-0.818348624,-0.812844037,-0.80733945,-0.8,-0.79266055,
-0.785321101,-0.777981651,-0.770642202,-0.763302752,-0.755963303,-0.748623853,
-0.741284404,-0.733944954,-0.726605505,-0.719266055,-0.710091743,-0.702752294,
-0.695412844,-0.688073394,-0.678899083,-0.671559633,-0.664220183,-0.656880734,
-0.649541284,-0.642201835,-0.634862385,-0.627522936,-0.620183486,-0.612844037,
-0.605504587,-0.598165138,-0.590825688,-0.583486239,-0.576146789,-0.568807339,
-0.559633028,-0.552293578,-0.544954128,-0.537614679,-0.530275229,-0.521100917,
-0.511926606,-0.502752294,-0.493577982,-0.478899083,-0.469724771,-0.460550459,
-0.451376147,-0.442201835,-0.433027523,-0.423853211,-0.414678899,-0.405504587,
-0.396330275,-0.387155963,-0.374311927,-0.363302752,-0.352293578,-0.341284404,
-0.330275229,-0.319266055,-0.308256881,-0.297247706,-0.286238532,-0.275229358,
-0.264220183,-0.253211009,-0.242201835,-0.231192661,-0.220183486,-0.209174312,
-0.198165138,-0.187155963,-0.176146789,-0.165137615,-0.15412844,-0.143172102),
 .UNSPECIFIED.);
#24434=B_SPLINE_CURVE_WITH_KNOTS('',3,(#249116,#249117,#249118,#249119,
#249120,#249121,#249122,#249123,#249124,#249125,#249126,#249127,#249128,
#249129,#249130,#249131,#249132,#249133,#249134,#249135,#249136,#249137,
#249138,#249139,#249140,#249141,#249142,#249143,#249144,#249145,#249146,
#249147,#249148,#249149,#249150,#249151,#249152,#249153,#249154,#249155,
#249156,#249157,#249158,#249159,#249160,#249161,#249162,#249163,#249164,
#249165,#249166,#249167,#249168,#249169,#249170,#249171,#249172,#249173,
#249174,#249175,#249176,#249177,#249178,#249179,#249180,#249181,#249182,
#249183,#249184,#249185,#249186,#249187,#249188,#249189,#249190,#249191,
#249192,#249193,#249194,#249195,#249196,#249197,#249198,#249199,#249200,
#249201,#249202,#249203,#249204,#249205,#249206,#249207,#249208,#249209,
#249210,#249211,#249212,#249213,#249214,#249215,#249216,#249217,#249218,
#249219,#249220,#249221,#249222,#249223,#249224,#249225,#249226,#249227,
#249228,#249229,#249230,#249231,#249232,#249233,#249234,#249235,#249236,
#249237,#249238,#249239,#249240,#249241,#249242,#249243,#249244,#249245,
#249246,#249247,#249248,#249249,#249250,#249251,#249252,#249253,#249254,
#249255,#249256,#249257,#249258,#249259,#249260,#249261,#249262,#249263,
#249264,#249265,#249266,#249267,#249268,#249269,#249270,#249271,#249272,
#249273,#249274,#249275,#249276,#249277,#249278,#249279,#249280,#249281,
#249282,#249283,#249284,#249285,#249286,#249287,#249288,#249289,#249290,
#249291,#249292,#249293,#249294,#249295,#249296,#249297,#249298,#249299,
#249300,#249301,#249302,#249303,#249304,#249305,#249306,#249307,#249308,
#249309,#249310,#249311,#249312,#249313,#249314,#249315,#249316,#249317,
#249318,#249319,#249320,#249321,#249322,#249323,#249324,#249325,#249326,
#249327,#249328,#249329,#249330,#249331,#249332,#249333,#249334,#249335,
#249336,#249337,#249338,#249339,#249340,#249341,#249342,#249343,#249344,
#249345,#249346,#249347,#249348,#249349,#249350,#249351,#249352,#249353,
#249354,#249355,#249356,#249357,#249358,#249359,#249360,#249361,#249362,
#249363,#249364,#249365,#249366,#249367,#249368,#249369,#249370,#249371,
#249372,#249373,#249374,#249375,#249376,#249377,#249378,#249379,#249380,
#249381,#249382,#249383,#249384,#249385,#249386,#249387,#249388,#249389,
#249390,#249391,#249392,#249393,#249394,#249395,#249396,#249397,#249398,
#249399,#249400,#249401,#249402,#249403,#249404,#249405,#249406,#249407,
#249408,#249409,#249410,#249411,#249412,#249413,#249414,#249415,#249416,
#249417,#249418,#249419,#249420,#249421,#249422),.UNSPECIFIED.,.F.,.F.,
(4,3,3,3,3,3,3,3,3,3,3,3,3,3,3,3,3,3,3,3,3,3,3,3,3,3,3,3,3,3,3,3,3,3,3,
3,3,3,3,3,3,3,3,3,3,3,3,3,3,3,3,3,3,3,3,3,3,3,3,3,3,3,3,3,3,3,3,3,3,3,3,
3,3,3,3,3,3,3,3,3,3,3,3,3,3,3,3,3,3,3,3,3,3,3,3,3,3,3,3,3,3,3,4),(0.143172102,
0.15412844,0.165137615,0.176146789,0.187155963,0.198165138,0.209174312,
0.220183486,0.231192661,0.242201835,0.253211009,0.264220183,0.275229358,
0.288073394,0.299082569,0.310091743,0.32293578,0.333944954,0.344954128,
0.355963303,0.368807339,0.379816514,0.394495413,0.403669725,0.412844037,
0.422018349,0.433027523,0.442201835,0.451376147,0.462385321,0.471559633,
0.486238532,0.495412844,0.506422018,0.51559633,0.524770642,0.533944954,
0.544954128,0.55412844,0.563302752,0.570642202,0.577981651,0.585321101,
0.59266055,0.6,0.609174312,0.616513761,0.625688073,0.634862385,0.644036697,
0.651376147,0.658715596,0.667889908,0.67706422,0.68440367,0.691743119,0.699082569,
0.706422018,0.71559633,0.724770642,0.733944954,0.741284404,0.748623853,
0.755963303,0.763302752,0.770642202,0.777981651,0.785321101,0.79266055,
0.8,0.80733945,0.812844037,0.818348624,0.823853211,0.831192661,0.836697248,
0.842201835,0.847706422,0.853211009,0.858715596,0.864220183,0.869724771,
0.875229358,0.880733945,0.886238532,0.893577982,0.899082569,0.906422018,
0.911926606,0.919266055,0.924770642,0.930275229,0.935779817,0.943119266,
0.948623853,0.955963303,0.963302752,0.968807339,0.976146789,0.981651376,
0.988990826,0.994495413,1.),.UNSPECIFIED.);
#24435=B_SPLINE_CURVE_WITH_KNOTS('',3,(#250385,#250386,#250387,#250388,
#250389,#250390,#250391,#250392,#250393,#250394,#250395,#250396,#250397,
#250398,#250399,#250400,#250401,#250402,#250403,#250404,#250405,#250406,
#250407,#250408,#250409,#250410,#250411,#250412,#250413,#250414,#250415,
#250416,#250417,#250418,#250419,#250420,#250421,#250422,#250423,#250424,
#250425,#250426,#250427,#250428,#250429,#250430,#250431,#250432,#250433,
#250434,#250435,#250436,#250437,#250438,#250439,#250440,#250441,#250442,
#250443,#250444,#250445,#250446,#250447,#250448,#250449,#250450,#250451,
#250452,#250453,#250454,#250455,#250456,#250457,#250458,#250459,#250460,
#250461,#250462,#250463,#250464,#250465,#250466,#250467,#250468,#250469,
#250470,#250471,#250472,#250473,#250474,#250475,#250476,#250477,#250478,
#250479,#250480,#250481,#250482,#250483,#250484,#250485,#250486,#250487,
#250488,#250489,#250490,#250491,#250492,#250493,#250494,#250495,#250496,
#250497,#250498,#250499,#250500,#250501,#250502,#250503,#250504,#250505,
#250506,#250507,#250508,#250509,#250510,#250511,#250512,#250513,#250514,
#250515,#250516,#250517,#250518,#250519,#250520,#250521,#250522,#250523,
#250524,#250525,#250526,#250527,#250528,#250529,#250530,#250531,#250532,
#250533,#250534,#250535,#250536,#250537,#250538,#250539,#250540,#250541,
#250542,#250543,#250544,#250545,#250546,#250547,#250548,#250549,#250550,
#250551,#250552,#250553,#250554,#250555,#250556,#250557,#250558,#250559,
#250560,#250561,#250562,#250563,#250564,#250565,#250566,#250567,#250568,
#250569,#250570,#250571,#250572,#250573,#250574,#250575,#250576,#250577,
#250578,#250579,#250580,#250581,#250582,#250583,#250584,#250585,#250586,
#250587,#250588,#250589,#250590,#250591,#250592,#250593,#250594,#250595,
#250596,#250597,#250598,#250599,#250600,#250601,#250602,#250603,#250604,
#250605,#250606,#250607,#250608,#250609,#250610,#250611,#250612,#250613,
#250614,#250615,#250616,#250617,#250618,#250619,#250620,#250621,#250622,
#250623,#250624,#250625,#250626,#250627,#250628,#250629,#250630,#250631,
#250632,#250633,#250634,#250635,#250636,#250637,#250638,#250639,#250640,
#250641,#250642,#250643,#250644,#250645,#250646,#250647,#250648,#250649,
#250650,#250651,#250652,#250653,#250654,#250655,#250656,#250657,#250658,
#250659,#250660,#250661,#250662,#250663,#250664,#250665,#250666,#250667,
#250668,#250669,#250670,#250671,#250672,#250673,#250674,#250675,#250676,
#250677,#250678,#250679,#250680,#250681,#250682,#250683,#250684,#250685,
#250686,#250687,#250688,#250689,#250690,#250691,#250692,#250693,#250694,
#250695,#250696,#250697,#250698,#250699,#250700,#250701,#250702,#250703,
#250704,#250705,#250706,#250707,#250708,#250709,#250710,#250711,#250712),
 .UNSPECIFIED.,.F.,.F.,(4,3,3,3,3,3,3,3,3,3,3,3,3,3,3,3,3,3,3,3,3,3,3,3,
3,3,3,3,3,3,3,3,3,3,3,3,3,3,3,3,3,3,3,3,3,3,3,3,3,3,3,3,3,3,3,3,3,3,3,3,
3,3,3,3,3,3,3,3,3,3,3,3,3,3,3,3,3,3,3,3,3,3,3,3,3,3,3,3,3,3,3,3,3,3,3,3,
3,3,3,3,3,3,3,3,3,3,3,3,3,4),(-1.,-0.994495413,-0.988990826,-0.983486239,
-0.977981651,-0.972477064,-0.966972477,-0.96146789,-0.955963303,-0.950458716,
-0.944954128,-0.939449541,-0.932110092,-0.926605505,-0.921100917,-0.91559633,
-0.910091743,-0.904587156,-0.899082569,-0.893577982,-0.888073394,-0.882568807,
-0.87706422,-0.871559633,-0.866055046,-0.860550459,-0.855045872,-0.849541284,
-0.844036697,-0.83853211,-0.833027523,-0.827522936,-0.822018349,-0.814678899,
-0.809174312,-0.801834862,-0.794495413,-0.787155963,-0.779816514,-0.772477064,
-0.765137615,-0.757798165,-0.748623853,-0.741284404,-0.733944954,-0.726605505,
-0.719266055,-0.711926606,-0.704587156,-0.697247706,-0.689908257,-0.682568807,
-0.675229358,-0.667889908,-0.660550459,-0.653211009,-0.64587156,-0.63853211,
-0.631192661,-0.623853211,-0.616513761,-0.609174312,-0.601834862,-0.594495413,
-0.587155963,-0.579816514,-0.572477064,-0.565137615,-0.555963303,-0.548623853,
-0.541284404,-0.533944954,-0.526605505,-0.517431193,-0.508256881,-0.499082569,
-0.489908257,-0.480733945,-0.471559633,-0.462385321,-0.453211009,-0.442201835,
-0.433027523,-0.423853211,-0.414678899,-0.405504587,-0.396330275,-0.387155963,
-0.376146789,-0.365137615,-0.35412844,-0.343119266,-0.332110092,-0.321100917,
-0.308256881,-0.297247706,-0.286238532,-0.275229358,-0.264220183,-0.253211009,
-0.242201835,-0.231192661,-0.220183486,-0.209174312,-0.198165138,-0.187155963,
-0.176146789,-0.165137615,-0.15412844,-0.143172102),.UNSPECIFIED.);
#24436=B_SPLINE_CURVE_WITH_KNOTS('',3,(#250713,#250714,#250715,#250716,
#250717,#250718,#250719,#250720,#250721,#250722,#250723,#250724,#250725,
#250726,#250727,#250728,#250729,#250730,#250731,#250732,#250733,#250734,
#250735,#250736,#250737,#250738,#250739,#250740,#250741,#250742,#250743,
#250744,#250745,#250746,#250747,#250748,#250749,#250750,#250751,#250752,
#250753,#250754,#250755,#250756,#250757,#250758,#250759,#250760,#250761,
#250762,#250763,#250764,#250765,#250766,#250767,#250768,#250769,#250770,
#250771,#250772,#250773,#250774,#250775,#250776,#250777,#250778,#250779,
#250780,#250781,#250782,#250783,#250784,#250785,#250786,#250787,#250788,
#250789,#250790,#250791,#250792,#250793,#250794,#250795,#250796,#250797,
#250798,#250799,#250800,#250801,#250802,#250803,#250804,#250805,#250806,
#250807,#250808,#250809,#250810,#250811,#250812,#250813,#250814,#250815,
#250816,#250817,#250818,#250819,#250820,#250821,#250822,#250823,#250824,
#250825,#250826,#250827,#250828,#250829,#250830,#250831,#250832,#250833,
#250834,#250835,#250836,#250837,#250838,#250839,#250840,#250841,#250842,
#250843,#250844,#250845,#250846,#250847,#250848,#250849,#250850,#250851,
#250852,#250853,#250854,#250855,#250856,#250857,#250858,#250859,#250860,
#250861,#250862,#250863,#250864,#250865,#250866,#250867,#250868,#250869,
#250870,#250871,#250872,#250873,#250874,#250875,#250876,#250877,#250878,
#250879,#250880,#250881,#250882,#250883,#250884,#250885,#250886,#250887,
#250888,#250889,#250890,#250891,#250892,#250893,#250894,#250895,#250896,
#250897,#250898,#250899,#250900,#250901,#250902,#250903,#250904,#250905,
#250906,#250907,#250908,#250909,#250910,#250911,#250912,#250913,#250914,
#250915,#250916,#250917,#250918,#250919,#250920,#250921,#250922,#250923,
#250924,#250925,#250926,#250927,#250928,#250929,#250930,#250931,#250932,
#250933,#250934,#250935,#250936,#250937,#250938,#250939,#250940,#250941,
#250942,#250943,#250944,#250945,#250946,#250947,#250948,#250949,#250950,
#250951,#250952,#250953,#250954,#250955,#250956,#250957,#250958,#250959,
#250960,#250961,#250962,#250963,#250964,#250965,#250966,#250967,#250968,
#250969,#250970,#250971,#250972,#250973,#250974,#250975,#250976,#250977,
#250978,#250979,#250980,#250981,#250982,#250983,#250984,#250985,#250986,
#250987,#250988,#250989,#250990,#250991,#250992,#250993,#250994,#250995,
#250996,#250997,#250998,#250999,#251000,#251001,#251002,#251003,#251004,
#251005,#251006,#251007,#251008,#251009,#251010,#251011,#251012,#251013,
#251014,#251015,#251016,#251017,#251018,#251019,#251020,#251021,#251022),
 .UNSPECIFIED.,.F.,.F.,(4,3,3,3,3,3,3,3,3,3,3,3,3,3,3,3,3,3,3,3,3,3,3,3,
3,3,3,3,3,3,3,3,3,3,3,3,3,3,3,3,3,3,3,3,3,3,3,3,3,3,3,3,3,3,3,3,3,3,3,3,
3,3,3,3,3,3,3,3,3,3,3,3,3,3,3,3,3,3,3,3,3,3,3,3,3,3,3,3,3,3,3,3,3,3,3,3,
3,3,3,3,3,3,3,4),(0.143172102,0.15412844,0.165137615,0.176146789,0.187155963,
0.198165138,0.211009174,0.222018349,0.233027523,0.244036697,0.255045872,
0.266055046,0.27706422,0.288073394,0.299082569,0.310091743,0.321100917,
0.332110092,0.343119266,0.35412844,0.365137615,0.376146789,0.387155963,
0.396330275,0.405504587,0.414678899,0.423853211,0.433027523,0.44587156,
0.455045872,0.464220183,0.473394495,0.482568807,0.491743119,0.500917431,
0.510091743,0.519266055,0.528440367,0.535779817,0.543119266,0.550458716,
0.557798165,0.568807339,0.576146789,0.583486239,0.594495413,0.601834862,
0.611009174,0.618348624,0.625688073,0.633027523,0.640366972,0.647706422,
0.656880734,0.666055046,0.673394495,0.686238532,0.697247706,0.706422018,
0.713761468,0.721100917,0.732110092,0.739449541,0.748623853,0.755963303,
0.763302752,0.770642202,0.777981651,0.787155963,0.794495413,0.801834862,
0.812844037,0.818348624,0.823853211,0.829357798,0.836697248,0.842201835,
0.847706422,0.853211009,0.858715596,0.864220183,0.869724771,0.875229358,
0.880733945,0.888073394,0.893577982,0.899082569,0.904587156,0.910091743,
0.91559633,0.921100917,0.926605505,0.932110092,0.937614679,0.943119266,
0.952293578,0.957798165,0.963302752,0.968807339,0.974311927,0.979816514,
0.985321101,0.99266055,1.),.UNSPECIFIED.);
#24437=B_SPLINE_CURVE_WITH_KNOTS('',3,(#251967,#251968,#251969,#251970,
#251971,#251972,#251973,#251974,#251975,#251976,#251977,#251978,#251979,
#251980,#251981,#251982,#251983,#251984,#251985,#251986,#251987,#251988,
#251989,#251990,#251991,#251992,#251993,#251994,#251995,#251996,#251997,
#251998,#251999,#252000,#252001,#252002,#252003,#252004,#252005,#252006,
#252007,#252008,#252009,#252010,#252011,#252012,#252013,#252014,#252015,
#252016,#252017,#252018,#252019,#252020,#252021,#252022,#252023,#252024,
#252025,#252026,#252027,#252028,#252029,#252030,#252031,#252032,#252033,
#252034,#252035,#252036,#252037,#252038,#252039,#252040,#252041,#252042,
#252043,#252044,#252045,#252046,#252047,#252048,#252049,#252050,#252051,
#252052,#252053,#252054,#252055,#252056,#252057,#252058,#252059,#252060,
#252061,#252062,#252063,#252064,#252065,#252066,#252067,#252068,#252069,
#252070,#252071,#252072,#252073,#252074,#252075,#252076,#252077,#252078,
#252079,#252080,#252081,#252082,#252083,#252084,#252085,#252086,#252087,
#252088,#252089,#252090,#252091,#252092,#252093,#252094,#252095,#252096,
#252097,#252098,#252099,#252100,#252101,#252102,#252103,#252104,#252105,
#252106,#252107,#252108,#252109,#252110,#252111,#252112,#252113,#252114,
#252115,#252116,#252117,#252118,#252119,#252120,#252121,#252122,#252123,
#252124,#252125,#252126,#252127,#252128,#252129,#252130,#252131,#252132,
#252133,#252134,#252135,#252136,#252137,#252138,#252139,#252140,#252141,
#252142,#252143,#252144,#252145,#252146,#252147,#252148,#252149,#252150,
#252151,#252152,#252153,#252154,#252155,#252156,#252157,#252158,#252159,
#252160,#252161,#252162,#252163,#252164,#252165,#252166,#252167,#252168,
#252169,#252170,#252171,#252172,#252173,#252174,#252175,#252176,#252177,
#252178,#252179,#252180,#252181,#252182,#252183,#252184,#252185,#252186,
#252187,#252188,#252189,#252190,#252191,#252192,#252193,#252194,#252195,
#252196,#252197,#252198,#252199,#252200,#252201,#252202,#252203,#252204,
#252205,#252206,#252207,#252208,#252209,#252210,#252211,#252212,#252213,
#252214,#252215,#252216,#252217,#252218,#252219,#252220,#252221,#252222,
#252223,#252224,#252225,#252226,#252227,#252228,#252229,#252230,#252231,
#252232,#252233,#252234,#252235,#252236,#252237,#252238,#252239,#252240,
#252241,#252242,#252243,#252244,#252245,#252246,#252247,#252248,#252249,
#252250,#252251,#252252,#252253,#252254,#252255,#252256,#252257,#252258,
#252259,#252260,#252261,#252262,#252263,#252264,#252265,#252266,#252267,
#252268,#252269,#252270,#252271,#252272,#252273),.UNSPECIFIED.,.F.,.F.,
(4,3,3,3,3,3,3,3,3,3,3,3,3,3,3,3,3,3,3,3,3,3,3,3,3,3,3,3,3,3,3,3,3,3,3,
3,3,3,3,3,3,3,3,3,3,3,3,3,3,3,3,3,3,3,3,3,3,3,3,3,3,3,3,3,3,3,3,3,3,3,3,
3,3,3,3,3,3,3,3,3,3,3,3,3,3,3,3,3,3,3,3,3,3,3,3,3,3,3,3,3,3,3,4),(0.143172102,
0.15412844,0.165137615,0.176146789,0.187155963,0.198165138,0.209174312,
0.220183486,0.231192661,0.242201835,0.253211009,0.264220183,0.27706422,
0.288073394,0.299082569,0.310091743,0.321100917,0.332110092,0.343119266,
0.35412844,0.366972477,0.377981651,0.388990826,0.398165138,0.40733945,0.416513761,
0.425688073,0.434862385,0.444036697,0.456880734,0.466055046,0.475229358,
0.48440367,0.493577982,0.502752294,0.511926606,0.521100917,0.530275229,
0.537614679,0.544954128,0.55412844,0.56146789,0.570642202,0.577981651,0.585321101,
0.594495413,0.601834862,0.612844037,0.620183486,0.629357798,0.63853211,
0.649541284,0.656880734,0.664220183,0.671559633,0.678899083,0.686238532,
0.693577982,0.700917431,0.708256881,0.71559633,0.72293578,0.732110092,0.739449541,
0.746788991,0.75412844,0.76146789,0.768807339,0.776146789,0.785321101,0.79266055,
0.801834862,0.811009174,0.816513761,0.822018349,0.831192661,0.836697248,
0.844036697,0.849541284,0.855045872,0.862385321,0.871559633,0.87706422,
0.882568807,0.891743119,0.897247706,0.902752294,0.908256881,0.913761468,
0.921100917,0.926605505,0.932110092,0.937614679,0.943119266,0.950458716,
0.955963303,0.96146789,0.966972477,0.974311927,0.979816514,0.985321101,
0.994495413,1.),.UNSPECIFIED.);
#24438=B_SPLINE_CURVE_WITH_KNOTS('',3,(#252274,#252275,#252276,#252277,
#252278,#252279,#252280,#252281,#252282,#252283,#252284,#252285,#252286,
#252287,#252288,#252289,#252290,#252291,#252292,#252293,#252294,#252295,
#252296,#252297,#252298,#252299,#252300,#252301,#252302,#252303,#252304,
#252305,#252306,#252307,#252308,#252309,#252310,#252311,#252312,#252313,
#252314,#252315,#252316,#252317,#252318,#252319,#252320,#252321,#252322,
#252323,#252324,#252325,#252326,#252327,#252328,#252329,#252330,#252331,
#252332,#252333,#252334,#252335,#252336,#252337,#252338,#252339,#252340,
#252341,#252342,#252343,#252344,#252345,#252346,#252347,#252348,#252349,
#252350,#252351,#252352,#252353,#252354,#252355,#252356,#252357,#252358,
#252359,#252360,#252361,#252362,#252363,#252364,#252365,#252366,#252367,
#252368,#252369,#252370,#252371,#252372,#252373,#252374,#252375,#252376,
#252377,#252378,#252379,#252380,#252381,#252382,#252383,#252384,#252385,
#252386,#252387,#252388,#252389,#252390,#252391,#252392,#252393,#252394,
#252395,#252396,#252397,#252398,#252399,#252400,#252401,#252402,#252403,
#252404,#252405,#252406,#252407,#252408,#252409,#252410,#252411,#252412,
#252413,#252414,#252415,#252416,#252417,#252418,#252419,#252420,#252421,
#252422,#252423,#252424,#252425,#252426,#252427,#252428,#252429,#252430,
#252431,#252432,#252433,#252434,#252435,#252436,#252437,#252438,#252439,
#252440,#252441,#252442,#252443,#252444,#252445,#252446,#252447,#252448,
#252449,#252450,#252451,#252452,#252453,#252454,#252455,#252456,#252457,
#252458,#252459,#252460,#252461,#252462,#252463,#252464,#252465,#252466,
#252467,#252468,#252469,#252470,#252471,#252472,#252473,#252474,#252475,
#252476,#252477,#252478,#252479,#252480,#252481,#252482,#252483,#252484,
#252485,#252486,#252487,#252488,#252489,#252490,#252491,#252492,#252493,
#252494,#252495,#252496,#252497,#252498,#252499,#252500,#252501,#252502,
#252503,#252504,#252505,#252506,#252507,#252508,#252509,#252510,#252511,
#252512,#252513,#252514,#252515,#252516,#252517,#252518,#252519,#252520,
#252521,#252522,#252523,#252524,#252525,#252526,#252527,#252528,#252529,
#252530,#252531,#252532,#252533,#252534,#252535,#252536,#252537,#252538,
#252539,#252540,#252541,#252542,#252543,#252544,#252545,#252546,#252547,
#252548,#252549,#252550,#252551,#252552,#252553,#252554,#252555,#252556,
#252557,#252558,#252559,#252560,#252561,#252562,#252563,#252564,#252565,
#252566,#252567,#252568,#252569,#252570,#252571,#252572,#252573,#252574,
#252575,#252576,#252577,#252578,#252579,#252580,#252581,#252582,#252583,
#252584,#252585,#252586,#252587,#252588,#252589,#252590,#252591,#252592,
#252593,#252594,#252595),.UNSPECIFIED.,.F.,.F.,(4,3,3,3,3,3,3,3,3,3,3,3,
3,3,3,3,3,3,3,3,3,3,3,3,3,3,3,3,3,3,3,3,3,3,3,3,3,3,3,3,3,3,3,3,3,3,3,3,
3,3,3,3,3,3,3,3,3,3,3,3,3,3,3,3,3,3,3,3,3,3,3,3,3,3,3,3,3,3,3,3,3,3,3,3,
3,3,3,3,3,3,3,3,3,3,3,3,3,3,3,3,3,3,3,3,3,3,3,4),(0.143172102,0.15412844,
0.165137615,0.176146789,0.187155963,0.198165138,0.209174312,0.220183486,
0.231192661,0.242201835,0.253211009,0.264220183,0.27706422,0.288073394,
0.299082569,0.310091743,0.321100917,0.332110092,0.343119266,0.35412844,
0.365137615,0.376146789,0.387155963,0.396330275,0.405504587,0.414678899,
0.423853211,0.433027523,0.442201835,0.451376147,0.460550459,0.469724771,
0.478899083,0.489908257,0.499082569,0.510091743,0.519266055,0.528440367,
0.535779817,0.544954128,0.552293578,0.559633028,0.566972477,0.574311927,
0.581651376,0.588990826,0.596330275,0.603669725,0.611009174,0.618348624,
0.625688073,0.633027523,0.640366972,0.647706422,0.655045872,0.664220183,
0.671559633,0.678899083,0.686238532,0.693577982,0.700917431,0.708256881,
0.71559633,0.72293578,0.732110092,0.739449541,0.746788991,0.75412844,0.76146789,
0.768807339,0.776146789,0.783486239,0.790825688,0.798165138,0.805504587,
0.811009174,0.816513761,0.822018349,0.827522936,0.833027523,0.842201835,
0.849541284,0.855045872,0.860550459,0.866055046,0.871559633,0.87706422,
0.882568807,0.888073394,0.893577982,0.900917431,0.906422018,0.911926606,
0.917431193,0.924770642,0.930275229,0.935779817,0.941284404,0.946788991,
0.95412844,0.959633028,0.965137615,0.972477064,0.977981651,0.983486239,
0.988990826,0.994495413,1.),.UNSPECIFIED.);
#24439=B_SPLINE_CURVE_WITH_KNOTS('',3,(#253555,#253556,#253557,#253558,
#253559,#253560,#253561,#253562,#253563,#253564,#253565,#253566,#253567,
#253568,#253569,#253570,#253571,#253572,#253573,#253574,#253575,#253576,
#253577,#253578,#253579,#253580,#253581,#253582,#253583,#253584,#253585,
#253586,#253587,#253588,#253589,#253590,#253591,#253592,#253593,#253594,
#253595,#253596,#253597,#253598,#253599,#253600,#253601,#253602,#253603,
#253604,#253605,#253606,#253607,#253608,#253609,#253610,#253611,#253612,
#253613,#253614,#253615,#253616,#253617,#253618,#253619,#253620,#253621,
#253622,#253623,#253624,#253625,#253626,#253627,#253628,#253629,#253630,
#253631,#253632,#253633,#253634,#253635,#253636,#253637,#253638,#253639,
#253640,#253641,#253642,#253643,#253644,#253645,#253646,#253647,#253648,
#253649,#253650,#253651,#253652,#253653,#253654,#253655,#253656,#253657,
#253658,#253659,#253660,#253661,#253662,#253663,#253664,#253665,#253666,
#253667,#253668,#253669,#253670,#253671,#253672,#253673,#253674,#253675,
#253676,#253677,#253678,#253679,#253680,#253681,#253682,#253683,#253684,
#253685,#253686,#253687,#253688,#253689,#253690,#253691,#253692,#253693,
#253694,#253695,#253696,#253697,#253698,#253699,#253700,#253701,#253702,
#253703,#253704,#253705,#253706,#253707,#253708,#253709,#253710,#253711,
#253712,#253713,#253714,#253715,#253716,#253717,#253718,#253719,#253720,
#253721,#253722,#253723,#253724,#253725,#253726,#253727,#253728,#253729,
#253730,#253731,#253732,#253733,#253734,#253735,#253736,#253737,#253738,
#253739,#253740,#253741,#253742,#253743,#253744,#253745,#253746,#253747,
#253748,#253749,#253750,#253751,#253752,#253753,#253754,#253755,#253756,
#253757,#253758,#253759,#253760,#253761,#253762,#253763,#253764,#253765,
#253766,#253767,#253768,#253769,#253770,#253771,#253772,#253773,#253774,
#253775,#253776,#253777,#253778,#253779,#253780,#253781,#253782,#253783,
#253784,#253785,#253786,#253787,#253788,#253789,#253790,#253791,#253792,
#253793,#253794,#253795,#253796,#253797,#253798,#253799,#253800,#253801,
#253802,#253803,#253804,#253805,#253806,#253807,#253808,#253809,#253810,
#253811,#253812,#253813,#253814,#253815,#253816,#253817,#253818,#253819,
#253820,#253821,#253822,#253823,#253824,#253825,#253826,#253827,#253828,
#253829,#253830,#253831,#253832,#253833,#253834,#253835,#253836,#253837,
#253838,#253839,#253840,#253841,#253842,#253843,#253844,#253845,#253846),
 .UNSPECIFIED.,.F.,.F.,(4,3,3,3,3,3,3,3,3,3,3,3,3,3,3,3,3,3,3,3,3,3,3,3,
3,3,3,3,3,3,3,3,3,3,3,3,3,3,3,3,3,3,3,3,3,3,3,3,3,3,3,3,3,3,3,3,3,3,3,3,
3,3,3,3,3,3,3,3,3,3,3,3,3,3,3,3,3,3,3,3,3,3,3,3,3,3,3,3,3,3,3,3,3,3,3,3,
3,4),(0.143172102,0.15412844,0.165137615,0.176146789,0.187155963,0.198165138,
0.209174312,0.220183486,0.231192661,0.242201835,0.253211009,0.264220183,
0.275229358,0.286238532,0.297247706,0.308256881,0.319266055,0.330275229,
0.341284404,0.352293578,0.363302752,0.376146789,0.388990826,0.398165138,
0.40733945,0.416513761,0.425688073,0.434862385,0.444036697,0.453211009,
0.462385321,0.475229358,0.48440367,0.495412844,0.506422018,0.51559633,0.524770642,
0.533944954,0.541284404,0.548623853,0.555963303,0.563302752,0.570642202,
0.577981651,0.590825688,0.598165138,0.605504587,0.618348624,0.625688073,
0.634862385,0.642201835,0.651376147,0.664220183,0.675229358,0.682568807,
0.691743119,0.699082569,0.706422018,0.717431193,0.724770642,0.735779817,
0.743119266,0.752293578,0.759633028,0.768807339,0.781651376,0.788990826,
0.796330275,0.80733945,0.812844037,0.818348624,0.823853211,0.829357798,
0.83853211,0.84587156,0.851376147,0.860550459,0.867889908,0.87706422,0.882568807,
0.889908257,0.895412844,0.900917431,0.910091743,0.919266055,0.926605505,
0.933944954,0.939449541,0.944954128,0.950458716,0.955963303,0.963302752,
0.968807339,0.974311927,0.981651376,0.987155963,0.994495413,1.),
 .UNSPECIFIED.);
#24440=B_SPLINE_CURVE_WITH_KNOTS('',3,(#253847,#253848,#253849,#253850,
#253851,#253852,#253853,#253854,#253855,#253856,#253857,#253858,#253859,
#253860,#253861,#253862,#253863,#253864,#253865,#253866,#253867,#253868,
#253869,#253870,#253871,#253872,#253873,#253874,#253875,#253876,#253877,
#253878,#253879,#253880,#253881,#253882,#253883,#253884,#253885,#253886,
#253887,#253888,#253889,#253890,#253891,#253892,#253893,#253894,#253895,
#253896,#253897,#253898,#253899,#253900,#253901,#253902,#253903,#253904,
#253905,#253906,#253907,#253908,#253909,#253910,#253911,#253912,#253913,
#253914,#253915,#253916,#253917,#253918,#253919,#253920,#253921,#253922,
#253923,#253924,#253925,#253926,#253927,#253928,#253929,#253930,#253931,
#253932,#253933,#253934,#253935,#253936,#253937,#253938,#253939,#253940,
#253941,#253942,#253943,#253944,#253945,#253946,#253947,#253948,#253949,
#253950,#253951,#253952,#253953,#253954,#253955,#253956,#253957,#253958,
#253959,#253960,#253961,#253962,#253963,#253964,#253965,#253966,#253967,
#253968,#253969,#253970,#253971,#253972,#253973,#253974,#253975,#253976,
#253977,#253978,#253979,#253980,#253981,#253982,#253983,#253984,#253985,
#253986,#253987,#253988,#253989,#253990,#253991,#253992,#253993,#253994,
#253995,#253996,#253997,#253998,#253999,#254000,#254001,#254002,#254003,
#254004,#254005,#254006,#254007,#254008,#254009,#254010,#254011,#254012,
#254013,#254014,#254015,#254016,#254017,#254018,#254019,#254020,#254021,
#254022,#254023,#254024,#254025,#254026,#254027,#254028,#254029,#254030,
#254031,#254032,#254033,#254034,#254035,#254036,#254037,#254038,#254039,
#254040,#254041,#254042,#254043,#254044,#254045,#254046,#254047,#254048,
#254049,#254050,#254051,#254052,#254053,#254054,#254055,#254056,#254057,
#254058,#254059,#254060,#254061,#254062,#254063,#254064,#254065,#254066,
#254067,#254068,#254069,#254070,#254071,#254072,#254073,#254074,#254075,
#254076,#254077,#254078,#254079,#254080,#254081,#254082,#254083,#254084,
#254085,#254086,#254087,#254088,#254089,#254090,#254091,#254092,#254093,
#254094,#254095,#254096,#254097,#254098,#254099,#254100,#254101,#254102,
#254103,#254104,#254105,#254106,#254107,#254108,#254109,#254110,#254111,
#254112,#254113,#254114,#254115,#254116,#254117,#254118,#254119,#254120,
#254121,#254122,#254123,#254124,#254125,#254126,#254127,#254128,#254129,
#254130,#254131,#254132,#254133,#254134,#254135,#254136,#254137,#254138,
#254139,#254140,#254141,#254142,#254143,#254144,#254145,#254146,#254147,
#254148,#254149,#254150,#254151,#254152,#254153,#254154,#254155,#254156,
#254157,#254158,#254159,#254160,#254161,#254162,#254163,#254164,#254165),
 .UNSPECIFIED.,.F.,.F.,(4,3,3,3,3,3,3,3,3,3,3,3,3,3,3,3,3,3,3,3,3,3,3,3,
3,3,3,3,3,3,3,3,3,3,3,3,3,3,3,3,3,3,3,3,3,3,3,3,3,3,3,3,3,3,3,3,3,3,3,3,
3,3,3,3,3,3,3,3,3,3,3,3,3,3,3,3,3,3,3,3,3,3,3,3,3,3,3,3,3,3,3,3,3,3,3,3,
3,3,3,3,3,3,3,3,3,3,4),(0.143172102,0.15412844,0.165137615,0.176146789,
0.187155963,0.198165138,0.209174312,0.220183486,0.231192661,0.242201835,
0.253211009,0.266055046,0.27706422,0.288073394,0.300917431,0.311926606,
0.32293578,0.333944954,0.344954128,0.355963303,0.366972477,0.377981651,
0.390825688,0.4,0.409174312,0.418348624,0.429357798,0.43853211,0.447706422,
0.456880734,0.466055046,0.475229358,0.48440367,0.493577982,0.502752294,
0.511926606,0.521100917,0.530275229,0.537614679,0.544954128,0.552293578,
0.559633028,0.566972477,0.574311927,0.581651376,0.588990826,0.596330275,
0.603669725,0.611009174,0.618348624,0.625688073,0.633027523,0.640366972,
0.647706422,0.655045872,0.662385321,0.671559633,0.678899083,0.686238532,
0.693577982,0.700917431,0.708256881,0.71559633,0.72293578,0.730275229,0.737614679,
0.744954128,0.752293578,0.759633028,0.766972477,0.774311927,0.781651376,
0.788990826,0.796330275,0.805504587,0.811009174,0.816513761,0.822018349,
0.827522936,0.834862385,0.840366972,0.84587156,0.853211009,0.858715596,
0.864220183,0.869724771,0.875229358,0.882568807,0.888073394,0.893577982,
0.900917431,0.906422018,0.911926606,0.917431193,0.924770642,0.930275229,
0.935779817,0.941284404,0.946788991,0.95412844,0.959633028,0.968807339,
0.976146789,0.981651376,0.987155963,0.99266055,1.),.UNSPECIFIED.);
#24441=B_SPLINE_CURVE_WITH_KNOTS('',3,(#255113,#255114,#255115,#255116,
#255117,#255118,#255119,#255120,#255121,#255122,#255123,#255124,#255125,
#255126,#255127,#255128,#255129,#255130,#255131,#255132,#255133,#255134,
#255135,#255136,#255137,#255138,#255139,#255140,#255141,#255142,#255143,
#255144,#255145,#255146,#255147,#255148,#255149,#255150,#255151,#255152,
#255153,#255154,#255155,#255156,#255157,#255158,#255159,#255160,#255161,
#255162,#255163,#255164,#255165,#255166,#255167,#255168,#255169,#255170,
#255171,#255172,#255173,#255174,#255175,#255176,#255177,#255178,#255179,
#255180,#255181,#255182,#255183,#255184,#255185,#255186,#255187,#255188,
#255189,#255190,#255191,#255192,#255193,#255194,#255195,#255196,#255197,
#255198,#255199,#255200,#255201,#255202,#255203,#255204,#255205,#255206,
#255207,#255208,#255209,#255210,#255211,#255212,#255213,#255214,#255215,
#255216,#255217,#255218,#255219,#255220,#255221,#255222,#255223,#255224,
#255225,#255226,#255227,#255228,#255229,#255230,#255231,#255232,#255233,
#255234,#255235,#255236,#255237,#255238,#255239,#255240,#255241,#255242,
#255243,#255244,#255245,#255246,#255247,#255248,#255249,#255250,#255251,
#255252,#255253,#255254,#255255,#255256,#255257,#255258,#255259,#255260,
#255261,#255262,#255263,#255264,#255265,#255266,#255267,#255268,#255269,
#255270,#255271,#255272,#255273,#255274,#255275,#255276,#255277,#255278,
#255279,#255280,#255281,#255282,#255283,#255284,#255285,#255286,#255287,
#255288,#255289,#255290,#255291,#255292,#255293,#255294,#255295,#255296,
#255297,#255298,#255299,#255300,#255301,#255302,#255303,#255304,#255305,
#255306,#255307,#255308,#255309,#255310,#255311,#255312,#255313,#255314,
#255315,#255316,#255317,#255318,#255319,#255320,#255321,#255322,#255323,
#255324,#255325,#255326,#255327,#255328,#255329,#255330,#255331,#255332,
#255333,#255334,#255335,#255336,#255337,#255338,#255339,#255340,#255341,
#255342,#255343,#255344,#255345,#255346,#255347,#255348,#255349,#255350,
#255351,#255352,#255353,#255354,#255355,#255356,#255357,#255358,#255359,
#255360,#255361,#255362,#255363,#255364,#255365,#255366,#255367,#255368,
#255369,#255370,#255371,#255372,#255373,#255374,#255375,#255376,#255377,
#255378,#255379,#255380,#255381,#255382,#255383,#255384,#255385,#255386,
#255387,#255388,#255389,#255390,#255391,#255392,#255393,#255394,#255395,
#255396,#255397,#255398,#255399,#255400,#255401,#255402,#255403,#255404,
#255405,#255406,#255407,#255408,#255409,#255410,#255411,#255412,#255413,
#255414,#255415,#255416,#255417,#255418,#255419,#255420,#255421,#255422,
#255423,#255424,#255425,#255426,#255427,#255428,#255429,#255430,#255431,
#255432,#255433,#255434),.UNSPECIFIED.,.F.,.F.,(4,3,3,3,3,3,3,3,3,3,3,3,
3,3,3,3,3,3,3,3,3,3,3,3,3,3,3,3,3,3,3,3,3,3,3,3,3,3,3,3,3,3,3,3,3,3,3,3,
3,3,3,3,3,3,3,3,3,3,3,3,3,3,3,3,3,3,3,3,3,3,3,3,3,3,3,3,3,3,3,3,3,3,3,3,
3,3,3,3,3,3,3,3,3,3,3,3,3,3,3,3,3,3,3,3,3,3,3,4),(-1.,-0.994495413,-0.988990826,
-0.983486239,-0.977981651,-0.972477064,-0.966972477,-0.959633028,-0.95412844,
-0.948623853,-0.943119266,-0.937614679,-0.932110092,-0.926605505,-0.919266055,
-0.913761468,-0.908256881,-0.902752294,-0.897247706,-0.891743119,-0.886238532,
-0.880733945,-0.875229358,-0.867889908,-0.860550459,-0.855045872,-0.849541284,
-0.844036697,-0.83853211,-0.833027523,-0.827522936,-0.822018349,-0.814678899,
-0.809174312,-0.801834862,-0.794495413,-0.787155963,-0.779816514,-0.772477064,
-0.765137615,-0.757798165,-0.750458716,-0.743119266,-0.735779817,-0.728440367,
-0.721100917,-0.711926606,-0.704587156,-0.697247706,-0.689908257,-0.682568807,
-0.675229358,-0.667889908,-0.660550459,-0.653211009,-0.644036697,-0.636697248,
-0.629357798,-0.622018349,-0.614678899,-0.60733945,-0.6,-0.59266055,-0.585321101,
-0.577981651,-0.570642202,-0.563302752,-0.555963303,-0.548623853,-0.541284404,
-0.533944954,-0.524770642,-0.513761468,-0.504587156,-0.495412844,-0.486238532,
-0.47706422,-0.467889908,-0.458715596,-0.449541284,-0.440366972,-0.431192661,
-0.422018349,-0.412844037,-0.403669725,-0.39266055,-0.381651376,-0.370642202,
-0.359633028,-0.348623853,-0.337614679,-0.326605505,-0.31559633,-0.304587156,
-0.291743119,-0.278899083,-0.267889908,-0.256880734,-0.24587156,-0.234862385,
-0.223853211,-0.212844037,-0.201834862,-0.190825688,-0.179816514,-0.168807339,
-0.157798165,-0.143172102),.UNSPECIFIED.);
#24442=B_SPLINE_CURVE_WITH_KNOTS('',3,(#255435,#255436,#255437,#255438,
#255439,#255440,#255441,#255442,#255443,#255444,#255445,#255446,#255447,
#255448,#255449,#255450,#255451,#255452,#255453,#255454,#255455,#255456,
#255457,#255458,#255459,#255460,#255461,#255462,#255463,#255464,#255465,
#255466,#255467,#255468,#255469,#255470,#255471,#255472,#255473,#255474,
#255475,#255476,#255477,#255478,#255479,#255480,#255481,#255482,#255483,
#255484,#255485,#255486,#255487,#255488,#255489,#255490,#255491,#255492,
#255493,#255494,#255495,#255496,#255497,#255498,#255499,#255500,#255501,
#255502,#255503,#255504,#255505,#255506,#255507,#255508,#255509,#255510,
#255511,#255512,#255513,#255514,#255515,#255516,#255517,#255518,#255519,
#255520,#255521,#255522,#255523,#255524,#255525,#255526,#255527,#255528,
#255529,#255530,#255531,#255532,#255533,#255534,#255535,#255536,#255537,
#255538,#255539,#255540,#255541,#255542,#255543,#255544,#255545,#255546,
#255547,#255548,#255549,#255550,#255551,#255552,#255553,#255554,#255555,
#255556,#255557,#255558,#255559,#255560,#255561,#255562,#255563,#255564,
#255565,#255566,#255567,#255568,#255569,#255570,#255571,#255572,#255573,
#255574,#255575,#255576,#255577,#255578,#255579,#255580,#255581,#255582,
#255583,#255584,#255585,#255586,#255587,#255588,#255589,#255590,#255591,
#255592,#255593,#255594,#255595,#255596,#255597,#255598,#255599,#255600,
#255601,#255602,#255603,#255604,#255605,#255606,#255607,#255608,#255609,
#255610,#255611,#255612,#255613,#255614,#255615,#255616,#255617,#255618,
#255619,#255620,#255621,#255622,#255623,#255624,#255625,#255626,#255627,
#255628,#255629,#255630,#255631,#255632,#255633,#255634,#255635,#255636,
#255637,#255638,#255639,#255640,#255641,#255642,#255643,#255644,#255645,
#255646,#255647,#255648,#255649,#255650,#255651,#255652,#255653,#255654,
#255655,#255656,#255657,#255658,#255659,#255660,#255661,#255662,#255663,
#255664,#255665,#255666,#255667,#255668,#255669,#255670,#255671,#255672,
#255673,#255674,#255675,#255676,#255677,#255678,#255679,#255680,#255681,
#255682,#255683,#255684,#255685,#255686,#255687,#255688,#255689,#255690,
#255691,#255692,#255693,#255694,#255695,#255696,#255697,#255698,#255699,
#255700,#255701,#255702,#255703,#255704,#255705,#255706,#255707,#255708,
#255709,#255710,#255711,#255712,#255713,#255714,#255715,#255716,#255717,
#255718,#255719,#255720,#255721,#255722,#255723,#255724,#255725,#255726,
#255727,#255728,#255729,#255730,#255731,#255732,#255733,#255734,#255735,
#255736,#255737,#255738,#255739,#255740,#255741,#255742,#255743,#255744,
#255745,#255746,#255747),.UNSPECIFIED.,.F.,.F.,(4,3,3,3,3,3,3,3,3,3,3,3,
3,3,3,3,3,3,3,3,3,3,3,3,3,3,3,3,3,3,3,3,3,3,3,3,3,3,3,3,3,3,3,3,3,3,3,3,
3,3,3,3,3,3,3,3,3,3,3,3,3,3,3,3,3,3,3,3,3,3,3,3,3,3,3,3,3,3,3,3,3,3,3,3,
3,3,3,3,3,3,3,3,3,3,3,3,3,3,3,3,3,3,3,3,4),(0.143172102,0.15412844,0.165137615,
0.176146789,0.187155963,0.198165138,0.211009174,0.222018349,0.233027523,
0.244036697,0.255045872,0.266055046,0.27706422,0.288073394,0.299082569,
0.310091743,0.321100917,0.332110092,0.343119266,0.35412844,0.365137615,
0.376146789,0.387155963,0.396330275,0.405504587,0.414678899,0.423853211,
0.433027523,0.442201835,0.451376147,0.460550459,0.469724771,0.478899083,
0.488073394,0.497247706,0.506422018,0.519266055,0.528440367,0.537614679,
0.544954128,0.55412844,0.56146789,0.568807339,0.576146789,0.583486239,0.590825688,
0.598165138,0.605504587,0.612844037,0.620183486,0.627522936,0.63853211,
0.647706422,0.655045872,0.666055046,0.673394495,0.680733945,0.688073394,
0.695412844,0.702752294,0.710091743,0.719266055,0.726605505,0.733944954,
0.741284404,0.748623853,0.755963303,0.763302752,0.770642202,0.777981651,
0.787155963,0.794495413,0.801834862,0.809174312,0.818348624,0.823853211,
0.829357798,0.834862385,0.840366972,0.847706422,0.853211009,0.858715596,
0.864220183,0.873394495,0.878899083,0.888073394,0.893577982,0.899082569,
0.906422018,0.911926606,0.917431193,0.92293578,0.928440367,0.937614679,
0.943119266,0.948623853,0.95412844,0.959633028,0.966972477,0.972477064,
0.977981651,0.983486239,0.988990826,0.994495413,1.),.UNSPECIFIED.);
#24443=B_SPLINE_CURVE_WITH_KNOTS('',3,(#256710,#256711,#256712,#256713,
#256714,#256715,#256716,#256717,#256718,#256719,#256720,#256721,#256722,
#256723,#256724,#256725,#256726,#256727,#256728,#256729,#256730,#256731,
#256732,#256733,#256734,#256735,#256736,#256737,#256738,#256739,#256740,
#256741,#256742,#256743,#256744,#256745,#256746,#256747,#256748,#256749,
#256750,#256751,#256752,#256753,#256754,#256755,#256756,#256757,#256758,
#256759,#256760,#256761,#256762,#256763,#256764,#256765,#256766,#256767,
#256768,#256769,#256770,#256771,#256772,#256773,#256774,#256775,#256776,
#256777,#256778,#256779,#256780,#256781,#256782,#256783,#256784,#256785,
#256786,#256787,#256788,#256789,#256790,#256791,#256792,#256793,#256794,
#256795,#256796,#256797,#256798,#256799,#256800,#256801,#256802,#256803,
#256804,#256805,#256806,#256807,#256808,#256809,#256810,#256811,#256812,
#256813,#256814,#256815,#256816,#256817,#256818,#256819,#256820,#256821,
#256822,#256823,#256824,#256825,#256826,#256827,#256828,#256829,#256830,
#256831,#256832,#256833,#256834,#256835,#256836,#256837,#256838,#256839,
#256840,#256841,#256842,#256843,#256844,#256845,#256846,#256847,#256848,
#256849,#256850,#256851,#256852,#256853,#256854,#256855,#256856,#256857,
#256858,#256859,#256860,#256861,#256862,#256863,#256864,#256865,#256866,
#256867,#256868,#256869,#256870,#256871,#256872,#256873,#256874,#256875,
#256876,#256877,#256878,#256879,#256880,#256881,#256882,#256883,#256884,
#256885,#256886,#256887,#256888,#256889,#256890,#256891,#256892,#256893,
#256894,#256895,#256896,#256897,#256898,#256899,#256900,#256901,#256902,
#256903,#256904,#256905,#256906,#256907,#256908,#256909,#256910,#256911,
#256912,#256913,#256914,#256915,#256916,#256917,#256918,#256919,#256920,
#256921,#256922,#256923,#256924,#256925,#256926,#256927,#256928,#256929,
#256930,#256931,#256932,#256933,#256934,#256935,#256936,#256937,#256938,
#256939,#256940,#256941,#256942,#256943,#256944,#256945,#256946,#256947,
#256948,#256949,#256950,#256951,#256952,#256953,#256954,#256955,#256956,
#256957,#256958,#256959,#256960,#256961,#256962,#256963,#256964,#256965,
#256966,#256967,#256968,#256969,#256970,#256971,#256972,#256973,#256974,
#256975,#256976,#256977,#256978,#256979,#256980,#256981,#256982,#256983,
#256984,#256985,#256986,#256987,#256988,#256989,#256990,#256991,#256992,
#256993,#256994,#256995,#256996,#256997,#256998,#256999,#257000,#257001,
#257002,#257003,#257004,#257005,#257006,#257007,#257008,#257009,#257010,
#257011,#257012,#257013,#257014,#257015,#257016,#257017,#257018,#257019,
#257020,#257021,#257022,#257023,#257024,#257025,#257026,#257027,#257028,
#257029,#257030,#257031),.UNSPECIFIED.,.F.,.F.,(4,3,3,3,3,3,3,3,3,3,3,3,
3,3,3,3,3,3,3,3,3,3,3,3,3,3,3,3,3,3,3,3,3,3,3,3,3,3,3,3,3,3,3,3,3,3,3,3,
3,3,3,3,3,3,3,3,3,3,3,3,3,3,3,3,3,3,3,3,3,3,3,3,3,3,3,3,3,3,3,3,3,3,3,3,
3,3,3,3,3,3,3,3,3,3,3,3,3,3,3,3,3,3,3,3,3,3,3,4),(-1.,-0.99266055,-0.987155963,
-0.981651376,-0.976146789,-0.970642202,-0.965137615,-0.959633028,-0.95412844,
-0.948623853,-0.941284404,-0.935779817,-0.930275229,-0.924770642,-0.919266055,
-0.913761468,-0.908256881,-0.902752294,-0.897247706,-0.889908257,-0.88440367,
-0.878899083,-0.873394495,-0.867889908,-0.862385321,-0.855045872,-0.849541284,
-0.844036697,-0.83853211,-0.833027523,-0.827522936,-0.822018349,-0.814678899,
-0.809174312,-0.8,-0.79266055,-0.785321101,-0.777981651,-0.770642202,-0.763302752,
-0.755963303,-0.748623853,-0.741284404,-0.733944954,-0.726605505,-0.719266055,
-0.710091743,-0.702752294,-0.695412844,-0.688073394,-0.680733945,-0.671559633,
-0.664220183,-0.656880734,-0.649541284,-0.642201835,-0.634862385,-0.627522936,
-0.620183486,-0.612844037,-0.605504587,-0.598165138,-0.590825688,-0.583486239,
-0.576146789,-0.568807339,-0.56146789,-0.55412844,-0.546788991,-0.539449541,
-0.532110092,-0.521100917,-0.511926606,-0.502752294,-0.493577982,-0.48440367,
-0.475229358,-0.466055046,-0.456880734,-0.447706422,-0.43853211,-0.429357798,
-0.420183486,-0.411009174,-0.401834862,-0.39266055,-0.381651376,-0.370642202,
-0.359633028,-0.348623853,-0.337614679,-0.326605505,-0.31559633,-0.304587156,
-0.293577982,-0.282568807,-0.271559633,-0.260550459,-0.249541284,-0.23853211,
-0.227522936,-0.216513761,-0.205504587,-0.194495413,-0.183486239,-0.172477064,
-0.16146789,-0.143172102),.UNSPECIFIED.);
#24444=B_SPLINE_CURVE_WITH_KNOTS('',3,(#257032,#257033,#257034,#257035,
#257036,#257037,#257038,#257039,#257040,#257041,#257042,#257043,#257044,
#257045,#257046,#257047,#257048,#257049,#257050,#257051,#257052,#257053,
#257054,#257055,#257056,#257057,#257058,#257059,#257060,#257061,#257062,
#257063,#257064,#257065,#257066,#257067,#257068,#257069,#257070,#257071,
#257072,#257073,#257074,#257075,#257076,#257077,#257078,#257079,#257080,
#257081,#257082,#257083,#257084,#257085,#257086,#257087,#257088,#257089,
#257090,#257091,#257092,#257093,#257094,#257095,#257096,#257097,#257098,
#257099,#257100,#257101,#257102,#257103,#257104,#257105,#257106,#257107,
#257108,#257109,#257110,#257111,#257112,#257113,#257114,#257115,#257116,
#257117,#257118,#257119,#257120,#257121,#257122,#257123,#257124,#257125,
#257126,#257127,#257128,#257129,#257130,#257131,#257132,#257133,#257134,
#257135,#257136,#257137,#257138,#257139,#257140,#257141,#257142,#257143,
#257144,#257145,#257146,#257147,#257148,#257149,#257150,#257151,#257152,
#257153,#257154,#257155,#257156,#257157,#257158,#257159,#257160,#257161,
#257162,#257163,#257164,#257165,#257166,#257167,#257168,#257169,#257170,
#257171,#257172,#257173,#257174,#257175,#257176,#257177,#257178,#257179,
#257180,#257181,#257182,#257183,#257184,#257185,#257186,#257187,#257188,
#257189,#257190,#257191,#257192,#257193,#257194,#257195,#257196,#257197,
#257198,#257199,#257200,#257201,#257202,#257203,#257204,#257205,#257206,
#257207,#257208,#257209,#257210,#257211,#257212,#257213,#257214,#257215,
#257216,#257217,#257218,#257219,#257220,#257221,#257222,#257223,#257224,
#257225,#257226,#257227,#257228,#257229,#257230,#257231,#257232,#257233,
#257234,#257235,#257236,#257237,#257238,#257239,#257240,#257241,#257242,
#257243,#257244,#257245,#257246,#257247,#257248,#257249,#257250,#257251,
#257252,#257253,#257254,#257255,#257256,#257257,#257258,#257259,#257260,
#257261,#257262,#257263,#257264,#257265,#257266,#257267,#257268,#257269,
#257270,#257271,#257272,#257273,#257274,#257275,#257276,#257277,#257278,
#257279,#257280,#257281,#257282,#257283,#257284,#257285,#257286,#257287,
#257288,#257289,#257290,#257291,#257292,#257293,#257294,#257295,#257296,
#257297,#257298,#257299,#257300,#257301,#257302,#257303,#257304,#257305,
#257306,#257307,#257308,#257309,#257310,#257311,#257312,#257313,#257314,
#257315,#257316,#257317,#257318,#257319,#257320,#257321,#257322,#257323,
#257324,#257325,#257326,#257327,#257328,#257329,#257330,#257331,#257332,
#257333,#257334,#257335,#257336,#257337,#257338),.UNSPECIFIED.,.F.,.F.,
(4,3,3,3,3,3,3,3,3,3,3,3,3,3,3,3,3,3,3,3,3,3,3,3,3,3,3,3,3,3,3,3,3,3,3,
3,3,3,3,3,3,3,3,3,3,3,3,3,3,3,3,3,3,3,3,3,3,3,3,3,3,3,3,3,3,3,3,3,3,3,3,
3,3,3,3,3,3,3,3,3,3,3,3,3,3,3,3,3,3,3,3,3,3,3,3,3,3,3,3,3,3,3,4),(0.143172102,
0.15412844,0.165137615,0.176146789,0.187155963,0.198165138,0.211009174,
0.222018349,0.233027523,0.244036697,0.255045872,0.266055046,0.27706422,
0.288073394,0.299082569,0.310091743,0.321100917,0.332110092,0.344954128,
0.355963303,0.366972477,0.377981651,0.388990826,0.398165138,0.40733945,
0.416513761,0.427522936,0.436697248,0.44587156,0.456880734,0.467889908,
0.47706422,0.488073394,0.497247706,0.506422018,0.519266055,0.528440367,
0.537614679,0.544954128,0.55412844,0.56146789,0.568807339,0.576146789,0.587155963,
0.598165138,0.60733945,0.616513761,0.623853211,0.631192661,0.640366972,
0.649541284,0.656880734,0.667889908,0.675229358,0.682568807,0.689908257,
0.697247706,0.704587156,0.713761468,0.721100917,0.730275229,0.741284404,
0.748623853,0.755963303,0.763302752,0.770642202,0.777981651,0.785321101,
0.79266055,0.803669725,0.811009174,0.818348624,0.823853211,0.829357798,
0.834862385,0.840366972,0.84587156,0.851376147,0.856880734,0.862385321,
0.867889908,0.873394495,0.878899083,0.88440367,0.893577982,0.899082569,
0.904587156,0.910091743,0.91559633,0.921100917,0.928440367,0.935779817,
0.941284404,0.946788991,0.952293578,0.957798165,0.963302752,0.968807339,
0.974311927,0.979816514,0.985321101,0.99266055,1.),.UNSPECIFIED.);
#24445=B_SPLINE_CURVE_WITH_KNOTS('',3,(#258283,#258284,#258285,#258286,
#258287,#258288,#258289,#258290,#258291,#258292,#258293,#258294,#258295,
#258296,#258297,#258298,#258299,#258300,#258301,#258302,#258303,#258304,
#258305,#258306,#258307,#258308,#258309,#258310,#258311,#258312,#258313,
#258314,#258315,#258316,#258317,#258318,#258319,#258320,#258321,#258322,
#258323,#258324,#258325,#258326,#258327,#258328,#258329,#258330,#258331,
#258332,#258333,#258334,#258335,#258336,#258337,#258338,#258339,#258340,
#258341,#258342,#258343,#258344,#258345,#258346,#258347,#258348,#258349,
#258350,#258351,#258352,#258353,#258354,#258355,#258356,#258357,#258358,
#258359,#258360,#258361,#258362,#258363,#258364,#258365,#258366,#258367,
#258368,#258369,#258370,#258371,#258372,#258373,#258374,#258375,#258376,
#258377,#258378,#258379,#258380,#258381,#258382,#258383,#258384,#258385,
#258386,#258387,#258388,#258389,#258390,#258391,#258392,#258393,#258394,
#258395,#258396,#258397,#258398,#258399,#258400,#258401,#258402,#258403,
#258404,#258405,#258406,#258407,#258408,#258409,#258410,#258411,#258412,
#258413,#258414,#258415,#258416,#258417,#258418,#258419,#258420,#258421,
#258422,#258423,#258424,#258425,#258426,#258427,#258428,#258429,#258430,
#258431,#258432,#258433,#258434,#258435,#258436,#258437,#258438,#258439,
#258440,#258441,#258442,#258443,#258444,#258445,#258446,#258447,#258448,
#258449,#258450,#258451,#258452,#258453,#258454,#258455,#258456,#258457,
#258458,#258459,#258460,#258461,#258462,#258463,#258464,#258465,#258466,
#258467,#258468,#258469,#258470,#258471,#258472,#258473,#258474,#258475,
#258476,#258477,#258478,#258479,#258480,#258481,#258482,#258483,#258484,
#258485,#258486,#258487,#258488,#258489,#258490,#258491,#258492,#258493,
#258494,#258495,#258496,#258497,#258498,#258499,#258500,#258501,#258502,
#258503,#258504,#258505,#258506,#258507,#258508,#258509,#258510,#258511,
#258512,#258513,#258514,#258515,#258516,#258517,#258518,#258519,#258520,
#258521,#258522,#258523,#258524,#258525,#258526,#258527,#258528,#258529,
#258530,#258531,#258532,#258533,#258534,#258535,#258536,#258537,#258538,
#258539,#258540,#258541,#258542,#258543,#258544,#258545,#258546,#258547,
#258548,#258549,#258550,#258551,#258552,#258553,#258554,#258555,#258556,
#258557,#258558,#258559,#258560,#258561,#258562,#258563,#258564,#258565,
#258566,#258567,#258568,#258569,#258570,#258571,#258572,#258573,#258574),
 .UNSPECIFIED.,.F.,.F.,(4,3,3,3,3,3,3,3,3,3,3,3,3,3,3,3,3,3,3,3,3,3,3,3,
3,3,3,3,3,3,3,3,3,3,3,3,3,3,3,3,3,3,3,3,3,3,3,3,3,3,3,3,3,3,3,3,3,3,3,3,
3,3,3,3,3,3,3,3,3,3,3,3,3,3,3,3,3,3,3,3,3,3,3,3,3,3,3,3,3,3,3,3,3,3,3,3,
3,4),(0.143172102,0.15412844,0.165137615,0.176146789,0.187155963,0.198165138,
0.211009174,0.222018349,0.234862385,0.24587156,0.256880734,0.267889908,
0.278899083,0.289908257,0.300917431,0.311926606,0.32293578,0.333944954,
0.346788991,0.357798165,0.368807339,0.379816514,0.39266055,0.403669725,
0.412844037,0.423853211,0.433027523,0.444036697,0.453211009,0.466055046,
0.482568807,0.491743119,0.500917431,0.510091743,0.519266055,0.533944954,
0.541284404,0.548623853,0.555963303,0.565137615,0.572477064,0.579816514,
0.587155963,0.596330275,0.605504587,0.614678899,0.622018349,0.629357798,
0.636697248,0.64587156,0.655045872,0.664220183,0.67706422,0.686238532,0.693577982,
0.700917431,0.710091743,0.721100917,0.728440367,0.735779817,0.743119266,
0.750458716,0.757798165,0.766972477,0.774311927,0.781651376,0.790825688,
0.798165138,0.80733945,0.812844037,0.818348624,0.825688073,0.831192661,
0.836697248,0.842201835,0.851376147,0.856880734,0.864220183,0.873394495,
0.878899083,0.888073394,0.893577982,0.900917431,0.908256881,0.91559633,
0.92293578,0.930275229,0.939449541,0.944954128,0.950458716,0.955963303,
0.96146789,0.966972477,0.974311927,0.981651376,0.988990826,0.994495413,
1.),.UNSPECIFIED.);
#24446=B_SPLINE_CURVE_WITH_KNOTS('',3,(#258575,#258576,#258577,#258578,
#258579,#258580,#258581,#258582,#258583,#258584,#258585,#258586,#258587,
#258588,#258589,#258590,#258591,#258592,#258593,#258594,#258595,#258596,
#258597,#258598,#258599,#258600,#258601,#258602,#258603,#258604,#258605,
#258606,#258607,#258608,#258609,#258610,#258611,#258612,#258613,#258614,
#258615,#258616,#258617,#258618,#258619,#258620,#258621,#258622,#258623,
#258624,#258625,#258626,#258627,#258628,#258629,#258630,#258631,#258632,
#258633,#258634,#258635,#258636,#258637,#258638,#258639,#258640,#258641,
#258642,#258643,#258644,#258645,#258646,#258647,#258648,#258649,#258650,
#258651,#258652,#258653,#258654,#258655,#258656,#258657,#258658,#258659,
#258660,#258661,#258662,#258663,#258664,#258665,#258666,#258667,#258668,
#258669,#258670,#258671,#258672,#258673,#258674,#258675,#258676,#258677,
#258678,#258679,#258680,#258681,#258682,#258683,#258684,#258685,#258686,
#258687,#258688,#258689,#258690,#258691,#258692,#258693,#258694,#258695,
#258696,#258697,#258698,#258699,#258700,#258701,#258702,#258703,#258704,
#258705,#258706,#258707,#258708,#258709,#258710,#258711,#258712,#258713,
#258714,#258715,#258716,#258717,#258718,#258719,#258720,#258721,#258722,
#258723,#258724,#258725,#258726,#258727,#258728,#258729,#258730,#258731,
#258732,#258733,#258734,#258735,#258736,#258737,#258738,#258739,#258740,
#258741,#258742,#258743,#258744,#258745,#258746,#258747,#258748,#258749,
#258750,#258751,#258752,#258753,#258754,#258755,#258756,#258757,#258758,
#258759,#258760,#258761,#258762,#258763,#258764,#258765,#258766,#258767,
#258768,#258769,#258770,#258771,#258772,#258773,#258774,#258775,#258776,
#258777,#258778,#258779,#258780,#258781,#258782,#258783,#258784,#258785,
#258786,#258787,#258788,#258789,#258790,#258791,#258792,#258793,#258794,
#258795,#258796,#258797,#258798,#258799,#258800,#258801,#258802,#258803,
#258804,#258805,#258806,#258807,#258808,#258809,#258810,#258811,#258812,
#258813,#258814,#258815,#258816,#258817,#258818,#258819,#258820,#258821,
#258822,#258823,#258824,#258825,#258826,#258827,#258828,#258829,#258830,
#258831,#258832,#258833,#258834,#258835,#258836,#258837,#258838,#258839,
#258840,#258841,#258842,#258843,#258844,#258845,#258846,#258847,#258848,
#258849,#258850,#258851,#258852,#258853,#258854,#258855,#258856,#258857,
#258858,#258859,#258860,#258861,#258862,#258863,#258864,#258865,#258866,
#258867,#258868,#258869,#258870,#258871,#258872,#258873,#258874,#258875,
#258876,#258877,#258878,#258879,#258880,#258881,#258882,#258883,#258884,
#258885,#258886,#258887,#258888,#258889,#258890,#258891,#258892,#258893,
#258894,#258895,#258896),.UNSPECIFIED.,.F.,.F.,(4,3,3,3,3,3,3,3,3,3,3,3,
3,3,3,3,3,3,3,3,3,3,3,3,3,3,3,3,3,3,3,3,3,3,3,3,3,3,3,3,3,3,3,3,3,3,3,3,
3,3,3,3,3,3,3,3,3,3,3,3,3,3,3,3,3,3,3,3,3,3,3,3,3,3,3,3,3,3,3,3,3,3,3,3,
3,3,3,3,3,3,3,3,3,3,3,3,3,3,3,3,3,3,3,3,3,3,3,4),(0.143172102,0.15412844,
0.165137615,0.176146789,0.187155963,0.198165138,0.209174312,0.220183486,
0.231192661,0.244036697,0.255045872,0.266055046,0.27706422,0.288073394,
0.299082569,0.310091743,0.321100917,0.332110092,0.343119266,0.355963303,
0.368807339,0.379816514,0.39266055,0.401834862,0.411009174,0.420183486,
0.429357798,0.43853211,0.447706422,0.456880734,0.466055046,0.475229358,
0.48440367,0.493577982,0.502752294,0.511926606,0.521100917,0.530275229,
0.537614679,0.546788991,0.55412844,0.56146789,0.568807339,0.576146789,0.583486239,
0.590825688,0.6,0.60733945,0.614678899,0.622018349,0.629357798,0.636697248,
0.644036697,0.651376147,0.658715596,0.667889908,0.675229358,0.682568807,
0.689908257,0.697247706,0.704587156,0.711926606,0.719266055,0.726605505,
0.733944954,0.743119266,0.750458716,0.757798165,0.765137615,0.772477064,
0.779816514,0.787155963,0.794495413,0.801834862,0.809174312,0.816513761,
0.822018349,0.827522936,0.833027523,0.83853211,0.844036697,0.849541284,
0.855045872,0.860550459,0.866055046,0.871559633,0.87706422,0.882568807,
0.888073394,0.893577982,0.899082569,0.904587156,0.910091743,0.91559633,
0.921100917,0.928440367,0.933944954,0.939449541,0.944954128,0.950458716,
0.955963303,0.96146789,0.966972477,0.972477064,0.979816514,0.987155963,
0.99266055,1.),.UNSPECIFIED.);
#24447=B_SPLINE_CURVE_WITH_KNOTS('',5,(#259856,#259857,#259858,#259859,
#259860,#259861,#259862,#259863,#259864,#259865,#259866,#259867,#259868,
#259869,#259870,#259871,#259872,#259873,#259874,#259875,#259876,#259877,
#259878,#259879,#259880,#259881,#259882,#259883,#259884,#259885,#259886,
#259887,#259888,#259889,#259890,#259891,#259892,#259893,#259894,#259895,
#259896,#259897,#259898,#259899,#259900,#259901,#259902,#259903,#259904,
#259905,#259906,#259907,#259908,#259909,#259910,#259911,#259912,#259913,
#259914,#259915,#259916,#259917,#259918,#259919,#259920,#259921,#259922,
#259923,#259924,#259925,#259926,#259927,#259928,#259929,#259930,#259931,
#259932,#259933,#259934,#259935,#259936,#259937,#259938,#259939,#259940,
#259941,#259942,#259943,#259944,#259945,#259946,#259947,#259948,#259949,
#259950,#259951,#259952,#259953,#259954,#259955,#259956,#259957,#259958,
#259959,#259960,#259961,#259962,#259963,#259964,#259965,#259966,#259967,
#259968,#259969,#259970,#259971,#259972,#259973,#259974,#259975,#259976,
#259977,#259978,#259979,#259980,#259981,#259982,#259983,#259984,#259985,
#259986,#259987,#259988,#259989,#259990,#259991,#259992,#259993,#259994,
#259995,#259996,#259997,#259998,#259999,#260000,#260001,#260002,#260003,
#260004,#260005,#260006,#260007,#260008,#260009,#260010,#260011,#260012,
#260013,#260014,#260015,#260016,#260017,#260018,#260019,#260020,#260021,
#260022,#260023,#260024,#260025,#260026,#260027,#260028,#260029,#260030,
#260031,#260032,#260033,#260034,#260035,#260036,#260037,#260038,#260039,
#260040,#260041,#260042,#260043,#260044,#260045,#260046,#260047,#260048,
#260049,#260050,#260051,#260052,#260053,#260054,#260055,#260056,#260057,
#260058,#260059,#260060,#260061,#260062,#260063,#260064,#260065,#260066,
#260067,#260068,#260069,#260070,#260071,#260072,#260073,#260074,#260075,
#260076,#260077,#260078,#260079,#260080,#260081,#260082,#260083,#260084,
#260085,#260086,#260087,#260088,#260089,#260090,#260091,#260092,#260093,
#260094,#260095,#260096,#260097,#260098,#260099,#260100,#260101,#260102,
#260103,#260104,#260105,#260106,#260107,#260108,#260109,#260110,#260111,
#260112,#260113,#260114,#260115,#260116,#260117,#260118,#260119,#260120,
#260121,#260122,#260123,#260124,#260125,#260126,#260127,#260128,#260129,
#260130,#260131,#260132,#260133,#260134,#260135,#260136,#260137,#260138,
#260139,#260140,#260141,#260142,#260143,#260144,#260145,#260146,#260147,
#260148,#260149,#260150,#260151,#260152,#260153,#260154,#260155,#260156,
#260157,#260158,#260159,#260160,#260161,#260162,#260163,#260164,#260165,
#260166,#260167,#260168,#260169,#260170,#260171,#260172,#260173,#260174,
#260175,#260176,#260177,#260178,#260179,#260180,#260181,#260182,#260183,
#260184,#260185,#260186,#260187,#260188,#260189,#260190,#260191,#260192,
#260193,#260194,#260195,#260196,#260197,#260198,#260199,#260200,#260201,
#260202,#260203,#260204,#260205,#260206,#260207,#260208,#260209,#260210,
#260211,#260212,#260213,#260214,#260215,#260216,#260217,#260218,#260219,
#260220,#260221,#260222,#260223,#260224,#260225,#260226,#260227,#260228,
#260229,#260230,#260231,#260232,#260233,#260234,#260235,#260236,#260237,
#260238,#260239,#260240,#260241,#260242,#260243,#260244,#260245,#260246,
#260247,#260248,#260249,#260250,#260251,#260252,#260253,#260254,#260255,
#260256,#260257,#260258,#260259,#260260,#260261,#260262,#260263,#260264,
#260265,#260266,#260267,#260268,#260269,#260270,#260271,#260272,#260273,
#260274,#260275,#260276,#260277,#260278,#260279,#260280,#260281,#260282,
#260283,#260284,#260285,#260286,#260287,#260288,#260289,#260290,#260291,
#260292,#260293,#260294,#260295,#260296,#260297,#260298,#260299,#260300,
#260301,#260302,#260303,#260304,#260305,#260306,#260307,#260308,#260309,
#260310,#260311,#260312,#260313,#260314,#260315,#260316,#260317,#260318,
#260319,#260320,#260321,#260322,#260323,#260324,#260325,#260326),
 .UNSPECIFIED.,.F.,.F.,(6,1,1,1,1,1,1,1,1,1,1,1,1,1,1,1,1,1,1,1,1,1,1,1,
1,1,1,1,1,1,1,1,1,1,1,1,1,1,1,1,1,1,1,1,1,1,1,1,1,1,1,1,1,1,1,1,1,1,1,1,
1,1,1,1,1,1,1,1,1,1,1,1,1,1,1,1,1,1,1,1,1,1,1,1,1,1,1,1,1,1,1,1,1,1,1,1,
1,1,1,1,1,1,1,1,1,1,1,1,1,1,1,1,1,1,1,1,1,1,1,1,1,1,1,1,1,1,1,1,1,1,1,1,
1,1,1,1,1,1,1,1,1,1,1,1,1,1,1,1,1,1,1,1,1,1,1,1,1,1,1,1,1,1,1,1,1,1,1,1,
1,1,1,1,1,1,1,1,1,1,1,1,1,1,1,1,1,1,1,1,1,1,1,1,1,1,1,1,1,1,1,1,1,1,1,1,
1,1,1,1,1,1,1,1,1,1,1,1,1,1,1,1,1,1,1,1,1,1,1,1,1,1,1,1,1,1,1,1,1,1,1,1,
1,1,1,1,1,1,1,1,1,1,1,1,1,1,1,1,1,1,1,1,1,1,1,1,1,1,1,1,1,1,1,1,1,1,1,1,
1,1,1,1,1,1,1,1,1,1,1,1,1,1,1,1,1,1,1,1,1,1,1,1,1,1,1,1,1,1,1,1,1,1,1,1,
1,1,1,1,1,1,1,1,1,1,1,1,1,1,1,1,1,1,1,1,1,1,1,1,1,1,1,1,1,1,1,1,1,1,1,1,
1,1,1,1,1,1,1,1,1,1,1,1,1,1,1,1,1,1,1,1,1,1,1,1,1,1,1,1,1,1,1,1,1,1,1,1,
1,1,1,1,1,1,1,1,1,1,1,1,1,1,1,1,1,1,1,1,1,1,1,1,1,1,1,1,1,1,1,1,1,1,1,1,
1,1,1,1,1,1,1,1,1,1,1,1,1,1,1,1,1,1,1,1,1,1,1,1,1,1,1,1,1,1,1,1,1,1,1,1,
1,1,1,1,1,1,1,1,1,1,6),(0.143172102,0.144954128,0.146788991,0.148623853,
0.150458716,0.152293578,0.15412844,0.155963303,0.157798165,0.159633028,
0.16146789,0.163302752,0.165137615,0.166972477,0.168807339,0.170642202,
0.172477064,0.174311927,0.176146789,0.177981651,0.179816514,0.181651376,
0.183486239,0.185321101,0.187155963,0.188990826,0.190825688,0.19266055,
0.194495413,0.196330275,0.198165138,0.2,0.201834862,0.203669725,0.205504587,
0.20733945,0.209174312,0.211009174,0.212844037,0.214678899,0.216513761,
0.218348624,0.220183486,0.222018349,0.223853211,0.225688073,0.227522936,
0.229357798,0.231192661,0.233027523,0.234862385,0.236697248,0.23853211,
0.240366972,0.242201835,0.244036697,0.24587156,0.247706422,0.249541284,
0.251376147,0.253211009,0.255045872,0.256880734,0.258715596,0.260550459,
0.262385321,0.264220183,0.266055046,0.267889908,0.269724771,0.271559633,
0.273394495,0.275229358,0.27706422,0.278899083,0.280733945,0.282568807,
0.28440367,0.286238532,0.288073394,0.289908257,0.291743119,0.293577982,
0.295412844,0.297247706,0.299082569,0.300917431,0.302752294,0.304587156,
0.306422018,0.308256881,0.310091743,0.311926606,0.313761468,0.31559633,
0.317431193,0.319266055,0.321100917,0.32293578,0.324770642,0.326605505,
0.328440367,0.330275229,0.332110092,0.333944954,0.335779817,0.337614679,
0.339449541,0.341284404,0.343119266,0.344954128,0.346788991,0.348623853,
0.350458716,0.352293578,0.35412844,0.355963303,0.357798165,0.359633028,
0.36146789,0.363302752,0.365137615,0.366972477,0.368807339,0.370642202,
0.372477064,0.374311927,0.376146789,0.377981651,0.379816514,0.381651376,
0.383486239,0.385321101,0.387155963,0.388990826,0.390825688,0.39266055,
0.394495413,0.396330275,0.398165138,0.4,0.401834862,0.403669725,0.405504587,
0.40733945,0.409174312,0.411009174,0.412844037,0.414678899,0.416513761,
0.418348624,0.420183486,0.422018349,0.423853211,0.425688073,0.427522936,
0.429357798,0.431192661,0.433027523,0.434862385,0.436697248,0.43853211,
0.440366972,0.442201835,0.444036697,0.44587156,0.447706422,0.449541284,
0.451376147,0.453211009,0.455045872,0.456880734,0.458715596,0.460550459,
0.462385321,0.464220183,0.466055046,0.467889908,0.469724771,0.471559633,
0.473394495,0.475229358,0.47706422,0.478899083,0.480733945,0.482568807,
0.48440367,0.486238532,0.488073394,0.489908257,0.491743119,0.493577982,
0.495412844,0.497247706,0.499082569,0.500917431,0.502752294,0.504587156,
0.506422018,0.508256881,0.510091743,0.511926606,0.513761468,0.51559633,
0.517431193,0.519266055,0.521100917,0.52293578,0.524770642,0.526605505,
0.528440367,0.530275229,0.532110092,0.533944954,0.535779817,0.537614679,
0.539449541,0.541284404,0.543119266,0.544954128,0.546788991,0.548623853,
0.550458716,0.552293578,0.55412844,0.555963303,0.557798165,0.559633028,
0.56146789,0.563302752,0.565137615,0.566972477,0.568807339,0.570642202,
0.572477064,0.574311927,0.577981651,0.579816514,0.581651376,0.583486239,
0.585321101,0.587155963,0.588990826,0.590825688,0.59266055,0.594495413,
0.596330275,0.598165138,0.6,0.601834862,0.603669725,0.605504587,0.60733945,
0.609174312,0.611009174,0.612844037,0.614678899,0.616513761,0.618348624,
0.620183486,0.622018349,0.623853211,0.625688073,0.627522936,0.629357798,
0.631192661,0.633027523,0.634862385,0.636697248,0.63853211,0.640366972,
0.642201835,0.644036697,0.64587156,0.647706422,0.649541284,0.651376147,
0.653211009,0.655045872,0.656880734,0.658715596,0.660550459,0.662385321,
0.664220183,0.666055046,0.667889908,0.669724771,0.671559633,0.673394495,
0.675229358,0.67706422,0.678899083,0.680733945,0.682568807,0.68440367,0.686238532,
0.688073394,0.689908257,0.691743119,0.693577982,0.695412844,0.697247706,
0.699082569,0.700917431,0.702752294,0.704587156,0.706422018,0.708256881,
0.710091743,0.711926606,0.713761468,0.71559633,0.717431193,0.719266055,
0.721100917,0.72293578,0.724770642,0.726605505,0.728440367,0.730275229,
0.732110092,0.733944954,0.735779817,0.737614679,0.739449541,0.741284404,
0.743119266,0.744954128,0.746788991,0.748623853,0.750458716,0.752293578,
0.75412844,0.755963303,0.757798165,0.759633028,0.76146789,0.763302752,0.765137615,
0.766972477,0.768807339,0.770642202,0.772477064,0.774311927,0.776146789,
0.777981651,0.779816514,0.781651376,0.783486239,0.785321101,0.787155963,
0.788990826,0.790825688,0.79266055,0.794495413,0.796330275,0.798165138,
0.8,0.801834862,0.803669725,0.805504587,0.80733945,0.809174312,0.811009174,
0.812844037,0.814678899,0.816513761,0.818348624,0.820183486,0.822018349,
0.823853211,0.825688073,0.827522936,0.829357798,0.831192661,0.833027523,
0.834862385,0.836697248,0.83853211,0.840366972,0.842201835,0.844036697,
0.84587156,0.847706422,0.849541284,0.851376147,0.853211009,0.855045872,
0.856880734,0.858715596,0.860550459,0.862385321,0.864220183,0.866055046,
0.867889908,0.869724771,0.871559633,0.873394495,0.875229358,0.87706422,
0.878899083,0.880733945,0.882568807,0.88440367,0.886238532,0.888073394,
0.889908257,0.891743119,0.893577982,0.895412844,0.897247706,0.899082569,
0.900917431,0.902752294,0.904587156,0.906422018,0.908256881,0.910091743,
0.911926606,0.913761468,0.91559633,0.917431193,0.919266055,0.921100917,
0.92293578,0.924770642,0.926605505,0.928440367,0.930275229,0.932110092,
0.933944954,0.935779817,0.937614679,0.939449541,0.941284404,0.943119266,
0.944954128,0.946788991,0.948623853,0.950458716,0.952293578,0.95412844,
0.955963303,0.957798165,0.959633028,0.96146789,0.963302752,0.965137615,
0.966972477,0.968807339,0.970642202,0.972477064,0.974311927,0.976146789,
0.977981651,0.979816514,0.981651376,0.983486239,0.985321101,0.987155963,
0.988990826,0.990825688,0.99266055,0.994495413,0.996330275,0.998165138,
1.),.UNSPECIFIED.);
#24448=B_SPLINE_CURVE_WITH_KNOTS('',5,(#260327,#260328,#260329,#260330,
#260331,#260332,#260333,#260334,#260335,#260336,#260337,#260338,#260339,
#260340,#260341,#260342,#260343,#260344,#260345,#260346,#260347,#260348,
#260349,#260350,#260351,#260352,#260353,#260354,#260355,#260356,#260357,
#260358,#260359,#260360,#260361,#260362,#260363,#260364,#260365,#260366,
#260367,#260368,#260369,#260370,#260371,#260372,#260373,#260374,#260375,
#260376,#260377,#260378,#260379,#260380,#260381,#260382,#260383,#260384,
#260385,#260386,#260387,#260388,#260389,#260390,#260391,#260392,#260393,
#260394,#260395,#260396,#260397,#260398,#260399,#260400,#260401,#260402,
#260403,#260404,#260405,#260406,#260407,#260408,#260409,#260410,#260411,
#260412,#260413,#260414,#260415,#260416,#260417,#260418,#260419,#260420,
#260421,#260422,#260423,#260424,#260425,#260426,#260427,#260428,#260429,
#260430,#260431,#260432,#260433,#260434,#260435,#260436,#260437,#260438,
#260439,#260440,#260441,#260442,#260443,#260444,#260445,#260446,#260447,
#260448,#260449,#260450,#260451,#260452,#260453,#260454,#260455,#260456,
#260457,#260458,#260459,#260460,#260461,#260462,#260463,#260464,#260465,
#260466,#260467,#260468,#260469,#260470,#260471,#260472,#260473,#260474,
#260475,#260476,#260477,#260478,#260479,#260480,#260481,#260482,#260483,
#260484,#260485,#260486,#260487,#260488,#260489,#260490,#260491,#260492,
#260493,#260494,#260495,#260496,#260497,#260498,#260499,#260500,#260501,
#260502,#260503,#260504,#260505,#260506,#260507,#260508,#260509,#260510,
#260511,#260512,#260513,#260514,#260515,#260516,#260517,#260518,#260519,
#260520,#260521,#260522,#260523,#260524,#260525,#260526,#260527,#260528,
#260529,#260530,#260531,#260532,#260533,#260534,#260535,#260536,#260537,
#260538,#260539,#260540,#260541,#260542,#260543,#260544,#260545,#260546,
#260547,#260548,#260549,#260550,#260551,#260552,#260553,#260554,#260555,
#260556,#260557,#260558,#260559,#260560,#260561,#260562,#260563,#260564,
#260565,#260566,#260567,#260568,#260569,#260570,#260571,#260572,#260573,
#260574,#260575,#260576,#260577,#260578,#260579,#260580,#260581,#260582,
#260583,#260584,#260585,#260586,#260587,#260588,#260589,#260590,#260591,
#260592,#260593,#260594,#260595,#260596,#260597,#260598,#260599,#260600,
#260601,#260602,#260603,#260604,#260605,#260606,#260607,#260608,#260609,
#260610,#260611,#260612,#260613,#260614,#260615,#260616,#260617,#260618,
#260619,#260620,#260621,#260622,#260623,#260624,#260625,#260626,#260627,
#260628,#260629,#260630,#260631,#260632,#260633,#260634,#260635,#260636,
#260637,#260638,#260639,#260640,#260641,#260642,#260643,#260644,#260645,
#260646,#260647,#260648,#260649,#260650,#260651,#260652,#260653,#260654,
#260655,#260656,#260657,#260658,#260659,#260660,#260661,#260662,#260663,
#260664,#260665,#260666,#260667,#260668,#260669,#260670,#260671,#260672,
#260673,#260674,#260675,#260676,#260677,#260678,#260679,#260680,#260681,
#260682,#260683,#260684,#260685,#260686,#260687,#260688,#260689,#260690,
#260691,#260692,#260693,#260694,#260695,#260696,#260697,#260698,#260699,
#260700,#260701,#260702,#260703,#260704,#260705,#260706,#260707,#260708,
#260709,#260710,#260711,#260712,#260713,#260714,#260715,#260716,#260717,
#260718,#260719,#260720,#260721,#260722,#260723,#260724,#260725,#260726,
#260727,#260728,#260729,#260730,#260731,#260732,#260733,#260734,#260735,
#260736,#260737,#260738,#260739,#260740,#260741,#260742,#260743,#260744,
#260745,#260746,#260747,#260748,#260749,#260750,#260751,#260752,#260753,
#260754,#260755,#260756,#260757,#260758,#260759,#260760,#260761,#260762,
#260763,#260764,#260765,#260766,#260767,#260768,#260769,#260770,#260771,
#260772,#260773,#260774,#260775,#260776,#260777,#260778,#260779,#260780,
#260781,#260782,#260783,#260784,#260785,#260786,#260787,#260788,#260789,
#260790,#260791,#260792,#260793,#260794,#260795,#260796,#260797),
 .UNSPECIFIED.,.F.,.F.,(6,1,1,1,1,1,1,1,1,1,1,1,1,1,1,1,1,1,1,1,1,1,1,1,
1,1,1,1,1,1,1,1,1,1,1,1,1,1,1,1,1,1,1,1,1,1,1,1,1,1,1,1,1,1,1,1,1,1,1,1,
1,1,1,1,1,1,1,1,1,1,1,1,1,1,1,1,1,1,1,1,1,1,1,1,1,1,1,1,1,1,1,1,1,1,1,1,
1,1,1,1,1,1,1,1,1,1,1,1,1,1,1,1,1,1,1,1,1,1,1,1,1,1,1,1,1,1,1,1,1,1,1,1,
1,1,1,1,1,1,1,1,1,1,1,1,1,1,1,1,1,1,1,1,1,1,1,1,1,1,1,1,1,1,1,1,1,1,1,1,
1,1,1,1,1,1,1,1,1,1,1,1,1,1,1,1,1,1,1,1,1,1,1,1,1,1,1,1,1,1,1,1,1,1,1,1,
1,1,1,1,1,1,1,1,1,1,1,1,1,1,1,1,1,1,1,1,1,1,1,1,1,1,1,1,1,1,1,1,1,1,1,1,
1,1,1,1,1,1,1,1,1,1,1,1,1,1,1,1,1,1,1,1,1,1,1,1,1,1,1,1,1,1,1,1,1,1,1,1,
1,1,1,1,1,1,1,1,1,1,1,1,1,1,1,1,1,1,1,1,1,1,1,1,1,1,1,1,1,1,1,1,1,1,1,1,
1,1,1,1,1,1,1,1,1,1,1,1,1,1,1,1,1,1,1,1,1,1,1,1,1,1,1,1,1,1,1,1,1,1,1,1,
1,1,1,1,1,1,1,1,1,1,1,1,1,1,1,1,1,1,1,1,1,1,1,1,1,1,1,1,1,1,1,1,1,1,1,1,
1,1,1,1,1,1,1,1,1,1,1,1,1,1,1,1,1,1,1,1,1,1,1,1,1,1,1,1,1,1,1,1,1,1,1,1,
1,1,1,1,1,1,1,1,1,1,1,1,1,1,1,1,1,1,1,1,1,1,1,1,1,1,1,1,1,1,1,1,1,1,1,1,
1,1,1,1,1,1,1,1,1,1,6),(0.143172102,0.144954128,0.146788991,0.148623853,
0.150458716,0.152293578,0.15412844,0.155963303,0.157798165,0.159633028,
0.16146789,0.163302752,0.165137615,0.166972477,0.168807339,0.170642202,
0.172477064,0.174311927,0.176146789,0.177981651,0.179816514,0.181651376,
0.183486239,0.185321101,0.187155963,0.188990826,0.190825688,0.19266055,
0.194495413,0.196330275,0.198165138,0.2,0.201834862,0.203669725,0.205504587,
0.20733945,0.209174312,0.211009174,0.212844037,0.214678899,0.216513761,
0.218348624,0.220183486,0.222018349,0.223853211,0.225688073,0.227522936,
0.229357798,0.231192661,0.233027523,0.234862385,0.236697248,0.23853211,
0.240366972,0.242201835,0.244036697,0.24587156,0.247706422,0.249541284,
0.251376147,0.253211009,0.255045872,0.256880734,0.258715596,0.260550459,
0.262385321,0.264220183,0.266055046,0.267889908,0.269724771,0.271559633,
0.273394495,0.275229358,0.27706422,0.278899083,0.280733945,0.282568807,
0.28440367,0.286238532,0.288073394,0.289908257,0.291743119,0.293577982,
0.295412844,0.297247706,0.299082569,0.300917431,0.302752294,0.304587156,
0.306422018,0.308256881,0.310091743,0.311926606,0.313761468,0.31559633,
0.317431193,0.319266055,0.321100917,0.32293578,0.324770642,0.326605505,
0.328440367,0.330275229,0.332110092,0.333944954,0.335779817,0.337614679,
0.339449541,0.341284404,0.343119266,0.344954128,0.346788991,0.348623853,
0.350458716,0.352293578,0.35412844,0.355963303,0.357798165,0.359633028,
0.36146789,0.363302752,0.365137615,0.366972477,0.368807339,0.370642202,
0.372477064,0.374311927,0.376146789,0.377981651,0.379816514,0.381651376,
0.383486239,0.385321101,0.387155963,0.388990826,0.390825688,0.39266055,
0.394495413,0.396330275,0.398165138,0.4,0.401834862,0.403669725,0.405504587,
0.40733945,0.409174312,0.411009174,0.412844037,0.414678899,0.416513761,
0.418348624,0.420183486,0.422018349,0.423853211,0.425688073,0.427522936,
0.429357798,0.431192661,0.433027523,0.434862385,0.436697248,0.43853211,
0.440366972,0.442201835,0.444036697,0.44587156,0.447706422,0.449541284,
0.451376147,0.453211009,0.455045872,0.456880734,0.458715596,0.460550459,
0.462385321,0.464220183,0.466055046,0.467889908,0.469724771,0.471559633,
0.473394495,0.475229358,0.47706422,0.478899083,0.480733945,0.482568807,
0.48440367,0.486238532,0.488073394,0.489908257,0.491743119,0.493577982,
0.495412844,0.497247706,0.499082569,0.500917431,0.502752294,0.504587156,
0.506422018,0.508256881,0.510091743,0.511926606,0.513761468,0.51559633,
0.517431193,0.519266055,0.521100917,0.52293578,0.524770642,0.526605505,
0.528440367,0.530275229,0.532110092,0.533944954,0.535779817,0.537614679,
0.539449541,0.541284404,0.543119266,0.544954128,0.546788991,0.548623853,
0.550458716,0.552293578,0.55412844,0.555963303,0.557798165,0.559633028,
0.56146789,0.563302752,0.565137615,0.566972477,0.568807339,0.570642202,
0.572477064,0.574311927,0.577981651,0.579816514,0.581651376,0.583486239,
0.585321101,0.587155963,0.588990826,0.590825688,0.59266055,0.594495413,
0.596330275,0.598165138,0.6,0.601834862,0.603669725,0.605504587,0.60733945,
0.609174312,0.611009174,0.612844037,0.614678899,0.616513761,0.618348624,
0.620183486,0.622018349,0.623853211,0.625688073,0.627522936,0.629357798,
0.631192661,0.633027523,0.634862385,0.636697248,0.63853211,0.640366972,
0.642201835,0.644036697,0.64587156,0.647706422,0.649541284,0.651376147,
0.653211009,0.655045872,0.656880734,0.658715596,0.660550459,0.662385321,
0.664220183,0.666055046,0.667889908,0.669724771,0.671559633,0.673394495,
0.675229358,0.67706422,0.678899083,0.680733945,0.682568807,0.68440367,0.686238532,
0.688073394,0.689908257,0.691743119,0.693577982,0.695412844,0.697247706,
0.699082569,0.700917431,0.702752294,0.704587156,0.706422018,0.708256881,
0.710091743,0.711926606,0.713761468,0.71559633,0.717431193,0.719266055,
0.721100917,0.72293578,0.724770642,0.726605505,0.728440367,0.730275229,
0.732110092,0.733944954,0.735779817,0.737614679,0.739449541,0.741284404,
0.743119266,0.744954128,0.746788991,0.748623853,0.750458716,0.752293578,
0.75412844,0.755963303,0.757798165,0.759633028,0.76146789,0.763302752,0.765137615,
0.766972477,0.768807339,0.770642202,0.772477064,0.774311927,0.776146789,
0.777981651,0.779816514,0.781651376,0.783486239,0.785321101,0.787155963,
0.788990826,0.790825688,0.79266055,0.794495413,0.796330275,0.798165138,
0.8,0.801834862,0.803669725,0.805504587,0.80733945,0.809174312,0.811009174,
0.812844037,0.814678899,0.816513761,0.818348624,0.820183486,0.822018349,
0.823853211,0.825688073,0.827522936,0.829357798,0.831192661,0.833027523,
0.834862385,0.836697248,0.83853211,0.840366972,0.842201835,0.844036697,
0.84587156,0.847706422,0.849541284,0.851376147,0.853211009,0.855045872,
0.856880734,0.858715596,0.860550459,0.862385321,0.864220183,0.866055046,
0.867889908,0.869724771,0.871559633,0.873394495,0.875229358,0.87706422,
0.878899083,0.880733945,0.882568807,0.88440367,0.886238532,0.888073394,
0.889908257,0.891743119,0.893577982,0.895412844,0.897247706,0.899082569,
0.900917431,0.902752294,0.904587156,0.906422018,0.908256881,0.910091743,
0.911926606,0.913761468,0.91559633,0.917431193,0.919266055,0.921100917,
0.92293578,0.924770642,0.926605505,0.928440367,0.930275229,0.932110092,
0.933944954,0.935779817,0.937614679,0.939449541,0.941284404,0.943119266,
0.944954128,0.946788991,0.948623853,0.950458716,0.952293578,0.95412844,
0.955963303,0.957798165,0.959633028,0.96146789,0.963302752,0.965137615,
0.966972477,0.968807339,0.970642202,0.972477064,0.974311927,0.976146789,
0.977981651,0.979816514,0.981651376,0.983486239,0.985321101,0.987155963,
0.988990826,0.990825688,0.99266055,0.994495413,0.996330275,0.998165138,
1.),.UNSPECIFIED.);
#24449=B_SPLINE_CURVE_WITH_KNOTS('',5,(#261745,#261746,#261747,#261748,
#261749,#261750,#261751,#261752,#261753,#261754,#261755,#261756,#261757,
#261758,#261759,#261760,#261761,#261762,#261763,#261764,#261765,#261766,
#261767,#261768,#261769,#261770,#261771,#261772,#261773,#261774,#261775,
#261776,#261777,#261778,#261779,#261780,#261781,#261782,#261783,#261784,
#261785,#261786,#261787,#261788,#261789,#261790,#261791,#261792,#261793,
#261794,#261795,#261796,#261797,#261798,#261799,#261800,#261801,#261802,
#261803,#261804,#261805,#261806,#261807,#261808,#261809,#261810,#261811,
#261812,#261813,#261814,#261815,#261816,#261817,#261818,#261819,#261820,
#261821,#261822,#261823,#261824,#261825,#261826,#261827,#261828,#261829,
#261830,#261831,#261832,#261833,#261834,#261835,#261836,#261837,#261838,
#261839,#261840,#261841,#261842,#261843,#261844,#261845,#261846,#261847,
#261848,#261849,#261850,#261851,#261852,#261853,#261854,#261855,#261856,
#261857,#261858,#261859,#261860,#261861,#261862,#261863,#261864,#261865,
#261866,#261867,#261868,#261869,#261870,#261871,#261872,#261873,#261874,
#261875,#261876,#261877,#261878,#261879,#261880,#261881,#261882,#261883,
#261884,#261885,#261886,#261887,#261888,#261889,#261890,#261891,#261892,
#261893,#261894,#261895,#261896,#261897,#261898,#261899,#261900,#261901,
#261902,#261903,#261904,#261905,#261906,#261907,#261908,#261909,#261910,
#261911,#261912,#261913,#261914,#261915,#261916,#261917,#261918,#261919,
#261920,#261921,#261922,#261923,#261924,#261925,#261926,#261927,#261928,
#261929,#261930,#261931,#261932,#261933,#261934,#261935,#261936,#261937,
#261938,#261939,#261940,#261941,#261942,#261943,#261944,#261945,#261946,
#261947,#261948,#261949,#261950,#261951,#261952,#261953,#261954,#261955,
#261956,#261957,#261958,#261959,#261960,#261961,#261962,#261963,#261964,
#261965,#261966,#261967,#261968,#261969,#261970,#261971,#261972,#261973,
#261974,#261975,#261976,#261977,#261978,#261979,#261980,#261981,#261982,
#261983,#261984,#261985,#261986,#261987,#261988,#261989,#261990,#261991,
#261992,#261993,#261994,#261995,#261996,#261997,#261998,#261999,#262000,
#262001,#262002,#262003,#262004,#262005,#262006,#262007,#262008,#262009,
#262010,#262011,#262012,#262013,#262014,#262015,#262016,#262017,#262018,
#262019,#262020,#262021,#262022,#262023,#262024,#262025,#262026,#262027,
#262028,#262029,#262030,#262031,#262032,#262033,#262034,#262035,#262036,
#262037,#262038,#262039,#262040,#262041,#262042,#262043,#262044,#262045,
#262046,#262047,#262048,#262049,#262050,#262051,#262052,#262053,#262054,
#262055,#262056,#262057,#262058,#262059,#262060,#262061,#262062,#262063,
#262064,#262065,#262066,#262067,#262068,#262069,#262070,#262071,#262072,
#262073,#262074,#262075,#262076,#262077,#262078,#262079,#262080,#262081,
#262082,#262083,#262084,#262085,#262086,#262087,#262088,#262089,#262090,
#262091,#262092,#262093,#262094,#262095,#262096,#262097,#262098,#262099,
#262100,#262101,#262102,#262103,#262104,#262105,#262106,#262107,#262108,
#262109,#262110,#262111,#262112,#262113,#262114,#262115,#262116,#262117,
#262118,#262119,#262120,#262121,#262122,#262123,#262124,#262125,#262126,
#262127,#262128,#262129,#262130,#262131,#262132,#262133,#262134,#262135,
#262136,#262137,#262138,#262139,#262140,#262141,#262142,#262143,#262144,
#262145,#262146,#262147,#262148,#262149,#262150,#262151,#262152,#262153,
#262154,#262155,#262156,#262157,#262158,#262159,#262160,#262161,#262162,
#262163,#262164,#262165,#262166,#262167,#262168,#262169,#262170,#262171,
#262172,#262173,#262174,#262175,#262176,#262177,#262178,#262179,#262180,
#262181,#262182,#262183,#262184,#262185,#262186,#262187,#262188,#262189,
#262190,#262191,#262192,#262193,#262194,#262195,#262196,#262197,#262198,
#262199,#262200,#262201,#262202,#262203,#262204,#262205,#262206,#262207,
#262208,#262209,#262210,#262211,#262212,#262213,#262214,#262215,#262216),
 .UNSPECIFIED.,.F.,.F.,(6,1,1,1,1,1,1,1,1,1,1,1,1,1,1,1,1,1,1,1,1,1,1,1,
1,1,1,1,1,1,1,1,1,1,1,1,1,1,1,1,1,1,1,1,1,1,1,1,1,1,1,1,1,1,1,1,1,1,1,1,
1,1,1,1,1,1,1,1,1,1,1,1,1,1,1,1,1,1,1,1,1,1,1,1,1,1,1,1,1,1,1,1,1,1,1,1,
1,1,1,1,1,1,1,1,1,1,1,1,1,1,1,1,1,1,1,1,1,1,1,1,1,1,1,1,1,1,1,1,1,1,1,1,
1,1,1,1,1,1,1,1,1,1,1,1,1,1,1,1,1,1,1,1,1,1,1,1,1,1,1,1,1,1,1,1,1,1,1,1,
1,1,1,1,1,1,1,1,1,1,1,1,1,1,1,1,1,1,1,1,1,1,1,1,1,1,1,1,1,1,1,1,1,1,1,1,
1,1,1,1,1,1,1,1,1,1,1,1,1,1,1,1,1,1,1,1,1,1,1,1,1,1,1,1,1,1,1,1,1,1,1,1,
1,1,1,1,1,1,1,1,1,1,1,1,1,1,1,1,1,1,1,1,1,1,1,1,1,1,1,1,1,1,1,1,1,1,1,1,
1,1,1,1,1,1,1,1,1,1,1,1,1,1,1,1,1,1,1,1,1,1,1,1,1,1,1,1,1,1,1,1,1,1,1,1,
1,1,1,1,1,1,1,1,1,1,1,1,1,1,1,1,1,1,1,1,1,1,1,1,1,1,1,1,1,1,1,1,1,1,1,1,
1,1,1,1,1,1,1,1,1,1,1,1,1,1,1,1,1,1,1,1,1,1,1,1,1,1,1,1,1,1,1,1,1,1,1,1,
1,1,1,1,1,1,1,1,1,1,1,1,1,1,1,1,1,1,1,1,1,1,1,1,1,1,1,1,1,1,1,1,1,1,1,1,
1,1,1,1,1,1,1,1,1,1,1,1,1,1,1,1,1,1,1,1,1,1,1,1,1,1,1,1,1,1,1,1,1,1,1,1,
1,1,1,1,1,1,1,1,1,1,1,6),(-1.,-0.998165138,-0.996330275,-0.994495413,-0.99266055,
-0.990825688,-0.988990826,-0.987155963,-0.985321101,-0.983486239,-0.981651376,
-0.979816514,-0.977981651,-0.976146789,-0.974311927,-0.972477064,-0.970642202,
-0.968807339,-0.966972477,-0.965137615,-0.963302752,-0.96146789,-0.959633028,
-0.957798165,-0.955963303,-0.95412844,-0.952293578,-0.950458716,-0.948623853,
-0.946788991,-0.944954128,-0.943119266,-0.941284404,-0.939449541,-0.937614679,
-0.935779817,-0.933944954,-0.932110092,-0.930275229,-0.928440367,-0.926605505,
-0.924770642,-0.92293578,-0.921100917,-0.919266055,-0.917431193,-0.91559633,
-0.913761468,-0.911926606,-0.910091743,-0.908256881,-0.906422018,-0.904587156,
-0.902752294,-0.900917431,-0.899082569,-0.897247706,-0.895412844,-0.893577982,
-0.891743119,-0.889908257,-0.888073394,-0.886238532,-0.88440367,-0.882568807,
-0.880733945,-0.878899083,-0.87706422,-0.875229358,-0.873394495,-0.871559633,
-0.869724771,-0.867889908,-0.866055046,-0.864220183,-0.862385321,-0.860550459,
-0.858715596,-0.856880734,-0.855045872,-0.853211009,-0.851376147,-0.849541284,
-0.847706422,-0.84587156,-0.844036697,-0.842201835,-0.840366972,-0.83853211,
-0.836697248,-0.834862385,-0.833027523,-0.831192661,-0.829357798,-0.827522936,
-0.825688073,-0.823853211,-0.822018349,-0.820183486,-0.818348624,-0.816513761,
-0.814678899,-0.812844037,-0.811009174,-0.809174312,-0.80733945,-0.805504587,
-0.803669725,-0.801834862,-0.8,-0.798165138,-0.796330275,-0.794495413,-0.79266055,
-0.790825688,-0.788990826,-0.787155963,-0.785321101,-0.783486239,-0.781651376,
-0.779816514,-0.777981651,-0.776146789,-0.774311927,-0.772477064,-0.770642202,
-0.768807339,-0.766972477,-0.765137615,-0.763302752,-0.76146789,-0.759633028,
-0.757798165,-0.755963303,-0.75412844,-0.752293578,-0.750458716,-0.748623853,
-0.746788991,-0.744954128,-0.743119266,-0.741284404,-0.739449541,-0.737614679,
-0.735779817,-0.733944954,-0.732110092,-0.730275229,-0.728440367,-0.726605505,
-0.724770642,-0.72293578,-0.721100917,-0.719266055,-0.717431193,-0.71559633,
-0.713761468,-0.711926606,-0.710091743,-0.708256881,-0.706422018,-0.704587156,
-0.702752294,-0.700917431,-0.699082569,-0.697247706,-0.695412844,-0.693577982,
-0.691743119,-0.689908257,-0.688073394,-0.686238532,-0.68440367,-0.682568807,
-0.680733945,-0.678899083,-0.67706422,-0.675229358,-0.673394495,-0.671559633,
-0.669724771,-0.667889908,-0.666055046,-0.664220183,-0.662385321,-0.660550459,
-0.658715596,-0.656880734,-0.655045872,-0.653211009,-0.651376147,-0.649541284,
-0.647706422,-0.64587156,-0.644036697,-0.642201835,-0.640366972,-0.63853211,
-0.636697248,-0.634862385,-0.633027523,-0.631192661,-0.629357798,-0.627522936,
-0.625688073,-0.623853211,-0.622018349,-0.620183486,-0.618348624,-0.616513761,
-0.614678899,-0.612844037,-0.611009174,-0.609174312,-0.60733945,-0.605504587,
-0.603669725,-0.601834862,-0.6,-0.598165138,-0.596330275,-0.594495413,-0.59266055,
-0.590825688,-0.588990826,-0.587155963,-0.585321101,-0.583486239,-0.581651376,
-0.579816514,-0.577981651,-0.576146789,-0.574311927,-0.572477064,-0.570642202,
-0.568807339,-0.566972477,-0.565137615,-0.563302752,-0.56146789,-0.559633028,
-0.557798165,-0.555963303,-0.55412844,-0.552293578,-0.550458716,-0.548623853,
-0.546788991,-0.544954128,-0.543119266,-0.541284404,-0.539449541,-0.537614679,
-0.535779817,-0.533944954,-0.532110092,-0.530275229,-0.528440367,-0.526605505,
-0.524770642,-0.52293578,-0.521100917,-0.519266055,-0.517431193,-0.51559633,
-0.513761468,-0.511926606,-0.510091743,-0.508256881,-0.506422018,-0.504587156,
-0.502752294,-0.500917431,-0.499082569,-0.497247706,-0.495412844,-0.493577982,
-0.491743119,-0.489908257,-0.488073394,-0.486238532,-0.48440367,-0.482568807,
-0.480733945,-0.478899083,-0.47706422,-0.475229358,-0.473394495,-0.471559633,
-0.469724771,-0.467889908,-0.466055046,-0.464220183,-0.462385321,-0.460550459,
-0.458715596,-0.456880734,-0.455045872,-0.453211009,-0.451376147,-0.449541284,
-0.447706422,-0.44587156,-0.444036697,-0.442201835,-0.440366972,-0.43853211,
-0.436697248,-0.434862385,-0.433027523,-0.431192661,-0.429357798,-0.427522936,
-0.425688073,-0.423853211,-0.422018349,-0.420183486,-0.418348624,-0.416513761,
-0.414678899,-0.412844037,-0.411009174,-0.409174312,-0.40733945,-0.405504587,
-0.403669725,-0.401834862,-0.4,-0.398165138,-0.396330275,-0.394495413,-0.39266055,
-0.390825688,-0.388990826,-0.387155963,-0.385321101,-0.383486239,-0.381651376,
-0.379816514,-0.377981651,-0.376146789,-0.374311927,-0.372477064,-0.370642202,
-0.368807339,-0.366972477,-0.365137615,-0.363302752,-0.36146789,-0.359633028,
-0.357798165,-0.355963303,-0.35412844,-0.352293578,-0.350458716,-0.348623853,
-0.346788991,-0.344954128,-0.343119266,-0.341284404,-0.339449541,-0.337614679,
-0.335779817,-0.333944954,-0.332110092,-0.330275229,-0.328440367,-0.326605505,
-0.324770642,-0.32293578,-0.321100917,-0.319266055,-0.317431193,-0.31559633,
-0.313761468,-0.311926606,-0.310091743,-0.308256881,-0.306422018,-0.304587156,
-0.302752294,-0.300917431,-0.299082569,-0.297247706,-0.295412844,-0.293577982,
-0.291743119,-0.289908257,-0.288073394,-0.286238532,-0.28440367,-0.282568807,
-0.280733945,-0.278899083,-0.27706422,-0.275229358,-0.273394495,-0.271559633,
-0.269724771,-0.267889908,-0.266055046,-0.264220183,-0.262385321,-0.260550459,
-0.258715596,-0.256880734,-0.255045872,-0.253211009,-0.251376147,-0.249541284,
-0.247706422,-0.24587156,-0.244036697,-0.242201835,-0.240366972,-0.23853211,
-0.236697248,-0.234862385,-0.233027523,-0.231192661,-0.229357798,-0.227522936,
-0.225688073,-0.223853211,-0.222018349,-0.220183486,-0.218348624,-0.216513761,
-0.214678899,-0.212844037,-0.211009174,-0.209174312,-0.20733945,-0.205504587,
-0.203669725,-0.201834862,-0.2,-0.198165138,-0.196330275,-0.194495413,-0.19266055,
-0.190825688,-0.188990826,-0.187155963,-0.185321101,-0.183486239,-0.181651376,
-0.179816514,-0.177981651,-0.176146789,-0.174311927,-0.172477064,-0.170642202,
-0.168807339,-0.166972477,-0.165137615,-0.163302752,-0.16146789,-0.159633028,
-0.157798165,-0.155963303,-0.15412844,-0.152293578,-0.150458716,-0.148623853,
-0.146788991,-0.144954128,-0.143172102),.UNSPECIFIED.);
#24450=B_SPLINE_CURVE_WITH_KNOTS('',5,(#262217,#262218,#262219,#262220,
#262221,#262222,#262223,#262224,#262225,#262226,#262227,#262228,#262229,
#262230,#262231,#262232,#262233,#262234,#262235,#262236,#262237,#262238,
#262239,#262240,#262241,#262242,#262243,#262244,#262245,#262246,#262247,
#262248,#262249,#262250,#262251,#262252,#262253,#262254,#262255,#262256,
#262257,#262258,#262259,#262260,#262261,#262262,#262263,#262264,#262265,
#262266,#262267,#262268,#262269,#262270,#262271,#262272,#262273,#262274,
#262275,#262276,#262277,#262278,#262279,#262280,#262281,#262282,#262283,
#262284,#262285,#262286,#262287,#262288,#262289,#262290,#262291,#262292,
#262293,#262294,#262295,#262296,#262297,#262298,#262299,#262300,#262301,
#262302,#262303,#262304,#262305,#262306,#262307,#262308,#262309,#262310,
#262311,#262312,#262313,#262314,#262315,#262316,#262317,#262318,#262319,
#262320,#262321,#262322,#262323,#262324,#262325,#262326,#262327,#262328,
#262329,#262330,#262331,#262332,#262333,#262334,#262335,#262336,#262337,
#262338,#262339,#262340,#262341,#262342,#262343,#262344,#262345,#262346,
#262347,#262348,#262349,#262350,#262351,#262352,#262353,#262354,#262355,
#262356,#262357,#262358,#262359,#262360,#262361,#262362,#262363,#262364,
#262365,#262366,#262367,#262368,#262369,#262370,#262371,#262372,#262373,
#262374,#262375,#262376,#262377,#262378,#262379,#262380,#262381,#262382,
#262383,#262384,#262385,#262386,#262387,#262388,#262389,#262390,#262391,
#262392,#262393,#262394,#262395,#262396,#262397,#262398,#262399,#262400,
#262401,#262402,#262403,#262404,#262405,#262406,#262407,#262408,#262409,
#262410,#262411,#262412,#262413,#262414,#262415,#262416,#262417,#262418,
#262419,#262420,#262421,#262422,#262423,#262424,#262425,#262426,#262427,
#262428,#262429,#262430,#262431,#262432,#262433,#262434,#262435,#262436,
#262437,#262438,#262439,#262440,#262441,#262442,#262443,#262444,#262445,
#262446,#262447,#262448,#262449,#262450,#262451,#262452,#262453,#262454,
#262455,#262456,#262457,#262458,#262459,#262460,#262461,#262462,#262463,
#262464,#262465,#262466,#262467,#262468,#262469,#262470,#262471,#262472,
#262473,#262474,#262475,#262476,#262477,#262478,#262479,#262480,#262481,
#262482,#262483,#262484,#262485,#262486,#262487,#262488,#262489,#262490,
#262491,#262492,#262493,#262494,#262495,#262496,#262497,#262498,#262499,
#262500,#262501,#262502,#262503,#262504,#262505,#262506,#262507,#262508,
#262509,#262510,#262511,#262512,#262513,#262514,#262515,#262516,#262517,
#262518,#262519,#262520,#262521,#262522,#262523,#262524,#262525,#262526,
#262527,#262528,#262529,#262530,#262531,#262532,#262533,#262534,#262535,
#262536,#262537,#262538,#262539,#262540,#262541,#262542,#262543,#262544,
#262545,#262546,#262547,#262548,#262549,#262550,#262551,#262552,#262553,
#262554,#262555,#262556,#262557,#262558,#262559,#262560,#262561,#262562,
#262563,#262564,#262565,#262566,#262567,#262568,#262569,#262570,#262571,
#262572,#262573,#262574,#262575,#262576,#262577,#262578,#262579,#262580,
#262581,#262582,#262583,#262584,#262585,#262586,#262587,#262588,#262589,
#262590,#262591,#262592,#262593,#262594,#262595,#262596,#262597,#262598,
#262599,#262600,#262601,#262602,#262603,#262604,#262605,#262606,#262607,
#262608,#262609,#262610,#262611,#262612,#262613,#262614,#262615,#262616,
#262617,#262618,#262619,#262620,#262621,#262622,#262623,#262624,#262625,
#262626,#262627,#262628,#262629,#262630,#262631,#262632,#262633,#262634,
#262635,#262636,#262637,#262638,#262639,#262640,#262641,#262642,#262643,
#262644,#262645,#262646,#262647,#262648,#262649,#262650,#262651,#262652,
#262653,#262654,#262655,#262656,#262657,#262658,#262659,#262660,#262661,
#262662,#262663,#262664,#262665,#262666,#262667,#262668,#262669,#262670,
#262671,#262672,#262673,#262674,#262675,#262676,#262677,#262678,#262679,
#262680,#262681,#262682,#262683,#262684,#262685,#262686,#262687,#262688),
 .UNSPECIFIED.,.F.,.F.,(6,1,1,1,1,1,1,1,1,1,1,1,1,1,1,1,1,1,1,1,1,1,1,1,
1,1,1,1,1,1,1,1,1,1,1,1,1,1,1,1,1,1,1,1,1,1,1,1,1,1,1,1,1,1,1,1,1,1,1,1,
1,1,1,1,1,1,1,1,1,1,1,1,1,1,1,1,1,1,1,1,1,1,1,1,1,1,1,1,1,1,1,1,1,1,1,1,
1,1,1,1,1,1,1,1,1,1,1,1,1,1,1,1,1,1,1,1,1,1,1,1,1,1,1,1,1,1,1,1,1,1,1,1,
1,1,1,1,1,1,1,1,1,1,1,1,1,1,1,1,1,1,1,1,1,1,1,1,1,1,1,1,1,1,1,1,1,1,1,1,
1,1,1,1,1,1,1,1,1,1,1,1,1,1,1,1,1,1,1,1,1,1,1,1,1,1,1,1,1,1,1,1,1,1,1,1,
1,1,1,1,1,1,1,1,1,1,1,1,1,1,1,1,1,1,1,1,1,1,1,1,1,1,1,1,1,1,1,1,1,1,1,1,
1,1,1,1,1,1,1,1,1,1,1,1,1,1,1,1,1,1,1,1,1,1,1,1,1,1,1,1,1,1,1,1,1,1,1,1,
1,1,1,1,1,1,1,1,1,1,1,1,1,1,1,1,1,1,1,1,1,1,1,1,1,1,1,1,1,1,1,1,1,1,1,1,
1,1,1,1,1,1,1,1,1,1,1,1,1,1,1,1,1,1,1,1,1,1,1,1,1,1,1,1,1,1,1,1,1,1,1,1,
1,1,1,1,1,1,1,1,1,1,1,1,1,1,1,1,1,1,1,1,1,1,1,1,1,1,1,1,1,1,1,1,1,1,1,1,
1,1,1,1,1,1,1,1,1,1,1,1,1,1,1,1,1,1,1,1,1,1,1,1,1,1,1,1,1,1,1,1,1,1,1,1,
1,1,1,1,1,1,1,1,1,1,1,1,1,1,1,1,1,1,1,1,1,1,1,1,1,1,1,1,1,1,1,1,1,1,1,1,
1,1,1,1,1,1,1,1,1,1,1,6),(0.143172102,0.144954128,0.146788991,0.148623853,
0.150458716,0.152293578,0.15412844,0.155963303,0.157798165,0.159633028,
0.16146789,0.163302752,0.165137615,0.166972477,0.168807339,0.170642202,
0.172477064,0.174311927,0.176146789,0.177981651,0.179816514,0.181651376,
0.183486239,0.185321101,0.187155963,0.188990826,0.190825688,0.19266055,
0.194495413,0.196330275,0.198165138,0.2,0.201834862,0.203669725,0.205504587,
0.20733945,0.209174312,0.211009174,0.212844037,0.214678899,0.216513761,
0.218348624,0.220183486,0.222018349,0.223853211,0.225688073,0.227522936,
0.229357798,0.231192661,0.233027523,0.234862385,0.236697248,0.23853211,
0.240366972,0.242201835,0.244036697,0.24587156,0.247706422,0.249541284,
0.251376147,0.253211009,0.255045872,0.256880734,0.258715596,0.260550459,
0.262385321,0.264220183,0.266055046,0.267889908,0.269724771,0.271559633,
0.273394495,0.275229358,0.27706422,0.278899083,0.280733945,0.282568807,
0.28440367,0.286238532,0.288073394,0.289908257,0.291743119,0.293577982,
0.295412844,0.297247706,0.299082569,0.300917431,0.302752294,0.304587156,
0.306422018,0.308256881,0.310091743,0.311926606,0.313761468,0.31559633,
0.317431193,0.319266055,0.321100917,0.32293578,0.324770642,0.326605505,
0.328440367,0.330275229,0.332110092,0.333944954,0.335779817,0.337614679,
0.339449541,0.341284404,0.343119266,0.344954128,0.346788991,0.348623853,
0.350458716,0.352293578,0.35412844,0.355963303,0.357798165,0.359633028,
0.36146789,0.363302752,0.365137615,0.366972477,0.368807339,0.370642202,
0.372477064,0.374311927,0.376146789,0.377981651,0.379816514,0.381651376,
0.383486239,0.385321101,0.387155963,0.388990826,0.390825688,0.39266055,
0.394495413,0.396330275,0.398165138,0.4,0.401834862,0.403669725,0.405504587,
0.40733945,0.409174312,0.411009174,0.412844037,0.414678899,0.416513761,
0.418348624,0.420183486,0.422018349,0.423853211,0.425688073,0.427522936,
0.429357798,0.431192661,0.433027523,0.434862385,0.436697248,0.43853211,
0.440366972,0.442201835,0.444036697,0.44587156,0.447706422,0.449541284,
0.451376147,0.453211009,0.455045872,0.456880734,0.458715596,0.460550459,
0.462385321,0.464220183,0.466055046,0.467889908,0.469724771,0.471559633,
0.473394495,0.475229358,0.47706422,0.478899083,0.480733945,0.482568807,
0.48440367,0.486238532,0.488073394,0.489908257,0.491743119,0.493577982,
0.495412844,0.497247706,0.499082569,0.500917431,0.502752294,0.504587156,
0.506422018,0.508256881,0.510091743,0.511926606,0.513761468,0.51559633,
0.517431193,0.519266055,0.521100917,0.52293578,0.524770642,0.526605505,
0.528440367,0.530275229,0.532110092,0.533944954,0.535779817,0.537614679,
0.539449541,0.541284404,0.543119266,0.544954128,0.546788991,0.548623853,
0.550458716,0.552293578,0.55412844,0.555963303,0.557798165,0.559633028,
0.56146789,0.563302752,0.565137615,0.566972477,0.568807339,0.570642202,
0.572477064,0.574311927,0.576146789,0.577981651,0.579816514,0.581651376,
0.583486239,0.585321101,0.587155963,0.588990826,0.590825688,0.59266055,
0.594495413,0.596330275,0.598165138,0.6,0.601834862,0.603669725,0.605504587,
0.60733945,0.609174312,0.611009174,0.612844037,0.614678899,0.616513761,
0.618348624,0.620183486,0.622018349,0.623853211,0.625688073,0.627522936,
0.629357798,0.631192661,0.633027523,0.634862385,0.636697248,0.63853211,
0.640366972,0.642201835,0.644036697,0.64587156,0.647706422,0.649541284,
0.651376147,0.653211009,0.655045872,0.656880734,0.658715596,0.660550459,
0.662385321,0.664220183,0.666055046,0.667889908,0.669724771,0.671559633,
0.673394495,0.675229358,0.67706422,0.678899083,0.680733945,0.682568807,
0.68440367,0.686238532,0.688073394,0.689908257,0.691743119,0.693577982,
0.695412844,0.697247706,0.699082569,0.700917431,0.702752294,0.704587156,
0.706422018,0.708256881,0.710091743,0.711926606,0.713761468,0.71559633,
0.717431193,0.719266055,0.721100917,0.72293578,0.724770642,0.726605505,
0.728440367,0.730275229,0.732110092,0.733944954,0.735779817,0.737614679,
0.739449541,0.741284404,0.743119266,0.744954128,0.746788991,0.748623853,
0.750458716,0.752293578,0.75412844,0.755963303,0.757798165,0.759633028,
0.76146789,0.763302752,0.765137615,0.766972477,0.768807339,0.770642202,
0.772477064,0.774311927,0.776146789,0.777981651,0.779816514,0.781651376,
0.783486239,0.785321101,0.787155963,0.788990826,0.790825688,0.79266055,
0.794495413,0.796330275,0.798165138,0.8,0.801834862,0.803669725,0.805504587,
0.80733945,0.809174312,0.811009174,0.812844037,0.814678899,0.816513761,
0.818348624,0.820183486,0.822018349,0.823853211,0.825688073,0.827522936,
0.829357798,0.831192661,0.833027523,0.834862385,0.836697248,0.83853211,
0.840366972,0.842201835,0.844036697,0.84587156,0.847706422,0.849541284,
0.851376147,0.853211009,0.855045872,0.856880734,0.858715596,0.860550459,
0.862385321,0.864220183,0.866055046,0.867889908,0.869724771,0.871559633,
0.873394495,0.875229358,0.87706422,0.878899083,0.880733945,0.882568807,
0.88440367,0.886238532,0.888073394,0.889908257,0.891743119,0.893577982,
0.895412844,0.897247706,0.899082569,0.900917431,0.902752294,0.904587156,
0.906422018,0.908256881,0.910091743,0.911926606,0.913761468,0.91559633,
0.917431193,0.919266055,0.921100917,0.92293578,0.924770642,0.926605505,
0.928440367,0.930275229,0.932110092,0.933944954,0.935779817,0.937614679,
0.939449541,0.941284404,0.943119266,0.944954128,0.946788991,0.948623853,
0.950458716,0.952293578,0.95412844,0.955963303,0.957798165,0.959633028,
0.96146789,0.963302752,0.965137615,0.966972477,0.968807339,0.970642202,
0.972477064,0.974311927,0.976146789,0.977981651,0.979816514,0.981651376,
0.983486239,0.985321101,0.987155963,0.988990826,0.990825688,0.99266055,
0.994495413,0.996330275,0.998165138,1.),.UNSPECIFIED.);
#24451=B_SPLINE_CURVE_WITH_KNOTS('',3,(#263651,#263652,#263653,#263654,
#263655,#263656,#263657,#263658,#263659,#263660,#263661,#263662,#263663,
#263664,#263665,#263666,#263667,#263668,#263669,#263670,#263671,#263672,
#263673,#263674,#263675,#263676,#263677,#263678,#263679,#263680,#263681,
#263682,#263683,#263684,#263685,#263686,#263687,#263688,#263689,#263690,
#263691,#263692,#263693,#263694,#263695,#263696,#263697,#263698,#263699,
#263700,#263701,#263702,#263703,#263704,#263705,#263706,#263707,#263708,
#263709,#263710,#263711,#263712,#263713,#263714,#263715,#263716,#263717,
#263718,#263719,#263720,#263721,#263722,#263723,#263724,#263725,#263726,
#263727,#263728,#263729,#263730,#263731,#263732,#263733,#263734,#263735,
#263736,#263737,#263738,#263739,#263740,#263741,#263742,#263743,#263744,
#263745,#263746,#263747,#263748,#263749,#263750,#263751,#263752,#263753,
#263754,#263755,#263756,#263757,#263758,#263759,#263760,#263761,#263762,
#263763,#263764,#263765,#263766,#263767,#263768,#263769,#263770,#263771,
#263772,#263773,#263774,#263775,#263776,#263777,#263778,#263779,#263780,
#263781,#263782,#263783,#263784,#263785,#263786,#263787,#263788,#263789,
#263790,#263791,#263792,#263793,#263794,#263795,#263796,#263797,#263798,
#263799,#263800,#263801,#263802,#263803,#263804,#263805,#263806,#263807,
#263808,#263809,#263810,#263811,#263812,#263813,#263814,#263815,#263816,
#263817,#263818,#263819,#263820,#263821,#263822,#263823,#263824,#263825,
#263826,#263827,#263828,#263829,#263830,#263831,#263832,#263833,#263834,
#263835,#263836,#263837,#263838,#263839,#263840,#263841,#263842,#263843,
#263844,#263845,#263846,#263847,#263848,#263849,#263850,#263851,#263852,
#263853,#263854,#263855,#263856,#263857,#263858,#263859,#263860,#263861,
#263862,#263863,#263864,#263865,#263866,#263867,#263868,#263869,#263870,
#263871,#263872,#263873,#263874,#263875,#263876,#263877,#263878,#263879,
#263880,#263881,#263882,#263883,#263884,#263885,#263886,#263887,#263888,
#263889,#263890,#263891,#263892,#263893,#263894,#263895,#263896,#263897,
#263898,#263899,#263900,#263901,#263902,#263903,#263904,#263905,#263906,
#263907,#263908,#263909,#263910,#263911,#263912,#263913,#263914,#263915,
#263916,#263917,#263918,#263919,#263920,#263921,#263922,#263923,#263924,
#263925,#263926,#263927,#263928,#263929,#263930,#263931,#263932,#263933,
#263934,#263935,#263936,#263937,#263938,#263939,#263940,#263941,#263942,
#263943,#263944,#263945,#263946,#263947,#263948,#263949,#263950,#263951,
#263952,#263953,#263954,#263955,#263956,#263957,#263958,#263959,#263960,
#263961,#263962,#263963),.UNSPECIFIED.,.F.,.F.,(4,3,3,3,3,3,3,3,3,3,3,3,
3,3,3,3,3,3,3,3,3,3,3,3,3,3,3,3,3,3,3,3,3,3,3,3,3,3,3,3,3,3,3,3,3,3,3,3,
3,3,3,3,3,3,3,3,3,3,3,3,3,3,3,3,3,3,3,3,3,3,3,3,3,3,3,3,3,3,3,3,3,3,3,3,
3,3,3,3,3,3,3,3,3,3,3,3,3,3,3,3,3,3,3,3,4),(-1.,-0.994495413,-0.988990826,
-0.981651376,-0.976146789,-0.970642202,-0.965137615,-0.959633028,-0.95412844,
-0.948623853,-0.943119266,-0.937614679,-0.932110092,-0.926605505,-0.921100917,
-0.913761468,-0.908256881,-0.900917431,-0.895412844,-0.889908257,-0.88440367,
-0.878899083,-0.873394495,-0.867889908,-0.860550459,-0.855045872,-0.849541284,
-0.844036697,-0.83853211,-0.833027523,-0.827522936,-0.822018349,-0.816513761,
-0.809174312,-0.8,-0.79266055,-0.783486239,-0.774311927,-0.766972477,-0.759633028,
-0.752293578,-0.744954128,-0.737614679,-0.728440367,-0.721100917,-0.711926606,
-0.704587156,-0.697247706,-0.689908257,-0.682568807,-0.675229358,-0.667889908,
-0.660550459,-0.653211009,-0.644036697,-0.636697248,-0.627522936,-0.620183486,
-0.612844037,-0.605504587,-0.598165138,-0.590825688,-0.583486239,-0.576146789,
-0.568807339,-0.56146789,-0.55412844,-0.546788991,-0.539449541,-0.532110092,
-0.52293578,-0.513761468,-0.504587156,-0.495412844,-0.486238532,-0.47706422,
-0.466055046,-0.455045872,-0.442201835,-0.433027523,-0.420183486,-0.411009174,
-0.401834862,-0.39266055,-0.381651376,-0.370642202,-0.359633028,-0.348623853,
-0.337614679,-0.324770642,-0.313761468,-0.302752294,-0.291743119,-0.280733945,
-0.269724771,-0.256880734,-0.242201835,-0.231192661,-0.220183486,-0.209174312,
-0.196330275,-0.183486239,-0.172477064,-0.16146789,-0.143172102),
 .UNSPECIFIED.);
#24452=B_SPLINE_CURVE_WITH_KNOTS('',3,(#263964,#263965,#263966,#263967,
#263968,#263969,#263970,#263971,#263972,#263973,#263974,#263975,#263976,
#263977,#263978,#263979,#263980,#263981,#263982,#263983,#263984,#263985,
#263986,#263987,#263988,#263989,#263990,#263991,#263992,#263993,#263994,
#263995,#263996,#263997,#263998,#263999,#264000,#264001,#264002,#264003,
#264004,#264005,#264006,#264007,#264008,#264009,#264010,#264011,#264012,
#264013,#264014,#264015,#264016,#264017,#264018,#264019,#264020,#264021,
#264022,#264023,#264024,#264025,#264026,#264027,#264028,#264029,#264030,
#264031,#264032,#264033,#264034,#264035,#264036,#264037,#264038,#264039,
#264040,#264041,#264042,#264043,#264044,#264045,#264046,#264047,#264048,
#264049,#264050,#264051,#264052,#264053,#264054,#264055,#264056,#264057,
#264058,#264059,#264060,#264061,#264062,#264063,#264064,#264065,#264066,
#264067,#264068,#264069,#264070,#264071,#264072,#264073,#264074,#264075,
#264076,#264077,#264078,#264079,#264080,#264081,#264082,#264083,#264084,
#264085,#264086,#264087,#264088,#264089,#264090,#264091,#264092,#264093,
#264094,#264095,#264096,#264097,#264098,#264099,#264100,#264101,#264102,
#264103,#264104,#264105,#264106,#264107,#264108,#264109,#264110,#264111,
#264112,#264113,#264114,#264115,#264116,#264117,#264118,#264119,#264120,
#264121,#264122,#264123,#264124,#264125,#264126,#264127,#264128,#264129,
#264130,#264131,#264132,#264133,#264134,#264135,#264136,#264137,#264138,
#264139,#264140,#264141,#264142,#264143,#264144,#264145,#264146,#264147,
#264148,#264149,#264150,#264151,#264152,#264153,#264154,#264155,#264156,
#264157,#264158,#264159,#264160,#264161,#264162,#264163,#264164,#264165,
#264166,#264167,#264168,#264169,#264170,#264171,#264172,#264173,#264174,
#264175,#264176,#264177,#264178,#264179,#264180,#264181,#264182,#264183,
#264184,#264185,#264186,#264187,#264188,#264189,#264190,#264191,#264192,
#264193,#264194,#264195,#264196,#264197,#264198,#264199,#264200,#264201,
#264202,#264203,#264204,#264205,#264206,#264207,#264208,#264209,#264210,
#264211,#264212,#264213,#264214,#264215,#264216,#264217,#264218,#264219,
#264220,#264221,#264222,#264223,#264224,#264225,#264226,#264227,#264228,
#264229,#264230,#264231,#264232,#264233,#264234,#264235,#264236,#264237,
#264238,#264239,#264240,#264241,#264242,#264243,#264244,#264245,#264246,
#264247,#264248,#264249,#264250,#264251,#264252,#264253,#264254,#264255,
#264256,#264257,#264258),.UNSPECIFIED.,.F.,.F.,(4,3,3,3,3,3,3,3,3,3,3,3,
3,3,3,3,3,3,3,3,3,3,3,3,3,3,3,3,3,3,3,3,3,3,3,3,3,3,3,3,3,3,3,3,3,3,3,3,
3,3,3,3,3,3,3,3,3,3,3,3,3,3,3,3,3,3,3,3,3,3,3,3,3,3,3,3,3,3,3,3,3,3,3,3,
3,3,3,3,3,3,3,3,3,3,3,3,3,3,4),(0.143172102,0.15412844,0.165137615,0.177981651,
0.188990826,0.201834862,0.212844037,0.223853211,0.234862385,0.24587156,
0.256880734,0.267889908,0.278899083,0.289908257,0.300917431,0.311926606,
0.32293578,0.335779817,0.346788991,0.363302752,0.374311927,0.388990826,
0.4,0.409174312,0.418348624,0.427522936,0.436697248,0.44587156,0.455045872,
0.464220183,0.473394495,0.48440367,0.493577982,0.506422018,0.51559633,0.524770642,
0.533944954,0.543119266,0.552293578,0.559633028,0.566972477,0.577981651,
0.587155963,0.594495413,0.601834862,0.609174312,0.616513761,0.625688073,
0.633027523,0.640366972,0.649541284,0.656880734,0.669724771,0.67706422,
0.686238532,0.693577982,0.700917431,0.708256881,0.717431193,0.724770642,
0.733944954,0.743119266,0.750458716,0.759633028,0.766972477,0.777981651,
0.785321101,0.79266055,0.8,0.80733945,0.812844037,0.822018349,0.827522936,
0.834862385,0.840366972,0.84587156,0.851376147,0.858715596,0.864220183,
0.869724771,0.875229358,0.88440367,0.889908257,0.895412844,0.904587156,
0.913761468,0.921100917,0.930275229,0.935779817,0.943119266,0.948623853,
0.95412844,0.959633028,0.965137615,0.970642202,0.977981651,0.987155963,
0.99266055,1.),.UNSPECIFIED.);
#24453=B_SPLINE_CURVE_WITH_KNOTS('',5,(#265203,#265204,#265205,#265206,
#265207,#265208,#265209,#265210,#265211,#265212,#265213,#265214,#265215,
#265216,#265217,#265218,#265219,#265220,#265221,#265222,#265223,#265224,
#265225,#265226,#265227,#265228,#265229,#265230,#265231,#265232,#265233,
#265234,#265235,#265236,#265237,#265238,#265239,#265240,#265241,#265242,
#265243,#265244,#265245,#265246,#265247,#265248,#265249,#265250,#265251,
#265252,#265253,#265254,#265255,#265256,#265257,#265258,#265259,#265260,
#265261,#265262,#265263,#265264,#265265,#265266,#265267,#265268,#265269,
#265270,#265271,#265272,#265273,#265274,#265275,#265276,#265277,#265278,
#265279,#265280,#265281,#265282,#265283,#265284,#265285,#265286,#265287,
#265288,#265289,#265290,#265291,#265292,#265293,#265294,#265295,#265296,
#265297,#265298,#265299,#265300,#265301,#265302,#265303,#265304,#265305,
#265306,#265307,#265308,#265309,#265310,#265311,#265312,#265313,#265314,
#265315,#265316,#265317,#265318,#265319,#265320,#265321,#265322,#265323,
#265324,#265325,#265326,#265327,#265328,#265329,#265330,#265331,#265332,
#265333,#265334,#265335,#265336,#265337,#265338,#265339,#265340,#265341,
#265342,#265343,#265344,#265345,#265346,#265347,#265348,#265349,#265350,
#265351,#265352,#265353,#265354,#265355,#265356,#265357,#265358,#265359,
#265360,#265361,#265362,#265363,#265364,#265365,#265366,#265367,#265368,
#265369,#265370,#265371,#265372,#265373,#265374,#265375,#265376,#265377,
#265378,#265379,#265380,#265381,#265382,#265383,#265384,#265385,#265386,
#265387,#265388,#265389,#265390,#265391,#265392,#265393,#265394,#265395,
#265396,#265397,#265398,#265399,#265400,#265401,#265402,#265403,#265404,
#265405,#265406,#265407,#265408,#265409,#265410,#265411,#265412,#265413,
#265414,#265415,#265416,#265417,#265418,#265419,#265420,#265421,#265422,
#265423,#265424,#265425,#265426,#265427,#265428,#265429,#265430,#265431,
#265432,#265433,#265434,#265435,#265436,#265437,#265438,#265439,#265440,
#265441,#265442,#265443,#265444,#265445,#265446,#265447,#265448,#265449,
#265450,#265451,#265452,#265453,#265454,#265455,#265456,#265457,#265458,
#265459,#265460,#265461,#265462,#265463,#265464,#265465,#265466,#265467,
#265468,#265469,#265470,#265471,#265472,#265473,#265474,#265475,#265476,
#265477,#265478,#265479,#265480,#265481,#265482,#265483,#265484,#265485,
#265486,#265487,#265488,#265489,#265490,#265491,#265492,#265493,#265494,
#265495,#265496,#265497,#265498,#265499,#265500,#265501,#265502,#265503,
#265504,#265505,#265506,#265507,#265508,#265509,#265510,#265511,#265512,
#265513,#265514,#265515,#265516,#265517,#265518,#265519,#265520,#265521,
#265522,#265523,#265524,#265525,#265526,#265527,#265528,#265529,#265530,
#265531,#265532,#265533,#265534,#265535,#265536,#265537,#265538,#265539,
#265540,#265541,#265542,#265543,#265544,#265545,#265546,#265547,#265548,
#265549,#265550,#265551,#265552,#265553,#265554,#265555,#265556,#265557,
#265558,#265559,#265560,#265561,#265562,#265563,#265564,#265565,#265566,
#265567,#265568,#265569,#265570,#265571,#265572,#265573,#265574,#265575,
#265576,#265577,#265578,#265579,#265580,#265581,#265582,#265583,#265584,
#265585,#265586,#265587,#265588,#265589,#265590,#265591,#265592,#265593,
#265594,#265595,#265596,#265597,#265598,#265599,#265600,#265601,#265602,
#265603,#265604,#265605,#265606,#265607,#265608,#265609,#265610,#265611,
#265612,#265613,#265614,#265615,#265616,#265617,#265618,#265619,#265620,
#265621,#265622,#265623,#265624,#265625,#265626,#265627,#265628,#265629,
#265630,#265631,#265632,#265633,#265634,#265635,#265636,#265637,#265638,
#265639,#265640,#265641,#265642,#265643,#265644,#265645,#265646,#265647,
#265648,#265649,#265650,#265651,#265652,#265653,#265654,#265655,#265656,
#265657,#265658,#265659,#265660,#265661,#265662,#265663,#265664,#265665,
#265666,#265667,#265668,#265669,#265670,#265671,#265672),.UNSPECIFIED.,
 .F.,.F.,(6,1,1,1,1,1,1,1,1,1,1,1,1,1,1,1,1,1,1,1,1,1,1,1,1,1,1,1,1,1,1,
1,1,1,1,1,1,1,1,1,1,1,1,1,1,1,1,1,1,1,1,1,1,1,1,1,1,1,1,1,1,1,1,1,1,1,1,
1,1,1,1,1,1,1,1,1,1,1,1,1,1,1,1,1,1,1,1,1,1,1,1,1,1,1,1,1,1,1,1,1,1,1,1,
1,1,1,1,1,1,1,1,1,1,1,1,1,1,1,1,1,1,1,1,1,1,1,1,1,1,1,1,1,1,1,1,1,1,1,1,
1,1,1,1,1,1,1,1,1,1,1,1,1,1,1,1,1,1,1,1,1,1,1,1,1,1,1,1,1,1,1,1,1,1,1,1,
1,1,1,1,1,1,1,1,1,1,1,1,1,1,1,1,1,1,1,1,1,1,1,1,1,1,1,1,1,1,1,1,1,1,1,1,
1,1,1,1,1,1,1,1,1,1,1,1,1,1,1,1,1,1,1,1,1,1,1,1,1,1,1,1,1,1,1,1,1,1,1,1,
1,1,1,1,1,1,1,1,1,1,1,1,1,1,1,1,1,1,1,1,1,1,1,1,1,1,1,1,1,1,1,1,1,1,1,1,
1,1,1,1,1,1,1,1,1,1,1,1,1,1,1,1,1,1,1,1,1,1,1,1,1,1,1,1,1,1,1,1,1,1,1,1,
1,1,1,1,1,1,1,1,1,1,1,1,1,1,1,1,1,1,1,1,1,1,1,1,1,1,1,1,1,1,1,1,1,1,1,1,
1,1,1,1,1,1,1,1,1,1,1,1,1,1,1,1,1,1,1,1,1,1,1,1,1,1,1,1,1,1,1,1,1,1,1,1,
1,1,1,1,1,1,1,1,1,1,1,1,1,1,1,1,1,1,1,1,1,1,1,1,1,1,1,1,1,1,1,1,1,1,1,1,
1,1,1,1,1,1,1,1,1,1,1,1,1,1,1,1,1,1,1,1,1,1,1,1,1,1,1,1,1,1,1,1,1,1,1,1,
1,1,6),(0.143172102,0.144954128,0.146788991,0.148623853,0.150458716,0.152293578,
0.15412844,0.155963303,0.157798165,0.159633028,0.16146789,0.163302752,0.165137615,
0.166972477,0.168807339,0.170642202,0.172477064,0.174311927,0.176146789,
0.177981651,0.179816514,0.181651376,0.183486239,0.185321101,0.187155963,
0.188990826,0.190825688,0.19266055,0.194495413,0.196330275,0.198165138,
0.2,0.201834862,0.203669725,0.205504587,0.20733945,0.209174312,0.211009174,
0.212844037,0.214678899,0.216513761,0.218348624,0.220183486,0.222018349,
0.223853211,0.225688073,0.227522936,0.229357798,0.231192661,0.233027523,
0.234862385,0.236697248,0.23853211,0.240366972,0.242201835,0.244036697,
0.24587156,0.247706422,0.249541284,0.251376147,0.253211009,0.255045872,
0.256880734,0.258715596,0.260550459,0.262385321,0.264220183,0.266055046,
0.267889908,0.269724771,0.271559633,0.273394495,0.275229358,0.27706422,
0.278899083,0.280733945,0.282568807,0.28440367,0.286238532,0.288073394,
0.289908257,0.291743119,0.293577982,0.295412844,0.297247706,0.299082569,
0.300917431,0.302752294,0.304587156,0.306422018,0.308256881,0.310091743,
0.311926606,0.313761468,0.31559633,0.317431193,0.319266055,0.321100917,
0.32293578,0.324770642,0.326605505,0.328440367,0.330275229,0.333944954,
0.335779817,0.337614679,0.339449541,0.341284404,0.343119266,0.344954128,
0.346788991,0.348623853,0.350458716,0.352293578,0.35412844,0.355963303,
0.357798165,0.359633028,0.36146789,0.363302752,0.365137615,0.366972477,
0.368807339,0.370642202,0.372477064,0.374311927,0.376146789,0.377981651,
0.379816514,0.381651376,0.383486239,0.385321101,0.387155963,0.388990826,
0.390825688,0.39266055,0.394495413,0.396330275,0.398165138,0.4,0.401834862,
0.403669725,0.405504587,0.40733945,0.409174312,0.411009174,0.412844037,
0.414678899,0.416513761,0.418348624,0.420183486,0.422018349,0.423853211,
0.425688073,0.427522936,0.429357798,0.431192661,0.433027523,0.434862385,
0.436697248,0.43853211,0.440366972,0.442201835,0.444036697,0.44587156,0.447706422,
0.449541284,0.451376147,0.453211009,0.455045872,0.456880734,0.458715596,
0.460550459,0.462385321,0.464220183,0.466055046,0.467889908,0.469724771,
0.471559633,0.473394495,0.475229358,0.47706422,0.478899083,0.480733945,
0.482568807,0.48440367,0.486238532,0.488073394,0.489908257,0.491743119,
0.493577982,0.495412844,0.497247706,0.499082569,0.500917431,0.502752294,
0.504587156,0.506422018,0.508256881,0.511926606,0.513761468,0.51559633,
0.517431193,0.519266055,0.521100917,0.52293578,0.524770642,0.526605505,
0.528440367,0.530275229,0.532110092,0.533944954,0.535779817,0.537614679,
0.539449541,0.541284404,0.543119266,0.544954128,0.546788991,0.548623853,
0.550458716,0.552293578,0.55412844,0.555963303,0.557798165,0.559633028,
0.56146789,0.563302752,0.565137615,0.566972477,0.568807339,0.570642202,
0.572477064,0.574311927,0.576146789,0.577981651,0.579816514,0.581651376,
0.583486239,0.585321101,0.587155963,0.588990826,0.590825688,0.59266055,
0.594495413,0.596330275,0.598165138,0.6,0.601834862,0.603669725,0.605504587,
0.60733945,0.609174312,0.611009174,0.612844037,0.614678899,0.616513761,
0.618348624,0.620183486,0.622018349,0.623853211,0.625688073,0.627522936,
0.629357798,0.631192661,0.633027523,0.634862385,0.636697248,0.63853211,
0.640366972,0.642201835,0.644036697,0.64587156,0.647706422,0.649541284,
0.651376147,0.653211009,0.655045872,0.656880734,0.658715596,0.660550459,
0.662385321,0.664220183,0.666055046,0.667889908,0.669724771,0.671559633,
0.673394495,0.675229358,0.67706422,0.678899083,0.680733945,0.682568807,
0.68440367,0.686238532,0.688073394,0.689908257,0.691743119,0.693577982,
0.695412844,0.697247706,0.699082569,0.700917431,0.702752294,0.704587156,
0.706422018,0.708256881,0.710091743,0.711926606,0.713761468,0.71559633,
0.717431193,0.719266055,0.721100917,0.72293578,0.724770642,0.726605505,
0.728440367,0.730275229,0.732110092,0.733944954,0.735779817,0.737614679,
0.739449541,0.741284404,0.743119266,0.744954128,0.746788991,0.748623853,
0.750458716,0.752293578,0.75412844,0.755963303,0.757798165,0.759633028,
0.76146789,0.763302752,0.765137615,0.766972477,0.768807339,0.770642202,
0.772477064,0.774311927,0.776146789,0.777981651,0.779816514,0.781651376,
0.783486239,0.785321101,0.787155963,0.788990826,0.790825688,0.79266055,
0.794495413,0.796330275,0.798165138,0.8,0.801834862,0.803669725,0.805504587,
0.80733945,0.809174312,0.811009174,0.812844037,0.814678899,0.816513761,
0.818348624,0.820183486,0.822018349,0.823853211,0.825688073,0.827522936,
0.829357798,0.831192661,0.833027523,0.834862385,0.836697248,0.83853211,
0.840366972,0.842201835,0.844036697,0.84587156,0.847706422,0.849541284,
0.851376147,0.853211009,0.855045872,0.856880734,0.858715596,0.860550459,
0.862385321,0.864220183,0.866055046,0.867889908,0.869724771,0.871559633,
0.873394495,0.875229358,0.87706422,0.878899083,0.880733945,0.882568807,
0.88440367,0.886238532,0.888073394,0.889908257,0.891743119,0.893577982,
0.895412844,0.897247706,0.899082569,0.900917431,0.902752294,0.904587156,
0.906422018,0.908256881,0.910091743,0.911926606,0.913761468,0.91559633,
0.917431193,0.919266055,0.921100917,0.92293578,0.924770642,0.926605505,
0.928440367,0.930275229,0.932110092,0.933944954,0.935779817,0.937614679,
0.939449541,0.941284404,0.943119266,0.944954128,0.946788991,0.948623853,
0.950458716,0.952293578,0.95412844,0.955963303,0.957798165,0.959633028,
0.96146789,0.963302752,0.965137615,0.966972477,0.968807339,0.970642202,
0.972477064,0.974311927,0.976146789,0.977981651,0.979816514,0.981651376,
0.983486239,0.985321101,0.987155963,0.988990826,0.990825688,0.99266055,
0.994495413,0.996330275,0.998165138,1.),.UNSPECIFIED.);
#24454=B_SPLINE_CURVE_WITH_KNOTS('',5,(#265673,#265674,#265675,#265676,
#265677,#265678,#265679,#265680,#265681,#265682,#265683,#265684,#265685,
#265686,#265687,#265688,#265689,#265690,#265691,#265692,#265693,#265694,
#265695,#265696,#265697,#265698,#265699,#265700,#265701,#265702,#265703,
#265704,#265705,#265706,#265707,#265708,#265709,#265710,#265711,#265712,
#265713,#265714,#265715,#265716,#265717,#265718,#265719,#265720,#265721,
#265722,#265723,#265724,#265725,#265726,#265727,#265728,#265729,#265730,
#265731,#265732,#265733,#265734,#265735,#265736,#265737,#265738,#265739,
#265740,#265741,#265742,#265743,#265744,#265745,#265746,#265747,#265748,
#265749,#265750,#265751,#265752,#265753,#265754,#265755,#265756,#265757,
#265758,#265759,#265760,#265761,#265762,#265763,#265764,#265765,#265766,
#265767,#265768,#265769,#265770,#265771,#265772,#265773,#265774,#265775,
#265776,#265777,#265778,#265779,#265780,#265781,#265782,#265783,#265784,
#265785,#265786,#265787,#265788,#265789,#265790,#265791,#265792,#265793,
#265794,#265795,#265796,#265797,#265798,#265799,#265800,#265801,#265802,
#265803,#265804,#265805,#265806,#265807,#265808,#265809,#265810,#265811,
#265812,#265813,#265814,#265815,#265816,#265817,#265818,#265819,#265820,
#265821,#265822,#265823,#265824,#265825,#265826,#265827,#265828,#265829,
#265830,#265831,#265832,#265833,#265834,#265835,#265836,#265837,#265838,
#265839,#265840,#265841,#265842,#265843,#265844,#265845,#265846,#265847,
#265848,#265849,#265850,#265851,#265852,#265853,#265854,#265855,#265856,
#265857,#265858,#265859,#265860,#265861,#265862,#265863,#265864,#265865,
#265866,#265867,#265868,#265869,#265870,#265871,#265872,#265873,#265874,
#265875,#265876,#265877,#265878,#265879,#265880,#265881,#265882,#265883,
#265884,#265885,#265886,#265887,#265888,#265889,#265890,#265891,#265892,
#265893,#265894,#265895,#265896,#265897,#265898,#265899,#265900,#265901,
#265902,#265903,#265904,#265905,#265906,#265907,#265908,#265909,#265910,
#265911,#265912,#265913,#265914,#265915,#265916,#265917,#265918,#265919,
#265920,#265921,#265922,#265923,#265924,#265925,#265926,#265927,#265928,
#265929,#265930,#265931,#265932,#265933,#265934,#265935,#265936,#265937,
#265938,#265939,#265940,#265941,#265942,#265943,#265944,#265945,#265946,
#265947,#265948,#265949,#265950,#265951,#265952,#265953,#265954,#265955,
#265956,#265957,#265958,#265959,#265960,#265961,#265962,#265963,#265964,
#265965,#265966,#265967,#265968,#265969,#265970,#265971,#265972,#265973,
#265974,#265975,#265976,#265977,#265978,#265979,#265980,#265981,#265982,
#265983,#265984,#265985,#265986,#265987,#265988,#265989,#265990,#265991,
#265992,#265993,#265994,#265995,#265996,#265997,#265998,#265999,#266000,
#266001,#266002,#266003,#266004,#266005,#266006,#266007,#266008,#266009,
#266010,#266011,#266012,#266013,#266014,#266015,#266016,#266017,#266018,
#266019,#266020,#266021,#266022,#266023,#266024,#266025,#266026,#266027,
#266028,#266029,#266030,#266031,#266032,#266033,#266034,#266035,#266036,
#266037,#266038,#266039,#266040,#266041,#266042,#266043,#266044,#266045,
#266046,#266047,#266048,#266049,#266050,#266051,#266052,#266053,#266054,
#266055,#266056,#266057,#266058,#266059,#266060,#266061,#266062,#266063,
#266064,#266065,#266066,#266067,#266068,#266069,#266070,#266071,#266072,
#266073,#266074,#266075,#266076,#266077,#266078,#266079,#266080,#266081,
#266082,#266083,#266084,#266085,#266086,#266087,#266088,#266089,#266090,
#266091,#266092,#266093,#266094,#266095,#266096,#266097,#266098,#266099,
#266100,#266101,#266102,#266103,#266104,#266105,#266106,#266107,#266108,
#266109,#266110,#266111,#266112,#266113,#266114,#266115,#266116,#266117,
#266118,#266119,#266120,#266121,#266122,#266123,#266124,#266125,#266126,
#266127,#266128,#266129,#266130,#266131,#266132,#266133,#266134,#266135,
#266136,#266137,#266138,#266139,#266140,#266141,#266142),.UNSPECIFIED.,
 .F.,.F.,(6,1,1,1,1,1,1,1,1,1,1,1,1,1,1,1,1,1,1,1,1,1,1,1,1,1,1,1,1,1,1,
1,1,1,1,1,1,1,1,1,1,1,1,1,1,1,1,1,1,1,1,1,1,1,1,1,1,1,1,1,1,1,1,1,1,1,1,
1,1,1,1,1,1,1,1,1,1,1,1,1,1,1,1,1,1,1,1,1,1,1,1,1,1,1,1,1,1,1,1,1,1,1,1,
1,1,1,1,1,1,1,1,1,1,1,1,1,1,1,1,1,1,1,1,1,1,1,1,1,1,1,1,1,1,1,1,1,1,1,1,
1,1,1,1,1,1,1,1,1,1,1,1,1,1,1,1,1,1,1,1,1,1,1,1,1,1,1,1,1,1,1,1,1,1,1,1,
1,1,1,1,1,1,1,1,1,1,1,1,1,1,1,1,1,1,1,1,1,1,1,1,1,1,1,1,1,1,1,1,1,1,1,1,
1,1,1,1,1,1,1,1,1,1,1,1,1,1,1,1,1,1,1,1,1,1,1,1,1,1,1,1,1,1,1,1,1,1,1,1,
1,1,1,1,1,1,1,1,1,1,1,1,1,1,1,1,1,1,1,1,1,1,1,1,1,1,1,1,1,1,1,1,1,1,1,1,
1,1,1,1,1,1,1,1,1,1,1,1,1,1,1,1,1,1,1,1,1,1,1,1,1,1,1,1,1,1,1,1,1,1,1,1,
1,1,1,1,1,1,1,1,1,1,1,1,1,1,1,1,1,1,1,1,1,1,1,1,1,1,1,1,1,1,1,1,1,1,1,1,
1,1,1,1,1,1,1,1,1,1,1,1,1,1,1,1,1,1,1,1,1,1,1,1,1,1,1,1,1,1,1,1,1,1,1,1,
1,1,1,1,1,1,1,1,1,1,1,1,1,1,1,1,1,1,1,1,1,1,1,1,1,1,1,1,1,1,1,1,1,1,1,1,
1,1,1,1,1,1,1,1,1,1,1,1,1,1,1,1,1,1,1,1,1,1,1,1,1,1,1,1,1,1,1,1,1,1,1,1,
1,1,6),(0.143172102,0.144954128,0.146788991,0.148623853,0.150458716,0.152293578,
0.15412844,0.155963303,0.157798165,0.159633028,0.16146789,0.163302752,0.165137615,
0.166972477,0.168807339,0.170642202,0.172477064,0.174311927,0.176146789,
0.177981651,0.179816514,0.181651376,0.183486239,0.185321101,0.187155963,
0.188990826,0.190825688,0.19266055,0.194495413,0.196330275,0.198165138,
0.2,0.201834862,0.203669725,0.205504587,0.20733945,0.209174312,0.211009174,
0.212844037,0.214678899,0.216513761,0.218348624,0.220183486,0.222018349,
0.223853211,0.225688073,0.227522936,0.229357798,0.231192661,0.233027523,
0.234862385,0.236697248,0.23853211,0.240366972,0.242201835,0.244036697,
0.24587156,0.247706422,0.249541284,0.251376147,0.253211009,0.255045872,
0.256880734,0.258715596,0.260550459,0.262385321,0.264220183,0.266055046,
0.267889908,0.269724771,0.271559633,0.273394495,0.275229358,0.27706422,
0.278899083,0.280733945,0.282568807,0.28440367,0.286238532,0.288073394,
0.289908257,0.291743119,0.293577982,0.295412844,0.297247706,0.299082569,
0.300917431,0.302752294,0.304587156,0.306422018,0.308256881,0.310091743,
0.311926606,0.313761468,0.31559633,0.317431193,0.319266055,0.321100917,
0.32293578,0.324770642,0.326605505,0.328440367,0.330275229,0.333944954,
0.335779817,0.337614679,0.339449541,0.341284404,0.343119266,0.344954128,
0.346788991,0.348623853,0.350458716,0.352293578,0.35412844,0.355963303,
0.357798165,0.359633028,0.36146789,0.363302752,0.365137615,0.366972477,
0.368807339,0.370642202,0.372477064,0.374311927,0.376146789,0.377981651,
0.379816514,0.381651376,0.383486239,0.385321101,0.387155963,0.388990826,
0.390825688,0.39266055,0.394495413,0.396330275,0.398165138,0.4,0.401834862,
0.403669725,0.405504587,0.40733945,0.409174312,0.411009174,0.412844037,
0.414678899,0.416513761,0.418348624,0.420183486,0.422018349,0.423853211,
0.425688073,0.427522936,0.429357798,0.431192661,0.433027523,0.434862385,
0.436697248,0.43853211,0.440366972,0.442201835,0.444036697,0.44587156,0.447706422,
0.449541284,0.451376147,0.453211009,0.455045872,0.456880734,0.458715596,
0.460550459,0.462385321,0.464220183,0.466055046,0.467889908,0.469724771,
0.471559633,0.473394495,0.475229358,0.47706422,0.478899083,0.480733945,
0.482568807,0.48440367,0.486238532,0.488073394,0.489908257,0.491743119,
0.493577982,0.495412844,0.497247706,0.499082569,0.500917431,0.502752294,
0.504587156,0.506422018,0.508256881,0.511926606,0.513761468,0.51559633,
0.517431193,0.519266055,0.521100917,0.52293578,0.524770642,0.526605505,
0.528440367,0.530275229,0.532110092,0.533944954,0.535779817,0.537614679,
0.539449541,0.541284404,0.543119266,0.544954128,0.546788991,0.548623853,
0.550458716,0.552293578,0.55412844,0.555963303,0.557798165,0.559633028,
0.56146789,0.563302752,0.565137615,0.566972477,0.568807339,0.570642202,
0.572477064,0.574311927,0.576146789,0.577981651,0.579816514,0.581651376,
0.583486239,0.585321101,0.587155963,0.588990826,0.590825688,0.59266055,
0.594495413,0.596330275,0.598165138,0.6,0.601834862,0.603669725,0.605504587,
0.60733945,0.609174312,0.611009174,0.612844037,0.614678899,0.616513761,
0.618348624,0.620183486,0.622018349,0.623853211,0.625688073,0.627522936,
0.629357798,0.631192661,0.633027523,0.634862385,0.636697248,0.63853211,
0.640366972,0.642201835,0.644036697,0.64587156,0.647706422,0.649541284,
0.651376147,0.653211009,0.655045872,0.656880734,0.658715596,0.660550459,
0.662385321,0.664220183,0.666055046,0.667889908,0.669724771,0.671559633,
0.673394495,0.675229358,0.67706422,0.678899083,0.680733945,0.682568807,
0.68440367,0.686238532,0.688073394,0.689908257,0.691743119,0.693577982,
0.695412844,0.697247706,0.699082569,0.700917431,0.702752294,0.704587156,
0.706422018,0.708256881,0.710091743,0.711926606,0.713761468,0.71559633,
0.717431193,0.719266055,0.721100917,0.72293578,0.724770642,0.726605505,
0.728440367,0.730275229,0.732110092,0.733944954,0.735779817,0.737614679,
0.739449541,0.741284404,0.743119266,0.744954128,0.746788991,0.748623853,
0.750458716,0.752293578,0.75412844,0.755963303,0.757798165,0.759633028,
0.76146789,0.763302752,0.765137615,0.766972477,0.768807339,0.770642202,
0.772477064,0.774311927,0.776146789,0.777981651,0.779816514,0.781651376,
0.783486239,0.785321101,0.787155963,0.788990826,0.790825688,0.79266055,
0.794495413,0.796330275,0.798165138,0.8,0.801834862,0.803669725,0.805504587,
0.80733945,0.809174312,0.811009174,0.812844037,0.814678899,0.816513761,
0.818348624,0.820183486,0.822018349,0.823853211,0.825688073,0.827522936,
0.829357798,0.831192661,0.833027523,0.834862385,0.836697248,0.83853211,
0.840366972,0.842201835,0.844036697,0.84587156,0.847706422,0.849541284,
0.851376147,0.853211009,0.855045872,0.856880734,0.858715596,0.860550459,
0.862385321,0.864220183,0.866055046,0.867889908,0.869724771,0.871559633,
0.873394495,0.875229358,0.87706422,0.878899083,0.880733945,0.882568807,
0.88440367,0.886238532,0.888073394,0.889908257,0.891743119,0.893577982,
0.895412844,0.897247706,0.899082569,0.900917431,0.902752294,0.904587156,
0.906422018,0.908256881,0.910091743,0.911926606,0.913761468,0.91559633,
0.917431193,0.919266055,0.921100917,0.92293578,0.924770642,0.926605505,
0.928440367,0.930275229,0.932110092,0.933944954,0.935779817,0.937614679,
0.939449541,0.941284404,0.943119266,0.944954128,0.946788991,0.948623853,
0.950458716,0.952293578,0.95412844,0.955963303,0.957798165,0.959633028,
0.96146789,0.963302752,0.965137615,0.966972477,0.968807339,0.970642202,
0.972477064,0.974311927,0.976146789,0.977981651,0.979816514,0.981651376,
0.983486239,0.985321101,0.987155963,0.988990826,0.990825688,0.99266055,
0.994495413,0.996330275,0.998165138,1.),.UNSPECIFIED.);
#24455=B_SPLINE_CURVE_WITH_KNOTS('',3,(#267102,#267103,#267104,#267105,
#267106,#267107,#267108,#267109,#267110,#267111,#267112,#267113,#267114,
#267115,#267116,#267117,#267118,#267119,#267120,#267121,#267122,#267123,
#267124,#267125,#267126,#267127,#267128,#267129,#267130,#267131,#267132,
#267133,#267134,#267135,#267136,#267137,#267138,#267139,#267140,#267141,
#267142,#267143,#267144,#267145,#267146,#267147,#267148,#267149,#267150,
#267151,#267152,#267153,#267154,#267155,#267156,#267157,#267158,#267159,
#267160,#267161,#267162,#267163,#267164,#267165,#267166,#267167,#267168,
#267169,#267170,#267171,#267172,#267173,#267174,#267175,#267176,#267177,
#267178,#267179,#267180,#267181,#267182,#267183,#267184,#267185,#267186,
#267187,#267188,#267189,#267190,#267191,#267192,#267193,#267194,#267195,
#267196,#267197,#267198,#267199,#267200,#267201,#267202,#267203,#267204,
#267205,#267206,#267207,#267208,#267209,#267210,#267211,#267212,#267213,
#267214,#267215,#267216,#267217,#267218,#267219,#267220,#267221,#267222,
#267223,#267224,#267225,#267226,#267227,#267228,#267229,#267230,#267231,
#267232,#267233,#267234,#267235,#267236,#267237,#267238,#267239,#267240,
#267241,#267242,#267243,#267244,#267245,#267246,#267247,#267248,#267249,
#267250,#267251,#267252,#267253,#267254,#267255,#267256,#267257,#267258,
#267259,#267260,#267261,#267262,#267263,#267264,#267265,#267266,#267267,
#267268,#267269,#267270,#267271,#267272,#267273,#267274,#267275,#267276,
#267277,#267278,#267279,#267280,#267281,#267282,#267283,#267284,#267285,
#267286,#267287,#267288,#267289,#267290,#267291,#267292,#267293,#267294,
#267295,#267296,#267297,#267298,#267299,#267300,#267301,#267302,#267303,
#267304,#267305,#267306,#267307,#267308,#267309,#267310,#267311,#267312,
#267313,#267314,#267315,#267316,#267317,#267318,#267319,#267320,#267321,
#267322,#267323,#267324,#267325,#267326,#267327,#267328,#267329,#267330,
#267331,#267332,#267333,#267334,#267335,#267336,#267337,#267338,#267339,
#267340,#267341,#267342,#267343,#267344,#267345,#267346,#267347,#267348,
#267349,#267350,#267351,#267352,#267353,#267354,#267355,#267356,#267357,
#267358,#267359,#267360,#267361,#267362,#267363,#267364,#267365,#267366,
#267367,#267368,#267369,#267370,#267371,#267372,#267373,#267374,#267375,
#267376,#267377,#267378,#267379,#267380,#267381,#267382,#267383,#267384,
#267385,#267386,#267387,#267388,#267389,#267390,#267391,#267392,#267393,
#267394,#267395,#267396,#267397,#267398,#267399,#267400,#267401,#267402,
#267403,#267404,#267405,#267406,#267407,#267408,#267409,#267410,#267411,
#267412,#267413,#267414),.UNSPECIFIED.,.F.,.F.,(4,3,3,3,3,3,3,3,3,3,3,3,
3,3,3,3,3,3,3,3,3,3,3,3,3,3,3,3,3,3,3,3,3,3,3,3,3,3,3,3,3,3,3,3,3,3,3,3,
3,3,3,3,3,3,3,3,3,3,3,3,3,3,3,3,3,3,3,3,3,3,3,3,3,3,3,3,3,3,3,3,3,3,3,3,
3,3,3,3,3,3,3,3,3,3,3,3,3,3,3,3,3,3,3,3,4),(0.143172102,0.15412844,0.165137615,
0.176146789,0.187155963,0.198165138,0.209174312,0.222018349,0.233027523,
0.244036697,0.255045872,0.266055046,0.27706422,0.288073394,0.299082569,
0.310091743,0.32293578,0.333944954,0.344954128,0.355963303,0.368807339,
0.379816514,0.390825688,0.4,0.409174312,0.418348624,0.429357798,0.43853211,
0.447706422,0.458715596,0.467889908,0.478899083,0.488073394,0.497247706,
0.506422018,0.517431193,0.526605505,0.535779817,0.544954128,0.552293578,
0.559633028,0.566972477,0.574311927,0.581651376,0.588990826,0.596330275,
0.603669725,0.611009174,0.618348624,0.627522936,0.634862385,0.642201835,
0.649541284,0.658715596,0.666055046,0.675229358,0.68440367,0.693577982,
0.700917431,0.711926606,0.719266055,0.726605505,0.735779817,0.743119266,
0.750458716,0.759633028,0.766972477,0.774311927,0.781651376,0.788990826,
0.798165138,0.80733945,0.812844037,0.818348624,0.823853211,0.829357798,
0.834862385,0.840366972,0.84587156,0.851376147,0.856880734,0.862385321,
0.869724771,0.875229358,0.880733945,0.886238532,0.891743119,0.897247706,
0.902752294,0.908256881,0.913761468,0.919266055,0.926605505,0.932110092,
0.937614679,0.943119266,0.948623853,0.95412844,0.963302752,0.968807339,
0.976146789,0.983486239,0.988990826,0.994495413,1.),.UNSPECIFIED.);
#24456=B_SPLINE_CURVE_WITH_KNOTS('',3,(#267415,#267416,#267417,#267418,
#267419,#267420,#267421,#267422,#267423,#267424,#267425,#267426,#267427,
#267428,#267429,#267430,#267431,#267432,#267433,#267434,#267435,#267436,
#267437,#267438,#267439,#267440,#267441,#267442,#267443,#267444,#267445,
#267446,#267447,#267448,#267449,#267450,#267451,#267452,#267453,#267454,
#267455,#267456,#267457,#267458,#267459,#267460,#267461,#267462,#267463,
#267464,#267465,#267466,#267467,#267468,#267469,#267470,#267471,#267472,
#267473,#267474,#267475,#267476,#267477,#267478,#267479,#267480,#267481,
#267482,#267483,#267484,#267485,#267486,#267487,#267488,#267489,#267490,
#267491,#267492,#267493,#267494,#267495,#267496,#267497,#267498,#267499,
#267500,#267501,#267502,#267503,#267504,#267505,#267506,#267507,#267508,
#267509,#267510,#267511,#267512,#267513,#267514,#267515,#267516,#267517,
#267518,#267519,#267520,#267521,#267522,#267523,#267524,#267525,#267526,
#267527,#267528,#267529,#267530,#267531,#267532,#267533,#267534,#267535,
#267536,#267537,#267538,#267539,#267540,#267541,#267542,#267543,#267544,
#267545,#267546,#267547,#267548,#267549,#267550,#267551,#267552,#267553,
#267554,#267555,#267556,#267557,#267558,#267559,#267560,#267561,#267562,
#267563,#267564,#267565,#267566,#267567,#267568,#267569,#267570,#267571,
#267572,#267573,#267574,#267575,#267576,#267577,#267578,#267579,#267580,
#267581,#267582,#267583,#267584,#267585,#267586,#267587,#267588,#267589,
#267590,#267591,#267592,#267593,#267594,#267595,#267596,#267597,#267598,
#267599,#267600,#267601,#267602,#267603,#267604,#267605,#267606,#267607,
#267608,#267609,#267610,#267611,#267612,#267613,#267614,#267615,#267616,
#267617,#267618,#267619,#267620,#267621,#267622,#267623,#267624,#267625,
#267626,#267627,#267628,#267629,#267630,#267631,#267632,#267633,#267634,
#267635,#267636,#267637,#267638,#267639,#267640,#267641,#267642,#267643,
#267644,#267645,#267646,#267647,#267648,#267649,#267650,#267651,#267652,
#267653,#267654,#267655,#267656,#267657,#267658,#267659,#267660,#267661,
#267662,#267663,#267664,#267665,#267666,#267667,#267668,#267669,#267670,
#267671,#267672,#267673,#267674,#267675,#267676,#267677,#267678,#267679,
#267680,#267681,#267682,#267683,#267684,#267685,#267686,#267687,#267688,
#267689,#267690,#267691,#267692,#267693,#267694,#267695,#267696,#267697,
#267698,#267699,#267700,#267701,#267702,#267703,#267704,#267705,#267706,
#267707,#267708,#267709,#267710,#267711,#267712,#267713,#267714,#267715,
#267716,#267717,#267718,#267719,#267720,#267721,#267722,#267723,#267724,
#267725,#267726,#267727,#267728,#267729,#267730,#267731,#267732,#267733,
#267734,#267735,#267736,#267737,#267738,#267739,#267740,#267741,#267742),
 .UNSPECIFIED.,.F.,.F.,(4,3,3,3,3,3,3,3,3,3,3,3,3,3,3,3,3,3,3,3,3,3,3,3,
3,3,3,3,3,3,3,3,3,3,3,3,3,3,3,3,3,3,3,3,3,3,3,3,3,3,3,3,3,3,3,3,3,3,3,3,
3,3,3,3,3,3,3,3,3,3,3,3,3,3,3,3,3,3,3,3,3,3,3,3,3,3,3,3,3,3,3,3,3,3,3,3,
3,3,3,3,3,3,3,3,3,3,3,3,3,4),(0.143172102,0.15412844,0.165137615,0.176146789,
0.187155963,0.198165138,0.209174312,0.220183486,0.231192661,0.242201835,
0.253211009,0.266055046,0.27706422,0.288073394,0.299082569,0.310091743,
0.321100917,0.332110092,0.343119266,0.355963303,0.366972477,0.377981651,
0.388990826,0.398165138,0.40733945,0.416513761,0.425688073,0.434862385,
0.444036697,0.453211009,0.462385321,0.471559633,0.480733945,0.489908257,
0.499082569,0.508256881,0.517431193,0.526605505,0.533944954,0.541284404,
0.548623853,0.555963303,0.563302752,0.570642202,0.579816514,0.587155963,
0.594495413,0.601834862,0.609174312,0.616513761,0.623853211,0.631192661,
0.63853211,0.64587156,0.653211009,0.660550459,0.667889908,0.675229358,0.682568807,
0.689908257,0.697247706,0.704587156,0.711926606,0.719266055,0.726605505,
0.733944954,0.743119266,0.750458716,0.757798165,0.765137615,0.772477064,
0.779816514,0.787155963,0.794495413,0.801834862,0.809174312,0.814678899,
0.820183486,0.825688073,0.831192661,0.836697248,0.842201835,0.849541284,
0.855045872,0.860550459,0.866055046,0.871559633,0.87706422,0.882568807,
0.888073394,0.893577982,0.899082569,0.904587156,0.910091743,0.91559633,
0.921100917,0.926605505,0.932110092,0.937614679,0.943119266,0.948623853,
0.95412844,0.959633028,0.965137615,0.972477064,0.977981651,0.983486239,
0.988990826,0.994495413,1.),.UNSPECIFIED.);
#24457=B_SPLINE_CURVE_WITH_KNOTS('',5,(#268690,#268691,#268692,#268693,
#268694,#268695,#268696,#268697,#268698,#268699,#268700,#268701,#268702,
#268703,#268704,#268705,#268706,#268707,#268708,#268709,#268710,#268711,
#268712,#268713,#268714,#268715,#268716,#268717,#268718,#268719,#268720,
#268721,#268722,#268723,#268724,#268725,#268726,#268727,#268728,#268729,
#268730,#268731,#268732,#268733,#268734,#268735,#268736,#268737,#268738,
#268739,#268740,#268741,#268742,#268743,#268744,#268745,#268746,#268747,
#268748,#268749,#268750,#268751,#268752,#268753,#268754,#268755,#268756,
#268757,#268758,#268759,#268760,#268761,#268762,#268763,#268764,#268765,
#268766,#268767,#268768,#268769,#268770,#268771,#268772,#268773,#268774,
#268775,#268776,#268777,#268778,#268779,#268780,#268781,#268782,#268783,
#268784,#268785,#268786,#268787,#268788,#268789,#268790,#268791,#268792,
#268793,#268794,#268795,#268796,#268797,#268798,#268799,#268800,#268801,
#268802,#268803,#268804,#268805,#268806,#268807,#268808,#268809,#268810,
#268811,#268812,#268813,#268814,#268815,#268816,#268817,#268818,#268819,
#268820,#268821,#268822,#268823,#268824,#268825,#268826,#268827,#268828,
#268829,#268830,#268831,#268832,#268833,#268834,#268835,#268836,#268837,
#268838,#268839,#268840,#268841,#268842,#268843,#268844,#268845,#268846,
#268847,#268848,#268849,#268850,#268851,#268852,#268853,#268854,#268855,
#268856,#268857,#268858,#268859,#268860,#268861,#268862,#268863,#268864,
#268865,#268866,#268867,#268868,#268869,#268870,#268871,#268872,#268873,
#268874,#268875,#268876,#268877,#268878,#268879,#268880,#268881,#268882,
#268883,#268884,#268885,#268886,#268887,#268888,#268889,#268890,#268891,
#268892,#268893,#268894,#268895,#268896,#268897,#268898,#268899,#268900,
#268901,#268902,#268903,#268904,#268905,#268906,#268907,#268908,#268909,
#268910,#268911,#268912,#268913,#268914,#268915,#268916,#268917,#268918,
#268919,#268920,#268921,#268922,#268923,#268924,#268925,#268926,#268927,
#268928,#268929,#268930,#268931,#268932,#268933,#268934,#268935,#268936,
#268937,#268938,#268939,#268940,#268941,#268942,#268943,#268944,#268945,
#268946,#268947,#268948,#268949,#268950,#268951,#268952,#268953,#268954,
#268955,#268956,#268957,#268958,#268959,#268960,#268961,#268962,#268963,
#268964,#268965,#268966,#268967,#268968,#268969,#268970,#268971,#268972,
#268973,#268974,#268975,#268976,#268977,#268978,#268979,#268980,#268981,
#268982,#268983,#268984,#268985,#268986,#268987,#268988,#268989,#268990,
#268991,#268992,#268993,#268994,#268995,#268996,#268997,#268998,#268999,
#269000,#269001,#269002,#269003,#269004,#269005,#269006,#269007,#269008,
#269009,#269010,#269011,#269012,#269013,#269014,#269015,#269016,#269017,
#269018,#269019,#269020,#269021,#269022,#269023,#269024,#269025,#269026,
#269027,#269028,#269029,#269030,#269031,#269032,#269033,#269034,#269035,
#269036,#269037,#269038,#269039,#269040,#269041,#269042,#269043,#269044,
#269045,#269046,#269047,#269048,#269049,#269050,#269051,#269052,#269053,
#269054,#269055,#269056,#269057,#269058,#269059,#269060,#269061,#269062,
#269063,#269064,#269065,#269066,#269067,#269068,#269069,#269070,#269071,
#269072,#269073,#269074,#269075,#269076,#269077,#269078,#269079,#269080,
#269081,#269082,#269083,#269084,#269085,#269086,#269087,#269088,#269089,
#269090,#269091,#269092,#269093,#269094,#269095,#269096,#269097,#269098,
#269099,#269100,#269101,#269102,#269103,#269104,#269105,#269106,#269107,
#269108,#269109,#269110,#269111,#269112,#269113,#269114,#269115,#269116,
#269117,#269118,#269119,#269120,#269121,#269122,#269123,#269124,#269125,
#269126,#269127,#269128,#269129,#269130,#269131,#269132,#269133,#269134,
#269135,#269136,#269137,#269138,#269139,#269140,#269141,#269142,#269143,
#269144,#269145,#269146,#269147,#269148,#269149,#269150,#269151,#269152,
#269153,#269154,#269155,#269156,#269157,#269158,#269159,#269160),
 .UNSPECIFIED.,.F.,.F.,(6,1,1,1,1,1,1,1,1,1,1,1,1,1,1,1,1,1,1,1,1,1,1,1,
1,1,1,1,1,1,1,1,1,1,1,1,1,1,1,1,1,1,1,1,1,1,1,1,1,1,1,1,1,1,1,1,1,1,1,1,
1,1,1,1,1,1,1,1,1,1,1,1,1,1,1,1,1,1,1,1,1,1,1,1,1,1,1,1,1,1,1,1,1,1,1,1,
1,1,1,1,1,1,1,1,1,1,1,1,1,1,1,1,1,1,1,1,1,1,1,1,1,1,1,1,1,1,1,1,1,1,1,1,
1,1,1,1,1,1,1,1,1,1,1,1,1,1,1,1,1,1,1,1,1,1,1,1,1,1,1,1,1,1,1,1,1,1,1,1,
1,1,1,1,1,1,1,1,1,1,1,1,1,1,1,1,1,1,1,1,1,1,1,1,1,1,1,1,1,1,1,1,1,1,1,1,
1,1,1,1,1,1,1,1,1,1,1,1,1,1,1,1,1,1,1,1,1,1,1,1,1,1,1,1,1,1,1,1,1,1,1,1,
1,1,1,1,1,1,1,1,1,1,1,1,1,1,1,1,1,1,1,1,1,1,1,1,1,1,1,1,1,1,1,1,1,1,1,1,
1,1,1,1,1,1,1,1,1,1,1,1,1,1,1,1,1,1,1,1,1,1,1,1,1,1,1,1,1,1,1,1,1,1,1,1,
1,1,1,1,1,1,1,1,1,1,1,1,1,1,1,1,1,1,1,1,1,1,1,1,1,1,1,1,1,1,1,1,1,1,1,1,
1,1,1,1,1,1,1,1,1,1,1,1,1,1,1,1,1,1,1,1,1,1,1,1,1,1,1,1,1,1,1,1,1,1,1,1,
1,1,1,1,1,1,1,1,1,1,1,1,1,1,1,1,1,1,1,1,1,1,1,1,1,1,1,1,1,1,1,1,1,1,1,1,
1,1,1,1,1,1,1,1,1,1,1,1,1,1,1,1,1,1,1,1,1,1,1,1,1,1,1,1,1,1,1,1,1,1,1,1,
1,1,1,1,1,1,1,1,1,1,6),(-1.,-0.998165138,-0.996330275,-0.994495413,-0.99266055,
-0.990825688,-0.988990826,-0.987155963,-0.985321101,-0.983486239,-0.981651376,
-0.979816514,-0.977981651,-0.976146789,-0.974311927,-0.972477064,-0.970642202,
-0.968807339,-0.966972477,-0.965137615,-0.963302752,-0.96146789,-0.959633028,
-0.957798165,-0.955963303,-0.95412844,-0.952293578,-0.950458716,-0.948623853,
-0.946788991,-0.944954128,-0.943119266,-0.941284404,-0.939449541,-0.937614679,
-0.935779817,-0.933944954,-0.932110092,-0.930275229,-0.928440367,-0.926605505,
-0.924770642,-0.92293578,-0.921100917,-0.919266055,-0.917431193,-0.91559633,
-0.913761468,-0.911926606,-0.910091743,-0.908256881,-0.906422018,-0.904587156,
-0.902752294,-0.900917431,-0.899082569,-0.897247706,-0.895412844,-0.893577982,
-0.891743119,-0.889908257,-0.888073394,-0.886238532,-0.88440367,-0.882568807,
-0.880733945,-0.878899083,-0.87706422,-0.875229358,-0.873394495,-0.871559633,
-0.869724771,-0.867889908,-0.866055046,-0.864220183,-0.862385321,-0.860550459,
-0.858715596,-0.856880734,-0.855045872,-0.853211009,-0.851376147,-0.849541284,
-0.847706422,-0.84587156,-0.844036697,-0.842201835,-0.840366972,-0.83853211,
-0.836697248,-0.834862385,-0.833027523,-0.831192661,-0.829357798,-0.827522936,
-0.825688073,-0.823853211,-0.822018349,-0.820183486,-0.818348624,-0.816513761,
-0.814678899,-0.812844037,-0.811009174,-0.809174312,-0.80733945,-0.805504587,
-0.803669725,-0.801834862,-0.8,-0.798165138,-0.796330275,-0.794495413,-0.79266055,
-0.790825688,-0.788990826,-0.787155963,-0.785321101,-0.783486239,-0.781651376,
-0.779816514,-0.777981651,-0.776146789,-0.774311927,-0.772477064,-0.770642202,
-0.768807339,-0.766972477,-0.765137615,-0.763302752,-0.76146789,-0.759633028,
-0.757798165,-0.755963303,-0.75412844,-0.752293578,-0.750458716,-0.748623853,
-0.746788991,-0.744954128,-0.743119266,-0.741284404,-0.739449541,-0.737614679,
-0.735779817,-0.733944954,-0.732110092,-0.730275229,-0.728440367,-0.726605505,
-0.724770642,-0.72293578,-0.721100917,-0.719266055,-0.717431193,-0.71559633,
-0.713761468,-0.711926606,-0.710091743,-0.708256881,-0.706422018,-0.704587156,
-0.702752294,-0.700917431,-0.699082569,-0.697247706,-0.695412844,-0.693577982,
-0.691743119,-0.689908257,-0.688073394,-0.686238532,-0.68440367,-0.682568807,
-0.680733945,-0.678899083,-0.67706422,-0.675229358,-0.673394495,-0.671559633,
-0.669724771,-0.667889908,-0.666055046,-0.664220183,-0.662385321,-0.660550459,
-0.658715596,-0.656880734,-0.655045872,-0.653211009,-0.651376147,-0.649541284,
-0.647706422,-0.64587156,-0.644036697,-0.640366972,-0.63853211,-0.636697248,
-0.634862385,-0.633027523,-0.631192661,-0.629357798,-0.627522936,-0.625688073,
-0.623853211,-0.622018349,-0.620183486,-0.618348624,-0.616513761,-0.614678899,
-0.612844037,-0.611009174,-0.609174312,-0.60733945,-0.605504587,-0.603669725,
-0.601834862,-0.6,-0.598165138,-0.596330275,-0.594495413,-0.59266055,-0.590825688,
-0.588990826,-0.587155963,-0.585321101,-0.583486239,-0.581651376,-0.579816514,
-0.577981651,-0.576146789,-0.574311927,-0.572477064,-0.570642202,-0.568807339,
-0.566972477,-0.565137615,-0.563302752,-0.56146789,-0.559633028,-0.557798165,
-0.555963303,-0.55412844,-0.552293578,-0.550458716,-0.548623853,-0.546788991,
-0.544954128,-0.543119266,-0.541284404,-0.539449541,-0.537614679,-0.535779817,
-0.533944954,-0.532110092,-0.530275229,-0.528440367,-0.526605505,-0.524770642,
-0.52293578,-0.521100917,-0.519266055,-0.517431193,-0.51559633,-0.513761468,
-0.511926606,-0.510091743,-0.508256881,-0.506422018,-0.504587156,-0.502752294,
-0.500917431,-0.499082569,-0.497247706,-0.495412844,-0.493577982,-0.491743119,
-0.489908257,-0.488073394,-0.486238532,-0.48440367,-0.482568807,-0.480733945,
-0.478899083,-0.47706422,-0.475229358,-0.473394495,-0.471559633,-0.469724771,
-0.467889908,-0.466055046,-0.464220183,-0.462385321,-0.460550459,-0.458715596,
-0.456880734,-0.455045872,-0.453211009,-0.451376147,-0.449541284,-0.447706422,
-0.44587156,-0.444036697,-0.442201835,-0.440366972,-0.43853211,-0.436697248,
-0.434862385,-0.433027523,-0.431192661,-0.429357798,-0.427522936,-0.425688073,
-0.423853211,-0.422018349,-0.420183486,-0.418348624,-0.416513761,-0.414678899,
-0.412844037,-0.411009174,-0.409174312,-0.40733945,-0.405504587,-0.403669725,
-0.401834862,-0.4,-0.398165138,-0.396330275,-0.394495413,-0.39266055,-0.390825688,
-0.388990826,-0.387155963,-0.385321101,-0.383486239,-0.381651376,-0.379816514,
-0.377981651,-0.376146789,-0.374311927,-0.372477064,-0.370642202,-0.368807339,
-0.366972477,-0.365137615,-0.363302752,-0.36146789,-0.359633028,-0.357798165,
-0.355963303,-0.35412844,-0.352293578,-0.350458716,-0.348623853,-0.346788991,
-0.344954128,-0.343119266,-0.341284404,-0.339449541,-0.337614679,-0.335779817,
-0.333944954,-0.332110092,-0.330275229,-0.328440367,-0.326605505,-0.324770642,
-0.32293578,-0.321100917,-0.319266055,-0.317431193,-0.31559633,-0.313761468,
-0.311926606,-0.310091743,-0.308256881,-0.306422018,-0.304587156,-0.302752294,
-0.300917431,-0.299082569,-0.297247706,-0.295412844,-0.293577982,-0.291743119,
-0.289908257,-0.288073394,-0.286238532,-0.28440367,-0.282568807,-0.280733945,
-0.278899083,-0.27706422,-0.275229358,-0.273394495,-0.271559633,-0.269724771,
-0.267889908,-0.266055046,-0.264220183,-0.262385321,-0.260550459,-0.258715596,
-0.256880734,-0.255045872,-0.253211009,-0.251376147,-0.249541284,-0.247706422,
-0.24587156,-0.244036697,-0.242201835,-0.240366972,-0.23853211,-0.236697248,
-0.234862385,-0.233027523,-0.231192661,-0.229357798,-0.227522936,-0.225688073,
-0.223853211,-0.222018349,-0.220183486,-0.218348624,-0.216513761,-0.214678899,
-0.212844037,-0.211009174,-0.209174312,-0.20733945,-0.205504587,-0.203669725,
-0.201834862,-0.2,-0.198165138,-0.196330275,-0.194495413,-0.19266055,-0.190825688,
-0.188990826,-0.187155963,-0.185321101,-0.183486239,-0.181651376,-0.179816514,
-0.177981651,-0.176146789,-0.174311927,-0.172477064,-0.170642202,-0.168807339,
-0.166972477,-0.165137615,-0.163302752,-0.16146789,-0.159633028,-0.157798165,
-0.155963303,-0.15412844,-0.152293578,-0.150458716,-0.148623853,-0.146788991,
-0.144954128,-0.143172102),.UNSPECIFIED.);
#24458=B_SPLINE_CURVE_WITH_KNOTS('',5,(#269161,#269162,#269163,#269164,
#269165,#269166,#269167,#269168,#269169,#269170,#269171,#269172,#269173,
#269174,#269175,#269176,#269177,#269178,#269179,#269180,#269181,#269182,
#269183,#269184,#269185,#269186,#269187,#269188,#269189,#269190,#269191,
#269192,#269193,#269194,#269195,#269196,#269197,#269198,#269199,#269200,
#269201,#269202,#269203,#269204,#269205,#269206,#269207,#269208,#269209,
#269210,#269211,#269212,#269213,#269214,#269215,#269216,#269217,#269218,
#269219,#269220,#269221,#269222,#269223,#269224,#269225,#269226,#269227,
#269228,#269229,#269230,#269231,#269232,#269233,#269234,#269235,#269236,
#269237,#269238,#269239,#269240,#269241,#269242,#269243,#269244,#269245,
#269246,#269247,#269248,#269249,#269250,#269251,#269252,#269253,#269254,
#269255,#269256,#269257,#269258,#269259,#269260,#269261,#269262,#269263,
#269264,#269265,#269266,#269267,#269268,#269269,#269270,#269271,#269272,
#269273,#269274,#269275,#269276,#269277,#269278,#269279,#269280,#269281,
#269282,#269283,#269284,#269285,#269286,#269287,#269288,#269289,#269290,
#269291,#269292,#269293,#269294,#269295,#269296,#269297,#269298,#269299,
#269300,#269301,#269302,#269303,#269304,#269305,#269306,#269307,#269308,
#269309,#269310,#269311,#269312,#269313,#269314,#269315,#269316,#269317,
#269318,#269319,#269320,#269321,#269322,#269323,#269324,#269325,#269326,
#269327,#269328,#269329,#269330,#269331,#269332,#269333,#269334,#269335,
#269336,#269337,#269338,#269339,#269340,#269341,#269342,#269343,#269344,
#269345,#269346,#269347,#269348,#269349,#269350,#269351,#269352,#269353,
#269354,#269355,#269356,#269357,#269358,#269359,#269360,#269361,#269362,
#269363,#269364,#269365,#269366,#269367,#269368,#269369,#269370,#269371,
#269372,#269373,#269374,#269375,#269376,#269377,#269378,#269379,#269380,
#269381,#269382,#269383,#269384,#269385,#269386,#269387,#269388,#269389,
#269390,#269391,#269392,#269393,#269394,#269395,#269396,#269397,#269398,
#269399,#269400,#269401,#269402,#269403,#269404,#269405,#269406,#269407,
#269408,#269409,#269410,#269411,#269412,#269413,#269414,#269415,#269416,
#269417,#269418,#269419,#269420,#269421,#269422,#269423,#269424,#269425,
#269426,#269427,#269428,#269429,#269430,#269431,#269432,#269433,#269434,
#269435,#269436,#269437,#269438,#269439,#269440,#269441,#269442,#269443,
#269444,#269445,#269446,#269447,#269448,#269449,#269450,#269451,#269452,
#269453,#269454,#269455,#269456,#269457,#269458,#269459,#269460,#269461,
#269462,#269463,#269464,#269465,#269466,#269467,#269468,#269469,#269470,
#269471,#269472,#269473,#269474,#269475,#269476,#269477,#269478,#269479,
#269480,#269481,#269482,#269483,#269484,#269485,#269486,#269487,#269488,
#269489,#269490,#269491,#269492,#269493,#269494,#269495,#269496,#269497,
#269498,#269499,#269500,#269501,#269502,#269503,#269504,#269505,#269506,
#269507,#269508,#269509,#269510,#269511,#269512,#269513,#269514,#269515,
#269516,#269517,#269518,#269519,#269520,#269521,#269522,#269523,#269524,
#269525,#269526,#269527,#269528,#269529,#269530,#269531,#269532,#269533,
#269534,#269535,#269536,#269537,#269538,#269539,#269540,#269541,#269542,
#269543,#269544,#269545,#269546,#269547,#269548,#269549,#269550,#269551,
#269552,#269553,#269554,#269555,#269556,#269557,#269558,#269559,#269560,
#269561,#269562,#269563,#269564,#269565,#269566,#269567,#269568,#269569,
#269570,#269571,#269572,#269573,#269574,#269575,#269576,#269577,#269578,
#269579,#269580,#269581,#269582,#269583,#269584,#269585,#269586,#269587,
#269588,#269589,#269590,#269591,#269592,#269593,#269594,#269595,#269596,
#269597,#269598,#269599,#269600,#269601,#269602,#269603,#269604,#269605,
#269606,#269607,#269608,#269609,#269610,#269611,#269612,#269613,#269614,
#269615,#269616,#269617,#269618,#269619,#269620,#269621,#269622,#269623,
#269624,#269625,#269626,#269627,#269628,#269629,#269630,#269631),
 .UNSPECIFIED.,.F.,.F.,(6,1,1,1,1,1,1,1,1,1,1,1,1,1,1,1,1,1,1,1,1,1,1,1,
1,1,1,1,1,1,1,1,1,1,1,1,1,1,1,1,1,1,1,1,1,1,1,1,1,1,1,1,1,1,1,1,1,1,1,1,
1,1,1,1,1,1,1,1,1,1,1,1,1,1,1,1,1,1,1,1,1,1,1,1,1,1,1,1,1,1,1,1,1,1,1,1,
1,1,1,1,1,1,1,1,1,1,1,1,1,1,1,1,1,1,1,1,1,1,1,1,1,1,1,1,1,1,1,1,1,1,1,1,
1,1,1,1,1,1,1,1,1,1,1,1,1,1,1,1,1,1,1,1,1,1,1,1,1,1,1,1,1,1,1,1,1,1,1,1,
1,1,1,1,1,1,1,1,1,1,1,1,1,1,1,1,1,1,1,1,1,1,1,1,1,1,1,1,1,1,1,1,1,1,1,1,
1,1,1,1,1,1,1,1,1,1,1,1,1,1,1,1,1,1,1,1,1,1,1,1,1,1,1,1,1,1,1,1,1,1,1,1,
1,1,1,1,1,1,1,1,1,1,1,1,1,1,1,1,1,1,1,1,1,1,1,1,1,1,1,1,1,1,1,1,1,1,1,1,
1,1,1,1,1,1,1,1,1,1,1,1,1,1,1,1,1,1,1,1,1,1,1,1,1,1,1,1,1,1,1,1,1,1,1,1,
1,1,1,1,1,1,1,1,1,1,1,1,1,1,1,1,1,1,1,1,1,1,1,1,1,1,1,1,1,1,1,1,1,1,1,1,
1,1,1,1,1,1,1,1,1,1,1,1,1,1,1,1,1,1,1,1,1,1,1,1,1,1,1,1,1,1,1,1,1,1,1,1,
1,1,1,1,1,1,1,1,1,1,1,1,1,1,1,1,1,1,1,1,1,1,1,1,1,1,1,1,1,1,1,1,1,1,1,1,
1,1,1,1,1,1,1,1,1,1,1,1,1,1,1,1,1,1,1,1,1,1,1,1,1,1,1,1,1,1,1,1,1,1,1,1,
1,1,1,1,1,1,1,1,1,1,6),(0.143172102,0.144954128,0.146788991,0.148623853,
0.150458716,0.152293578,0.15412844,0.155963303,0.157798165,0.159633028,
0.16146789,0.163302752,0.165137615,0.166972477,0.168807339,0.170642202,
0.172477064,0.174311927,0.176146789,0.177981651,0.179816514,0.181651376,
0.183486239,0.185321101,0.187155963,0.188990826,0.190825688,0.19266055,
0.194495413,0.196330275,0.198165138,0.2,0.201834862,0.203669725,0.205504587,
0.20733945,0.209174312,0.211009174,0.212844037,0.214678899,0.216513761,
0.218348624,0.220183486,0.222018349,0.223853211,0.225688073,0.227522936,
0.229357798,0.231192661,0.233027523,0.234862385,0.236697248,0.23853211,
0.240366972,0.242201835,0.244036697,0.24587156,0.247706422,0.249541284,
0.251376147,0.253211009,0.255045872,0.256880734,0.258715596,0.260550459,
0.262385321,0.264220183,0.266055046,0.267889908,0.269724771,0.271559633,
0.273394495,0.275229358,0.27706422,0.278899083,0.280733945,0.282568807,
0.28440367,0.286238532,0.288073394,0.289908257,0.291743119,0.293577982,
0.295412844,0.297247706,0.299082569,0.300917431,0.302752294,0.304587156,
0.306422018,0.308256881,0.310091743,0.311926606,0.313761468,0.31559633,
0.317431193,0.319266055,0.321100917,0.32293578,0.324770642,0.326605505,
0.328440367,0.330275229,0.332110092,0.333944954,0.335779817,0.337614679,
0.339449541,0.341284404,0.343119266,0.344954128,0.346788991,0.348623853,
0.350458716,0.352293578,0.35412844,0.355963303,0.357798165,0.359633028,
0.36146789,0.363302752,0.365137615,0.366972477,0.368807339,0.370642202,
0.372477064,0.374311927,0.376146789,0.377981651,0.379816514,0.381651376,
0.383486239,0.385321101,0.387155963,0.388990826,0.390825688,0.39266055,
0.394495413,0.396330275,0.398165138,0.4,0.401834862,0.403669725,0.405504587,
0.40733945,0.409174312,0.411009174,0.412844037,0.414678899,0.416513761,
0.418348624,0.420183486,0.422018349,0.423853211,0.425688073,0.427522936,
0.429357798,0.431192661,0.433027523,0.434862385,0.436697248,0.43853211,
0.440366972,0.442201835,0.444036697,0.44587156,0.447706422,0.449541284,
0.451376147,0.453211009,0.455045872,0.456880734,0.458715596,0.460550459,
0.462385321,0.464220183,0.466055046,0.467889908,0.469724771,0.471559633,
0.473394495,0.475229358,0.47706422,0.478899083,0.480733945,0.482568807,
0.48440367,0.486238532,0.488073394,0.489908257,0.491743119,0.493577982,
0.495412844,0.497247706,0.499082569,0.500917431,0.502752294,0.504587156,
0.506422018,0.508256881,0.510091743,0.511926606,0.513761468,0.51559633,
0.517431193,0.519266055,0.521100917,0.52293578,0.524770642,0.526605505,
0.528440367,0.530275229,0.532110092,0.533944954,0.535779817,0.537614679,
0.539449541,0.541284404,0.543119266,0.544954128,0.546788991,0.548623853,
0.550458716,0.552293578,0.55412844,0.555963303,0.557798165,0.559633028,
0.56146789,0.563302752,0.565137615,0.566972477,0.568807339,0.570642202,
0.572477064,0.574311927,0.576146789,0.577981651,0.579816514,0.581651376,
0.583486239,0.585321101,0.587155963,0.588990826,0.590825688,0.59266055,
0.594495413,0.596330275,0.598165138,0.6,0.601834862,0.603669725,0.605504587,
0.60733945,0.609174312,0.611009174,0.612844037,0.614678899,0.616513761,
0.618348624,0.620183486,0.622018349,0.623853211,0.625688073,0.627522936,
0.629357798,0.631192661,0.633027523,0.634862385,0.636697248,0.63853211,
0.640366972,0.644036697,0.64587156,0.647706422,0.649541284,0.651376147,
0.653211009,0.655045872,0.656880734,0.658715596,0.660550459,0.662385321,
0.664220183,0.666055046,0.667889908,0.669724771,0.671559633,0.673394495,
0.675229358,0.67706422,0.678899083,0.680733945,0.682568807,0.68440367,0.686238532,
0.688073394,0.689908257,0.691743119,0.693577982,0.695412844,0.697247706,
0.699082569,0.700917431,0.702752294,0.704587156,0.706422018,0.708256881,
0.710091743,0.711926606,0.713761468,0.71559633,0.717431193,0.719266055,
0.721100917,0.72293578,0.724770642,0.726605505,0.728440367,0.730275229,
0.732110092,0.733944954,0.735779817,0.737614679,0.739449541,0.741284404,
0.743119266,0.744954128,0.746788991,0.748623853,0.750458716,0.752293578,
0.75412844,0.755963303,0.757798165,0.759633028,0.76146789,0.763302752,0.765137615,
0.766972477,0.768807339,0.770642202,0.772477064,0.774311927,0.776146789,
0.777981651,0.779816514,0.781651376,0.783486239,0.785321101,0.787155963,
0.788990826,0.790825688,0.79266055,0.794495413,0.796330275,0.798165138,
0.8,0.801834862,0.803669725,0.805504587,0.80733945,0.809174312,0.811009174,
0.812844037,0.814678899,0.816513761,0.818348624,0.820183486,0.822018349,
0.823853211,0.825688073,0.827522936,0.829357798,0.831192661,0.833027523,
0.834862385,0.836697248,0.83853211,0.840366972,0.842201835,0.844036697,
0.84587156,0.847706422,0.849541284,0.851376147,0.853211009,0.855045872,
0.856880734,0.858715596,0.860550459,0.862385321,0.864220183,0.866055046,
0.867889908,0.869724771,0.871559633,0.873394495,0.875229358,0.87706422,
0.878899083,0.880733945,0.882568807,0.88440367,0.886238532,0.888073394,
0.889908257,0.891743119,0.893577982,0.895412844,0.897247706,0.899082569,
0.900917431,0.902752294,0.904587156,0.906422018,0.908256881,0.910091743,
0.911926606,0.913761468,0.91559633,0.917431193,0.919266055,0.921100917,
0.92293578,0.924770642,0.926605505,0.928440367,0.930275229,0.932110092,
0.933944954,0.935779817,0.937614679,0.939449541,0.941284404,0.943119266,
0.944954128,0.946788991,0.948623853,0.950458716,0.952293578,0.95412844,
0.955963303,0.957798165,0.959633028,0.96146789,0.963302752,0.965137615,
0.966972477,0.968807339,0.970642202,0.972477064,0.974311927,0.976146789,
0.977981651,0.979816514,0.981651376,0.983486239,0.985321101,0.987155963,
0.988990826,0.990825688,0.99266055,0.994495413,0.996330275,0.998165138,
1.),.UNSPECIFIED.);
#24459=B_SPLINE_CURVE_WITH_KNOTS('',3,(#270594,#270595,#270596,#270597,
#270598,#270599,#270600,#270601,#270602,#270603,#270604,#270605,#270606,
#270607,#270608,#270609,#270610,#270611,#270612,#270613,#270614,#270615,
#270616,#270617,#270618,#270619,#270620,#270621,#270622,#270623,#270624,
#270625,#270626,#270627,#270628,#270629,#270630,#270631,#270632,#270633,
#270634,#270635,#270636,#270637,#270638,#270639,#270640,#270641,#270642,
#270643,#270644,#270645,#270646,#270647,#270648,#270649,#270650,#270651,
#270652,#270653,#270654,#270655,#270656,#270657,#270658,#270659,#270660,
#270661,#270662,#270663,#270664,#270665,#270666,#270667,#270668,#270669,
#270670,#270671,#270672,#270673,#270674,#270675,#270676,#270677,#270678,
#270679,#270680,#270681,#270682,#270683,#270684,#270685,#270686,#270687,
#270688,#270689,#270690,#270691,#270692,#270693,#270694,#270695,#270696,
#270697,#270698,#270699,#270700,#270701,#270702,#270703,#270704,#270705,
#270706,#270707,#270708,#270709,#270710,#270711,#270712,#270713,#270714,
#270715,#270716,#270717,#270718,#270719,#270720,#270721,#270722,#270723,
#270724,#270725,#270726,#270727,#270728,#270729,#270730,#270731,#270732,
#270733,#270734,#270735,#270736,#270737,#270738,#270739,#270740,#270741,
#270742,#270743,#270744,#270745,#270746,#270747,#270748,#270749,#270750,
#270751,#270752,#270753,#270754,#270755,#270756,#270757,#270758,#270759,
#270760,#270761,#270762,#270763,#270764,#270765,#270766,#270767,#270768,
#270769,#270770,#270771,#270772,#270773,#270774,#270775,#270776,#270777,
#270778,#270779,#270780,#270781,#270782,#270783,#270784,#270785,#270786,
#270787,#270788,#270789,#270790,#270791,#270792,#270793,#270794,#270795,
#270796,#270797,#270798,#270799,#270800,#270801,#270802,#270803,#270804,
#270805,#270806,#270807,#270808,#270809,#270810,#270811,#270812,#270813,
#270814,#270815,#270816,#270817,#270818,#270819,#270820,#270821,#270822,
#270823,#270824,#270825,#270826,#270827,#270828,#270829,#270830,#270831,
#270832,#270833,#270834,#270835,#270836,#270837,#270838,#270839,#270840,
#270841,#270842,#270843,#270844,#270845,#270846,#270847,#270848,#270849,
#270850,#270851,#270852,#270853,#270854,#270855,#270856,#270857,#270858,
#270859,#270860,#270861,#270862,#270863,#270864,#270865,#270866,#270867,
#270868,#270869,#270870,#270871,#270872,#270873,#270874,#270875,#270876,
#270877,#270878,#270879,#270880,#270881,#270882,#270883,#270884,#270885,
#270886,#270887,#270888,#270889,#270890,#270891,#270892,#270893,#270894,
#270895,#270896,#270897,#270898,#270899,#270900,#270901,#270902,#270903,
#270904,#270905,#270906,#270907,#270908,#270909,#270910,#270911,#270912,
#270913,#270914,#270915),.UNSPECIFIED.,.F.,.F.,(4,3,3,3,3,3,3,3,3,3,3,3,
3,3,3,3,3,3,3,3,3,3,3,3,3,3,3,3,3,3,3,3,3,3,3,3,3,3,3,3,3,3,3,3,3,3,3,3,
3,3,3,3,3,3,3,3,3,3,3,3,3,3,3,3,3,3,3,3,3,3,3,3,3,3,3,3,3,3,3,3,3,3,3,3,
3,3,3,3,3,3,3,3,3,3,3,3,3,3,3,3,3,3,3,3,3,3,3,4),(-1.,-0.994495413,-0.988990826,
-0.983486239,-0.977981651,-0.972477064,-0.966972477,-0.957798165,-0.952293578,
-0.946788991,-0.941284404,-0.935779817,-0.930275229,-0.92293578,-0.917431193,
-0.910091743,-0.904587156,-0.899082569,-0.893577982,-0.888073394,-0.882568807,
-0.87706422,-0.871559633,-0.866055046,-0.860550459,-0.855045872,-0.849541284,
-0.844036697,-0.83853211,-0.833027523,-0.827522936,-0.822018349,-0.816513761,
-0.811009174,-0.803669725,-0.796330275,-0.788990826,-0.779816514,-0.772477064,
-0.765137615,-0.757798165,-0.746788991,-0.739449541,-0.732110092,-0.724770642,
-0.717431193,-0.710091743,-0.702752294,-0.695412844,-0.688073394,-0.678899083,
-0.671559633,-0.664220183,-0.656880734,-0.649541284,-0.642201835,-0.633027523,
-0.625688073,-0.618348624,-0.611009174,-0.603669725,-0.596330275,-0.588990826,
-0.579816514,-0.572477064,-0.565137615,-0.557798165,-0.550458716,-0.543119266,
-0.535779817,-0.528440367,-0.519266055,-0.510091743,-0.500917431,-0.491743119,
-0.482568807,-0.473394495,-0.464220183,-0.455045872,-0.44587156,-0.436697248,
-0.427522936,-0.418348624,-0.409174312,-0.4,-0.390825688,-0.379816514,-0.368807339,
-0.357798165,-0.346788991,-0.335779817,-0.324770642,-0.313761468,-0.302752294,
-0.291743119,-0.278899083,-0.267889908,-0.256880734,-0.24587156,-0.234862385,
-0.223853211,-0.212844037,-0.201834862,-0.190825688,-0.179816514,-0.168807339,
-0.157798165,-0.143172102),.UNSPECIFIED.);
#24460=B_SPLINE_CURVE_WITH_KNOTS('',3,(#270916,#270917,#270918,#270919,
#270920,#270921,#270922,#270923,#270924,#270925,#270926,#270927,#270928,
#270929,#270930,#270931,#270932,#270933,#270934,#270935,#270936,#270937,
#270938,#270939,#270940,#270941,#270942,#270943,#270944,#270945,#270946,
#270947,#270948,#270949,#270950,#270951,#270952,#270953,#270954,#270955,
#270956,#270957,#270958,#270959,#270960,#270961,#270962,#270963,#270964,
#270965,#270966,#270967,#270968,#270969,#270970,#270971,#270972,#270973,
#270974,#270975,#270976,#270977,#270978,#270979,#270980,#270981,#270982,
#270983,#270984,#270985,#270986,#270987,#270988,#270989,#270990,#270991,
#270992,#270993,#270994,#270995,#270996,#270997,#270998,#270999,#271000,
#271001,#271002,#271003,#271004,#271005,#271006,#271007,#271008,#271009,
#271010,#271011,#271012,#271013,#271014,#271015,#271016,#271017,#271018,
#271019,#271020,#271021,#271022,#271023,#271024,#271025,#271026,#271027,
#271028,#271029,#271030,#271031,#271032,#271033,#271034,#271035,#271036,
#271037,#271038,#271039,#271040,#271041,#271042,#271043,#271044,#271045,
#271046,#271047,#271048,#271049,#271050,#271051,#271052,#271053,#271054,
#271055,#271056,#271057,#271058,#271059,#271060,#271061,#271062,#271063,
#271064,#271065,#271066,#271067,#271068,#271069,#271070,#271071,#271072,
#271073,#271074,#271075,#271076,#271077,#271078,#271079,#271080,#271081,
#271082,#271083,#271084,#271085,#271086,#271087,#271088,#271089,#271090,
#271091,#271092,#271093,#271094,#271095,#271096,#271097,#271098,#271099,
#271100,#271101,#271102,#271103,#271104,#271105,#271106,#271107,#271108,
#271109,#271110,#271111,#271112,#271113,#271114,#271115,#271116,#271117,
#271118,#271119,#271120,#271121,#271122,#271123,#271124,#271125,#271126,
#271127,#271128,#271129,#271130,#271131,#271132,#271133,#271134,#271135,
#271136,#271137,#271138,#271139,#271140,#271141,#271142,#271143,#271144,
#271145,#271146,#271147,#271148,#271149,#271150,#271151,#271152,#271153,
#271154,#271155,#271156,#271157,#271158,#271159,#271160,#271161,#271162,
#271163,#271164,#271165,#271166,#271167,#271168,#271169,#271170,#271171,
#271172,#271173,#271174,#271175,#271176,#271177,#271178,#271179,#271180,
#271181,#271182,#271183,#271184,#271185,#271186,#271187,#271188,#271189,
#271190,#271191,#271192,#271193,#271194,#271195,#271196,#271197,#271198,
#271199,#271200,#271201,#271202,#271203,#271204,#271205,#271206,#271207,
#271208,#271209,#271210,#271211,#271212,#271213,#271214,#271215,#271216,
#271217,#271218,#271219,#271220,#271221,#271222,#271223,#271224,#271225,
#271226,#271227,#271228,#271229,#271230,#271231,#271232,#271233,#271234),
 .UNSPECIFIED.,.F.,.F.,(4,3,3,3,3,3,3,3,3,3,3,3,3,3,3,3,3,3,3,3,3,3,3,3,
3,3,3,3,3,3,3,3,3,3,3,3,3,3,3,3,3,3,3,3,3,3,3,3,3,3,3,3,3,3,3,3,3,3,3,3,
3,3,3,3,3,3,3,3,3,3,3,3,3,3,3,3,3,3,3,3,3,3,3,3,3,3,3,3,3,3,3,3,3,3,3,3,
3,3,3,3,3,3,3,3,3,3,4),(0.143172102,0.15412844,0.165137615,0.176146789,
0.187155963,0.198165138,0.209174312,0.220183486,0.231192661,0.242201835,
0.255045872,0.266055046,0.27706422,0.288073394,0.299082569,0.310091743,
0.321100917,0.332110092,0.343119266,0.35412844,0.366972477,0.377981651,
0.388990826,0.398165138,0.40733945,0.416513761,0.425688073,0.434862385,
0.44587156,0.455045872,0.464220183,0.473394495,0.482568807,0.491743119,
0.502752294,0.511926606,0.521100917,0.530275229,0.537614679,0.544954128,
0.552293578,0.559633028,0.566972477,0.574311927,0.581651376,0.588990826,
0.596330275,0.603669725,0.611009174,0.618348624,0.625688073,0.633027523,
0.640366972,0.647706422,0.655045872,0.662385321,0.669724771,0.67706422,
0.68440367,0.691743119,0.700917431,0.708256881,0.71559633,0.724770642,0.732110092,
0.739449541,0.748623853,0.755963303,0.763302752,0.772477064,0.779816514,
0.787155963,0.796330275,0.805504587,0.812844037,0.818348624,0.823853211,
0.829357798,0.834862385,0.840366972,0.84587156,0.853211009,0.858715596,
0.864220183,0.869724771,0.87706422,0.882568807,0.888073394,0.893577982,
0.899082569,0.906422018,0.911926606,0.919266055,0.924770642,0.930275229,
0.935779817,0.941284404,0.946788991,0.952293578,0.957798165,0.963302752,
0.968807339,0.974311927,0.979816514,0.985321101,0.990825688,1.),
 .UNSPECIFIED.);
#24461=B_SPLINE_CURVE_WITH_KNOTS('',3,(#272179,#272180,#272181,#272182,
#272183,#272184,#272185,#272186,#272187,#272188,#272189,#272190,#272191,
#272192,#272193,#272194,#272195,#272196,#272197,#272198,#272199,#272200,
#272201,#272202,#272203,#272204,#272205,#272206,#272207,#272208,#272209,
#272210,#272211,#272212,#272213,#272214,#272215,#272216,#272217,#272218,
#272219,#272220,#272221,#272222,#272223,#272224,#272225,#272226,#272227,
#272228,#272229,#272230,#272231,#272232,#272233,#272234,#272235,#272236,
#272237,#272238,#272239,#272240,#272241,#272242,#272243,#272244,#272245,
#272246,#272247,#272248,#272249,#272250,#272251,#272252,#272253,#272254,
#272255,#272256,#272257,#272258,#272259,#272260,#272261,#272262,#272263,
#272264,#272265,#272266,#272267,#272268,#272269,#272270,#272271,#272272,
#272273,#272274,#272275,#272276,#272277,#272278,#272279,#272280,#272281,
#272282,#272283,#272284,#272285,#272286,#272287,#272288,#272289,#272290,
#272291,#272292,#272293,#272294,#272295,#272296,#272297,#272298,#272299,
#272300,#272301,#272302,#272303,#272304,#272305,#272306,#272307,#272308,
#272309,#272310,#272311,#272312,#272313,#272314,#272315,#272316,#272317,
#272318,#272319,#272320,#272321,#272322,#272323,#272324,#272325,#272326,
#272327,#272328,#272329,#272330,#272331,#272332,#272333,#272334,#272335,
#272336,#272337,#272338,#272339,#272340,#272341,#272342,#272343,#272344,
#272345,#272346,#272347,#272348,#272349,#272350,#272351,#272352,#272353,
#272354,#272355,#272356,#272357,#272358,#272359,#272360,#272361,#272362,
#272363,#272364,#272365,#272366,#272367,#272368,#272369,#272370,#272371,
#272372,#272373,#272374,#272375,#272376,#272377,#272378,#272379,#272380,
#272381,#272382,#272383,#272384,#272385,#272386,#272387,#272388,#272389,
#272390,#272391,#272392,#272393,#272394,#272395,#272396,#272397,#272398,
#272399,#272400,#272401,#272402,#272403,#272404,#272405,#272406,#272407,
#272408,#272409,#272410,#272411,#272412,#272413,#272414,#272415,#272416,
#272417,#272418,#272419,#272420,#272421,#272422,#272423,#272424,#272425,
#272426,#272427,#272428,#272429,#272430,#272431,#272432,#272433,#272434,
#272435,#272436,#272437,#272438,#272439,#272440,#272441,#272442,#272443,
#272444,#272445,#272446,#272447,#272448,#272449,#272450,#272451,#272452,
#272453,#272454,#272455,#272456,#272457,#272458,#272459,#272460,#272461,
#272462,#272463,#272464,#272465,#272466,#272467,#272468,#272469,#272470,
#272471,#272472,#272473,#272474,#272475,#272476,#272477,#272478,#272479,
#272480,#272481,#272482,#272483,#272484,#272485,#272486,#272487,#272488,
#272489,#272490,#272491,#272492,#272493,#272494,#272495,#272496,#272497,
#272498,#272499,#272500,#272501,#272502,#272503),.UNSPECIFIED.,.F.,.F.,
(4,3,3,3,3,3,3,3,3,3,3,3,3,3,3,3,3,3,3,3,3,3,3,3,3,3,3,3,3,3,3,3,3,3,3,
3,3,3,3,3,3,3,3,3,3,3,3,3,3,3,3,3,3,3,3,3,3,3,3,3,3,3,3,3,3,3,3,3,3,3,3,
3,3,3,3,3,3,3,3,3,3,3,3,3,3,3,3,3,3,3,3,3,3,3,3,3,3,3,3,3,3,3,3,3,3,3,3,
3,4),(0.143172102,0.15412844,0.165137615,0.176146789,0.187155963,0.198165138,
0.209174312,0.220183486,0.231192661,0.242201835,0.253211009,0.264220183,
0.275229358,0.286238532,0.297247706,0.308256881,0.319266055,0.330275229,
0.341284404,0.352293578,0.363302752,0.374311927,0.385321101,0.396330275,
0.405504587,0.414678899,0.423853211,0.433027523,0.442201835,0.451376147,
0.460550459,0.469724771,0.478899083,0.488073394,0.497247706,0.506422018,
0.51559633,0.524770642,0.535779817,0.543119266,0.550458716,0.557798165,
0.565137615,0.572477064,0.579816514,0.587155963,0.594495413,0.601834862,
0.611009174,0.618348624,0.625688073,0.633027523,0.640366972,0.647706422,
0.655045872,0.662385321,0.669724771,0.67706422,0.68440367,0.691743119,0.699082569,
0.706422018,0.713761468,0.721100917,0.728440367,0.735779817,0.743119266,
0.750458716,0.757798165,0.765137615,0.772477064,0.779816514,0.787155963,
0.794495413,0.801834862,0.809174312,0.816513761,0.822018349,0.827522936,
0.833027523,0.83853211,0.84587156,0.851376147,0.856880734,0.862385321,0.867889908,
0.873394495,0.878899083,0.88440367,0.889908257,0.895412844,0.900917431,
0.906422018,0.911926606,0.917431193,0.92293578,0.928440367,0.933944954,
0.941284404,0.946788991,0.952293578,0.959633028,0.966972477,0.972477064,
0.977981651,0.983486239,0.988990826,0.994495413,1.),.UNSPECIFIED.);
#24462=B_SPLINE_CURVE_WITH_KNOTS('',3,(#272504,#272505,#272506,#272507,
#272508,#272509,#272510,#272511,#272512,#272513,#272514,#272515,#272516,
#272517,#272518,#272519,#272520,#272521,#272522,#272523,#272524,#272525,
#272526,#272527,#272528,#272529,#272530,#272531,#272532,#272533,#272534,
#272535,#272536,#272537,#272538,#272539,#272540,#272541,#272542,#272543,
#272544,#272545,#272546,#272547,#272548,#272549,#272550,#272551,#272552,
#272553,#272554,#272555,#272556,#272557,#272558,#272559,#272560,#272561,
#272562,#272563,#272564,#272565,#272566,#272567,#272568,#272569,#272570,
#272571,#272572,#272573,#272574,#272575,#272576,#272577,#272578,#272579,
#272580,#272581,#272582,#272583,#272584,#272585,#272586,#272587,#272588,
#272589,#272590,#272591,#272592,#272593,#272594,#272595,#272596,#272597,
#272598,#272599,#272600,#272601,#272602,#272603,#272604,#272605,#272606,
#272607,#272608,#272609,#272610,#272611,#272612,#272613,#272614,#272615,
#272616,#272617,#272618,#272619,#272620,#272621,#272622,#272623,#272624,
#272625,#272626,#272627,#272628,#272629,#272630,#272631,#272632,#272633,
#272634,#272635,#272636,#272637,#272638,#272639,#272640,#272641,#272642,
#272643,#272644,#272645,#272646,#272647,#272648,#272649,#272650,#272651,
#272652,#272653,#272654,#272655,#272656,#272657,#272658,#272659,#272660,
#272661,#272662,#272663,#272664,#272665,#272666,#272667,#272668,#272669,
#272670,#272671,#272672,#272673,#272674,#272675,#272676,#272677,#272678,
#272679,#272680,#272681,#272682,#272683,#272684,#272685,#272686,#272687,
#272688,#272689,#272690,#272691,#272692,#272693,#272694,#272695,#272696,
#272697,#272698,#272699,#272700,#272701,#272702,#272703,#272704,#272705,
#272706,#272707,#272708,#272709,#272710,#272711,#272712,#272713,#272714,
#272715,#272716,#272717,#272718,#272719,#272720,#272721,#272722,#272723,
#272724,#272725,#272726,#272727,#272728,#272729,#272730,#272731,#272732,
#272733,#272734,#272735,#272736,#272737,#272738,#272739,#272740,#272741,
#272742,#272743,#272744,#272745,#272746,#272747,#272748,#272749,#272750,
#272751,#272752,#272753,#272754,#272755,#272756,#272757,#272758,#272759,
#272760,#272761,#272762,#272763,#272764,#272765,#272766,#272767,#272768,
#272769,#272770,#272771,#272772,#272773,#272774,#272775,#272776,#272777,
#272778,#272779,#272780,#272781,#272782,#272783,#272784,#272785,#272786,
#272787,#272788,#272789,#272790,#272791,#272792,#272793,#272794,#272795,
#272796,#272797,#272798,#272799,#272800,#272801,#272802,#272803,#272804,
#272805,#272806,#272807,#272808,#272809,#272810,#272811,#272812,#272813,
#272814,#272815,#272816,#272817,#272818,#272819,#272820,#272821,#272822,
#272823,#272824,#272825,#272826,#272827,#272828),.UNSPECIFIED.,.F.,.F.,
(4,3,3,3,3,3,3,3,3,3,3,3,3,3,3,3,3,3,3,3,3,3,3,3,3,3,3,3,3,3,3,3,3,3,3,
3,3,3,3,3,3,3,3,3,3,3,3,3,3,3,3,3,3,3,3,3,3,3,3,3,3,3,3,3,3,3,3,3,3,3,3,
3,3,3,3,3,3,3,3,3,3,3,3,3,3,3,3,3,3,3,3,3,3,3,3,3,3,3,3,3,3,3,3,3,3,3,3,
3,4),(0.143172102,0.15412844,0.165137615,0.176146789,0.187155963,0.198165138,
0.209174312,0.220183486,0.231192661,0.242201835,0.253211009,0.264220183,
0.275229358,0.286238532,0.297247706,0.308256881,0.319266055,0.330275229,
0.341284404,0.352293578,0.363302752,0.374311927,0.385321101,0.396330275,
0.405504587,0.414678899,0.423853211,0.433027523,0.442201835,0.451376147,
0.460550459,0.469724771,0.478899083,0.488073394,0.499082569,0.508256881,
0.517431193,0.526605505,0.533944954,0.543119266,0.550458716,0.557798165,
0.565137615,0.572477064,0.579816514,0.587155963,0.594495413,0.601834862,
0.609174312,0.616513761,0.623853211,0.631192661,0.63853211,0.64587156,0.653211009,
0.660550459,0.667889908,0.675229358,0.682568807,0.689908257,0.697247706,
0.704587156,0.711926606,0.719266055,0.726605505,0.733944954,0.743119266,
0.750458716,0.757798165,0.765137615,0.772477064,0.779816514,0.787155963,
0.794495413,0.801834862,0.809174312,0.816513761,0.822018349,0.827522936,
0.833027523,0.83853211,0.844036697,0.849541284,0.855045872,0.860550459,
0.866055046,0.871559633,0.87706422,0.882568807,0.888073394,0.893577982,
0.900917431,0.906422018,0.911926606,0.921100917,0.926605505,0.932110092,
0.937614679,0.943119266,0.948623853,0.95412844,0.959633028,0.966972477,
0.972477064,0.977981651,0.983486239,0.988990826,0.994495413,1.),
 .UNSPECIFIED.);
#24463=B_SPLINE_CURVE_WITH_KNOTS('',3,(#273788,#273789,#273790,#273791,
#273792,#273793,#273794,#273795,#273796,#273797,#273798,#273799,#273800,
#273801,#273802,#273803,#273804,#273805,#273806,#273807,#273808,#273809,
#273810,#273811,#273812,#273813,#273814,#273815,#273816,#273817,#273818,
#273819,#273820,#273821,#273822,#273823,#273824,#273825,#273826,#273827,
#273828,#273829,#273830,#273831,#273832,#273833,#273834,#273835,#273836,
#273837,#273838,#273839,#273840,#273841,#273842,#273843,#273844,#273845,
#273846,#273847,#273848,#273849,#273850,#273851,#273852,#273853,#273854,
#273855,#273856,#273857,#273858,#273859,#273860,#273861,#273862,#273863,
#273864,#273865,#273866,#273867,#273868,#273869,#273870,#273871,#273872,
#273873,#273874,#273875,#273876,#273877,#273878,#273879,#273880,#273881,
#273882,#273883,#273884,#273885,#273886,#273887,#273888,#273889,#273890,
#273891,#273892,#273893,#273894,#273895,#273896,#273897,#273898,#273899,
#273900,#273901,#273902,#273903,#273904,#273905,#273906,#273907,#273908,
#273909,#273910,#273911,#273912,#273913,#273914,#273915,#273916,#273917,
#273918,#273919,#273920,#273921,#273922,#273923,#273924,#273925,#273926,
#273927,#273928,#273929,#273930,#273931,#273932,#273933,#273934,#273935,
#273936,#273937,#273938,#273939,#273940,#273941,#273942,#273943,#273944,
#273945,#273946,#273947,#273948,#273949,#273950,#273951,#273952,#273953,
#273954,#273955,#273956,#273957,#273958,#273959,#273960,#273961,#273962,
#273963,#273964,#273965,#273966,#273967,#273968,#273969,#273970,#273971,
#273972,#273973,#273974,#273975,#273976,#273977,#273978,#273979,#273980,
#273981,#273982,#273983,#273984,#273985,#273986,#273987,#273988,#273989,
#273990,#273991,#273992,#273993,#273994,#273995,#273996,#273997,#273998,
#273999,#274000,#274001,#274002,#274003,#274004,#274005,#274006,#274007,
#274008,#274009,#274010,#274011,#274012,#274013,#274014,#274015,#274016,
#274017,#274018,#274019,#274020,#274021,#274022,#274023,#274024,#274025,
#274026,#274027,#274028,#274029,#274030,#274031,#274032,#274033,#274034,
#274035,#274036,#274037,#274038,#274039,#274040,#274041,#274042,#274043,
#274044,#274045,#274046,#274047,#274048,#274049,#274050,#274051,#274052,
#274053,#274054,#274055,#274056,#274057,#274058,#274059,#274060,#274061,
#274062,#274063,#274064,#274065,#274066,#274067,#274068,#274069,#274070,
#274071,#274072,#274073,#274074,#274075,#274076,#274077,#274078,#274079,
#274080,#274081,#274082,#274083,#274084,#274085,#274086,#274087,#274088,
#274089,#274090,#274091,#274092,#274093,#274094,#274095,#274096,#274097,
#274098,#274099,#274100,#274101,#274102,#274103,#274104,#274105,#274106,
#274107,#274108,#274109,#274110,#274111,#274112),.UNSPECIFIED.,.F.,.F.,
(4,3,3,3,3,3,3,3,3,3,3,3,3,3,3,3,3,3,3,3,3,3,3,3,3,3,3,3,3,3,3,3,3,3,3,
3,3,3,3,3,3,3,3,3,3,3,3,3,3,3,3,3,3,3,3,3,3,3,3,3,3,3,3,3,3,3,3,3,3,3,3,
3,3,3,3,3,3,3,3,3,3,3,3,3,3,3,3,3,3,3,3,3,3,3,3,3,3,3,3,3,3,3,3,3,3,3,3,
3,4),(0.143172102,0.15412844,0.165137615,0.176146789,0.187155963,0.198165138,
0.209174312,0.220183486,0.231192661,0.242201835,0.253211009,0.264220183,
0.275229358,0.286238532,0.297247706,0.308256881,0.319266055,0.330275229,
0.341284404,0.352293578,0.363302752,0.374311927,0.385321101,0.396330275,
0.405504587,0.414678899,0.423853211,0.433027523,0.442201835,0.451376147,
0.460550459,0.469724771,0.478899083,0.488073394,0.497247706,0.506422018,
0.517431193,0.526605505,0.533944954,0.541284404,0.548623853,0.555963303,
0.563302752,0.570642202,0.577981651,0.585321101,0.59266055,0.6,0.60733945,
0.614678899,0.622018349,0.629357798,0.636697248,0.64587156,0.655045872,
0.662385321,0.669724771,0.67706422,0.68440367,0.691743119,0.699082569,0.706422018,
0.713761468,0.721100917,0.728440367,0.735779817,0.743119266,0.750458716,
0.757798165,0.765137615,0.774311927,0.781651376,0.788990826,0.796330275,
0.803669725,0.811009174,0.816513761,0.822018349,0.827522936,0.833027523,
0.83853211,0.844036697,0.849541284,0.855045872,0.860550459,0.869724771,
0.875229358,0.880733945,0.886238532,0.891743119,0.897247706,0.902752294,
0.908256881,0.913761468,0.919266055,0.926605505,0.932110092,0.937614679,
0.943119266,0.948623853,0.95412844,0.959633028,0.966972477,0.972477064,
0.977981651,0.983486239,0.988990826,0.994495413,1.),.UNSPECIFIED.);
#24464=B_SPLINE_CURVE_WITH_KNOTS('',3,(#274113,#274114,#274115,#274116,
#274117,#274118,#274119,#274120,#274121,#274122,#274123,#274124,#274125,
#274126,#274127,#274128,#274129,#274130,#274131,#274132,#274133,#274134,
#274135,#274136,#274137,#274138,#274139,#274140,#274141,#274142,#274143,
#274144,#274145,#274146,#274147,#274148,#274149,#274150,#274151,#274152,
#274153,#274154,#274155,#274156,#274157,#274158,#274159,#274160,#274161,
#274162,#274163,#274164,#274165,#274166,#274167,#274168,#274169,#274170,
#274171,#274172,#274173,#274174,#274175,#274176,#274177,#274178,#274179,
#274180,#274181,#274182,#274183,#274184,#274185,#274186,#274187,#274188,
#274189,#274190,#274191,#274192,#274193,#274194,#274195,#274196,#274197,
#274198,#274199,#274200,#274201,#274202,#274203,#274204,#274205,#274206,
#274207,#274208,#274209,#274210,#274211,#274212,#274213,#274214,#274215,
#274216,#274217,#274218,#274219,#274220,#274221,#274222,#274223,#274224,
#274225,#274226,#274227,#274228,#274229,#274230,#274231,#274232,#274233,
#274234,#274235,#274236,#274237,#274238,#274239,#274240,#274241,#274242,
#274243,#274244,#274245,#274246,#274247,#274248,#274249,#274250,#274251,
#274252,#274253,#274254,#274255,#274256,#274257,#274258,#274259,#274260,
#274261,#274262,#274263,#274264,#274265,#274266,#274267,#274268,#274269,
#274270,#274271,#274272,#274273,#274274,#274275,#274276,#274277,#274278,
#274279,#274280,#274281,#274282,#274283,#274284,#274285,#274286,#274287,
#274288,#274289,#274290,#274291,#274292,#274293,#274294,#274295,#274296,
#274297,#274298,#274299,#274300,#274301,#274302,#274303,#274304,#274305,
#274306,#274307,#274308,#274309,#274310,#274311,#274312,#274313,#274314,
#274315,#274316,#274317,#274318,#274319,#274320,#274321,#274322,#274323,
#274324,#274325,#274326,#274327,#274328,#274329,#274330,#274331,#274332,
#274333,#274334,#274335,#274336,#274337,#274338,#274339,#274340,#274341,
#274342,#274343,#274344,#274345,#274346,#274347,#274348,#274349,#274350,
#274351,#274352,#274353,#274354,#274355,#274356,#274357,#274358,#274359,
#274360,#274361,#274362,#274363,#274364,#274365,#274366,#274367,#274368,
#274369,#274370,#274371,#274372,#274373,#274374,#274375,#274376,#274377,
#274378,#274379,#274380,#274381,#274382,#274383,#274384,#274385,#274386,
#274387,#274388,#274389,#274390,#274391,#274392,#274393,#274394,#274395,
#274396,#274397,#274398,#274399,#274400,#274401,#274402,#274403,#274404,
#274405,#274406,#274407,#274408,#274409,#274410,#274411,#274412,#274413,
#274414,#274415,#274416,#274417,#274418,#274419,#274420,#274421,#274422,
#274423,#274424,#274425,#274426,#274427,#274428,#274429,#274430,#274431,
#274432,#274433,#274434,#274435,#274436,#274437),.UNSPECIFIED.,.F.,.F.,
(4,3,3,3,3,3,3,3,3,3,3,3,3,3,3,3,3,3,3,3,3,3,3,3,3,3,3,3,3,3,3,3,3,3,3,
3,3,3,3,3,3,3,3,3,3,3,3,3,3,3,3,3,3,3,3,3,3,3,3,3,3,3,3,3,3,3,3,3,3,3,3,
3,3,3,3,3,3,3,3,3,3,3,3,3,3,3,3,3,3,3,3,3,3,3,3,3,3,3,3,3,3,3,3,3,3,3,3,
3,4),(0.143172102,0.15412844,0.165137615,0.176146789,0.187155963,0.198165138,
0.209174312,0.220183486,0.231192661,0.242201835,0.253211009,0.264220183,
0.275229358,0.286238532,0.297247706,0.308256881,0.319266055,0.330275229,
0.341284404,0.352293578,0.363302752,0.374311927,0.385321101,0.396330275,
0.405504587,0.414678899,0.423853211,0.433027523,0.442201835,0.451376147,
0.460550459,0.469724771,0.478899083,0.488073394,0.497247706,0.506422018,
0.51559633,0.524770642,0.533944954,0.541284404,0.548623853,0.555963303,
0.563302752,0.570642202,0.577981651,0.585321101,0.59266055,0.6,0.60733945,
0.614678899,0.622018349,0.629357798,0.636697248,0.644036697,0.651376147,
0.658715596,0.666055046,0.673394495,0.680733945,0.688073394,0.695412844,
0.706422018,0.713761468,0.721100917,0.728440367,0.735779817,0.743119266,
0.750458716,0.757798165,0.766972477,0.774311927,0.781651376,0.788990826,
0.796330275,0.803669725,0.811009174,0.816513761,0.822018349,0.827522936,
0.833027523,0.83853211,0.844036697,0.849541284,0.855045872,0.860550459,
0.869724771,0.875229358,0.880733945,0.886238532,0.891743119,0.897247706,
0.902752294,0.908256881,0.913761468,0.921100917,0.926605505,0.932110092,
0.937614679,0.943119266,0.948623853,0.95412844,0.959633028,0.966972477,
0.972477064,0.977981651,0.983486239,0.988990826,0.994495413,1.),
 .UNSPECIFIED.);
#24465=B_SPLINE_CURVE_WITH_KNOTS('',3,(#275385,#275386,#275387,#275388,
#275389,#275390,#275391,#275392,#275393,#275394,#275395,#275396,#275397,
#275398,#275399,#275400,#275401,#275402,#275403,#275404,#275405,#275406,
#275407,#275408,#275409,#275410,#275411,#275412,#275413,#275414,#275415,
#275416,#275417,#275418,#275419,#275420,#275421,#275422,#275423,#275424,
#275425,#275426,#275427,#275428,#275429,#275430,#275431,#275432,#275433,
#275434,#275435,#275436,#275437,#275438,#275439,#275440,#275441,#275442,
#275443,#275444,#275445,#275446,#275447,#275448,#275449,#275450,#275451,
#275452,#275453,#275454,#275455,#275456,#275457,#275458,#275459,#275460,
#275461,#275462,#275463,#275464,#275465,#275466,#275467,#275468,#275469,
#275470,#275471,#275472,#275473,#275474,#275475,#275476,#275477,#275478,
#275479,#275480,#275481,#275482,#275483,#275484,#275485,#275486,#275487,
#275488,#275489,#275490,#275491,#275492,#275493,#275494,#275495,#275496,
#275497,#275498,#275499,#275500,#275501,#275502,#275503,#275504,#275505,
#275506,#275507,#275508,#275509,#275510,#275511,#275512,#275513,#275514,
#275515,#275516,#275517,#275518,#275519,#275520,#275521,#275522,#275523,
#275524,#275525,#275526,#275527,#275528,#275529,#275530,#275531,#275532,
#275533,#275534,#275535,#275536,#275537,#275538,#275539,#275540,#275541,
#275542,#275543,#275544,#275545,#275546,#275547,#275548,#275549,#275550,
#275551,#275552,#275553,#275554,#275555,#275556,#275557,#275558,#275559,
#275560,#275561,#275562,#275563,#275564,#275565,#275566,#275567,#275568,
#275569,#275570,#275571,#275572,#275573,#275574,#275575,#275576,#275577,
#275578,#275579,#275580,#275581,#275582,#275583,#275584,#275585,#275586,
#275587,#275588,#275589,#275590,#275591,#275592,#275593,#275594,#275595,
#275596,#275597,#275598,#275599,#275600,#275601,#275602,#275603,#275604,
#275605,#275606,#275607,#275608,#275609,#275610,#275611,#275612,#275613,
#275614,#275615,#275616,#275617,#275618,#275619,#275620,#275621,#275622,
#275623,#275624,#275625,#275626,#275627,#275628,#275629,#275630,#275631,
#275632,#275633,#275634,#275635,#275636,#275637,#275638,#275639,#275640,
#275641,#275642,#275643,#275644,#275645,#275646,#275647,#275648,#275649,
#275650,#275651,#275652,#275653,#275654,#275655,#275656,#275657,#275658,
#275659,#275660,#275661,#275662,#275663,#275664,#275665,#275666,#275667,
#275668,#275669,#275670,#275671,#275672,#275673,#275674,#275675,#275676,
#275677,#275678,#275679,#275680,#275681,#275682,#275683,#275684,#275685,
#275686,#275687,#275688,#275689,#275690,#275691,#275692,#275693,#275694,
#275695,#275696,#275697,#275698,#275699,#275700,#275701,#275702,#275703,
#275704,#275705,#275706,#275707,#275708,#275709),.UNSPECIFIED.,.F.,.F.,
(4,3,3,3,3,3,3,3,3,3,3,3,3,3,3,3,3,3,3,3,3,3,3,3,3,3,3,3,3,3,3,3,3,3,3,
3,3,3,3,3,3,3,3,3,3,3,3,3,3,3,3,3,3,3,3,3,3,3,3,3,3,3,3,3,3,3,3,3,3,3,3,
3,3,3,3,3,3,3,3,3,3,3,3,3,3,3,3,3,3,3,3,3,3,3,3,3,3,3,3,3,3,3,3,3,3,3,3,
3,4),(-1.,-0.99266055,-0.987155963,-0.981651376,-0.976146789,-0.970642202,
-0.965137615,-0.959633028,-0.95412844,-0.948623853,-0.943119266,-0.935779817,
-0.930275229,-0.924770642,-0.919266055,-0.913761468,-0.908256881,-0.900917431,
-0.895412844,-0.889908257,-0.88440367,-0.878899083,-0.873394495,-0.867889908,
-0.862385321,-0.856880734,-0.851376147,-0.84587156,-0.840366972,-0.834862385,
-0.829357798,-0.823853211,-0.818348624,-0.812844037,-0.80733945,-0.8,-0.79266055,
-0.781651376,-0.774311927,-0.766972477,-0.759633028,-0.752293578,-0.744954128,
-0.737614679,-0.730275229,-0.72293578,-0.711926606,-0.704587156,-0.697247706,
-0.689908257,-0.682568807,-0.673394495,-0.666055046,-0.658715596,-0.651376147,
-0.644036697,-0.636697248,-0.629357798,-0.622018349,-0.614678899,-0.60733945,
-0.6,-0.59266055,-0.585321101,-0.577981651,-0.570642202,-0.563302752,-0.555963303,
-0.548623853,-0.541284404,-0.533944954,-0.526605505,-0.517431193,-0.508256881,
-0.499082569,-0.489908257,-0.480733945,-0.471559633,-0.462385321,-0.453211009,
-0.444036697,-0.434862385,-0.425688073,-0.416513761,-0.40733945,-0.398165138,
-0.388990826,-0.377981651,-0.366972477,-0.355963303,-0.344954128,-0.333944954,
-0.32293578,-0.311926606,-0.300917431,-0.289908257,-0.278899083,-0.267889908,
-0.256880734,-0.24587156,-0.234862385,-0.223853211,-0.212844037,-0.201834862,
-0.190825688,-0.179816514,-0.168807339,-0.157798165,-0.143172102),
 .UNSPECIFIED.);
#24466=B_SPLINE_CURVE_WITH_KNOTS('',3,(#275710,#275711,#275712,#275713,
#275714,#275715,#275716,#275717,#275718,#275719,#275720,#275721,#275722,
#275723,#275724,#275725,#275726,#275727,#275728,#275729,#275730,#275731,
#275732,#275733,#275734,#275735,#275736,#275737,#275738,#275739,#275740,
#275741,#275742,#275743,#275744,#275745,#275746,#275747,#275748,#275749,
#275750,#275751,#275752,#275753,#275754,#275755,#275756,#275757,#275758,
#275759,#275760,#275761,#275762,#275763,#275764,#275765,#275766,#275767,
#275768,#275769,#275770,#275771,#275772,#275773,#275774,#275775,#275776,
#275777,#275778,#275779,#275780,#275781,#275782,#275783,#275784,#275785,
#275786,#275787,#275788,#275789,#275790,#275791,#275792,#275793,#275794,
#275795,#275796,#275797,#275798,#275799,#275800,#275801,#275802,#275803,
#275804,#275805,#275806,#275807,#275808,#275809,#275810,#275811,#275812,
#275813,#275814,#275815,#275816,#275817,#275818,#275819,#275820,#275821,
#275822,#275823,#275824,#275825,#275826,#275827,#275828,#275829,#275830,
#275831,#275832,#275833,#275834,#275835,#275836,#275837,#275838,#275839,
#275840,#275841,#275842,#275843,#275844,#275845,#275846,#275847,#275848,
#275849,#275850,#275851,#275852,#275853,#275854,#275855,#275856,#275857,
#275858,#275859,#275860,#275861,#275862,#275863,#275864,#275865,#275866,
#275867,#275868,#275869,#275870,#275871,#275872,#275873,#275874,#275875,
#275876,#275877,#275878,#275879,#275880,#275881,#275882,#275883,#275884,
#275885,#275886,#275887,#275888,#275889,#275890,#275891,#275892,#275893,
#275894,#275895,#275896,#275897,#275898,#275899,#275900,#275901,#275902,
#275903,#275904,#275905,#275906,#275907,#275908,#275909,#275910,#275911,
#275912,#275913,#275914,#275915,#275916,#275917,#275918,#275919,#275920,
#275921,#275922,#275923,#275924,#275925,#275926,#275927,#275928,#275929,
#275930,#275931,#275932,#275933,#275934,#275935,#275936,#275937,#275938,
#275939,#275940,#275941,#275942,#275943,#275944,#275945,#275946,#275947,
#275948,#275949,#275950,#275951,#275952,#275953,#275954,#275955,#275956,
#275957,#275958,#275959,#275960,#275961,#275962,#275963,#275964,#275965,
#275966,#275967,#275968,#275969,#275970,#275971,#275972,#275973,#275974,
#275975,#275976,#275977,#275978,#275979,#275980,#275981,#275982,#275983,
#275984,#275985,#275986,#275987,#275988,#275989,#275990,#275991,#275992,
#275993,#275994,#275995,#275996,#275997,#275998,#275999,#276000,#276001,
#276002,#276003,#276004,#276005,#276006,#276007,#276008,#276009,#276010,
#276011,#276012,#276013,#276014,#276015,#276016,#276017,#276018,#276019,
#276020,#276021,#276022,#276023,#276024,#276025,#276026,#276027,#276028,
#276029,#276030,#276031),.UNSPECIFIED.,.F.,.F.,(4,3,3,3,3,3,3,3,3,3,3,3,
3,3,3,3,3,3,3,3,3,3,3,3,3,3,3,3,3,3,3,3,3,3,3,3,3,3,3,3,3,3,3,3,3,3,3,3,
3,3,3,3,3,3,3,3,3,3,3,3,3,3,3,3,3,3,3,3,3,3,3,3,3,3,3,3,3,3,3,3,3,3,3,3,
3,3,3,3,3,3,3,3,3,3,3,3,3,3,3,3,3,3,3,3,3,3,3,4),(0.143172102,0.15412844,
0.165137615,0.176146789,0.187155963,0.198165138,0.209174312,0.220183486,
0.231192661,0.242201835,0.253211009,0.264220183,0.275229358,0.286238532,
0.297247706,0.308256881,0.319266055,0.330275229,0.341284404,0.352293578,
0.363302752,0.374311927,0.385321101,0.396330275,0.405504587,0.414678899,
0.423853211,0.433027523,0.442201835,0.451376147,0.460550459,0.469724771,
0.478899083,0.488073394,0.497247706,0.506422018,0.51559633,0.524770642,
0.533944954,0.543119266,0.552293578,0.559633028,0.566972477,0.574311927,
0.581651376,0.588990826,0.596330275,0.603669725,0.611009174,0.618348624,
0.625688073,0.633027523,0.640366972,0.647706422,0.655045872,0.662385321,
0.669724771,0.67706422,0.68440367,0.691743119,0.699082569,0.706422018,0.713761468,
0.721100917,0.728440367,0.737614679,0.744954128,0.752293578,0.759633028,
0.766972477,0.774311927,0.781651376,0.788990826,0.796330275,0.805504587,
0.812844037,0.818348624,0.823853211,0.829357798,0.834862385,0.840366972,
0.84587156,0.851376147,0.856880734,0.862385321,0.867889908,0.873394495,
0.878899083,0.886238532,0.891743119,0.897247706,0.902752294,0.910091743,
0.91559633,0.921100917,0.928440367,0.933944954,0.939449541,0.944954128,
0.950458716,0.957798165,0.963302752,0.968807339,0.974311927,0.979816514,
0.985321101,0.990825688,1.),.UNSPECIFIED.);
#24467=B_SPLINE_CURVE_WITH_KNOTS('',5,(#276994,#276995,#276996,#276997,
#276998,#276999,#277000,#277001,#277002,#277003,#277004,#277005,#277006,
#277007,#277008,#277009,#277010,#277011,#277012,#277013,#277014,#277015,
#277016,#277017,#277018,#277019,#277020,#277021,#277022,#277023,#277024,
#277025,#277026,#277027,#277028,#277029,#277030,#277031,#277032,#277033,
#277034,#277035,#277036,#277037,#277038,#277039,#277040,#277041,#277042,
#277043,#277044,#277045,#277046,#277047,#277048,#277049,#277050,#277051,
#277052,#277053,#277054,#277055,#277056,#277057,#277058,#277059,#277060,
#277061,#277062,#277063,#277064,#277065,#277066,#277067,#277068,#277069,
#277070,#277071,#277072,#277073,#277074,#277075,#277076,#277077,#277078,
#277079,#277080,#277081,#277082,#277083,#277084,#277085,#277086,#277087,
#277088,#277089,#277090,#277091,#277092,#277093,#277094,#277095,#277096,
#277097,#277098,#277099,#277100,#277101,#277102,#277103,#277104,#277105,
#277106,#277107,#277108,#277109,#277110,#277111,#277112,#277113,#277114,
#277115,#277116,#277117,#277118,#277119,#277120,#277121,#277122,#277123,
#277124,#277125,#277126,#277127,#277128,#277129,#277130,#277131,#277132,
#277133,#277134,#277135,#277136,#277137,#277138,#277139,#277140,#277141,
#277142,#277143,#277144,#277145,#277146,#277147,#277148,#277149,#277150,
#277151,#277152,#277153,#277154,#277155,#277156,#277157,#277158,#277159,
#277160,#277161,#277162,#277163,#277164,#277165,#277166,#277167,#277168,
#277169,#277170,#277171,#277172,#277173,#277174,#277175,#277176,#277177,
#277178,#277179,#277180,#277181,#277182,#277183,#277184,#277185,#277186,
#277187,#277188,#277189,#277190,#277191,#277192,#277193,#277194,#277195,
#277196,#277197,#277198,#277199,#277200,#277201,#277202,#277203,#277204,
#277205,#277206,#277207,#277208,#277209,#277210,#277211,#277212,#277213,
#277214,#277215,#277216,#277217,#277218,#277219,#277220,#277221,#277222,
#277223,#277224,#277225,#277226,#277227,#277228,#277229,#277230,#277231,
#277232,#277233,#277234,#277235,#277236,#277237,#277238,#277239,#277240,
#277241,#277242,#277243,#277244,#277245,#277246,#277247,#277248,#277249,
#277250,#277251,#277252,#277253,#277254,#277255,#277256,#277257,#277258,
#277259,#277260,#277261,#277262,#277263,#277264,#277265,#277266,#277267,
#277268,#277269,#277270,#277271,#277272,#277273,#277274,#277275,#277276,
#277277,#277278,#277279,#277280,#277281,#277282,#277283,#277284,#277285,
#277286,#277287,#277288,#277289,#277290,#277291,#277292,#277293,#277294,
#277295,#277296,#277297,#277298,#277299,#277300,#277301,#277302,#277303,
#277304,#277305,#277306,#277307,#277308,#277309,#277310,#277311,#277312,
#277313,#277314,#277315,#277316,#277317,#277318,#277319,#277320,#277321,
#277322,#277323,#277324,#277325,#277326,#277327,#277328,#277329,#277330,
#277331,#277332,#277333,#277334,#277335,#277336,#277337,#277338,#277339,
#277340,#277341,#277342,#277343,#277344,#277345,#277346,#277347,#277348,
#277349,#277350,#277351,#277352,#277353,#277354,#277355,#277356,#277357,
#277358,#277359,#277360,#277361,#277362,#277363,#277364,#277365,#277366,
#277367,#277368,#277369,#277370,#277371,#277372,#277373,#277374,#277375,
#277376,#277377,#277378,#277379,#277380,#277381,#277382,#277383,#277384,
#277385,#277386,#277387,#277388,#277389,#277390,#277391,#277392,#277393,
#277394,#277395,#277396,#277397,#277398,#277399,#277400,#277401,#277402,
#277403,#277404,#277405,#277406,#277407,#277408,#277409,#277410,#277411,
#277412,#277413,#277414,#277415,#277416,#277417,#277418,#277419,#277420,
#277421,#277422,#277423,#277424,#277425,#277426,#277427,#277428,#277429,
#277430,#277431,#277432,#277433,#277434,#277435,#277436,#277437,#277438,
#277439,#277440,#277441,#277442,#277443,#277444,#277445,#277446,#277447,
#277448,#277449,#277450,#277451,#277452,#277453,#277454,#277455,#277456,
#277457,#277458,#277459,#277460,#277461,#277462,#277463,#277464),
 .UNSPECIFIED.,.F.,.F.,(6,1,1,1,1,1,1,1,1,1,1,1,1,1,1,1,1,1,1,1,1,1,1,1,
1,1,1,1,1,1,1,1,1,1,1,1,1,1,1,1,1,1,1,1,1,1,1,1,1,1,1,1,1,1,1,1,1,1,1,1,
1,1,1,1,1,1,1,1,1,1,1,1,1,1,1,1,1,1,1,1,1,1,1,1,1,1,1,1,1,1,1,1,1,1,1,1,
1,1,1,1,1,1,1,1,1,1,1,1,1,1,1,1,1,1,1,1,1,1,1,1,1,1,1,1,1,1,1,1,1,1,1,1,
1,1,1,1,1,1,1,1,1,1,1,1,1,1,1,1,1,1,1,1,1,1,1,1,1,1,1,1,1,1,1,1,1,1,1,1,
1,1,1,1,1,1,1,1,1,1,1,1,1,1,1,1,1,1,1,1,1,1,1,1,1,1,1,1,1,1,1,1,1,1,1,1,
1,1,1,1,1,1,1,1,1,1,1,1,1,1,1,1,1,1,1,1,1,1,1,1,1,1,1,1,1,1,1,1,1,1,1,1,
1,1,1,1,1,1,1,1,1,1,1,1,1,1,1,1,1,1,1,1,1,1,1,1,1,1,1,1,1,1,1,1,1,1,1,1,
1,1,1,1,1,1,1,1,1,1,1,1,1,1,1,1,1,1,1,1,1,1,1,1,1,1,1,1,1,1,1,1,1,1,1,1,
1,1,1,1,1,1,1,1,1,1,1,1,1,1,1,1,1,1,1,1,1,1,1,1,1,1,1,1,1,1,1,1,1,1,1,1,
1,1,1,1,1,1,1,1,1,1,1,1,1,1,1,1,1,1,1,1,1,1,1,1,1,1,1,1,1,1,1,1,1,1,1,1,
1,1,1,1,1,1,1,1,1,1,1,1,1,1,1,1,1,1,1,1,1,1,1,1,1,1,1,1,1,1,1,1,1,1,1,1,
1,1,1,1,1,1,1,1,1,1,1,1,1,1,1,1,1,1,1,1,1,1,1,1,1,1,1,1,1,1,1,1,1,1,1,1,
1,1,1,1,1,1,1,1,1,1,6),(-1.,-0.998165138,-0.996330275,-0.994495413,-0.99266055,
-0.990825688,-0.988990826,-0.987155963,-0.985321101,-0.983486239,-0.981651376,
-0.979816514,-0.977981651,-0.976146789,-0.974311927,-0.972477064,-0.970642202,
-0.968807339,-0.966972477,-0.965137615,-0.963302752,-0.96146789,-0.959633028,
-0.957798165,-0.955963303,-0.95412844,-0.952293578,-0.950458716,-0.948623853,
-0.946788991,-0.944954128,-0.943119266,-0.941284404,-0.939449541,-0.937614679,
-0.935779817,-0.933944954,-0.932110092,-0.930275229,-0.928440367,-0.926605505,
-0.924770642,-0.92293578,-0.921100917,-0.919266055,-0.917431193,-0.91559633,
-0.913761468,-0.911926606,-0.910091743,-0.908256881,-0.906422018,-0.904587156,
-0.902752294,-0.900917431,-0.899082569,-0.897247706,-0.895412844,-0.893577982,
-0.889908257,-0.888073394,-0.886238532,-0.88440367,-0.882568807,-0.880733945,
-0.878899083,-0.87706422,-0.875229358,-0.873394495,-0.871559633,-0.869724771,
-0.867889908,-0.866055046,-0.864220183,-0.862385321,-0.860550459,-0.858715596,
-0.856880734,-0.855045872,-0.853211009,-0.851376147,-0.849541284,-0.847706422,
-0.84587156,-0.844036697,-0.842201835,-0.840366972,-0.83853211,-0.836697248,
-0.834862385,-0.833027523,-0.831192661,-0.829357798,-0.827522936,-0.825688073,
-0.823853211,-0.822018349,-0.820183486,-0.818348624,-0.816513761,-0.814678899,
-0.812844037,-0.811009174,-0.809174312,-0.80733945,-0.805504587,-0.803669725,
-0.801834862,-0.8,-0.798165138,-0.796330275,-0.794495413,-0.79266055,-0.790825688,
-0.788990826,-0.787155963,-0.785321101,-0.783486239,-0.781651376,-0.779816514,
-0.777981651,-0.776146789,-0.774311927,-0.772477064,-0.770642202,-0.768807339,
-0.766972477,-0.765137615,-0.763302752,-0.76146789,-0.759633028,-0.757798165,
-0.755963303,-0.75412844,-0.752293578,-0.750458716,-0.748623853,-0.746788991,
-0.744954128,-0.743119266,-0.741284404,-0.739449541,-0.737614679,-0.735779817,
-0.733944954,-0.732110092,-0.730275229,-0.728440367,-0.726605505,-0.724770642,
-0.72293578,-0.721100917,-0.719266055,-0.717431193,-0.71559633,-0.713761468,
-0.711926606,-0.710091743,-0.708256881,-0.706422018,-0.704587156,-0.702752294,
-0.700917431,-0.699082569,-0.697247706,-0.695412844,-0.693577982,-0.691743119,
-0.689908257,-0.688073394,-0.686238532,-0.68440367,-0.682568807,-0.680733945,
-0.678899083,-0.67706422,-0.675229358,-0.673394495,-0.671559633,-0.669724771,
-0.667889908,-0.666055046,-0.664220183,-0.662385321,-0.660550459,-0.658715596,
-0.656880734,-0.655045872,-0.653211009,-0.651376147,-0.649541284,-0.647706422,
-0.64587156,-0.644036697,-0.642201835,-0.640366972,-0.63853211,-0.636697248,
-0.634862385,-0.633027523,-0.631192661,-0.629357798,-0.627522936,-0.625688073,
-0.623853211,-0.622018349,-0.620183486,-0.618348624,-0.616513761,-0.614678899,
-0.612844037,-0.611009174,-0.609174312,-0.60733945,-0.605504587,-0.603669725,
-0.601834862,-0.6,-0.598165138,-0.596330275,-0.594495413,-0.59266055,-0.590825688,
-0.588990826,-0.587155963,-0.585321101,-0.583486239,-0.581651376,-0.579816514,
-0.577981651,-0.576146789,-0.574311927,-0.572477064,-0.570642202,-0.568807339,
-0.566972477,-0.565137615,-0.563302752,-0.56146789,-0.559633028,-0.557798165,
-0.555963303,-0.55412844,-0.552293578,-0.550458716,-0.548623853,-0.546788991,
-0.544954128,-0.543119266,-0.541284404,-0.539449541,-0.537614679,-0.535779817,
-0.533944954,-0.532110092,-0.530275229,-0.528440367,-0.526605505,-0.524770642,
-0.52293578,-0.521100917,-0.519266055,-0.517431193,-0.51559633,-0.513761468,
-0.511926606,-0.510091743,-0.508256881,-0.506422018,-0.504587156,-0.502752294,
-0.500917431,-0.499082569,-0.497247706,-0.495412844,-0.493577982,-0.491743119,
-0.489908257,-0.488073394,-0.486238532,-0.48440367,-0.482568807,-0.480733945,
-0.478899083,-0.47706422,-0.475229358,-0.473394495,-0.471559633,-0.469724771,
-0.467889908,-0.466055046,-0.464220183,-0.462385321,-0.460550459,-0.458715596,
-0.456880734,-0.455045872,-0.453211009,-0.451376147,-0.449541284,-0.447706422,
-0.44587156,-0.444036697,-0.442201835,-0.440366972,-0.43853211,-0.436697248,
-0.434862385,-0.433027523,-0.431192661,-0.429357798,-0.427522936,-0.425688073,
-0.423853211,-0.422018349,-0.420183486,-0.418348624,-0.416513761,-0.414678899,
-0.412844037,-0.411009174,-0.409174312,-0.40733945,-0.405504587,-0.403669725,
-0.401834862,-0.4,-0.398165138,-0.396330275,-0.394495413,-0.39266055,-0.390825688,
-0.388990826,-0.387155963,-0.385321101,-0.383486239,-0.381651376,-0.379816514,
-0.377981651,-0.376146789,-0.374311927,-0.372477064,-0.370642202,-0.368807339,
-0.366972477,-0.365137615,-0.363302752,-0.36146789,-0.359633028,-0.357798165,
-0.355963303,-0.35412844,-0.352293578,-0.350458716,-0.348623853,-0.346788991,
-0.344954128,-0.343119266,-0.341284404,-0.339449541,-0.337614679,-0.335779817,
-0.333944954,-0.332110092,-0.330275229,-0.328440367,-0.326605505,-0.324770642,
-0.32293578,-0.321100917,-0.319266055,-0.317431193,-0.31559633,-0.313761468,
-0.311926606,-0.310091743,-0.308256881,-0.306422018,-0.304587156,-0.302752294,
-0.300917431,-0.299082569,-0.297247706,-0.295412844,-0.293577982,-0.291743119,
-0.289908257,-0.288073394,-0.286238532,-0.28440367,-0.282568807,-0.280733945,
-0.278899083,-0.27706422,-0.275229358,-0.273394495,-0.271559633,-0.269724771,
-0.267889908,-0.266055046,-0.264220183,-0.262385321,-0.260550459,-0.258715596,
-0.256880734,-0.255045872,-0.253211009,-0.251376147,-0.249541284,-0.247706422,
-0.24587156,-0.244036697,-0.242201835,-0.240366972,-0.23853211,-0.236697248,
-0.234862385,-0.233027523,-0.231192661,-0.229357798,-0.227522936,-0.225688073,
-0.223853211,-0.222018349,-0.220183486,-0.218348624,-0.216513761,-0.214678899,
-0.212844037,-0.211009174,-0.209174312,-0.20733945,-0.205504587,-0.203669725,
-0.201834862,-0.2,-0.198165138,-0.196330275,-0.194495413,-0.19266055,-0.190825688,
-0.188990826,-0.187155963,-0.185321101,-0.183486239,-0.181651376,-0.179816514,
-0.177981651,-0.176146789,-0.174311927,-0.172477064,-0.170642202,-0.168807339,
-0.166972477,-0.165137615,-0.163302752,-0.16146789,-0.159633028,-0.157798165,
-0.155963303,-0.15412844,-0.152293578,-0.150458716,-0.148623853,-0.146788991,
-0.144954128,-0.143172102),.UNSPECIFIED.);
#24468=B_SPLINE_CURVE_WITH_KNOTS('',5,(#277465,#277466,#277467,#277468,
#277469,#277470,#277471,#277472,#277473,#277474,#277475,#277476,#277477,
#277478,#277479,#277480,#277481,#277482,#277483,#277484,#277485,#277486,
#277487,#277488,#277489,#277490,#277491,#277492,#277493,#277494,#277495,
#277496,#277497,#277498,#277499,#277500,#277501,#277502,#277503,#277504,
#277505,#277506,#277507,#277508,#277509,#277510,#277511,#277512,#277513,
#277514,#277515,#277516,#277517,#277518,#277519,#277520,#277521,#277522,
#277523,#277524,#277525,#277526,#277527,#277528,#277529,#277530,#277531,
#277532,#277533,#277534,#277535,#277536,#277537,#277538,#277539,#277540,
#277541,#277542,#277543,#277544,#277545,#277546,#277547,#277548,#277549,
#277550,#277551,#277552,#277553,#277554,#277555,#277556,#277557,#277558,
#277559,#277560,#277561,#277562,#277563,#277564,#277565,#277566,#277567,
#277568,#277569,#277570,#277571,#277572,#277573,#277574,#277575,#277576,
#277577,#277578,#277579,#277580,#277581,#277582,#277583,#277584,#277585,
#277586,#277587,#277588,#277589,#277590,#277591,#277592,#277593,#277594,
#277595,#277596,#277597,#277598,#277599,#277600,#277601,#277602,#277603,
#277604,#277605,#277606,#277607,#277608,#277609,#277610,#277611,#277612,
#277613,#277614,#277615,#277616,#277617,#277618,#277619,#277620,#277621,
#277622,#277623,#277624,#277625,#277626,#277627,#277628,#277629,#277630,
#277631,#277632,#277633,#277634,#277635,#277636,#277637,#277638,#277639,
#277640,#277641,#277642,#277643,#277644,#277645,#277646,#277647,#277648,
#277649,#277650,#277651,#277652,#277653,#277654,#277655,#277656,#277657,
#277658,#277659,#277660,#277661,#277662,#277663,#277664,#277665,#277666,
#277667,#277668,#277669,#277670,#277671,#277672,#277673,#277674,#277675,
#277676,#277677,#277678,#277679,#277680,#277681,#277682,#277683,#277684,
#277685,#277686,#277687,#277688,#277689,#277690,#277691,#277692,#277693,
#277694,#277695,#277696,#277697,#277698,#277699,#277700,#277701,#277702,
#277703,#277704,#277705,#277706,#277707,#277708,#277709,#277710,#277711,
#277712,#277713,#277714,#277715,#277716,#277717,#277718,#277719,#277720,
#277721,#277722,#277723,#277724,#277725,#277726,#277727,#277728,#277729,
#277730,#277731,#277732,#277733,#277734,#277735,#277736,#277737,#277738,
#277739,#277740,#277741,#277742,#277743,#277744,#277745,#277746,#277747,
#277748,#277749,#277750,#277751,#277752,#277753,#277754,#277755,#277756,
#277757,#277758,#277759,#277760,#277761,#277762,#277763,#277764,#277765,
#277766,#277767,#277768,#277769,#277770,#277771,#277772,#277773,#277774,
#277775,#277776,#277777,#277778,#277779,#277780,#277781,#277782,#277783,
#277784,#277785,#277786,#277787,#277788,#277789,#277790,#277791,#277792,
#277793,#277794,#277795,#277796,#277797,#277798,#277799,#277800,#277801,
#277802,#277803,#277804,#277805,#277806,#277807,#277808,#277809,#277810,
#277811,#277812,#277813,#277814,#277815,#277816,#277817,#277818,#277819,
#277820,#277821,#277822,#277823,#277824,#277825,#277826,#277827,#277828,
#277829,#277830,#277831,#277832,#277833,#277834,#277835,#277836,#277837,
#277838,#277839,#277840,#277841,#277842,#277843,#277844,#277845,#277846,
#277847,#277848,#277849,#277850,#277851,#277852,#277853,#277854,#277855,
#277856,#277857,#277858,#277859,#277860,#277861,#277862,#277863,#277864,
#277865,#277866,#277867,#277868,#277869,#277870,#277871,#277872,#277873,
#277874,#277875,#277876,#277877,#277878,#277879,#277880,#277881,#277882,
#277883,#277884,#277885,#277886,#277887,#277888,#277889,#277890,#277891,
#277892,#277893,#277894,#277895,#277896,#277897,#277898,#277899,#277900,
#277901,#277902,#277903,#277904,#277905,#277906,#277907,#277908,#277909,
#277910,#277911,#277912,#277913,#277914,#277915,#277916,#277917,#277918,
#277919,#277920,#277921,#277922,#277923,#277924,#277925,#277926,#277927,
#277928,#277929,#277930,#277931,#277932,#277933,#277934,#277935),
 .UNSPECIFIED.,.F.,.F.,(6,1,1,1,1,1,1,1,1,1,1,1,1,1,1,1,1,1,1,1,1,1,1,1,
1,1,1,1,1,1,1,1,1,1,1,1,1,1,1,1,1,1,1,1,1,1,1,1,1,1,1,1,1,1,1,1,1,1,1,1,
1,1,1,1,1,1,1,1,1,1,1,1,1,1,1,1,1,1,1,1,1,1,1,1,1,1,1,1,1,1,1,1,1,1,1,1,
1,1,1,1,1,1,1,1,1,1,1,1,1,1,1,1,1,1,1,1,1,1,1,1,1,1,1,1,1,1,1,1,1,1,1,1,
1,1,1,1,1,1,1,1,1,1,1,1,1,1,1,1,1,1,1,1,1,1,1,1,1,1,1,1,1,1,1,1,1,1,1,1,
1,1,1,1,1,1,1,1,1,1,1,1,1,1,1,1,1,1,1,1,1,1,1,1,1,1,1,1,1,1,1,1,1,1,1,1,
1,1,1,1,1,1,1,1,1,1,1,1,1,1,1,1,1,1,1,1,1,1,1,1,1,1,1,1,1,1,1,1,1,1,1,1,
1,1,1,1,1,1,1,1,1,1,1,1,1,1,1,1,1,1,1,1,1,1,1,1,1,1,1,1,1,1,1,1,1,1,1,1,
1,1,1,1,1,1,1,1,1,1,1,1,1,1,1,1,1,1,1,1,1,1,1,1,1,1,1,1,1,1,1,1,1,1,1,1,
1,1,1,1,1,1,1,1,1,1,1,1,1,1,1,1,1,1,1,1,1,1,1,1,1,1,1,1,1,1,1,1,1,1,1,1,
1,1,1,1,1,1,1,1,1,1,1,1,1,1,1,1,1,1,1,1,1,1,1,1,1,1,1,1,1,1,1,1,1,1,1,1,
1,1,1,1,1,1,1,1,1,1,1,1,1,1,1,1,1,1,1,1,1,1,1,1,1,1,1,1,1,1,1,1,1,1,1,1,
1,1,1,1,1,1,1,1,1,1,1,1,1,1,1,1,1,1,1,1,1,1,1,1,1,1,1,1,1,1,1,1,1,1,1,1,
1,1,1,1,1,1,1,1,1,1,6),(0.143172102,0.144954128,0.146788991,0.148623853,
0.150458716,0.152293578,0.15412844,0.155963303,0.157798165,0.159633028,
0.16146789,0.163302752,0.165137615,0.166972477,0.168807339,0.170642202,
0.172477064,0.174311927,0.176146789,0.177981651,0.179816514,0.181651376,
0.183486239,0.185321101,0.187155963,0.188990826,0.190825688,0.19266055,
0.194495413,0.196330275,0.198165138,0.2,0.201834862,0.203669725,0.205504587,
0.20733945,0.209174312,0.211009174,0.212844037,0.214678899,0.216513761,
0.218348624,0.220183486,0.222018349,0.223853211,0.225688073,0.227522936,
0.229357798,0.231192661,0.233027523,0.234862385,0.236697248,0.23853211,
0.240366972,0.242201835,0.244036697,0.24587156,0.247706422,0.249541284,
0.251376147,0.253211009,0.255045872,0.256880734,0.258715596,0.260550459,
0.262385321,0.264220183,0.266055046,0.267889908,0.269724771,0.271559633,
0.273394495,0.275229358,0.27706422,0.278899083,0.280733945,0.282568807,
0.28440367,0.286238532,0.288073394,0.289908257,0.291743119,0.293577982,
0.295412844,0.297247706,0.299082569,0.300917431,0.302752294,0.304587156,
0.306422018,0.308256881,0.310091743,0.311926606,0.313761468,0.31559633,
0.317431193,0.319266055,0.321100917,0.32293578,0.324770642,0.326605505,
0.328440367,0.330275229,0.332110092,0.333944954,0.335779817,0.337614679,
0.339449541,0.341284404,0.343119266,0.344954128,0.346788991,0.348623853,
0.350458716,0.352293578,0.35412844,0.355963303,0.357798165,0.359633028,
0.36146789,0.363302752,0.365137615,0.366972477,0.368807339,0.370642202,
0.372477064,0.374311927,0.376146789,0.377981651,0.379816514,0.381651376,
0.383486239,0.385321101,0.387155963,0.388990826,0.390825688,0.39266055,
0.394495413,0.396330275,0.398165138,0.4,0.401834862,0.403669725,0.405504587,
0.40733945,0.409174312,0.411009174,0.412844037,0.414678899,0.416513761,
0.418348624,0.420183486,0.422018349,0.423853211,0.425688073,0.427522936,
0.429357798,0.431192661,0.433027523,0.434862385,0.436697248,0.43853211,
0.440366972,0.442201835,0.444036697,0.44587156,0.447706422,0.449541284,
0.451376147,0.453211009,0.455045872,0.456880734,0.458715596,0.460550459,
0.462385321,0.464220183,0.466055046,0.467889908,0.469724771,0.471559633,
0.473394495,0.475229358,0.47706422,0.478899083,0.480733945,0.482568807,
0.48440367,0.486238532,0.488073394,0.489908257,0.491743119,0.493577982,
0.495412844,0.497247706,0.499082569,0.500917431,0.502752294,0.504587156,
0.506422018,0.508256881,0.510091743,0.511926606,0.513761468,0.51559633,
0.517431193,0.519266055,0.521100917,0.52293578,0.524770642,0.526605505,
0.528440367,0.530275229,0.532110092,0.533944954,0.535779817,0.537614679,
0.539449541,0.541284404,0.543119266,0.544954128,0.546788991,0.548623853,
0.550458716,0.552293578,0.55412844,0.555963303,0.557798165,0.559633028,
0.56146789,0.563302752,0.565137615,0.566972477,0.568807339,0.570642202,
0.572477064,0.574311927,0.576146789,0.577981651,0.579816514,0.581651376,
0.583486239,0.585321101,0.587155963,0.588990826,0.590825688,0.59266055,
0.594495413,0.596330275,0.598165138,0.6,0.601834862,0.603669725,0.605504587,
0.60733945,0.609174312,0.611009174,0.612844037,0.614678899,0.616513761,
0.618348624,0.620183486,0.622018349,0.623853211,0.625688073,0.627522936,
0.629357798,0.631192661,0.633027523,0.634862385,0.636697248,0.63853211,
0.640366972,0.642201835,0.644036697,0.64587156,0.647706422,0.649541284,
0.651376147,0.653211009,0.655045872,0.656880734,0.658715596,0.660550459,
0.662385321,0.664220183,0.666055046,0.667889908,0.669724771,0.671559633,
0.673394495,0.675229358,0.67706422,0.678899083,0.680733945,0.682568807,
0.68440367,0.686238532,0.688073394,0.689908257,0.691743119,0.693577982,
0.695412844,0.697247706,0.699082569,0.700917431,0.702752294,0.704587156,
0.706422018,0.708256881,0.710091743,0.711926606,0.713761468,0.71559633,
0.717431193,0.719266055,0.721100917,0.72293578,0.724770642,0.726605505,
0.728440367,0.730275229,0.732110092,0.733944954,0.735779817,0.737614679,
0.739449541,0.741284404,0.743119266,0.744954128,0.746788991,0.748623853,
0.750458716,0.752293578,0.75412844,0.755963303,0.757798165,0.759633028,
0.76146789,0.763302752,0.765137615,0.766972477,0.768807339,0.770642202,
0.772477064,0.774311927,0.776146789,0.777981651,0.779816514,0.781651376,
0.783486239,0.785321101,0.787155963,0.788990826,0.790825688,0.79266055,
0.794495413,0.796330275,0.798165138,0.8,0.801834862,0.803669725,0.805504587,
0.80733945,0.809174312,0.811009174,0.812844037,0.814678899,0.816513761,
0.818348624,0.820183486,0.822018349,0.823853211,0.825688073,0.827522936,
0.829357798,0.831192661,0.833027523,0.834862385,0.836697248,0.83853211,
0.840366972,0.842201835,0.844036697,0.84587156,0.847706422,0.849541284,
0.851376147,0.853211009,0.855045872,0.856880734,0.858715596,0.860550459,
0.862385321,0.864220183,0.866055046,0.867889908,0.869724771,0.871559633,
0.873394495,0.875229358,0.87706422,0.878899083,0.880733945,0.882568807,
0.88440367,0.886238532,0.888073394,0.889908257,0.893577982,0.895412844,
0.897247706,0.899082569,0.900917431,0.902752294,0.904587156,0.906422018,
0.908256881,0.910091743,0.911926606,0.913761468,0.91559633,0.917431193,
0.919266055,0.921100917,0.92293578,0.924770642,0.926605505,0.928440367,
0.930275229,0.932110092,0.933944954,0.935779817,0.937614679,0.939449541,
0.941284404,0.943119266,0.944954128,0.946788991,0.948623853,0.950458716,
0.952293578,0.95412844,0.955963303,0.957798165,0.959633028,0.96146789,0.963302752,
0.965137615,0.966972477,0.968807339,0.970642202,0.972477064,0.974311927,
0.976146789,0.977981651,0.979816514,0.981651376,0.983486239,0.985321101,
0.987155963,0.988990826,0.990825688,0.99266055,0.994495413,0.996330275,
0.998165138,1.),.UNSPECIFIED.);
#24469=B_SPLINE_CURVE_WITH_KNOTS('',3,(#278880,#278881,#278882,#278883,
#278884,#278885,#278886,#278887,#278888,#278889,#278890,#278891,#278892,
#278893,#278894,#278895,#278896,#278897,#278898,#278899,#278900,#278901,
#278902,#278903,#278904,#278905,#278906,#278907,#278908,#278909,#278910,
#278911,#278912,#278913,#278914,#278915,#278916,#278917,#278918,#278919,
#278920,#278921,#278922,#278923,#278924,#278925,#278926,#278927,#278928,
#278929,#278930,#278931,#278932,#278933,#278934,#278935,#278936,#278937,
#278938,#278939,#278940,#278941,#278942,#278943,#278944,#278945,#278946,
#278947,#278948,#278949,#278950,#278951,#278952,#278953,#278954,#278955,
#278956,#278957,#278958,#278959,#278960,#278961,#278962,#278963,#278964,
#278965,#278966,#278967,#278968,#278969,#278970,#278971,#278972,#278973,
#278974,#278975,#278976,#278977,#278978,#278979,#278980,#278981,#278982,
#278983,#278984,#278985,#278986,#278987,#278988,#278989,#278990,#278991,
#278992,#278993,#278994,#278995,#278996,#278997,#278998,#278999,#279000,
#279001,#279002,#279003,#279004,#279005,#279006,#279007,#279008,#279009,
#279010,#279011,#279012,#279013,#279014,#279015,#279016,#279017,#279018,
#279019,#279020,#279021,#279022,#279023,#279024,#279025,#279026,#279027,
#279028,#279029,#279030,#279031,#279032,#279033,#279034,#279035,#279036,
#279037,#279038,#279039,#279040,#279041,#279042,#279043,#279044,#279045,
#279046,#279047,#279048,#279049,#279050,#279051,#279052,#279053,#279054,
#279055,#279056,#279057,#279058,#279059,#279060,#279061,#279062,#279063,
#279064,#279065,#279066,#279067,#279068,#279069,#279070,#279071,#279072,
#279073,#279074,#279075,#279076,#279077,#279078,#279079,#279080,#279081,
#279082,#279083,#279084,#279085,#279086,#279087,#279088,#279089,#279090,
#279091,#279092,#279093,#279094,#279095,#279096,#279097,#279098,#279099,
#279100,#279101,#279102,#279103,#279104,#279105,#279106,#279107,#279108,
#279109,#279110,#279111,#279112,#279113,#279114,#279115,#279116,#279117,
#279118,#279119,#279120,#279121,#279122,#279123,#279124,#279125,#279126,
#279127,#279128,#279129,#279130,#279131,#279132,#279133,#279134,#279135,
#279136,#279137,#279138,#279139,#279140,#279141,#279142,#279143,#279144,
#279145,#279146,#279147,#279148,#279149,#279150,#279151,#279152,#279153,
#279154,#279155,#279156,#279157,#279158,#279159,#279160,#279161,#279162,
#279163,#279164,#279165,#279166,#279167,#279168,#279169,#279170,#279171,
#279172,#279173,#279174,#279175,#279176,#279177,#279178,#279179,#279180,
#279181,#279182,#279183,#279184,#279185,#279186,#279187,#279188,#279189,
#279190,#279191,#279192,#279193,#279194,#279195,#279196,#279197,#279198,
#279199,#279200,#279201),.UNSPECIFIED.,.F.,.F.,(4,3,3,3,3,3,3,3,3,3,3,3,
3,3,3,3,3,3,3,3,3,3,3,3,3,3,3,3,3,3,3,3,3,3,3,3,3,3,3,3,3,3,3,3,3,3,3,3,
3,3,3,3,3,3,3,3,3,3,3,3,3,3,3,3,3,3,3,3,3,3,3,3,3,3,3,3,3,3,3,3,3,3,3,3,
3,3,3,3,3,3,3,3,3,3,3,3,3,3,3,3,3,3,3,3,3,3,3,4),(0.143172102,0.15412844,
0.165137615,0.176146789,0.187155963,0.198165138,0.209174312,0.220183486,
0.231192661,0.242201835,0.253211009,0.264220183,0.275229358,0.286238532,
0.297247706,0.308256881,0.319266055,0.330275229,0.341284404,0.352293578,
0.363302752,0.374311927,0.385321101,0.396330275,0.405504587,0.414678899,
0.423853211,0.433027523,0.442201835,0.451376147,0.460550459,0.469724771,
0.478899083,0.488073394,0.497247706,0.506422018,0.51559633,0.524770642,
0.533944954,0.541284404,0.548623853,0.555963303,0.563302752,0.570642202,
0.577981651,0.585321101,0.59266055,0.6,0.60733945,0.614678899,0.622018349,
0.631192661,0.63853211,0.64587156,0.655045872,0.662385321,0.669724771,0.67706422,
0.68440367,0.691743119,0.699082569,0.708256881,0.71559633,0.72293578,0.730275229,
0.737614679,0.746788991,0.75412844,0.76146789,0.768807339,0.776146789,0.783486239,
0.790825688,0.798165138,0.805504587,0.811009174,0.816513761,0.822018349,
0.827522936,0.833027523,0.840366972,0.84587156,0.851376147,0.856880734,
0.862385321,0.867889908,0.873394495,0.878899083,0.88440367,0.889908257,
0.895412844,0.902752294,0.908256881,0.913761468,0.919266055,0.928440367,
0.935779817,0.941284404,0.946788991,0.952293578,0.959633028,0.966972477,
0.972477064,0.977981651,0.983486239,0.988990826,0.994495413,1.),
 .UNSPECIFIED.);
#24470=B_SPLINE_CURVE_WITH_KNOTS('',3,(#279202,#279203,#279204,#279205,
#279206,#279207,#279208,#279209,#279210,#279211,#279212,#279213,#279214,
#279215,#279216,#279217,#279218,#279219,#279220,#279221,#279222,#279223,
#279224,#279225,#279226,#279227,#279228,#279229,#279230,#279231,#279232,
#279233,#279234,#279235,#279236,#279237,#279238,#279239,#279240,#279241,
#279242,#279243,#279244,#279245,#279246,#279247,#279248,#279249,#279250,
#279251,#279252,#279253,#279254,#279255,#279256,#279257,#279258,#279259,
#279260,#279261,#279262,#279263,#279264,#279265,#279266,#279267,#279268,
#279269,#279270,#279271,#279272,#279273,#279274,#279275,#279276,#279277,
#279278,#279279,#279280,#279281,#279282,#279283,#279284,#279285,#279286,
#279287,#279288,#279289,#279290,#279291,#279292,#279293,#279294,#279295,
#279296,#279297,#279298,#279299,#279300,#279301,#279302,#279303,#279304,
#279305,#279306,#279307,#279308,#279309,#279310,#279311,#279312,#279313,
#279314,#279315,#279316,#279317,#279318,#279319,#279320,#279321,#279322,
#279323,#279324,#279325,#279326,#279327,#279328,#279329,#279330,#279331,
#279332,#279333,#279334,#279335,#279336,#279337,#279338,#279339,#279340,
#279341,#279342,#279343,#279344,#279345,#279346,#279347,#279348,#279349,
#279350,#279351,#279352,#279353,#279354,#279355,#279356,#279357,#279358,
#279359,#279360,#279361,#279362,#279363,#279364,#279365,#279366,#279367,
#279368,#279369,#279370,#279371,#279372,#279373,#279374,#279375,#279376,
#279377,#279378,#279379,#279380,#279381,#279382,#279383,#279384,#279385,
#279386,#279387,#279388,#279389,#279390,#279391,#279392,#279393,#279394,
#279395,#279396,#279397,#279398,#279399,#279400,#279401,#279402,#279403,
#279404,#279405,#279406,#279407,#279408,#279409,#279410,#279411,#279412,
#279413,#279414,#279415,#279416,#279417,#279418,#279419,#279420,#279421,
#279422,#279423,#279424,#279425,#279426,#279427,#279428,#279429,#279430,
#279431,#279432,#279433,#279434,#279435,#279436,#279437,#279438,#279439,
#279440,#279441,#279442,#279443,#279444,#279445,#279446,#279447,#279448,
#279449,#279450,#279451,#279452,#279453,#279454,#279455,#279456,#279457,
#279458,#279459,#279460,#279461,#279462,#279463,#279464,#279465,#279466,
#279467,#279468,#279469,#279470,#279471,#279472,#279473,#279474,#279475,
#279476,#279477,#279478,#279479,#279480,#279481,#279482,#279483,#279484,
#279485,#279486,#279487,#279488,#279489,#279490,#279491,#279492,#279493,
#279494,#279495,#279496,#279497,#279498,#279499,#279500,#279501,#279502,
#279503,#279504,#279505,#279506,#279507,#279508,#279509,#279510,#279511,
#279512,#279513,#279514,#279515,#279516,#279517,#279518,#279519,#279520,
#279521,#279522,#279523,#279524,#279525,#279526),.UNSPECIFIED.,.F.,.F.,
(4,3,3,3,3,3,3,3,3,3,3,3,3,3,3,3,3,3,3,3,3,3,3,3,3,3,3,3,3,3,3,3,3,3,3,
3,3,3,3,3,3,3,3,3,3,3,3,3,3,3,3,3,3,3,3,3,3,3,3,3,3,3,3,3,3,3,3,3,3,3,3,
3,3,3,3,3,3,3,3,3,3,3,3,3,3,3,3,3,3,3,3,3,3,3,3,3,3,3,3,3,3,3,3,3,3,3,3,
3,4),(0.143172102,0.15412844,0.165137615,0.176146789,0.187155963,0.198165138,
0.209174312,0.220183486,0.231192661,0.242201835,0.253211009,0.264220183,
0.275229358,0.286238532,0.297247706,0.308256881,0.319266055,0.330275229,
0.341284404,0.352293578,0.363302752,0.374311927,0.385321101,0.396330275,
0.405504587,0.414678899,0.423853211,0.433027523,0.442201835,0.451376147,
0.460550459,0.469724771,0.478899083,0.488073394,0.497247706,0.506422018,
0.51559633,0.524770642,0.533944954,0.541284404,0.548623853,0.555963303,
0.563302752,0.570642202,0.579816514,0.587155963,0.594495413,0.601834862,
0.609174312,0.616513761,0.623853211,0.631192661,0.63853211,0.64587156,0.653211009,
0.664220183,0.671559633,0.678899083,0.686238532,0.693577982,0.700917431,
0.708256881,0.71559633,0.72293578,0.730275229,0.737614679,0.744954128,0.752293578,
0.759633028,0.766972477,0.774311927,0.781651376,0.788990826,0.796330275,
0.803669725,0.811009174,0.816513761,0.822018349,0.827522936,0.833027523,
0.83853211,0.844036697,0.849541284,0.855045872,0.860550459,0.866055046,
0.871559633,0.87706422,0.882568807,0.889908257,0.895412844,0.902752294,
0.908256881,0.913761468,0.919266055,0.924770642,0.930275229,0.935779817,
0.941284404,0.946788991,0.952293578,0.957798165,0.966972477,0.972477064,
0.977981651,0.983486239,0.988990826,0.994495413,1.),.UNSPECIFIED.);
#24471=B_SPLINE_CURVE_WITH_KNOTS('',3,(#280486,#280487,#280488,#280489,
#280490,#280491,#280492,#280493,#280494,#280495,#280496,#280497,#280498,
#280499,#280500,#280501,#280502,#280503,#280504,#280505,#280506,#280507,
#280508,#280509,#280510,#280511,#280512,#280513,#280514,#280515,#280516,
#280517,#280518,#280519,#280520,#280521,#280522,#280523,#280524,#280525,
#280526,#280527,#280528,#280529,#280530,#280531,#280532,#280533,#280534,
#280535,#280536,#280537,#280538,#280539,#280540,#280541,#280542,#280543,
#280544,#280545,#280546,#280547,#280548,#280549,#280550,#280551,#280552,
#280553,#280554,#280555,#280556,#280557,#280558,#280559,#280560,#280561,
#280562,#280563,#280564,#280565,#280566,#280567,#280568,#280569,#280570,
#280571,#280572,#280573,#280574,#280575,#280576,#280577,#280578,#280579,
#280580,#280581,#280582,#280583,#280584,#280585,#280586,#280587,#280588,
#280589,#280590,#280591,#280592,#280593,#280594,#280595,#280596,#280597,
#280598,#280599,#280600,#280601,#280602,#280603,#280604,#280605,#280606,
#280607,#280608,#280609,#280610,#280611,#280612,#280613,#280614,#280615,
#280616,#280617,#280618,#280619,#280620,#280621,#280622,#280623,#280624,
#280625,#280626,#280627,#280628,#280629,#280630,#280631,#280632,#280633,
#280634,#280635,#280636,#280637,#280638,#280639,#280640,#280641,#280642,
#280643,#280644,#280645,#280646,#280647,#280648,#280649,#280650,#280651,
#280652,#280653,#280654,#280655,#280656,#280657,#280658,#280659,#280660,
#280661,#280662,#280663,#280664,#280665,#280666,#280667,#280668,#280669,
#280670,#280671,#280672,#280673,#280674,#280675,#280676,#280677,#280678,
#280679,#280680,#280681,#280682,#280683,#280684,#280685,#280686,#280687,
#280688,#280689,#280690,#280691,#280692,#280693,#280694,#280695,#280696,
#280697,#280698,#280699,#280700,#280701,#280702,#280703,#280704,#280705,
#280706,#280707,#280708,#280709,#280710,#280711,#280712,#280713,#280714,
#280715,#280716,#280717,#280718,#280719,#280720,#280721,#280722,#280723,
#280724,#280725,#280726,#280727,#280728,#280729,#280730,#280731,#280732,
#280733,#280734,#280735,#280736,#280737,#280738,#280739,#280740,#280741,
#280742,#280743,#280744,#280745,#280746,#280747,#280748,#280749,#280750,
#280751,#280752,#280753,#280754,#280755,#280756,#280757,#280758,#280759,
#280760,#280761,#280762,#280763,#280764,#280765,#280766,#280767,#280768,
#280769,#280770,#280771,#280772,#280773,#280774,#280775,#280776,#280777,
#280778,#280779,#280780,#280781,#280782,#280783,#280784,#280785,#280786,
#280787,#280788,#280789,#280790,#280791,#280792,#280793,#280794,#280795,
#280796,#280797,#280798,#280799,#280800,#280801,#280802,#280803,#280804,
#280805,#280806,#280807,#280808,#280809,#280810),.UNSPECIFIED.,.F.,.F.,
(4,3,3,3,3,3,3,3,3,3,3,3,3,3,3,3,3,3,3,3,3,3,3,3,3,3,3,3,3,3,3,3,3,3,3,
3,3,3,3,3,3,3,3,3,3,3,3,3,3,3,3,3,3,3,3,3,3,3,3,3,3,3,3,3,3,3,3,3,3,3,3,
3,3,3,3,3,3,3,3,3,3,3,3,3,3,3,3,3,3,3,3,3,3,3,3,3,3,3,3,3,3,3,3,3,3,3,3,
3,4),(0.143172102,0.15412844,0.165137615,0.176146789,0.187155963,0.198165138,
0.209174312,0.220183486,0.231192661,0.242201835,0.253211009,0.264220183,
0.275229358,0.286238532,0.297247706,0.308256881,0.319266055,0.330275229,
0.341284404,0.352293578,0.363302752,0.374311927,0.385321101,0.396330275,
0.405504587,0.414678899,0.423853211,0.433027523,0.442201835,0.451376147,
0.460550459,0.469724771,0.478899083,0.488073394,0.497247706,0.506422018,
0.51559633,0.526605505,0.533944954,0.541284404,0.550458716,0.557798165,
0.565137615,0.572477064,0.579816514,0.587155963,0.594495413,0.601834862,
0.611009174,0.618348624,0.625688073,0.633027523,0.640366972,0.647706422,
0.655045872,0.662385321,0.671559633,0.678899083,0.686238532,0.693577982,
0.700917431,0.708256881,0.71559633,0.72293578,0.730275229,0.737614679,0.744954128,
0.752293578,0.759633028,0.766972477,0.774311927,0.781651376,0.788990826,
0.798165138,0.80733945,0.812844037,0.818348624,0.823853211,0.829357798,
0.834862385,0.840366972,0.84587156,0.851376147,0.856880734,0.862385321,
0.867889908,0.873394495,0.878899083,0.88440367,0.889908257,0.895412844,
0.902752294,0.908256881,0.913761468,0.919266055,0.924770642,0.930275229,
0.935779817,0.941284404,0.946788991,0.952293578,0.959633028,0.965137615,
0.970642202,0.976146789,0.981651376,0.987155963,0.99266055,1.),
 .UNSPECIFIED.);
#24472=B_SPLINE_CURVE_WITH_KNOTS('',3,(#280811,#280812,#280813,#280814,
#280815,#280816,#280817,#280818,#280819,#280820,#280821,#280822,#280823,
#280824,#280825,#280826,#280827,#280828,#280829,#280830,#280831,#280832,
#280833,#280834,#280835,#280836,#280837,#280838,#280839,#280840,#280841,
#280842,#280843,#280844,#280845,#280846,#280847,#280848,#280849,#280850,
#280851,#280852,#280853,#280854,#280855,#280856,#280857,#280858,#280859,
#280860,#280861,#280862,#280863,#280864,#280865,#280866,#280867,#280868,
#280869,#280870,#280871,#280872,#280873,#280874,#280875,#280876,#280877,
#280878,#280879,#280880,#280881,#280882,#280883,#280884,#280885,#280886,
#280887,#280888,#280889,#280890,#280891,#280892,#280893,#280894,#280895,
#280896,#280897,#280898,#280899,#280900,#280901,#280902,#280903,#280904,
#280905,#280906,#280907,#280908,#280909,#280910,#280911,#280912,#280913,
#280914,#280915,#280916,#280917,#280918,#280919,#280920,#280921,#280922,
#280923,#280924,#280925,#280926,#280927,#280928,#280929,#280930,#280931,
#280932,#280933,#280934,#280935,#280936,#280937,#280938,#280939,#280940,
#280941,#280942,#280943,#280944,#280945,#280946,#280947,#280948,#280949,
#280950,#280951,#280952,#280953,#280954,#280955,#280956,#280957,#280958,
#280959,#280960,#280961,#280962,#280963,#280964,#280965,#280966,#280967,
#280968,#280969,#280970,#280971,#280972,#280973,#280974,#280975,#280976,
#280977,#280978,#280979,#280980,#280981,#280982,#280983,#280984,#280985,
#280986,#280987,#280988,#280989,#280990,#280991,#280992,#280993,#280994,
#280995,#280996,#280997,#280998,#280999,#281000,#281001,#281002,#281003,
#281004,#281005,#281006,#281007,#281008,#281009,#281010,#281011,#281012,
#281013,#281014,#281015,#281016,#281017,#281018,#281019,#281020,#281021,
#281022,#281023,#281024,#281025,#281026,#281027,#281028,#281029,#281030,
#281031,#281032,#281033,#281034,#281035,#281036,#281037,#281038,#281039,
#281040,#281041,#281042,#281043,#281044,#281045,#281046,#281047,#281048,
#281049,#281050,#281051,#281052,#281053,#281054,#281055,#281056,#281057,
#281058,#281059,#281060,#281061,#281062,#281063,#281064,#281065,#281066,
#281067,#281068,#281069,#281070,#281071,#281072,#281073,#281074,#281075,
#281076,#281077,#281078,#281079,#281080,#281081,#281082,#281083,#281084,
#281085,#281086,#281087,#281088,#281089,#281090,#281091,#281092,#281093,
#281094,#281095,#281096,#281097,#281098,#281099,#281100,#281101,#281102,
#281103,#281104,#281105,#281106,#281107,#281108,#281109,#281110,#281111,
#281112,#281113,#281114,#281115,#281116,#281117,#281118,#281119,#281120,
#281121,#281122,#281123,#281124,#281125,#281126,#281127,#281128,#281129,
#281130,#281131,#281132),.UNSPECIFIED.,.F.,.F.,(4,3,3,3,3,3,3,3,3,3,3,3,
3,3,3,3,3,3,3,3,3,3,3,3,3,3,3,3,3,3,3,3,3,3,3,3,3,3,3,3,3,3,3,3,3,3,3,3,
3,3,3,3,3,3,3,3,3,3,3,3,3,3,3,3,3,3,3,3,3,3,3,3,3,3,3,3,3,3,3,3,3,3,3,3,
3,3,3,3,3,3,3,3,3,3,3,3,3,3,3,3,3,3,3,3,3,3,3,4),(0.143172102,0.15412844,
0.165137615,0.176146789,0.187155963,0.198165138,0.209174312,0.220183486,
0.231192661,0.242201835,0.253211009,0.264220183,0.275229358,0.286238532,
0.297247706,0.308256881,0.319266055,0.330275229,0.341284404,0.352293578,
0.363302752,0.374311927,0.385321101,0.396330275,0.405504587,0.414678899,
0.423853211,0.433027523,0.442201835,0.451376147,0.460550459,0.469724771,
0.478899083,0.488073394,0.497247706,0.506422018,0.51559633,0.524770642,
0.533944954,0.543119266,0.550458716,0.557798165,0.565137615,0.572477064,
0.579816514,0.587155963,0.594495413,0.601834862,0.609174312,0.616513761,
0.623853211,0.631192661,0.63853211,0.64587156,0.653211009,0.660550459,0.667889908,
0.67706422,0.68440367,0.691743119,0.699082569,0.706422018,0.713761468,0.721100917,
0.728440367,0.735779817,0.743119266,0.750458716,0.757798165,0.765137615,
0.772477064,0.779816514,0.787155963,0.794495413,0.803669725,0.811009174,
0.818348624,0.823853211,0.829357798,0.834862385,0.840366972,0.84587156,
0.851376147,0.856880734,0.862385321,0.867889908,0.873394495,0.878899083,
0.886238532,0.891743119,0.899082569,0.904587156,0.910091743,0.91559633,
0.921100917,0.926605505,0.932110092,0.937614679,0.943119266,0.948623853,
0.95412844,0.959633028,0.965137615,0.972477064,0.979816514,0.985321101,
0.990825688,1.),.UNSPECIFIED.);
#24473=B_SPLINE_CURVE_WITH_KNOTS('',3,(#282080,#282081,#282082,#282083,
#282084,#282085,#282086,#282087,#282088,#282089,#282090,#282091,#282092,
#282093,#282094,#282095,#282096,#282097,#282098,#282099,#282100,#282101,
#282102,#282103,#282104,#282105,#282106,#282107,#282108,#282109,#282110,
#282111,#282112,#282113,#282114,#282115,#282116,#282117,#282118,#282119,
#282120,#282121,#282122,#282123,#282124,#282125,#282126,#282127,#282128,
#282129,#282130,#282131,#282132,#282133,#282134,#282135,#282136,#282137,
#282138,#282139,#282140,#282141,#282142,#282143,#282144,#282145,#282146,
#282147,#282148,#282149,#282150,#282151,#282152,#282153,#282154,#282155,
#282156,#282157,#282158,#282159,#282160,#282161,#282162,#282163,#282164,
#282165,#282166,#282167,#282168,#282169,#282170,#282171,#282172,#282173,
#282174,#282175,#282176,#282177,#282178,#282179,#282180,#282181,#282182,
#282183,#282184,#282185,#282186,#282187,#282188,#282189,#282190,#282191,
#282192,#282193,#282194,#282195,#282196,#282197,#282198,#282199,#282200,
#282201,#282202,#282203,#282204,#282205,#282206,#282207,#282208,#282209,
#282210,#282211,#282212,#282213,#282214,#282215,#282216,#282217,#282218,
#282219,#282220,#282221,#282222,#282223,#282224,#282225,#282226,#282227,
#282228,#282229,#282230,#282231,#282232,#282233,#282234,#282235,#282236,
#282237,#282238,#282239,#282240,#282241,#282242,#282243,#282244,#282245,
#282246,#282247,#282248,#282249,#282250,#282251,#282252,#282253,#282254,
#282255,#282256,#282257,#282258,#282259,#282260,#282261,#282262,#282263,
#282264,#282265,#282266,#282267,#282268,#282269,#282270,#282271,#282272,
#282273,#282274,#282275,#282276,#282277,#282278,#282279,#282280,#282281,
#282282,#282283,#282284,#282285,#282286,#282287,#282288,#282289,#282290,
#282291,#282292,#282293,#282294,#282295,#282296,#282297,#282298,#282299,
#282300,#282301,#282302,#282303,#282304,#282305,#282306,#282307,#282308,
#282309,#282310,#282311,#282312,#282313,#282314,#282315,#282316,#282317,
#282318,#282319,#282320,#282321,#282322,#282323,#282324,#282325,#282326,
#282327,#282328,#282329,#282330,#282331,#282332,#282333,#282334,#282335,
#282336,#282337,#282338,#282339,#282340,#282341,#282342,#282343,#282344,
#282345,#282346,#282347,#282348,#282349,#282350,#282351,#282352,#282353,
#282354,#282355,#282356,#282357,#282358,#282359,#282360,#282361,#282362,
#282363,#282364,#282365,#282366,#282367,#282368,#282369,#282370,#282371,
#282372,#282373,#282374,#282375,#282376,#282377,#282378,#282379,#282380,
#282381,#282382,#282383,#282384,#282385,#282386,#282387,#282388,#282389,
#282390,#282391,#282392,#282393,#282394,#282395,#282396,#282397,#282398,
#282399,#282400,#282401,#282402,#282403,#282404,#282405,#282406,#282407),
 .UNSPECIFIED.,.F.,.F.,(4,3,3,3,3,3,3,3,3,3,3,3,3,3,3,3,3,3,3,3,3,3,3,3,
3,3,3,3,3,3,3,3,3,3,3,3,3,3,3,3,3,3,3,3,3,3,3,3,3,3,3,3,3,3,3,3,3,3,3,3,
3,3,3,3,3,3,3,3,3,3,3,3,3,3,3,3,3,3,3,3,3,3,3,3,3,3,3,3,3,3,3,3,3,3,3,3,
3,3,3,3,3,3,3,3,3,3,3,3,3,4),(-1.,-0.994495413,-0.988990826,-0.983486239,
-0.977981651,-0.972477064,-0.966972477,-0.959633028,-0.95412844,-0.948623853,
-0.943119266,-0.937614679,-0.932110092,-0.926605505,-0.921100917,-0.91559633,
-0.910091743,-0.904587156,-0.899082569,-0.893577982,-0.888073394,-0.882568807,
-0.87706422,-0.871559633,-0.866055046,-0.860550459,-0.855045872,-0.849541284,
-0.844036697,-0.83853211,-0.833027523,-0.827522936,-0.822018349,-0.816513761,
-0.811009174,-0.805504587,-0.798165138,-0.790825688,-0.783486239,-0.776146789,
-0.768807339,-0.76146789,-0.75412844,-0.746788991,-0.739449541,-0.732110092,
-0.724770642,-0.717431193,-0.710091743,-0.702752294,-0.695412844,-0.688073394,
-0.680733945,-0.673394495,-0.666055046,-0.658715596,-0.651376147,-0.644036697,
-0.636697248,-0.629357798,-0.622018349,-0.614678899,-0.60733945,-0.6,-0.59266055,
-0.585321101,-0.577981651,-0.570642202,-0.559633028,-0.552293578,-0.544954128,
-0.537614679,-0.530275229,-0.521100917,-0.511926606,-0.502752294,-0.493577982,
-0.48440367,-0.475229358,-0.466055046,-0.456880734,-0.447706422,-0.43853211,
-0.429357798,-0.420183486,-0.411009174,-0.401834862,-0.39266055,-0.381651376,
-0.370642202,-0.359633028,-0.348623853,-0.337614679,-0.326605505,-0.31559633,
-0.304587156,-0.293577982,-0.282568807,-0.271559633,-0.260550459,-0.249541284,
-0.23853211,-0.227522936,-0.216513761,-0.205504587,-0.194495413,-0.183486239,
-0.172477064,-0.16146789,-0.143172102),.UNSPECIFIED.);
#24474=B_SPLINE_CURVE_WITH_KNOTS('',3,(#282408,#282409,#282410,#282411,
#282412,#282413,#282414,#282415,#282416,#282417,#282418,#282419,#282420,
#282421,#282422,#282423,#282424,#282425,#282426,#282427,#282428,#282429,
#282430,#282431,#282432,#282433,#282434,#282435,#282436,#282437,#282438,
#282439,#282440,#282441,#282442,#282443,#282444,#282445,#282446,#282447,
#282448,#282449,#282450,#282451,#282452,#282453,#282454,#282455,#282456,
#282457,#282458,#282459,#282460,#282461,#282462,#282463,#282464,#282465,
#282466,#282467,#282468,#282469,#282470,#282471,#282472,#282473,#282474,
#282475,#282476,#282477,#282478,#282479,#282480,#282481,#282482,#282483,
#282484,#282485,#282486,#282487,#282488,#282489,#282490,#282491,#282492,
#282493,#282494,#282495,#282496,#282497,#282498,#282499,#282500,#282501,
#282502,#282503,#282504,#282505,#282506,#282507,#282508,#282509,#282510,
#282511,#282512,#282513,#282514,#282515,#282516,#282517,#282518,#282519,
#282520,#282521,#282522,#282523,#282524,#282525,#282526,#282527,#282528,
#282529,#282530,#282531,#282532,#282533,#282534,#282535,#282536,#282537,
#282538,#282539,#282540,#282541,#282542,#282543,#282544,#282545,#282546,
#282547,#282548,#282549,#282550,#282551,#282552,#282553,#282554,#282555,
#282556,#282557,#282558,#282559,#282560,#282561,#282562,#282563,#282564,
#282565,#282566,#282567,#282568,#282569,#282570,#282571,#282572,#282573,
#282574,#282575,#282576,#282577,#282578,#282579,#282580,#282581,#282582,
#282583,#282584,#282585,#282586,#282587,#282588,#282589,#282590,#282591,
#282592,#282593,#282594,#282595,#282596,#282597,#282598,#282599,#282600,
#282601,#282602,#282603,#282604,#282605,#282606,#282607,#282608,#282609,
#282610,#282611,#282612,#282613,#282614,#282615,#282616,#282617,#282618,
#282619,#282620,#282621,#282622,#282623,#282624,#282625,#282626,#282627,
#282628,#282629,#282630,#282631,#282632,#282633,#282634,#282635,#282636,
#282637,#282638,#282639,#282640,#282641,#282642,#282643,#282644,#282645,
#282646,#282647,#282648,#282649,#282650,#282651,#282652,#282653,#282654,
#282655,#282656,#282657,#282658,#282659,#282660,#282661,#282662,#282663,
#282664,#282665,#282666,#282667,#282668,#282669,#282670,#282671,#282672,
#282673,#282674,#282675,#282676,#282677,#282678,#282679,#282680,#282681,
#282682,#282683,#282684,#282685,#282686,#282687,#282688,#282689,#282690,
#282691,#282692,#282693,#282694,#282695,#282696,#282697,#282698,#282699,
#282700,#282701,#282702,#282703,#282704,#282705,#282706,#282707,#282708,
#282709,#282710,#282711,#282712,#282713,#282714,#282715,#282716,#282717,
#282718,#282719,#282720,#282721,#282722,#282723,#282724,#282725,#282726,
#282727,#282728,#282729,#282730,#282731,#282732,#282733,#282734,#282735),
 .UNSPECIFIED.,.F.,.F.,(4,3,3,3,3,3,3,3,3,3,3,3,3,3,3,3,3,3,3,3,3,3,3,3,
3,3,3,3,3,3,3,3,3,3,3,3,3,3,3,3,3,3,3,3,3,3,3,3,3,3,3,3,3,3,3,3,3,3,3,3,
3,3,3,3,3,3,3,3,3,3,3,3,3,3,3,3,3,3,3,3,3,3,3,3,3,3,3,3,3,3,3,3,3,3,3,3,
3,3,3,3,3,3,3,3,3,3,3,3,3,4),(0.143172102,0.15412844,0.165137615,0.176146789,
0.187155963,0.198165138,0.209174312,0.220183486,0.231192661,0.242201835,
0.253211009,0.264220183,0.275229358,0.286238532,0.297247706,0.308256881,
0.319266055,0.330275229,0.341284404,0.352293578,0.363302752,0.374311927,
0.385321101,0.396330275,0.405504587,0.414678899,0.423853211,0.433027523,
0.442201835,0.451376147,0.460550459,0.469724771,0.478899083,0.488073394,
0.497247706,0.506422018,0.51559633,0.524770642,0.533944954,0.541284404,
0.548623853,0.555963303,0.563302752,0.572477064,0.579816514,0.587155963,
0.594495413,0.601834862,0.609174312,0.616513761,0.623853211,0.631192661,
0.63853211,0.64587156,0.653211009,0.660550459,0.667889908,0.675229358,0.682568807,
0.689908257,0.697247706,0.704587156,0.711926606,0.719266055,0.726605505,
0.733944954,0.741284404,0.748623853,0.755963303,0.763302752,0.770642202,
0.777981651,0.785321101,0.79266055,0.8,0.809174312,0.814678899,0.820183486,
0.825688073,0.831192661,0.836697248,0.842201835,0.847706422,0.853211009,
0.858715596,0.864220183,0.869724771,0.875229358,0.880733945,0.886238532,
0.891743119,0.897247706,0.902752294,0.908256881,0.913761468,0.919266055,
0.924770642,0.930275229,0.935779817,0.941284404,0.946788991,0.952293578,
0.957798165,0.963302752,0.968807339,0.974311927,0.979816514,0.985321101,
0.990825688,1.),.UNSPECIFIED.);
#24475=B_SPLINE_CURVE_WITH_KNOTS('',5,(#283698,#283699,#283700,#283701,
#283702,#283703,#283704,#283705,#283706,#283707,#283708,#283709,#283710,
#283711,#283712,#283713,#283714,#283715,#283716,#283717,#283718,#283719,
#283720,#283721,#283722,#283723,#283724,#283725,#283726,#283727,#283728,
#283729,#283730,#283731,#283732,#283733,#283734,#283735,#283736,#283737,
#283738,#283739,#283740,#283741,#283742,#283743,#283744,#283745,#283746,
#283747,#283748,#283749,#283750,#283751,#283752,#283753,#283754,#283755,
#283756,#283757,#283758,#283759,#283760,#283761,#283762,#283763,#283764,
#283765,#283766,#283767,#283768,#283769,#283770,#283771,#283772,#283773,
#283774,#283775,#283776,#283777,#283778,#283779,#283780,#283781,#283782,
#283783,#283784,#283785,#283786,#283787,#283788,#283789,#283790,#283791,
#283792,#283793,#283794,#283795,#283796,#283797,#283798,#283799,#283800,
#283801,#283802,#283803,#283804,#283805,#283806,#283807,#283808,#283809,
#283810,#283811,#283812,#283813,#283814,#283815,#283816,#283817,#283818,
#283819,#283820,#283821,#283822,#283823,#283824,#283825,#283826,#283827,
#283828,#283829,#283830,#283831,#283832,#283833,#283834,#283835,#283836,
#283837,#283838,#283839,#283840,#283841,#283842,#283843,#283844,#283845,
#283846,#283847,#283848,#283849,#283850,#283851,#283852,#283853,#283854,
#283855,#283856,#283857,#283858,#283859,#283860,#283861,#283862,#283863,
#283864,#283865,#283866,#283867,#283868,#283869,#283870,#283871,#283872,
#283873,#283874,#283875,#283876,#283877,#283878,#283879,#283880,#283881,
#283882,#283883,#283884,#283885,#283886,#283887,#283888,#283889,#283890,
#283891,#283892,#283893,#283894,#283895,#283896,#283897,#283898,#283899,
#283900,#283901,#283902,#283903,#283904,#283905,#283906,#283907,#283908,
#283909,#283910,#283911,#283912,#283913,#283914,#283915,#283916,#283917,
#283918,#283919,#283920,#283921,#283922,#283923,#283924,#283925,#283926,
#283927,#283928,#283929,#283930,#283931,#283932,#283933,#283934,#283935,
#283936,#283937,#283938,#283939,#283940,#283941,#283942,#283943,#283944,
#283945,#283946,#283947,#283948,#283949,#283950,#283951,#283952,#283953,
#283954,#283955,#283956,#283957,#283958,#283959,#283960,#283961,#283962,
#283963,#283964,#283965,#283966,#283967,#283968,#283969,#283970,#283971,
#283972,#283973,#283974,#283975,#283976,#283977,#283978,#283979,#283980,
#283981,#283982,#283983,#283984,#283985,#283986,#283987,#283988,#283989,
#283990,#283991,#283992,#283993,#283994,#283995,#283996,#283997,#283998,
#283999,#284000,#284001,#284002,#284003,#284004,#284005,#284006,#284007,
#284008,#284009,#284010,#284011,#284012,#284013,#284014,#284015,#284016,
#284017,#284018,#284019,#284020,#284021,#284022,#284023,#284024,#284025,
#284026,#284027,#284028,#284029,#284030,#284031,#284032,#284033,#284034,
#284035,#284036,#284037,#284038,#284039,#284040,#284041,#284042,#284043,
#284044,#284045,#284046,#284047,#284048,#284049,#284050,#284051,#284052,
#284053,#284054,#284055,#284056,#284057,#284058,#284059,#284060,#284061,
#284062,#284063,#284064,#284065,#284066,#284067,#284068,#284069,#284070,
#284071,#284072,#284073,#284074,#284075,#284076,#284077,#284078,#284079,
#284080,#284081,#284082,#284083,#284084,#284085,#284086,#284087,#284088,
#284089,#284090,#284091,#284092,#284093,#284094,#284095,#284096,#284097,
#284098,#284099,#284100,#284101,#284102,#284103,#284104,#284105,#284106,
#284107,#284108,#284109,#284110,#284111,#284112,#284113,#284114,#284115,
#284116,#284117,#284118,#284119,#284120,#284121,#284122,#284123,#284124,
#284125,#284126,#284127,#284128,#284129,#284130,#284131,#284132,#284133,
#284134,#284135,#284136,#284137,#284138,#284139,#284140,#284141,#284142,
#284143,#284144,#284145,#284146,#284147,#284148,#284149,#284150,#284151,
#284152,#284153,#284154,#284155,#284156,#284157,#284158,#284159,#284160,
#284161,#284162,#284163,#284164,#284165,#284166,#284167,#284168,#284169),
 .UNSPECIFIED.,.F.,.F.,(6,1,1,1,1,1,1,1,1,1,1,1,1,1,1,1,1,1,1,1,1,1,1,1,
1,1,1,1,1,1,1,1,1,1,1,1,1,1,1,1,1,1,1,1,1,1,1,1,1,1,1,1,1,1,1,1,1,1,1,1,
1,1,1,1,1,1,1,1,1,1,1,1,1,1,1,1,1,1,1,1,1,1,1,1,1,1,1,1,1,1,1,1,1,1,1,1,
1,1,1,1,1,1,1,1,1,1,1,1,1,1,1,1,1,1,1,1,1,1,1,1,1,1,1,1,1,1,1,1,1,1,1,1,
1,1,1,1,1,1,1,1,1,1,1,1,1,1,1,1,1,1,1,1,1,1,1,1,1,1,1,1,1,1,1,1,1,1,1,1,
1,1,1,1,1,1,1,1,1,1,1,1,1,1,1,1,1,1,1,1,1,1,1,1,1,1,1,1,1,1,1,1,1,1,1,1,
1,1,1,1,1,1,1,1,1,1,1,1,1,1,1,1,1,1,1,1,1,1,1,1,1,1,1,1,1,1,1,1,1,1,1,1,
1,1,1,1,1,1,1,1,1,1,1,1,1,1,1,1,1,1,1,1,1,1,1,1,1,1,1,1,1,1,1,1,1,1,1,1,
1,1,1,1,1,1,1,1,1,1,1,1,1,1,1,1,1,1,1,1,1,1,1,1,1,1,1,1,1,1,1,1,1,1,1,1,
1,1,1,1,1,1,1,1,1,1,1,1,1,1,1,1,1,1,1,1,1,1,1,1,1,1,1,1,1,1,1,1,1,1,1,1,
1,1,1,1,1,1,1,1,1,1,1,1,1,1,1,1,1,1,1,1,1,1,1,1,1,1,1,1,1,1,1,1,1,1,1,1,
1,1,1,1,1,1,1,1,1,1,1,1,1,1,1,1,1,1,1,1,1,1,1,1,1,1,1,1,1,1,1,1,1,1,1,1,
1,1,1,1,1,1,1,1,1,1,1,1,1,1,1,1,1,1,1,1,1,1,1,1,1,1,1,1,1,1,1,1,1,1,1,1,
1,1,1,1,1,1,1,1,1,1,1,6),(-1.,-0.998165138,-0.996330275,-0.994495413,-0.99266055,
-0.990825688,-0.988990826,-0.987155963,-0.985321101,-0.983486239,-0.981651376,
-0.979816514,-0.977981651,-0.976146789,-0.974311927,-0.972477064,-0.970642202,
-0.968807339,-0.966972477,-0.965137615,-0.963302752,-0.96146789,-0.959633028,
-0.957798165,-0.955963303,-0.95412844,-0.952293578,-0.950458716,-0.948623853,
-0.946788991,-0.944954128,-0.943119266,-0.941284404,-0.939449541,-0.937614679,
-0.935779817,-0.933944954,-0.932110092,-0.930275229,-0.928440367,-0.926605505,
-0.924770642,-0.92293578,-0.921100917,-0.919266055,-0.917431193,-0.91559633,
-0.913761468,-0.911926606,-0.910091743,-0.908256881,-0.906422018,-0.904587156,
-0.902752294,-0.900917431,-0.899082569,-0.897247706,-0.895412844,-0.893577982,
-0.891743119,-0.889908257,-0.888073394,-0.886238532,-0.88440367,-0.882568807,
-0.880733945,-0.878899083,-0.87706422,-0.875229358,-0.873394495,-0.871559633,
-0.869724771,-0.867889908,-0.866055046,-0.864220183,-0.862385321,-0.860550459,
-0.858715596,-0.856880734,-0.855045872,-0.853211009,-0.851376147,-0.849541284,
-0.847706422,-0.84587156,-0.844036697,-0.842201835,-0.840366972,-0.83853211,
-0.836697248,-0.834862385,-0.833027523,-0.831192661,-0.829357798,-0.827522936,
-0.825688073,-0.823853211,-0.822018349,-0.820183486,-0.818348624,-0.816513761,
-0.814678899,-0.812844037,-0.811009174,-0.809174312,-0.80733945,-0.805504587,
-0.803669725,-0.801834862,-0.8,-0.798165138,-0.796330275,-0.794495413,-0.79266055,
-0.790825688,-0.788990826,-0.787155963,-0.785321101,-0.783486239,-0.781651376,
-0.779816514,-0.777981651,-0.776146789,-0.774311927,-0.772477064,-0.770642202,
-0.768807339,-0.766972477,-0.765137615,-0.763302752,-0.76146789,-0.759633028,
-0.757798165,-0.755963303,-0.75412844,-0.752293578,-0.750458716,-0.748623853,
-0.746788991,-0.744954128,-0.743119266,-0.741284404,-0.739449541,-0.737614679,
-0.735779817,-0.733944954,-0.732110092,-0.730275229,-0.728440367,-0.726605505,
-0.724770642,-0.72293578,-0.721100917,-0.719266055,-0.717431193,-0.71559633,
-0.713761468,-0.711926606,-0.710091743,-0.708256881,-0.706422018,-0.704587156,
-0.702752294,-0.700917431,-0.699082569,-0.697247706,-0.695412844,-0.693577982,
-0.691743119,-0.689908257,-0.688073394,-0.686238532,-0.68440367,-0.682568807,
-0.680733945,-0.678899083,-0.67706422,-0.675229358,-0.673394495,-0.671559633,
-0.669724771,-0.667889908,-0.666055046,-0.664220183,-0.662385321,-0.660550459,
-0.658715596,-0.656880734,-0.655045872,-0.653211009,-0.651376147,-0.649541284,
-0.647706422,-0.64587156,-0.644036697,-0.642201835,-0.640366972,-0.63853211,
-0.636697248,-0.634862385,-0.633027523,-0.631192661,-0.629357798,-0.627522936,
-0.625688073,-0.623853211,-0.622018349,-0.620183486,-0.618348624,-0.616513761,
-0.614678899,-0.612844037,-0.611009174,-0.609174312,-0.60733945,-0.605504587,
-0.603669725,-0.601834862,-0.6,-0.598165138,-0.596330275,-0.594495413,-0.59266055,
-0.590825688,-0.588990826,-0.587155963,-0.585321101,-0.583486239,-0.581651376,
-0.579816514,-0.577981651,-0.576146789,-0.574311927,-0.572477064,-0.570642202,
-0.568807339,-0.566972477,-0.565137615,-0.563302752,-0.56146789,-0.559633028,
-0.557798165,-0.555963303,-0.55412844,-0.552293578,-0.550458716,-0.548623853,
-0.546788991,-0.544954128,-0.543119266,-0.541284404,-0.539449541,-0.537614679,
-0.535779817,-0.533944954,-0.532110092,-0.530275229,-0.528440367,-0.526605505,
-0.524770642,-0.52293578,-0.521100917,-0.519266055,-0.517431193,-0.51559633,
-0.513761468,-0.511926606,-0.510091743,-0.508256881,-0.506422018,-0.504587156,
-0.502752294,-0.500917431,-0.499082569,-0.497247706,-0.495412844,-0.493577982,
-0.491743119,-0.489908257,-0.488073394,-0.486238532,-0.48440367,-0.482568807,
-0.480733945,-0.478899083,-0.47706422,-0.475229358,-0.473394495,-0.471559633,
-0.469724771,-0.467889908,-0.466055046,-0.464220183,-0.462385321,-0.460550459,
-0.458715596,-0.456880734,-0.455045872,-0.453211009,-0.451376147,-0.449541284,
-0.447706422,-0.44587156,-0.444036697,-0.442201835,-0.440366972,-0.43853211,
-0.436697248,-0.434862385,-0.433027523,-0.431192661,-0.429357798,-0.427522936,
-0.425688073,-0.423853211,-0.422018349,-0.420183486,-0.418348624,-0.416513761,
-0.414678899,-0.412844037,-0.411009174,-0.409174312,-0.40733945,-0.405504587,
-0.403669725,-0.401834862,-0.4,-0.398165138,-0.396330275,-0.394495413,-0.39266055,
-0.390825688,-0.388990826,-0.387155963,-0.385321101,-0.383486239,-0.381651376,
-0.379816514,-0.377981651,-0.376146789,-0.374311927,-0.372477064,-0.370642202,
-0.368807339,-0.366972477,-0.365137615,-0.363302752,-0.36146789,-0.359633028,
-0.357798165,-0.355963303,-0.35412844,-0.352293578,-0.350458716,-0.348623853,
-0.346788991,-0.344954128,-0.343119266,-0.341284404,-0.339449541,-0.337614679,
-0.335779817,-0.333944954,-0.332110092,-0.330275229,-0.328440367,-0.326605505,
-0.324770642,-0.32293578,-0.321100917,-0.319266055,-0.317431193,-0.31559633,
-0.313761468,-0.311926606,-0.310091743,-0.308256881,-0.306422018,-0.304587156,
-0.302752294,-0.300917431,-0.299082569,-0.297247706,-0.295412844,-0.293577982,
-0.291743119,-0.289908257,-0.288073394,-0.286238532,-0.28440367,-0.282568807,
-0.280733945,-0.278899083,-0.27706422,-0.275229358,-0.273394495,-0.271559633,
-0.269724771,-0.267889908,-0.266055046,-0.264220183,-0.262385321,-0.260550459,
-0.258715596,-0.256880734,-0.255045872,-0.253211009,-0.251376147,-0.249541284,
-0.247706422,-0.24587156,-0.244036697,-0.242201835,-0.240366972,-0.23853211,
-0.236697248,-0.234862385,-0.233027523,-0.231192661,-0.229357798,-0.227522936,
-0.225688073,-0.223853211,-0.222018349,-0.220183486,-0.218348624,-0.216513761,
-0.214678899,-0.212844037,-0.211009174,-0.209174312,-0.20733945,-0.205504587,
-0.203669725,-0.201834862,-0.2,-0.198165138,-0.196330275,-0.194495413,-0.19266055,
-0.190825688,-0.188990826,-0.187155963,-0.185321101,-0.183486239,-0.181651376,
-0.179816514,-0.177981651,-0.176146789,-0.174311927,-0.172477064,-0.170642202,
-0.168807339,-0.166972477,-0.165137615,-0.163302752,-0.16146789,-0.159633028,
-0.157798165,-0.155963303,-0.15412844,-0.152293578,-0.150458716,-0.148623853,
-0.146788991,-0.144954128,-0.143172102),.UNSPECIFIED.);
#24476=B_SPLINE_CURVE_WITH_KNOTS('',5,(#284170,#284171,#284172,#284173,
#284174,#284175,#284176,#284177,#284178,#284179,#284180,#284181,#284182,
#284183,#284184,#284185,#284186,#284187,#284188,#284189,#284190,#284191,
#284192,#284193,#284194,#284195,#284196,#284197,#284198,#284199,#284200,
#284201,#284202,#284203,#284204,#284205,#284206,#284207,#284208,#284209,
#284210,#284211,#284212,#284213,#284214,#284215,#284216,#284217,#284218,
#284219,#284220,#284221,#284222,#284223,#284224,#284225,#284226,#284227,
#284228,#284229,#284230,#284231,#284232,#284233,#284234,#284235,#284236,
#284237,#284238,#284239,#284240,#284241,#284242,#284243,#284244,#284245,
#284246,#284247,#284248,#284249,#284250,#284251,#284252,#284253,#284254,
#284255,#284256,#284257,#284258,#284259,#284260,#284261,#284262,#284263,
#284264,#284265,#284266,#284267,#284268,#284269,#284270,#284271,#284272,
#284273,#284274,#284275,#284276,#284277,#284278,#284279,#284280,#284281,
#284282,#284283,#284284,#284285,#284286,#284287,#284288,#284289,#284290,
#284291,#284292,#284293,#284294,#284295,#284296,#284297,#284298,#284299,
#284300,#284301,#284302,#284303,#284304,#284305,#284306,#284307,#284308,
#284309,#284310,#284311,#284312,#284313,#284314,#284315,#284316,#284317,
#284318,#284319,#284320,#284321,#284322,#284323,#284324,#284325,#284326,
#284327,#284328,#284329,#284330,#284331,#284332,#284333,#284334,#284335,
#284336,#284337,#284338,#284339,#284340,#284341,#284342,#284343,#284344,
#284345,#284346,#284347,#284348,#284349,#284350,#284351,#284352,#284353,
#284354,#284355,#284356,#284357,#284358,#284359,#284360,#284361,#284362,
#284363,#284364,#284365,#284366,#284367,#284368,#284369,#284370,#284371,
#284372,#284373,#284374,#284375,#284376,#284377,#284378,#284379,#284380,
#284381,#284382,#284383,#284384,#284385,#284386,#284387,#284388,#284389,
#284390,#284391,#284392,#284393,#284394,#284395,#284396,#284397,#284398,
#284399,#284400,#284401,#284402,#284403,#284404,#284405,#284406,#284407,
#284408,#284409,#284410,#284411,#284412,#284413,#284414,#284415,#284416,
#284417,#284418,#284419,#284420,#284421,#284422,#284423,#284424,#284425,
#284426,#284427,#284428,#284429,#284430,#284431,#284432,#284433,#284434,
#284435,#284436,#284437,#284438,#284439,#284440,#284441,#284442,#284443,
#284444,#284445,#284446,#284447,#284448,#284449,#284450,#284451,#284452,
#284453,#284454,#284455,#284456,#284457,#284458,#284459,#284460,#284461,
#284462,#284463,#284464,#284465,#284466,#284467,#284468,#284469,#284470,
#284471,#284472,#284473,#284474,#284475,#284476,#284477,#284478,#284479,
#284480,#284481,#284482,#284483,#284484,#284485,#284486,#284487,#284488,
#284489,#284490,#284491,#284492,#284493,#284494,#284495,#284496,#284497,
#284498,#284499,#284500,#284501,#284502,#284503,#284504,#284505,#284506,
#284507,#284508,#284509,#284510,#284511,#284512,#284513,#284514,#284515,
#284516,#284517,#284518,#284519,#284520,#284521,#284522,#284523,#284524,
#284525,#284526,#284527,#284528,#284529,#284530,#284531,#284532,#284533,
#284534,#284535,#284536,#284537,#284538,#284539,#284540,#284541,#284542,
#284543,#284544,#284545,#284546,#284547,#284548,#284549,#284550,#284551,
#284552,#284553,#284554,#284555,#284556,#284557,#284558,#284559,#284560,
#284561,#284562,#284563,#284564,#284565,#284566,#284567,#284568,#284569,
#284570,#284571,#284572,#284573,#284574,#284575,#284576,#284577,#284578,
#284579,#284580,#284581,#284582,#284583,#284584,#284585,#284586,#284587,
#284588,#284589,#284590,#284591,#284592,#284593,#284594,#284595,#284596,
#284597,#284598,#284599,#284600,#284601,#284602,#284603,#284604,#284605,
#284606,#284607,#284608,#284609,#284610,#284611,#284612,#284613,#284614,
#284615,#284616,#284617,#284618,#284619,#284620,#284621,#284622,#284623,
#284624,#284625,#284626,#284627,#284628,#284629,#284630,#284631,#284632,
#284633,#284634,#284635,#284636,#284637,#284638,#284639,#284640,#284641),
 .UNSPECIFIED.,.F.,.F.,(6,1,1,1,1,1,1,1,1,1,1,1,1,1,1,1,1,1,1,1,1,1,1,1,
1,1,1,1,1,1,1,1,1,1,1,1,1,1,1,1,1,1,1,1,1,1,1,1,1,1,1,1,1,1,1,1,1,1,1,1,
1,1,1,1,1,1,1,1,1,1,1,1,1,1,1,1,1,1,1,1,1,1,1,1,1,1,1,1,1,1,1,1,1,1,1,1,
1,1,1,1,1,1,1,1,1,1,1,1,1,1,1,1,1,1,1,1,1,1,1,1,1,1,1,1,1,1,1,1,1,1,1,1,
1,1,1,1,1,1,1,1,1,1,1,1,1,1,1,1,1,1,1,1,1,1,1,1,1,1,1,1,1,1,1,1,1,1,1,1,
1,1,1,1,1,1,1,1,1,1,1,1,1,1,1,1,1,1,1,1,1,1,1,1,1,1,1,1,1,1,1,1,1,1,1,1,
1,1,1,1,1,1,1,1,1,1,1,1,1,1,1,1,1,1,1,1,1,1,1,1,1,1,1,1,1,1,1,1,1,1,1,1,
1,1,1,1,1,1,1,1,1,1,1,1,1,1,1,1,1,1,1,1,1,1,1,1,1,1,1,1,1,1,1,1,1,1,1,1,
1,1,1,1,1,1,1,1,1,1,1,1,1,1,1,1,1,1,1,1,1,1,1,1,1,1,1,1,1,1,1,1,1,1,1,1,
1,1,1,1,1,1,1,1,1,1,1,1,1,1,1,1,1,1,1,1,1,1,1,1,1,1,1,1,1,1,1,1,1,1,1,1,
1,1,1,1,1,1,1,1,1,1,1,1,1,1,1,1,1,1,1,1,1,1,1,1,1,1,1,1,1,1,1,1,1,1,1,1,
1,1,1,1,1,1,1,1,1,1,1,1,1,1,1,1,1,1,1,1,1,1,1,1,1,1,1,1,1,1,1,1,1,1,1,1,
1,1,1,1,1,1,1,1,1,1,1,1,1,1,1,1,1,1,1,1,1,1,1,1,1,1,1,1,1,1,1,1,1,1,1,1,
1,1,1,1,1,1,1,1,1,1,1,6),(0.143172102,0.144954128,0.146788991,0.148623853,
0.150458716,0.152293578,0.15412844,0.155963303,0.157798165,0.159633028,
0.16146789,0.163302752,0.165137615,0.166972477,0.168807339,0.170642202,
0.172477064,0.174311927,0.176146789,0.177981651,0.179816514,0.181651376,
0.183486239,0.185321101,0.187155963,0.188990826,0.190825688,0.19266055,
0.194495413,0.196330275,0.198165138,0.2,0.201834862,0.203669725,0.205504587,
0.20733945,0.209174312,0.211009174,0.212844037,0.214678899,0.216513761,
0.218348624,0.220183486,0.222018349,0.223853211,0.225688073,0.227522936,
0.229357798,0.231192661,0.233027523,0.234862385,0.236697248,0.23853211,
0.240366972,0.242201835,0.244036697,0.24587156,0.247706422,0.249541284,
0.251376147,0.253211009,0.255045872,0.256880734,0.258715596,0.260550459,
0.262385321,0.264220183,0.266055046,0.267889908,0.269724771,0.271559633,
0.273394495,0.275229358,0.27706422,0.278899083,0.280733945,0.282568807,
0.28440367,0.286238532,0.288073394,0.289908257,0.291743119,0.293577982,
0.295412844,0.297247706,0.299082569,0.300917431,0.302752294,0.304587156,
0.306422018,0.308256881,0.310091743,0.311926606,0.313761468,0.31559633,
0.317431193,0.319266055,0.321100917,0.32293578,0.324770642,0.326605505,
0.328440367,0.330275229,0.332110092,0.333944954,0.335779817,0.337614679,
0.339449541,0.341284404,0.343119266,0.344954128,0.346788991,0.348623853,
0.350458716,0.352293578,0.35412844,0.355963303,0.357798165,0.359633028,
0.36146789,0.363302752,0.365137615,0.366972477,0.368807339,0.370642202,
0.372477064,0.374311927,0.376146789,0.377981651,0.379816514,0.381651376,
0.383486239,0.385321101,0.387155963,0.388990826,0.390825688,0.39266055,
0.394495413,0.396330275,0.398165138,0.4,0.401834862,0.403669725,0.405504587,
0.40733945,0.409174312,0.411009174,0.412844037,0.414678899,0.416513761,
0.418348624,0.420183486,0.422018349,0.423853211,0.425688073,0.427522936,
0.429357798,0.431192661,0.433027523,0.434862385,0.436697248,0.43853211,
0.440366972,0.442201835,0.444036697,0.44587156,0.447706422,0.449541284,
0.451376147,0.453211009,0.455045872,0.456880734,0.458715596,0.460550459,
0.462385321,0.464220183,0.466055046,0.467889908,0.469724771,0.471559633,
0.473394495,0.475229358,0.47706422,0.478899083,0.480733945,0.482568807,
0.48440367,0.486238532,0.488073394,0.489908257,0.491743119,0.493577982,
0.495412844,0.497247706,0.499082569,0.500917431,0.502752294,0.504587156,
0.506422018,0.508256881,0.510091743,0.511926606,0.513761468,0.51559633,
0.517431193,0.519266055,0.521100917,0.52293578,0.524770642,0.526605505,
0.528440367,0.530275229,0.532110092,0.533944954,0.535779817,0.537614679,
0.539449541,0.541284404,0.543119266,0.544954128,0.546788991,0.548623853,
0.550458716,0.552293578,0.55412844,0.555963303,0.557798165,0.559633028,
0.56146789,0.563302752,0.565137615,0.566972477,0.568807339,0.570642202,
0.572477064,0.574311927,0.576146789,0.577981651,0.579816514,0.581651376,
0.583486239,0.585321101,0.587155963,0.588990826,0.590825688,0.59266055,
0.594495413,0.596330275,0.598165138,0.6,0.601834862,0.603669725,0.605504587,
0.60733945,0.609174312,0.611009174,0.612844037,0.614678899,0.616513761,
0.618348624,0.620183486,0.622018349,0.623853211,0.625688073,0.627522936,
0.629357798,0.631192661,0.633027523,0.634862385,0.636697248,0.63853211,
0.640366972,0.642201835,0.644036697,0.64587156,0.647706422,0.649541284,
0.651376147,0.653211009,0.655045872,0.656880734,0.658715596,0.660550459,
0.662385321,0.664220183,0.666055046,0.667889908,0.669724771,0.671559633,
0.673394495,0.675229358,0.67706422,0.678899083,0.680733945,0.682568807,
0.68440367,0.686238532,0.688073394,0.689908257,0.691743119,0.693577982,
0.695412844,0.697247706,0.699082569,0.700917431,0.702752294,0.704587156,
0.706422018,0.708256881,0.710091743,0.711926606,0.713761468,0.71559633,
0.717431193,0.719266055,0.721100917,0.72293578,0.724770642,0.726605505,
0.728440367,0.730275229,0.732110092,0.733944954,0.735779817,0.737614679,
0.739449541,0.741284404,0.743119266,0.744954128,0.746788991,0.748623853,
0.750458716,0.752293578,0.75412844,0.755963303,0.757798165,0.759633028,
0.76146789,0.763302752,0.765137615,0.766972477,0.768807339,0.770642202,
0.772477064,0.774311927,0.776146789,0.777981651,0.779816514,0.781651376,
0.783486239,0.785321101,0.787155963,0.788990826,0.790825688,0.79266055,
0.794495413,0.796330275,0.798165138,0.8,0.801834862,0.803669725,0.805504587,
0.80733945,0.809174312,0.811009174,0.812844037,0.814678899,0.816513761,
0.818348624,0.820183486,0.822018349,0.823853211,0.825688073,0.827522936,
0.829357798,0.831192661,0.833027523,0.834862385,0.836697248,0.83853211,
0.840366972,0.842201835,0.844036697,0.84587156,0.847706422,0.849541284,
0.851376147,0.853211009,0.855045872,0.856880734,0.858715596,0.860550459,
0.862385321,0.864220183,0.866055046,0.867889908,0.869724771,0.871559633,
0.873394495,0.875229358,0.87706422,0.878899083,0.880733945,0.882568807,
0.88440367,0.886238532,0.888073394,0.889908257,0.891743119,0.893577982,
0.895412844,0.897247706,0.899082569,0.900917431,0.902752294,0.904587156,
0.906422018,0.908256881,0.910091743,0.911926606,0.913761468,0.91559633,
0.917431193,0.919266055,0.921100917,0.92293578,0.924770642,0.926605505,
0.928440367,0.930275229,0.932110092,0.933944954,0.935779817,0.937614679,
0.939449541,0.941284404,0.943119266,0.944954128,0.946788991,0.948623853,
0.950458716,0.952293578,0.95412844,0.955963303,0.957798165,0.959633028,
0.96146789,0.963302752,0.965137615,0.966972477,0.968807339,0.970642202,
0.972477064,0.974311927,0.976146789,0.977981651,0.979816514,0.981651376,
0.983486239,0.985321101,0.987155963,0.988990826,0.990825688,0.99266055,
0.994495413,0.996330275,0.998165138,1.),.UNSPECIFIED.);
#24477=B_SPLINE_CURVE_WITH_KNOTS('',5,(#285586,#285587,#285588,#285589,
#285590,#285591,#285592,#285593,#285594,#285595,#285596,#285597,#285598,
#285599,#285600,#285601,#285602,#285603,#285604,#285605,#285606,#285607,
#285608,#285609,#285610,#285611,#285612,#285613,#285614,#285615,#285616,
#285617,#285618,#285619,#285620,#285621,#285622,#285623,#285624,#285625,
#285626,#285627,#285628,#285629,#285630,#285631,#285632,#285633,#285634,
#285635,#285636,#285637,#285638,#285639,#285640,#285641,#285642,#285643,
#285644,#285645,#285646,#285647,#285648,#285649,#285650,#285651,#285652,
#285653,#285654,#285655,#285656,#285657,#285658,#285659,#285660,#285661,
#285662,#285663,#285664,#285665,#285666,#285667,#285668,#285669,#285670,
#285671,#285672,#285673,#285674,#285675,#285676,#285677,#285678,#285679,
#285680,#285681,#285682,#285683,#285684,#285685,#285686,#285687,#285688,
#285689,#285690,#285691,#285692,#285693,#285694,#285695,#285696,#285697,
#285698,#285699,#285700,#285701,#285702,#285703,#285704,#285705,#285706,
#285707,#285708,#285709,#285710,#285711,#285712,#285713,#285714,#285715,
#285716,#285717,#285718,#285719,#285720,#285721,#285722,#285723,#285724,
#285725,#285726,#285727,#285728,#285729,#285730,#285731,#285732,#285733,
#285734,#285735,#285736,#285737,#285738,#285739,#285740,#285741,#285742,
#285743,#285744,#285745,#285746,#285747,#285748,#285749,#285750,#285751,
#285752,#285753,#285754,#285755,#285756,#285757,#285758,#285759,#285760,
#285761,#285762,#285763,#285764,#285765,#285766,#285767,#285768,#285769,
#285770,#285771,#285772,#285773,#285774,#285775,#285776,#285777,#285778,
#285779,#285780,#285781,#285782,#285783,#285784,#285785,#285786,#285787,
#285788,#285789,#285790,#285791,#285792,#285793,#285794,#285795,#285796,
#285797,#285798,#285799,#285800,#285801,#285802,#285803,#285804,#285805,
#285806,#285807,#285808,#285809,#285810,#285811,#285812,#285813,#285814,
#285815,#285816,#285817,#285818,#285819,#285820,#285821,#285822,#285823,
#285824,#285825,#285826,#285827,#285828,#285829,#285830,#285831,#285832,
#285833,#285834,#285835,#285836,#285837,#285838,#285839,#285840,#285841,
#285842,#285843,#285844,#285845,#285846,#285847,#285848,#285849,#285850,
#285851,#285852,#285853,#285854,#285855,#285856,#285857,#285858,#285859,
#285860,#285861,#285862,#285863,#285864,#285865,#285866,#285867,#285868,
#285869,#285870,#285871,#285872,#285873,#285874,#285875,#285876,#285877,
#285878,#285879,#285880,#285881,#285882,#285883,#285884,#285885,#285886,
#285887,#285888,#285889,#285890,#285891,#285892,#285893,#285894,#285895,
#285896,#285897,#285898,#285899,#285900,#285901,#285902,#285903,#285904,
#285905,#285906,#285907,#285908,#285909,#285910,#285911,#285912,#285913,
#285914,#285915,#285916,#285917,#285918,#285919,#285920,#285921,#285922,
#285923,#285924,#285925,#285926,#285927,#285928,#285929,#285930,#285931,
#285932,#285933,#285934,#285935,#285936,#285937,#285938,#285939,#285940,
#285941,#285942,#285943,#285944,#285945,#285946,#285947,#285948,#285949,
#285950,#285951,#285952,#285953,#285954,#285955,#285956,#285957,#285958,
#285959,#285960,#285961,#285962,#285963,#285964,#285965,#285966,#285967,
#285968,#285969,#285970,#285971,#285972,#285973,#285974,#285975,#285976,
#285977,#285978,#285979,#285980,#285981,#285982,#285983,#285984,#285985,
#285986,#285987,#285988,#285989,#285990,#285991,#285992,#285993,#285994,
#285995,#285996,#285997,#285998,#285999,#286000,#286001,#286002,#286003,
#286004,#286005,#286006,#286007,#286008,#286009,#286010,#286011,#286012,
#286013,#286014,#286015,#286016,#286017,#286018,#286019,#286020,#286021,
#286022,#286023,#286024,#286025,#286026,#286027,#286028,#286029,#286030,
#286031,#286032,#286033,#286034,#286035,#286036,#286037,#286038,#286039,
#286040,#286041,#286042,#286043,#286044,#286045,#286046,#286047,#286048,
#286049,#286050,#286051,#286052,#286053,#286054,#286055,#286056,#286057),
 .UNSPECIFIED.,.F.,.F.,(6,1,1,1,1,1,1,1,1,1,1,1,1,1,1,1,1,1,1,1,1,1,1,1,
1,1,1,1,1,1,1,1,1,1,1,1,1,1,1,1,1,1,1,1,1,1,1,1,1,1,1,1,1,1,1,1,1,1,1,1,
1,1,1,1,1,1,1,1,1,1,1,1,1,1,1,1,1,1,1,1,1,1,1,1,1,1,1,1,1,1,1,1,1,1,1,1,
1,1,1,1,1,1,1,1,1,1,1,1,1,1,1,1,1,1,1,1,1,1,1,1,1,1,1,1,1,1,1,1,1,1,1,1,
1,1,1,1,1,1,1,1,1,1,1,1,1,1,1,1,1,1,1,1,1,1,1,1,1,1,1,1,1,1,1,1,1,1,1,1,
1,1,1,1,1,1,1,1,1,1,1,1,1,1,1,1,1,1,1,1,1,1,1,1,1,1,1,1,1,1,1,1,1,1,1,1,
1,1,1,1,1,1,1,1,1,1,1,1,1,1,1,1,1,1,1,1,1,1,1,1,1,1,1,1,1,1,1,1,1,1,1,1,
1,1,1,1,1,1,1,1,1,1,1,1,1,1,1,1,1,1,1,1,1,1,1,1,1,1,1,1,1,1,1,1,1,1,1,1,
1,1,1,1,1,1,1,1,1,1,1,1,1,1,1,1,1,1,1,1,1,1,1,1,1,1,1,1,1,1,1,1,1,1,1,1,
1,1,1,1,1,1,1,1,1,1,1,1,1,1,1,1,1,1,1,1,1,1,1,1,1,1,1,1,1,1,1,1,1,1,1,1,
1,1,1,1,1,1,1,1,1,1,1,1,1,1,1,1,1,1,1,1,1,1,1,1,1,1,1,1,1,1,1,1,1,1,1,1,
1,1,1,1,1,1,1,1,1,1,1,1,1,1,1,1,1,1,1,1,1,1,1,1,1,1,1,1,1,1,1,1,1,1,1,1,
1,1,1,1,1,1,1,1,1,1,1,1,1,1,1,1,1,1,1,1,1,1,1,1,1,1,1,1,1,1,1,1,1,1,1,1,
1,1,1,1,1,1,1,1,1,1,1,6),(0.143172102,0.144954128,0.146788991,0.148623853,
0.150458716,0.152293578,0.15412844,0.155963303,0.157798165,0.159633028,
0.16146789,0.163302752,0.165137615,0.166972477,0.168807339,0.170642202,
0.172477064,0.174311927,0.176146789,0.177981651,0.179816514,0.181651376,
0.183486239,0.185321101,0.187155963,0.188990826,0.190825688,0.19266055,
0.194495413,0.196330275,0.198165138,0.2,0.201834862,0.203669725,0.205504587,
0.20733945,0.209174312,0.211009174,0.212844037,0.214678899,0.216513761,
0.218348624,0.220183486,0.222018349,0.223853211,0.225688073,0.227522936,
0.229357798,0.231192661,0.233027523,0.234862385,0.236697248,0.23853211,
0.240366972,0.242201835,0.244036697,0.24587156,0.247706422,0.249541284,
0.251376147,0.253211009,0.255045872,0.256880734,0.258715596,0.260550459,
0.262385321,0.264220183,0.266055046,0.267889908,0.269724771,0.271559633,
0.273394495,0.275229358,0.27706422,0.278899083,0.280733945,0.282568807,
0.28440367,0.286238532,0.288073394,0.289908257,0.291743119,0.293577982,
0.295412844,0.297247706,0.299082569,0.300917431,0.302752294,0.304587156,
0.306422018,0.308256881,0.310091743,0.311926606,0.313761468,0.31559633,
0.317431193,0.319266055,0.321100917,0.32293578,0.324770642,0.326605505,
0.328440367,0.330275229,0.332110092,0.333944954,0.335779817,0.337614679,
0.339449541,0.341284404,0.343119266,0.344954128,0.346788991,0.348623853,
0.350458716,0.352293578,0.35412844,0.355963303,0.357798165,0.359633028,
0.36146789,0.363302752,0.365137615,0.366972477,0.368807339,0.370642202,
0.372477064,0.374311927,0.376146789,0.377981651,0.379816514,0.381651376,
0.383486239,0.385321101,0.387155963,0.388990826,0.390825688,0.39266055,
0.394495413,0.396330275,0.398165138,0.4,0.401834862,0.403669725,0.405504587,
0.40733945,0.409174312,0.411009174,0.412844037,0.414678899,0.416513761,
0.418348624,0.420183486,0.422018349,0.423853211,0.425688073,0.427522936,
0.429357798,0.431192661,0.433027523,0.434862385,0.436697248,0.43853211,
0.440366972,0.442201835,0.444036697,0.44587156,0.447706422,0.449541284,
0.451376147,0.453211009,0.455045872,0.456880734,0.458715596,0.460550459,
0.462385321,0.464220183,0.466055046,0.467889908,0.469724771,0.471559633,
0.473394495,0.475229358,0.47706422,0.478899083,0.480733945,0.482568807,
0.48440367,0.486238532,0.488073394,0.489908257,0.491743119,0.493577982,
0.495412844,0.497247706,0.499082569,0.500917431,0.502752294,0.504587156,
0.506422018,0.508256881,0.510091743,0.511926606,0.513761468,0.51559633,
0.517431193,0.519266055,0.521100917,0.52293578,0.524770642,0.526605505,
0.528440367,0.530275229,0.532110092,0.533944954,0.535779817,0.537614679,
0.539449541,0.541284404,0.543119266,0.544954128,0.546788991,0.548623853,
0.550458716,0.552293578,0.55412844,0.555963303,0.557798165,0.559633028,
0.56146789,0.563302752,0.565137615,0.566972477,0.568807339,0.570642202,
0.572477064,0.574311927,0.576146789,0.577981651,0.579816514,0.581651376,
0.583486239,0.585321101,0.587155963,0.588990826,0.590825688,0.59266055,
0.594495413,0.596330275,0.598165138,0.6,0.601834862,0.603669725,0.605504587,
0.60733945,0.609174312,0.611009174,0.612844037,0.614678899,0.616513761,
0.618348624,0.620183486,0.622018349,0.623853211,0.625688073,0.627522936,
0.629357798,0.631192661,0.633027523,0.634862385,0.636697248,0.63853211,
0.640366972,0.642201835,0.644036697,0.64587156,0.647706422,0.649541284,
0.651376147,0.653211009,0.655045872,0.656880734,0.658715596,0.660550459,
0.662385321,0.664220183,0.666055046,0.667889908,0.669724771,0.671559633,
0.673394495,0.675229358,0.67706422,0.678899083,0.680733945,0.682568807,
0.68440367,0.686238532,0.688073394,0.689908257,0.691743119,0.693577982,
0.695412844,0.697247706,0.699082569,0.700917431,0.702752294,0.704587156,
0.706422018,0.708256881,0.710091743,0.711926606,0.713761468,0.71559633,
0.717431193,0.719266055,0.721100917,0.72293578,0.724770642,0.726605505,
0.728440367,0.730275229,0.732110092,0.733944954,0.735779817,0.737614679,
0.739449541,0.741284404,0.743119266,0.744954128,0.746788991,0.748623853,
0.750458716,0.752293578,0.75412844,0.755963303,0.757798165,0.759633028,
0.76146789,0.763302752,0.765137615,0.766972477,0.768807339,0.770642202,
0.772477064,0.774311927,0.776146789,0.777981651,0.779816514,0.781651376,
0.783486239,0.785321101,0.787155963,0.788990826,0.790825688,0.79266055,
0.794495413,0.796330275,0.798165138,0.8,0.801834862,0.803669725,0.805504587,
0.80733945,0.809174312,0.811009174,0.812844037,0.814678899,0.816513761,
0.818348624,0.820183486,0.822018349,0.823853211,0.825688073,0.827522936,
0.829357798,0.831192661,0.833027523,0.834862385,0.836697248,0.83853211,
0.840366972,0.842201835,0.844036697,0.84587156,0.847706422,0.849541284,
0.851376147,0.853211009,0.855045872,0.856880734,0.858715596,0.860550459,
0.862385321,0.864220183,0.866055046,0.867889908,0.869724771,0.871559633,
0.873394495,0.875229358,0.87706422,0.878899083,0.880733945,0.882568807,
0.88440367,0.886238532,0.888073394,0.889908257,0.891743119,0.893577982,
0.895412844,0.897247706,0.899082569,0.900917431,0.902752294,0.904587156,
0.906422018,0.908256881,0.910091743,0.911926606,0.913761468,0.91559633,
0.917431193,0.919266055,0.921100917,0.92293578,0.924770642,0.926605505,
0.928440367,0.930275229,0.932110092,0.933944954,0.935779817,0.937614679,
0.939449541,0.941284404,0.943119266,0.944954128,0.946788991,0.948623853,
0.950458716,0.952293578,0.95412844,0.955963303,0.957798165,0.959633028,
0.96146789,0.963302752,0.965137615,0.966972477,0.968807339,0.970642202,
0.972477064,0.974311927,0.976146789,0.977981651,0.979816514,0.981651376,
0.983486239,0.985321101,0.987155963,0.988990826,0.990825688,0.99266055,
0.994495413,0.996330275,0.998165138,1.),.UNSPECIFIED.);
#24478=B_SPLINE_CURVE_WITH_KNOTS('',5,(#286058,#286059,#286060,#286061,
#286062,#286063,#286064,#286065,#286066,#286067,#286068,#286069,#286070,
#286071,#286072,#286073,#286074,#286075,#286076,#286077,#286078,#286079,
#286080,#286081,#286082,#286083,#286084,#286085,#286086,#286087,#286088,
#286089,#286090,#286091,#286092,#286093,#286094,#286095,#286096,#286097,
#286098,#286099,#286100,#286101,#286102,#286103,#286104,#286105,#286106,
#286107,#286108,#286109,#286110,#286111,#286112,#286113,#286114,#286115,
#286116,#286117,#286118,#286119,#286120,#286121,#286122,#286123,#286124,
#286125,#286126,#286127,#286128,#286129,#286130,#286131,#286132,#286133,
#286134,#286135,#286136,#286137,#286138,#286139,#286140,#286141,#286142,
#286143,#286144,#286145,#286146,#286147,#286148,#286149,#286150,#286151,
#286152,#286153,#286154,#286155,#286156,#286157,#286158,#286159,#286160,
#286161,#286162,#286163,#286164,#286165,#286166,#286167,#286168,#286169,
#286170,#286171,#286172,#286173,#286174,#286175,#286176,#286177,#286178,
#286179,#286180,#286181,#286182,#286183,#286184,#286185,#286186,#286187,
#286188,#286189,#286190,#286191,#286192,#286193,#286194,#286195,#286196,
#286197,#286198,#286199,#286200,#286201,#286202,#286203,#286204,#286205,
#286206,#286207,#286208,#286209,#286210,#286211,#286212,#286213,#286214,
#286215,#286216,#286217,#286218,#286219,#286220,#286221,#286222,#286223,
#286224,#286225,#286226,#286227,#286228,#286229,#286230,#286231,#286232,
#286233,#286234,#286235,#286236,#286237,#286238,#286239,#286240,#286241,
#286242,#286243,#286244,#286245,#286246,#286247,#286248,#286249,#286250,
#286251,#286252,#286253,#286254,#286255,#286256,#286257,#286258,#286259,
#286260,#286261,#286262,#286263,#286264,#286265,#286266,#286267,#286268,
#286269,#286270,#286271,#286272,#286273,#286274,#286275,#286276,#286277,
#286278,#286279,#286280,#286281,#286282,#286283,#286284,#286285,#286286,
#286287,#286288,#286289,#286290,#286291,#286292,#286293,#286294,#286295,
#286296,#286297,#286298,#286299,#286300,#286301,#286302,#286303,#286304,
#286305,#286306,#286307,#286308,#286309,#286310,#286311,#286312,#286313,
#286314,#286315,#286316,#286317,#286318,#286319,#286320,#286321,#286322,
#286323,#286324,#286325,#286326,#286327,#286328,#286329,#286330,#286331,
#286332,#286333,#286334,#286335,#286336,#286337,#286338,#286339,#286340,
#286341,#286342,#286343,#286344,#286345,#286346,#286347,#286348,#286349,
#286350,#286351,#286352,#286353,#286354,#286355,#286356,#286357,#286358,
#286359,#286360,#286361,#286362,#286363,#286364,#286365,#286366,#286367,
#286368,#286369,#286370,#286371,#286372,#286373,#286374,#286375,#286376,
#286377,#286378,#286379,#286380,#286381,#286382,#286383,#286384,#286385,
#286386,#286387,#286388,#286389,#286390,#286391,#286392,#286393,#286394,
#286395,#286396,#286397,#286398,#286399,#286400,#286401,#286402,#286403,
#286404,#286405,#286406,#286407,#286408,#286409,#286410,#286411,#286412,
#286413,#286414,#286415,#286416,#286417,#286418,#286419,#286420,#286421,
#286422,#286423,#286424,#286425,#286426,#286427,#286428,#286429,#286430,
#286431,#286432,#286433,#286434,#286435,#286436,#286437,#286438,#286439,
#286440,#286441,#286442,#286443,#286444,#286445,#286446,#286447,#286448,
#286449,#286450,#286451,#286452,#286453,#286454,#286455,#286456,#286457,
#286458,#286459,#286460,#286461,#286462,#286463,#286464,#286465,#286466,
#286467,#286468,#286469,#286470,#286471,#286472,#286473,#286474,#286475,
#286476,#286477,#286478,#286479,#286480,#286481,#286482,#286483,#286484,
#286485,#286486,#286487,#286488,#286489,#286490,#286491,#286492,#286493,
#286494,#286495,#286496,#286497,#286498,#286499,#286500,#286501,#286502,
#286503,#286504,#286505,#286506,#286507,#286508,#286509,#286510,#286511,
#286512,#286513,#286514,#286515,#286516,#286517,#286518,#286519,#286520,
#286521,#286522,#286523,#286524,#286525,#286526,#286527,#286528,#286529),
 .UNSPECIFIED.,.F.,.F.,(6,1,1,1,1,1,1,1,1,1,1,1,1,1,1,1,1,1,1,1,1,1,1,1,
1,1,1,1,1,1,1,1,1,1,1,1,1,1,1,1,1,1,1,1,1,1,1,1,1,1,1,1,1,1,1,1,1,1,1,1,
1,1,1,1,1,1,1,1,1,1,1,1,1,1,1,1,1,1,1,1,1,1,1,1,1,1,1,1,1,1,1,1,1,1,1,1,
1,1,1,1,1,1,1,1,1,1,1,1,1,1,1,1,1,1,1,1,1,1,1,1,1,1,1,1,1,1,1,1,1,1,1,1,
1,1,1,1,1,1,1,1,1,1,1,1,1,1,1,1,1,1,1,1,1,1,1,1,1,1,1,1,1,1,1,1,1,1,1,1,
1,1,1,1,1,1,1,1,1,1,1,1,1,1,1,1,1,1,1,1,1,1,1,1,1,1,1,1,1,1,1,1,1,1,1,1,
1,1,1,1,1,1,1,1,1,1,1,1,1,1,1,1,1,1,1,1,1,1,1,1,1,1,1,1,1,1,1,1,1,1,1,1,
1,1,1,1,1,1,1,1,1,1,1,1,1,1,1,1,1,1,1,1,1,1,1,1,1,1,1,1,1,1,1,1,1,1,1,1,
1,1,1,1,1,1,1,1,1,1,1,1,1,1,1,1,1,1,1,1,1,1,1,1,1,1,1,1,1,1,1,1,1,1,1,1,
1,1,1,1,1,1,1,1,1,1,1,1,1,1,1,1,1,1,1,1,1,1,1,1,1,1,1,1,1,1,1,1,1,1,1,1,
1,1,1,1,1,1,1,1,1,1,1,1,1,1,1,1,1,1,1,1,1,1,1,1,1,1,1,1,1,1,1,1,1,1,1,1,
1,1,1,1,1,1,1,1,1,1,1,1,1,1,1,1,1,1,1,1,1,1,1,1,1,1,1,1,1,1,1,1,1,1,1,1,
1,1,1,1,1,1,1,1,1,1,1,1,1,1,1,1,1,1,1,1,1,1,1,1,1,1,1,1,1,1,1,1,1,1,1,1,
1,1,1,1,1,1,1,1,1,1,1,6),(0.143172102,0.144954128,0.146788991,0.148623853,
0.150458716,0.152293578,0.15412844,0.155963303,0.157798165,0.159633028,
0.16146789,0.163302752,0.165137615,0.166972477,0.168807339,0.170642202,
0.172477064,0.174311927,0.176146789,0.177981651,0.179816514,0.181651376,
0.183486239,0.185321101,0.187155963,0.188990826,0.190825688,0.19266055,
0.194495413,0.196330275,0.198165138,0.2,0.201834862,0.203669725,0.205504587,
0.20733945,0.209174312,0.211009174,0.212844037,0.214678899,0.216513761,
0.218348624,0.220183486,0.222018349,0.223853211,0.225688073,0.227522936,
0.229357798,0.231192661,0.233027523,0.234862385,0.236697248,0.23853211,
0.240366972,0.242201835,0.244036697,0.24587156,0.247706422,0.249541284,
0.251376147,0.253211009,0.255045872,0.256880734,0.258715596,0.260550459,
0.262385321,0.264220183,0.266055046,0.267889908,0.269724771,0.271559633,
0.273394495,0.275229358,0.27706422,0.278899083,0.280733945,0.282568807,
0.28440367,0.286238532,0.288073394,0.289908257,0.291743119,0.293577982,
0.295412844,0.297247706,0.299082569,0.300917431,0.302752294,0.304587156,
0.306422018,0.308256881,0.310091743,0.311926606,0.313761468,0.31559633,
0.317431193,0.319266055,0.321100917,0.32293578,0.324770642,0.326605505,
0.328440367,0.330275229,0.332110092,0.333944954,0.335779817,0.337614679,
0.339449541,0.341284404,0.343119266,0.344954128,0.346788991,0.348623853,
0.350458716,0.352293578,0.35412844,0.355963303,0.357798165,0.359633028,
0.36146789,0.363302752,0.365137615,0.366972477,0.368807339,0.370642202,
0.372477064,0.374311927,0.376146789,0.377981651,0.379816514,0.381651376,
0.383486239,0.385321101,0.387155963,0.388990826,0.390825688,0.39266055,
0.394495413,0.396330275,0.398165138,0.4,0.401834862,0.403669725,0.405504587,
0.40733945,0.409174312,0.411009174,0.412844037,0.414678899,0.416513761,
0.418348624,0.420183486,0.422018349,0.423853211,0.425688073,0.427522936,
0.429357798,0.431192661,0.433027523,0.434862385,0.436697248,0.43853211,
0.440366972,0.442201835,0.444036697,0.44587156,0.447706422,0.449541284,
0.451376147,0.453211009,0.455045872,0.456880734,0.458715596,0.460550459,
0.462385321,0.464220183,0.466055046,0.467889908,0.469724771,0.471559633,
0.473394495,0.475229358,0.47706422,0.478899083,0.480733945,0.482568807,
0.48440367,0.486238532,0.488073394,0.489908257,0.491743119,0.493577982,
0.495412844,0.497247706,0.499082569,0.500917431,0.502752294,0.504587156,
0.506422018,0.508256881,0.510091743,0.511926606,0.513761468,0.51559633,
0.517431193,0.519266055,0.521100917,0.52293578,0.524770642,0.526605505,
0.528440367,0.530275229,0.532110092,0.533944954,0.535779817,0.537614679,
0.539449541,0.541284404,0.543119266,0.544954128,0.546788991,0.548623853,
0.550458716,0.552293578,0.55412844,0.555963303,0.557798165,0.559633028,
0.56146789,0.563302752,0.565137615,0.566972477,0.568807339,0.570642202,
0.572477064,0.574311927,0.576146789,0.577981651,0.579816514,0.581651376,
0.583486239,0.585321101,0.587155963,0.588990826,0.590825688,0.59266055,
0.594495413,0.596330275,0.598165138,0.6,0.601834862,0.603669725,0.605504587,
0.60733945,0.609174312,0.611009174,0.612844037,0.614678899,0.616513761,
0.618348624,0.620183486,0.622018349,0.623853211,0.625688073,0.627522936,
0.629357798,0.631192661,0.633027523,0.634862385,0.636697248,0.63853211,
0.640366972,0.642201835,0.644036697,0.64587156,0.647706422,0.649541284,
0.651376147,0.653211009,0.655045872,0.656880734,0.658715596,0.660550459,
0.662385321,0.664220183,0.666055046,0.667889908,0.669724771,0.671559633,
0.673394495,0.675229358,0.67706422,0.678899083,0.680733945,0.682568807,
0.68440367,0.686238532,0.688073394,0.689908257,0.691743119,0.693577982,
0.695412844,0.697247706,0.699082569,0.700917431,0.702752294,0.704587156,
0.706422018,0.708256881,0.710091743,0.711926606,0.713761468,0.71559633,
0.717431193,0.719266055,0.721100917,0.72293578,0.724770642,0.726605505,
0.728440367,0.730275229,0.732110092,0.733944954,0.735779817,0.737614679,
0.739449541,0.741284404,0.743119266,0.744954128,0.746788991,0.748623853,
0.750458716,0.752293578,0.75412844,0.755963303,0.757798165,0.759633028,
0.76146789,0.763302752,0.765137615,0.766972477,0.768807339,0.770642202,
0.772477064,0.774311927,0.776146789,0.777981651,0.779816514,0.781651376,
0.783486239,0.785321101,0.787155963,0.788990826,0.790825688,0.79266055,
0.794495413,0.796330275,0.798165138,0.8,0.801834862,0.803669725,0.805504587,
0.80733945,0.809174312,0.811009174,0.812844037,0.814678899,0.816513761,
0.818348624,0.820183486,0.822018349,0.823853211,0.825688073,0.827522936,
0.829357798,0.831192661,0.833027523,0.834862385,0.836697248,0.83853211,
0.840366972,0.842201835,0.844036697,0.84587156,0.847706422,0.849541284,
0.851376147,0.853211009,0.855045872,0.856880734,0.858715596,0.860550459,
0.862385321,0.864220183,0.866055046,0.867889908,0.869724771,0.871559633,
0.873394495,0.875229358,0.87706422,0.878899083,0.880733945,0.882568807,
0.88440367,0.886238532,0.888073394,0.889908257,0.891743119,0.893577982,
0.895412844,0.897247706,0.899082569,0.900917431,0.902752294,0.904587156,
0.906422018,0.908256881,0.910091743,0.911926606,0.913761468,0.91559633,
0.917431193,0.919266055,0.921100917,0.92293578,0.924770642,0.926605505,
0.928440367,0.930275229,0.932110092,0.933944954,0.935779817,0.937614679,
0.939449541,0.941284404,0.943119266,0.944954128,0.946788991,0.948623853,
0.950458716,0.952293578,0.95412844,0.955963303,0.957798165,0.959633028,
0.96146789,0.963302752,0.965137615,0.966972477,0.968807339,0.970642202,
0.972477064,0.974311927,0.976146789,0.977981651,0.979816514,0.981651376,
0.983486239,0.985321101,0.987155963,0.988990826,0.990825688,0.99266055,
0.994495413,0.996330275,0.998165138,1.),.UNSPECIFIED.);
#24479=B_SPLINE_CURVE_WITH_KNOTS('',5,(#287489,#287490,#287491,#287492,
#287493,#287494,#287495,#287496,#287497,#287498,#287499,#287500,#287501,
#287502,#287503,#287504,#287505,#287506,#287507,#287508,#287509,#287510,
#287511,#287512,#287513,#287514,#287515,#287516,#287517,#287518,#287519,
#287520,#287521,#287522,#287523,#287524,#287525,#287526,#287527,#287528,
#287529,#287530,#287531,#287532,#287533,#287534,#287535,#287536,#287537,
#287538,#287539,#287540,#287541,#287542,#287543,#287544,#287545,#287546,
#287547,#287548,#287549,#287550,#287551,#287552,#287553,#287554,#287555,
#287556,#287557,#287558,#287559,#287560,#287561,#287562,#287563,#287564,
#287565,#287566,#287567,#287568,#287569,#287570,#287571,#287572,#287573,
#287574,#287575,#287576,#287577,#287578,#287579,#287580,#287581,#287582,
#287583,#287584,#287585,#287586,#287587,#287588,#287589,#287590,#287591,
#287592,#287593,#287594,#287595,#287596,#287597,#287598,#287599,#287600,
#287601,#287602,#287603,#287604,#287605,#287606,#287607,#287608,#287609,
#287610,#287611,#287612,#287613,#287614,#287615,#287616,#287617,#287618,
#287619,#287620,#287621,#287622,#287623,#287624,#287625,#287626,#287627,
#287628,#287629,#287630,#287631,#287632,#287633,#287634,#287635,#287636,
#287637,#287638,#287639,#287640,#287641,#287642,#287643,#287644,#287645,
#287646,#287647,#287648,#287649,#287650,#287651,#287652,#287653,#287654,
#287655,#287656,#287657,#287658,#287659,#287660,#287661,#287662,#287663,
#287664,#287665,#287666,#287667,#287668,#287669,#287670,#287671,#287672,
#287673,#287674,#287675,#287676,#287677,#287678,#287679,#287680,#287681,
#287682,#287683,#287684,#287685,#287686,#287687,#287688,#287689,#287690,
#287691,#287692,#287693,#287694,#287695,#287696,#287697,#287698,#287699,
#287700,#287701,#287702,#287703,#287704,#287705,#287706,#287707,#287708,
#287709,#287710,#287711,#287712,#287713,#287714,#287715,#287716,#287717,
#287718,#287719,#287720,#287721,#287722,#287723,#287724,#287725,#287726,
#287727,#287728,#287729,#287730,#287731,#287732,#287733,#287734,#287735,
#287736,#287737,#287738,#287739,#287740,#287741,#287742,#287743,#287744,
#287745,#287746,#287747,#287748,#287749,#287750,#287751,#287752,#287753,
#287754,#287755,#287756,#287757,#287758,#287759,#287760,#287761,#287762,
#287763,#287764,#287765,#287766,#287767,#287768,#287769,#287770,#287771,
#287772,#287773,#287774,#287775,#287776,#287777,#287778,#287779,#287780,
#287781,#287782,#287783,#287784,#287785,#287786,#287787,#287788,#287789,
#287790,#287791,#287792,#287793,#287794,#287795,#287796,#287797,#287798,
#287799,#287800,#287801,#287802,#287803,#287804,#287805,#287806,#287807,
#287808,#287809,#287810,#287811,#287812,#287813,#287814,#287815,#287816,
#287817,#287818,#287819,#287820,#287821,#287822,#287823,#287824,#287825,
#287826,#287827,#287828,#287829,#287830,#287831,#287832,#287833,#287834,
#287835,#287836,#287837,#287838,#287839,#287840,#287841,#287842,#287843,
#287844,#287845,#287846,#287847,#287848,#287849,#287850,#287851,#287852,
#287853,#287854,#287855,#287856,#287857,#287858,#287859,#287860,#287861,
#287862,#287863,#287864,#287865,#287866,#287867,#287868,#287869,#287870,
#287871,#287872,#287873,#287874,#287875,#287876,#287877,#287878,#287879,
#287880,#287881,#287882,#287883,#287884,#287885,#287886,#287887,#287888,
#287889,#287890,#287891,#287892,#287893,#287894,#287895,#287896,#287897,
#287898,#287899,#287900,#287901,#287902,#287903,#287904,#287905,#287906,
#287907,#287908,#287909,#287910,#287911,#287912,#287913,#287914,#287915,
#287916,#287917,#287918,#287919,#287920,#287921,#287922,#287923,#287924,
#287925,#287926,#287927,#287928,#287929,#287930,#287931,#287932,#287933,
#287934,#287935,#287936,#287937,#287938,#287939,#287940,#287941,#287942,
#287943,#287944,#287945,#287946,#287947,#287948,#287949,#287950,#287951,
#287952,#287953,#287954,#287955,#287956,#287957,#287958,#287959),
 .UNSPECIFIED.,.F.,.F.,(6,1,1,1,1,1,1,1,1,1,1,1,1,1,1,1,1,1,1,1,1,1,1,1,
1,1,1,1,1,1,1,1,1,1,1,1,1,1,1,1,1,1,1,1,1,1,1,1,1,1,1,1,1,1,1,1,1,1,1,1,
1,1,1,1,1,1,1,1,1,1,1,1,1,1,1,1,1,1,1,1,1,1,1,1,1,1,1,1,1,1,1,1,1,1,1,1,
1,1,1,1,1,1,1,1,1,1,1,1,1,1,1,1,1,1,1,1,1,1,1,1,1,1,1,1,1,1,1,1,1,1,1,1,
1,1,1,1,1,1,1,1,1,1,1,1,1,1,1,1,1,1,1,1,1,1,1,1,1,1,1,1,1,1,1,1,1,1,1,1,
1,1,1,1,1,1,1,1,1,1,1,1,1,1,1,1,1,1,1,1,1,1,1,1,1,1,1,1,1,1,1,1,1,1,1,1,
1,1,1,1,1,1,1,1,1,1,1,1,1,1,1,1,1,1,1,1,1,1,1,1,1,1,1,1,1,1,1,1,1,1,1,1,
1,1,1,1,1,1,1,1,1,1,1,1,1,1,1,1,1,1,1,1,1,1,1,1,1,1,1,1,1,1,1,1,1,1,1,1,
1,1,1,1,1,1,1,1,1,1,1,1,1,1,1,1,1,1,1,1,1,1,1,1,1,1,1,1,1,1,1,1,1,1,1,1,
1,1,1,1,1,1,1,1,1,1,1,1,1,1,1,1,1,1,1,1,1,1,1,1,1,1,1,1,1,1,1,1,1,1,1,1,
1,1,1,1,1,1,1,1,1,1,1,1,1,1,1,1,1,1,1,1,1,1,1,1,1,1,1,1,1,1,1,1,1,1,1,1,
1,1,1,1,1,1,1,1,1,1,1,1,1,1,1,1,1,1,1,1,1,1,1,1,1,1,1,1,1,1,1,1,1,1,1,1,
1,1,1,1,1,1,1,1,1,1,1,1,1,1,1,1,1,1,1,1,1,1,1,1,1,1,1,1,1,1,1,1,1,1,1,1,
1,1,1,1,1,1,1,1,1,1,6),(0.143172102,0.144954128,0.146788991,0.148623853,
0.150458716,0.152293578,0.15412844,0.155963303,0.157798165,0.159633028,
0.16146789,0.163302752,0.165137615,0.166972477,0.168807339,0.170642202,
0.172477064,0.174311927,0.176146789,0.177981651,0.179816514,0.181651376,
0.183486239,0.185321101,0.187155963,0.188990826,0.190825688,0.19266055,
0.194495413,0.196330275,0.198165138,0.2,0.201834862,0.203669725,0.205504587,
0.20733945,0.209174312,0.211009174,0.212844037,0.214678899,0.216513761,
0.218348624,0.220183486,0.222018349,0.223853211,0.225688073,0.227522936,
0.229357798,0.231192661,0.233027523,0.234862385,0.236697248,0.23853211,
0.240366972,0.242201835,0.244036697,0.24587156,0.247706422,0.249541284,
0.251376147,0.253211009,0.255045872,0.256880734,0.258715596,0.260550459,
0.262385321,0.264220183,0.266055046,0.267889908,0.269724771,0.271559633,
0.273394495,0.275229358,0.27706422,0.278899083,0.280733945,0.282568807,
0.28440367,0.286238532,0.288073394,0.289908257,0.291743119,0.293577982,
0.295412844,0.297247706,0.299082569,0.300917431,0.302752294,0.304587156,
0.306422018,0.308256881,0.310091743,0.311926606,0.313761468,0.31559633,
0.317431193,0.319266055,0.321100917,0.32293578,0.324770642,0.326605505,
0.328440367,0.330275229,0.332110092,0.333944954,0.335779817,0.337614679,
0.339449541,0.341284404,0.343119266,0.344954128,0.346788991,0.348623853,
0.350458716,0.352293578,0.35412844,0.355963303,0.357798165,0.359633028,
0.36146789,0.363302752,0.365137615,0.366972477,0.368807339,0.370642202,
0.372477064,0.374311927,0.376146789,0.377981651,0.379816514,0.381651376,
0.383486239,0.385321101,0.387155963,0.388990826,0.390825688,0.39266055,
0.394495413,0.396330275,0.398165138,0.4,0.401834862,0.403669725,0.405504587,
0.40733945,0.409174312,0.411009174,0.412844037,0.414678899,0.416513761,
0.418348624,0.420183486,0.422018349,0.423853211,0.425688073,0.427522936,
0.429357798,0.431192661,0.433027523,0.434862385,0.436697248,0.43853211,
0.440366972,0.442201835,0.444036697,0.44587156,0.447706422,0.449541284,
0.451376147,0.453211009,0.455045872,0.456880734,0.458715596,0.460550459,
0.462385321,0.464220183,0.466055046,0.467889908,0.469724771,0.471559633,
0.473394495,0.475229358,0.47706422,0.478899083,0.480733945,0.482568807,
0.48440367,0.486238532,0.488073394,0.489908257,0.491743119,0.493577982,
0.495412844,0.497247706,0.499082569,0.500917431,0.502752294,0.504587156,
0.506422018,0.508256881,0.510091743,0.511926606,0.513761468,0.51559633,
0.517431193,0.519266055,0.521100917,0.52293578,0.524770642,0.526605505,
0.528440367,0.530275229,0.532110092,0.533944954,0.535779817,0.537614679,
0.539449541,0.541284404,0.543119266,0.544954128,0.546788991,0.548623853,
0.550458716,0.552293578,0.55412844,0.555963303,0.557798165,0.559633028,
0.56146789,0.563302752,0.565137615,0.566972477,0.568807339,0.570642202,
0.572477064,0.574311927,0.576146789,0.577981651,0.579816514,0.581651376,
0.583486239,0.585321101,0.587155963,0.588990826,0.590825688,0.59266055,
0.594495413,0.596330275,0.598165138,0.6,0.601834862,0.603669725,0.605504587,
0.60733945,0.609174312,0.611009174,0.612844037,0.614678899,0.616513761,
0.618348624,0.620183486,0.622018349,0.623853211,0.625688073,0.627522936,
0.629357798,0.631192661,0.633027523,0.634862385,0.636697248,0.63853211,
0.640366972,0.642201835,0.644036697,0.64587156,0.647706422,0.649541284,
0.651376147,0.653211009,0.655045872,0.656880734,0.658715596,0.660550459,
0.662385321,0.664220183,0.666055046,0.667889908,0.669724771,0.673394495,
0.675229358,0.67706422,0.678899083,0.680733945,0.682568807,0.68440367,0.686238532,
0.688073394,0.689908257,0.691743119,0.693577982,0.695412844,0.697247706,
0.699082569,0.700917431,0.702752294,0.704587156,0.706422018,0.708256881,
0.710091743,0.711926606,0.713761468,0.71559633,0.717431193,0.719266055,
0.721100917,0.72293578,0.724770642,0.726605505,0.728440367,0.730275229,
0.732110092,0.733944954,0.735779817,0.737614679,0.739449541,0.741284404,
0.743119266,0.744954128,0.746788991,0.748623853,0.750458716,0.752293578,
0.75412844,0.755963303,0.757798165,0.759633028,0.76146789,0.763302752,0.765137615,
0.766972477,0.768807339,0.770642202,0.772477064,0.774311927,0.776146789,
0.777981651,0.779816514,0.781651376,0.783486239,0.785321101,0.787155963,
0.788990826,0.790825688,0.79266055,0.794495413,0.796330275,0.798165138,
0.8,0.801834862,0.803669725,0.805504587,0.80733945,0.809174312,0.811009174,
0.812844037,0.814678899,0.816513761,0.818348624,0.820183486,0.822018349,
0.823853211,0.825688073,0.827522936,0.829357798,0.831192661,0.833027523,
0.834862385,0.836697248,0.83853211,0.840366972,0.842201835,0.844036697,
0.84587156,0.847706422,0.849541284,0.851376147,0.853211009,0.855045872,
0.856880734,0.858715596,0.860550459,0.862385321,0.864220183,0.866055046,
0.867889908,0.869724771,0.871559633,0.873394495,0.875229358,0.87706422,
0.878899083,0.880733945,0.882568807,0.88440367,0.886238532,0.888073394,
0.889908257,0.891743119,0.893577982,0.895412844,0.897247706,0.899082569,
0.900917431,0.902752294,0.904587156,0.906422018,0.908256881,0.910091743,
0.911926606,0.913761468,0.91559633,0.917431193,0.919266055,0.921100917,
0.92293578,0.924770642,0.926605505,0.928440367,0.930275229,0.932110092,
0.933944954,0.935779817,0.937614679,0.939449541,0.941284404,0.943119266,
0.944954128,0.946788991,0.948623853,0.950458716,0.952293578,0.95412844,
0.955963303,0.957798165,0.959633028,0.96146789,0.963302752,0.965137615,
0.966972477,0.968807339,0.970642202,0.972477064,0.974311927,0.976146789,
0.977981651,0.979816514,0.981651376,0.983486239,0.985321101,0.987155963,
0.988990826,0.990825688,0.99266055,0.994495413,0.996330275,0.998165138,
1.),.UNSPECIFIED.);
#24480=B_SPLINE_CURVE_WITH_KNOTS('',5,(#287960,#287961,#287962,#287963,
#287964,#287965,#287966,#287967,#287968,#287969,#287970,#287971,#287972,
#287973,#287974,#287975,#287976,#287977,#287978,#287979,#287980,#287981,
#287982,#287983,#287984,#287985,#287986,#287987,#287988,#287989,#287990,
#287991,#287992,#287993,#287994,#287995,#287996,#287997,#287998,#287999,
#288000,#288001,#288002,#288003,#288004,#288005,#288006,#288007,#288008,
#288009,#288010,#288011,#288012,#288013,#288014,#288015,#288016,#288017,
#288018,#288019,#288020,#288021,#288022,#288023,#288024,#288025,#288026,
#288027,#288028,#288029,#288030,#288031,#288032,#288033,#288034,#288035,
#288036,#288037,#288038,#288039,#288040,#288041,#288042,#288043,#288044,
#288045,#288046,#288047,#288048,#288049,#288050,#288051,#288052,#288053,
#288054,#288055,#288056,#288057,#288058,#288059,#288060,#288061,#288062,
#288063,#288064,#288065,#288066,#288067,#288068,#288069,#288070,#288071,
#288072,#288073,#288074,#288075,#288076,#288077,#288078,#288079,#288080,
#288081,#288082,#288083,#288084,#288085,#288086,#288087,#288088,#288089,
#288090,#288091,#288092,#288093,#288094,#288095,#288096,#288097,#288098,
#288099,#288100,#288101,#288102,#288103,#288104,#288105,#288106,#288107,
#288108,#288109,#288110,#288111,#288112,#288113,#288114,#288115,#288116,
#288117,#288118,#288119,#288120,#288121,#288122,#288123,#288124,#288125,
#288126,#288127,#288128,#288129,#288130,#288131,#288132,#288133,#288134,
#288135,#288136,#288137,#288138,#288139,#288140,#288141,#288142,#288143,
#288144,#288145,#288146,#288147,#288148,#288149,#288150,#288151,#288152,
#288153,#288154,#288155,#288156,#288157,#288158,#288159,#288160,#288161,
#288162,#288163,#288164,#288165,#288166,#288167,#288168,#288169,#288170,
#288171,#288172,#288173,#288174,#288175,#288176,#288177,#288178,#288179,
#288180,#288181,#288182,#288183,#288184,#288185,#288186,#288187,#288188,
#288189,#288190,#288191,#288192,#288193,#288194,#288195,#288196,#288197,
#288198,#288199,#288200,#288201,#288202,#288203,#288204,#288205,#288206,
#288207,#288208,#288209,#288210,#288211,#288212,#288213,#288214,#288215,
#288216,#288217,#288218,#288219,#288220,#288221,#288222,#288223,#288224,
#288225,#288226,#288227,#288228,#288229,#288230,#288231,#288232,#288233,
#288234,#288235,#288236,#288237,#288238,#288239,#288240,#288241,#288242,
#288243,#288244,#288245,#288246,#288247,#288248,#288249,#288250,#288251,
#288252,#288253,#288254,#288255,#288256,#288257,#288258,#288259,#288260,
#288261,#288262,#288263,#288264,#288265,#288266,#288267,#288268,#288269,
#288270,#288271,#288272,#288273,#288274,#288275,#288276,#288277,#288278,
#288279,#288280,#288281,#288282,#288283,#288284,#288285,#288286,#288287,
#288288,#288289,#288290,#288291,#288292,#288293,#288294,#288295,#288296,
#288297,#288298,#288299,#288300,#288301,#288302,#288303,#288304,#288305,
#288306,#288307,#288308,#288309,#288310,#288311,#288312,#288313,#288314,
#288315,#288316,#288317,#288318,#288319,#288320,#288321,#288322,#288323,
#288324,#288325,#288326,#288327,#288328,#288329,#288330,#288331,#288332,
#288333,#288334,#288335,#288336,#288337,#288338,#288339,#288340,#288341,
#288342,#288343,#288344,#288345,#288346,#288347,#288348,#288349,#288350,
#288351,#288352,#288353,#288354,#288355,#288356,#288357,#288358,#288359,
#288360,#288361,#288362,#288363,#288364,#288365,#288366,#288367,#288368,
#288369,#288370,#288371,#288372,#288373,#288374,#288375,#288376,#288377,
#288378,#288379,#288380,#288381,#288382,#288383,#288384,#288385,#288386,
#288387,#288388,#288389,#288390,#288391,#288392,#288393,#288394,#288395,
#288396,#288397,#288398,#288399,#288400,#288401,#288402,#288403,#288404,
#288405,#288406,#288407,#288408,#288409,#288410,#288411,#288412,#288413,
#288414,#288415,#288416,#288417,#288418,#288419,#288420,#288421,#288422,
#288423,#288424,#288425,#288426,#288427,#288428,#288429,#288430),
 .UNSPECIFIED.,.F.,.F.,(6,1,1,1,1,1,1,1,1,1,1,1,1,1,1,1,1,1,1,1,1,1,1,1,
1,1,1,1,1,1,1,1,1,1,1,1,1,1,1,1,1,1,1,1,1,1,1,1,1,1,1,1,1,1,1,1,1,1,1,1,
1,1,1,1,1,1,1,1,1,1,1,1,1,1,1,1,1,1,1,1,1,1,1,1,1,1,1,1,1,1,1,1,1,1,1,1,
1,1,1,1,1,1,1,1,1,1,1,1,1,1,1,1,1,1,1,1,1,1,1,1,1,1,1,1,1,1,1,1,1,1,1,1,
1,1,1,1,1,1,1,1,1,1,1,1,1,1,1,1,1,1,1,1,1,1,1,1,1,1,1,1,1,1,1,1,1,1,1,1,
1,1,1,1,1,1,1,1,1,1,1,1,1,1,1,1,1,1,1,1,1,1,1,1,1,1,1,1,1,1,1,1,1,1,1,1,
1,1,1,1,1,1,1,1,1,1,1,1,1,1,1,1,1,1,1,1,1,1,1,1,1,1,1,1,1,1,1,1,1,1,1,1,
1,1,1,1,1,1,1,1,1,1,1,1,1,1,1,1,1,1,1,1,1,1,1,1,1,1,1,1,1,1,1,1,1,1,1,1,
1,1,1,1,1,1,1,1,1,1,1,1,1,1,1,1,1,1,1,1,1,1,1,1,1,1,1,1,1,1,1,1,1,1,1,1,
1,1,1,1,1,1,1,1,1,1,1,1,1,1,1,1,1,1,1,1,1,1,1,1,1,1,1,1,1,1,1,1,1,1,1,1,
1,1,1,1,1,1,1,1,1,1,1,1,1,1,1,1,1,1,1,1,1,1,1,1,1,1,1,1,1,1,1,1,1,1,1,1,
1,1,1,1,1,1,1,1,1,1,1,1,1,1,1,1,1,1,1,1,1,1,1,1,1,1,1,1,1,1,1,1,1,1,1,1,
1,1,1,1,1,1,1,1,1,1,1,1,1,1,1,1,1,1,1,1,1,1,1,1,1,1,1,1,1,1,1,1,1,1,1,1,
1,1,1,1,1,1,1,1,1,1,6),(0.143172102,0.144954128,0.146788991,0.148623853,
0.150458716,0.152293578,0.15412844,0.155963303,0.157798165,0.159633028,
0.16146789,0.163302752,0.165137615,0.166972477,0.168807339,0.170642202,
0.172477064,0.174311927,0.176146789,0.177981651,0.179816514,0.181651376,
0.183486239,0.185321101,0.187155963,0.188990826,0.190825688,0.19266055,
0.194495413,0.196330275,0.198165138,0.2,0.201834862,0.203669725,0.205504587,
0.20733945,0.209174312,0.211009174,0.212844037,0.214678899,0.216513761,
0.218348624,0.220183486,0.222018349,0.223853211,0.225688073,0.227522936,
0.229357798,0.231192661,0.233027523,0.234862385,0.236697248,0.23853211,
0.240366972,0.242201835,0.244036697,0.24587156,0.247706422,0.249541284,
0.251376147,0.253211009,0.255045872,0.256880734,0.258715596,0.260550459,
0.262385321,0.264220183,0.266055046,0.267889908,0.269724771,0.271559633,
0.273394495,0.275229358,0.27706422,0.278899083,0.280733945,0.282568807,
0.28440367,0.286238532,0.288073394,0.289908257,0.291743119,0.293577982,
0.295412844,0.297247706,0.299082569,0.300917431,0.302752294,0.304587156,
0.306422018,0.308256881,0.310091743,0.311926606,0.313761468,0.31559633,
0.317431193,0.319266055,0.321100917,0.32293578,0.324770642,0.326605505,
0.328440367,0.330275229,0.332110092,0.333944954,0.335779817,0.337614679,
0.339449541,0.341284404,0.343119266,0.344954128,0.346788991,0.348623853,
0.350458716,0.352293578,0.35412844,0.355963303,0.357798165,0.359633028,
0.36146789,0.363302752,0.365137615,0.366972477,0.368807339,0.370642202,
0.372477064,0.374311927,0.376146789,0.377981651,0.379816514,0.381651376,
0.383486239,0.385321101,0.387155963,0.388990826,0.390825688,0.39266055,
0.394495413,0.396330275,0.398165138,0.4,0.401834862,0.403669725,0.405504587,
0.40733945,0.409174312,0.411009174,0.412844037,0.414678899,0.416513761,
0.418348624,0.420183486,0.422018349,0.423853211,0.425688073,0.427522936,
0.429357798,0.431192661,0.433027523,0.434862385,0.436697248,0.43853211,
0.440366972,0.442201835,0.444036697,0.44587156,0.447706422,0.449541284,
0.451376147,0.453211009,0.455045872,0.456880734,0.458715596,0.460550459,
0.462385321,0.464220183,0.466055046,0.467889908,0.469724771,0.471559633,
0.473394495,0.475229358,0.47706422,0.478899083,0.480733945,0.482568807,
0.48440367,0.486238532,0.488073394,0.489908257,0.491743119,0.493577982,
0.495412844,0.497247706,0.499082569,0.500917431,0.502752294,0.504587156,
0.506422018,0.508256881,0.510091743,0.511926606,0.513761468,0.51559633,
0.517431193,0.519266055,0.521100917,0.52293578,0.524770642,0.526605505,
0.528440367,0.530275229,0.532110092,0.533944954,0.535779817,0.537614679,
0.539449541,0.541284404,0.543119266,0.544954128,0.546788991,0.548623853,
0.550458716,0.552293578,0.55412844,0.555963303,0.557798165,0.559633028,
0.56146789,0.563302752,0.565137615,0.566972477,0.568807339,0.570642202,
0.572477064,0.574311927,0.576146789,0.577981651,0.579816514,0.581651376,
0.583486239,0.585321101,0.587155963,0.588990826,0.590825688,0.59266055,
0.594495413,0.596330275,0.598165138,0.6,0.601834862,0.603669725,0.605504587,
0.60733945,0.609174312,0.611009174,0.612844037,0.614678899,0.616513761,
0.618348624,0.620183486,0.622018349,0.623853211,0.625688073,0.627522936,
0.629357798,0.631192661,0.633027523,0.634862385,0.636697248,0.63853211,
0.640366972,0.642201835,0.644036697,0.64587156,0.647706422,0.649541284,
0.651376147,0.653211009,0.655045872,0.656880734,0.658715596,0.660550459,
0.662385321,0.664220183,0.666055046,0.667889908,0.669724771,0.673394495,
0.675229358,0.67706422,0.678899083,0.680733945,0.682568807,0.68440367,0.686238532,
0.688073394,0.689908257,0.691743119,0.693577982,0.695412844,0.697247706,
0.699082569,0.700917431,0.702752294,0.704587156,0.706422018,0.708256881,
0.710091743,0.711926606,0.713761468,0.71559633,0.717431193,0.719266055,
0.721100917,0.72293578,0.724770642,0.726605505,0.728440367,0.730275229,
0.732110092,0.733944954,0.735779817,0.737614679,0.739449541,0.741284404,
0.743119266,0.744954128,0.746788991,0.748623853,0.750458716,0.752293578,
0.75412844,0.755963303,0.757798165,0.759633028,0.76146789,0.763302752,0.765137615,
0.766972477,0.768807339,0.770642202,0.772477064,0.774311927,0.776146789,
0.777981651,0.779816514,0.781651376,0.783486239,0.785321101,0.787155963,
0.788990826,0.790825688,0.79266055,0.794495413,0.796330275,0.798165138,
0.8,0.801834862,0.803669725,0.805504587,0.80733945,0.809174312,0.811009174,
0.812844037,0.814678899,0.816513761,0.818348624,0.820183486,0.822018349,
0.823853211,0.825688073,0.827522936,0.829357798,0.831192661,0.833027523,
0.834862385,0.836697248,0.83853211,0.840366972,0.842201835,0.844036697,
0.84587156,0.847706422,0.849541284,0.851376147,0.853211009,0.855045872,
0.856880734,0.858715596,0.860550459,0.862385321,0.864220183,0.866055046,
0.867889908,0.869724771,0.871559633,0.873394495,0.875229358,0.87706422,
0.878899083,0.880733945,0.882568807,0.88440367,0.886238532,0.888073394,
0.889908257,0.891743119,0.893577982,0.895412844,0.897247706,0.899082569,
0.900917431,0.902752294,0.904587156,0.906422018,0.908256881,0.910091743,
0.911926606,0.913761468,0.91559633,0.917431193,0.919266055,0.921100917,
0.92293578,0.924770642,0.926605505,0.928440367,0.930275229,0.932110092,
0.933944954,0.935779817,0.937614679,0.939449541,0.941284404,0.943119266,
0.944954128,0.946788991,0.948623853,0.950458716,0.952293578,0.95412844,
0.955963303,0.957798165,0.959633028,0.96146789,0.963302752,0.965137615,
0.966972477,0.968807339,0.970642202,0.972477064,0.974311927,0.976146789,
0.977981651,0.979816514,0.981651376,0.983486239,0.985321101,0.987155963,
0.988990826,0.990825688,0.99266055,0.994495413,0.996330275,0.998165138,
1.),.UNSPECIFIED.);
#24481=B_SPLINE_CURVE_WITH_KNOTS('',3,(#289378,#289379,#289380,#289381,
#289382,#289383,#289384,#289385,#289386,#289387,#289388,#289389,#289390,
#289391,#289392,#289393,#289394,#289395,#289396,#289397,#289398,#289399,
#289400,#289401,#289402,#289403,#289404,#289405,#289406,#289407,#289408,
#289409,#289410,#289411,#289412,#289413,#289414,#289415,#289416,#289417,
#289418,#289419,#289420,#289421,#289422,#289423,#289424,#289425,#289426,
#289427,#289428,#289429,#289430,#289431,#289432,#289433,#289434,#289435,
#289436,#289437,#289438,#289439,#289440,#289441,#289442,#289443,#289444,
#289445,#289446,#289447,#289448,#289449,#289450,#289451,#289452,#289453,
#289454,#289455,#289456,#289457,#289458,#289459,#289460,#289461,#289462,
#289463,#289464,#289465,#289466,#289467,#289468,#289469,#289470,#289471,
#289472,#289473,#289474,#289475,#289476,#289477,#289478,#289479,#289480,
#289481,#289482,#289483,#289484,#289485,#289486,#289487,#289488,#289489,
#289490,#289491,#289492,#289493,#289494,#289495,#289496,#289497,#289498,
#289499,#289500,#289501,#289502,#289503,#289504,#289505,#289506,#289507,
#289508,#289509,#289510,#289511,#289512,#289513,#289514,#289515,#289516,
#289517,#289518,#289519,#289520,#289521,#289522,#289523,#289524,#289525,
#289526,#289527,#289528,#289529,#289530,#289531,#289532,#289533,#289534,
#289535,#289536,#289537,#289538,#289539,#289540,#289541,#289542,#289543,
#289544,#289545,#289546,#289547,#289548,#289549,#289550,#289551,#289552,
#289553,#289554,#289555,#289556,#289557,#289558,#289559,#289560,#289561,
#289562,#289563,#289564,#289565,#289566,#289567,#289568,#289569,#289570,
#289571,#289572,#289573,#289574,#289575,#289576,#289577,#289578,#289579,
#289580,#289581,#289582,#289583,#289584,#289585,#289586,#289587,#289588,
#289589,#289590,#289591,#289592,#289593,#289594,#289595,#289596,#289597,
#289598,#289599,#289600,#289601,#289602,#289603,#289604,#289605,#289606,
#289607,#289608,#289609,#289610,#289611,#289612,#289613,#289614,#289615,
#289616,#289617,#289618,#289619,#289620,#289621,#289622,#289623,#289624,
#289625,#289626,#289627,#289628,#289629,#289630,#289631,#289632,#289633,
#289634,#289635,#289636,#289637,#289638,#289639,#289640,#289641,#289642,
#289643,#289644,#289645,#289646,#289647,#289648,#289649,#289650,#289651,
#289652,#289653,#289654,#289655,#289656,#289657,#289658,#289659,#289660,
#289661,#289662,#289663,#289664,#289665,#289666,#289667,#289668,#289669,
#289670,#289671,#289672,#289673,#289674,#289675,#289676,#289677,#289678,
#289679,#289680,#289681,#289682,#289683,#289684,#289685,#289686,#289687,
#289688,#289689,#289690,#289691,#289692,#289693,#289694,#289695,#289696,
#289697,#289698,#289699,#289700,#289701,#289702),.UNSPECIFIED.,.F.,.F.,
(4,3,3,3,3,3,3,3,3,3,3,3,3,3,3,3,3,3,3,3,3,3,3,3,3,3,3,3,3,3,3,3,3,3,3,
3,3,3,3,3,3,3,3,3,3,3,3,3,3,3,3,3,3,3,3,3,3,3,3,3,3,3,3,3,3,3,3,3,3,3,3,
3,3,3,3,3,3,3,3,3,3,3,3,3,3,3,3,3,3,3,3,3,3,3,3,3,3,3,3,3,3,3,3,3,3,3,3,
3,4),(-1.,-0.994495413,-0.988990826,-0.983486239,-0.977981651,-0.972477064,
-0.966972477,-0.959633028,-0.95412844,-0.948623853,-0.943119266,-0.937614679,
-0.932110092,-0.926605505,-0.921100917,-0.913761468,-0.908256881,-0.902752294,
-0.897247706,-0.891743119,-0.886238532,-0.880733945,-0.875229358,-0.867889908,
-0.862385321,-0.856880734,-0.851376147,-0.84587156,-0.840366972,-0.834862385,
-0.829357798,-0.823853211,-0.818348624,-0.812844037,-0.80733945,-0.798165138,
-0.790825688,-0.783486239,-0.776146789,-0.768807339,-0.76146789,-0.75412844,
-0.746788991,-0.737614679,-0.730275229,-0.72293578,-0.71559633,-0.708256881,
-0.700917431,-0.693577982,-0.686238532,-0.678899083,-0.671559633,-0.664220183,
-0.656880734,-0.649541284,-0.642201835,-0.634862385,-0.627522936,-0.620183486,
-0.611009174,-0.603669725,-0.596330275,-0.588990826,-0.581651376,-0.574311927,
-0.566972477,-0.559633028,-0.552293578,-0.544954128,-0.537614679,-0.530275229,
-0.521100917,-0.511926606,-0.502752294,-0.493577982,-0.482568807,-0.473394495,
-0.464220183,-0.455045872,-0.44587156,-0.436697248,-0.427522936,-0.418348624,
-0.409174312,-0.4,-0.390825688,-0.379816514,-0.368807339,-0.357798165,-0.346788991,
-0.335779817,-0.324770642,-0.313761468,-0.302752294,-0.291743119,-0.280733945,
-0.269724771,-0.258715596,-0.247706422,-0.234862385,-0.223853211,-0.212844037,
-0.201834862,-0.190825688,-0.179816514,-0.168807339,-0.157798165,-0.143172102),
 .UNSPECIFIED.);
#24482=B_SPLINE_CURVE_WITH_KNOTS('',3,(#289703,#289704,#289705,#289706,
#289707,#289708,#289709,#289710,#289711,#289712,#289713,#289714,#289715,
#289716,#289717,#289718,#289719,#289720,#289721,#289722,#289723,#289724,
#289725,#289726,#289727,#289728,#289729,#289730,#289731,#289732,#289733,
#289734,#289735,#289736,#289737,#289738,#289739,#289740,#289741,#289742,
#289743,#289744,#289745,#289746,#289747,#289748,#289749,#289750,#289751,
#289752,#289753,#289754,#289755,#289756,#289757,#289758,#289759,#289760,
#289761,#289762,#289763,#289764,#289765,#289766,#289767,#289768,#289769,
#289770,#289771,#289772,#289773,#289774,#289775,#289776,#289777,#289778,
#289779,#289780,#289781,#289782,#289783,#289784,#289785,#289786,#289787,
#289788,#289789,#289790,#289791,#289792,#289793,#289794,#289795,#289796,
#289797,#289798,#289799,#289800,#289801,#289802,#289803,#289804,#289805,
#289806,#289807,#289808,#289809,#289810,#289811,#289812,#289813,#289814,
#289815,#289816,#289817,#289818,#289819,#289820,#289821,#289822,#289823,
#289824,#289825,#289826,#289827,#289828,#289829,#289830,#289831,#289832,
#289833,#289834,#289835,#289836,#289837,#289838,#289839,#289840,#289841,
#289842,#289843,#289844,#289845,#289846,#289847,#289848,#289849,#289850,
#289851,#289852,#289853,#289854,#289855,#289856,#289857,#289858,#289859,
#289860,#289861,#289862,#289863,#289864,#289865,#289866,#289867,#289868,
#289869,#289870,#289871,#289872,#289873,#289874,#289875,#289876,#289877,
#289878,#289879,#289880,#289881,#289882,#289883,#289884,#289885,#289886,
#289887,#289888,#289889,#289890,#289891,#289892,#289893,#289894,#289895,
#289896,#289897,#289898,#289899,#289900,#289901,#289902,#289903,#289904,
#289905,#289906,#289907,#289908,#289909,#289910,#289911,#289912,#289913,
#289914,#289915,#289916,#289917,#289918,#289919,#289920,#289921,#289922,
#289923,#289924,#289925,#289926,#289927,#289928,#289929,#289930,#289931,
#289932,#289933,#289934,#289935,#289936,#289937,#289938,#289939,#289940,
#289941,#289942,#289943,#289944,#289945,#289946,#289947,#289948,#289949,
#289950,#289951,#289952,#289953,#289954,#289955,#289956,#289957,#289958,
#289959,#289960,#289961,#289962,#289963,#289964,#289965,#289966,#289967,
#289968,#289969,#289970,#289971,#289972,#289973,#289974,#289975,#289976,
#289977,#289978,#289979,#289980,#289981,#289982,#289983,#289984,#289985,
#289986,#289987,#289988,#289989,#289990,#289991,#289992,#289993,#289994,
#289995,#289996,#289997,#289998,#289999,#290000,#290001,#290002,#290003,
#290004,#290005,#290006,#290007,#290008,#290009,#290010,#290011,#290012,
#290013,#290014,#290015,#290016,#290017,#290018,#290019,#290020,#290021,
#290022,#290023,#290024),.UNSPECIFIED.,.F.,.F.,(4,3,3,3,3,3,3,3,3,3,3,3,
3,3,3,3,3,3,3,3,3,3,3,3,3,3,3,3,3,3,3,3,3,3,3,3,3,3,3,3,3,3,3,3,3,3,3,3,
3,3,3,3,3,3,3,3,3,3,3,3,3,3,3,3,3,3,3,3,3,3,3,3,3,3,3,3,3,3,3,3,3,3,3,3,
3,3,3,3,3,3,3,3,3,3,3,3,3,3,3,3,3,3,3,3,3,3,3,4),(0.143172102,0.15412844,
0.165137615,0.176146789,0.187155963,0.198165138,0.209174312,0.220183486,
0.231192661,0.242201835,0.253211009,0.264220183,0.275229358,0.286238532,
0.297247706,0.308256881,0.319266055,0.330275229,0.341284404,0.352293578,
0.363302752,0.374311927,0.385321101,0.396330275,0.405504587,0.414678899,
0.423853211,0.433027523,0.442201835,0.451376147,0.460550459,0.471559633,
0.480733945,0.491743119,0.500917431,0.510091743,0.519266055,0.528440367,
0.535779817,0.543119266,0.550458716,0.557798165,0.565137615,0.572477064,
0.579816514,0.587155963,0.594495413,0.601834862,0.609174312,0.616513761,
0.623853211,0.631192661,0.63853211,0.64587156,0.653211009,0.662385321,0.669724771,
0.67706422,0.68440367,0.691743119,0.699082569,0.706422018,0.713761468,0.721100917,
0.728440367,0.737614679,0.744954128,0.752293578,0.759633028,0.766972477,
0.776146789,0.783486239,0.790825688,0.798165138,0.805504587,0.811009174,
0.820183486,0.825688073,0.831192661,0.840366972,0.84587156,0.851376147,
0.856880734,0.862385321,0.867889908,0.873394495,0.878899083,0.88440367,
0.889908257,0.895412844,0.900917431,0.906422018,0.911926606,0.917431193,
0.92293578,0.928440367,0.933944954,0.939449541,0.944954128,0.950458716,
0.955963303,0.963302752,0.968807339,0.974311927,0.981651376,0.987155963,
0.99266055,1.),.UNSPECIFIED.);
#24483=B_SPLINE_CURVE_WITH_KNOTS('',3,(#290987,#290988,#290989,#290990,
#290991,#290992,#290993,#290994,#290995,#290996,#290997,#290998,#290999,
#291000,#291001,#291002,#291003,#291004,#291005,#291006,#291007,#291008,
#291009,#291010,#291011,#291012,#291013,#291014,#291015,#291016,#291017,
#291018,#291019,#291020,#291021,#291022,#291023,#291024,#291025,#291026,
#291027,#291028,#291029,#291030,#291031,#291032,#291033,#291034,#291035,
#291036,#291037,#291038,#291039,#291040,#291041,#291042,#291043,#291044,
#291045,#291046,#291047,#291048,#291049,#291050,#291051,#291052,#291053,
#291054,#291055,#291056,#291057,#291058,#291059,#291060,#291061,#291062,
#291063,#291064,#291065,#291066,#291067,#291068,#291069,#291070,#291071,
#291072,#291073,#291074,#291075,#291076,#291077,#291078,#291079,#291080,
#291081,#291082,#291083,#291084,#291085,#291086,#291087,#291088,#291089,
#291090,#291091,#291092,#291093,#291094,#291095,#291096,#291097,#291098,
#291099,#291100,#291101,#291102,#291103,#291104,#291105,#291106,#291107,
#291108,#291109,#291110,#291111,#291112,#291113,#291114,#291115,#291116,
#291117,#291118,#291119,#291120,#291121,#291122,#291123,#291124,#291125,
#291126,#291127,#291128,#291129,#291130,#291131,#291132,#291133,#291134,
#291135,#291136,#291137,#291138,#291139,#291140,#291141,#291142,#291143,
#291144,#291145,#291146,#291147,#291148,#291149,#291150,#291151,#291152,
#291153,#291154,#291155,#291156,#291157,#291158,#291159,#291160,#291161,
#291162,#291163,#291164,#291165,#291166,#291167,#291168,#291169,#291170,
#291171,#291172,#291173,#291174,#291175,#291176,#291177,#291178,#291179,
#291180,#291181,#291182,#291183,#291184,#291185,#291186,#291187,#291188,
#291189,#291190,#291191,#291192,#291193,#291194,#291195,#291196,#291197,
#291198,#291199,#291200,#291201,#291202,#291203,#291204,#291205,#291206,
#291207,#291208,#291209,#291210,#291211,#291212,#291213,#291214,#291215,
#291216,#291217,#291218,#291219,#291220,#291221,#291222,#291223,#291224,
#291225,#291226,#291227,#291228,#291229,#291230,#291231,#291232,#291233,
#291234,#291235,#291236,#291237,#291238,#291239,#291240,#291241,#291242,
#291243,#291244,#291245,#291246,#291247,#291248,#291249,#291250,#291251,
#291252,#291253,#291254,#291255,#291256,#291257,#291258,#291259,#291260,
#291261,#291262,#291263,#291264,#291265,#291266,#291267,#291268,#291269,
#291270,#291271,#291272,#291273,#291274,#291275,#291276,#291277,#291278,
#291279,#291280,#291281,#291282,#291283,#291284,#291285,#291286,#291287,
#291288,#291289,#291290,#291291,#291292,#291293,#291294,#291295,#291296,
#291297,#291298,#291299,#291300,#291301,#291302,#291303,#291304,#291305,
#291306,#291307,#291308,#291309,#291310,#291311),.UNSPECIFIED.,.F.,.F.,
(4,3,3,3,3,3,3,3,3,3,3,3,3,3,3,3,3,3,3,3,3,3,3,3,3,3,3,3,3,3,3,3,3,3,3,
3,3,3,3,3,3,3,3,3,3,3,3,3,3,3,3,3,3,3,3,3,3,3,3,3,3,3,3,3,3,3,3,3,3,3,3,
3,3,3,3,3,3,3,3,3,3,3,3,3,3,3,3,3,3,3,3,3,3,3,3,3,3,3,3,3,3,3,3,3,3,3,3,
3,4),(-1.,-0.994495413,-0.988990826,-0.983486239,-0.977981651,-0.972477064,
-0.965137615,-0.957798165,-0.952293578,-0.946788991,-0.941284404,-0.935779817,
-0.930275229,-0.924770642,-0.919266055,-0.913761468,-0.908256881,-0.900917431,
-0.895412844,-0.889908257,-0.88440367,-0.878899083,-0.873394495,-0.867889908,
-0.862385321,-0.856880734,-0.851376147,-0.84587156,-0.840366972,-0.834862385,
-0.829357798,-0.823853211,-0.814678899,-0.809174312,-0.801834862,-0.794495413,
-0.787155963,-0.779816514,-0.772477064,-0.765137615,-0.757798165,-0.750458716,
-0.743119266,-0.735779817,-0.728440367,-0.721100917,-0.713761468,-0.706422018,
-0.699082569,-0.691743119,-0.68440367,-0.67706422,-0.669724771,-0.662385321,
-0.655045872,-0.647706422,-0.640366972,-0.633027523,-0.625688073,-0.618348624,
-0.611009174,-0.603669725,-0.596330275,-0.588990826,-0.581651376,-0.574311927,
-0.566972477,-0.557798165,-0.550458716,-0.543119266,-0.535779817,-0.528440367,
-0.519266055,-0.510091743,-0.500917431,-0.491743119,-0.482568807,-0.473394495,
-0.464220183,-0.455045872,-0.44587156,-0.436697248,-0.427522936,-0.418348624,
-0.409174312,-0.4,-0.390825688,-0.379816514,-0.368807339,-0.357798165,-0.346788991,
-0.335779817,-0.324770642,-0.313761468,-0.302752294,-0.291743119,-0.280733945,
-0.269724771,-0.258715596,-0.247706422,-0.236697248,-0.225688073,-0.214678899,
-0.203669725,-0.19266055,-0.181651376,-0.170642202,-0.159633028,-0.143172102),
 .UNSPECIFIED.);
#24484=B_SPLINE_CURVE_WITH_KNOTS('',3,(#291312,#291313,#291314,#291315,
#291316,#291317,#291318,#291319,#291320,#291321,#291322,#291323,#291324,
#291325,#291326,#291327,#291328,#291329,#291330,#291331,#291332,#291333,
#291334,#291335,#291336,#291337,#291338,#291339,#291340,#291341,#291342,
#291343,#291344,#291345,#291346,#291347,#291348,#291349,#291350,#291351,
#291352,#291353,#291354,#291355,#291356,#291357,#291358,#291359,#291360,
#291361,#291362,#291363,#291364,#291365,#291366,#291367,#291368,#291369,
#291370,#291371,#291372,#291373,#291374,#291375,#291376,#291377,#291378,
#291379,#291380,#291381,#291382,#291383,#291384,#291385,#291386,#291387,
#291388,#291389,#291390,#291391,#291392,#291393,#291394,#291395,#291396,
#291397,#291398,#291399,#291400,#291401,#291402,#291403,#291404,#291405,
#291406,#291407,#291408,#291409,#291410,#291411,#291412,#291413,#291414,
#291415,#291416,#291417,#291418,#291419,#291420,#291421,#291422,#291423,
#291424,#291425,#291426,#291427,#291428,#291429,#291430,#291431,#291432,
#291433,#291434,#291435,#291436,#291437,#291438,#291439,#291440,#291441,
#291442,#291443,#291444,#291445,#291446,#291447,#291448,#291449,#291450,
#291451,#291452,#291453,#291454,#291455,#291456,#291457,#291458,#291459,
#291460,#291461,#291462,#291463,#291464,#291465,#291466,#291467,#291468,
#291469,#291470,#291471,#291472,#291473,#291474,#291475,#291476,#291477,
#291478,#291479,#291480,#291481,#291482,#291483,#291484,#291485,#291486,
#291487,#291488,#291489,#291490,#291491,#291492,#291493,#291494,#291495,
#291496,#291497,#291498,#291499,#291500,#291501,#291502,#291503,#291504,
#291505,#291506,#291507,#291508,#291509,#291510,#291511,#291512,#291513,
#291514,#291515,#291516,#291517,#291518,#291519,#291520,#291521,#291522,
#291523,#291524,#291525,#291526,#291527,#291528,#291529,#291530,#291531,
#291532,#291533,#291534,#291535,#291536,#291537,#291538,#291539,#291540,
#291541,#291542,#291543,#291544,#291545,#291546,#291547,#291548,#291549,
#291550,#291551,#291552,#291553,#291554,#291555,#291556,#291557,#291558,
#291559,#291560,#291561,#291562,#291563,#291564,#291565,#291566,#291567,
#291568,#291569,#291570,#291571,#291572,#291573,#291574,#291575,#291576,
#291577,#291578,#291579,#291580,#291581,#291582,#291583,#291584,#291585,
#291586,#291587,#291588,#291589,#291590,#291591,#291592,#291593,#291594,
#291595,#291596,#291597,#291598,#291599,#291600,#291601,#291602,#291603,
#291604,#291605,#291606,#291607,#291608,#291609,#291610,#291611,#291612,
#291613,#291614,#291615,#291616,#291617,#291618,#291619,#291620,#291621,
#291622,#291623,#291624,#291625,#291626,#291627,#291628,#291629,#291630,
#291631,#291632,#291633),.UNSPECIFIED.,.F.,.F.,(4,3,3,3,3,3,3,3,3,3,3,3,
3,3,3,3,3,3,3,3,3,3,3,3,3,3,3,3,3,3,3,3,3,3,3,3,3,3,3,3,3,3,3,3,3,3,3,3,
3,3,3,3,3,3,3,3,3,3,3,3,3,3,3,3,3,3,3,3,3,3,3,3,3,3,3,3,3,3,3,3,3,3,3,3,
3,3,3,3,3,3,3,3,3,3,3,3,3,3,3,3,3,3,3,3,3,3,3,4),(0.143172102,0.15412844,
0.165137615,0.176146789,0.187155963,0.198165138,0.209174312,0.220183486,
0.231192661,0.242201835,0.253211009,0.264220183,0.275229358,0.286238532,
0.297247706,0.308256881,0.319266055,0.330275229,0.341284404,0.352293578,
0.363302752,0.374311927,0.385321101,0.396330275,0.405504587,0.414678899,
0.423853211,0.433027523,0.442201835,0.451376147,0.460550459,0.469724771,
0.478899083,0.488073394,0.497247706,0.506422018,0.51559633,0.524770642,
0.533944954,0.541284404,0.548623853,0.555963303,0.563302752,0.572477064,
0.579816514,0.587155963,0.594495413,0.601834862,0.609174312,0.616513761,
0.623853211,0.631192661,0.63853211,0.64587156,0.653211009,0.662385321,0.669724771,
0.67706422,0.68440367,0.691743119,0.699082569,0.706422018,0.713761468,0.721100917,
0.728440367,0.737614679,0.744954128,0.752293578,0.759633028,0.766972477,
0.776146789,0.783486239,0.790825688,0.798165138,0.805504587,0.811009174,
0.820183486,0.825688073,0.831192661,0.840366972,0.84587156,0.853211009,
0.858715596,0.864220183,0.869724771,0.875229358,0.880733945,0.886238532,
0.891743119,0.897247706,0.902752294,0.910091743,0.91559633,0.921100917,
0.926605505,0.932110092,0.937614679,0.943119266,0.948623853,0.95412844,
0.96146789,0.966972477,0.972477064,0.977981651,0.983486239,0.988990826,
0.994495413,1.),.UNSPECIFIED.);
#24485=B_SPLINE_CURVE_WITH_KNOTS('',3,(#292578,#292579,#292580,#292581,
#292582,#292583,#292584,#292585,#292586,#292587,#292588,#292589,#292590,
#292591,#292592,#292593,#292594,#292595,#292596,#292597,#292598,#292599,
#292600,#292601,#292602,#292603,#292604,#292605,#292606,#292607,#292608,
#292609,#292610,#292611,#292612,#292613,#292614,#292615,#292616,#292617,
#292618,#292619,#292620,#292621,#292622,#292623,#292624,#292625,#292626,
#292627,#292628,#292629,#292630,#292631,#292632,#292633,#292634,#292635,
#292636,#292637,#292638,#292639,#292640,#292641,#292642,#292643,#292644,
#292645,#292646,#292647,#292648,#292649,#292650,#292651,#292652,#292653,
#292654,#292655,#292656,#292657,#292658,#292659,#292660,#292661,#292662,
#292663,#292664,#292665,#292666,#292667,#292668,#292669,#292670,#292671,
#292672,#292673,#292674,#292675,#292676,#292677,#292678,#292679,#292680,
#292681,#292682,#292683,#292684,#292685,#292686,#292687,#292688,#292689,
#292690,#292691,#292692,#292693,#292694,#292695,#292696,#292697,#292698,
#292699,#292700,#292701,#292702,#292703,#292704,#292705,#292706,#292707,
#292708,#292709,#292710,#292711,#292712,#292713,#292714,#292715,#292716,
#292717,#292718,#292719,#292720,#292721,#292722,#292723,#292724,#292725,
#292726,#292727,#292728,#292729,#292730,#292731,#292732,#292733,#292734,
#292735,#292736,#292737,#292738,#292739,#292740,#292741,#292742,#292743,
#292744,#292745,#292746,#292747,#292748,#292749,#292750,#292751,#292752,
#292753,#292754,#292755,#292756,#292757,#292758,#292759,#292760,#292761,
#292762,#292763,#292764,#292765,#292766,#292767,#292768,#292769,#292770,
#292771,#292772,#292773,#292774,#292775,#292776,#292777,#292778,#292779,
#292780,#292781,#292782,#292783,#292784,#292785,#292786,#292787,#292788,
#292789,#292790,#292791,#292792,#292793,#292794,#292795,#292796,#292797,
#292798,#292799,#292800,#292801,#292802,#292803,#292804,#292805,#292806,
#292807,#292808,#292809,#292810,#292811,#292812,#292813,#292814,#292815,
#292816,#292817,#292818,#292819,#292820,#292821,#292822,#292823,#292824,
#292825,#292826,#292827,#292828,#292829,#292830,#292831,#292832,#292833,
#292834,#292835,#292836,#292837,#292838,#292839,#292840,#292841,#292842,
#292843,#292844,#292845,#292846,#292847,#292848,#292849,#292850,#292851,
#292852,#292853,#292854,#292855,#292856,#292857,#292858,#292859,#292860,
#292861,#292862,#292863,#292864,#292865,#292866,#292867,#292868,#292869,
#292870,#292871,#292872,#292873,#292874,#292875,#292876,#292877,#292878,
#292879,#292880,#292881,#292882,#292883,#292884,#292885,#292886,#292887,
#292888,#292889,#292890),.UNSPECIFIED.,.F.,.F.,(4,3,3,3,3,3,3,3,3,3,3,3,
3,3,3,3,3,3,3,3,3,3,3,3,3,3,3,3,3,3,3,3,3,3,3,3,3,3,3,3,3,3,3,3,3,3,3,3,
3,3,3,3,3,3,3,3,3,3,3,3,3,3,3,3,3,3,3,3,3,3,3,3,3,3,3,3,3,3,3,3,3,3,3,3,
3,3,3,3,3,3,3,3,3,3,3,3,3,3,3,3,3,3,3,3,4),(0.143172102,0.15412844,0.165137615,
0.176146789,0.187155963,0.198165138,0.209174312,0.220183486,0.231192661,
0.242201835,0.253211009,0.264220183,0.275229358,0.286238532,0.297247706,
0.308256881,0.319266055,0.330275229,0.341284404,0.352293578,0.365137615,
0.376146789,0.388990826,0.398165138,0.40733945,0.416513761,0.425688073,
0.436697248,0.44587156,0.455045872,0.464220183,0.473394495,0.482568807,
0.495412844,0.504587156,0.513761468,0.52293578,0.532110092,0.539449541,
0.546788991,0.55412844,0.56146789,0.568807339,0.576146789,0.583486239,0.590825688,
0.598165138,0.60733945,0.614678899,0.622018349,0.631192661,0.63853211,0.64587156,
0.653211009,0.660550459,0.667889908,0.678899083,0.686238532,0.693577982,
0.702752294,0.711926606,0.719266055,0.726605505,0.735779817,0.743119266,
0.750458716,0.759633028,0.766972477,0.774311927,0.781651376,0.788990826,
0.796330275,0.803669725,0.812844037,0.818348624,0.823853211,0.831192661,
0.836697248,0.842201835,0.847706422,0.853211009,0.860550459,0.866055046,
0.871559633,0.878899083,0.88440367,0.889908257,0.895412844,0.902752294,
0.908256881,0.913761468,0.919266055,0.928440367,0.935779817,0.941284404,
0.946788991,0.952293578,0.96146789,0.966972477,0.972477064,0.977981651,
0.983486239,0.988990826,0.994495413,1.),.UNSPECIFIED.);
#24486=B_SPLINE_CURVE_WITH_KNOTS('',3,(#292891,#292892,#292893,#292894,
#292895,#292896,#292897,#292898,#292899,#292900,#292901,#292902,#292903,
#292904,#292905,#292906,#292907,#292908,#292909,#292910,#292911,#292912,
#292913,#292914,#292915,#292916,#292917,#292918,#292919,#292920,#292921,
#292922,#292923,#292924,#292925,#292926,#292927,#292928,#292929,#292930,
#292931,#292932,#292933,#292934,#292935,#292936,#292937,#292938,#292939,
#292940,#292941,#292942,#292943,#292944,#292945,#292946,#292947,#292948,
#292949,#292950,#292951,#292952,#292953,#292954,#292955,#292956,#292957,
#292958,#292959,#292960,#292961,#292962,#292963,#292964,#292965,#292966,
#292967,#292968,#292969,#292970,#292971,#292972,#292973,#292974,#292975,
#292976,#292977,#292978,#292979,#292980,#292981,#292982,#292983,#292984,
#292985,#292986,#292987,#292988,#292989,#292990,#292991,#292992,#292993,
#292994,#292995,#292996,#292997,#292998,#292999,#293000,#293001,#293002,
#293003,#293004,#293005,#293006,#293007,#293008,#293009,#293010,#293011,
#293012,#293013,#293014,#293015,#293016,#293017,#293018,#293019,#293020,
#293021,#293022,#293023,#293024,#293025,#293026,#293027,#293028,#293029,
#293030,#293031,#293032,#293033,#293034,#293035,#293036,#293037,#293038,
#293039,#293040,#293041,#293042,#293043,#293044,#293045,#293046,#293047,
#293048,#293049,#293050,#293051,#293052,#293053,#293054,#293055,#293056,
#293057,#293058,#293059,#293060,#293061,#293062,#293063,#293064,#293065,
#293066,#293067,#293068,#293069,#293070,#293071,#293072,#293073,#293074,
#293075,#293076,#293077,#293078,#293079,#293080,#293081,#293082,#293083,
#293084,#293085,#293086,#293087,#293088,#293089,#293090,#293091,#293092,
#293093,#293094,#293095,#293096,#293097,#293098,#293099,#293100,#293101,
#293102,#293103,#293104,#293105,#293106,#293107,#293108,#293109,#293110,
#293111,#293112,#293113,#293114,#293115,#293116,#293117,#293118,#293119,
#293120,#293121,#293122,#293123,#293124,#293125,#293126,#293127,#293128,
#293129,#293130,#293131,#293132,#293133,#293134,#293135,#293136,#293137,
#293138,#293139,#293140,#293141,#293142,#293143,#293144,#293145,#293146,
#293147,#293148,#293149,#293150,#293151,#293152,#293153,#293154,#293155,
#293156,#293157,#293158,#293159,#293160,#293161,#293162,#293163,#293164,
#293165,#293166,#293167,#293168,#293169,#293170,#293171,#293172,#293173,
#293174,#293175,#293176,#293177,#293178,#293179,#293180,#293181,#293182,
#293183,#293184,#293185,#293186,#293187,#293188,#293189,#293190,#293191,
#293192,#293193,#293194,#293195,#293196,#293197,#293198,#293199,#293200,
#293201,#293202,#293203,#293204,#293205,#293206,#293207,#293208,#293209,
#293210,#293211,#293212),.UNSPECIFIED.,.F.,.F.,(4,3,3,3,3,3,3,3,3,3,3,3,
3,3,3,3,3,3,3,3,3,3,3,3,3,3,3,3,3,3,3,3,3,3,3,3,3,3,3,3,3,3,3,3,3,3,3,3,
3,3,3,3,3,3,3,3,3,3,3,3,3,3,3,3,3,3,3,3,3,3,3,3,3,3,3,3,3,3,3,3,3,3,3,3,
3,3,3,3,3,3,3,3,3,3,3,3,3,3,3,3,3,3,3,3,3,3,3,4),(0.143172102,0.15412844,
0.165137615,0.176146789,0.187155963,0.198165138,0.209174312,0.220183486,
0.231192661,0.242201835,0.253211009,0.264220183,0.275229358,0.286238532,
0.297247706,0.308256881,0.319266055,0.330275229,0.341284404,0.352293578,
0.363302752,0.374311927,0.385321101,0.396330275,0.405504587,0.414678899,
0.423853211,0.433027523,0.442201835,0.451376147,0.460550459,0.469724771,
0.478899083,0.488073394,0.499082569,0.508256881,0.517431193,0.526605505,
0.533944954,0.541284404,0.548623853,0.555963303,0.563302752,0.570642202,
0.577981651,0.585321101,0.59266055,0.6,0.60733945,0.614678899,0.622018349,
0.629357798,0.636697248,0.644036697,0.651376147,0.658715596,0.666055046,
0.673394495,0.680733945,0.688073394,0.695412844,0.702752294,0.710091743,
0.717431193,0.724770642,0.732110092,0.739449541,0.748623853,0.755963303,
0.763302752,0.770642202,0.777981651,0.785321101,0.79266055,0.8,0.80733945,
0.812844037,0.820183486,0.827522936,0.833027523,0.842201835,0.847706422,
0.853211009,0.858715596,0.864220183,0.869724771,0.875229358,0.880733945,
0.886238532,0.891743119,0.897247706,0.902752294,0.908256881,0.913761468,
0.919266055,0.924770642,0.930275229,0.935779817,0.941284404,0.946788991,
0.952293578,0.957798165,0.966972477,0.972477064,0.979816514,0.985321101,
0.990825688,1.),.UNSPECIFIED.);
#24487=B_SPLINE_CURVE_WITH_KNOTS('',3,(#294172,#294173,#294174,#294175,
#294176,#294177,#294178,#294179,#294180,#294181,#294182,#294183,#294184,
#294185,#294186,#294187,#294188,#294189,#294190,#294191,#294192,#294193,
#294194,#294195,#294196,#294197,#294198,#294199,#294200,#294201,#294202,
#294203,#294204,#294205,#294206,#294207,#294208,#294209,#294210,#294211,
#294212,#294213,#294214,#294215,#294216,#294217,#294218,#294219,#294220,
#294221,#294222,#294223,#294224,#294225,#294226,#294227,#294228,#294229,
#294230,#294231,#294232,#294233,#294234,#294235,#294236,#294237,#294238,
#294239,#294240,#294241,#294242,#294243,#294244,#294245,#294246,#294247,
#294248,#294249,#294250,#294251,#294252,#294253,#294254,#294255,#294256,
#294257,#294258,#294259,#294260,#294261,#294262,#294263,#294264,#294265,
#294266,#294267,#294268,#294269,#294270,#294271,#294272,#294273,#294274,
#294275,#294276,#294277,#294278,#294279,#294280,#294281,#294282,#294283,
#294284,#294285,#294286,#294287,#294288,#294289,#294290,#294291,#294292,
#294293,#294294,#294295,#294296,#294297,#294298,#294299,#294300,#294301,
#294302,#294303,#294304,#294305,#294306,#294307,#294308,#294309,#294310,
#294311,#294312,#294313,#294314,#294315,#294316,#294317,#294318,#294319,
#294320,#294321,#294322,#294323,#294324,#294325,#294326,#294327,#294328,
#294329,#294330,#294331,#294332,#294333,#294334,#294335,#294336,#294337,
#294338,#294339,#294340,#294341,#294342,#294343,#294344,#294345,#294346,
#294347,#294348,#294349,#294350,#294351,#294352,#294353,#294354,#294355,
#294356,#294357,#294358,#294359,#294360,#294361,#294362,#294363,#294364,
#294365,#294366,#294367,#294368,#294369,#294370,#294371,#294372,#294373,
#294374,#294375,#294376,#294377,#294378,#294379,#294380,#294381,#294382,
#294383,#294384,#294385,#294386,#294387,#294388,#294389,#294390,#294391,
#294392,#294393,#294394,#294395,#294396,#294397,#294398,#294399,#294400,
#294401,#294402,#294403,#294404,#294405,#294406,#294407,#294408,#294409,
#294410,#294411,#294412,#294413,#294414,#294415,#294416,#294417,#294418,
#294419,#294420,#294421,#294422,#294423,#294424,#294425,#294426,#294427,
#294428,#294429,#294430,#294431,#294432,#294433,#294434,#294435,#294436,
#294437,#294438,#294439,#294440,#294441,#294442,#294443,#294444,#294445,
#294446,#294447,#294448,#294449,#294450,#294451,#294452,#294453,#294454,
#294455,#294456,#294457,#294458,#294459,#294460,#294461,#294462,#294463,
#294464,#294465,#294466,#294467,#294468,#294469,#294470,#294471,#294472,
#294473,#294474,#294475,#294476,#294477,#294478,#294479,#294480,#294481,
#294482,#294483,#294484,#294485,#294486,#294487),.UNSPECIFIED.,.F.,.F.,
(4,3,3,3,3,3,3,3,3,3,3,3,3,3,3,3,3,3,3,3,3,3,3,3,3,3,3,3,3,3,3,3,3,3,3,
3,3,3,3,3,3,3,3,3,3,3,3,3,3,3,3,3,3,3,3,3,3,3,3,3,3,3,3,3,3,3,3,3,3,3,3,
3,3,3,3,3,3,3,3,3,3,3,3,3,3,3,3,3,3,3,3,3,3,3,3,3,3,3,3,3,3,3,3,3,3,4),
(0.143172102,0.15412844,0.165137615,0.176146789,0.187155963,0.198165138,
0.209174312,0.220183486,0.231192661,0.242201835,0.253211009,0.264220183,
0.275229358,0.286238532,0.297247706,0.308256881,0.319266055,0.330275229,
0.341284404,0.352293578,0.363302752,0.374311927,0.385321101,0.396330275,
0.405504587,0.414678899,0.423853211,0.433027523,0.442201835,0.451376147,
0.460550459,0.469724771,0.478899083,0.488073394,0.499082569,0.508256881,
0.517431193,0.526605505,0.533944954,0.541284404,0.548623853,0.555963303,
0.565137615,0.572477064,0.579816514,0.587155963,0.594495413,0.601834862,
0.609174312,0.616513761,0.623853211,0.631192661,0.63853211,0.64587156,0.653211009,
0.660550459,0.667889908,0.678899083,0.686238532,0.693577982,0.700917431,
0.711926606,0.719266055,0.726605505,0.733944954,0.741284404,0.750458716,
0.757798165,0.765137615,0.772477064,0.779816514,0.788990826,0.796330275,
0.803669725,0.812844037,0.818348624,0.823853211,0.831192661,0.836697248,
0.842201835,0.847706422,0.855045872,0.860550459,0.866055046,0.871559633,
0.87706422,0.882568807,0.888073394,0.893577982,0.902752294,0.908256881,
0.913761468,0.919266055,0.928440367,0.935779817,0.941284404,0.946788991,
0.952293578,0.957798165,0.963302752,0.970642202,0.976146789,0.981651376,
0.987155963,0.99266055,1.),.UNSPECIFIED.);
#24488=B_SPLINE_CURVE_WITH_KNOTS('',3,(#294488,#294489,#294490,#294491,
#294492,#294493,#294494,#294495,#294496,#294497,#294498,#294499,#294500,
#294501,#294502,#294503,#294504,#294505,#294506,#294507,#294508,#294509,
#294510,#294511,#294512,#294513,#294514,#294515,#294516,#294517,#294518,
#294519,#294520,#294521,#294522,#294523,#294524,#294525,#294526,#294527,
#294528,#294529,#294530,#294531,#294532,#294533,#294534,#294535,#294536,
#294537,#294538,#294539,#294540,#294541,#294542,#294543,#294544,#294545,
#294546,#294547,#294548,#294549,#294550,#294551,#294552,#294553,#294554,
#294555,#294556,#294557,#294558,#294559,#294560,#294561,#294562,#294563,
#294564,#294565,#294566,#294567,#294568,#294569,#294570,#294571,#294572,
#294573,#294574,#294575,#294576,#294577,#294578,#294579,#294580,#294581,
#294582,#294583,#294584,#294585,#294586,#294587,#294588,#294589,#294590,
#294591,#294592,#294593,#294594,#294595,#294596,#294597,#294598,#294599,
#294600,#294601,#294602,#294603,#294604,#294605,#294606,#294607,#294608,
#294609,#294610,#294611,#294612,#294613,#294614,#294615,#294616,#294617,
#294618,#294619,#294620,#294621,#294622,#294623,#294624,#294625,#294626,
#294627,#294628,#294629,#294630,#294631,#294632,#294633,#294634,#294635,
#294636,#294637,#294638,#294639,#294640,#294641,#294642,#294643,#294644,
#294645,#294646,#294647,#294648,#294649,#294650,#294651,#294652,#294653,
#294654,#294655,#294656,#294657,#294658,#294659,#294660,#294661,#294662,
#294663,#294664,#294665,#294666,#294667,#294668,#294669,#294670,#294671,
#294672,#294673,#294674,#294675,#294676,#294677,#294678,#294679,#294680,
#294681,#294682,#294683,#294684,#294685,#294686,#294687,#294688,#294689,
#294690,#294691,#294692,#294693,#294694,#294695,#294696,#294697,#294698,
#294699,#294700,#294701,#294702,#294703,#294704,#294705,#294706,#294707,
#294708,#294709,#294710,#294711,#294712,#294713,#294714,#294715,#294716,
#294717,#294718,#294719,#294720,#294721,#294722,#294723,#294724,#294725,
#294726,#294727,#294728,#294729,#294730,#294731,#294732,#294733,#294734,
#294735,#294736,#294737,#294738,#294739,#294740,#294741,#294742,#294743,
#294744,#294745,#294746,#294747,#294748,#294749,#294750,#294751,#294752,
#294753,#294754,#294755,#294756,#294757,#294758,#294759,#294760,#294761,
#294762,#294763,#294764,#294765,#294766,#294767,#294768,#294769,#294770,
#294771,#294772,#294773,#294774,#294775,#294776,#294777,#294778,#294779,
#294780,#294781,#294782,#294783,#294784,#294785,#294786,#294787,#294788,
#294789,#294790,#294791,#294792,#294793,#294794,#294795,#294796,#294797,
#294798,#294799,#294800,#294801,#294802,#294803,#294804,#294805,#294806),
 .UNSPECIFIED.,.F.,.F.,(4,3,3,3,3,3,3,3,3,3,3,3,3,3,3,3,3,3,3,3,3,3,3,3,
3,3,3,3,3,3,3,3,3,3,3,3,3,3,3,3,3,3,3,3,3,3,3,3,3,3,3,3,3,3,3,3,3,3,3,3,
3,3,3,3,3,3,3,3,3,3,3,3,3,3,3,3,3,3,3,3,3,3,3,3,3,3,3,3,3,3,3,3,3,3,3,3,
3,3,3,3,3,3,3,3,3,3,4),(0.143172102,0.15412844,0.165137615,0.176146789,
0.187155963,0.198165138,0.209174312,0.220183486,0.231192661,0.242201835,
0.253211009,0.264220183,0.275229358,0.286238532,0.297247706,0.308256881,
0.319266055,0.330275229,0.341284404,0.352293578,0.363302752,0.374311927,
0.385321101,0.396330275,0.405504587,0.414678899,0.423853211,0.433027523,
0.442201835,0.451376147,0.460550459,0.469724771,0.478899083,0.488073394,
0.499082569,0.508256881,0.517431193,0.526605505,0.533944954,0.543119266,
0.550458716,0.559633028,0.566972477,0.574311927,0.581651376,0.588990826,
0.596330275,0.603669725,0.612844037,0.620183486,0.627522936,0.634862385,
0.642201835,0.649541284,0.656880734,0.664220183,0.673394495,0.680733945,
0.688073394,0.695412844,0.702752294,0.710091743,0.717431193,0.724770642,
0.733944954,0.741284404,0.748623853,0.755963303,0.763302752,0.772477064,
0.781651376,0.788990826,0.796330275,0.805504587,0.811009174,0.816513761,
0.822018349,0.827522936,0.833027523,0.83853211,0.844036697,0.849541284,
0.855045872,0.860550459,0.866055046,0.871559633,0.87706422,0.882568807,
0.888073394,0.893577982,0.900917431,0.906422018,0.911926606,0.921100917,
0.930275229,0.935779817,0.941284404,0.946788991,0.952293578,0.957798165,
0.963302752,0.968807339,0.976146789,0.981651376,0.987155963,0.994495413,
1.),.UNSPECIFIED.);
#24489=B_SPLINE_CURVE_WITH_KNOTS('',5,(#295754,#295755,#295756,#295757,
#295758,#295759,#295760,#295761,#295762,#295763,#295764,#295765,#295766,
#295767,#295768,#295769,#295770,#295771,#295772,#295773,#295774,#295775,
#295776,#295777,#295778,#295779,#295780,#295781,#295782,#295783,#295784,
#295785,#295786,#295787,#295788,#295789,#295790,#295791,#295792,#295793,
#295794,#295795,#295796,#295797,#295798,#295799,#295800,#295801,#295802,
#295803,#295804,#295805,#295806,#295807,#295808,#295809,#295810,#295811,
#295812,#295813,#295814,#295815,#295816,#295817,#295818,#295819,#295820,
#295821,#295822,#295823,#295824,#295825,#295826,#295827,#295828,#295829,
#295830,#295831,#295832,#295833,#295834,#295835,#295836,#295837,#295838,
#295839,#295840,#295841,#295842,#295843,#295844,#295845,#295846,#295847,
#295848,#295849,#295850,#295851,#295852,#295853,#295854,#295855,#295856,
#295857,#295858,#295859,#295860,#295861,#295862,#295863,#295864,#295865,
#295866,#295867,#295868,#295869,#295870,#295871,#295872,#295873,#295874,
#295875,#295876,#295877,#295878,#295879,#295880,#295881,#295882,#295883,
#295884,#295885,#295886,#295887,#295888,#295889,#295890,#295891,#295892,
#295893,#295894,#295895,#295896,#295897,#295898,#295899,#295900,#295901,
#295902,#295903,#295904,#295905,#295906,#295907,#295908,#295909,#295910,
#295911,#295912,#295913,#295914,#295915,#295916,#295917,#295918,#295919,
#295920,#295921,#295922,#295923,#295924,#295925,#295926,#295927,#295928,
#295929,#295930,#295931,#295932,#295933,#295934,#295935,#295936,#295937,
#295938,#295939,#295940,#295941,#295942,#295943,#295944,#295945,#295946,
#295947,#295948,#295949,#295950,#295951,#295952,#295953,#295954,#295955,
#295956,#295957,#295958,#295959,#295960,#295961,#295962,#295963,#295964,
#295965,#295966,#295967,#295968,#295969,#295970,#295971,#295972,#295973,
#295974,#295975,#295976,#295977,#295978,#295979,#295980,#295981,#295982,
#295983,#295984,#295985,#295986,#295987,#295988,#295989,#295990,#295991,
#295992,#295993,#295994,#295995,#295996,#295997,#295998,#295999,#296000,
#296001,#296002,#296003,#296004,#296005,#296006,#296007,#296008,#296009,
#296010,#296011,#296012,#296013,#296014,#296015,#296016,#296017,#296018,
#296019,#296020,#296021,#296022,#296023,#296024,#296025,#296026,#296027,
#296028,#296029,#296030,#296031,#296032,#296033,#296034,#296035,#296036,
#296037,#296038,#296039,#296040,#296041,#296042,#296043,#296044,#296045,
#296046,#296047,#296048,#296049,#296050,#296051,#296052,#296053,#296054,
#296055,#296056,#296057,#296058,#296059,#296060,#296061,#296062,#296063,
#296064,#296065,#296066,#296067,#296068,#296069,#296070,#296071,#296072,
#296073,#296074,#296075,#296076,#296077,#296078,#296079,#296080,#296081,
#296082,#296083,#296084,#296085,#296086,#296087,#296088,#296089,#296090,
#296091,#296092,#296093,#296094,#296095,#296096,#296097,#296098,#296099,
#296100,#296101,#296102,#296103,#296104,#296105,#296106,#296107,#296108,
#296109,#296110,#296111,#296112,#296113,#296114,#296115,#296116,#296117,
#296118,#296119,#296120,#296121,#296122,#296123,#296124,#296125,#296126,
#296127,#296128,#296129,#296130,#296131,#296132,#296133,#296134,#296135,
#296136,#296137,#296138,#296139,#296140,#296141,#296142,#296143,#296144,
#296145,#296146,#296147,#296148,#296149,#296150,#296151,#296152,#296153,
#296154,#296155,#296156,#296157,#296158,#296159,#296160,#296161,#296162,
#296163,#296164,#296165,#296166,#296167,#296168,#296169,#296170,#296171,
#296172,#296173,#296174,#296175,#296176,#296177,#296178,#296179,#296180,
#296181,#296182,#296183,#296184,#296185,#296186,#296187,#296188,#296189,
#296190,#296191,#296192,#296193,#296194,#296195,#296196,#296197,#296198,
#296199,#296200,#296201,#296202,#296203,#296204,#296205,#296206,#296207,
#296208,#296209,#296210,#296211,#296212,#296213,#296214,#296215,#296216,
#296217,#296218,#296219,#296220,#296221,#296222,#296223,#296224,#296225),
 .UNSPECIFIED.,.F.,.F.,(6,1,1,1,1,1,1,1,1,1,1,1,1,1,1,1,1,1,1,1,1,1,1,1,
1,1,1,1,1,1,1,1,1,1,1,1,1,1,1,1,1,1,1,1,1,1,1,1,1,1,1,1,1,1,1,1,1,1,1,1,
1,1,1,1,1,1,1,1,1,1,1,1,1,1,1,1,1,1,1,1,1,1,1,1,1,1,1,1,1,1,1,1,1,1,1,1,
1,1,1,1,1,1,1,1,1,1,1,1,1,1,1,1,1,1,1,1,1,1,1,1,1,1,1,1,1,1,1,1,1,1,1,1,
1,1,1,1,1,1,1,1,1,1,1,1,1,1,1,1,1,1,1,1,1,1,1,1,1,1,1,1,1,1,1,1,1,1,1,1,
1,1,1,1,1,1,1,1,1,1,1,1,1,1,1,1,1,1,1,1,1,1,1,1,1,1,1,1,1,1,1,1,1,1,1,1,
1,1,1,1,1,1,1,1,1,1,1,1,1,1,1,1,1,1,1,1,1,1,1,1,1,1,1,1,1,1,1,1,1,1,1,1,
1,1,1,1,1,1,1,1,1,1,1,1,1,1,1,1,1,1,1,1,1,1,1,1,1,1,1,1,1,1,1,1,1,1,1,1,
1,1,1,1,1,1,1,1,1,1,1,1,1,1,1,1,1,1,1,1,1,1,1,1,1,1,1,1,1,1,1,1,1,1,1,1,
1,1,1,1,1,1,1,1,1,1,1,1,1,1,1,1,1,1,1,1,1,1,1,1,1,1,1,1,1,1,1,1,1,1,1,1,
1,1,1,1,1,1,1,1,1,1,1,1,1,1,1,1,1,1,1,1,1,1,1,1,1,1,1,1,1,1,1,1,1,1,1,1,
1,1,1,1,1,1,1,1,1,1,1,1,1,1,1,1,1,1,1,1,1,1,1,1,1,1,1,1,1,1,1,1,1,1,1,1,
1,1,1,1,1,1,1,1,1,1,1,1,1,1,1,1,1,1,1,1,1,1,1,1,1,1,1,1,1,1,1,1,1,1,1,1,
1,1,1,1,1,1,1,1,1,1,1,6),(-1.,-0.998165138,-0.996330275,-0.994495413,-0.99266055,
-0.990825688,-0.988990826,-0.987155963,-0.985321101,-0.983486239,-0.981651376,
-0.979816514,-0.977981651,-0.976146789,-0.974311927,-0.972477064,-0.970642202,
-0.968807339,-0.966972477,-0.965137615,-0.963302752,-0.96146789,-0.959633028,
-0.957798165,-0.955963303,-0.95412844,-0.952293578,-0.950458716,-0.948623853,
-0.946788991,-0.944954128,-0.943119266,-0.941284404,-0.939449541,-0.937614679,
-0.935779817,-0.933944954,-0.932110092,-0.930275229,-0.928440367,-0.926605505,
-0.924770642,-0.92293578,-0.921100917,-0.919266055,-0.917431193,-0.91559633,
-0.913761468,-0.911926606,-0.910091743,-0.908256881,-0.906422018,-0.904587156,
-0.902752294,-0.900917431,-0.899082569,-0.897247706,-0.895412844,-0.893577982,
-0.891743119,-0.889908257,-0.888073394,-0.886238532,-0.88440367,-0.882568807,
-0.880733945,-0.878899083,-0.87706422,-0.875229358,-0.873394495,-0.871559633,
-0.869724771,-0.867889908,-0.866055046,-0.864220183,-0.862385321,-0.860550459,
-0.858715596,-0.856880734,-0.855045872,-0.853211009,-0.851376147,-0.849541284,
-0.847706422,-0.84587156,-0.844036697,-0.842201835,-0.840366972,-0.83853211,
-0.836697248,-0.834862385,-0.833027523,-0.831192661,-0.829357798,-0.827522936,
-0.825688073,-0.823853211,-0.822018349,-0.820183486,-0.818348624,-0.816513761,
-0.814678899,-0.812844037,-0.811009174,-0.809174312,-0.80733945,-0.805504587,
-0.803669725,-0.801834862,-0.8,-0.798165138,-0.796330275,-0.794495413,-0.79266055,
-0.790825688,-0.788990826,-0.787155963,-0.785321101,-0.783486239,-0.781651376,
-0.779816514,-0.777981651,-0.776146789,-0.774311927,-0.772477064,-0.770642202,
-0.768807339,-0.766972477,-0.765137615,-0.763302752,-0.76146789,-0.759633028,
-0.757798165,-0.755963303,-0.75412844,-0.752293578,-0.750458716,-0.748623853,
-0.746788991,-0.744954128,-0.743119266,-0.741284404,-0.739449541,-0.737614679,
-0.735779817,-0.733944954,-0.732110092,-0.730275229,-0.728440367,-0.726605505,
-0.724770642,-0.72293578,-0.721100917,-0.719266055,-0.717431193,-0.71559633,
-0.713761468,-0.711926606,-0.710091743,-0.708256881,-0.706422018,-0.704587156,
-0.702752294,-0.700917431,-0.699082569,-0.697247706,-0.695412844,-0.693577982,
-0.691743119,-0.689908257,-0.688073394,-0.686238532,-0.68440367,-0.682568807,
-0.680733945,-0.678899083,-0.67706422,-0.675229358,-0.673394495,-0.671559633,
-0.669724771,-0.667889908,-0.666055046,-0.664220183,-0.662385321,-0.660550459,
-0.658715596,-0.656880734,-0.655045872,-0.653211009,-0.651376147,-0.649541284,
-0.647706422,-0.64587156,-0.644036697,-0.642201835,-0.640366972,-0.63853211,
-0.636697248,-0.634862385,-0.633027523,-0.631192661,-0.629357798,-0.627522936,
-0.625688073,-0.623853211,-0.622018349,-0.620183486,-0.618348624,-0.616513761,
-0.614678899,-0.612844037,-0.611009174,-0.609174312,-0.60733945,-0.605504587,
-0.603669725,-0.601834862,-0.6,-0.598165138,-0.596330275,-0.594495413,-0.59266055,
-0.590825688,-0.588990826,-0.587155963,-0.585321101,-0.583486239,-0.581651376,
-0.579816514,-0.577981651,-0.576146789,-0.574311927,-0.572477064,-0.570642202,
-0.568807339,-0.566972477,-0.565137615,-0.563302752,-0.56146789,-0.559633028,
-0.557798165,-0.555963303,-0.55412844,-0.552293578,-0.550458716,-0.548623853,
-0.546788991,-0.544954128,-0.543119266,-0.541284404,-0.539449541,-0.537614679,
-0.535779817,-0.533944954,-0.532110092,-0.530275229,-0.528440367,-0.526605505,
-0.524770642,-0.52293578,-0.521100917,-0.519266055,-0.517431193,-0.51559633,
-0.513761468,-0.511926606,-0.510091743,-0.508256881,-0.506422018,-0.504587156,
-0.502752294,-0.500917431,-0.499082569,-0.497247706,-0.495412844,-0.493577982,
-0.491743119,-0.489908257,-0.488073394,-0.486238532,-0.48440367,-0.482568807,
-0.480733945,-0.478899083,-0.47706422,-0.475229358,-0.473394495,-0.471559633,
-0.469724771,-0.467889908,-0.466055046,-0.464220183,-0.462385321,-0.460550459,
-0.458715596,-0.456880734,-0.455045872,-0.453211009,-0.451376147,-0.449541284,
-0.447706422,-0.44587156,-0.444036697,-0.442201835,-0.440366972,-0.43853211,
-0.436697248,-0.434862385,-0.433027523,-0.431192661,-0.429357798,-0.427522936,
-0.425688073,-0.423853211,-0.422018349,-0.420183486,-0.418348624,-0.416513761,
-0.414678899,-0.412844037,-0.411009174,-0.409174312,-0.40733945,-0.405504587,
-0.403669725,-0.401834862,-0.4,-0.398165138,-0.396330275,-0.394495413,-0.39266055,
-0.390825688,-0.388990826,-0.387155963,-0.385321101,-0.383486239,-0.381651376,
-0.379816514,-0.377981651,-0.376146789,-0.374311927,-0.372477064,-0.370642202,
-0.368807339,-0.366972477,-0.365137615,-0.363302752,-0.36146789,-0.359633028,
-0.357798165,-0.355963303,-0.35412844,-0.352293578,-0.350458716,-0.348623853,
-0.346788991,-0.344954128,-0.343119266,-0.341284404,-0.339449541,-0.337614679,
-0.335779817,-0.333944954,-0.332110092,-0.330275229,-0.328440367,-0.326605505,
-0.324770642,-0.32293578,-0.321100917,-0.319266055,-0.317431193,-0.31559633,
-0.313761468,-0.311926606,-0.310091743,-0.308256881,-0.306422018,-0.304587156,
-0.302752294,-0.300917431,-0.299082569,-0.297247706,-0.295412844,-0.293577982,
-0.291743119,-0.289908257,-0.288073394,-0.286238532,-0.28440367,-0.282568807,
-0.280733945,-0.278899083,-0.27706422,-0.275229358,-0.273394495,-0.271559633,
-0.269724771,-0.267889908,-0.266055046,-0.264220183,-0.262385321,-0.260550459,
-0.258715596,-0.256880734,-0.255045872,-0.253211009,-0.251376147,-0.249541284,
-0.247706422,-0.24587156,-0.244036697,-0.242201835,-0.240366972,-0.23853211,
-0.236697248,-0.234862385,-0.233027523,-0.231192661,-0.229357798,-0.227522936,
-0.225688073,-0.223853211,-0.222018349,-0.220183486,-0.218348624,-0.216513761,
-0.214678899,-0.212844037,-0.211009174,-0.209174312,-0.20733945,-0.205504587,
-0.203669725,-0.201834862,-0.2,-0.198165138,-0.196330275,-0.194495413,-0.19266055,
-0.190825688,-0.188990826,-0.187155963,-0.185321101,-0.183486239,-0.181651376,
-0.179816514,-0.177981651,-0.176146789,-0.174311927,-0.172477064,-0.170642202,
-0.168807339,-0.166972477,-0.165137615,-0.163302752,-0.16146789,-0.159633028,
-0.157798165,-0.155963303,-0.15412844,-0.152293578,-0.150458716,-0.148623853,
-0.146788991,-0.144954128,-0.143172102),.UNSPECIFIED.);
#24490=B_SPLINE_CURVE_WITH_KNOTS('',5,(#296226,#296227,#296228,#296229,
#296230,#296231,#296232,#296233,#296234,#296235,#296236,#296237,#296238,
#296239,#296240,#296241,#296242,#296243,#296244,#296245,#296246,#296247,
#296248,#296249,#296250,#296251,#296252,#296253,#296254,#296255,#296256,
#296257,#296258,#296259,#296260,#296261,#296262,#296263,#296264,#296265,
#296266,#296267,#296268,#296269,#296270,#296271,#296272,#296273,#296274,
#296275,#296276,#296277,#296278,#296279,#296280,#296281,#296282,#296283,
#296284,#296285,#296286,#296287,#296288,#296289,#296290,#296291,#296292,
#296293,#296294,#296295,#296296,#296297,#296298,#296299,#296300,#296301,
#296302,#296303,#296304,#296305,#296306,#296307,#296308,#296309,#296310,
#296311,#296312,#296313,#296314,#296315,#296316,#296317,#296318,#296319,
#296320,#296321,#296322,#296323,#296324,#296325,#296326,#296327,#296328,
#296329,#296330,#296331,#296332,#296333,#296334,#296335,#296336,#296337,
#296338,#296339,#296340,#296341,#296342,#296343,#296344,#296345,#296346,
#296347,#296348,#296349,#296350,#296351,#296352,#296353,#296354,#296355,
#296356,#296357,#296358,#296359,#296360,#296361,#296362,#296363,#296364,
#296365,#296366,#296367,#296368,#296369,#296370,#296371,#296372,#296373,
#296374,#296375,#296376,#296377,#296378,#296379,#296380,#296381,#296382,
#296383,#296384,#296385,#296386,#296387,#296388,#296389,#296390,#296391,
#296392,#296393,#296394,#296395,#296396,#296397,#296398,#296399,#296400,
#296401,#296402,#296403,#296404,#296405,#296406,#296407,#296408,#296409,
#296410,#296411,#296412,#296413,#296414,#296415,#296416,#296417,#296418,
#296419,#296420,#296421,#296422,#296423,#296424,#296425,#296426,#296427,
#296428,#296429,#296430,#296431,#296432,#296433,#296434,#296435,#296436,
#296437,#296438,#296439,#296440,#296441,#296442,#296443,#296444,#296445,
#296446,#296447,#296448,#296449,#296450,#296451,#296452,#296453,#296454,
#296455,#296456,#296457,#296458,#296459,#296460,#296461,#296462,#296463,
#296464,#296465,#296466,#296467,#296468,#296469,#296470,#296471,#296472,
#296473,#296474,#296475,#296476,#296477,#296478,#296479,#296480,#296481,
#296482,#296483,#296484,#296485,#296486,#296487,#296488,#296489,#296490,
#296491,#296492,#296493,#296494,#296495,#296496,#296497,#296498,#296499,
#296500,#296501,#296502,#296503,#296504,#296505,#296506,#296507,#296508,
#296509,#296510,#296511,#296512,#296513,#296514,#296515,#296516,#296517,
#296518,#296519,#296520,#296521,#296522,#296523,#296524,#296525,#296526,
#296527,#296528,#296529,#296530,#296531,#296532,#296533,#296534,#296535,
#296536,#296537,#296538,#296539,#296540,#296541,#296542,#296543,#296544,
#296545,#296546,#296547,#296548,#296549,#296550,#296551,#296552,#296553,
#296554,#296555,#296556,#296557,#296558,#296559,#296560,#296561,#296562,
#296563,#296564,#296565,#296566,#296567,#296568,#296569,#296570,#296571,
#296572,#296573,#296574,#296575,#296576,#296577,#296578,#296579,#296580,
#296581,#296582,#296583,#296584,#296585,#296586,#296587,#296588,#296589,
#296590,#296591,#296592,#296593,#296594,#296595,#296596,#296597,#296598,
#296599,#296600,#296601,#296602,#296603,#296604,#296605,#296606,#296607,
#296608,#296609,#296610,#296611,#296612,#296613,#296614,#296615,#296616,
#296617,#296618,#296619,#296620,#296621,#296622,#296623,#296624,#296625,
#296626,#296627,#296628,#296629,#296630,#296631,#296632,#296633,#296634,
#296635,#296636,#296637,#296638,#296639,#296640,#296641,#296642,#296643,
#296644,#296645,#296646,#296647,#296648,#296649,#296650,#296651,#296652,
#296653,#296654,#296655,#296656,#296657,#296658,#296659,#296660,#296661,
#296662,#296663,#296664,#296665,#296666,#296667,#296668,#296669,#296670,
#296671,#296672,#296673,#296674,#296675,#296676,#296677,#296678,#296679,
#296680,#296681,#296682,#296683,#296684,#296685,#296686,#296687,#296688,
#296689,#296690,#296691,#296692,#296693,#296694,#296695,#296696,#296697),
 .UNSPECIFIED.,.F.,.F.,(6,1,1,1,1,1,1,1,1,1,1,1,1,1,1,1,1,1,1,1,1,1,1,1,
1,1,1,1,1,1,1,1,1,1,1,1,1,1,1,1,1,1,1,1,1,1,1,1,1,1,1,1,1,1,1,1,1,1,1,1,
1,1,1,1,1,1,1,1,1,1,1,1,1,1,1,1,1,1,1,1,1,1,1,1,1,1,1,1,1,1,1,1,1,1,1,1,
1,1,1,1,1,1,1,1,1,1,1,1,1,1,1,1,1,1,1,1,1,1,1,1,1,1,1,1,1,1,1,1,1,1,1,1,
1,1,1,1,1,1,1,1,1,1,1,1,1,1,1,1,1,1,1,1,1,1,1,1,1,1,1,1,1,1,1,1,1,1,1,1,
1,1,1,1,1,1,1,1,1,1,1,1,1,1,1,1,1,1,1,1,1,1,1,1,1,1,1,1,1,1,1,1,1,1,1,1,
1,1,1,1,1,1,1,1,1,1,1,1,1,1,1,1,1,1,1,1,1,1,1,1,1,1,1,1,1,1,1,1,1,1,1,1,
1,1,1,1,1,1,1,1,1,1,1,1,1,1,1,1,1,1,1,1,1,1,1,1,1,1,1,1,1,1,1,1,1,1,1,1,
1,1,1,1,1,1,1,1,1,1,1,1,1,1,1,1,1,1,1,1,1,1,1,1,1,1,1,1,1,1,1,1,1,1,1,1,
1,1,1,1,1,1,1,1,1,1,1,1,1,1,1,1,1,1,1,1,1,1,1,1,1,1,1,1,1,1,1,1,1,1,1,1,
1,1,1,1,1,1,1,1,1,1,1,1,1,1,1,1,1,1,1,1,1,1,1,1,1,1,1,1,1,1,1,1,1,1,1,1,
1,1,1,1,1,1,1,1,1,1,1,1,1,1,1,1,1,1,1,1,1,1,1,1,1,1,1,1,1,1,1,1,1,1,1,1,
1,1,1,1,1,1,1,1,1,1,1,1,1,1,1,1,1,1,1,1,1,1,1,1,1,1,1,1,1,1,1,1,1,1,1,1,
1,1,1,1,1,1,1,1,1,1,1,6),(0.143172102,0.144954128,0.146788991,0.148623853,
0.150458716,0.152293578,0.15412844,0.155963303,0.157798165,0.159633028,
0.16146789,0.163302752,0.165137615,0.166972477,0.168807339,0.170642202,
0.172477064,0.174311927,0.176146789,0.177981651,0.179816514,0.181651376,
0.183486239,0.185321101,0.187155963,0.188990826,0.190825688,0.19266055,
0.194495413,0.196330275,0.198165138,0.2,0.201834862,0.203669725,0.205504587,
0.20733945,0.209174312,0.211009174,0.212844037,0.214678899,0.216513761,
0.218348624,0.220183486,0.222018349,0.223853211,0.225688073,0.227522936,
0.229357798,0.231192661,0.233027523,0.234862385,0.236697248,0.23853211,
0.240366972,0.242201835,0.244036697,0.24587156,0.247706422,0.249541284,
0.251376147,0.253211009,0.255045872,0.256880734,0.258715596,0.260550459,
0.262385321,0.264220183,0.266055046,0.267889908,0.269724771,0.271559633,
0.273394495,0.275229358,0.27706422,0.278899083,0.280733945,0.282568807,
0.28440367,0.286238532,0.288073394,0.289908257,0.291743119,0.293577982,
0.295412844,0.297247706,0.299082569,0.300917431,0.302752294,0.304587156,
0.306422018,0.308256881,0.310091743,0.311926606,0.313761468,0.31559633,
0.317431193,0.319266055,0.321100917,0.32293578,0.324770642,0.326605505,
0.328440367,0.330275229,0.332110092,0.333944954,0.335779817,0.337614679,
0.339449541,0.341284404,0.343119266,0.344954128,0.346788991,0.348623853,
0.350458716,0.352293578,0.35412844,0.355963303,0.357798165,0.359633028,
0.36146789,0.363302752,0.365137615,0.366972477,0.368807339,0.370642202,
0.372477064,0.374311927,0.376146789,0.377981651,0.379816514,0.381651376,
0.383486239,0.385321101,0.387155963,0.388990826,0.390825688,0.39266055,
0.394495413,0.396330275,0.398165138,0.4,0.401834862,0.403669725,0.405504587,
0.40733945,0.409174312,0.411009174,0.412844037,0.414678899,0.416513761,
0.418348624,0.420183486,0.422018349,0.423853211,0.425688073,0.427522936,
0.429357798,0.431192661,0.433027523,0.434862385,0.436697248,0.43853211,
0.440366972,0.442201835,0.444036697,0.44587156,0.447706422,0.449541284,
0.451376147,0.453211009,0.455045872,0.456880734,0.458715596,0.460550459,
0.462385321,0.464220183,0.466055046,0.467889908,0.469724771,0.471559633,
0.473394495,0.475229358,0.47706422,0.478899083,0.480733945,0.482568807,
0.48440367,0.486238532,0.488073394,0.489908257,0.491743119,0.493577982,
0.495412844,0.497247706,0.499082569,0.500917431,0.502752294,0.504587156,
0.506422018,0.508256881,0.510091743,0.511926606,0.513761468,0.51559633,
0.517431193,0.519266055,0.521100917,0.52293578,0.524770642,0.526605505,
0.528440367,0.530275229,0.532110092,0.533944954,0.535779817,0.537614679,
0.539449541,0.541284404,0.543119266,0.544954128,0.546788991,0.548623853,
0.550458716,0.552293578,0.55412844,0.555963303,0.557798165,0.559633028,
0.56146789,0.563302752,0.565137615,0.566972477,0.568807339,0.570642202,
0.572477064,0.574311927,0.576146789,0.577981651,0.579816514,0.581651376,
0.583486239,0.585321101,0.587155963,0.588990826,0.590825688,0.59266055,
0.594495413,0.596330275,0.598165138,0.6,0.601834862,0.603669725,0.605504587,
0.60733945,0.609174312,0.611009174,0.612844037,0.614678899,0.616513761,
0.618348624,0.620183486,0.622018349,0.623853211,0.625688073,0.627522936,
0.629357798,0.631192661,0.633027523,0.634862385,0.636697248,0.63853211,
0.640366972,0.642201835,0.644036697,0.64587156,0.647706422,0.649541284,
0.651376147,0.653211009,0.655045872,0.656880734,0.658715596,0.660550459,
0.662385321,0.664220183,0.666055046,0.667889908,0.669724771,0.671559633,
0.673394495,0.675229358,0.67706422,0.678899083,0.680733945,0.682568807,
0.68440367,0.686238532,0.688073394,0.689908257,0.691743119,0.693577982,
0.695412844,0.697247706,0.699082569,0.700917431,0.702752294,0.704587156,
0.706422018,0.708256881,0.710091743,0.711926606,0.713761468,0.71559633,
0.717431193,0.719266055,0.721100917,0.72293578,0.724770642,0.726605505,
0.728440367,0.730275229,0.732110092,0.733944954,0.735779817,0.737614679,
0.739449541,0.741284404,0.743119266,0.744954128,0.746788991,0.748623853,
0.750458716,0.752293578,0.75412844,0.755963303,0.757798165,0.759633028,
0.76146789,0.763302752,0.765137615,0.766972477,0.768807339,0.770642202,
0.772477064,0.774311927,0.776146789,0.777981651,0.779816514,0.781651376,
0.783486239,0.785321101,0.787155963,0.788990826,0.790825688,0.79266055,
0.794495413,0.796330275,0.798165138,0.8,0.801834862,0.803669725,0.805504587,
0.80733945,0.809174312,0.811009174,0.812844037,0.814678899,0.816513761,
0.818348624,0.820183486,0.822018349,0.823853211,0.825688073,0.827522936,
0.829357798,0.831192661,0.833027523,0.834862385,0.836697248,0.83853211,
0.840366972,0.842201835,0.844036697,0.84587156,0.847706422,0.849541284,
0.851376147,0.853211009,0.855045872,0.856880734,0.858715596,0.860550459,
0.862385321,0.864220183,0.866055046,0.867889908,0.869724771,0.871559633,
0.873394495,0.875229358,0.87706422,0.878899083,0.880733945,0.882568807,
0.88440367,0.886238532,0.888073394,0.889908257,0.891743119,0.893577982,
0.895412844,0.897247706,0.899082569,0.900917431,0.902752294,0.904587156,
0.906422018,0.908256881,0.910091743,0.911926606,0.913761468,0.91559633,
0.917431193,0.919266055,0.921100917,0.92293578,0.924770642,0.926605505,
0.928440367,0.930275229,0.932110092,0.933944954,0.935779817,0.937614679,
0.939449541,0.941284404,0.943119266,0.944954128,0.946788991,0.948623853,
0.950458716,0.952293578,0.95412844,0.955963303,0.957798165,0.959633028,
0.96146789,0.963302752,0.965137615,0.966972477,0.968807339,0.970642202,
0.972477064,0.974311927,0.976146789,0.977981651,0.979816514,0.981651376,
0.983486239,0.985321101,0.987155963,0.988990826,0.990825688,0.99266055,
0.994495413,0.996330275,0.998165138,1.),.UNSPECIFIED.);
#24491=B_SPLINE_CURVE_WITH_KNOTS('',5,(#296704,#296705,#296706,#296707,
#296708,#296709,#296710,#296711,#296712,#296713,#296714,#296715,#296716,
#296717,#296718,#296719,#296720,#296721,#296722,#296723,#296724,#296725,
#296726,#296727,#296728,#296729,#296730,#296731,#296732,#296733,#296734,
#296735,#296736,#296737,#296738,#296739,#296740,#296741,#296742,#296743,
#296744,#296745,#296746,#296747,#296748,#296749,#296750,#296751,#296752,
#296753,#296754,#296755,#296756,#296757,#296758,#296759,#296760,#296761,
#296762,#296763,#296764,#296765,#296766,#296767,#296768,#296769,#296770,
#296771,#296772,#296773,#296774,#296775,#296776,#296777,#296778,#296779,
#296780,#296781,#296782,#296783,#296784,#296785,#296786,#296787,#296788,
#296789,#296790,#296791,#296792,#296793,#296794,#296795,#296796,#296797,
#296798,#296799,#296800,#296801,#296802,#296803,#296804,#296805,#296806,
#296807,#296808,#296809,#296810,#296811,#296812,#296813,#296814,#296815,
#296816,#296817,#296818,#296819,#296820,#296821,#296822,#296823,#296824,
#296825,#296826,#296827,#296828,#296829,#296830,#296831,#296832,#296833,
#296834,#296835,#296836,#296837,#296838,#296839,#296840,#296841,#296842,
#296843,#296844,#296845,#296846,#296847,#296848,#296849,#296850,#296851,
#296852,#296853,#296854,#296855,#296856,#296857,#296858,#296859,#296860,
#296861,#296862,#296863,#296864,#296865,#296866,#296867,#296868,#296869,
#296870,#296871,#296872,#296873,#296874,#296875,#296876,#296877,#296878,
#296879,#296880,#296881,#296882,#296883,#296884,#296885,#296886,#296887,
#296888,#296889,#296890,#296891,#296892,#296893,#296894,#296895,#296896,
#296897,#296898,#296899,#296900,#296901,#296902,#296903,#296904,#296905,
#296906,#296907,#296908,#296909,#296910,#296911,#296912,#296913,#296914,
#296915,#296916,#296917,#296918,#296919,#296920,#296921,#296922,#296923,
#296924,#296925,#296926,#296927,#296928,#296929,#296930,#296931,#296932,
#296933,#296934,#296935,#296936,#296937,#296938,#296939,#296940,#296941,
#296942,#296943,#296944,#296945,#296946,#296947,#296948,#296949,#296950,
#296951,#296952,#296953,#296954,#296955,#296956,#296957,#296958,#296959,
#296960,#296961,#296962,#296963,#296964,#296965,#296966,#296967,#296968,
#296969,#296970,#296971,#296972,#296973,#296974,#296975,#296976,#296977,
#296978,#296979,#296980,#296981,#296982,#296983,#296984,#296985,#296986,
#296987,#296988,#296989,#296990,#296991,#296992,#296993,#296994,#296995,
#296996,#296997,#296998,#296999,#297000,#297001,#297002,#297003,#297004,
#297005,#297006,#297007,#297008,#297009,#297010,#297011,#297012,#297013,
#297014,#297015,#297016,#297017,#297018,#297019,#297020,#297021,#297022,
#297023,#297024,#297025,#297026,#297027,#297028,#297029,#297030,#297031,
#297032,#297033,#297034,#297035,#297036,#297037,#297038,#297039,#297040,
#297041,#297042,#297043,#297044,#297045,#297046,#297047,#297048,#297049,
#297050,#297051,#297052,#297053,#297054,#297055,#297056,#297057,#297058,
#297059,#297060,#297061,#297062,#297063,#297064,#297065,#297066,#297067,
#297068,#297069,#297070,#297071,#297072,#297073,#297074,#297075,#297076,
#297077,#297078,#297079,#297080,#297081,#297082,#297083,#297084,#297085,
#297086,#297087,#297088,#297089,#297090,#297091,#297092,#297093,#297094,
#297095,#297096,#297097,#297098,#297099,#297100,#297101,#297102,#297103,
#297104,#297105,#297106,#297107,#297108,#297109,#297110,#297111,#297112,
#297113,#297114,#297115,#297116,#297117,#297118,#297119,#297120,#297121,
#297122,#297123,#297124,#297125,#297126,#297127,#297128,#297129,#297130,
#297131,#297132,#297133,#297134,#297135,#297136,#297137,#297138,#297139,
#297140,#297141,#297142,#297143,#297144,#297145,#297146,#297147,#297148,
#297149,#297150,#297151,#297152,#297153,#297154,#297155,#297156,#297157,
#297158,#297159,#297160,#297161,#297162,#297163,#297164,#297165,#297166,
#297167,#297168,#297169,#297170,#297171,#297172,#297173,#297174),
 .UNSPECIFIED.,.F.,.F.,(6,1,1,1,1,1,1,1,1,1,1,1,1,1,1,1,1,1,1,1,1,1,1,1,
1,1,1,1,1,1,1,1,1,1,1,1,1,1,1,1,1,1,1,1,1,1,1,1,1,1,1,1,1,1,1,1,1,1,1,1,
1,1,1,1,1,1,1,1,1,1,1,1,1,1,1,1,1,1,1,1,1,1,1,1,1,1,1,1,1,1,1,1,1,1,1,1,
1,1,1,1,1,1,1,1,1,1,1,1,1,1,1,1,1,1,1,1,1,1,1,1,1,1,1,1,1,1,1,1,1,1,1,1,
1,1,1,1,1,1,1,1,1,1,1,1,1,1,1,1,1,1,1,1,1,1,1,1,1,1,1,1,1,1,1,1,1,1,1,1,
1,1,1,1,1,1,1,1,1,1,1,1,1,1,1,1,1,1,1,1,1,1,1,1,1,1,1,1,1,1,1,1,1,1,1,1,
1,1,1,1,1,1,1,1,1,1,1,1,1,1,1,1,1,1,1,1,1,1,1,1,1,1,1,1,1,1,1,1,1,1,1,1,
1,1,1,1,1,1,1,1,1,1,1,1,1,1,1,1,1,1,1,1,1,1,1,1,1,1,1,1,1,1,1,1,1,1,1,1,
1,1,1,1,1,1,1,1,1,1,1,1,1,1,1,1,1,1,1,1,1,1,1,1,1,1,1,1,1,1,1,1,1,1,1,1,
1,1,1,1,1,1,1,1,1,1,1,1,1,1,1,1,1,1,1,1,1,1,1,1,1,1,1,1,1,1,1,1,1,1,1,1,
1,1,1,1,1,1,1,1,1,1,1,1,1,1,1,1,1,1,1,1,1,1,1,1,1,1,1,1,1,1,1,1,1,1,1,1,
1,1,1,1,1,1,1,1,1,1,1,1,1,1,1,1,1,1,1,1,1,1,1,1,1,1,1,1,1,1,1,1,1,1,1,1,
1,1,1,1,1,1,1,1,1,1,1,1,1,1,1,1,1,1,1,1,1,1,1,1,1,1,1,1,1,1,1,1,1,1,1,1,
1,1,1,1,1,1,1,1,1,1,6),(0.143172102,0.144954128,0.146788991,0.148623853,
0.150458716,0.152293578,0.15412844,0.155963303,0.157798165,0.159633028,
0.16146789,0.163302752,0.165137615,0.166972477,0.168807339,0.170642202,
0.172477064,0.174311927,0.176146789,0.177981651,0.179816514,0.181651376,
0.183486239,0.185321101,0.187155963,0.188990826,0.190825688,0.19266055,
0.194495413,0.196330275,0.198165138,0.2,0.201834862,0.203669725,0.205504587,
0.20733945,0.209174312,0.211009174,0.212844037,0.214678899,0.216513761,
0.218348624,0.220183486,0.222018349,0.223853211,0.225688073,0.227522936,
0.229357798,0.231192661,0.233027523,0.234862385,0.236697248,0.23853211,
0.240366972,0.242201835,0.244036697,0.24587156,0.247706422,0.249541284,
0.251376147,0.253211009,0.255045872,0.256880734,0.258715596,0.260550459,
0.262385321,0.264220183,0.266055046,0.267889908,0.269724771,0.271559633,
0.273394495,0.275229358,0.27706422,0.278899083,0.280733945,0.282568807,
0.28440367,0.286238532,0.288073394,0.289908257,0.291743119,0.293577982,
0.295412844,0.297247706,0.299082569,0.300917431,0.302752294,0.304587156,
0.306422018,0.308256881,0.310091743,0.311926606,0.313761468,0.31559633,
0.317431193,0.319266055,0.321100917,0.32293578,0.324770642,0.326605505,
0.328440367,0.330275229,0.332110092,0.333944954,0.335779817,0.337614679,
0.339449541,0.341284404,0.343119266,0.344954128,0.346788991,0.348623853,
0.350458716,0.352293578,0.35412844,0.355963303,0.357798165,0.359633028,
0.36146789,0.363302752,0.365137615,0.366972477,0.368807339,0.370642202,
0.372477064,0.374311927,0.376146789,0.377981651,0.379816514,0.381651376,
0.383486239,0.385321101,0.387155963,0.388990826,0.390825688,0.39266055,
0.394495413,0.396330275,0.398165138,0.4,0.401834862,0.403669725,0.405504587,
0.40733945,0.409174312,0.411009174,0.412844037,0.414678899,0.416513761,
0.418348624,0.420183486,0.422018349,0.423853211,0.425688073,0.427522936,
0.429357798,0.431192661,0.433027523,0.434862385,0.436697248,0.43853211,
0.440366972,0.442201835,0.444036697,0.44587156,0.447706422,0.449541284,
0.451376147,0.453211009,0.455045872,0.456880734,0.458715596,0.460550459,
0.462385321,0.464220183,0.466055046,0.467889908,0.469724771,0.471559633,
0.473394495,0.475229358,0.47706422,0.478899083,0.480733945,0.482568807,
0.48440367,0.486238532,0.488073394,0.489908257,0.491743119,0.493577982,
0.495412844,0.497247706,0.499082569,0.500917431,0.502752294,0.504587156,
0.506422018,0.508256881,0.511926606,0.513761468,0.51559633,0.517431193,
0.519266055,0.521100917,0.52293578,0.524770642,0.526605505,0.528440367,
0.530275229,0.532110092,0.533944954,0.535779817,0.537614679,0.539449541,
0.541284404,0.543119266,0.544954128,0.546788991,0.548623853,0.550458716,
0.552293578,0.55412844,0.555963303,0.557798165,0.559633028,0.56146789,0.563302752,
0.565137615,0.566972477,0.568807339,0.570642202,0.572477064,0.574311927,
0.576146789,0.577981651,0.579816514,0.581651376,0.583486239,0.585321101,
0.587155963,0.588990826,0.590825688,0.59266055,0.594495413,0.596330275,
0.598165138,0.6,0.601834862,0.603669725,0.605504587,0.60733945,0.609174312,
0.611009174,0.612844037,0.614678899,0.616513761,0.618348624,0.620183486,
0.622018349,0.623853211,0.625688073,0.627522936,0.629357798,0.631192661,
0.633027523,0.634862385,0.636697248,0.63853211,0.640366972,0.642201835,
0.644036697,0.64587156,0.647706422,0.649541284,0.651376147,0.653211009,
0.655045872,0.656880734,0.658715596,0.660550459,0.662385321,0.664220183,
0.666055046,0.667889908,0.669724771,0.671559633,0.673394495,0.675229358,
0.67706422,0.678899083,0.680733945,0.682568807,0.68440367,0.686238532,0.688073394,
0.689908257,0.691743119,0.693577982,0.695412844,0.697247706,0.699082569,
0.700917431,0.702752294,0.704587156,0.706422018,0.708256881,0.710091743,
0.711926606,0.713761468,0.71559633,0.717431193,0.719266055,0.721100917,
0.72293578,0.724770642,0.726605505,0.728440367,0.730275229,0.732110092,
0.733944954,0.735779817,0.737614679,0.739449541,0.741284404,0.743119266,
0.744954128,0.746788991,0.748623853,0.750458716,0.752293578,0.75412844,
0.755963303,0.757798165,0.759633028,0.76146789,0.763302752,0.765137615,
0.766972477,0.768807339,0.770642202,0.772477064,0.774311927,0.776146789,
0.777981651,0.779816514,0.781651376,0.783486239,0.785321101,0.787155963,
0.788990826,0.790825688,0.79266055,0.794495413,0.796330275,0.798165138,
0.8,0.801834862,0.803669725,0.805504587,0.80733945,0.809174312,0.811009174,
0.812844037,0.814678899,0.816513761,0.818348624,0.820183486,0.822018349,
0.823853211,0.825688073,0.827522936,0.829357798,0.831192661,0.833027523,
0.834862385,0.836697248,0.83853211,0.840366972,0.842201835,0.844036697,
0.84587156,0.847706422,0.849541284,0.851376147,0.853211009,0.855045872,
0.856880734,0.858715596,0.860550459,0.862385321,0.864220183,0.866055046,
0.867889908,0.869724771,0.871559633,0.873394495,0.875229358,0.87706422,
0.878899083,0.880733945,0.882568807,0.88440367,0.886238532,0.888073394,
0.889908257,0.891743119,0.893577982,0.895412844,0.897247706,0.899082569,
0.900917431,0.902752294,0.904587156,0.906422018,0.908256881,0.910091743,
0.911926606,0.913761468,0.91559633,0.917431193,0.919266055,0.921100917,
0.92293578,0.924770642,0.926605505,0.928440367,0.930275229,0.932110092,
0.933944954,0.935779817,0.937614679,0.939449541,0.941284404,0.943119266,
0.944954128,0.946788991,0.948623853,0.950458716,0.952293578,0.95412844,
0.955963303,0.957798165,0.959633028,0.96146789,0.963302752,0.965137615,
0.966972477,0.968807339,0.970642202,0.972477064,0.974311927,0.976146789,
0.977981651,0.979816514,0.981651376,0.983486239,0.985321101,0.987155963,
0.988990826,0.990825688,0.99266055,0.994495413,0.996330275,0.998165138,
1.),.UNSPECIFIED.);
#24492=B_SPLINE_CURVE_WITH_KNOTS('',3,(#297177,#297178,#297179,#297180,
#297181,#297182,#297183,#297184,#297185,#297186,#297187,#297188,#297189,
#297190,#297191,#297192,#297193,#297194,#297195,#297196,#297197,#297198,
#297199,#297200,#297201,#297202,#297203,#297204,#297205,#297206,#297207,
#297208,#297209,#297210,#297211,#297212,#297213,#297214,#297215,#297216,
#297217,#297218,#297219,#297220,#297221,#297222,#297223,#297224,#297225,
#297226,#297227,#297228,#297229,#297230,#297231,#297232,#297233,#297234,
#297235,#297236,#297237,#297238,#297239,#297240,#297241,#297242,#297243,
#297244,#297245,#297246,#297247,#297248,#297249,#297250,#297251,#297252,
#297253,#297254,#297255,#297256,#297257,#297258,#297259,#297260,#297261,
#297262,#297263,#297264,#297265,#297266,#297267,#297268,#297269,#297270,
#297271,#297272,#297273,#297274,#297275,#297276,#297277,#297278,#297279,
#297280,#297281,#297282,#297283,#297284,#297285,#297286,#297287,#297288,
#297289,#297290,#297291,#297292,#297293,#297294,#297295,#297296,#297297,
#297298,#297299,#297300,#297301,#297302,#297303,#297304,#297305,#297306,
#297307,#297308,#297309,#297310,#297311,#297312,#297313,#297314,#297315,
#297316,#297317,#297318,#297319,#297320,#297321,#297322,#297323,#297324,
#297325,#297326,#297327,#297328,#297329,#297330,#297331,#297332,#297333,
#297334,#297335,#297336,#297337,#297338,#297339,#297340,#297341,#297342,
#297343,#297344,#297345,#297346,#297347,#297348,#297349,#297350,#297351,
#297352,#297353,#297354,#297355,#297356,#297357,#297358,#297359,#297360,
#297361,#297362,#297363,#297364,#297365,#297366,#297367,#297368,#297369,
#297370,#297371,#297372,#297373,#297374,#297375,#297376,#297377,#297378,
#297379,#297380,#297381,#297382,#297383,#297384,#297385,#297386,#297387,
#297388,#297389,#297390,#297391,#297392,#297393,#297394,#297395,#297396,
#297397,#297398,#297399,#297400,#297401,#297402,#297403,#297404,#297405,
#297406,#297407,#297408,#297409,#297410,#297411,#297412,#297413,#297414,
#297415,#297416,#297417,#297418,#297419,#297420,#297421,#297422,#297423,
#297424,#297425,#297426,#297427,#297428,#297429,#297430,#297431,#297432,
#297433,#297434,#297435,#297436,#297437,#297438,#297439,#297440,#297441,
#297442,#297443,#297444,#297445,#297446,#297447,#297448,#297449,#297450,
#297451,#297452,#297453,#297454,#297455,#297456,#297457,#297458,#297459,
#297460,#297461,#297462,#297463,#297464,#297465,#297466,#297467,#297468,
#297469,#297470,#297471,#297472,#297473,#297474,#297475,#297476,#297477,
#297478,#297479,#297480,#297481,#297482,#297483,#297484,#297485,#297486,
#297487,#297488,#297489,#297490,#297491,#297492,#297493,#297494,#297495,
#297496,#297497,#297498),.UNSPECIFIED.,.F.,.F.,(4,3,3,3,3,3,3,3,3,3,3,3,
3,3,3,3,3,3,3,3,3,3,3,3,3,3,3,3,3,3,3,3,3,3,3,3,3,3,3,3,3,3,3,3,3,3,3,3,
3,3,3,3,3,3,3,3,3,3,3,3,3,3,3,3,3,3,3,3,3,3,3,3,3,3,3,3,3,3,3,3,3,3,3,3,
3,3,3,3,3,3,3,3,3,3,3,3,3,3,3,3,3,3,3,3,3,3,3,4),(0.143172102,0.15412844,
0.165137615,0.176146789,0.187155963,0.198165138,0.209174312,0.220183486,
0.231192661,0.242201835,0.253211009,0.264220183,0.275229358,0.286238532,
0.297247706,0.308256881,0.319266055,0.330275229,0.341284404,0.352293578,
0.366972477,0.377981651,0.388990826,0.398165138,0.40733945,0.416513761,
0.425688073,0.434862385,0.444036697,0.455045872,0.464220183,0.473394495,
0.48440367,0.493577982,0.502752294,0.511926606,0.52293578,0.532110092,0.539449541,
0.546788991,0.555963303,0.565137615,0.572477064,0.579816514,0.587155963,
0.594495413,0.601834862,0.611009174,0.618348624,0.625688073,0.633027523,
0.640366972,0.647706422,0.655045872,0.662385321,0.669724771,0.67706422,
0.68440367,0.691743119,0.699082569,0.706422018,0.713761468,0.721100917,
0.728440367,0.735779817,0.743119266,0.750458716,0.757798165,0.765137615,
0.774311927,0.783486239,0.790825688,0.798165138,0.805504587,0.812844037,
0.818348624,0.823853211,0.829357798,0.834862385,0.840366972,0.84587156,
0.851376147,0.856880734,0.862385321,0.867889908,0.873394495,0.878899083,
0.88440367,0.889908257,0.895412844,0.902752294,0.908256881,0.913761468,
0.919266055,0.928440367,0.933944954,0.939449541,0.944954128,0.950458716,
0.955963303,0.96146789,0.966972477,0.972477064,0.977981651,0.983486239,
0.988990826,0.994495413,1.),.UNSPECIFIED.);
#24493=B_SPLINE_CURVE_WITH_KNOTS('',5,(#298459,#298460,#298461,#298462,
#298463,#298464,#298465,#298466,#298467,#298468,#298469,#298470,#298471,
#298472,#298473,#298474,#298475,#298476,#298477,#298478,#298479,#298480,
#298481,#298482,#298483,#298484,#298485,#298486,#298487,#298488,#298489,
#298490,#298491,#298492,#298493,#298494,#298495,#298496,#298497,#298498,
#298499,#298500,#298501,#298502,#298503,#298504,#298505,#298506,#298507,
#298508,#298509,#298510,#298511,#298512,#298513,#298514,#298515,#298516,
#298517,#298518,#298519,#298520,#298521,#298522,#298523,#298524,#298525,
#298526,#298527,#298528,#298529,#298530,#298531,#298532,#298533,#298534,
#298535,#298536,#298537,#298538,#298539,#298540,#298541,#298542,#298543,
#298544,#298545,#298546,#298547,#298548,#298549,#298550,#298551,#298552,
#298553,#298554,#298555,#298556,#298557,#298558,#298559,#298560,#298561,
#298562,#298563,#298564,#298565,#298566,#298567,#298568,#298569,#298570,
#298571,#298572,#298573,#298574,#298575,#298576,#298577,#298578,#298579,
#298580,#298581,#298582,#298583,#298584,#298585,#298586,#298587,#298588,
#298589,#298590,#298591,#298592,#298593,#298594,#298595,#298596,#298597,
#298598,#298599,#298600,#298601,#298602,#298603,#298604,#298605,#298606,
#298607,#298608,#298609,#298610,#298611,#298612,#298613,#298614,#298615,
#298616,#298617,#298618,#298619,#298620,#298621,#298622,#298623,#298624,
#298625,#298626,#298627,#298628,#298629,#298630,#298631,#298632,#298633,
#298634,#298635,#298636,#298637,#298638,#298639,#298640,#298641,#298642,
#298643,#298644,#298645,#298646,#298647,#298648,#298649,#298650,#298651,
#298652,#298653,#298654,#298655,#298656,#298657,#298658,#298659,#298660,
#298661,#298662,#298663,#298664,#298665,#298666,#298667,#298668,#298669,
#298670,#298671,#298672,#298673,#298674,#298675,#298676,#298677,#298678,
#298679,#298680,#298681,#298682,#298683,#298684,#298685,#298686,#298687,
#298688,#298689,#298690,#298691,#298692,#298693,#298694,#298695,#298696,
#298697,#298698,#298699,#298700,#298701,#298702,#298703,#298704,#298705,
#298706,#298707,#298708,#298709,#298710,#298711,#298712,#298713,#298714,
#298715,#298716,#298717,#298718,#298719,#298720,#298721,#298722,#298723,
#298724,#298725,#298726,#298727,#298728,#298729,#298730,#298731,#298732,
#298733,#298734,#298735,#298736,#298737,#298738,#298739,#298740,#298741,
#298742,#298743,#298744,#298745,#298746,#298747,#298748,#298749,#298750,
#298751,#298752,#298753,#298754,#298755,#298756,#298757,#298758,#298759,
#298760,#298761,#298762,#298763,#298764,#298765,#298766,#298767,#298768,
#298769,#298770,#298771,#298772,#298773,#298774,#298775,#298776,#298777,
#298778,#298779,#298780,#298781,#298782,#298783,#298784,#298785,#298786,
#298787,#298788,#298789,#298790,#298791,#298792,#298793,#298794,#298795,
#298796,#298797,#298798,#298799,#298800,#298801,#298802,#298803,#298804,
#298805,#298806,#298807,#298808,#298809,#298810,#298811,#298812,#298813,
#298814,#298815,#298816,#298817,#298818,#298819,#298820,#298821,#298822,
#298823,#298824,#298825,#298826,#298827,#298828,#298829,#298830,#298831,
#298832,#298833,#298834,#298835,#298836,#298837,#298838,#298839,#298840,
#298841,#298842,#298843,#298844,#298845,#298846,#298847,#298848,#298849,
#298850,#298851,#298852,#298853,#298854,#298855,#298856,#298857,#298858,
#298859,#298860,#298861,#298862,#298863,#298864,#298865,#298866,#298867,
#298868,#298869,#298870,#298871,#298872,#298873,#298874,#298875,#298876,
#298877,#298878,#298879,#298880,#298881,#298882,#298883,#298884,#298885,
#298886,#298887,#298888,#298889,#298890,#298891,#298892,#298893,#298894,
#298895,#298896,#298897,#298898,#298899,#298900,#298901,#298902,#298903,
#298904,#298905,#298906,#298907,#298908,#298909,#298910,#298911,#298912,
#298913,#298914,#298915,#298916,#298917,#298918,#298919,#298920,#298921,
#298922,#298923,#298924,#298925,#298926,#298927,#298928,#298929),
 .UNSPECIFIED.,.F.,.F.,(6,1,1,1,1,1,1,1,1,1,1,1,1,1,1,1,1,1,1,1,1,1,1,1,
1,1,1,1,1,1,1,1,1,1,1,1,1,1,1,1,1,1,1,1,1,1,1,1,1,1,1,1,1,1,1,1,1,1,1,1,
1,1,1,1,1,1,1,1,1,1,1,1,1,1,1,1,1,1,1,1,1,1,1,1,1,1,1,1,1,1,1,1,1,1,1,1,
1,1,1,1,1,1,1,1,1,1,1,1,1,1,1,1,1,1,1,1,1,1,1,1,1,1,1,1,1,1,1,1,1,1,1,1,
1,1,1,1,1,1,1,1,1,1,1,1,1,1,1,1,1,1,1,1,1,1,1,1,1,1,1,1,1,1,1,1,1,1,1,1,
1,1,1,1,1,1,1,1,1,1,1,1,1,1,1,1,1,1,1,1,1,1,1,1,1,1,1,1,1,1,1,1,1,1,1,1,
1,1,1,1,1,1,1,1,1,1,1,1,1,1,1,1,1,1,1,1,1,1,1,1,1,1,1,1,1,1,1,1,1,1,1,1,
1,1,1,1,1,1,1,1,1,1,1,1,1,1,1,1,1,1,1,1,1,1,1,1,1,1,1,1,1,1,1,1,1,1,1,1,
1,1,1,1,1,1,1,1,1,1,1,1,1,1,1,1,1,1,1,1,1,1,1,1,1,1,1,1,1,1,1,1,1,1,1,1,
1,1,1,1,1,1,1,1,1,1,1,1,1,1,1,1,1,1,1,1,1,1,1,1,1,1,1,1,1,1,1,1,1,1,1,1,
1,1,1,1,1,1,1,1,1,1,1,1,1,1,1,1,1,1,1,1,1,1,1,1,1,1,1,1,1,1,1,1,1,1,1,1,
1,1,1,1,1,1,1,1,1,1,1,1,1,1,1,1,1,1,1,1,1,1,1,1,1,1,1,1,1,1,1,1,1,1,1,1,
1,1,1,1,1,1,1,1,1,1,1,1,1,1,1,1,1,1,1,1,1,1,1,1,1,1,1,1,1,1,1,1,1,1,1,1,
1,1,1,1,1,1,1,1,1,1,6),(-1.,-0.998165138,-0.996330275,-0.994495413,-0.99266055,
-0.990825688,-0.988990826,-0.987155963,-0.985321101,-0.983486239,-0.981651376,
-0.979816514,-0.977981651,-0.976146789,-0.974311927,-0.972477064,-0.970642202,
-0.968807339,-0.966972477,-0.965137615,-0.963302752,-0.96146789,-0.959633028,
-0.957798165,-0.955963303,-0.95412844,-0.952293578,-0.950458716,-0.948623853,
-0.946788991,-0.944954128,-0.943119266,-0.941284404,-0.939449541,-0.937614679,
-0.935779817,-0.933944954,-0.932110092,-0.930275229,-0.928440367,-0.926605505,
-0.924770642,-0.92293578,-0.921100917,-0.919266055,-0.917431193,-0.91559633,
-0.913761468,-0.911926606,-0.910091743,-0.908256881,-0.906422018,-0.904587156,
-0.902752294,-0.900917431,-0.899082569,-0.897247706,-0.895412844,-0.893577982,
-0.891743119,-0.889908257,-0.888073394,-0.886238532,-0.88440367,-0.882568807,
-0.880733945,-0.878899083,-0.87706422,-0.875229358,-0.873394495,-0.871559633,
-0.869724771,-0.867889908,-0.866055046,-0.864220183,-0.862385321,-0.860550459,
-0.858715596,-0.856880734,-0.855045872,-0.853211009,-0.851376147,-0.849541284,
-0.847706422,-0.84587156,-0.844036697,-0.842201835,-0.840366972,-0.83853211,
-0.836697248,-0.834862385,-0.833027523,-0.831192661,-0.829357798,-0.827522936,
-0.825688073,-0.823853211,-0.822018349,-0.820183486,-0.818348624,-0.816513761,
-0.814678899,-0.812844037,-0.811009174,-0.809174312,-0.80733945,-0.805504587,
-0.803669725,-0.801834862,-0.8,-0.798165138,-0.796330275,-0.794495413,-0.79266055,
-0.790825688,-0.788990826,-0.787155963,-0.785321101,-0.783486239,-0.781651376,
-0.779816514,-0.777981651,-0.776146789,-0.774311927,-0.772477064,-0.770642202,
-0.768807339,-0.766972477,-0.765137615,-0.763302752,-0.76146789,-0.759633028,
-0.757798165,-0.755963303,-0.75412844,-0.752293578,-0.750458716,-0.748623853,
-0.746788991,-0.744954128,-0.743119266,-0.741284404,-0.739449541,-0.737614679,
-0.735779817,-0.733944954,-0.732110092,-0.730275229,-0.728440367,-0.726605505,
-0.724770642,-0.72293578,-0.721100917,-0.719266055,-0.717431193,-0.71559633,
-0.713761468,-0.711926606,-0.710091743,-0.708256881,-0.706422018,-0.704587156,
-0.702752294,-0.700917431,-0.699082569,-0.697247706,-0.695412844,-0.693577982,
-0.691743119,-0.689908257,-0.688073394,-0.686238532,-0.68440367,-0.682568807,
-0.680733945,-0.678899083,-0.67706422,-0.675229358,-0.673394495,-0.671559633,
-0.669724771,-0.667889908,-0.666055046,-0.664220183,-0.662385321,-0.660550459,
-0.658715596,-0.656880734,-0.655045872,-0.653211009,-0.651376147,-0.649541284,
-0.647706422,-0.64587156,-0.644036697,-0.642201835,-0.640366972,-0.63853211,
-0.636697248,-0.634862385,-0.633027523,-0.631192661,-0.629357798,-0.627522936,
-0.625688073,-0.623853211,-0.622018349,-0.620183486,-0.618348624,-0.616513761,
-0.614678899,-0.612844037,-0.611009174,-0.609174312,-0.60733945,-0.605504587,
-0.603669725,-0.601834862,-0.6,-0.598165138,-0.596330275,-0.594495413,-0.59266055,
-0.590825688,-0.588990826,-0.587155963,-0.585321101,-0.583486239,-0.581651376,
-0.579816514,-0.577981651,-0.576146789,-0.574311927,-0.572477064,-0.570642202,
-0.568807339,-0.566972477,-0.565137615,-0.563302752,-0.56146789,-0.559633028,
-0.557798165,-0.555963303,-0.55412844,-0.552293578,-0.550458716,-0.548623853,
-0.546788991,-0.544954128,-0.543119266,-0.541284404,-0.539449541,-0.537614679,
-0.535779817,-0.533944954,-0.532110092,-0.530275229,-0.528440367,-0.526605505,
-0.524770642,-0.52293578,-0.521100917,-0.519266055,-0.517431193,-0.51559633,
-0.513761468,-0.511926606,-0.508256881,-0.506422018,-0.504587156,-0.502752294,
-0.500917431,-0.499082569,-0.497247706,-0.495412844,-0.493577982,-0.491743119,
-0.489908257,-0.488073394,-0.486238532,-0.48440367,-0.482568807,-0.480733945,
-0.478899083,-0.47706422,-0.475229358,-0.473394495,-0.471559633,-0.469724771,
-0.467889908,-0.466055046,-0.464220183,-0.462385321,-0.460550459,-0.458715596,
-0.456880734,-0.455045872,-0.453211009,-0.451376147,-0.449541284,-0.447706422,
-0.44587156,-0.444036697,-0.442201835,-0.440366972,-0.43853211,-0.436697248,
-0.434862385,-0.433027523,-0.431192661,-0.429357798,-0.427522936,-0.425688073,
-0.423853211,-0.422018349,-0.420183486,-0.418348624,-0.416513761,-0.414678899,
-0.412844037,-0.411009174,-0.409174312,-0.40733945,-0.405504587,-0.403669725,
-0.401834862,-0.4,-0.398165138,-0.396330275,-0.394495413,-0.39266055,-0.390825688,
-0.388990826,-0.387155963,-0.385321101,-0.383486239,-0.381651376,-0.379816514,
-0.377981651,-0.376146789,-0.374311927,-0.372477064,-0.370642202,-0.368807339,
-0.366972477,-0.365137615,-0.363302752,-0.36146789,-0.359633028,-0.357798165,
-0.355963303,-0.35412844,-0.352293578,-0.350458716,-0.348623853,-0.346788991,
-0.344954128,-0.343119266,-0.341284404,-0.339449541,-0.337614679,-0.335779817,
-0.333944954,-0.332110092,-0.330275229,-0.328440367,-0.326605505,-0.324770642,
-0.32293578,-0.321100917,-0.319266055,-0.317431193,-0.31559633,-0.313761468,
-0.311926606,-0.310091743,-0.308256881,-0.306422018,-0.304587156,-0.302752294,
-0.300917431,-0.299082569,-0.297247706,-0.295412844,-0.293577982,-0.291743119,
-0.289908257,-0.288073394,-0.286238532,-0.28440367,-0.282568807,-0.280733945,
-0.278899083,-0.27706422,-0.275229358,-0.273394495,-0.271559633,-0.269724771,
-0.267889908,-0.266055046,-0.264220183,-0.262385321,-0.260550459,-0.258715596,
-0.256880734,-0.255045872,-0.253211009,-0.251376147,-0.249541284,-0.247706422,
-0.24587156,-0.244036697,-0.242201835,-0.240366972,-0.23853211,-0.236697248,
-0.234862385,-0.233027523,-0.231192661,-0.229357798,-0.227522936,-0.225688073,
-0.223853211,-0.222018349,-0.220183486,-0.218348624,-0.216513761,-0.214678899,
-0.212844037,-0.211009174,-0.209174312,-0.20733945,-0.205504587,-0.203669725,
-0.201834862,-0.2,-0.198165138,-0.196330275,-0.194495413,-0.19266055,-0.190825688,
-0.188990826,-0.187155963,-0.185321101,-0.183486239,-0.181651376,-0.179816514,
-0.177981651,-0.176146789,-0.174311927,-0.172477064,-0.170642202,-0.168807339,
-0.166972477,-0.165137615,-0.163302752,-0.16146789,-0.159633028,-0.157798165,
-0.155963303,-0.15412844,-0.152293578,-0.150458716,-0.148623853,-0.146788991,
-0.144954128,-0.143172102),.UNSPECIFIED.);
#24494=B_SPLINE_CURVE_WITH_KNOTS('',3,(#299874,#299875,#299876,#299877,
#299878,#299879,#299880,#299881,#299882,#299883,#299884,#299885,#299886,
#299887,#299888,#299889,#299890,#299891,#299892,#299893,#299894,#299895,
#299896,#299897,#299898,#299899,#299900,#299901,#299902,#299903,#299904,
#299905,#299906,#299907,#299908,#299909,#299910,#299911,#299912,#299913,
#299914,#299915,#299916,#299917,#299918,#299919,#299920,#299921,#299922,
#299923,#299924,#299925,#299926,#299927,#299928,#299929,#299930,#299931,
#299932,#299933,#299934,#299935,#299936,#299937,#299938,#299939,#299940,
#299941,#299942,#299943,#299944,#299945,#299946,#299947,#299948,#299949,
#299950,#299951,#299952,#299953,#299954,#299955,#299956,#299957,#299958,
#299959,#299960,#299961,#299962,#299963,#299964,#299965,#299966,#299967,
#299968,#299969,#299970,#299971,#299972,#299973,#299974,#299975,#299976,
#299977,#299978,#299979,#299980,#299981,#299982,#299983,#299984,#299985,
#299986,#299987,#299988,#299989,#299990,#299991,#299992,#299993,#299994,
#299995,#299996,#299997,#299998,#299999,#300000,#300001,#300002,#300003,
#300004,#300005,#300006,#300007,#300008,#300009,#300010,#300011,#300012,
#300013,#300014,#300015,#300016,#300017,#300018,#300019,#300020,#300021,
#300022,#300023,#300024,#300025,#300026,#300027,#300028,#300029,#300030,
#300031,#300032,#300033,#300034,#300035,#300036,#300037,#300038,#300039,
#300040,#300041,#300042,#300043,#300044,#300045,#300046,#300047,#300048,
#300049,#300050,#300051,#300052,#300053,#300054,#300055,#300056,#300057,
#300058,#300059,#300060,#300061,#300062,#300063,#300064,#300065,#300066,
#300067,#300068,#300069,#300070,#300071,#300072,#300073,#300074,#300075,
#300076,#300077,#300078,#300079,#300080,#300081,#300082,#300083,#300084,
#300085,#300086,#300087,#300088,#300089,#300090,#300091,#300092,#300093,
#300094,#300095,#300096,#300097,#300098,#300099,#300100,#300101,#300102,
#300103,#300104,#300105,#300106,#300107,#300108,#300109,#300110,#300111,
#300112,#300113,#300114,#300115,#300116,#300117,#300118,#300119,#300120,
#300121,#300122,#300123,#300124,#300125,#300126,#300127,#300128,#300129,
#300130,#300131,#300132,#300133,#300134,#300135,#300136,#300137,#300138,
#300139,#300140,#300141,#300142,#300143,#300144,#300145,#300146,#300147,
#300148,#300149,#300150,#300151,#300152,#300153,#300154,#300155,#300156,
#300157,#300158,#300159,#300160,#300161,#300162,#300163,#300164,#300165,
#300166,#300167,#300168,#300169,#300170,#300171,#300172,#300173,#300174,
#300175,#300176,#300177,#300178,#300179,#300180,#300181,#300182,#300183,
#300184,#300185,#300186,#300187,#300188,#300189,#300190,#300191,#300192,
#300193,#300194,#300195),.UNSPECIFIED.,.F.,.F.,(4,3,3,3,3,3,3,3,3,3,3,3,
3,3,3,3,3,3,3,3,3,3,3,3,3,3,3,3,3,3,3,3,3,3,3,3,3,3,3,3,3,3,3,3,3,3,3,3,
3,3,3,3,3,3,3,3,3,3,3,3,3,3,3,3,3,3,3,3,3,3,3,3,3,3,3,3,3,3,3,3,3,3,3,3,
3,3,3,3,3,3,3,3,3,3,3,3,3,3,3,3,3,3,3,3,3,3,3,4),(0.143172102,0.15412844,
0.165137615,0.176146789,0.187155963,0.198165138,0.209174312,0.220183486,
0.231192661,0.242201835,0.253211009,0.264220183,0.275229358,0.286238532,
0.297247706,0.308256881,0.319266055,0.330275229,0.341284404,0.352293578,
0.363302752,0.374311927,0.385321101,0.396330275,0.405504587,0.414678899,
0.423853211,0.433027523,0.442201835,0.451376147,0.460550459,0.471559633,
0.480733945,0.489908257,0.499082569,0.508256881,0.517431193,0.526605505,
0.533944954,0.541284404,0.550458716,0.557798165,0.565137615,0.572477064,
0.579816514,0.587155963,0.594495413,0.601834862,0.609174312,0.616513761,
0.623853211,0.631192661,0.63853211,0.64587156,0.653211009,0.660550459,0.667889908,
0.675229358,0.682568807,0.689908257,0.697247706,0.706422018,0.713761468,
0.72293578,0.733944954,0.741284404,0.748623853,0.755963303,0.763302752,
0.770642202,0.777981651,0.785321101,0.79266055,0.8,0.80733945,0.812844037,
0.818348624,0.823853211,0.829357798,0.834862385,0.842201835,0.847706422,
0.853211009,0.858715596,0.864220183,0.869724771,0.875229358,0.880733945,
0.886238532,0.891743119,0.897247706,0.902752294,0.908256881,0.913761468,
0.921100917,0.928440367,0.933944954,0.939449541,0.944954128,0.950458716,
0.955963303,0.96146789,0.966972477,0.972477064,0.979816514,0.985321101,
0.990825688,1.),.UNSPECIFIED.);
#24495=B_SPLINE_CURVE_WITH_KNOTS('',3,(#300224,#300225,#300226,#300227,
#300228,#300229,#300230,#300231,#300232,#300233,#300234,#300235,#300236,
#300237),.UNSPECIFIED.,.F.,.F.,(4,2,2,2,2,2,4),(2.25701232429112E-11,0.00014460912609736,
0.000387015548692996,0.00125700195661841,0.00435168228607041,0.0129718164294565,
0.0227694264116158),.UNSPECIFIED.);
#24496=B_SPLINE_CURVE_WITH_KNOTS('',3,(#300241,#300242,#300243,#300244,
#300245,#300246,#300247,#300248,#300249,#300250,#300251,#300252,#300253,
#300254,#300255,#300256,#300257,#300258,#300259,#300260,#300261,#300262,
#300263,#300264,#300265,#300266,#300267,#300268,#300269,#300270,#300271,
#300272,#300273,#300274,#300275,#300276,#300277,#300278,#300279,#300280,
#300281,#300282,#300283),.UNSPECIFIED.,.F.,.F.,(4,3,3,3,3,3,3,3,3,3,3,3,
3,3,4),(0.,9.41174796889181E-5,0.000189798325007615,0.000281495822455474,
0.000370505462955499,0.000455579152157681,0.000536999972207846,0.000612533789895692,
0.000685472418224339,0.000755118709112169,0.000789941854556085,0.000807353427278042,
0.000816059213639021,0.000822483140370077,0.000824765),.UNSPECIFIED.);
#24497=B_SPLINE_CURVE_WITH_KNOTS('',3,(#300291,#300292,#300293,#300294,
#300295,#300296,#300297,#300298,#300299,#300300,#300301,#300302,#300303,
#300304,#300305,#300306),.UNSPECIFIED.,.F.,.F.,(4,2,2,2,2,2,2,4),(7.39439642544424E-11,
8.13967315243824E-5,0.000253968783894778,0.000853738707014911,0.00300176120327824,
0.0106434682371973,0.0317998204262259,0.0557341748263668),.UNSPECIFIED.);
#24498=B_SPLINE_CURVE_WITH_KNOTS('',3,(#300310,#300311,#300312,#300313,
#300314,#300315,#300316,#300317,#300318,#300319,#300320,#300321,#300322,
#300323,#300324,#300325,#300326,#300327,#300328,#300329,#300330,#300331,
#300332,#300333,#300334,#300335,#300336,#300337,#300338,#300339,#300340,
#300341,#300342,#300343,#300344,#300345,#300346,#300347,#300348,#300349,
#300350,#300351,#300352,#300353,#300354,#300355),.UNSPECIFIED.,.F.,.F.,
(4,3,3,3,3,3,3,3,3,3,3,3,3,3,3,4),(0.,4.941415498036E-5,0.000146434010607815,
0.000239410220049695,0.000329337302265598,0.000416482292794944,0.00049829791801492,
0.00058011668851119,0.000653699456822933,0.000724251506183855,0.000774912253091927,
0.000800242626545964,0.000812907813272982,0.000820432326079254,0.000824400885159964,
0.000825573),.UNSPECIFIED.);
#24499=B_SPLINE_CURVE_WITH_KNOTS('',3,(#300363,#300364,#300365,#300366,
#300367,#300368,#300369,#300370,#300371,#300372,#300373,#300374,#300375,
#300376,#300377,#300378),.UNSPECIFIED.,.F.,.F.,(4,2,2,2,2,2,2,4),(2.13294581190719E-11,
8.13972158757993E-5,0.000254130774603711,0.00085480314270949,0.00300872290067678,
0.0106706763397779,0.0320130172357565,0.0562945640523578),.UNSPECIFIED.);
#24500=B_SPLINE_CURVE_WITH_KNOTS('',3,(#300382,#300383,#300384,#300385,
#300386,#300387,#300388,#300389,#300390,#300391,#300392,#300393,#300394,
#300395,#300396,#300397,#300398,#300399,#300400,#300401,#300402,#300403,
#300404,#300405,#300406,#300407,#300408,#300409,#300410,#300411,#300412,
#300413,#300414,#300415,#300416,#300417,#300418,#300419,#300420,#300421,
#300422,#300423,#300424,#300425,#300426,#300427),.UNSPECIFIED.,.F.,.F.,
(4,3,3,3,3,3,3,3,3,3,3,3,3,3,3,4),(0.,5.42807591518338E-5,0.000150811400407988,
0.000244155385409474,0.000333984770718417,0.000420334676603205,0.000503129576977275,
0.000583740432732957,0.000657800501529321,0.000728470586106261,0.000777021793053131,
0.000801297396526565,0.000813435198263283,0.000820820805650379,0.000824774446497117,
0.000825573),.UNSPECIFIED.);
#24501=B_SPLINE_CURVE_WITH_KNOTS('',3,(#300435,#300436,#300437,#300438,
#300439,#300440,#300441,#300442,#300443,#300444,#300445,#300446,#300447,
#300448,#300449,#300450),.UNSPECIFIED.,.F.,.F.,(4,2,2,2,2,2,2,4),(6.59801867899649E-11,
8.13970156620257E-5,0.000253894448343603,0.000852930654053306,0.00300001860986496,
0.0106403949523925,0.0318561104701801,0.055916116834572),.UNSPECIFIED.);
#24502=B_SPLINE_CURVE_WITH_KNOTS('',3,(#300454,#300455,#300456,#300457,
#300458,#300459,#300460,#300461,#300462,#300463,#300464,#300465,#300466,
#300467,#300468,#300469,#300470,#300471,#300472,#300473,#300474,#300475,
#300476,#300477,#300478,#300479,#300480,#300481,#300482,#300483,#300484,
#300485,#300486,#300487,#300488,#300489,#300490,#300491,#300492,#300493,
#300494,#300495,#300496,#300497,#300498,#300499),.UNSPECIFIED.,.F.,.F.,
(4,3,3,3,3,3,3,3,3,3,3,3,3,3,3,4),(0.,5.29278932285465E-5,0.000149986829614398,
0.000243421723444812,0.000333607658851719,0.000420839426742773,0.000504993867908082,
0.000585138650931061,0.000659165774865394,0.000730100379889144,0.000777836689944572,
0.000801704844972286,0.000813638922486143,0.000820965828956536,0.000825017897538137,
0.000825573),.UNSPECIFIED.);
#24503=B_SPLINE_CURVE_WITH_KNOTS('',3,(#300507,#300508,#300509,#300510,
#300511,#300512,#300513,#300514,#300515,#300516,#300517,#300518,#300519,
#300520),.UNSPECIFIED.,.F.,.F.,(4,2,2,2,2,2,4),(0.,5.18053291669203E-5,
0.000134730876905741,0.000431948787567479,0.0014896022211569,0.00442861890037952,
0.00776247261062754),.UNSPECIFIED.);
#24504=B_SPLINE_CURVE_WITH_KNOTS('',3,(#300524,#300525,#300526,#300527,
#300528,#300529,#300530,#300531,#300532,#300533,#300534,#300535,#300536,
#300537,#300538,#300539,#300540,#300541,#300542,#300543,#300544,#300545,
#300546,#300547,#300548,#300549,#300550,#300551,#300552,#300553,#300554,
#300555,#300556,#300557,#300558,#300559,#300560,#300561,#300562,#300563,
#300564,#300565,#300566),.UNSPECIFIED.,.F.,.F.,(4,3,3,3,3,3,3,3,3,3,3,3,
3,3,4),(0.,6.51902922437498E-5,0.000162212835330501,0.000255542669811936,
0.00034594997855667,0.000431821393210348,0.000515057799381166,0.000592686599535874,
0.000666391521959597,0.000737527223809127,0.000781550111904564,0.000803561555952282,
0.000814567277976141,0.000821645382533787,0.000825573),.UNSPECIFIED.);
#24505=B_SPLINE_CURVE_WITH_KNOTS('',3,(#300574,#300575,#300576,#300577,
#300578,#300579,#300580,#300581,#300582,#300583,#300584,#300585,#300586,
#300587,#300588,#300589),.UNSPECIFIED.,.F.,.F.,(4,2,2,2,2,2,2,4),(3.51269554446888E-11,
8.1397365043496E-5,0.000254102099395071,0.000854503471652061,0.00300783666884981,
0.0106666072947153,0.03195064404952,0.0561014629629725),.UNSPECIFIED.);
#24506=B_SPLINE_CURVE_WITH_KNOTS('',3,(#300593,#300594,#300595,#300596,
#300597,#300598,#300599,#300600,#300601,#300602,#300603,#300604,#300605,
#300606,#300607,#300608),.UNSPECIFIED.,.F.,.F.,(4,2,2,2,2,2,2,4),(0.,0.0414356907890881,
0.078170361387943,0.0913935848277746,0.0950979482415805,0.0961248369214223,
0.0964175430082423,0.0964926788806888),.UNSPECIFIED.);
#24507=B_SPLINE_CURVE_WITH_KNOTS('',3,(#300616,#300617,#300618,#300619,
#300620,#300621,#300622,#300623,#300624,#300625,#300626,#300627,#300628,
#300629,#300630,#300631),.UNSPECIFIED.,.F.,.F.,(4,2,2,2,2,2,2,4),(0.,8.13972245530873E-5,
0.00025378453400524,0.000851890925250522,0.00299507223923743,0.0106160714793745,
0.0318434026249517,0.0559770818334918),.UNSPECIFIED.);
#24508=B_SPLINE_CURVE_WITH_KNOTS('',3,(#300635,#300636,#300637,#300638,
#300639,#300640,#300641,#300642,#300643,#300644,#300645,#300646,#300647,
#300648,#300649,#300650,#300651,#300652,#300653,#300654,#300655,#300656,
#300657,#300658,#300659,#300660,#300661,#300662,#300663,#300664,#300665,
#300666,#300667,#300668,#300669,#300670,#300671,#300672,#300673,#300674,
#300675,#300676,#300677,#300678,#300679,#300680),.UNSPECIFIED.,.F.,.F.,
(4,3,3,3,3,3,3,3,3,3,3,3,3,3,3,4),(0.,5.66433572362371E-5,0.000153093585172818,
0.000245871068686411,0.000336099718589312,0.000423313353825591,0.000506253798565061,
0.000586083598923796,0.000659559573703011,0.000729754691205078,0.000777663845602539,
0.00080161842280127,0.000813595711400635,0.000820938523245592,0.000824948241415582,
0.000825573),.UNSPECIFIED.);
#24509=B_SPLINE_CURVE_WITH_KNOTS('',3,(#300688,#300689,#300690,#300691,
#300692,#300693,#300694,#300695,#300696,#300697,#300698,#300699,#300700,
#300701,#300702,#300703),.UNSPECIFIED.,.F.,.F.,(4,2,2,2,2,2,2,4),(2.38027376745489E-11,
8.13970695358414E-5,0.000253842437580032,0.00085198275120837,0.00299535207411838,
0.0106223872937026,0.0317449404823533,0.0556503449296871),.UNSPECIFIED.);
#24510=B_SPLINE_CURVE_WITH_KNOTS('',3,(#300707,#300708,#300709,#300710,
#300711,#300712,#300713,#300714,#300715,#300716),.UNSPECIFIED.,.F.,.F.,
(4,2,2,2,4),(0.,0.0415132221635862,0.0782472088689811,0.0914322683673314,
0.100763837421976),.UNSPECIFIED.);
#24511=B_SPLINE_CURVE_WITH_KNOTS('',3,(#300724,#300725,#300726,#300727,
#300728,#300729,#300730,#300731,#300732,#300733,#300734,#300735,#300736,
#300737,#300738,#300739),.UNSPECIFIED.,.F.,.F.,(4,2,2,2,2,2,2,4),(2.53031513835136E-11,
8.13974294458811E-5,0.000254077418613046,0.000853925999930095,0.00300624123794232,
0.0106626452969989,0.0319062118029417,0.0559886272275276),.UNSPECIFIED.);
#24512=B_SPLINE_CURVE_WITH_KNOTS('',3,(#300743,#300744,#300745,#300746,
#300747,#300748,#300749,#300750,#300751,#300752,#300753,#300754,#300755,
#300756,#300757,#300758,#300759,#300760,#300761,#300762,#300763,#300764,
#300765,#300766,#300767,#300768,#300769,#300770,#300771,#300772,#300773,
#300774,#300775,#300776,#300777,#300778,#300779,#300780,#300781,#300782,
#300783,#300784,#300785),.UNSPECIFIED.,.F.,.F.,(4,3,3,3,3,3,3,3,3,3,3,3,
3,3,4),(0.,5.2655145774557E-5,0.000149453317664655,0.00024236950728625,
0.00033244565288107,0.000419142399915971,0.000502353712462079,0.00058294328434656,
0.000656613938861597,0.000727097094331266,0.000775904547165633,0.000800308273582816,
0.000812510136791408,0.000820061384306642,0.000824712),.UNSPECIFIED.);
#24513=B_SPLINE_CURVE_WITH_KNOTS('',3,(#300793,#300794,#300795,#300796,
#300797,#300798,#300799,#300800,#300801,#300802,#300803,#300804,#300805,
#300806,#300807,#300808),.UNSPECIFIED.,.F.,.F.,(4,2,2,2,2,2,2,4),(0.,8.13968219775296E-5,
0.000253912214223537,0.000852767064929133,0.00299685323830034,0.0106260266679204,
0.0318487307217364,0.0559555570626083),.UNSPECIFIED.);
#24514=B_SPLINE_CURVE_WITH_KNOTS('',3,(#300812,#300813,#300814,#300815,
#300816,#300817,#300818,#300819,#300820,#300821,#300822,#300823,#300824,
#300825,#300826,#300827,#300828,#300829,#300830,#300831,#300832,#300833,
#300834,#300835,#300836,#300837,#300838,#300839,#300840,#300841,#300842,
#300843,#300844,#300845,#300846,#300847,#300848,#300849,#300850,#300851,
#300852,#300853,#300854),.UNSPECIFIED.,.F.,.F.,(4,3,3,3,3,3,3,3,3,3,3,3,
3,3,4),(0.,7.64101055378754E-5,0.000172695683197778,0.000265061951152557,
0.000354046629123992,0.000439529472553468,0.000521166539457513,0.000597300157860763,
0.000670487364037656,0.000740507990601729,0.000782608495300864,0.000803658747650432,
0.000814183873825216,0.000821298407202764,0.000824709),.UNSPECIFIED.);
#24515=B_SPLINE_CURVE_WITH_KNOTS('',3,(#300862,#300863,#300864,#300865,
#300866,#300867,#300868,#300869,#300870,#300871,#300872,#300873,#300874,
#300875,#300876,#300877),.UNSPECIFIED.,.F.,.F.,(4,2,2,2,2,2,2,4),(1.23364205350419E-12,
8.13969099647976E-5,0.000253632227414641,0.00085030471521368,0.00299164645435722,
0.0106059199915171,0.0317135536556019,0.0556224300991424),.UNSPECIFIED.);
#24516=B_SPLINE_CURVE_WITH_KNOTS('',3,(#300881,#300882,#300883,#300884,
#300885,#300886,#300887,#300888,#300889,#300890,#300891,#300892,#300893,
#300894,#300895,#300896),.UNSPECIFIED.,.F.,.F.,(4,2,2,2,2,2,2,4),(0.,0.0414635861754931,
0.0780958470122907,0.0912237647252485,0.0949045241674999,0.0959245951421665,
0.0962158581650039,0.0962727721750899),.UNSPECIFIED.);
#24517=B_SPLINE_CURVE_WITH_KNOTS('',3,(#300904,#300905,#300906,#300907,
#300908,#300909,#300910,#300911,#300912,#300913,#300914,#300915,#300916,
#300917,#300918,#300919),.UNSPECIFIED.,.F.,.F.,(4,2,2,2,2,2,2,4),(0.,8.13968331260338E-5,
0.000253734977402965,0.000851565104860571,0.00299597558175975,0.0106208094079658,
0.0318922880572177,0.0561185877997889),.UNSPECIFIED.);
#24518=B_SPLINE_CURVE_WITH_KNOTS('',3,(#300923,#300924,#300925,#300926,
#300927,#300928,#300929,#300930,#300931,#300932,#300933,#300934,#300935,
#300936,#300937,#300938,#300939,#300940,#300941,#300942,#300943,#300944,
#300945,#300946,#300947,#300948,#300949,#300950,#300951,#300952,#300953,
#300954,#300955,#300956,#300957,#300958,#300959,#300960,#300961,#300962,
#300963,#300964,#300965),.UNSPECIFIED.,.F.,.F.,(4,3,3,3,3,3,3,3,3,3,3,3,
3,3,4),(0.,7.71827982783351E-5,0.000173267568397164,0.000265457127481624,
0.0003540795695718,0.000439673818397658,0.000522355464935158,0.000598683552368119,
0.0006716060037561,0.000741338134319915,0.000783024567159957,0.000803867783579979,
0.000814289391789989,0.000821380251972883,0.000824711),.UNSPECIFIED.);
#24519=B_SPLINE_CURVE_WITH_KNOTS('',3,(#300973,#300974,#300975,#300976,
#300977,#300978,#300979,#300980,#300981,#300982,#300983,#300984,#300985,
#300986,#300987,#300988),.UNSPECIFIED.,.F.,.F.,(4,2,2,2,2,2,2,4),(1.6950339357606E-6,
8.82509104672641E-5,0.000704155174850886,0.00283747057980027,0.0104852329216673,
0.0376789761788421,0.11313592873392,0.19853018900161),.UNSPECIFIED.);
#24520=B_SPLINE_CURVE_WITH_KNOTS('',3,(#300992,#300993,#300994,#300995,
#300996,#300997,#300998,#300999,#301000,#301001,#301002,#301003,#301004,
#301005,#301006,#301007),.UNSPECIFIED.,.F.,.F.,(4,2,2,2,2,2,2,4),(0.,0.0413890254871353,
0.0780848812299061,0.0912986210594108,0.0950019425466635,0.0960280210265948,
0.0963205431802688,0.0964550788246295),.UNSPECIFIED.);
#24521=B_SPLINE_CURVE_WITH_KNOTS('',3,(#301015,#301016,#301017,#301018,
#301019,#301020,#301021,#301022,#301023,#301024,#301025,#301026,#301027,
#301028,#301029,#301030),.UNSPECIFIED.,.F.,.F.,(4,2,2,2,2,2,2,4),(7.86880354660446E-11,
8.13969307468172E-5,0.000254285399398094,0.000856228019329295,0.00301522849587095,
0.0106963537451455,0.0320464903672051,0.0562777029252997),.UNSPECIFIED.);
#24522=B_SPLINE_CURVE_WITH_KNOTS('',3,(#301034,#301035,#301036,#301037,
#301038,#301039,#301040,#301041,#301042,#301043,#301044,#301045,#301046,
#301047,#301048,#301049,#301050,#301051,#301052,#301053,#301054,#301055,
#301056,#301057,#301058,#301059,#301060,#301061,#301062,#301063,#301064,
#301065,#301066,#301067,#301068,#301069,#301070,#301071,#301072,#301073,
#301074,#301075,#301076),.UNSPECIFIED.,.F.,.F.,(4,3,3,3,3,3,3,3,3,3,3,3,
3,3,4),(0.,6.16345978401115E-5,0.000157957361618997,0.000250880688269924,
0.000340624421210286,0.000427077761505101,0.000509302370494405,0.000588154777870804,
0.000661875915878424,0.000732225403571121,0.00077846870178556,0.00080159035089278,
0.00081315117544639,0.000820521674856106,0.000824712),.UNSPECIFIED.);
#24523=B_SPLINE_CURVE_WITH_KNOTS('',3,(#301084,#301085,#301086,#301087,
#301088,#301089,#301090,#301091,#301092,#301093,#301094,#301095,#301096,
#301097,#301098,#301099),.UNSPECIFIED.,.F.,.F.,(4,2,2,2,2,2,2,4),(1.62974308173078E-11,
8.13975100572819E-5,0.000253856508698745,0.000852553741698134,0.0030001595828361,
0.0106431662956009,0.0318223136662569,0.0558016233755454),.UNSPECIFIED.);
#24524=B_SPLINE_CURVE_WITH_KNOTS('',3,(#301103,#301104,#301105,#301106,
#301107,#301108,#301109,#301110,#301111,#301112,#301113,#301114,#301115,
#301116,#301117,#301118,#301119,#301120,#301121,#301122,#301123,#301124,
#301125,#301126,#301127,#301128,#301129,#301130,#301131,#301132,#301133,
#301134,#301135,#301136,#301137,#301138,#301139,#301140,#301141,#301142,
#301143,#301144,#301145),.UNSPECIFIED.,.F.,.F.,(4,3,3,3,3,3,3,3,3,3,3,3,
3,3,4),(0.,6.92664471239441E-5,0.000165721395816546,0.000258076923380911,
0.000348102201228441,0.000435018589131858,0.000517171174703187,0.000594273881027391,
0.000667353678705221,0.000738000738388034,0.000781791369194017,0.000803686684597008,
0.000814634342298504,0.000821856532347001,0.000825582),.UNSPECIFIED.);
#24525=B_SPLINE_CURVE_WITH_KNOTS('',3,(#301153,#301154,#301155,#301156,
#301157,#301158,#301159,#301160,#301161,#301162,#301163,#301164,#301165,
#301166),.UNSPECIFIED.,.F.,.F.,(4,2,2,2,2,2,4),(0.,5.18051394548469E-5,
0.000128367922845272,0.000402522208456775,0.00137771990788599,0.00408898979740982,
0.00716687083262862),.UNSPECIFIED.);
#24526=B_SPLINE_CURVE_WITH_KNOTS('',3,(#301170,#301171,#301172,#301173,
#301174,#301175,#301176,#301177,#301178,#301179,#301180,#301181,#301182,
#301183,#301184,#301185,#301186,#301187,#301188,#301189,#301190,#301191,
#301192,#301193,#301194,#301195,#301196,#301197,#301198,#301199,#301200,
#301201,#301202,#301203,#301204,#301205,#301206,#301207,#301208,#301209,
#301210,#301211,#301212),.UNSPECIFIED.,.F.,.F.,(4,3,3,3,3,3,3,3,3,3,3,3,
3,3,4),(0.,5.58746352433121E-5,0.000152354364357929,0.000245709469640099,
0.000335378676716353,0.000422057938872853,0.000505266205972759,0.00058512740447957,
0.000658497474695901,0.000728864330876048,0.000776787665438024,0.000800749332719012,
0.000812730166359506,0.000820221726102288,0.000824711),.UNSPECIFIED.);
#24527=B_SPLINE_CURVE_WITH_KNOTS('',3,(#301220,#301221,#301222,#301223,
#301224,#301225,#301226,#301227,#301228,#301229,#301230,#301231,#301232,
#301233,#301234,#301235),.UNSPECIFIED.,.F.,.F.,(4,2,2,2,2,2,2,4),(0.,8.14316271732823E-5,
0.000254019368615236,0.000852992249264539,0.00300118055688404,0.0106403867837904,
0.0318742301277796,0.055957326667169),.UNSPECIFIED.);
#24528=B_SPLINE_CURVE_WITH_KNOTS('',3,(#301238,#301239,#301240,#301241,
#301242,#301243,#301244,#301245,#301246,#301247,#301248,#301249,#301250,
#301251,#301252,#301253,#301254,#301255,#301256,#301257,#301258,#301259,
#301260,#301261,#301262,#301263,#301264,#301265,#301266,#301267,#301268,
#301269,#301270,#301271,#301272,#301273,#301274,#301275,#301276,#301277,
#301278,#301279,#301280),.UNSPECIFIED.,.F.,.F.,(4,3,3,3,3,3,3,3,3,3,3,3,
3,3,4),(0.,5.65234098039017E-5,0.000152655733578414,0.000245589277354889,
0.000335372303709341,0.000421703798891314,0.000505835941831361,0.000585772456373521,
0.000659530275651245,0.000729462549350524,0.000777522274675262,0.000801552137337631,
0.000813567068668815,0.000821068664650334,0.000825582),.UNSPECIFIED.);
#24529=B_SPLINE_CURVE_WITH_KNOTS('',3,(#302948,#302949,#302950,#302951,
#302952,#302953,#302954,#302955),.UNSPECIFIED.,.F.,.F.,(4,2,2,4),(-0.0072109809393628,
-0.00368662560464412,-5.07022257993201E-5,0.),.UNSPECIFIED.);
#24530=B_SPLINE_CURVE_WITH_KNOTS('',3,(#304623,#304624,#304625,#304626,
#304627,#304628,#304629,#304630),.UNSPECIFIED.,.F.,.F.,(4,2,2,4),(-0.132132384477265,
-0.103054333069165,-0.0714351436644779,0.),.UNSPECIFIED.);
#24531=B_SPLINE_CURVE_WITH_KNOTS('',3,(#306287,#306288,#306289,#306290,
#306291,#306292,#306293,#306294),.UNSPECIFIED.,.F.,.F.,(4,2,2,4),(-0.00667991057808912,
-0.00369121128660005,-5.07020425170668E-5,0.),.UNSPECIFIED.);
#24532=B_SPLINE_CURVE_WITH_KNOTS('',3,(#307962,#307963,#307964,#307965,
#307966,#307967,#307968,#307969,#307970,#307971,#307972,#307973),
 .UNSPECIFIED.,.F.,.F.,(4,2,2,2,2,4),(-0.14481831420152,-0.141838119346234,
-0.137576959447593,-0.122254984206309,-0.0793476321617013,0.),
 .UNSPECIFIED.);
#24533=B_SPLINE_CURVE_WITH_KNOTS('',3,(#309630,#309631,#309632,#309633,
#309634,#309635,#309636,#309637),.UNSPECIFIED.,.F.,.F.,(4,2,2,4),(-0.00705981267369703,
-0.00371696437757226,-5.07022406769822E-5,0.),.UNSPECIFIED.);
#24534=B_SPLINE_CURVE_WITH_KNOTS('',3,(#311302,#311303,#311304,#311305,
#311306,#311307,#311308,#311309,#311310,#311311,#311312,#311313),
 .UNSPECIFIED.,.F.,.F.,(4,2,2,2,2,4),(-0.141987502057799,-0.138780518129329,
-0.134636509194115,-0.119855977748107,-0.0784036114991811,0.),
 .UNSPECIFIED.);
#24535=B_SPLINE_CURVE_WITH_KNOTS('',3,(#312970,#312971,#312972,#312973,
#312974,#312975,#312976,#312977),.UNSPECIFIED.,.F.,.F.,(4,2,2,4),(-0.00741228757948683,
-0.0037123551597383,-5.07021491017289E-5,0.),.UNSPECIFIED.);
#24536=B_SPLINE_CURVE_WITH_KNOTS('',3,(#314645,#314646,#314647,#314648,
#314649,#314650,#314651,#314652,#314653,#314654,#314655,#314656,#314657,
#314658,#314659,#314660),.UNSPECIFIED.,.F.,.F.,(4,2,2,2,2,2,2,4),(-0.132441264289709,
-0.132301752201889,-0.132011244623169,-0.130974107930178,-0.127242136360118,
-0.113828931045309,-0.0760058952801183,0.),.UNSPECIFIED.);
#24537=B_SPLINE_CURVE_WITH_KNOTS('',3,(#316317,#316318,#316319,#316320,
#316321,#316322,#316323,#316324),.UNSPECIFIED.,.F.,.F.,(4,2,2,4),(-0.00163871356828074,
-0.00100690578806506,-0.00010312555215194,0.),.UNSPECIFIED.);
#24538=B_SPLINE_CURVE_WITH_KNOTS('',3,(#317992,#317993,#317994,#317995,
#317996,#317997,#317998,#317999,#318000,#318001,#318002,#318003,#318004,
#318005,#318006,#318007),.UNSPECIFIED.,.F.,.F.,(4,2,2,2,2,2,2,4),(-0.138323148368157,
-0.138172915844685,-0.137860160282058,-0.13674324792726,-0.132729597365935,
-0.11829388670653,-0.0778047121160501,0.),.UNSPECIFIED.);
#24539=B_SPLINE_CURVE_WITH_KNOTS('',3,(#319664,#319665,#319666,#319667,
#319668,#319669,#319670,#319671),.UNSPECIFIED.,.F.,.F.,(4,2,2,4),(-0.00683207530728584,
-0.00374062884194389,-5.07020744551543E-5,0.),.UNSPECIFIED.);
#24540=B_SPLINE_CURVE_WITH_KNOTS('',3,(#321339,#321340,#321341,#321342,
#321343,#321344,#321345,#321346,#321347,#321348,#321349,#321350,#321351,
#321352,#321353,#321354),.UNSPECIFIED.,.F.,.F.,(4,2,2,2,2,2,2,4),(-0.143767075145791,
-0.143608474326114,-0.143277668302111,-0.142095827417839,-0.137843826166185,
-0.122558719084724,-0.0796101518115738,0.),.UNSPECIFIED.);
#24541=B_SPLINE_CURVE_WITH_KNOTS('',3,(#323011,#323012,#323013,#323014,
#323015,#323016,#323017,#323018),.UNSPECIFIED.,.F.,.F.,(4,2,2,4),(-0.00719768080497297,
-0.00370110887005153,-5.07021894051734E-5,0.),.UNSPECIFIED.);
#24542=B_SPLINE_CURVE_WITH_KNOTS('',3,(#324686,#324687,#324688,#324689,
#324690,#324691,#324692,#324693,#324694,#324695,#324696,#324697,#324698,
#324699,#324700,#324701),.UNSPECIFIED.,.F.,.F.,(4,2,2,2,2,2,2,4),(-0.14363224299588,
-0.143472580603887,-0.143140928986925,-0.141961284557612,-0.137718803195773,
-0.122454797987602,-0.0795494190128052,0.),.UNSPECIFIED.);
#24543=B_SPLINE_CURVE_WITH_KNOTS('',3,(#326358,#326359,#326360,#326361,
#326362,#326363,#326364,#326365),.UNSPECIFIED.,.F.,.F.,(4,2,2,4),(-0.00605122429428347,
-0.00366238405600456,-4.18241591403333E-5,0.),.UNSPECIFIED.);
#24544=B_SPLINE_CURVE_WITH_KNOTS('',3,(#328033,#328034,#328035,#328036,
#328037,#328038,#328039,#328040,#328041,#328042,#328043,#328044),
 .UNSPECIFIED.,.F.,.F.,(4,2,2,2,2,4),(-0.119546192578266,-0.117359437610194,
-0.114219520548498,-0.102929956115504,-0.0710513220875969,0.),
 .UNSPECIFIED.);
#24545=B_SPLINE_CURVE_WITH_KNOTS('',3,(#329701,#329702,#329703,#329704,
#329705,#329706,#329707,#329708),.UNSPECIFIED.,.F.,.F.,(4,2,2,4),(-0.0418544645696711,
-0.0252942680361084,-6.99729050106145E-5,0.),.UNSPECIFIED.);
#24546=B_SPLINE_CURVE_WITH_KNOTS('',3,(#329719,#329720,#329721,#329722,
#329723,#329724,#329725,#329726,#329727,#329728,#329729,#329730,#329731,
#329732,#329733,#329734),.UNSPECIFIED.,.F.,.F.,(4,2,2,2,2,2,2,4),(-0.129150425464729,
-0.129016270743863,-0.128736621265872,-0.127737293228282,-0.124145204909972,
-0.111227880552902,-0.0748499805365921,0.),.UNSPECIFIED.);
#24547=B_SPLINE_CURVE_WITH_KNOTS('',3,(#329738,#329739,#329740,#329741,
#329742,#329743,#329744,#329745),.UNSPECIFIED.,.F.,.F.,(4,2,2,4),(-0.00689158150654533,
-0.00365899181017955,-4.19445996243972E-5,0.),.UNSPECIFIED.);
#24548=B_SPLINE_CURVE_WITH_KNOTS('',3,(#329753,#329754,#329755,#329756,
#329757,#329758,#329759,#329760,#329761,#329762,#329763,#329764,#329765,
#329766,#329767,#329768),.UNSPECIFIED.,.F.,.F.,(4,2,2,2,2,2,2,4),(-0.119393705608938,
-0.119274862081618,-0.119027348912843,-0.118143922497865,-0.114963738502735,
-0.103517110080035,-0.0713053200773227,0.),.UNSPECIFIED.);
#24549=B_SPLINE_CURVE_WITH_KNOTS('',3,(#329772,#329773,#329774,#329775,
#329776,#329777,#329778,#329779),.UNSPECIFIED.,.F.,.F.,(4,2,2,4),(-0.00148881294802438,
-0.000834884330736283,-3.083227021591E-5,0.),.UNSPECIFIED.);
#24550=B_SPLINE_CURVE_WITH_KNOTS('',3,(#329787,#329788,#329789,#329790,
#329791,#329792,#329793,#329794,#329795,#329796,#329797,#329798,#329799,
#329800,#329801,#329802),.UNSPECIFIED.,.F.,.F.,(4,2,2,2,2,2,2,4),(-0.135670819220167,
-0.135524749497021,-0.13522124870382,-0.134142504666,-0.130258362648282,
-0.116280070506163,-0.0769984882364565,0.),.UNSPECIFIED.);
#24551=B_SPLINE_CURVE_WITH_KNOTS('',3,(#329806,#329807,#329808,#329809,
#329810,#329811,#329812,#329813),.UNSPECIFIED.,.F.,.F.,(4,2,2,4),(-0.00613306070600771,
-0.00372520969540507,-5.07021786216344E-5,0.),.UNSPECIFIED.);
#24552=B_SPLINE_CURVE_WITH_KNOTS('',3,(#329821,#329822,#329823,#329824,
#329825,#329826,#329827,#329828,#329829,#329830,#329831,#329832),
 .UNSPECIFIED.,.F.,.F.,(4,2,2,2,2,4),(-0.143766791143142,-0.140872566153918,
-0.136680946811064,-0.121606689071448,-0.079163682256657,0.),
 .UNSPECIFIED.);
#24553=B_SPLINE_CURVE_WITH_KNOTS('',3,(#329836,#329837,#329838,#329839,
#329840,#329841,#329842,#329843),.UNSPECIFIED.,.F.,.F.,(4,2,2,4),(-0.00698848173989863,
-0.00380836019302225,-5.82110553478941E-5,0.),.UNSPECIFIED.);
#24554=B_SPLINE_CURVE_WITH_KNOTS('',3,(#329851,#329852,#329853,#329854,
#329855,#329856,#329857,#329858,#329859,#329860,#329861,#329862,#329863,
#329864,#329865,#329866),.UNSPECIFIED.,.F.,.F.,(4,2,2,2,2,2,2,4),(-0.135883900824496,
-0.13573820087219,-0.135435129549483,-0.134354905429447,-0.130469586234427,
-0.116508674488936,-0.077137265891236,0.),.UNSPECIFIED.);
#24555=B_SPLINE_CURVE_WITH_KNOTS('',3,(#329870,#329871,#329872,#329873,
#329874,#329875,#329876,#329877),.UNSPECIFIED.,.F.,.F.,(4,2,2,4),(-0.00128524516781947,
-0.000715215174727928,-4.8121161636398E-5,0.),.UNSPECIFIED.);
#24556=B_SPLINE_CURVE_WITH_KNOTS('',3,(#329885,#329886,#329887,#329888,
#329889,#329890,#329891,#329892,#329893,#329894,#329895,#329896,#329897,
#329898,#329899,#329900),.UNSPECIFIED.,.F.,.F.,(4,2,2,2,2,2,2,4),(-0.120303146869983,
-0.120182939666542,-0.119932412090095,-0.119036963258739,-0.115814297142423,
-0.104228098096731,-0.0716487624400435,0.),.UNSPECIFIED.);
#24557=B_SPLINE_CURVE_WITH_KNOTS('',3,(#329904,#329905,#329906,#329907,
#329908,#329909,#329910,#329911),.UNSPECIFIED.,.F.,.F.,(4,2,2,4),(-0.009308619177808,
-0.00476368906676523,-9.53428458459868E-5,0.),.UNSPECIFIED.);
#24558=B_SPLINE_CURVE_WITH_KNOTS('',3,(#329919,#329920,#329921,#329922,
#329923,#329924,#329925,#329926,#329927,#329928,#329929,#329930,#329931,
#329932,#329933,#329934),.UNSPECIFIED.,.F.,.F.,(4,2,2,2,2,2,2,4),(-0.143067411193629,
-0.143035855582011,-0.142707176832962,-0.141532914776148,-0.13731284965564,
-0.122133314646075,-0.0793821783049702,0.),.UNSPECIFIED.);
#24559=B_SPLINE_CURVE_WITH_KNOTS('',3,(#329938,#329939,#329940,#329941,
#329942,#329943,#329944,#329945),.UNSPECIFIED.,.F.,.F.,(4,2,2,4),(-0.00671278728818733,
-0.00366284788260162,-4.11768380858013E-5,0.),.UNSPECIFIED.);
#24560=B_SPLINE_CURVE_WITH_KNOTS('',3,(#329953,#329954,#329955,#329956,
#329957,#329958,#329959,#329960,#329961,#329962,#329963,#329964,#329965,
#329966),.UNSPECIFIED.,.F.,.F.,(4,2,2,2,2,2,4),(-0.127252636197906,-0.126633344669922,
-0.125660614619547,-0.122153555706485,-0.109544864528012,-0.0740863921140504,
0.),.UNSPECIFIED.);
#24561=B_SPLINE_CURVE_WITH_KNOTS('',3,(#329970,#329971,#329972,#329973,
#329974,#329975,#329976,#329977),.UNSPECIFIED.,.F.,.F.,(4,2,2,4),(-0.00702763263084672,
-0.00369143312405739,-5.07019646426106E-5,0.),.UNSPECIFIED.);
#24562=B_SPLINE_CURVE_WITH_KNOTS('',3,(#329984,#329985,#329986,#329987,
#329988,#329989,#329990,#329991,#329992,#329993),.UNSPECIFIED.,.F.,.F.,
(4,2,2,2,4),(-0.183717286685379,-0.168622483379294,-0.147423609245421,-0.0876957493345989,
0.),.UNSPECIFIED.);
#28487=LINE('',#153543,#32289);
#28488=LINE('',#153546,#32290);
#28489=LINE('',#154493,#32291);
#28490=LINE('',#156382,#32292);
#28491=LINE('',#157330,#32293);
#28492=LINE('',#157338,#32294);
#28493=LINE('',#157341,#32295);
#28494=LINE('',#158288,#32296);
#28495=LINE('',#160818,#32297);
#28496=LINE('',#160826,#32298);
#28497=LINE('',#160829,#32299);
#28498=LINE('',#163376,#32300);
#28499=LINE('',#164018,#32301);
#28500=LINE('',#164026,#32302);
#28501=LINE('',#164029,#32303);
#28502=LINE('',#164976,#32304);
#28503=LINE('',#167218,#32305);
#28504=LINE('',#167226,#32306);
#28505=LINE('',#167229,#32307);
#28506=LINE('',#170064,#32308);
#28507=LINE('',#171012,#32309);
#28508=LINE('',#171020,#32310);
#28509=LINE('',#171023,#32311);
#28510=LINE('',#171970,#32312);
#28511=LINE('',#174500,#32313);
#28512=LINE('',#174508,#32314);
#28513=LINE('',#174511,#32315);
#28514=LINE('',#177055,#32316);
#28515=LINE('',#177709,#32317);
#28516=LINE('',#177717,#32318);
#28517=LINE('',#177720,#32319);
#28518=LINE('',#178667,#32320);
#28519=LINE('',#181200,#32321);
#28520=LINE('',#181208,#32322);
#28521=LINE('',#181211,#32323);
#28522=LINE('',#183734,#32324);
#28523=LINE('',#184682,#32325);
#28524=LINE('',#184690,#32326);
#28525=LINE('',#184693,#32327);
#28526=LINE('',#185640,#32328);
#28527=LINE('',#187870,#32329);
#28528=LINE('',#187878,#32330);
#28529=LINE('',#187881,#32331);
#28530=LINE('',#190380,#32332);
#28531=LINE('',#191004,#32333);
#28532=LINE('',#191012,#32334);
#28533=LINE('',#191015,#32335);
#28534=LINE('',#191962,#32336);
#28535=LINE('',#194472,#32337);
#28536=LINE('',#194480,#32338);
#28537=LINE('',#194483,#32339);
#28538=LINE('',#197000,#32340);
#28539=LINE('',#197948,#32341);
#28540=LINE('',#197956,#32342);
#28541=LINE('',#197959,#32343);
#28542=LINE('',#198906,#32344);
#28543=LINE('',#201106,#32345);
#28544=LINE('',#201114,#32346);
#28545=LINE('',#201117,#32347);
#28546=LINE('',#203646,#32348);
#28547=LINE('',#204282,#32349);
#28548=LINE('',#204290,#32350);
#28549=LINE('',#204293,#32351);
#28550=LINE('',#205240,#32352);
#28551=LINE('',#207434,#32353);
#28552=LINE('',#207442,#32354);
#28553=LINE('',#207445,#32355);
#28554=LINE('',#209974,#32356);
#28555=LINE('',#210613,#32357);
#28556=LINE('',#210621,#32358);
#28557=LINE('',#210624,#32359);
#28558=LINE('',#211571,#32360);
#28559=LINE('',#213777,#32361);
#28560=LINE('',#213785,#32362);
#28561=LINE('',#213788,#32363);
#28562=LINE('',#216311,#32364);
#28563=LINE('',#216944,#32365);
#28564=LINE('',#216952,#32366);
#28565=LINE('',#216955,#32367);
#28566=LINE('',#217902,#32368);
#28567=LINE('',#220409,#32369);
#28568=LINE('',#220417,#32370);
#28569=LINE('',#220420,#32371);
#28570=LINE('',#222922,#32372);
#28571=LINE('',#223552,#32373);
#28572=LINE('',#223560,#32374);
#28573=LINE('',#223563,#32375);
#28574=LINE('',#224510,#32376);
#28575=LINE('',#226996,#32377);
#28576=LINE('',#227004,#32378);
#28577=LINE('',#227007,#32379);
#28578=LINE('',#229521,#32380);
#28579=LINE('',#230136,#32381);
#28580=LINE('',#230144,#32382);
#28581=LINE('',#230147,#32383);
#28582=LINE('',#231094,#32384);
#28583=LINE('',#233276,#32385);
#28584=LINE('',#233284,#32386);
#28585=LINE('',#233287,#32387);
#28586=LINE('',#235816,#32388);
#28587=LINE('',#236434,#32389);
#28588=LINE('',#236442,#32390);
#28589=LINE('',#236445,#32391);
#28590=LINE('',#237392,#32392);
#28591=LINE('',#239604,#32393);
#28592=LINE('',#239612,#32394);
#28593=LINE('',#239615,#32395);
#28594=LINE('',#242138,#32396);
#28595=LINE('',#242771,#32397);
#28596=LINE('',#242779,#32398);
#28597=LINE('',#242782,#32399);
#28598=LINE('',#243729,#32400);
#28599=LINE('',#246253,#32401);
#28600=LINE('',#246261,#32402);
#28601=LINE('',#246264,#32403);
#28602=LINE('',#248790,#32404);
#28603=LINE('',#249426,#32405);
#28604=LINE('',#249434,#32406);
#28605=LINE('',#249437,#32407);
#28606=LINE('',#250384,#32408);
#28607=LINE('',#252599,#32409);
#28608=LINE('',#252607,#32410);
#28609=LINE('',#252610,#32411);
#28610=LINE('',#255112,#32412);
#28611=LINE('',#255751,#32413);
#28612=LINE('',#255759,#32414);
#28613=LINE('',#255762,#32415);
#28614=LINE('',#256709,#32416);
#28615=LINE('',#258900,#32417);
#28616=LINE('',#258908,#32418);
#28617=LINE('',#258911,#32419);
#28618=LINE('',#261744,#32420);
#28619=LINE('',#262692,#32421);
#28620=LINE('',#262700,#32422);
#28621=LINE('',#262703,#32423);
#28622=LINE('',#263650,#32424);
#28623=LINE('',#266146,#32425);
#28624=LINE('',#266154,#32426);
#28625=LINE('',#266157,#32427);
#28626=LINE('',#268689,#32428);
#28627=LINE('',#269635,#32429);
#28628=LINE('',#269643,#32430);
#28629=LINE('',#269646,#32431);
#28630=LINE('',#270593,#32432);
#28631=LINE('',#272832,#32433);
#28632=LINE('',#272840,#32434);
#28633=LINE('',#272843,#32435);
#28634=LINE('',#275384,#32436);
#28635=LINE('',#276035,#32437);
#28636=LINE('',#276043,#32438);
#28637=LINE('',#276046,#32439);
#28638=LINE('',#276993,#32440);
#28639=LINE('',#279530,#32441);
#28640=LINE('',#279538,#32442);
#28641=LINE('',#279541,#32443);
#28642=LINE('',#282079,#32444);
#28643=LINE('',#282739,#32445);
#28644=LINE('',#282747,#32446);
#28645=LINE('',#282750,#32447);
#28646=LINE('',#283697,#32448);
#28647=LINE('',#286533,#32449);
#28648=LINE('',#286541,#32450);
#28649=LINE('',#286544,#32451);
#28650=LINE('',#289377,#32452);
#28651=LINE('',#290028,#32453);
#28652=LINE('',#290036,#32454);
#28653=LINE('',#290039,#32455);
#28654=LINE('',#290986,#32456);
#28655=LINE('',#293216,#32457);
#28656=LINE('',#293224,#32458);
#28657=LINE('',#293227,#32459);
#28658=LINE('',#295753,#32460);
#28659=LINE('',#297503,#32461);
#28660=LINE('',#297507,#32462);
#28661=LINE('',#297511,#32463);
#28662=LINE('',#297514,#32464);
#28663=LINE('',#300198,#32465);
#28664=LINE('',#300205,#32466);
#28665=LINE('',#300211,#32467);
#28666=LINE('',#300218,#32468);
#28667=LINE('',#300222,#32469);
#28668=LINE('',#300285,#32470);
#28669=LINE('',#300289,#32471);
#28670=LINE('',#300357,#32472);
#28671=LINE('',#300361,#32473);
#28672=LINE('',#300429,#32474);
#28673=LINE('',#300433,#32475);
#28674=LINE('',#300501,#32476);
#28675=LINE('',#300505,#32477);
#28676=LINE('',#300568,#32478);
#28677=LINE('',#300572,#32479);
#28678=LINE('',#300610,#32480);
#28679=LINE('',#300614,#32481);
#28680=LINE('',#300682,#32482);
#28681=LINE('',#300686,#32483);
#28682=LINE('',#300718,#32484);
#28683=LINE('',#300722,#32485);
#28684=LINE('',#300787,#32486);
#28685=LINE('',#300791,#32487);
#28686=LINE('',#300856,#32488);
#28687=LINE('',#300860,#32489);
#28688=LINE('',#300898,#32490);
#28689=LINE('',#300902,#32491);
#28690=LINE('',#300967,#32492);
#28691=LINE('',#300971,#32493);
#28692=LINE('',#301009,#32494);
#28693=LINE('',#301013,#32495);
#28694=LINE('',#301078,#32496);
#28695=LINE('',#301082,#32497);
#28696=LINE('',#301147,#32498);
#28697=LINE('',#301151,#32499);
#28698=LINE('',#301214,#32500);
#28699=LINE('',#301218,#32501);
#28700=LINE('',#301287,#32502);
#28701=LINE('',#301292,#32503);
#28702=LINE('',#301295,#32504);
#28703=LINE('',#302947,#32505);
#28704=LINE('',#302958,#32506);
#28705=LINE('',#302959,#32507);
#28706=LINE('',#302962,#32508);
#28707=LINE('',#302966,#32509);
#28708=LINE('',#302967,#32510);
#28709=LINE('',#304622,#32511);
#28710=LINE('',#304633,#32512);
#28711=LINE('',#306286,#32513);
#28712=LINE('',#306297,#32514);
#28713=LINE('',#306298,#32515);
#28714=LINE('',#306301,#32516);
#28715=LINE('',#306305,#32517);
#28716=LINE('',#306306,#32518);
#28717=LINE('',#307961,#32519);
#28718=LINE('',#307976,#32520);
#28719=LINE('',#309629,#32521);
#28720=LINE('',#309640,#32522);
#28721=LINE('',#309641,#32523);
#28722=LINE('',#309644,#32524);
#28723=LINE('',#309648,#32525);
#28724=LINE('',#309649,#32526);
#28725=LINE('',#311301,#32527);
#28726=LINE('',#311316,#32528);
#28727=LINE('',#312969,#32529);
#28728=LINE('',#312980,#32530);
#28729=LINE('',#312981,#32531);
#28730=LINE('',#312984,#32532);
#28731=LINE('',#312988,#32533);
#28732=LINE('',#312989,#32534);
#28733=LINE('',#314644,#32535);
#28734=LINE('',#314663,#32536);
#28735=LINE('',#316316,#32537);
#28736=LINE('',#316327,#32538);
#28737=LINE('',#316328,#32539);
#28738=LINE('',#316331,#32540);
#28739=LINE('',#316335,#32541);
#28740=LINE('',#316336,#32542);
#28741=LINE('',#317991,#32543);
#28742=LINE('',#318010,#32544);
#28743=LINE('',#319663,#32545);
#28744=LINE('',#319674,#32546);
#28745=LINE('',#319675,#32547);
#28746=LINE('',#319678,#32548);
#28747=LINE('',#319682,#32549);
#28748=LINE('',#319683,#32550);
#28749=LINE('',#321338,#32551);
#28750=LINE('',#321357,#32552);
#28751=LINE('',#323010,#32553);
#28752=LINE('',#323021,#32554);
#28753=LINE('',#323022,#32555);
#28754=LINE('',#323025,#32556);
#28755=LINE('',#323029,#32557);
#28756=LINE('',#323030,#32558);
#28757=LINE('',#324685,#32559);
#28758=LINE('',#324704,#32560);
#28759=LINE('',#326357,#32561);
#28760=LINE('',#326368,#32562);
#28761=LINE('',#326369,#32563);
#28762=LINE('',#326372,#32564);
#28763=LINE('',#326376,#32565);
#28764=LINE('',#326377,#32566);
#28765=LINE('',#328032,#32567);
#28766=LINE('',#328047,#32568);
#28767=LINE('',#329700,#32569);
#28768=LINE('',#329711,#32570);
#28769=LINE('',#329712,#32571);
#28770=LINE('',#329717,#32572);
#28771=LINE('',#329747,#32573);
#28772=LINE('',#329751,#32574);
#28773=LINE('',#329781,#32575);
#28774=LINE('',#329785,#32576);
#28775=LINE('',#329815,#32577);
#28776=LINE('',#329819,#32578);
#28777=LINE('',#329845,#32579);
#28778=LINE('',#329849,#32580);
#28779=LINE('',#329879,#32581);
#28780=LINE('',#329883,#32582);
#28781=LINE('',#329913,#32583);
#28782=LINE('',#329917,#32584);
#28783=LINE('',#329947,#32585);
#28784=LINE('',#329951,#32586);
#28785=LINE('',#329979,#32587);
#28786=LINE('',#329983,#32588);
#28787=LINE('',#329995,#32589);
#28788=LINE('',#329996,#32590);
#28789=LINE('',#331651,#32591);
#28790=LINE('',#331653,#32592);
#28791=LINE('',#333304,#32593);
#28792=LINE('',#333306,#32594);
#28793=LINE('',#334960,#32595);
#28794=LINE('',#334962,#32596);
#28795=LINE('',#334964,#32597);
#28796=LINE('',#334966,#32598);
#28797=LINE('',#334967,#32599);
#28798=LINE('',#334969,#32600);
#28799=LINE('',#336620,#32601);
#28800=LINE('',#336622,#32602);
#28801=LINE('',#338277,#32603);
#28802=LINE('',#338278,#32604);
#28803=LINE('',#338280,#32605);
#28804=LINE('',#338281,#32606);
#28805=LINE('',#339932,#32607);
#28806=LINE('',#339934,#32608);
#28807=LINE('',#341589,#32609);
#28808=LINE('',#341591,#32610);
#28809=LINE('',#343242,#32611);
#28810=LINE('',#343244,#32612);
#28811=LINE('',#344898,#32613);
#28812=LINE('',#344900,#32614);
#28813=LINE('',#344903,#32615);
#28814=LINE('',#344905,#32616);
#28815=LINE('',#344906,#32617);
#28816=LINE('',#344908,#32618);
#28817=LINE('',#346559,#32619);
#28818=LINE('',#346561,#32620);
#28819=LINE('',#348216,#32621);
#28820=LINE('',#348217,#32622);
#28821=LINE('',#348219,#32623);
#28822=LINE('',#348220,#32624);
#28823=LINE('',#349871,#32625);
#28824=LINE('',#349873,#32626);
#28825=LINE('',#351528,#32627);
#28826=LINE('',#351530,#32628);
#28827=LINE('',#353181,#32629);
#28828=LINE('',#353183,#32630);
#28829=LINE('',#354837,#32631);
#28830=LINE('',#354839,#32632);
#28831=LINE('',#354842,#32633);
#28832=LINE('',#354844,#32634);
#28833=LINE('',#354845,#32635);
#28834=LINE('',#354847,#32636);
#28835=LINE('',#356498,#32637);
#28836=LINE('',#356500,#32638);
#28837=LINE('',#358157,#32639);
#32289=VECTOR('',#114077,3.);
#32290=VECTOR('',#114080,3.);
#32291=VECTOR('',#114081,3.);
#32292=VECTOR('',#114082,3.);
#32293=VECTOR('',#114085,3.);
#32294=VECTOR('',#114094,3.);
#32295=VECTOR('',#114097,3.);
#32296=VECTOR('',#114098,3.);
#32297=VECTOR('',#114101,3.);
#32298=VECTOR('',#114110,3.);
#32299=VECTOR('',#114113,3.);
#32300=VECTOR('',#114114,3.);
#32301=VECTOR('',#114117,3.);
#32302=VECTOR('',#114126,3.);
#32303=VECTOR('',#114129,3.);
#32304=VECTOR('',#114130,3.);
#32305=VECTOR('',#114133,3.);
#32306=VECTOR('',#114142,3.);
#32307=VECTOR('',#114145,3.);
#32308=VECTOR('',#114146,3.);
#32309=VECTOR('',#114149,3.);
#32310=VECTOR('',#114158,3.);
#32311=VECTOR('',#114161,3.);
#32312=VECTOR('',#114162,3.);
#32313=VECTOR('',#114165,3.);
#32314=VECTOR('',#114174,3.);
#32315=VECTOR('',#114177,3.);
#32316=VECTOR('',#114178,3.);
#32317=VECTOR('',#114181,3.);
#32318=VECTOR('',#114190,3.);
#32319=VECTOR('',#114193,3.);
#32320=VECTOR('',#114194,3.);
#32321=VECTOR('',#114197,3.);
#32322=VECTOR('',#114206,3.);
#32323=VECTOR('',#114209,3.);
#32324=VECTOR('',#114210,3.);
#32325=VECTOR('',#114213,3.);
#32326=VECTOR('',#114222,3.);
#32327=VECTOR('',#114225,3.);
#32328=VECTOR('',#114226,3.);
#32329=VECTOR('',#114229,3.);
#32330=VECTOR('',#114238,3.);
#32331=VECTOR('',#114241,3.);
#32332=VECTOR('',#114242,3.);
#32333=VECTOR('',#114245,3.);
#32334=VECTOR('',#114254,3.);
#32335=VECTOR('',#114257,3.);
#32336=VECTOR('',#114258,3.);
#32337=VECTOR('',#114261,3.);
#32338=VECTOR('',#114270,3.);
#32339=VECTOR('',#114273,3.);
#32340=VECTOR('',#114274,3.);
#32341=VECTOR('',#114277,3.);
#32342=VECTOR('',#114286,3.);
#32343=VECTOR('',#114289,3.);
#32344=VECTOR('',#114290,3.);
#32345=VECTOR('',#114293,3.);
#32346=VECTOR('',#114302,3.);
#32347=VECTOR('',#114305,3.);
#32348=VECTOR('',#114306,3.);
#32349=VECTOR('',#114309,3.);
#32350=VECTOR('',#114318,3.);
#32351=VECTOR('',#114321,3.);
#32352=VECTOR('',#114322,3.);
#32353=VECTOR('',#114325,3.);
#32354=VECTOR('',#114334,3.);
#32355=VECTOR('',#114337,3.);
#32356=VECTOR('',#114338,3.);
#32357=VECTOR('',#114341,3.);
#32358=VECTOR('',#114350,3.);
#32359=VECTOR('',#114353,3.);
#32360=VECTOR('',#114354,3.);
#32361=VECTOR('',#114357,3.);
#32362=VECTOR('',#114366,3.);
#32363=VECTOR('',#114369,3.);
#32364=VECTOR('',#114370,3.);
#32365=VECTOR('',#114373,3.);
#32366=VECTOR('',#114382,3.);
#32367=VECTOR('',#114385,3.);
#32368=VECTOR('',#114386,3.);
#32369=VECTOR('',#114389,3.);
#32370=VECTOR('',#114398,3.);
#32371=VECTOR('',#114401,3.);
#32372=VECTOR('',#114402,3.);
#32373=VECTOR('',#114405,3.);
#32374=VECTOR('',#114414,3.);
#32375=VECTOR('',#114417,3.);
#32376=VECTOR('',#114418,3.);
#32377=VECTOR('',#114421,3.);
#32378=VECTOR('',#114430,3.);
#32379=VECTOR('',#114433,3.);
#32380=VECTOR('',#114434,3.);
#32381=VECTOR('',#114437,3.);
#32382=VECTOR('',#114446,3.);
#32383=VECTOR('',#114449,3.);
#32384=VECTOR('',#114450,3.);
#32385=VECTOR('',#114453,3.);
#32386=VECTOR('',#114462,3.);
#32387=VECTOR('',#114465,3.);
#32388=VECTOR('',#114466,3.);
#32389=VECTOR('',#114469,3.);
#32390=VECTOR('',#114478,3.);
#32391=VECTOR('',#114481,3.);
#32392=VECTOR('',#114482,3.);
#32393=VECTOR('',#114485,3.);
#32394=VECTOR('',#114494,3.);
#32395=VECTOR('',#114497,3.);
#32396=VECTOR('',#114498,3.);
#32397=VECTOR('',#114501,3.);
#32398=VECTOR('',#114510,3.);
#32399=VECTOR('',#114513,3.);
#32400=VECTOR('',#114514,3.);
#32401=VECTOR('',#114517,3.);
#32402=VECTOR('',#114526,3.);
#32403=VECTOR('',#114529,3.);
#32404=VECTOR('',#114530,3.);
#32405=VECTOR('',#114533,3.);
#32406=VECTOR('',#114542,3.);
#32407=VECTOR('',#114545,3.);
#32408=VECTOR('',#114546,3.);
#32409=VECTOR('',#114549,3.);
#32410=VECTOR('',#114558,3.);
#32411=VECTOR('',#114561,3.);
#32412=VECTOR('',#114562,3.);
#32413=VECTOR('',#114565,3.);
#32414=VECTOR('',#114574,3.);
#32415=VECTOR('',#114577,3.);
#32416=VECTOR('',#114578,3.);
#32417=VECTOR('',#114581,3.);
#32418=VECTOR('',#114590,3.);
#32419=VECTOR('',#114593,3.);
#32420=VECTOR('',#114594,3.);
#32421=VECTOR('',#114597,3.);
#32422=VECTOR('',#114606,3.);
#32423=VECTOR('',#114609,3.);
#32424=VECTOR('',#114610,3.);
#32425=VECTOR('',#114613,3.);
#32426=VECTOR('',#114622,3.);
#32427=VECTOR('',#114625,3.);
#32428=VECTOR('',#114626,3.);
#32429=VECTOR('',#114629,3.);
#32430=VECTOR('',#114638,3.);
#32431=VECTOR('',#114641,3.);
#32432=VECTOR('',#114642,3.);
#32433=VECTOR('',#114645,3.);
#32434=VECTOR('',#114654,3.);
#32435=VECTOR('',#114657,3.);
#32436=VECTOR('',#114658,3.);
#32437=VECTOR('',#114661,3.);
#32438=VECTOR('',#114670,3.);
#32439=VECTOR('',#114673,3.);
#32440=VECTOR('',#114674,3.);
#32441=VECTOR('',#114677,3.);
#32442=VECTOR('',#114686,3.);
#32443=VECTOR('',#114689,3.);
#32444=VECTOR('',#114690,3.);
#32445=VECTOR('',#114693,3.);
#32446=VECTOR('',#114702,3.);
#32447=VECTOR('',#114705,3.);
#32448=VECTOR('',#114706,3.);
#32449=VECTOR('',#114709,3.);
#32450=VECTOR('',#114718,3.);
#32451=VECTOR('',#114721,3.);
#32452=VECTOR('',#114722,3.);
#32453=VECTOR('',#114725,3.);
#32454=VECTOR('',#114734,3.);
#32455=VECTOR('',#114737,3.);
#32456=VECTOR('',#114738,3.);
#32457=VECTOR('',#114741,3.);
#32458=VECTOR('',#114750,3.);
#32459=VECTOR('',#114753,3.);
#32460=VECTOR('',#114754,3.);
#32461=VECTOR('',#114767,3.);
#32462=VECTOR('',#114772,3.);
#32463=VECTOR('',#114777,3.);
#32464=VECTOR('',#114780,3.);
#32465=VECTOR('',#114783,3.5);
#32466=VECTOR('',#114792,1.5);
#32467=VECTOR('',#114799,1.5);
#32468=VECTOR('',#114808,0.368727902070758);
#32469=VECTOR('',#114811,0.368744954930928);
#32470=VECTOR('',#114814,0.368727849984952);
#32471=VECTOR('',#114817,0.368744955088197);
#32472=VECTOR('',#114820,0.368727849938405);
#32473=VECTOR('',#114823,0.368744956005126);
#32474=VECTOR('',#114826,0.368727850051691);
#32475=VECTOR('',#114829,0.368744956006768);
#32476=VECTOR('',#114832,0.368727850019134);
#32477=VECTOR('',#114835,0.368744954912587);
#32478=VECTOR('',#114838,0.368727849038679);
#32479=VECTOR('',#114841,0.368744954818811);
#32480=VECTOR('',#114844,0.368727849942864);
#32481=VECTOR('',#114847,0.368744954945107);
#32482=VECTOR('',#114850,0.368727848847665);
#32483=VECTOR('',#114853,0.368744955050679);
#32484=VECTOR('',#114856,0.36872784901569);
#32485=VECTOR('',#114859,0.368744955038109);
#32486=VECTOR('',#114862,0.368727900991839);
#32487=VECTOR('',#114865,0.368744954973241);
#32488=VECTOR('',#114868,0.368727902134879);
#32489=VECTOR('',#114871,0.368744955084494);
#32490=VECTOR('',#114874,0.368727901012447);
#32491=VECTOR('',#114877,0.368744954201684);
#32492=VECTOR('',#114880,0.368727902088567);
#32493=VECTOR('',#114883,0.368744955058901);
#32494=VECTOR('',#114886,0.368727901040032);
#32495=VECTOR('',#114889,0.368744955063777);
#32496=VECTOR('',#114892,0.368727900880366);
#32497=VECTOR('',#114895,0.368744954861438);
#32498=VECTOR('',#114898,0.368727901937789);
#32499=VECTOR('',#114901,0.368744955126573);
#32500=VECTOR('',#114904,0.368727902027393);
#32501=VECTOR('',#114907,0.368744956235032);
#32502=VECTOR('',#114916,3.5);
#32503=VECTOR('',#114923,10.);
#32504=VECTOR('',#114926,10.);
#32505=VECTOR('',#114927,10.);
#32506=VECTOR('',#114930,10.);
#32507=VECTOR('',#114931,10.);
#32508=VECTOR('',#114934,10.);
#32509=VECTOR('',#114939,10.);
#32510=VECTOR('',#114940,10.);
#32511=VECTOR('',#114941,10.);
#32512=VECTOR('',#114944,10.);
#32513=VECTOR('',#114947,10.);
#32514=VECTOR('',#114950,10.);
#32515=VECTOR('',#114951,10.);
#32516=VECTOR('',#114954,10.);
#32517=VECTOR('',#114959,10.);
#32518=VECTOR('',#114960,10.);
#32519=VECTOR('',#114961,10.);
#32520=VECTOR('',#114964,10.);
#32521=VECTOR('',#114967,10.);
#32522=VECTOR('',#114970,10.);
#32523=VECTOR('',#114971,10.);
#32524=VECTOR('',#114974,10.);
#32525=VECTOR('',#114979,10.);
#32526=VECTOR('',#114980,10.);
#32527=VECTOR('',#114981,10.);
#32528=VECTOR('',#114984,10.);
#32529=VECTOR('',#114987,10.);
#32530=VECTOR('',#114990,10.);
#32531=VECTOR('',#114991,10.);
#32532=VECTOR('',#114994,10.);
#32533=VECTOR('',#114999,10.);
#32534=VECTOR('',#115000,10.);
#32535=VECTOR('',#115001,10.);
#32536=VECTOR('',#115004,10.);
#32537=VECTOR('',#115007,10.);
#32538=VECTOR('',#115010,10.);
#32539=VECTOR('',#115011,10.);
#32540=VECTOR('',#115014,10.);
#32541=VECTOR('',#115019,10.);
#32542=VECTOR('',#115020,10.);
#32543=VECTOR('',#115021,10.);
#32544=VECTOR('',#115024,10.);
#32545=VECTOR('',#115027,10.);
#32546=VECTOR('',#115030,10.);
#32547=VECTOR('',#115031,10.);
#32548=VECTOR('',#115034,10.);
#32549=VECTOR('',#115039,10.);
#32550=VECTOR('',#115040,10.);
#32551=VECTOR('',#115041,10.);
#32552=VECTOR('',#115044,10.);
#32553=VECTOR('',#115047,10.);
#32554=VECTOR('',#115050,10.);
#32555=VECTOR('',#115051,10.);
#32556=VECTOR('',#115054,10.);
#32557=VECTOR('',#115059,10.);
#32558=VECTOR('',#115060,10.);
#32559=VECTOR('',#115061,10.);
#32560=VECTOR('',#115064,10.);
#32561=VECTOR('',#115067,10.);
#32562=VECTOR('',#115070,10.);
#32563=VECTOR('',#115071,10.);
#32564=VECTOR('',#115074,10.);
#32565=VECTOR('',#115079,10.);
#32566=VECTOR('',#115080,10.);
#32567=VECTOR('',#115081,10.);
#32568=VECTOR('',#115084,10.);
#32569=VECTOR('',#115087,10.);
#32570=VECTOR('',#115090,10.);
#32571=VECTOR('',#115091,10.);
#32572=VECTOR('',#115096,10.);
#32573=VECTOR('',#115099,10.);
#32574=VECTOR('',#115102,10.);
#32575=VECTOR('',#115105,10.);
#32576=VECTOR('',#115108,10.);
#32577=VECTOR('',#115111,10.);
#32578=VECTOR('',#115114,10.);
#32579=VECTOR('',#115117,10.);
#32580=VECTOR('',#115120,10.);
#32581=VECTOR('',#115123,10.);
#32582=VECTOR('',#115126,10.);
#32583=VECTOR('',#115129,10.);
#32584=VECTOR('',#115132,10.);
#32585=VECTOR('',#115135,10.);
#32586=VECTOR('',#115138,10.);
#32587=VECTOR('',#115141,10.);
#32588=VECTOR('',#115144,10.);
#32589=VECTOR('',#115147,10.);
#32590=VECTOR('',#115148,10.);
#32591=VECTOR('',#115151,10.);
#32592=VECTOR('',#115154,10.);
#32593=VECTOR('',#115155,10.);
#32594=VECTOR('',#115158,10.);
#32595=VECTOR('',#115159,10.);
#32596=VECTOR('',#115162,10.);
#32597=VECTOR('',#115165,10.);
#32598=VECTOR('',#115168,10.);
#32599=VECTOR('',#115169,10.);
#32600=VECTOR('',#115172,10.);
#32601=VECTOR('',#115173,10.);
#32602=VECTOR('',#115176,10.);
#32603=VECTOR('',#115179,10.);
#32604=VECTOR('',#115180,10.);
#32605=VECTOR('',#115183,10.);
#32606=VECTOR('',#115184,10.);
#32607=VECTOR('',#115185,10.);
#32608=VECTOR('',#115188,10.);
#32609=VECTOR('',#115191,10.);
#32610=VECTOR('',#115194,10.);
#32611=VECTOR('',#115195,10.);
#32612=VECTOR('',#115198,10.);
#32613=VECTOR('',#115199,10.);
#32614=VECTOR('',#115202,10.);
#32615=VECTOR('',#115207,10.);
#32616=VECTOR('',#115210,10.);
#32617=VECTOR('',#115211,10.);
#32618=VECTOR('',#115214,10.);
#32619=VECTOR('',#115215,10.);
#32620=VECTOR('',#115218,10.);
#32621=VECTOR('',#115221,10.);
#32622=VECTOR('',#115222,10.);
#32623=VECTOR('',#115225,10.);
#32624=VECTOR('',#115226,10.);
#32625=VECTOR('',#115227,10.);
#32626=VECTOR('',#115230,10.);
#32627=VECTOR('',#115233,10.);
#32628=VECTOR('',#115236,10.);
#32629=VECTOR('',#115237,10.);
#32630=VECTOR('',#115240,10.);
#32631=VECTOR('',#115241,10.);
#32632=VECTOR('',#115244,10.);
#32633=VECTOR('',#115249,10.);
#32634=VECTOR('',#115252,10.);
#32635=VECTOR('',#115253,10.);
#32636=VECTOR('',#115256,10.);
#32637=VECTOR('',#115257,10.);
#32638=VECTOR('',#115260,10.);
#32639=VECTOR('',#115265,3.5);
#37452=VERTEX_POINT('',#153539);
#37453=VERTEX_POINT('',#153540);
#37454=VERTEX_POINT('',#153542);
#37455=VERTEX_POINT('',#153544);
#37456=VERTEX_POINT('',#154491);
#37457=VERTEX_POINT('',#154492);
#37458=VERTEX_POINT('',#156380);
#37459=VERTEX_POINT('',#156381);
#37460=VERTEX_POINT('',#157328);
#37461=VERTEX_POINT('',#157329);
#37462=VERTEX_POINT('',#157334);
#37463=VERTEX_POINT('',#157335);
#37464=VERTEX_POINT('',#157337);
#37465=VERTEX_POINT('',#157339);
#37466=VERTEX_POINT('',#158286);
#37467=VERTEX_POINT('',#158287);
#37468=VERTEX_POINT('',#160816);
#37469=VERTEX_POINT('',#160817);
#37470=VERTEX_POINT('',#160822);
#37471=VERTEX_POINT('',#160823);
#37472=VERTEX_POINT('',#160825);
#37473=VERTEX_POINT('',#160827);
#37474=VERTEX_POINT('',#163374);
#37475=VERTEX_POINT('',#163375);
#37476=VERTEX_POINT('',#164016);
#37477=VERTEX_POINT('',#164017);
#37478=VERTEX_POINT('',#164022);
#37479=VERTEX_POINT('',#164023);
#37480=VERTEX_POINT('',#164025);
#37481=VERTEX_POINT('',#164027);
#37482=VERTEX_POINT('',#164974);
#37483=VERTEX_POINT('',#164975);
#37484=VERTEX_POINT('',#167216);
#37485=VERTEX_POINT('',#167217);
#37486=VERTEX_POINT('',#167222);
#37487=VERTEX_POINT('',#167223);
#37488=VERTEX_POINT('',#167225);
#37489=VERTEX_POINT('',#167227);
#37490=VERTEX_POINT('',#170062);
#37491=VERTEX_POINT('',#170063);
#37492=VERTEX_POINT('',#171010);
#37493=VERTEX_POINT('',#171011);
#37494=VERTEX_POINT('',#171016);
#37495=VERTEX_POINT('',#171017);
#37496=VERTEX_POINT('',#171019);
#37497=VERTEX_POINT('',#171021);
#37498=VERTEX_POINT('',#171968);
#37499=VERTEX_POINT('',#171969);
#37500=VERTEX_POINT('',#174498);
#37501=VERTEX_POINT('',#174499);
#37502=VERTEX_POINT('',#174504);
#37503=VERTEX_POINT('',#174505);
#37504=VERTEX_POINT('',#174507);
#37505=VERTEX_POINT('',#174509);
#37506=VERTEX_POINT('',#177053);
#37507=VERTEX_POINT('',#177054);
#37508=VERTEX_POINT('',#177707);
#37509=VERTEX_POINT('',#177708);
#37510=VERTEX_POINT('',#177713);
#37511=VERTEX_POINT('',#177714);
#37512=VERTEX_POINT('',#177716);
#37513=VERTEX_POINT('',#177718);
#37514=VERTEX_POINT('',#178665);
#37515=VERTEX_POINT('',#178666);
#37516=VERTEX_POINT('',#181198);
#37517=VERTEX_POINT('',#181199);
#37518=VERTEX_POINT('',#181204);
#37519=VERTEX_POINT('',#181205);
#37520=VERTEX_POINT('',#181207);
#37521=VERTEX_POINT('',#181209);
#37522=VERTEX_POINT('',#183732);
#37523=VERTEX_POINT('',#183733);
#37524=VERTEX_POINT('',#184680);
#37525=VERTEX_POINT('',#184681);
#37526=VERTEX_POINT('',#184686);
#37527=VERTEX_POINT('',#184687);
#37528=VERTEX_POINT('',#184689);
#37529=VERTEX_POINT('',#184691);
#37530=VERTEX_POINT('',#185638);
#37531=VERTEX_POINT('',#185639);
#37532=VERTEX_POINT('',#187868);
#37533=VERTEX_POINT('',#187869);
#37534=VERTEX_POINT('',#187874);
#37535=VERTEX_POINT('',#187875);
#37536=VERTEX_POINT('',#187877);
#37537=VERTEX_POINT('',#187879);
#37538=VERTEX_POINT('',#190378);
#37539=VERTEX_POINT('',#190379);
#37540=VERTEX_POINT('',#191002);
#37541=VERTEX_POINT('',#191003);
#37542=VERTEX_POINT('',#191008);
#37543=VERTEX_POINT('',#191009);
#37544=VERTEX_POINT('',#191011);
#37545=VERTEX_POINT('',#191013);
#37546=VERTEX_POINT('',#191960);
#37547=VERTEX_POINT('',#191961);
#37548=VERTEX_POINT('',#194470);
#37549=VERTEX_POINT('',#194471);
#37550=VERTEX_POINT('',#194476);
#37551=VERTEX_POINT('',#194477);
#37552=VERTEX_POINT('',#194479);
#37553=VERTEX_POINT('',#194481);
#37554=VERTEX_POINT('',#196998);
#37555=VERTEX_POINT('',#196999);
#37556=VERTEX_POINT('',#197946);
#37557=VERTEX_POINT('',#197947);
#37558=VERTEX_POINT('',#197952);
#37559=VERTEX_POINT('',#197953);
#37560=VERTEX_POINT('',#197955);
#37561=VERTEX_POINT('',#197957);
#37562=VERTEX_POINT('',#198904);
#37563=VERTEX_POINT('',#198905);
#37564=VERTEX_POINT('',#201104);
#37565=VERTEX_POINT('',#201105);
#37566=VERTEX_POINT('',#201110);
#37567=VERTEX_POINT('',#201111);
#37568=VERTEX_POINT('',#201113);
#37569=VERTEX_POINT('',#201115);
#37570=VERTEX_POINT('',#203644);
#37571=VERTEX_POINT('',#203645);
#37572=VERTEX_POINT('',#204280);
#37573=VERTEX_POINT('',#204281);
#37574=VERTEX_POINT('',#204286);
#37575=VERTEX_POINT('',#204287);
#37576=VERTEX_POINT('',#204289);
#37577=VERTEX_POINT('',#204291);
#37578=VERTEX_POINT('',#205238);
#37579=VERTEX_POINT('',#205239);
#37580=VERTEX_POINT('',#207432);
#37581=VERTEX_POINT('',#207433);
#37582=VERTEX_POINT('',#207438);
#37583=VERTEX_POINT('',#207439);
#37584=VERTEX_POINT('',#207441);
#37585=VERTEX_POINT('',#207443);
#37586=VERTEX_POINT('',#209972);
#37587=VERTEX_POINT('',#209973);
#37588=VERTEX_POINT('',#210611);
#37589=VERTEX_POINT('',#210612);
#37590=VERTEX_POINT('',#210617);
#37591=VERTEX_POINT('',#210618);
#37592=VERTEX_POINT('',#210620);
#37593=VERTEX_POINT('',#210622);
#37594=VERTEX_POINT('',#211569);
#37595=VERTEX_POINT('',#211570);
#37596=VERTEX_POINT('',#213775);
#37597=VERTEX_POINT('',#213776);
#37598=VERTEX_POINT('',#213781);
#37599=VERTEX_POINT('',#213782);
#37600=VERTEX_POINT('',#213784);
#37601=VERTEX_POINT('',#213786);
#37602=VERTEX_POINT('',#216309);
#37603=VERTEX_POINT('',#216310);
#37604=VERTEX_POINT('',#216942);
#37605=VERTEX_POINT('',#216943);
#37606=VERTEX_POINT('',#216948);
#37607=VERTEX_POINT('',#216949);
#37608=VERTEX_POINT('',#216951);
#37609=VERTEX_POINT('',#216953);
#37610=VERTEX_POINT('',#217900);
#37611=VERTEX_POINT('',#217901);
#37612=VERTEX_POINT('',#220407);
#37613=VERTEX_POINT('',#220408);
#37614=VERTEX_POINT('',#220413);
#37615=VERTEX_POINT('',#220414);
#37616=VERTEX_POINT('',#220416);
#37617=VERTEX_POINT('',#220418);
#37618=VERTEX_POINT('',#222920);
#37619=VERTEX_POINT('',#222921);
#37620=VERTEX_POINT('',#223550);
#37621=VERTEX_POINT('',#223551);
#37622=VERTEX_POINT('',#223556);
#37623=VERTEX_POINT('',#223557);
#37624=VERTEX_POINT('',#223559);
#37625=VERTEX_POINT('',#223561);
#37626=VERTEX_POINT('',#224508);
#37627=VERTEX_POINT('',#224509);
#37628=VERTEX_POINT('',#226994);
#37629=VERTEX_POINT('',#226995);
#37630=VERTEX_POINT('',#227000);
#37631=VERTEX_POINT('',#227001);
#37632=VERTEX_POINT('',#227003);
#37633=VERTEX_POINT('',#227005);
#37634=VERTEX_POINT('',#229519);
#37635=VERTEX_POINT('',#229520);
#37636=VERTEX_POINT('',#230134);
#37637=VERTEX_POINT('',#230135);
#37638=VERTEX_POINT('',#230140);
#37639=VERTEX_POINT('',#230141);
#37640=VERTEX_POINT('',#230143);
#37641=VERTEX_POINT('',#230145);
#37642=VERTEX_POINT('',#231092);
#37643=VERTEX_POINT('',#231093);
#37644=VERTEX_POINT('',#233274);
#37645=VERTEX_POINT('',#233275);
#37646=VERTEX_POINT('',#233280);
#37647=VERTEX_POINT('',#233281);
#37648=VERTEX_POINT('',#233283);
#37649=VERTEX_POINT('',#233285);
#37650=VERTEX_POINT('',#235814);
#37651=VERTEX_POINT('',#235815);
#37652=VERTEX_POINT('',#236432);
#37653=VERTEX_POINT('',#236433);
#37654=VERTEX_POINT('',#236438);
#37655=VERTEX_POINT('',#236439);
#37656=VERTEX_POINT('',#236441);
#37657=VERTEX_POINT('',#236443);
#37658=VERTEX_POINT('',#237390);
#37659=VERTEX_POINT('',#237391);
#37660=VERTEX_POINT('',#239602);
#37661=VERTEX_POINT('',#239603);
#37662=VERTEX_POINT('',#239608);
#37663=VERTEX_POINT('',#239609);
#37664=VERTEX_POINT('',#239611);
#37665=VERTEX_POINT('',#239613);
#37666=VERTEX_POINT('',#242136);
#37667=VERTEX_POINT('',#242137);
#37668=VERTEX_POINT('',#242769);
#37669=VERTEX_POINT('',#242770);
#37670=VERTEX_POINT('',#242775);
#37671=VERTEX_POINT('',#242776);
#37672=VERTEX_POINT('',#242778);
#37673=VERTEX_POINT('',#242780);
#37674=VERTEX_POINT('',#243727);
#37675=VERTEX_POINT('',#243728);
#37676=VERTEX_POINT('',#246251);
#37677=VERTEX_POINT('',#246252);
#37678=VERTEX_POINT('',#246257);
#37679=VERTEX_POINT('',#246258);
#37680=VERTEX_POINT('',#246260);
#37681=VERTEX_POINT('',#246262);
#37682=VERTEX_POINT('',#248788);
#37683=VERTEX_POINT('',#248789);
#37684=VERTEX_POINT('',#249424);
#37685=VERTEX_POINT('',#249425);
#37686=VERTEX_POINT('',#249430);
#37687=VERTEX_POINT('',#249431);
#37688=VERTEX_POINT('',#249433);
#37689=VERTEX_POINT('',#249435);
#37690=VERTEX_POINT('',#250382);
#37691=VERTEX_POINT('',#250383);
#37692=VERTEX_POINT('',#252597);
#37693=VERTEX_POINT('',#252598);
#37694=VERTEX_POINT('',#252603);
#37695=VERTEX_POINT('',#252604);
#37696=VERTEX_POINT('',#252606);
#37697=VERTEX_POINT('',#252608);
#37698=VERTEX_POINT('',#255110);
#37699=VERTEX_POINT('',#255111);
#37700=VERTEX_POINT('',#255749);
#37701=VERTEX_POINT('',#255750);
#37702=VERTEX_POINT('',#255755);
#37703=VERTEX_POINT('',#255756);
#37704=VERTEX_POINT('',#255758);
#37705=VERTEX_POINT('',#255760);
#37706=VERTEX_POINT('',#256707);
#37707=VERTEX_POINT('',#256708);
#37708=VERTEX_POINT('',#258898);
#37709=VERTEX_POINT('',#258899);
#37710=VERTEX_POINT('',#258904);
#37711=VERTEX_POINT('',#258905);
#37712=VERTEX_POINT('',#258907);
#37713=VERTEX_POINT('',#258909);
#37714=VERTEX_POINT('',#261742);
#37715=VERTEX_POINT('',#261743);
#37716=VERTEX_POINT('',#262690);
#37717=VERTEX_POINT('',#262691);
#37718=VERTEX_POINT('',#262696);
#37719=VERTEX_POINT('',#262697);
#37720=VERTEX_POINT('',#262699);
#37721=VERTEX_POINT('',#262701);
#37722=VERTEX_POINT('',#263648);
#37723=VERTEX_POINT('',#263649);
#37724=VERTEX_POINT('',#266144);
#37725=VERTEX_POINT('',#266145);
#37726=VERTEX_POINT('',#266150);
#37727=VERTEX_POINT('',#266151);
#37728=VERTEX_POINT('',#266153);
#37729=VERTEX_POINT('',#266155);
#37730=VERTEX_POINT('',#268687);
#37731=VERTEX_POINT('',#268688);
#37732=VERTEX_POINT('',#269633);
#37733=VERTEX_POINT('',#269634);
#37734=VERTEX_POINT('',#269639);
#37735=VERTEX_POINT('',#269640);
#37736=VERTEX_POINT('',#269642);
#37737=VERTEX_POINT('',#269644);
#37738=VERTEX_POINT('',#270591);
#37739=VERTEX_POINT('',#270592);
#37740=VERTEX_POINT('',#272830);
#37741=VERTEX_POINT('',#272831);
#37742=VERTEX_POINT('',#272836);
#37743=VERTEX_POINT('',#272837);
#37744=VERTEX_POINT('',#272839);
#37745=VERTEX_POINT('',#272841);
#37746=VERTEX_POINT('',#275382);
#37747=VERTEX_POINT('',#275383);
#37748=VERTEX_POINT('',#276033);
#37749=VERTEX_POINT('',#276034);
#37750=VERTEX_POINT('',#276039);
#37751=VERTEX_POINT('',#276040);
#37752=VERTEX_POINT('',#276042);
#37753=VERTEX_POINT('',#276044);
#37754=VERTEX_POINT('',#276991);
#37755=VERTEX_POINT('',#276992);
#37756=VERTEX_POINT('',#279528);
#37757=VERTEX_POINT('',#279529);
#37758=VERTEX_POINT('',#279534);
#37759=VERTEX_POINT('',#279535);
#37760=VERTEX_POINT('',#279537);
#37761=VERTEX_POINT('',#279539);
#37762=VERTEX_POINT('',#282077);
#37763=VERTEX_POINT('',#282078);
#37764=VERTEX_POINT('',#282737);
#37765=VERTEX_POINT('',#282738);
#37766=VERTEX_POINT('',#282743);
#37767=VERTEX_POINT('',#282744);
#37768=VERTEX_POINT('',#282746);
#37769=VERTEX_POINT('',#282748);
#37770=VERTEX_POINT('',#283695);
#37771=VERTEX_POINT('',#283696);
#37772=VERTEX_POINT('',#286531);
#37773=VERTEX_POINT('',#286532);
#37774=VERTEX_POINT('',#286537);
#37775=VERTEX_POINT('',#286538);
#37776=VERTEX_POINT('',#286540);
#37777=VERTEX_POINT('',#286542);
#37778=VERTEX_POINT('',#289375);
#37779=VERTEX_POINT('',#289376);
#37780=VERTEX_POINT('',#290026);
#37781=VERTEX_POINT('',#290027);
#37782=VERTEX_POINT('',#290032);
#37783=VERTEX_POINT('',#290033);
#37784=VERTEX_POINT('',#290035);
#37785=VERTEX_POINT('',#290037);
#37786=VERTEX_POINT('',#290984);
#37787=VERTEX_POINT('',#290985);
#37788=VERTEX_POINT('',#293214);
#37789=VERTEX_POINT('',#293215);
#37790=VERTEX_POINT('',#293220);
#37791=VERTEX_POINT('',#293221);
#37792=VERTEX_POINT('',#293223);
#37793=VERTEX_POINT('',#293225);
#37794=VERTEX_POINT('',#295751);
#37795=VERTEX_POINT('',#295752);
#37796=VERTEX_POINT('',#296699);
#37797=VERTEX_POINT('',#296701);
#37798=VERTEX_POINT('',#296703);
#37799=VERTEX_POINT('',#297175);
#37800=VERTEX_POINT('',#297499);
#37801=VERTEX_POINT('',#297502);
#37802=VERTEX_POINT('',#297506);
#37803=VERTEX_POINT('',#297510);
#37804=VERTEX_POINT('',#297512);
#37805=VERTEX_POINT('',#300197);
#37806=VERTEX_POINT('',#300202);
#37807=VERTEX_POINT('',#300204);
#37808=VERTEX_POINT('',#300208);
#37809=VERTEX_POINT('',#300210);
#37810=VERTEX_POINT('',#300216);
#37811=VERTEX_POINT('',#300217);
#37812=VERTEX_POINT('',#300219);
#37813=VERTEX_POINT('',#300221);
#37814=VERTEX_POINT('',#300223);
#37815=VERTEX_POINT('',#300238);
#37816=VERTEX_POINT('',#300240);
#37817=VERTEX_POINT('',#300284);
#37818=VERTEX_POINT('',#300286);
#37819=VERTEX_POINT('',#300288);
#37820=VERTEX_POINT('',#300290);
#37821=VERTEX_POINT('',#300307);
#37822=VERTEX_POINT('',#300309);
#37823=VERTEX_POINT('',#300356);
#37824=VERTEX_POINT('',#300358);
#37825=VERTEX_POINT('',#300360);
#37826=VERTEX_POINT('',#300362);
#37827=VERTEX_POINT('',#300379);
#37828=VERTEX_POINT('',#300381);
#37829=VERTEX_POINT('',#300428);
#37830=VERTEX_POINT('',#300430);
#37831=VERTEX_POINT('',#300432);
#37832=VERTEX_POINT('',#300434);
#37833=VERTEX_POINT('',#300451);
#37834=VERTEX_POINT('',#300453);
#37835=VERTEX_POINT('',#300500);
#37836=VERTEX_POINT('',#300502);
#37837=VERTEX_POINT('',#300504);
#37838=VERTEX_POINT('',#300506);
#37839=VERTEX_POINT('',#300521);
#37840=VERTEX_POINT('',#300523);
#37841=VERTEX_POINT('',#300567);
#37842=VERTEX_POINT('',#300569);
#37843=VERTEX_POINT('',#300571);
#37844=VERTEX_POINT('',#300573);
#37845=VERTEX_POINT('',#300590);
#37846=VERTEX_POINT('',#300592);
#37847=VERTEX_POINT('',#300609);
#37848=VERTEX_POINT('',#300611);
#37849=VERTEX_POINT('',#300613);
#37850=VERTEX_POINT('',#300615);
#37851=VERTEX_POINT('',#300632);
#37852=VERTEX_POINT('',#300634);
#37853=VERTEX_POINT('',#300681);
#37854=VERTEX_POINT('',#300683);
#37855=VERTEX_POINT('',#300685);
#37856=VERTEX_POINT('',#300687);
#37857=VERTEX_POINT('',#300704);
#37858=VERTEX_POINT('',#300706);
#37859=VERTEX_POINT('',#300717);
#37860=VERTEX_POINT('',#300719);
#37861=VERTEX_POINT('',#300721);
#37862=VERTEX_POINT('',#300723);
#37863=VERTEX_POINT('',#300740);
#37864=VERTEX_POINT('',#300742);
#37865=VERTEX_POINT('',#300786);
#37866=VERTEX_POINT('',#300788);
#37867=VERTEX_POINT('',#300790);
#37868=VERTEX_POINT('',#300792);
#37869=VERTEX_POINT('',#300809);
#37870=VERTEX_POINT('',#300811);
#37871=VERTEX_POINT('',#300855);
#37872=VERTEX_POINT('',#300857);
#37873=VERTEX_POINT('',#300859);
#37874=VERTEX_POINT('',#300861);
#37875=VERTEX_POINT('',#300878);
#37876=VERTEX_POINT('',#300880);
#37877=VERTEX_POINT('',#300897);
#37878=VERTEX_POINT('',#300899);
#37879=VERTEX_POINT('',#300901);
#37880=VERTEX_POINT('',#300903);
#37881=VERTEX_POINT('',#300920);
#37882=VERTEX_POINT('',#300922);
#37883=VERTEX_POINT('',#300966);
#37884=VERTEX_POINT('',#300968);
#37885=VERTEX_POINT('',#300970);
#37886=VERTEX_POINT('',#300972);
#37887=VERTEX_POINT('',#300989);
#37888=VERTEX_POINT('',#300991);
#37889=VERTEX_POINT('',#301008);
#37890=VERTEX_POINT('',#301010);
#37891=VERTEX_POINT('',#301012);
#37892=VERTEX_POINT('',#301014);
#37893=VERTEX_POINT('',#301031);
#37894=VERTEX_POINT('',#301033);
#37895=VERTEX_POINT('',#301077);
#37896=VERTEX_POINT('',#301079);
#37897=VERTEX_POINT('',#301081);
#37898=VERTEX_POINT('',#301083);
#37899=VERTEX_POINT('',#301100);
#37900=VERTEX_POINT('',#301102);
#37901=VERTEX_POINT('',#301146);
#37902=VERTEX_POINT('',#301148);
#37903=VERTEX_POINT('',#301150);
#37904=VERTEX_POINT('',#301152);
#37905=VERTEX_POINT('',#301167);
#37906=VERTEX_POINT('',#301169);
#37907=VERTEX_POINT('',#301213);
#37908=VERTEX_POINT('',#301215);
#37909=VERTEX_POINT('',#301217);
#37910=VERTEX_POINT('',#301219);
#37911=VERTEX_POINT('',#301236);
#37912=VERTEX_POINT('',#301281);
#37913=VERTEX_POINT('',#301284);
#37914=VERTEX_POINT('',#301286);
#37915=VERTEX_POINT('',#301291);
#37916=VERTEX_POINT('',#301293);
#37917=VERTEX_POINT('',#302946);
#37918=VERTEX_POINT('',#302957);
#37919=VERTEX_POINT('',#302961);
#37920=VERTEX_POINT('',#302965);
#37921=VERTEX_POINT('',#304621);
#37922=VERTEX_POINT('',#304632);
#37923=VERTEX_POINT('',#306285);
#37924=VERTEX_POINT('',#306296);
#37925=VERTEX_POINT('',#306300);
#37926=VERTEX_POINT('',#306304);
#37927=VERTEX_POINT('',#307960);
#37928=VERTEX_POINT('',#307975);
#37929=VERTEX_POINT('',#309628);
#37930=VERTEX_POINT('',#309639);
#37931=VERTEX_POINT('',#309643);
#37932=VERTEX_POINT('',#309647);
#37933=VERTEX_POINT('',#311300);
#37934=VERTEX_POINT('',#311315);
#37935=VERTEX_POINT('',#312968);
#37936=VERTEX_POINT('',#312979);
#37937=VERTEX_POINT('',#312983);
#37938=VERTEX_POINT('',#312987);
#37939=VERTEX_POINT('',#314643);
#37940=VERTEX_POINT('',#314662);
#37941=VERTEX_POINT('',#316315);
#37942=VERTEX_POINT('',#316326);
#37943=VERTEX_POINT('',#316330);
#37944=VERTEX_POINT('',#316334);
#37945=VERTEX_POINT('',#317990);
#37946=VERTEX_POINT('',#318009);
#37947=VERTEX_POINT('',#319662);
#37948=VERTEX_POINT('',#319673);
#37949=VERTEX_POINT('',#319677);
#37950=VERTEX_POINT('',#319681);
#37951=VERTEX_POINT('',#321337);
#37952=VERTEX_POINT('',#321356);
#37953=VERTEX_POINT('',#323009);
#37954=VERTEX_POINT('',#323020);
#37955=VERTEX_POINT('',#323024);
#37956=VERTEX_POINT('',#323028);
#37957=VERTEX_POINT('',#324684);
#37958=VERTEX_POINT('',#324703);
#37959=VERTEX_POINT('',#326356);
#37960=VERTEX_POINT('',#326367);
#37961=VERTEX_POINT('',#326371);
#37962=VERTEX_POINT('',#326375);
#37963=VERTEX_POINT('',#328031);
#37964=VERTEX_POINT('',#328046);
#37965=VERTEX_POINT('',#329699);
#37966=VERTEX_POINT('',#329710);
#37967=VERTEX_POINT('',#329714);
#37968=VERTEX_POINT('',#329716);
#37969=VERTEX_POINT('',#329718);
#37970=VERTEX_POINT('',#329735);
#37971=VERTEX_POINT('',#329737);
#37972=VERTEX_POINT('',#329746);
#37973=VERTEX_POINT('',#329748);
#37974=VERTEX_POINT('',#329750);
#37975=VERTEX_POINT('',#329752);
#37976=VERTEX_POINT('',#329769);
#37977=VERTEX_POINT('',#329771);
#37978=VERTEX_POINT('',#329780);
#37979=VERTEX_POINT('',#329782);
#37980=VERTEX_POINT('',#329784);
#37981=VERTEX_POINT('',#329786);
#37982=VERTEX_POINT('',#329803);
#37983=VERTEX_POINT('',#329805);
#37984=VERTEX_POINT('',#329814);
#37985=VERTEX_POINT('',#329816);
#37986=VERTEX_POINT('',#329818);
#37987=VERTEX_POINT('',#329820);
#37988=VERTEX_POINT('',#329833);
#37989=VERTEX_POINT('',#329835);
#37990=VERTEX_POINT('',#329844);
#37991=VERTEX_POINT('',#329846);
#37992=VERTEX_POINT('',#329848);
#37993=VERTEX_POINT('',#329850);
#37994=VERTEX_POINT('',#329867);
#37995=VERTEX_POINT('',#329869);
#37996=VERTEX_POINT('',#329878);
#37997=VERTEX_POINT('',#329880);
#37998=VERTEX_POINT('',#329882);
#37999=VERTEX_POINT('',#329884);
#38000=VERTEX_POINT('',#329901);
#38001=VERTEX_POINT('',#329903);
#38002=VERTEX_POINT('',#329912);
#38003=VERTEX_POINT('',#329914);
#38004=VERTEX_POINT('',#329916);
#38005=VERTEX_POINT('',#329918);
#38006=VERTEX_POINT('',#329935);
#38007=VERTEX_POINT('',#329937);
#38008=VERTEX_POINT('',#329946);
#38009=VERTEX_POINT('',#329948);
#38010=VERTEX_POINT('',#329950);
#38011=VERTEX_POINT('',#329952);
#38012=VERTEX_POINT('',#329967);
#38013=VERTEX_POINT('',#329969);
#38014=VERTEX_POINT('',#329978);
#38015=VERTEX_POINT('',#329980);
#38016=VERTEX_POINT('',#329982);
#38017=VERTEX_POINT('',#358156);
#47864=EDGE_CURVE('',#37452,#37453,#20150,.T.);
#47865=EDGE_CURVE('',#37453,#37454,#28487,.T.);
#47866=EDGE_CURVE('',#37455,#37454,#20151,.T.);
#47867=EDGE_CURVE('',#37452,#37455,#28488,.T.);
#47868=EDGE_CURVE('',#37456,#37457,#28489,.T.);
#47869=EDGE_CURVE('',#37456,#37452,#24319,.T.);
#47870=EDGE_CURVE('',#37457,#37455,#24320,.T.);
#47871=EDGE_CURVE('',#37458,#37459,#28490,.T.);
#47872=EDGE_CURVE('',#37454,#37458,#24321,.T.);
#47873=EDGE_CURVE('',#37459,#37453,#24322,.T.);
#47874=EDGE_CURVE('',#37460,#37461,#28491,.T.);
#47875=EDGE_CURVE('',#37458,#37461,#20152,.T.);
#47876=EDGE_CURVE('',#37459,#37460,#20153,.T.);
#47877=EDGE_CURVE('',#37462,#37463,#20154,.T.);
#47878=EDGE_CURVE('',#37463,#37464,#28492,.T.);
#47879=EDGE_CURVE('',#37465,#37464,#20155,.T.);
#47880=EDGE_CURVE('',#37462,#37465,#28493,.T.);
#47881=EDGE_CURVE('',#37466,#37467,#28494,.T.);
#47882=EDGE_CURVE('',#37464,#37466,#24323,.T.);
#47883=EDGE_CURVE('',#37467,#37463,#24324,.T.);
#47884=EDGE_CURVE('',#37460,#37462,#24325,.T.);
#47885=EDGE_CURVE('',#37461,#37465,#24326,.T.);
#47886=EDGE_CURVE('',#37468,#37469,#28495,.T.);
#47887=EDGE_CURVE('',#37466,#37469,#20156,.T.);
#47888=EDGE_CURVE('',#37467,#37468,#20157,.T.);
#47889=EDGE_CURVE('',#37470,#37471,#20158,.T.);
#47890=EDGE_CURVE('',#37471,#37472,#28496,.T.);
#47891=EDGE_CURVE('',#37473,#37472,#20159,.T.);
#47892=EDGE_CURVE('',#37470,#37473,#28497,.T.);
#47893=EDGE_CURVE('',#37468,#37470,#24327,.T.);
#47894=EDGE_CURVE('',#37469,#37473,#24328,.T.);
#47895=EDGE_CURVE('',#37474,#37475,#28498,.T.);
#47896=EDGE_CURVE('',#37472,#37474,#24329,.T.);
#47897=EDGE_CURVE('',#37475,#37471,#24330,.T.);
#47898=EDGE_CURVE('',#37476,#37477,#28499,.T.);
#47899=EDGE_CURVE('',#37474,#37477,#20160,.T.);
#47900=EDGE_CURVE('',#37475,#37476,#20161,.T.);
#47901=EDGE_CURVE('',#37478,#37479,#20162,.T.);
#47902=EDGE_CURVE('',#37479,#37480,#28500,.T.);
#47903=EDGE_CURVE('',#37481,#37480,#20163,.T.);
#47904=EDGE_CURVE('',#37478,#37481,#28501,.T.);
#47905=EDGE_CURVE('',#37482,#37483,#28502,.T.);
#47906=EDGE_CURVE('',#37480,#37482,#24331,.T.);
#47907=EDGE_CURVE('',#37483,#37479,#24332,.T.);
#47908=EDGE_CURVE('',#37476,#37478,#24333,.T.);
#47909=EDGE_CURVE('',#37477,#37481,#24334,.T.);
#47910=EDGE_CURVE('',#37484,#37485,#28503,.T.);
#47911=EDGE_CURVE('',#37482,#37485,#20164,.T.);
#47912=EDGE_CURVE('',#37483,#37484,#20165,.T.);
#47913=EDGE_CURVE('',#37486,#37487,#20166,.T.);
#47914=EDGE_CURVE('',#37487,#37488,#28504,.T.);
#47915=EDGE_CURVE('',#37489,#37488,#20167,.T.);
#47916=EDGE_CURVE('',#37486,#37489,#28505,.T.);
#47917=EDGE_CURVE('',#37484,#37486,#24335,.T.);
#47918=EDGE_CURVE('',#37485,#37489,#24336,.T.);
#47919=EDGE_CURVE('',#37490,#37491,#28506,.T.);
#47920=EDGE_CURVE('',#37488,#37490,#24337,.T.);
#47921=EDGE_CURVE('',#37491,#37487,#24338,.T.);
#47922=EDGE_CURVE('',#37492,#37493,#28507,.T.);
#47923=EDGE_CURVE('',#37490,#37493,#20168,.T.);
#47924=EDGE_CURVE('',#37491,#37492,#20169,.T.);
#47925=EDGE_CURVE('',#37494,#37495,#20170,.T.);
#47926=EDGE_CURVE('',#37495,#37496,#28508,.T.);
#47927=EDGE_CURVE('',#37497,#37496,#20171,.T.);
#47928=EDGE_CURVE('',#37494,#37497,#28509,.T.);
#47929=EDGE_CURVE('',#37498,#37499,#28510,.T.);
#47930=EDGE_CURVE('',#37496,#37498,#24339,.T.);
#47931=EDGE_CURVE('',#37499,#37495,#24340,.T.);
#47932=EDGE_CURVE('',#37492,#37494,#24341,.T.);
#47933=EDGE_CURVE('',#37493,#37497,#24342,.T.);
#47934=EDGE_CURVE('',#37500,#37501,#28511,.T.);
#47935=EDGE_CURVE('',#37498,#37501,#20172,.T.);
#47936=EDGE_CURVE('',#37499,#37500,#20173,.T.);
#47937=EDGE_CURVE('',#37502,#37503,#20174,.T.);
#47938=EDGE_CURVE('',#37503,#37504,#28512,.T.);
#47939=EDGE_CURVE('',#37505,#37504,#20175,.T.);
#47940=EDGE_CURVE('',#37502,#37505,#28513,.T.);
#47941=EDGE_CURVE('',#37500,#37502,#24343,.T.);
#47942=EDGE_CURVE('',#37501,#37505,#24344,.T.);
#47943=EDGE_CURVE('',#37506,#37507,#28514,.T.);
#47944=EDGE_CURVE('',#37504,#37506,#24345,.T.);
#47945=EDGE_CURVE('',#37507,#37503,#24346,.T.);
#47946=EDGE_CURVE('',#37508,#37509,#28515,.T.);
#47947=EDGE_CURVE('',#37506,#37509,#20176,.T.);
#47948=EDGE_CURVE('',#37507,#37508,#20177,.T.);
#47949=EDGE_CURVE('',#37510,#37511,#20178,.T.);
#47950=EDGE_CURVE('',#37511,#37512,#28516,.T.);
#47951=EDGE_CURVE('',#37513,#37512,#20179,.T.);
#47952=EDGE_CURVE('',#37510,#37513,#28517,.T.);
#47953=EDGE_CURVE('',#37514,#37515,#28518,.T.);
#47954=EDGE_CURVE('',#37512,#37514,#24347,.T.);
#47955=EDGE_CURVE('',#37515,#37511,#24348,.T.);
#47956=EDGE_CURVE('',#37508,#37510,#24349,.T.);
#47957=EDGE_CURVE('',#37509,#37513,#24350,.T.);
#47958=EDGE_CURVE('',#37516,#37517,#28519,.T.);
#47959=EDGE_CURVE('',#37514,#37517,#20180,.T.);
#47960=EDGE_CURVE('',#37515,#37516,#20181,.T.);
#47961=EDGE_CURVE('',#37518,#37519,#20182,.T.);
#47962=EDGE_CURVE('',#37519,#37520,#28520,.T.);
#47963=EDGE_CURVE('',#37521,#37520,#20183,.T.);
#47964=EDGE_CURVE('',#37518,#37521,#28521,.T.);
#47965=EDGE_CURVE('',#37516,#37518,#24351,.T.);
#47966=EDGE_CURVE('',#37517,#37521,#24352,.T.);
#47967=EDGE_CURVE('',#37522,#37523,#28522,.T.);
#47968=EDGE_CURVE('',#37520,#37522,#24353,.T.);
#47969=EDGE_CURVE('',#37523,#37519,#24354,.T.);
#47970=EDGE_CURVE('',#37524,#37525,#28523,.T.);
#47971=EDGE_CURVE('',#37522,#37525,#20184,.T.);
#47972=EDGE_CURVE('',#37523,#37524,#20185,.T.);
#47973=EDGE_CURVE('',#37526,#37527,#20186,.T.);
#47974=EDGE_CURVE('',#37527,#37528,#28524,.T.);
#47975=EDGE_CURVE('',#37529,#37528,#20187,.T.);
#47976=EDGE_CURVE('',#37526,#37529,#28525,.T.);
#47977=EDGE_CURVE('',#37530,#37531,#28526,.T.);
#47978=EDGE_CURVE('',#37528,#37530,#24355,.T.);
#47979=EDGE_CURVE('',#37531,#37527,#24356,.T.);
#47980=EDGE_CURVE('',#37524,#37526,#24357,.T.);
#47981=EDGE_CURVE('',#37525,#37529,#24358,.T.);
#47982=EDGE_CURVE('',#37532,#37533,#28527,.T.);
#47983=EDGE_CURVE('',#37530,#37533,#20188,.T.);
#47984=EDGE_CURVE('',#37531,#37532,#20189,.T.);
#47985=EDGE_CURVE('',#37534,#37535,#20190,.T.);
#47986=EDGE_CURVE('',#37535,#37536,#28528,.T.);
#47987=EDGE_CURVE('',#37537,#37536,#20191,.T.);
#47988=EDGE_CURVE('',#37534,#37537,#28529,.T.);
#47989=EDGE_CURVE('',#37532,#37534,#24359,.T.);
#47990=EDGE_CURVE('',#37533,#37537,#24360,.T.);
#47991=EDGE_CURVE('',#37538,#37539,#28530,.T.);
#47992=EDGE_CURVE('',#37536,#37538,#24361,.T.);
#47993=EDGE_CURVE('',#37539,#37535,#24362,.T.);
#47994=EDGE_CURVE('',#37540,#37541,#28531,.T.);
#47995=EDGE_CURVE('',#37538,#37541,#20192,.T.);
#47996=EDGE_CURVE('',#37539,#37540,#20193,.T.);
#47997=EDGE_CURVE('',#37542,#37543,#20194,.T.);
#47998=EDGE_CURVE('',#37543,#37544,#28532,.T.);
#47999=EDGE_CURVE('',#37545,#37544,#20195,.T.);
#48000=EDGE_CURVE('',#37542,#37545,#28533,.T.);
#48001=EDGE_CURVE('',#37546,#37547,#28534,.T.);
#48002=EDGE_CURVE('',#37544,#37546,#24363,.T.);
#48003=EDGE_CURVE('',#37547,#37543,#24364,.T.);
#48004=EDGE_CURVE('',#37540,#37542,#24365,.T.);
#48005=EDGE_CURVE('',#37541,#37545,#24366,.T.);
#48006=EDGE_CURVE('',#37548,#37549,#28535,.T.);
#48007=EDGE_CURVE('',#37546,#37549,#20196,.T.);
#48008=EDGE_CURVE('',#37547,#37548,#20197,.T.);
#48009=EDGE_CURVE('',#37550,#37551,#20198,.T.);
#48010=EDGE_CURVE('',#37551,#37552,#28536,.T.);
#48011=EDGE_CURVE('',#37553,#37552,#20199,.T.);
#48012=EDGE_CURVE('',#37550,#37553,#28537,.T.);
#48013=EDGE_CURVE('',#37548,#37550,#24367,.T.);
#48014=EDGE_CURVE('',#37549,#37553,#24368,.T.);
#48015=EDGE_CURVE('',#37554,#37555,#28538,.T.);
#48016=EDGE_CURVE('',#37552,#37554,#24369,.T.);
#48017=EDGE_CURVE('',#37555,#37551,#24370,.T.);
#48018=EDGE_CURVE('',#37556,#37557,#28539,.T.);
#48019=EDGE_CURVE('',#37554,#37557,#20200,.T.);
#48020=EDGE_CURVE('',#37555,#37556,#20201,.T.);
#48021=EDGE_CURVE('',#37558,#37559,#20202,.T.);
#48022=EDGE_CURVE('',#37559,#37560,#28540,.T.);
#48023=EDGE_CURVE('',#37561,#37560,#20203,.T.);
#48024=EDGE_CURVE('',#37558,#37561,#28541,.T.);
#48025=EDGE_CURVE('',#37562,#37563,#28542,.T.);
#48026=EDGE_CURVE('',#37560,#37562,#24371,.T.);
#48027=EDGE_CURVE('',#37563,#37559,#24372,.T.);
#48028=EDGE_CURVE('',#37556,#37558,#24373,.T.);
#48029=EDGE_CURVE('',#37557,#37561,#24374,.T.);
#48030=EDGE_CURVE('',#37564,#37565,#28543,.T.);
#48031=EDGE_CURVE('',#37562,#37565,#20204,.T.);
#48032=EDGE_CURVE('',#37563,#37564,#20205,.T.);
#48033=EDGE_CURVE('',#37566,#37567,#20206,.T.);
#48034=EDGE_CURVE('',#37567,#37568,#28544,.T.);
#48035=EDGE_CURVE('',#37569,#37568,#20207,.T.);
#48036=EDGE_CURVE('',#37566,#37569,#28545,.T.);
#48037=EDGE_CURVE('',#37564,#37566,#24375,.T.);
#48038=EDGE_CURVE('',#37565,#37569,#24376,.T.);
#48039=EDGE_CURVE('',#37570,#37571,#28546,.T.);
#48040=EDGE_CURVE('',#37568,#37570,#24377,.T.);
#48041=EDGE_CURVE('',#37571,#37567,#24378,.T.);
#48042=EDGE_CURVE('',#37572,#37573,#28547,.T.);
#48043=EDGE_CURVE('',#37570,#37573,#20208,.T.);
#48044=EDGE_CURVE('',#37571,#37572,#20209,.T.);
#48045=EDGE_CURVE('',#37574,#37575,#20210,.T.);
#48046=EDGE_CURVE('',#37575,#37576,#28548,.T.);
#48047=EDGE_CURVE('',#37577,#37576,#20211,.T.);
#48048=EDGE_CURVE('',#37574,#37577,#28549,.T.);
#48049=EDGE_CURVE('',#37578,#37579,#28550,.T.);
#48050=EDGE_CURVE('',#37576,#37578,#24379,.T.);
#48051=EDGE_CURVE('',#37579,#37575,#24380,.T.);
#48052=EDGE_CURVE('',#37572,#37574,#24381,.T.);
#48053=EDGE_CURVE('',#37573,#37577,#24382,.T.);
#48054=EDGE_CURVE('',#37580,#37581,#28551,.T.);
#48055=EDGE_CURVE('',#37578,#37581,#20212,.T.);
#48056=EDGE_CURVE('',#37579,#37580,#20213,.T.);
#48057=EDGE_CURVE('',#37582,#37583,#20214,.T.);
#48058=EDGE_CURVE('',#37583,#37584,#28552,.T.);
#48059=EDGE_CURVE('',#37585,#37584,#20215,.T.);
#48060=EDGE_CURVE('',#37582,#37585,#28553,.T.);
#48061=EDGE_CURVE('',#37580,#37582,#24383,.T.);
#48062=EDGE_CURVE('',#37581,#37585,#24384,.T.);
#48063=EDGE_CURVE('',#37586,#37587,#28554,.T.);
#48064=EDGE_CURVE('',#37584,#37586,#24385,.T.);
#48065=EDGE_CURVE('',#37587,#37583,#24386,.T.);
#48066=EDGE_CURVE('',#37588,#37589,#28555,.T.);
#48067=EDGE_CURVE('',#37586,#37589,#20216,.T.);
#48068=EDGE_CURVE('',#37587,#37588,#20217,.T.);
#48069=EDGE_CURVE('',#37590,#37591,#20218,.T.);
#48070=EDGE_CURVE('',#37591,#37592,#28556,.T.);
#48071=EDGE_CURVE('',#37593,#37592,#20219,.T.);
#48072=EDGE_CURVE('',#37590,#37593,#28557,.T.);
#48073=EDGE_CURVE('',#37594,#37595,#28558,.T.);
#48074=EDGE_CURVE('',#37592,#37594,#24387,.T.);
#48075=EDGE_CURVE('',#37595,#37591,#24388,.T.);
#48076=EDGE_CURVE('',#37588,#37590,#24389,.T.);
#48077=EDGE_CURVE('',#37589,#37593,#24390,.T.);
#48078=EDGE_CURVE('',#37596,#37597,#28559,.T.);
#48079=EDGE_CURVE('',#37594,#37597,#20220,.T.);
#48080=EDGE_CURVE('',#37595,#37596,#20221,.T.);
#48081=EDGE_CURVE('',#37598,#37599,#20222,.T.);
#48082=EDGE_CURVE('',#37599,#37600,#28560,.T.);
#48083=EDGE_CURVE('',#37601,#37600,#20223,.T.);
#48084=EDGE_CURVE('',#37598,#37601,#28561,.T.);
#48085=EDGE_CURVE('',#37596,#37598,#24391,.T.);
#48086=EDGE_CURVE('',#37597,#37601,#24392,.T.);
#48087=EDGE_CURVE('',#37602,#37603,#28562,.T.);
#48088=EDGE_CURVE('',#37600,#37602,#24393,.T.);
#48089=EDGE_CURVE('',#37603,#37599,#24394,.T.);
#48090=EDGE_CURVE('',#37604,#37605,#28563,.T.);
#48091=EDGE_CURVE('',#37602,#37605,#20224,.T.);
#48092=EDGE_CURVE('',#37603,#37604,#20225,.T.);
#48093=EDGE_CURVE('',#37606,#37607,#20226,.T.);
#48094=EDGE_CURVE('',#37607,#37608,#28564,.T.);
#48095=EDGE_CURVE('',#37609,#37608,#20227,.T.);
#48096=EDGE_CURVE('',#37606,#37609,#28565,.T.);
#48097=EDGE_CURVE('',#37610,#37611,#28566,.T.);
#48098=EDGE_CURVE('',#37608,#37610,#24395,.T.);
#48099=EDGE_CURVE('',#37611,#37607,#24396,.T.);
#48100=EDGE_CURVE('',#37604,#37606,#24397,.T.);
#48101=EDGE_CURVE('',#37605,#37609,#24398,.T.);
#48102=EDGE_CURVE('',#37612,#37613,#28567,.T.);
#48103=EDGE_CURVE('',#37610,#37613,#20228,.T.);
#48104=EDGE_CURVE('',#37611,#37612,#20229,.T.);
#48105=EDGE_CURVE('',#37614,#37615,#20230,.T.);
#48106=EDGE_CURVE('',#37615,#37616,#28568,.T.);
#48107=EDGE_CURVE('',#37617,#37616,#20231,.T.);
#48108=EDGE_CURVE('',#37614,#37617,#28569,.T.);
#48109=EDGE_CURVE('',#37612,#37614,#24399,.T.);
#48110=EDGE_CURVE('',#37613,#37617,#24400,.T.);
#48111=EDGE_CURVE('',#37618,#37619,#28570,.T.);
#48112=EDGE_CURVE('',#37616,#37618,#24401,.T.);
#48113=EDGE_CURVE('',#37619,#37615,#24402,.T.);
#48114=EDGE_CURVE('',#37620,#37621,#28571,.T.);
#48115=EDGE_CURVE('',#37618,#37621,#20232,.T.);
#48116=EDGE_CURVE('',#37619,#37620,#20233,.T.);
#48117=EDGE_CURVE('',#37622,#37623,#20234,.T.);
#48118=EDGE_CURVE('',#37623,#37624,#28572,.T.);
#48119=EDGE_CURVE('',#37625,#37624,#20235,.T.);
#48120=EDGE_CURVE('',#37622,#37625,#28573,.T.);
#48121=EDGE_CURVE('',#37626,#37627,#28574,.T.);
#48122=EDGE_CURVE('',#37624,#37626,#24403,.T.);
#48123=EDGE_CURVE('',#37627,#37623,#24404,.T.);
#48124=EDGE_CURVE('',#37620,#37622,#24405,.T.);
#48125=EDGE_CURVE('',#37621,#37625,#24406,.T.);
#48126=EDGE_CURVE('',#37628,#37629,#28575,.T.);
#48127=EDGE_CURVE('',#37626,#37629,#20236,.T.);
#48128=EDGE_CURVE('',#37627,#37628,#20237,.T.);
#48129=EDGE_CURVE('',#37630,#37631,#20238,.T.);
#48130=EDGE_CURVE('',#37631,#37632,#28576,.T.);
#48131=EDGE_CURVE('',#37633,#37632,#20239,.T.);
#48132=EDGE_CURVE('',#37630,#37633,#28577,.T.);
#48133=EDGE_CURVE('',#37628,#37630,#24407,.T.);
#48134=EDGE_CURVE('',#37629,#37633,#24408,.T.);
#48135=EDGE_CURVE('',#37634,#37635,#28578,.T.);
#48136=EDGE_CURVE('',#37632,#37634,#24409,.T.);
#48137=EDGE_CURVE('',#37635,#37631,#24410,.T.);
#48138=EDGE_CURVE('',#37636,#37637,#28579,.T.);
#48139=EDGE_CURVE('',#37634,#37637,#20240,.T.);
#48140=EDGE_CURVE('',#37635,#37636,#20241,.T.);
#48141=EDGE_CURVE('',#37638,#37639,#20242,.T.);
#48142=EDGE_CURVE('',#37639,#37640,#28580,.T.);
#48143=EDGE_CURVE('',#37641,#37640,#20243,.T.);
#48144=EDGE_CURVE('',#37638,#37641,#28581,.T.);
#48145=EDGE_CURVE('',#37642,#37643,#28582,.T.);
#48146=EDGE_CURVE('',#37640,#37642,#24411,.T.);
#48147=EDGE_CURVE('',#37643,#37639,#24412,.T.);
#48148=EDGE_CURVE('',#37636,#37638,#24413,.T.);
#48149=EDGE_CURVE('',#37637,#37641,#24414,.T.);
#48150=EDGE_CURVE('',#37644,#37645,#28583,.T.);
#48151=EDGE_CURVE('',#37642,#37645,#20244,.T.);
#48152=EDGE_CURVE('',#37643,#37644,#20245,.T.);
#48153=EDGE_CURVE('',#37646,#37647,#20246,.T.);
#48154=EDGE_CURVE('',#37647,#37648,#28584,.T.);
#48155=EDGE_CURVE('',#37649,#37648,#20247,.T.);
#48156=EDGE_CURVE('',#37646,#37649,#28585,.T.);
#48157=EDGE_CURVE('',#37644,#37646,#24415,.T.);
#48158=EDGE_CURVE('',#37645,#37649,#24416,.T.);
#48159=EDGE_CURVE('',#37650,#37651,#28586,.T.);
#48160=EDGE_CURVE('',#37648,#37650,#24417,.T.);
#48161=EDGE_CURVE('',#37651,#37647,#24418,.T.);
#48162=EDGE_CURVE('',#37652,#37653,#28587,.T.);
#48163=EDGE_CURVE('',#37650,#37653,#20248,.T.);
#48164=EDGE_CURVE('',#37651,#37652,#20249,.T.);
#48165=EDGE_CURVE('',#37654,#37655,#20250,.T.);
#48166=EDGE_CURVE('',#37655,#37656,#28588,.T.);
#48167=EDGE_CURVE('',#37657,#37656,#20251,.T.);
#48168=EDGE_CURVE('',#37654,#37657,#28589,.T.);
#48169=EDGE_CURVE('',#37658,#37659,#28590,.T.);
#48170=EDGE_CURVE('',#37656,#37658,#24419,.T.);
#48171=EDGE_CURVE('',#37659,#37655,#24420,.T.);
#48172=EDGE_CURVE('',#37652,#37654,#24421,.T.);
#48173=EDGE_CURVE('',#37653,#37657,#24422,.T.);
#48174=EDGE_CURVE('',#37660,#37661,#28591,.T.);
#48175=EDGE_CURVE('',#37658,#37661,#20252,.T.);
#48176=EDGE_CURVE('',#37659,#37660,#20253,.T.);
#48177=EDGE_CURVE('',#37662,#37663,#20254,.T.);
#48178=EDGE_CURVE('',#37663,#37664,#28592,.T.);
#48179=EDGE_CURVE('',#37665,#37664,#20255,.T.);
#48180=EDGE_CURVE('',#37662,#37665,#28593,.T.);
#48181=EDGE_CURVE('',#37660,#37662,#24423,.T.);
#48182=EDGE_CURVE('',#37661,#37665,#24424,.T.);
#48183=EDGE_CURVE('',#37666,#37667,#28594,.T.);
#48184=EDGE_CURVE('',#37664,#37666,#24425,.T.);
#48185=EDGE_CURVE('',#37667,#37663,#24426,.T.);
#48186=EDGE_CURVE('',#37668,#37669,#28595,.T.);
#48187=EDGE_CURVE('',#37666,#37669,#20256,.T.);
#48188=EDGE_CURVE('',#37667,#37668,#20257,.T.);
#48189=EDGE_CURVE('',#37670,#37671,#20258,.T.);
#48190=EDGE_CURVE('',#37671,#37672,#28596,.T.);
#48191=EDGE_CURVE('',#37673,#37672,#20259,.T.);
#48192=EDGE_CURVE('',#37670,#37673,#28597,.T.);
#48193=EDGE_CURVE('',#37674,#37675,#28598,.T.);
#48194=EDGE_CURVE('',#37672,#37674,#24427,.T.);
#48195=EDGE_CURVE('',#37675,#37671,#24428,.T.);
#48196=EDGE_CURVE('',#37668,#37670,#24429,.T.);
#48197=EDGE_CURVE('',#37669,#37673,#24430,.T.);
#48198=EDGE_CURVE('',#37676,#37677,#28599,.T.);
#48199=EDGE_CURVE('',#37674,#37677,#20260,.T.);
#48200=EDGE_CURVE('',#37675,#37676,#20261,.T.);
#48201=EDGE_CURVE('',#37678,#37679,#20262,.T.);
#48202=EDGE_CURVE('',#37679,#37680,#28600,.T.);
#48203=EDGE_CURVE('',#37681,#37680,#20263,.T.);
#48204=EDGE_CURVE('',#37678,#37681,#28601,.T.);
#48205=EDGE_CURVE('',#37676,#37678,#24431,.T.);
#48206=EDGE_CURVE('',#37677,#37681,#24432,.T.);
#48207=EDGE_CURVE('',#37682,#37683,#28602,.T.);
#48208=EDGE_CURVE('',#37680,#37682,#24433,.T.);
#48209=EDGE_CURVE('',#37683,#37679,#24434,.T.);
#48210=EDGE_CURVE('',#37684,#37685,#28603,.T.);
#48211=EDGE_CURVE('',#37682,#37685,#20264,.T.);
#48212=EDGE_CURVE('',#37683,#37684,#20265,.T.);
#48213=EDGE_CURVE('',#37686,#37687,#20266,.T.);
#48214=EDGE_CURVE('',#37687,#37688,#28604,.T.);
#48215=EDGE_CURVE('',#37689,#37688,#20267,.T.);
#48216=EDGE_CURVE('',#37686,#37689,#28605,.T.);
#48217=EDGE_CURVE('',#37690,#37691,#28606,.T.);
#48218=EDGE_CURVE('',#37688,#37690,#24435,.T.);
#48219=EDGE_CURVE('',#37691,#37687,#24436,.T.);
#48220=EDGE_CURVE('',#37684,#37686,#24437,.T.);
#48221=EDGE_CURVE('',#37685,#37689,#24438,.T.);
#48222=EDGE_CURVE('',#37692,#37693,#28607,.T.);
#48223=EDGE_CURVE('',#37690,#37693,#20268,.T.);
#48224=EDGE_CURVE('',#37691,#37692,#20269,.T.);
#48225=EDGE_CURVE('',#37694,#37695,#20270,.T.);
#48226=EDGE_CURVE('',#37695,#37696,#28608,.T.);
#48227=EDGE_CURVE('',#37697,#37696,#20271,.T.);
#48228=EDGE_CURVE('',#37694,#37697,#28609,.T.);
#48229=EDGE_CURVE('',#37692,#37694,#24439,.T.);
#48230=EDGE_CURVE('',#37693,#37697,#24440,.T.);
#48231=EDGE_CURVE('',#37698,#37699,#28610,.T.);
#48232=EDGE_CURVE('',#37696,#37698,#24441,.T.);
#48233=EDGE_CURVE('',#37699,#37695,#24442,.T.);
#48234=EDGE_CURVE('',#37700,#37701,#28611,.T.);
#48235=EDGE_CURVE('',#37698,#37701,#20272,.T.);
#48236=EDGE_CURVE('',#37699,#37700,#20273,.T.);
#48237=EDGE_CURVE('',#37702,#37703,#20274,.T.);
#48238=EDGE_CURVE('',#37703,#37704,#28612,.T.);
#48239=EDGE_CURVE('',#37705,#37704,#20275,.T.);
#48240=EDGE_CURVE('',#37702,#37705,#28613,.T.);
#48241=EDGE_CURVE('',#37706,#37707,#28614,.T.);
#48242=EDGE_CURVE('',#37704,#37706,#24443,.T.);
#48243=EDGE_CURVE('',#37707,#37703,#24444,.T.);
#48244=EDGE_CURVE('',#37700,#37702,#24445,.T.);
#48245=EDGE_CURVE('',#37701,#37705,#24446,.T.);
#48246=EDGE_CURVE('',#37708,#37709,#28615,.T.);
#48247=EDGE_CURVE('',#37706,#37709,#20276,.T.);
#48248=EDGE_CURVE('',#37707,#37708,#20277,.T.);
#48249=EDGE_CURVE('',#37710,#37711,#20278,.T.);
#48250=EDGE_CURVE('',#37711,#37712,#28616,.T.);
#48251=EDGE_CURVE('',#37713,#37712,#20279,.T.);
#48252=EDGE_CURVE('',#37710,#37713,#28617,.T.);
#48253=EDGE_CURVE('',#37708,#37710,#24447,.T.);
#48254=EDGE_CURVE('',#37709,#37713,#24448,.T.);
#48255=EDGE_CURVE('',#37714,#37715,#28618,.T.);
#48256=EDGE_CURVE('',#37712,#37714,#24449,.T.);
#48257=EDGE_CURVE('',#37715,#37711,#24450,.T.);
#48258=EDGE_CURVE('',#37716,#37717,#28619,.T.);
#48259=EDGE_CURVE('',#37714,#37717,#20280,.T.);
#48260=EDGE_CURVE('',#37715,#37716,#20281,.T.);
#48261=EDGE_CURVE('',#37718,#37719,#20282,.T.);
#48262=EDGE_CURVE('',#37719,#37720,#28620,.T.);
#48263=EDGE_CURVE('',#37721,#37720,#20283,.T.);
#48264=EDGE_CURVE('',#37718,#37721,#28621,.T.);
#48265=EDGE_CURVE('',#37722,#37723,#28622,.T.);
#48266=EDGE_CURVE('',#37720,#37722,#24451,.T.);
#48267=EDGE_CURVE('',#37723,#37719,#24452,.T.);
#48268=EDGE_CURVE('',#37716,#37718,#24453,.T.);
#48269=EDGE_CURVE('',#37717,#37721,#24454,.T.);
#48270=EDGE_CURVE('',#37724,#37725,#28623,.T.);
#48271=EDGE_CURVE('',#37722,#37725,#20284,.T.);
#48272=EDGE_CURVE('',#37723,#37724,#20285,.T.);
#48273=EDGE_CURVE('',#37726,#37727,#20286,.T.);
#48274=EDGE_CURVE('',#37727,#37728,#28624,.T.);
#48275=EDGE_CURVE('',#37729,#37728,#20287,.T.);
#48276=EDGE_CURVE('',#37726,#37729,#28625,.T.);
#48277=EDGE_CURVE('',#37724,#37726,#24455,.T.);
#48278=EDGE_CURVE('',#37725,#37729,#24456,.T.);
#48279=EDGE_CURVE('',#37730,#37731,#28626,.T.);
#48280=EDGE_CURVE('',#37728,#37730,#24457,.T.);
#48281=EDGE_CURVE('',#37731,#37727,#24458,.T.);
#48282=EDGE_CURVE('',#37732,#37733,#28627,.T.);
#48283=EDGE_CURVE('',#37730,#37733,#20288,.T.);
#48284=EDGE_CURVE('',#37731,#37732,#20289,.T.);
#48285=EDGE_CURVE('',#37734,#37735,#20290,.T.);
#48286=EDGE_CURVE('',#37735,#37736,#28628,.T.);
#48287=EDGE_CURVE('',#37737,#37736,#20291,.T.);
#48288=EDGE_CURVE('',#37734,#37737,#28629,.T.);
#48289=EDGE_CURVE('',#37738,#37739,#28630,.T.);
#48290=EDGE_CURVE('',#37736,#37738,#24459,.T.);
#48291=EDGE_CURVE('',#37739,#37735,#24460,.T.);
#48292=EDGE_CURVE('',#37732,#37734,#24461,.T.);
#48293=EDGE_CURVE('',#37733,#37737,#24462,.T.);
#48294=EDGE_CURVE('',#37740,#37741,#28631,.T.);
#48295=EDGE_CURVE('',#37738,#37741,#20292,.T.);
#48296=EDGE_CURVE('',#37739,#37740,#20293,.T.);
#48297=EDGE_CURVE('',#37742,#37743,#20294,.T.);
#48298=EDGE_CURVE('',#37743,#37744,#28632,.T.);
#48299=EDGE_CURVE('',#37745,#37744,#20295,.T.);
#48300=EDGE_CURVE('',#37742,#37745,#28633,.T.);
#48301=EDGE_CURVE('',#37740,#37742,#24463,.T.);
#48302=EDGE_CURVE('',#37741,#37745,#24464,.T.);
#48303=EDGE_CURVE('',#37746,#37747,#28634,.T.);
#48304=EDGE_CURVE('',#37744,#37746,#24465,.T.);
#48305=EDGE_CURVE('',#37747,#37743,#24466,.T.);
#48306=EDGE_CURVE('',#37748,#37749,#28635,.T.);
#48307=EDGE_CURVE('',#37746,#37749,#20296,.T.);
#48308=EDGE_CURVE('',#37747,#37748,#20297,.T.);
#48309=EDGE_CURVE('',#37750,#37751,#20298,.T.);
#48310=EDGE_CURVE('',#37751,#37752,#28636,.T.);
#48311=EDGE_CURVE('',#37753,#37752,#20299,.T.);
#48312=EDGE_CURVE('',#37750,#37753,#28637,.T.);
#48313=EDGE_CURVE('',#37754,#37755,#28638,.T.);
#48314=EDGE_CURVE('',#37752,#37754,#24467,.T.);
#48315=EDGE_CURVE('',#37755,#37751,#24468,.T.);
#48316=EDGE_CURVE('',#37748,#37750,#24469,.T.);
#48317=EDGE_CURVE('',#37749,#37753,#24470,.T.);
#48318=EDGE_CURVE('',#37756,#37757,#28639,.T.);
#48319=EDGE_CURVE('',#37754,#37757,#20300,.T.);
#48320=EDGE_CURVE('',#37755,#37756,#20301,.T.);
#48321=EDGE_CURVE('',#37758,#37759,#20302,.T.);
#48322=EDGE_CURVE('',#37759,#37760,#28640,.T.);
#48323=EDGE_CURVE('',#37761,#37760,#20303,.T.);
#48324=EDGE_CURVE('',#37758,#37761,#28641,.T.);
#48325=EDGE_CURVE('',#37756,#37758,#24471,.T.);
#48326=EDGE_CURVE('',#37757,#37761,#24472,.T.);
#48327=EDGE_CURVE('',#37762,#37763,#28642,.T.);
#48328=EDGE_CURVE('',#37760,#37762,#24473,.T.);
#48329=EDGE_CURVE('',#37763,#37759,#24474,.T.);
#48330=EDGE_CURVE('',#37764,#37765,#28643,.T.);
#48331=EDGE_CURVE('',#37762,#37765,#20304,.T.);
#48332=EDGE_CURVE('',#37763,#37764,#20305,.T.);
#48333=EDGE_CURVE('',#37766,#37767,#20306,.T.);
#48334=EDGE_CURVE('',#37767,#37768,#28644,.T.);
#48335=EDGE_CURVE('',#37769,#37768,#20307,.T.);
#48336=EDGE_CURVE('',#37766,#37769,#28645,.T.);
#48337=EDGE_CURVE('',#37770,#37771,#28646,.T.);
#48338=EDGE_CURVE('',#37768,#37770,#24475,.T.);
#48339=EDGE_CURVE('',#37771,#37767,#24476,.T.);
#48340=EDGE_CURVE('',#37764,#37766,#24477,.T.);
#48341=EDGE_CURVE('',#37765,#37769,#24478,.T.);
#48342=EDGE_CURVE('',#37772,#37773,#28647,.T.);
#48343=EDGE_CURVE('',#37770,#37773,#20308,.T.);
#48344=EDGE_CURVE('',#37771,#37772,#20309,.T.);
#48345=EDGE_CURVE('',#37774,#37775,#20310,.T.);
#48346=EDGE_CURVE('',#37775,#37776,#28648,.T.);
#48347=EDGE_CURVE('',#37777,#37776,#20311,.T.);
#48348=EDGE_CURVE('',#37774,#37777,#28649,.T.);
#48349=EDGE_CURVE('',#37772,#37774,#24479,.T.);
#48350=EDGE_CURVE('',#37773,#37777,#24480,.T.);
#48351=EDGE_CURVE('',#37778,#37779,#28650,.T.);
#48352=EDGE_CURVE('',#37776,#37778,#24481,.T.);
#48353=EDGE_CURVE('',#37779,#37775,#24482,.T.);
#48354=EDGE_CURVE('',#37780,#37781,#28651,.T.);
#48355=EDGE_CURVE('',#37778,#37781,#20312,.T.);
#48356=EDGE_CURVE('',#37779,#37780,#20313,.T.);
#48357=EDGE_CURVE('',#37782,#37783,#20314,.T.);
#48358=EDGE_CURVE('',#37783,#37784,#28652,.T.);
#48359=EDGE_CURVE('',#37785,#37784,#20315,.T.);
#48360=EDGE_CURVE('',#37782,#37785,#28653,.T.);
#48361=EDGE_CURVE('',#37786,#37787,#28654,.T.);
#48362=EDGE_CURVE('',#37784,#37786,#24483,.T.);
#48363=EDGE_CURVE('',#37787,#37783,#24484,.T.);
#48364=EDGE_CURVE('',#37780,#37782,#24485,.T.);
#48365=EDGE_CURVE('',#37781,#37785,#24486,.T.);
#48366=EDGE_CURVE('',#37788,#37789,#28655,.T.);
#48367=EDGE_CURVE('',#37786,#37789,#20316,.T.);
#48368=EDGE_CURVE('',#37787,#37788,#20317,.T.);
#48369=EDGE_CURVE('',#37790,#37791,#20318,.T.);
#48370=EDGE_CURVE('',#37791,#37792,#28656,.T.);
#48371=EDGE_CURVE('',#37793,#37792,#20319,.T.);
#48372=EDGE_CURVE('',#37790,#37793,#28657,.T.);
#48373=EDGE_CURVE('',#37788,#37790,#24487,.T.);
#48374=EDGE_CURVE('',#37789,#37793,#24488,.T.);
#48375=EDGE_CURVE('',#37794,#37795,#28658,.T.);
#48376=EDGE_CURVE('',#37792,#37794,#24489,.T.);
#48377=EDGE_CURVE('',#37795,#37791,#24490,.T.);
#48378=EDGE_CURVE('',#37795,#37796,#20320,.T.);
#48379=EDGE_CURVE('',#37797,#37456,#20321,.T.);
#48380=EDGE_CURVE('',#37797,#37798,#24491,.T.);
#48381=EDGE_CURVE('',#37799,#37798,#20322,.T.);
#48382=EDGE_CURVE('',#37796,#37799,#24492,.T.);
#48383=EDGE_CURVE('',#37800,#37800,#20323,.T.);
#48384=EDGE_CURVE('',#37801,#37797,#28659,.T.);
#48385=EDGE_CURVE('',#37801,#37457,#20324,.T.);
#48386=EDGE_CURVE('',#37796,#37802,#28660,.T.);
#48387=EDGE_CURVE('',#37794,#37802,#20325,.T.);
#48388=EDGE_CURVE('',#37798,#37803,#28661,.T.);
#48389=EDGE_CURVE('',#37804,#37803,#20326,.T.);
#48390=EDGE_CURVE('',#37799,#37804,#28662,.T.);
#48391=EDGE_CURVE('',#37803,#37801,#24493,.T.);
#48392=EDGE_CURVE('',#37802,#37804,#24494,.T.);
#48393=EDGE_CURVE('',#37800,#37805,#28663,.T.);
#48394=EDGE_CURVE('',#37805,#37805,#20327,.T.);
#48395=EDGE_CURVE('',#37806,#37806,#20328,.T.);
#48396=EDGE_CURVE('',#37806,#37807,#28664,.T.);
#48397=EDGE_CURVE('',#37807,#37807,#20329,.T.);
#48398=EDGE_CURVE('',#37808,#37808,#20330,.F.);
#48399=EDGE_CURVE('',#37808,#37809,#28665,.T.);
#48400=EDGE_CURVE('',#37809,#37809,#20331,.T.);
#48401=EDGE_CURVE('',#37810,#37811,#28666,.T.);
#48402=EDGE_CURVE('',#37811,#37812,#20332,.T.);
#48403=EDGE_CURVE('',#37812,#37813,#28667,.T.);
#48404=EDGE_CURVE('',#37813,#37814,#24495,.T.);
#48405=EDGE_CURVE('',#37814,#37815,#20333,.T.);
#48406=EDGE_CURVE('',#37815,#37816,#24496,.T.);
#48407=EDGE_CURVE('',#37816,#37817,#28668,.T.);
#48408=EDGE_CURVE('',#37817,#37818,#20334,.T.);
#48409=EDGE_CURVE('',#37818,#37819,#28669,.T.);
#48410=EDGE_CURVE('',#37819,#37820,#24497,.T.);
#48411=EDGE_CURVE('',#37820,#37821,#20335,.T.);
#48412=EDGE_CURVE('',#37821,#37822,#24498,.T.);
#48413=EDGE_CURVE('',#37822,#37823,#28670,.T.);
#48414=EDGE_CURVE('',#37823,#37824,#20336,.T.);
#48415=EDGE_CURVE('',#37824,#37825,#28671,.T.);
#48416=EDGE_CURVE('',#37825,#37826,#24499,.T.);
#48417=EDGE_CURVE('',#37826,#37827,#20337,.T.);
#48418=EDGE_CURVE('',#37827,#37828,#24500,.T.);
#48419=EDGE_CURVE('',#37828,#37829,#28672,.T.);
#48420=EDGE_CURVE('',#37829,#37830,#20338,.T.);
#48421=EDGE_CURVE('',#37830,#37831,#28673,.T.);
#48422=EDGE_CURVE('',#37831,#37832,#24501,.T.);
#48423=EDGE_CURVE('',#37832,#37833,#20339,.T.);
#48424=EDGE_CURVE('',#37833,#37834,#24502,.T.);
#48425=EDGE_CURVE('',#37834,#37835,#28674,.T.);
#48426=EDGE_CURVE('',#37835,#37836,#20340,.T.);
#48427=EDGE_CURVE('',#37836,#37837,#28675,.T.);
#48428=EDGE_CURVE('',#37837,#37838,#24503,.T.);
#48429=EDGE_CURVE('',#37838,#37839,#20341,.T.);
#48430=EDGE_CURVE('',#37839,#37840,#24504,.T.);
#48431=EDGE_CURVE('',#37840,#37841,#28676,.T.);
#48432=EDGE_CURVE('',#37841,#37842,#20342,.T.);
#48433=EDGE_CURVE('',#37842,#37843,#28677,.T.);
#48434=EDGE_CURVE('',#37843,#37844,#24505,.T.);
#48435=EDGE_CURVE('',#37844,#37845,#20343,.T.);
#48436=EDGE_CURVE('',#37845,#37846,#24506,.T.);
#48437=EDGE_CURVE('',#37846,#37847,#28678,.T.);
#48438=EDGE_CURVE('',#37847,#37848,#20344,.T.);
#48439=EDGE_CURVE('',#37848,#37849,#28679,.T.);
#48440=EDGE_CURVE('',#37849,#37850,#24507,.T.);
#48441=EDGE_CURVE('',#37850,#37851,#20345,.T.);
#48442=EDGE_CURVE('',#37851,#37852,#24508,.T.);
#48443=EDGE_CURVE('',#37852,#37853,#28680,.T.);
#48444=EDGE_CURVE('',#37853,#37854,#20346,.T.);
#48445=EDGE_CURVE('',#37854,#37855,#28681,.T.);
#48446=EDGE_CURVE('',#37855,#37856,#24509,.T.);
#48447=EDGE_CURVE('',#37856,#37857,#20347,.T.);
#48448=EDGE_CURVE('',#37857,#37858,#24510,.T.);
#48449=EDGE_CURVE('',#37858,#37859,#28682,.T.);
#48450=EDGE_CURVE('',#37859,#37860,#20348,.T.);
#48451=EDGE_CURVE('',#37860,#37861,#28683,.T.);
#48452=EDGE_CURVE('',#37861,#37862,#24511,.T.);
#48453=EDGE_CURVE('',#37862,#37863,#20349,.T.);
#48454=EDGE_CURVE('',#37863,#37864,#24512,.T.);
#48455=EDGE_CURVE('',#37864,#37865,#28684,.T.);
#48456=EDGE_CURVE('',#37865,#37866,#20350,.T.);
#48457=EDGE_CURVE('',#37866,#37867,#28685,.T.);
#48458=EDGE_CURVE('',#37867,#37868,#24513,.T.);
#48459=EDGE_CURVE('',#37868,#37869,#20351,.T.);
#48460=EDGE_CURVE('',#37869,#37870,#24514,.T.);
#48461=EDGE_CURVE('',#37870,#37871,#28686,.T.);
#48462=EDGE_CURVE('',#37871,#37872,#20352,.T.);
#48463=EDGE_CURVE('',#37872,#37873,#28687,.T.);
#48464=EDGE_CURVE('',#37873,#37874,#24515,.T.);
#48465=EDGE_CURVE('',#37874,#37875,#20353,.T.);
#48466=EDGE_CURVE('',#37875,#37876,#24516,.T.);
#48467=EDGE_CURVE('',#37876,#37877,#28688,.T.);
#48468=EDGE_CURVE('',#37877,#37878,#20354,.T.);
#48469=EDGE_CURVE('',#37878,#37879,#28689,.T.);
#48470=EDGE_CURVE('',#37879,#37880,#24517,.T.);
#48471=EDGE_CURVE('',#37880,#37881,#20355,.T.);
#48472=EDGE_CURVE('',#37881,#37882,#24518,.T.);
#48473=EDGE_CURVE('',#37882,#37883,#28690,.T.);
#48474=EDGE_CURVE('',#37883,#37884,#20356,.T.);
#48475=EDGE_CURVE('',#37884,#37885,#28691,.T.);
#48476=EDGE_CURVE('',#37885,#37886,#24519,.T.);
#48477=EDGE_CURVE('',#37886,#37887,#20357,.T.);
#48478=EDGE_CURVE('',#37887,#37888,#24520,.T.);
#48479=EDGE_CURVE('',#37888,#37889,#28692,.T.);
#48480=EDGE_CURVE('',#37889,#37890,#20358,.T.);
#48481=EDGE_CURVE('',#37890,#37891,#28693,.T.);
#48482=EDGE_CURVE('',#37891,#37892,#24521,.T.);
#48483=EDGE_CURVE('',#37892,#37893,#20359,.T.);
#48484=EDGE_CURVE('',#37893,#37894,#24522,.T.);
#48485=EDGE_CURVE('',#37894,#37895,#28694,.T.);
#48486=EDGE_CURVE('',#37895,#37896,#20360,.T.);
#48487=EDGE_CURVE('',#37896,#37897,#28695,.T.);
#48488=EDGE_CURVE('',#37897,#37898,#24523,.T.);
#48489=EDGE_CURVE('',#37898,#37899,#20361,.T.);
#48490=EDGE_CURVE('',#37899,#37900,#24524,.T.);
#48491=EDGE_CURVE('',#37900,#37901,#28696,.T.);
#48492=EDGE_CURVE('',#37901,#37902,#20362,.T.);
#48493=EDGE_CURVE('',#37902,#37903,#28697,.T.);
#48494=EDGE_CURVE('',#37903,#37904,#24525,.T.);
#48495=EDGE_CURVE('',#37904,#37905,#20363,.T.);
#48496=EDGE_CURVE('',#37905,#37906,#24526,.T.);
#48497=EDGE_CURVE('',#37906,#37907,#28698,.T.);
#48498=EDGE_CURVE('',#37907,#37908,#20364,.T.);
#48499=EDGE_CURVE('',#37908,#37909,#28699,.T.);
#48500=EDGE_CURVE('',#37909,#37910,#24527,.T.);
#48501=EDGE_CURVE('',#37910,#37911,#20365,.T.);
#48502=EDGE_CURVE('',#37911,#37810,#24528,.T.);
#48503=EDGE_CURVE('',#37912,#37912,#20366,.T.);
#48504=EDGE_CURVE('',#37913,#37913,#20367,.F.);
#48505=EDGE_CURVE('',#37913,#37914,#28700,.T.);
#48506=EDGE_CURVE('',#37914,#37914,#20368,.T.);
#48507=EDGE_CURVE('',#37862,#37915,#28701,.T.);
#48508=EDGE_CURVE('',#37916,#37915,#20369,.T.);
#48509=EDGE_CURVE('',#37863,#37916,#28702,.T.);
#48510=EDGE_CURVE('',#37861,#37917,#28703,.T.);
#48511=EDGE_CURVE('',#37915,#37917,#24529,.T.);
#48512=EDGE_CURVE('',#37918,#37860,#28704,.T.);
#48513=EDGE_CURVE('',#37917,#37918,#28705,.T.);
#48514=EDGE_CURVE('',#37859,#37919,#28706,.T.);
#48515=EDGE_CURVE('',#37918,#37919,#20370,.T.);
#48516=EDGE_CURVE('',#37858,#37920,#28707,.T.);
#48517=EDGE_CURVE('',#37919,#37920,#28708,.T.);
#48518=EDGE_CURVE('',#37857,#37921,#28709,.T.);
#48519=EDGE_CURVE('',#37920,#37921,#24530,.T.);
#48520=EDGE_CURVE('',#37856,#37922,#28710,.T.);
#48521=EDGE_CURVE('',#37921,#37922,#20371,.T.);
#48522=EDGE_CURVE('',#37855,#37923,#28711,.T.);
#48523=EDGE_CURVE('',#37922,#37923,#24531,.T.);
#48524=EDGE_CURVE('',#37924,#37854,#28712,.T.);
#48525=EDGE_CURVE('',#37923,#37924,#28713,.T.);
#48526=EDGE_CURVE('',#37853,#37925,#28714,.T.);
#48527=EDGE_CURVE('',#37924,#37925,#20372,.T.);
#48528=EDGE_CURVE('',#37852,#37926,#28715,.T.);
#48529=EDGE_CURVE('',#37925,#37926,#28716,.T.);
#48530=EDGE_CURVE('',#37851,#37927,#28717,.T.);
#48531=EDGE_CURVE('',#37926,#37927,#24532,.T.);
#48532=EDGE_CURVE('',#37850,#37928,#28718,.T.);
#48533=EDGE_CURVE('',#37927,#37928,#20373,.T.);
#48534=EDGE_CURVE('',#37849,#37929,#28719,.T.);
#48535=EDGE_CURVE('',#37928,#37929,#24533,.T.);
#48536=EDGE_CURVE('',#37930,#37848,#28720,.T.);
#48537=EDGE_CURVE('',#37929,#37930,#28721,.T.);
#48538=EDGE_CURVE('',#37847,#37931,#28722,.T.);
#48539=EDGE_CURVE('',#37930,#37931,#20374,.T.);
#48540=EDGE_CURVE('',#37846,#37932,#28723,.T.);
#48541=EDGE_CURVE('',#37931,#37932,#28724,.T.);
#48542=EDGE_CURVE('',#37845,#37933,#28725,.T.);
#48543=EDGE_CURVE('',#37932,#37933,#24534,.T.);
#48544=EDGE_CURVE('',#37844,#37934,#28726,.T.);
#48545=EDGE_CURVE('',#37933,#37934,#20375,.T.);
#48546=EDGE_CURVE('',#37843,#37935,#28727,.T.);
#48547=EDGE_CURVE('',#37934,#37935,#24535,.T.);
#48548=EDGE_CURVE('',#37936,#37842,#28728,.T.);
#48549=EDGE_CURVE('',#37935,#37936,#28729,.T.);
#48550=EDGE_CURVE('',#37841,#37937,#28730,.T.);
#48551=EDGE_CURVE('',#37936,#37937,#20376,.T.);
#48552=EDGE_CURVE('',#37840,#37938,#28731,.T.);
#48553=EDGE_CURVE('',#37937,#37938,#28732,.T.);
#48554=EDGE_CURVE('',#37839,#37939,#28733,.T.);
#48555=EDGE_CURVE('',#37938,#37939,#24536,.T.);
#48556=EDGE_CURVE('',#37838,#37940,#28734,.T.);
#48557=EDGE_CURVE('',#37939,#37940,#20377,.T.);
#48558=EDGE_CURVE('',#37837,#37941,#28735,.T.);
#48559=EDGE_CURVE('',#37940,#37941,#24537,.T.);
#48560=EDGE_CURVE('',#37942,#37836,#28736,.T.);
#48561=EDGE_CURVE('',#37941,#37942,#28737,.T.);
#48562=EDGE_CURVE('',#37835,#37943,#28738,.T.);
#48563=EDGE_CURVE('',#37942,#37943,#20378,.T.);
#48564=EDGE_CURVE('',#37834,#37944,#28739,.T.);
#48565=EDGE_CURVE('',#37943,#37944,#28740,.T.);
#48566=EDGE_CURVE('',#37833,#37945,#28741,.T.);
#48567=EDGE_CURVE('',#37944,#37945,#24538,.T.);
#48568=EDGE_CURVE('',#37832,#37946,#28742,.T.);
#48569=EDGE_CURVE('',#37945,#37946,#20379,.T.);
#48570=EDGE_CURVE('',#37831,#37947,#28743,.T.);
#48571=EDGE_CURVE('',#37946,#37947,#24539,.T.);
#48572=EDGE_CURVE('',#37948,#37830,#28744,.T.);
#48573=EDGE_CURVE('',#37947,#37948,#28745,.T.);
#48574=EDGE_CURVE('',#37829,#37949,#28746,.T.);
#48575=EDGE_CURVE('',#37948,#37949,#20380,.T.);
#48576=EDGE_CURVE('',#37828,#37950,#28747,.T.);
#48577=EDGE_CURVE('',#37949,#37950,#28748,.T.);
#48578=EDGE_CURVE('',#37827,#37951,#28749,.T.);
#48579=EDGE_CURVE('',#37950,#37951,#24540,.T.);
#48580=EDGE_CURVE('',#37826,#37952,#28750,.T.);
#48581=EDGE_CURVE('',#37951,#37952,#20381,.T.);
#48582=EDGE_CURVE('',#37825,#37953,#28751,.T.);
#48583=EDGE_CURVE('',#37952,#37953,#24541,.T.);
#48584=EDGE_CURVE('',#37954,#37824,#28752,.T.);
#48585=EDGE_CURVE('',#37953,#37954,#28753,.T.);
#48586=EDGE_CURVE('',#37823,#37955,#28754,.T.);
#48587=EDGE_CURVE('',#37954,#37955,#20382,.T.);
#48588=EDGE_CURVE('',#37822,#37956,#28755,.T.);
#48589=EDGE_CURVE('',#37955,#37956,#28756,.T.);
#48590=EDGE_CURVE('',#37821,#37957,#28757,.T.);
#48591=EDGE_CURVE('',#37956,#37957,#24542,.T.);
#48592=EDGE_CURVE('',#37820,#37958,#28758,.T.);
#48593=EDGE_CURVE('',#37957,#37958,#20383,.T.);
#48594=EDGE_CURVE('',#37819,#37959,#28759,.T.);
#48595=EDGE_CURVE('',#37958,#37959,#24543,.T.);
#48596=EDGE_CURVE('',#37960,#37818,#28760,.T.);
#48597=EDGE_CURVE('',#37959,#37960,#28761,.T.);
#48598=EDGE_CURVE('',#37817,#37961,#28762,.T.);
#48599=EDGE_CURVE('',#37960,#37961,#20384,.T.);
#48600=EDGE_CURVE('',#37816,#37962,#28763,.T.);
#48601=EDGE_CURVE('',#37961,#37962,#28764,.T.);
#48602=EDGE_CURVE('',#37815,#37963,#28765,.T.);
#48603=EDGE_CURVE('',#37962,#37963,#24544,.T.);
#48604=EDGE_CURVE('',#37814,#37964,#28766,.T.);
#48605=EDGE_CURVE('',#37963,#37964,#20385,.T.);
#48606=EDGE_CURVE('',#37813,#37965,#28767,.T.);
#48607=EDGE_CURVE('',#37964,#37965,#24545,.T.);
#48608=EDGE_CURVE('',#37966,#37812,#28768,.T.);
#48609=EDGE_CURVE('',#37965,#37966,#28769,.T.);
#48610=EDGE_CURVE('',#37966,#37967,#20386,.T.);
#48611=EDGE_CURVE('',#37967,#37968,#28770,.T.);
#48612=EDGE_CURVE('',#37968,#37969,#24546,.T.);
#48613=EDGE_CURVE('',#37969,#37970,#20387,.T.);
#48614=EDGE_CURVE('',#37970,#37971,#24547,.T.);
#48615=EDGE_CURVE('',#37971,#37972,#28771,.T.);
#48616=EDGE_CURVE('',#37972,#37973,#20388,.T.);
#48617=EDGE_CURVE('',#37973,#37974,#28772,.T.);
#48618=EDGE_CURVE('',#37974,#37975,#24548,.T.);
#48619=EDGE_CURVE('',#37975,#37976,#20389,.T.);
#48620=EDGE_CURVE('',#37976,#37977,#24549,.T.);
#48621=EDGE_CURVE('',#37977,#37978,#28773,.T.);
#48622=EDGE_CURVE('',#37978,#37979,#20390,.T.);
#48623=EDGE_CURVE('',#37979,#37980,#28774,.T.);
#48624=EDGE_CURVE('',#37980,#37981,#24550,.T.);
#48625=EDGE_CURVE('',#37981,#37982,#20391,.T.);
#48626=EDGE_CURVE('',#37982,#37983,#24551,.T.);
#48627=EDGE_CURVE('',#37983,#37984,#28775,.T.);
#48628=EDGE_CURVE('',#37984,#37985,#20392,.T.);
#48629=EDGE_CURVE('',#37985,#37986,#28776,.T.);
#48630=EDGE_CURVE('',#37986,#37987,#24552,.T.);
#48631=EDGE_CURVE('',#37987,#37988,#20393,.T.);
#48632=EDGE_CURVE('',#37988,#37989,#24553,.T.);
#48633=EDGE_CURVE('',#37989,#37990,#28777,.T.);
#48634=EDGE_CURVE('',#37990,#37991,#20394,.T.);
#48635=EDGE_CURVE('',#37991,#37992,#28778,.T.);
#48636=EDGE_CURVE('',#37992,#37993,#24554,.T.);
#48637=EDGE_CURVE('',#37993,#37994,#20395,.T.);
#48638=EDGE_CURVE('',#37994,#37995,#24555,.T.);
#48639=EDGE_CURVE('',#37995,#37996,#28779,.T.);
#48640=EDGE_CURVE('',#37996,#37997,#20396,.T.);
#48641=EDGE_CURVE('',#37997,#37998,#28780,.T.);
#48642=EDGE_CURVE('',#37998,#37999,#24556,.T.);
#48643=EDGE_CURVE('',#37999,#38000,#20397,.T.);
#48644=EDGE_CURVE('',#38000,#38001,#24557,.T.);
#48645=EDGE_CURVE('',#38001,#38002,#28781,.T.);
#48646=EDGE_CURVE('',#38002,#38003,#20398,.T.);
#48647=EDGE_CURVE('',#38003,#38004,#28782,.T.);
#48648=EDGE_CURVE('',#38004,#38005,#24558,.T.);
#48649=EDGE_CURVE('',#38005,#38006,#20399,.T.);
#48650=EDGE_CURVE('',#38006,#38007,#24559,.T.);
#48651=EDGE_CURVE('',#38007,#38008,#28783,.T.);
#48652=EDGE_CURVE('',#38008,#38009,#20400,.T.);
#48653=EDGE_CURVE('',#38009,#38010,#28784,.T.);
#48654=EDGE_CURVE('',#38010,#38011,#24560,.T.);
#48655=EDGE_CURVE('',#38011,#38012,#20401,.T.);
#48656=EDGE_CURVE('',#38012,#38013,#24561,.T.);
#48657=EDGE_CURVE('',#38013,#38014,#28785,.T.);
#48658=EDGE_CURVE('',#38014,#38015,#20402,.T.);
#48659=EDGE_CURVE('',#38015,#38016,#28786,.T.);
#48660=EDGE_CURVE('',#38016,#37916,#24562,.T.);
#48661=EDGE_CURVE('',#37864,#38016,#28787,.T.);
#48662=EDGE_CURVE('',#37865,#38015,#28788,.T.);
#48663=EDGE_CURVE('',#38014,#37866,#28789,.T.);
#48664=EDGE_CURVE('',#37867,#38013,#28790,.T.);
#48665=EDGE_CURVE('',#37868,#38012,#28791,.T.);
#48666=EDGE_CURVE('',#37869,#38011,#28792,.T.);
#48667=EDGE_CURVE('',#37870,#38010,#28793,.T.);
#48668=EDGE_CURVE('',#37871,#38009,#28794,.T.);
#48669=EDGE_CURVE('',#38008,#37872,#28795,.T.);
#48670=EDGE_CURVE('',#37876,#38004,#28796,.T.);
#48671=EDGE_CURVE('',#37877,#38003,#28797,.T.);
#48672=EDGE_CURVE('',#37873,#38007,#28798,.T.);
#48673=EDGE_CURVE('',#37874,#38006,#28799,.T.);
#48674=EDGE_CURVE('',#37875,#38005,#28800,.T.);
#48675=EDGE_CURVE('',#38002,#37878,#28801,.T.);
#48676=EDGE_CURVE('',#37879,#38001,#28802,.T.);
#48677=EDGE_CURVE('',#37882,#37998,#28803,.T.);
#48678=EDGE_CURVE('',#37883,#37997,#28804,.T.);
#48679=EDGE_CURVE('',#37880,#38000,#28805,.T.);
#48680=EDGE_CURVE('',#37881,#37999,#28806,.T.);
#48681=EDGE_CURVE('',#37996,#37884,#28807,.T.);
#48682=EDGE_CURVE('',#37885,#37995,#28808,.T.);
#48683=EDGE_CURVE('',#37886,#37994,#28809,.T.);
#48684=EDGE_CURVE('',#37887,#37993,#28810,.T.);
#48685=EDGE_CURVE('',#37888,#37992,#28811,.T.);
#48686=EDGE_CURVE('',#37889,#37991,#28812,.T.);
#48687=EDGE_CURVE('',#37990,#37890,#28813,.T.);
#48688=EDGE_CURVE('',#37894,#37986,#28814,.T.);
#48689=EDGE_CURVE('',#37895,#37985,#28815,.T.);
#48690=EDGE_CURVE('',#37891,#37989,#28816,.T.);
#48691=EDGE_CURVE('',#37892,#37988,#28817,.T.);
#48692=EDGE_CURVE('',#37893,#37987,#28818,.T.);
#48693=EDGE_CURVE('',#37984,#37896,#28819,.T.);
#48694=EDGE_CURVE('',#37897,#37983,#28820,.T.);
#48695=EDGE_CURVE('',#37900,#37980,#28821,.T.);
#48696=EDGE_CURVE('',#37901,#37979,#28822,.T.);
#48697=EDGE_CURVE('',#37898,#37982,#28823,.T.);
#48698=EDGE_CURVE('',#37899,#37981,#28824,.T.);
#48699=EDGE_CURVE('',#37978,#37902,#28825,.T.);
#48700=EDGE_CURVE('',#37903,#37977,#28826,.T.);
#48701=EDGE_CURVE('',#37904,#37976,#28827,.T.);
#48702=EDGE_CURVE('',#37905,#37975,#28828,.T.);
#48703=EDGE_CURVE('',#37906,#37974,#28829,.T.);
#48704=EDGE_CURVE('',#37907,#37973,#28830,.T.);
#48705=EDGE_CURVE('',#37972,#37908,#28831,.T.);
#48706=EDGE_CURVE('',#37810,#37968,#28832,.T.);
#48707=EDGE_CURVE('',#37811,#37967,#28833,.T.);
#48708=EDGE_CURVE('',#37909,#37971,#28834,.T.);
#48709=EDGE_CURVE('',#37910,#37970,#28835,.T.);
#48710=EDGE_CURVE('',#37911,#37969,#28836,.T.);
#48711=EDGE_CURVE('',#37912,#38017,#28837,.T.);
#48712=EDGE_CURVE('',#38017,#38017,#20403,.T.);
#66724=ORIENTED_EDGE('',*,*,#47864,.T.);
#66725=ORIENTED_EDGE('',*,*,#47865,.T.);
#66726=ORIENTED_EDGE('',*,*,#47866,.F.);
#66727=ORIENTED_EDGE('',*,*,#47867,.F.);
#66728=ORIENTED_EDGE('',*,*,#47868,.F.);
#66729=ORIENTED_EDGE('',*,*,#47869,.T.);
#66730=ORIENTED_EDGE('',*,*,#47867,.T.);
#66731=ORIENTED_EDGE('',*,*,#47870,.F.);
#66732=ORIENTED_EDGE('',*,*,#47871,.F.);
#66733=ORIENTED_EDGE('',*,*,#47872,.F.);
#66734=ORIENTED_EDGE('',*,*,#47865,.F.);
#66735=ORIENTED_EDGE('',*,*,#47873,.F.);
#66736=ORIENTED_EDGE('',*,*,#47874,.T.);
#66737=ORIENTED_EDGE('',*,*,#47875,.F.);
#66738=ORIENTED_EDGE('',*,*,#47871,.T.);
#66739=ORIENTED_EDGE('',*,*,#47876,.T.);
#66740=ORIENTED_EDGE('',*,*,#47877,.T.);
#66741=ORIENTED_EDGE('',*,*,#47878,.T.);
#66742=ORIENTED_EDGE('',*,*,#47879,.F.);
#66743=ORIENTED_EDGE('',*,*,#47880,.F.);
#66744=ORIENTED_EDGE('',*,*,#47881,.F.);
#66745=ORIENTED_EDGE('',*,*,#47882,.F.);
#66746=ORIENTED_EDGE('',*,*,#47878,.F.);
#66747=ORIENTED_EDGE('',*,*,#47883,.F.);
#66748=ORIENTED_EDGE('',*,*,#47874,.F.);
#66749=ORIENTED_EDGE('',*,*,#47884,.T.);
#66750=ORIENTED_EDGE('',*,*,#47880,.T.);
#66751=ORIENTED_EDGE('',*,*,#47885,.F.);
#66752=ORIENTED_EDGE('',*,*,#47886,.T.);
#66753=ORIENTED_EDGE('',*,*,#47887,.F.);
#66754=ORIENTED_EDGE('',*,*,#47881,.T.);
#66755=ORIENTED_EDGE('',*,*,#47888,.T.);
#66756=ORIENTED_EDGE('',*,*,#47889,.T.);
#66757=ORIENTED_EDGE('',*,*,#47890,.T.);
#66758=ORIENTED_EDGE('',*,*,#47891,.F.);
#66759=ORIENTED_EDGE('',*,*,#47892,.F.);
#66760=ORIENTED_EDGE('',*,*,#47886,.F.);
#66761=ORIENTED_EDGE('',*,*,#47893,.T.);
#66762=ORIENTED_EDGE('',*,*,#47892,.T.);
#66763=ORIENTED_EDGE('',*,*,#47894,.F.);
#66764=ORIENTED_EDGE('',*,*,#47895,.F.);
#66765=ORIENTED_EDGE('',*,*,#47896,.F.);
#66766=ORIENTED_EDGE('',*,*,#47890,.F.);
#66767=ORIENTED_EDGE('',*,*,#47897,.F.);
#66768=ORIENTED_EDGE('',*,*,#47898,.T.);
#66769=ORIENTED_EDGE('',*,*,#47899,.F.);
#66770=ORIENTED_EDGE('',*,*,#47895,.T.);
#66771=ORIENTED_EDGE('',*,*,#47900,.T.);
#66772=ORIENTED_EDGE('',*,*,#47901,.T.);
#66773=ORIENTED_EDGE('',*,*,#47902,.T.);
#66774=ORIENTED_EDGE('',*,*,#47903,.F.);
#66775=ORIENTED_EDGE('',*,*,#47904,.F.);
#66776=ORIENTED_EDGE('',*,*,#47905,.F.);
#66777=ORIENTED_EDGE('',*,*,#47906,.F.);
#66778=ORIENTED_EDGE('',*,*,#47902,.F.);
#66779=ORIENTED_EDGE('',*,*,#47907,.F.);
#66780=ORIENTED_EDGE('',*,*,#47898,.F.);
#66781=ORIENTED_EDGE('',*,*,#47908,.T.);
#66782=ORIENTED_EDGE('',*,*,#47904,.T.);
#66783=ORIENTED_EDGE('',*,*,#47909,.F.);
#66784=ORIENTED_EDGE('',*,*,#47910,.T.);
#66785=ORIENTED_EDGE('',*,*,#47911,.F.);
#66786=ORIENTED_EDGE('',*,*,#47905,.T.);
#66787=ORIENTED_EDGE('',*,*,#47912,.T.);
#66788=ORIENTED_EDGE('',*,*,#47913,.T.);
#66789=ORIENTED_EDGE('',*,*,#47914,.T.);
#66790=ORIENTED_EDGE('',*,*,#47915,.F.);
#66791=ORIENTED_EDGE('',*,*,#47916,.F.);
#66792=ORIENTED_EDGE('',*,*,#47910,.F.);
#66793=ORIENTED_EDGE('',*,*,#47917,.T.);
#66794=ORIENTED_EDGE('',*,*,#47916,.T.);
#66795=ORIENTED_EDGE('',*,*,#47918,.F.);
#66796=ORIENTED_EDGE('',*,*,#47919,.F.);
#66797=ORIENTED_EDGE('',*,*,#47920,.F.);
#66798=ORIENTED_EDGE('',*,*,#47914,.F.);
#66799=ORIENTED_EDGE('',*,*,#47921,.F.);
#66800=ORIENTED_EDGE('',*,*,#47922,.T.);
#66801=ORIENTED_EDGE('',*,*,#47923,.F.);
#66802=ORIENTED_EDGE('',*,*,#47919,.T.);
#66803=ORIENTED_EDGE('',*,*,#47924,.T.);
#66804=ORIENTED_EDGE('',*,*,#47925,.T.);
#66805=ORIENTED_EDGE('',*,*,#47926,.T.);
#66806=ORIENTED_EDGE('',*,*,#47927,.F.);
#66807=ORIENTED_EDGE('',*,*,#47928,.F.);
#66808=ORIENTED_EDGE('',*,*,#47929,.F.);
#66809=ORIENTED_EDGE('',*,*,#47930,.F.);
#66810=ORIENTED_EDGE('',*,*,#47926,.F.);
#66811=ORIENTED_EDGE('',*,*,#47931,.F.);
#66812=ORIENTED_EDGE('',*,*,#47922,.F.);
#66813=ORIENTED_EDGE('',*,*,#47932,.T.);
#66814=ORIENTED_EDGE('',*,*,#47928,.T.);
#66815=ORIENTED_EDGE('',*,*,#47933,.F.);
#66816=ORIENTED_EDGE('',*,*,#47934,.T.);
#66817=ORIENTED_EDGE('',*,*,#47935,.F.);
#66818=ORIENTED_EDGE('',*,*,#47929,.T.);
#66819=ORIENTED_EDGE('',*,*,#47936,.T.);
#66820=ORIENTED_EDGE('',*,*,#47937,.T.);
#66821=ORIENTED_EDGE('',*,*,#47938,.T.);
#66822=ORIENTED_EDGE('',*,*,#47939,.F.);
#66823=ORIENTED_EDGE('',*,*,#47940,.F.);
#66824=ORIENTED_EDGE('',*,*,#47934,.F.);
#66825=ORIENTED_EDGE('',*,*,#47941,.T.);
#66826=ORIENTED_EDGE('',*,*,#47940,.T.);
#66827=ORIENTED_EDGE('',*,*,#47942,.F.);
#66828=ORIENTED_EDGE('',*,*,#47943,.F.);
#66829=ORIENTED_EDGE('',*,*,#47944,.F.);
#66830=ORIENTED_EDGE('',*,*,#47938,.F.);
#66831=ORIENTED_EDGE('',*,*,#47945,.F.);
#66832=ORIENTED_EDGE('',*,*,#47946,.T.);
#66833=ORIENTED_EDGE('',*,*,#47947,.F.);
#66834=ORIENTED_EDGE('',*,*,#47943,.T.);
#66835=ORIENTED_EDGE('',*,*,#47948,.T.);
#66836=ORIENTED_EDGE('',*,*,#47949,.T.);
#66837=ORIENTED_EDGE('',*,*,#47950,.T.);
#66838=ORIENTED_EDGE('',*,*,#47951,.F.);
#66839=ORIENTED_EDGE('',*,*,#47952,.F.);
#66840=ORIENTED_EDGE('',*,*,#47953,.F.);
#66841=ORIENTED_EDGE('',*,*,#47954,.F.);
#66842=ORIENTED_EDGE('',*,*,#47950,.F.);
#66843=ORIENTED_EDGE('',*,*,#47955,.F.);
#66844=ORIENTED_EDGE('',*,*,#47946,.F.);
#66845=ORIENTED_EDGE('',*,*,#47956,.T.);
#66846=ORIENTED_EDGE('',*,*,#47952,.T.);
#66847=ORIENTED_EDGE('',*,*,#47957,.F.);
#66848=ORIENTED_EDGE('',*,*,#47958,.T.);
#66849=ORIENTED_EDGE('',*,*,#47959,.F.);
#66850=ORIENTED_EDGE('',*,*,#47953,.T.);
#66851=ORIENTED_EDGE('',*,*,#47960,.T.);
#66852=ORIENTED_EDGE('',*,*,#47961,.T.);
#66853=ORIENTED_EDGE('',*,*,#47962,.T.);
#66854=ORIENTED_EDGE('',*,*,#47963,.F.);
#66855=ORIENTED_EDGE('',*,*,#47964,.F.);
#66856=ORIENTED_EDGE('',*,*,#47958,.F.);
#66857=ORIENTED_EDGE('',*,*,#47965,.T.);
#66858=ORIENTED_EDGE('',*,*,#47964,.T.);
#66859=ORIENTED_EDGE('',*,*,#47966,.F.);
#66860=ORIENTED_EDGE('',*,*,#47967,.F.);
#66861=ORIENTED_EDGE('',*,*,#47968,.F.);
#66862=ORIENTED_EDGE('',*,*,#47962,.F.);
#66863=ORIENTED_EDGE('',*,*,#47969,.F.);
#66864=ORIENTED_EDGE('',*,*,#47970,.T.);
#66865=ORIENTED_EDGE('',*,*,#47971,.F.);
#66866=ORIENTED_EDGE('',*,*,#47967,.T.);
#66867=ORIENTED_EDGE('',*,*,#47972,.T.);
#66868=ORIENTED_EDGE('',*,*,#47973,.T.);
#66869=ORIENTED_EDGE('',*,*,#47974,.T.);
#66870=ORIENTED_EDGE('',*,*,#47975,.F.);
#66871=ORIENTED_EDGE('',*,*,#47976,.F.);
#66872=ORIENTED_EDGE('',*,*,#47977,.F.);
#66873=ORIENTED_EDGE('',*,*,#47978,.F.);
#66874=ORIENTED_EDGE('',*,*,#47974,.F.);
#66875=ORIENTED_EDGE('',*,*,#47979,.F.);
#66876=ORIENTED_EDGE('',*,*,#47970,.F.);
#66877=ORIENTED_EDGE('',*,*,#47980,.T.);
#66878=ORIENTED_EDGE('',*,*,#47976,.T.);
#66879=ORIENTED_EDGE('',*,*,#47981,.F.);
#66880=ORIENTED_EDGE('',*,*,#47982,.T.);
#66881=ORIENTED_EDGE('',*,*,#47983,.F.);
#66882=ORIENTED_EDGE('',*,*,#47977,.T.);
#66883=ORIENTED_EDGE('',*,*,#47984,.T.);
#66884=ORIENTED_EDGE('',*,*,#47985,.T.);
#66885=ORIENTED_EDGE('',*,*,#47986,.T.);
#66886=ORIENTED_EDGE('',*,*,#47987,.F.);
#66887=ORIENTED_EDGE('',*,*,#47988,.F.);
#66888=ORIENTED_EDGE('',*,*,#47982,.F.);
#66889=ORIENTED_EDGE('',*,*,#47989,.T.);
#66890=ORIENTED_EDGE('',*,*,#47988,.T.);
#66891=ORIENTED_EDGE('',*,*,#47990,.F.);
#66892=ORIENTED_EDGE('',*,*,#47991,.F.);
#66893=ORIENTED_EDGE('',*,*,#47992,.F.);
#66894=ORIENTED_EDGE('',*,*,#47986,.F.);
#66895=ORIENTED_EDGE('',*,*,#47993,.F.);
#66896=ORIENTED_EDGE('',*,*,#47994,.T.);
#66897=ORIENTED_EDGE('',*,*,#47995,.F.);
#66898=ORIENTED_EDGE('',*,*,#47991,.T.);
#66899=ORIENTED_EDGE('',*,*,#47996,.T.);
#66900=ORIENTED_EDGE('',*,*,#47997,.T.);
#66901=ORIENTED_EDGE('',*,*,#47998,.T.);
#66902=ORIENTED_EDGE('',*,*,#47999,.F.);
#66903=ORIENTED_EDGE('',*,*,#48000,.F.);
#66904=ORIENTED_EDGE('',*,*,#48001,.F.);
#66905=ORIENTED_EDGE('',*,*,#48002,.F.);
#66906=ORIENTED_EDGE('',*,*,#47998,.F.);
#66907=ORIENTED_EDGE('',*,*,#48003,.F.);
#66908=ORIENTED_EDGE('',*,*,#47994,.F.);
#66909=ORIENTED_EDGE('',*,*,#48004,.T.);
#66910=ORIENTED_EDGE('',*,*,#48000,.T.);
#66911=ORIENTED_EDGE('',*,*,#48005,.F.);
#66912=ORIENTED_EDGE('',*,*,#48006,.T.);
#66913=ORIENTED_EDGE('',*,*,#48007,.F.);
#66914=ORIENTED_EDGE('',*,*,#48001,.T.);
#66915=ORIENTED_EDGE('',*,*,#48008,.T.);
#66916=ORIENTED_EDGE('',*,*,#48009,.T.);
#66917=ORIENTED_EDGE('',*,*,#48010,.T.);
#66918=ORIENTED_EDGE('',*,*,#48011,.F.);
#66919=ORIENTED_EDGE('',*,*,#48012,.F.);
#66920=ORIENTED_EDGE('',*,*,#48006,.F.);
#66921=ORIENTED_EDGE('',*,*,#48013,.T.);
#66922=ORIENTED_EDGE('',*,*,#48012,.T.);
#66923=ORIENTED_EDGE('',*,*,#48014,.F.);
#66924=ORIENTED_EDGE('',*,*,#48015,.F.);
#66925=ORIENTED_EDGE('',*,*,#48016,.F.);
#66926=ORIENTED_EDGE('',*,*,#48010,.F.);
#66927=ORIENTED_EDGE('',*,*,#48017,.F.);
#66928=ORIENTED_EDGE('',*,*,#48018,.T.);
#66929=ORIENTED_EDGE('',*,*,#48019,.F.);
#66930=ORIENTED_EDGE('',*,*,#48015,.T.);
#66931=ORIENTED_EDGE('',*,*,#48020,.T.);
#66932=ORIENTED_EDGE('',*,*,#48021,.T.);
#66933=ORIENTED_EDGE('',*,*,#48022,.T.);
#66934=ORIENTED_EDGE('',*,*,#48023,.F.);
#66935=ORIENTED_EDGE('',*,*,#48024,.F.);
#66936=ORIENTED_EDGE('',*,*,#48025,.F.);
#66937=ORIENTED_EDGE('',*,*,#48026,.F.);
#66938=ORIENTED_EDGE('',*,*,#48022,.F.);
#66939=ORIENTED_EDGE('',*,*,#48027,.F.);
#66940=ORIENTED_EDGE('',*,*,#48018,.F.);
#66941=ORIENTED_EDGE('',*,*,#48028,.T.);
#66942=ORIENTED_EDGE('',*,*,#48024,.T.);
#66943=ORIENTED_EDGE('',*,*,#48029,.F.);
#66944=ORIENTED_EDGE('',*,*,#48030,.T.);
#66945=ORIENTED_EDGE('',*,*,#48031,.F.);
#66946=ORIENTED_EDGE('',*,*,#48025,.T.);
#66947=ORIENTED_EDGE('',*,*,#48032,.T.);
#66948=ORIENTED_EDGE('',*,*,#48033,.T.);
#66949=ORIENTED_EDGE('',*,*,#48034,.T.);
#66950=ORIENTED_EDGE('',*,*,#48035,.F.);
#66951=ORIENTED_EDGE('',*,*,#48036,.F.);
#66952=ORIENTED_EDGE('',*,*,#48030,.F.);
#66953=ORIENTED_EDGE('',*,*,#48037,.T.);
#66954=ORIENTED_EDGE('',*,*,#48036,.T.);
#66955=ORIENTED_EDGE('',*,*,#48038,.F.);
#66956=ORIENTED_EDGE('',*,*,#48039,.F.);
#66957=ORIENTED_EDGE('',*,*,#48040,.F.);
#66958=ORIENTED_EDGE('',*,*,#48034,.F.);
#66959=ORIENTED_EDGE('',*,*,#48041,.F.);
#66960=ORIENTED_EDGE('',*,*,#48042,.T.);
#66961=ORIENTED_EDGE('',*,*,#48043,.F.);
#66962=ORIENTED_EDGE('',*,*,#48039,.T.);
#66963=ORIENTED_EDGE('',*,*,#48044,.T.);
#66964=ORIENTED_EDGE('',*,*,#48045,.T.);
#66965=ORIENTED_EDGE('',*,*,#48046,.T.);
#66966=ORIENTED_EDGE('',*,*,#48047,.F.);
#66967=ORIENTED_EDGE('',*,*,#48048,.F.);
#66968=ORIENTED_EDGE('',*,*,#48049,.F.);
#66969=ORIENTED_EDGE('',*,*,#48050,.F.);
#66970=ORIENTED_EDGE('',*,*,#48046,.F.);
#66971=ORIENTED_EDGE('',*,*,#48051,.F.);
#66972=ORIENTED_EDGE('',*,*,#48042,.F.);
#66973=ORIENTED_EDGE('',*,*,#48052,.T.);
#66974=ORIENTED_EDGE('',*,*,#48048,.T.);
#66975=ORIENTED_EDGE('',*,*,#48053,.F.);
#66976=ORIENTED_EDGE('',*,*,#48054,.T.);
#66977=ORIENTED_EDGE('',*,*,#48055,.F.);
#66978=ORIENTED_EDGE('',*,*,#48049,.T.);
#66979=ORIENTED_EDGE('',*,*,#48056,.T.);
#66980=ORIENTED_EDGE('',*,*,#48057,.T.);
#66981=ORIENTED_EDGE('',*,*,#48058,.T.);
#66982=ORIENTED_EDGE('',*,*,#48059,.F.);
#66983=ORIENTED_EDGE('',*,*,#48060,.F.);
#66984=ORIENTED_EDGE('',*,*,#48054,.F.);
#66985=ORIENTED_EDGE('',*,*,#48061,.T.);
#66986=ORIENTED_EDGE('',*,*,#48060,.T.);
#66987=ORIENTED_EDGE('',*,*,#48062,.F.);
#66988=ORIENTED_EDGE('',*,*,#48063,.F.);
#66989=ORIENTED_EDGE('',*,*,#48064,.F.);
#66990=ORIENTED_EDGE('',*,*,#48058,.F.);
#66991=ORIENTED_EDGE('',*,*,#48065,.F.);
#66992=ORIENTED_EDGE('',*,*,#48066,.T.);
#66993=ORIENTED_EDGE('',*,*,#48067,.F.);
#66994=ORIENTED_EDGE('',*,*,#48063,.T.);
#66995=ORIENTED_EDGE('',*,*,#48068,.T.);
#66996=ORIENTED_EDGE('',*,*,#48069,.T.);
#66997=ORIENTED_EDGE('',*,*,#48070,.T.);
#66998=ORIENTED_EDGE('',*,*,#48071,.F.);
#66999=ORIENTED_EDGE('',*,*,#48072,.F.);
#67000=ORIENTED_EDGE('',*,*,#48073,.F.);
#67001=ORIENTED_EDGE('',*,*,#48074,.F.);
#67002=ORIENTED_EDGE('',*,*,#48070,.F.);
#67003=ORIENTED_EDGE('',*,*,#48075,.F.);
#67004=ORIENTED_EDGE('',*,*,#48066,.F.);
#67005=ORIENTED_EDGE('',*,*,#48076,.T.);
#67006=ORIENTED_EDGE('',*,*,#48072,.T.);
#67007=ORIENTED_EDGE('',*,*,#48077,.F.);
#67008=ORIENTED_EDGE('',*,*,#48078,.T.);
#67009=ORIENTED_EDGE('',*,*,#48079,.F.);
#67010=ORIENTED_EDGE('',*,*,#48073,.T.);
#67011=ORIENTED_EDGE('',*,*,#48080,.T.);
#67012=ORIENTED_EDGE('',*,*,#48081,.T.);
#67013=ORIENTED_EDGE('',*,*,#48082,.T.);
#67014=ORIENTED_EDGE('',*,*,#48083,.F.);
#67015=ORIENTED_EDGE('',*,*,#48084,.F.);
#67016=ORIENTED_EDGE('',*,*,#48078,.F.);
#67017=ORIENTED_EDGE('',*,*,#48085,.T.);
#67018=ORIENTED_EDGE('',*,*,#48084,.T.);
#67019=ORIENTED_EDGE('',*,*,#48086,.F.);
#67020=ORIENTED_EDGE('',*,*,#48087,.F.);
#67021=ORIENTED_EDGE('',*,*,#48088,.F.);
#67022=ORIENTED_EDGE('',*,*,#48082,.F.);
#67023=ORIENTED_EDGE('',*,*,#48089,.F.);
#67024=ORIENTED_EDGE('',*,*,#48090,.T.);
#67025=ORIENTED_EDGE('',*,*,#48091,.F.);
#67026=ORIENTED_EDGE('',*,*,#48087,.T.);
#67027=ORIENTED_EDGE('',*,*,#48092,.T.);
#67028=ORIENTED_EDGE('',*,*,#48093,.T.);
#67029=ORIENTED_EDGE('',*,*,#48094,.T.);
#67030=ORIENTED_EDGE('',*,*,#48095,.F.);
#67031=ORIENTED_EDGE('',*,*,#48096,.F.);
#67032=ORIENTED_EDGE('',*,*,#48097,.F.);
#67033=ORIENTED_EDGE('',*,*,#48098,.F.);
#67034=ORIENTED_EDGE('',*,*,#48094,.F.);
#67035=ORIENTED_EDGE('',*,*,#48099,.F.);
#67036=ORIENTED_EDGE('',*,*,#48090,.F.);
#67037=ORIENTED_EDGE('',*,*,#48100,.T.);
#67038=ORIENTED_EDGE('',*,*,#48096,.T.);
#67039=ORIENTED_EDGE('',*,*,#48101,.F.);
#67040=ORIENTED_EDGE('',*,*,#48102,.T.);
#67041=ORIENTED_EDGE('',*,*,#48103,.F.);
#67042=ORIENTED_EDGE('',*,*,#48097,.T.);
#67043=ORIENTED_EDGE('',*,*,#48104,.T.);
#67044=ORIENTED_EDGE('',*,*,#48105,.T.);
#67045=ORIENTED_EDGE('',*,*,#48106,.T.);
#67046=ORIENTED_EDGE('',*,*,#48107,.F.);
#67047=ORIENTED_EDGE('',*,*,#48108,.F.);
#67048=ORIENTED_EDGE('',*,*,#48102,.F.);
#67049=ORIENTED_EDGE('',*,*,#48109,.T.);
#67050=ORIENTED_EDGE('',*,*,#48108,.T.);
#67051=ORIENTED_EDGE('',*,*,#48110,.F.);
#67052=ORIENTED_EDGE('',*,*,#48111,.F.);
#67053=ORIENTED_EDGE('',*,*,#48112,.F.);
#67054=ORIENTED_EDGE('',*,*,#48106,.F.);
#67055=ORIENTED_EDGE('',*,*,#48113,.F.);
#67056=ORIENTED_EDGE('',*,*,#48114,.T.);
#67057=ORIENTED_EDGE('',*,*,#48115,.F.);
#67058=ORIENTED_EDGE('',*,*,#48111,.T.);
#67059=ORIENTED_EDGE('',*,*,#48116,.T.);
#67060=ORIENTED_EDGE('',*,*,#48117,.T.);
#67061=ORIENTED_EDGE('',*,*,#48118,.T.);
#67062=ORIENTED_EDGE('',*,*,#48119,.F.);
#67063=ORIENTED_EDGE('',*,*,#48120,.F.);
#67064=ORIENTED_EDGE('',*,*,#48121,.F.);
#67065=ORIENTED_EDGE('',*,*,#48122,.F.);
#67066=ORIENTED_EDGE('',*,*,#48118,.F.);
#67067=ORIENTED_EDGE('',*,*,#48123,.F.);
#67068=ORIENTED_EDGE('',*,*,#48114,.F.);
#67069=ORIENTED_EDGE('',*,*,#48124,.T.);
#67070=ORIENTED_EDGE('',*,*,#48120,.T.);
#67071=ORIENTED_EDGE('',*,*,#48125,.F.);
#67072=ORIENTED_EDGE('',*,*,#48126,.T.);
#67073=ORIENTED_EDGE('',*,*,#48127,.F.);
#67074=ORIENTED_EDGE('',*,*,#48121,.T.);
#67075=ORIENTED_EDGE('',*,*,#48128,.T.);
#67076=ORIENTED_EDGE('',*,*,#48129,.T.);
#67077=ORIENTED_EDGE('',*,*,#48130,.T.);
#67078=ORIENTED_EDGE('',*,*,#48131,.F.);
#67079=ORIENTED_EDGE('',*,*,#48132,.F.);
#67080=ORIENTED_EDGE('',*,*,#48126,.F.);
#67081=ORIENTED_EDGE('',*,*,#48133,.T.);
#67082=ORIENTED_EDGE('',*,*,#48132,.T.);
#67083=ORIENTED_EDGE('',*,*,#48134,.F.);
#67084=ORIENTED_EDGE('',*,*,#48135,.F.);
#67085=ORIENTED_EDGE('',*,*,#48136,.F.);
#67086=ORIENTED_EDGE('',*,*,#48130,.F.);
#67087=ORIENTED_EDGE('',*,*,#48137,.F.);
#67088=ORIENTED_EDGE('',*,*,#48138,.T.);
#67089=ORIENTED_EDGE('',*,*,#48139,.F.);
#67090=ORIENTED_EDGE('',*,*,#48135,.T.);
#67091=ORIENTED_EDGE('',*,*,#48140,.T.);
#67092=ORIENTED_EDGE('',*,*,#48141,.T.);
#67093=ORIENTED_EDGE('',*,*,#48142,.T.);
#67094=ORIENTED_EDGE('',*,*,#48143,.F.);
#67095=ORIENTED_EDGE('',*,*,#48144,.F.);
#67096=ORIENTED_EDGE('',*,*,#48145,.F.);
#67097=ORIENTED_EDGE('',*,*,#48146,.F.);
#67098=ORIENTED_EDGE('',*,*,#48142,.F.);
#67099=ORIENTED_EDGE('',*,*,#48147,.F.);
#67100=ORIENTED_EDGE('',*,*,#48138,.F.);
#67101=ORIENTED_EDGE('',*,*,#48148,.T.);
#67102=ORIENTED_EDGE('',*,*,#48144,.T.);
#67103=ORIENTED_EDGE('',*,*,#48149,.F.);
#67104=ORIENTED_EDGE('',*,*,#48150,.T.);
#67105=ORIENTED_EDGE('',*,*,#48151,.F.);
#67106=ORIENTED_EDGE('',*,*,#48145,.T.);
#67107=ORIENTED_EDGE('',*,*,#48152,.T.);
#67108=ORIENTED_EDGE('',*,*,#48153,.T.);
#67109=ORIENTED_EDGE('',*,*,#48154,.T.);
#67110=ORIENTED_EDGE('',*,*,#48155,.F.);
#67111=ORIENTED_EDGE('',*,*,#48156,.F.);
#67112=ORIENTED_EDGE('',*,*,#48150,.F.);
#67113=ORIENTED_EDGE('',*,*,#48157,.T.);
#67114=ORIENTED_EDGE('',*,*,#48156,.T.);
#67115=ORIENTED_EDGE('',*,*,#48158,.F.);
#67116=ORIENTED_EDGE('',*,*,#48159,.F.);
#67117=ORIENTED_EDGE('',*,*,#48160,.F.);
#67118=ORIENTED_EDGE('',*,*,#48154,.F.);
#67119=ORIENTED_EDGE('',*,*,#48161,.F.);
#67120=ORIENTED_EDGE('',*,*,#48162,.T.);
#67121=ORIENTED_EDGE('',*,*,#48163,.F.);
#67122=ORIENTED_EDGE('',*,*,#48159,.T.);
#67123=ORIENTED_EDGE('',*,*,#48164,.T.);
#67124=ORIENTED_EDGE('',*,*,#48165,.T.);
#67125=ORIENTED_EDGE('',*,*,#48166,.T.);
#67126=ORIENTED_EDGE('',*,*,#48167,.F.);
#67127=ORIENTED_EDGE('',*,*,#48168,.F.);
#67128=ORIENTED_EDGE('',*,*,#48169,.F.);
#67129=ORIENTED_EDGE('',*,*,#48170,.F.);
#67130=ORIENTED_EDGE('',*,*,#48166,.F.);
#67131=ORIENTED_EDGE('',*,*,#48171,.F.);
#67132=ORIENTED_EDGE('',*,*,#48162,.F.);
#67133=ORIENTED_EDGE('',*,*,#48172,.T.);
#67134=ORIENTED_EDGE('',*,*,#48168,.T.);
#67135=ORIENTED_EDGE('',*,*,#48173,.F.);
#67136=ORIENTED_EDGE('',*,*,#48174,.T.);
#67137=ORIENTED_EDGE('',*,*,#48175,.F.);
#67138=ORIENTED_EDGE('',*,*,#48169,.T.);
#67139=ORIENTED_EDGE('',*,*,#48176,.T.);
#67140=ORIENTED_EDGE('',*,*,#48177,.T.);
#67141=ORIENTED_EDGE('',*,*,#48178,.T.);
#67142=ORIENTED_EDGE('',*,*,#48179,.F.);
#67143=ORIENTED_EDGE('',*,*,#48180,.F.);
#67144=ORIENTED_EDGE('',*,*,#48174,.F.);
#67145=ORIENTED_EDGE('',*,*,#48181,.T.);
#67146=ORIENTED_EDGE('',*,*,#48180,.T.);
#67147=ORIENTED_EDGE('',*,*,#48182,.F.);
#67148=ORIENTED_EDGE('',*,*,#48183,.F.);
#67149=ORIENTED_EDGE('',*,*,#48184,.F.);
#67150=ORIENTED_EDGE('',*,*,#48178,.F.);
#67151=ORIENTED_EDGE('',*,*,#48185,.F.);
#67152=ORIENTED_EDGE('',*,*,#48186,.T.);
#67153=ORIENTED_EDGE('',*,*,#48187,.F.);
#67154=ORIENTED_EDGE('',*,*,#48183,.T.);
#67155=ORIENTED_EDGE('',*,*,#48188,.T.);
#67156=ORIENTED_EDGE('',*,*,#48189,.T.);
#67157=ORIENTED_EDGE('',*,*,#48190,.T.);
#67158=ORIENTED_EDGE('',*,*,#48191,.F.);
#67159=ORIENTED_EDGE('',*,*,#48192,.F.);
#67160=ORIENTED_EDGE('',*,*,#48193,.F.);
#67161=ORIENTED_EDGE('',*,*,#48194,.F.);
#67162=ORIENTED_EDGE('',*,*,#48190,.F.);
#67163=ORIENTED_EDGE('',*,*,#48195,.F.);
#67164=ORIENTED_EDGE('',*,*,#48186,.F.);
#67165=ORIENTED_EDGE('',*,*,#48196,.T.);
#67166=ORIENTED_EDGE('',*,*,#48192,.T.);
#67167=ORIENTED_EDGE('',*,*,#48197,.F.);
#67168=ORIENTED_EDGE('',*,*,#48198,.T.);
#67169=ORIENTED_EDGE('',*,*,#48199,.F.);
#67170=ORIENTED_EDGE('',*,*,#48193,.T.);
#67171=ORIENTED_EDGE('',*,*,#48200,.T.);
#67172=ORIENTED_EDGE('',*,*,#48201,.T.);
#67173=ORIENTED_EDGE('',*,*,#48202,.T.);
#67174=ORIENTED_EDGE('',*,*,#48203,.F.);
#67175=ORIENTED_EDGE('',*,*,#48204,.F.);
#67176=ORIENTED_EDGE('',*,*,#48198,.F.);
#67177=ORIENTED_EDGE('',*,*,#48205,.T.);
#67178=ORIENTED_EDGE('',*,*,#48204,.T.);
#67179=ORIENTED_EDGE('',*,*,#48206,.F.);
#67180=ORIENTED_EDGE('',*,*,#48207,.F.);
#67181=ORIENTED_EDGE('',*,*,#48208,.F.);
#67182=ORIENTED_EDGE('',*,*,#48202,.F.);
#67183=ORIENTED_EDGE('',*,*,#48209,.F.);
#67184=ORIENTED_EDGE('',*,*,#48210,.T.);
#67185=ORIENTED_EDGE('',*,*,#48211,.F.);
#67186=ORIENTED_EDGE('',*,*,#48207,.T.);
#67187=ORIENTED_EDGE('',*,*,#48212,.T.);
#67188=ORIENTED_EDGE('',*,*,#48213,.T.);
#67189=ORIENTED_EDGE('',*,*,#48214,.T.);
#67190=ORIENTED_EDGE('',*,*,#48215,.F.);
#67191=ORIENTED_EDGE('',*,*,#48216,.F.);
#67192=ORIENTED_EDGE('',*,*,#48217,.F.);
#67193=ORIENTED_EDGE('',*,*,#48218,.F.);
#67194=ORIENTED_EDGE('',*,*,#48214,.F.);
#67195=ORIENTED_EDGE('',*,*,#48219,.F.);
#67196=ORIENTED_EDGE('',*,*,#48210,.F.);
#67197=ORIENTED_EDGE('',*,*,#48220,.T.);
#67198=ORIENTED_EDGE('',*,*,#48216,.T.);
#67199=ORIENTED_EDGE('',*,*,#48221,.F.);
#67200=ORIENTED_EDGE('',*,*,#48222,.T.);
#67201=ORIENTED_EDGE('',*,*,#48223,.F.);
#67202=ORIENTED_EDGE('',*,*,#48217,.T.);
#67203=ORIENTED_EDGE('',*,*,#48224,.T.);
#67204=ORIENTED_EDGE('',*,*,#48225,.T.);
#67205=ORIENTED_EDGE('',*,*,#48226,.T.);
#67206=ORIENTED_EDGE('',*,*,#48227,.F.);
#67207=ORIENTED_EDGE('',*,*,#48228,.F.);
#67208=ORIENTED_EDGE('',*,*,#48222,.F.);
#67209=ORIENTED_EDGE('',*,*,#48229,.T.);
#67210=ORIENTED_EDGE('',*,*,#48228,.T.);
#67211=ORIENTED_EDGE('',*,*,#48230,.F.);
#67212=ORIENTED_EDGE('',*,*,#48231,.F.);
#67213=ORIENTED_EDGE('',*,*,#48232,.F.);
#67214=ORIENTED_EDGE('',*,*,#48226,.F.);
#67215=ORIENTED_EDGE('',*,*,#48233,.F.);
#67216=ORIENTED_EDGE('',*,*,#48234,.T.);
#67217=ORIENTED_EDGE('',*,*,#48235,.F.);
#67218=ORIENTED_EDGE('',*,*,#48231,.T.);
#67219=ORIENTED_EDGE('',*,*,#48236,.T.);
#67220=ORIENTED_EDGE('',*,*,#48237,.T.);
#67221=ORIENTED_EDGE('',*,*,#48238,.T.);
#67222=ORIENTED_EDGE('',*,*,#48239,.F.);
#67223=ORIENTED_EDGE('',*,*,#48240,.F.);
#67224=ORIENTED_EDGE('',*,*,#48241,.F.);
#67225=ORIENTED_EDGE('',*,*,#48242,.F.);
#67226=ORIENTED_EDGE('',*,*,#48238,.F.);
#67227=ORIENTED_EDGE('',*,*,#48243,.F.);
#67228=ORIENTED_EDGE('',*,*,#48234,.F.);
#67229=ORIENTED_EDGE('',*,*,#48244,.T.);
#67230=ORIENTED_EDGE('',*,*,#48240,.T.);
#67231=ORIENTED_EDGE('',*,*,#48245,.F.);
#67232=ORIENTED_EDGE('',*,*,#48246,.T.);
#67233=ORIENTED_EDGE('',*,*,#48247,.F.);
#67234=ORIENTED_EDGE('',*,*,#48241,.T.);
#67235=ORIENTED_EDGE('',*,*,#48248,.T.);
#67236=ORIENTED_EDGE('',*,*,#48249,.T.);
#67237=ORIENTED_EDGE('',*,*,#48250,.T.);
#67238=ORIENTED_EDGE('',*,*,#48251,.F.);
#67239=ORIENTED_EDGE('',*,*,#48252,.F.);
#67240=ORIENTED_EDGE('',*,*,#48246,.F.);
#67241=ORIENTED_EDGE('',*,*,#48253,.T.);
#67242=ORIENTED_EDGE('',*,*,#48252,.T.);
#67243=ORIENTED_EDGE('',*,*,#48254,.F.);
#67244=ORIENTED_EDGE('',*,*,#48255,.F.);
#67245=ORIENTED_EDGE('',*,*,#48256,.F.);
#67246=ORIENTED_EDGE('',*,*,#48250,.F.);
#67247=ORIENTED_EDGE('',*,*,#48257,.F.);
#67248=ORIENTED_EDGE('',*,*,#48258,.T.);
#67249=ORIENTED_EDGE('',*,*,#48259,.F.);
#67250=ORIENTED_EDGE('',*,*,#48255,.T.);
#67251=ORIENTED_EDGE('',*,*,#48260,.T.);
#67252=ORIENTED_EDGE('',*,*,#48261,.T.);
#67253=ORIENTED_EDGE('',*,*,#48262,.T.);
#67254=ORIENTED_EDGE('',*,*,#48263,.F.);
#67255=ORIENTED_EDGE('',*,*,#48264,.F.);
#67256=ORIENTED_EDGE('',*,*,#48265,.F.);
#67257=ORIENTED_EDGE('',*,*,#48266,.F.);
#67258=ORIENTED_EDGE('',*,*,#48262,.F.);
#67259=ORIENTED_EDGE('',*,*,#48267,.F.);
#67260=ORIENTED_EDGE('',*,*,#48258,.F.);
#67261=ORIENTED_EDGE('',*,*,#48268,.T.);
#67262=ORIENTED_EDGE('',*,*,#48264,.T.);
#67263=ORIENTED_EDGE('',*,*,#48269,.F.);
#67264=ORIENTED_EDGE('',*,*,#48270,.T.);
#67265=ORIENTED_EDGE('',*,*,#48271,.F.);
#67266=ORIENTED_EDGE('',*,*,#48265,.T.);
#67267=ORIENTED_EDGE('',*,*,#48272,.T.);
#67268=ORIENTED_EDGE('',*,*,#48273,.T.);
#67269=ORIENTED_EDGE('',*,*,#48274,.T.);
#67270=ORIENTED_EDGE('',*,*,#48275,.F.);
#67271=ORIENTED_EDGE('',*,*,#48276,.F.);
#67272=ORIENTED_EDGE('',*,*,#48270,.F.);
#67273=ORIENTED_EDGE('',*,*,#48277,.T.);
#67274=ORIENTED_EDGE('',*,*,#48276,.T.);
#67275=ORIENTED_EDGE('',*,*,#48278,.F.);
#67276=ORIENTED_EDGE('',*,*,#48279,.F.);
#67277=ORIENTED_EDGE('',*,*,#48280,.F.);
#67278=ORIENTED_EDGE('',*,*,#48274,.F.);
#67279=ORIENTED_EDGE('',*,*,#48281,.F.);
#67280=ORIENTED_EDGE('',*,*,#48282,.T.);
#67281=ORIENTED_EDGE('',*,*,#48283,.F.);
#67282=ORIENTED_EDGE('',*,*,#48279,.T.);
#67283=ORIENTED_EDGE('',*,*,#48284,.T.);
#67284=ORIENTED_EDGE('',*,*,#48285,.T.);
#67285=ORIENTED_EDGE('',*,*,#48286,.T.);
#67286=ORIENTED_EDGE('',*,*,#48287,.F.);
#67287=ORIENTED_EDGE('',*,*,#48288,.F.);
#67288=ORIENTED_EDGE('',*,*,#48289,.F.);
#67289=ORIENTED_EDGE('',*,*,#48290,.F.);
#67290=ORIENTED_EDGE('',*,*,#48286,.F.);
#67291=ORIENTED_EDGE('',*,*,#48291,.F.);
#67292=ORIENTED_EDGE('',*,*,#48282,.F.);
#67293=ORIENTED_EDGE('',*,*,#48292,.T.);
#67294=ORIENTED_EDGE('',*,*,#48288,.T.);
#67295=ORIENTED_EDGE('',*,*,#48293,.F.);
#67296=ORIENTED_EDGE('',*,*,#48294,.T.);
#67297=ORIENTED_EDGE('',*,*,#48295,.F.);
#67298=ORIENTED_EDGE('',*,*,#48289,.T.);
#67299=ORIENTED_EDGE('',*,*,#48296,.T.);
#67300=ORIENTED_EDGE('',*,*,#48297,.T.);
#67301=ORIENTED_EDGE('',*,*,#48298,.T.);
#67302=ORIENTED_EDGE('',*,*,#48299,.F.);
#67303=ORIENTED_EDGE('',*,*,#48300,.F.);
#67304=ORIENTED_EDGE('',*,*,#48294,.F.);
#67305=ORIENTED_EDGE('',*,*,#48301,.T.);
#67306=ORIENTED_EDGE('',*,*,#48300,.T.);
#67307=ORIENTED_EDGE('',*,*,#48302,.F.);
#67308=ORIENTED_EDGE('',*,*,#48303,.F.);
#67309=ORIENTED_EDGE('',*,*,#48304,.F.);
#67310=ORIENTED_EDGE('',*,*,#48298,.F.);
#67311=ORIENTED_EDGE('',*,*,#48305,.F.);
#67312=ORIENTED_EDGE('',*,*,#48306,.T.);
#67313=ORIENTED_EDGE('',*,*,#48307,.F.);
#67314=ORIENTED_EDGE('',*,*,#48303,.T.);
#67315=ORIENTED_EDGE('',*,*,#48308,.T.);
#67316=ORIENTED_EDGE('',*,*,#48309,.T.);
#67317=ORIENTED_EDGE('',*,*,#48310,.T.);
#67318=ORIENTED_EDGE('',*,*,#48311,.F.);
#67319=ORIENTED_EDGE('',*,*,#48312,.F.);
#67320=ORIENTED_EDGE('',*,*,#48313,.F.);
#67321=ORIENTED_EDGE('',*,*,#48314,.F.);
#67322=ORIENTED_EDGE('',*,*,#48310,.F.);
#67323=ORIENTED_EDGE('',*,*,#48315,.F.);
#67324=ORIENTED_EDGE('',*,*,#48306,.F.);
#67325=ORIENTED_EDGE('',*,*,#48316,.T.);
#67326=ORIENTED_EDGE('',*,*,#48312,.T.);
#67327=ORIENTED_EDGE('',*,*,#48317,.F.);
#67328=ORIENTED_EDGE('',*,*,#48318,.T.);
#67329=ORIENTED_EDGE('',*,*,#48319,.F.);
#67330=ORIENTED_EDGE('',*,*,#48313,.T.);
#67331=ORIENTED_EDGE('',*,*,#48320,.T.);
#67332=ORIENTED_EDGE('',*,*,#48321,.T.);
#67333=ORIENTED_EDGE('',*,*,#48322,.T.);
#67334=ORIENTED_EDGE('',*,*,#48323,.F.);
#67335=ORIENTED_EDGE('',*,*,#48324,.F.);
#67336=ORIENTED_EDGE('',*,*,#48318,.F.);
#67337=ORIENTED_EDGE('',*,*,#48325,.T.);
#67338=ORIENTED_EDGE('',*,*,#48324,.T.);
#67339=ORIENTED_EDGE('',*,*,#48326,.F.);
#67340=ORIENTED_EDGE('',*,*,#48327,.F.);
#67341=ORIENTED_EDGE('',*,*,#48328,.F.);
#67342=ORIENTED_EDGE('',*,*,#48322,.F.);
#67343=ORIENTED_EDGE('',*,*,#48329,.F.);
#67344=ORIENTED_EDGE('',*,*,#48330,.T.);
#67345=ORIENTED_EDGE('',*,*,#48331,.F.);
#67346=ORIENTED_EDGE('',*,*,#48327,.T.);
#67347=ORIENTED_EDGE('',*,*,#48332,.T.);
#67348=ORIENTED_EDGE('',*,*,#48333,.T.);
#67349=ORIENTED_EDGE('',*,*,#48334,.T.);
#67350=ORIENTED_EDGE('',*,*,#48335,.F.);
#67351=ORIENTED_EDGE('',*,*,#48336,.F.);
#67352=ORIENTED_EDGE('',*,*,#48337,.F.);
#67353=ORIENTED_EDGE('',*,*,#48338,.F.);
#67354=ORIENTED_EDGE('',*,*,#48334,.F.);
#67355=ORIENTED_EDGE('',*,*,#48339,.F.);
#67356=ORIENTED_EDGE('',*,*,#48330,.F.);
#67357=ORIENTED_EDGE('',*,*,#48340,.T.);
#67358=ORIENTED_EDGE('',*,*,#48336,.T.);
#67359=ORIENTED_EDGE('',*,*,#48341,.F.);
#67360=ORIENTED_EDGE('',*,*,#48342,.T.);
#67361=ORIENTED_EDGE('',*,*,#48343,.F.);
#67362=ORIENTED_EDGE('',*,*,#48337,.T.);
#67363=ORIENTED_EDGE('',*,*,#48344,.T.);
#67364=ORIENTED_EDGE('',*,*,#48345,.T.);
#67365=ORIENTED_EDGE('',*,*,#48346,.T.);
#67366=ORIENTED_EDGE('',*,*,#48347,.F.);
#67367=ORIENTED_EDGE('',*,*,#48348,.F.);
#67368=ORIENTED_EDGE('',*,*,#48342,.F.);
#67369=ORIENTED_EDGE('',*,*,#48349,.T.);
#67370=ORIENTED_EDGE('',*,*,#48348,.T.);
#67371=ORIENTED_EDGE('',*,*,#48350,.F.);
#67372=ORIENTED_EDGE('',*,*,#48351,.F.);
#67373=ORIENTED_EDGE('',*,*,#48352,.F.);
#67374=ORIENTED_EDGE('',*,*,#48346,.F.);
#67375=ORIENTED_EDGE('',*,*,#48353,.F.);
#67376=ORIENTED_EDGE('',*,*,#48354,.T.);
#67377=ORIENTED_EDGE('',*,*,#48355,.F.);
#67378=ORIENTED_EDGE('',*,*,#48351,.T.);
#67379=ORIENTED_EDGE('',*,*,#48356,.T.);
#67380=ORIENTED_EDGE('',*,*,#48357,.T.);
#67381=ORIENTED_EDGE('',*,*,#48358,.T.);
#67382=ORIENTED_EDGE('',*,*,#48359,.F.);
#67383=ORIENTED_EDGE('',*,*,#48360,.F.);
#67384=ORIENTED_EDGE('',*,*,#48361,.F.);
#67385=ORIENTED_EDGE('',*,*,#48362,.F.);
#67386=ORIENTED_EDGE('',*,*,#48358,.F.);
#67387=ORIENTED_EDGE('',*,*,#48363,.F.);
#67388=ORIENTED_EDGE('',*,*,#48354,.F.);
#67389=ORIENTED_EDGE('',*,*,#48364,.T.);
#67390=ORIENTED_EDGE('',*,*,#48360,.T.);
#67391=ORIENTED_EDGE('',*,*,#48365,.F.);
#67392=ORIENTED_EDGE('',*,*,#48366,.T.);
#67393=ORIENTED_EDGE('',*,*,#48367,.F.);
#67394=ORIENTED_EDGE('',*,*,#48361,.T.);
#67395=ORIENTED_EDGE('',*,*,#48368,.T.);
#67396=ORIENTED_EDGE('',*,*,#48369,.T.);
#67397=ORIENTED_EDGE('',*,*,#48370,.T.);
#67398=ORIENTED_EDGE('',*,*,#48371,.F.);
#67399=ORIENTED_EDGE('',*,*,#48372,.F.);
#67400=ORIENTED_EDGE('',*,*,#48366,.F.);
#67401=ORIENTED_EDGE('',*,*,#48373,.T.);
#67402=ORIENTED_EDGE('',*,*,#48372,.T.);
#67403=ORIENTED_EDGE('',*,*,#48374,.F.);
#67404=ORIENTED_EDGE('',*,*,#48375,.F.);
#67405=ORIENTED_EDGE('',*,*,#48376,.F.);
#67406=ORIENTED_EDGE('',*,*,#48370,.F.);
#67407=ORIENTED_EDGE('',*,*,#48377,.F.);
#67408=ORIENTED_EDGE('',*,*,#48378,.F.);
#67409=ORIENTED_EDGE('',*,*,#48377,.T.);
#67410=ORIENTED_EDGE('',*,*,#48369,.F.);
#67411=ORIENTED_EDGE('',*,*,#48373,.F.);
#67412=ORIENTED_EDGE('',*,*,#48368,.F.);
#67413=ORIENTED_EDGE('',*,*,#48363,.T.);
#67414=ORIENTED_EDGE('',*,*,#48357,.F.);
#67415=ORIENTED_EDGE('',*,*,#48364,.F.);
#67416=ORIENTED_EDGE('',*,*,#48356,.F.);
#67417=ORIENTED_EDGE('',*,*,#48353,.T.);
#67418=ORIENTED_EDGE('',*,*,#48345,.F.);
#67419=ORIENTED_EDGE('',*,*,#48349,.F.);
#67420=ORIENTED_EDGE('',*,*,#48344,.F.);
#67421=ORIENTED_EDGE('',*,*,#48339,.T.);
#67422=ORIENTED_EDGE('',*,*,#48333,.F.);
#67423=ORIENTED_EDGE('',*,*,#48340,.F.);
#67424=ORIENTED_EDGE('',*,*,#48332,.F.);
#67425=ORIENTED_EDGE('',*,*,#48329,.T.);
#67426=ORIENTED_EDGE('',*,*,#48321,.F.);
#67427=ORIENTED_EDGE('',*,*,#48325,.F.);
#67428=ORIENTED_EDGE('',*,*,#48320,.F.);
#67429=ORIENTED_EDGE('',*,*,#48315,.T.);
#67430=ORIENTED_EDGE('',*,*,#48309,.F.);
#67431=ORIENTED_EDGE('',*,*,#48316,.F.);
#67432=ORIENTED_EDGE('',*,*,#48308,.F.);
#67433=ORIENTED_EDGE('',*,*,#48305,.T.);
#67434=ORIENTED_EDGE('',*,*,#48297,.F.);
#67435=ORIENTED_EDGE('',*,*,#48301,.F.);
#67436=ORIENTED_EDGE('',*,*,#48296,.F.);
#67437=ORIENTED_EDGE('',*,*,#48291,.T.);
#67438=ORIENTED_EDGE('',*,*,#48285,.F.);
#67439=ORIENTED_EDGE('',*,*,#48292,.F.);
#67440=ORIENTED_EDGE('',*,*,#48284,.F.);
#67441=ORIENTED_EDGE('',*,*,#48281,.T.);
#67442=ORIENTED_EDGE('',*,*,#48273,.F.);
#67443=ORIENTED_EDGE('',*,*,#48277,.F.);
#67444=ORIENTED_EDGE('',*,*,#48272,.F.);
#67445=ORIENTED_EDGE('',*,*,#48267,.T.);
#67446=ORIENTED_EDGE('',*,*,#48261,.F.);
#67447=ORIENTED_EDGE('',*,*,#48268,.F.);
#67448=ORIENTED_EDGE('',*,*,#48260,.F.);
#67449=ORIENTED_EDGE('',*,*,#48257,.T.);
#67450=ORIENTED_EDGE('',*,*,#48249,.F.);
#67451=ORIENTED_EDGE('',*,*,#48253,.F.);
#67452=ORIENTED_EDGE('',*,*,#48248,.F.);
#67453=ORIENTED_EDGE('',*,*,#48243,.T.);
#67454=ORIENTED_EDGE('',*,*,#48237,.F.);
#67455=ORIENTED_EDGE('',*,*,#48244,.F.);
#67456=ORIENTED_EDGE('',*,*,#48236,.F.);
#67457=ORIENTED_EDGE('',*,*,#48233,.T.);
#67458=ORIENTED_EDGE('',*,*,#48225,.F.);
#67459=ORIENTED_EDGE('',*,*,#48229,.F.);
#67460=ORIENTED_EDGE('',*,*,#48224,.F.);
#67461=ORIENTED_EDGE('',*,*,#48219,.T.);
#67462=ORIENTED_EDGE('',*,*,#48213,.F.);
#67463=ORIENTED_EDGE('',*,*,#48220,.F.);
#67464=ORIENTED_EDGE('',*,*,#48212,.F.);
#67465=ORIENTED_EDGE('',*,*,#48209,.T.);
#67466=ORIENTED_EDGE('',*,*,#48201,.F.);
#67467=ORIENTED_EDGE('',*,*,#48205,.F.);
#67468=ORIENTED_EDGE('',*,*,#48200,.F.);
#67469=ORIENTED_EDGE('',*,*,#48195,.T.);
#67470=ORIENTED_EDGE('',*,*,#48189,.F.);
#67471=ORIENTED_EDGE('',*,*,#48196,.F.);
#67472=ORIENTED_EDGE('',*,*,#48188,.F.);
#67473=ORIENTED_EDGE('',*,*,#48185,.T.);
#67474=ORIENTED_EDGE('',*,*,#48177,.F.);
#67475=ORIENTED_EDGE('',*,*,#48181,.F.);
#67476=ORIENTED_EDGE('',*,*,#48176,.F.);
#67477=ORIENTED_EDGE('',*,*,#48171,.T.);
#67478=ORIENTED_EDGE('',*,*,#48165,.F.);
#67479=ORIENTED_EDGE('',*,*,#48172,.F.);
#67480=ORIENTED_EDGE('',*,*,#48164,.F.);
#67481=ORIENTED_EDGE('',*,*,#48161,.T.);
#67482=ORIENTED_EDGE('',*,*,#48153,.F.);
#67483=ORIENTED_EDGE('',*,*,#48157,.F.);
#67484=ORIENTED_EDGE('',*,*,#48152,.F.);
#67485=ORIENTED_EDGE('',*,*,#48147,.T.);
#67486=ORIENTED_EDGE('',*,*,#48141,.F.);
#67487=ORIENTED_EDGE('',*,*,#48148,.F.);
#67488=ORIENTED_EDGE('',*,*,#48140,.F.);
#67489=ORIENTED_EDGE('',*,*,#48137,.T.);
#67490=ORIENTED_EDGE('',*,*,#48129,.F.);
#67491=ORIENTED_EDGE('',*,*,#48133,.F.);
#67492=ORIENTED_EDGE('',*,*,#48128,.F.);
#67493=ORIENTED_EDGE('',*,*,#48123,.T.);
#67494=ORIENTED_EDGE('',*,*,#48117,.F.);
#67495=ORIENTED_EDGE('',*,*,#48124,.F.);
#67496=ORIENTED_EDGE('',*,*,#48116,.F.);
#67497=ORIENTED_EDGE('',*,*,#48113,.T.);
#67498=ORIENTED_EDGE('',*,*,#48105,.F.);
#67499=ORIENTED_EDGE('',*,*,#48109,.F.);
#67500=ORIENTED_EDGE('',*,*,#48104,.F.);
#67501=ORIENTED_EDGE('',*,*,#48099,.T.);
#67502=ORIENTED_EDGE('',*,*,#48093,.F.);
#67503=ORIENTED_EDGE('',*,*,#48100,.F.);
#67504=ORIENTED_EDGE('',*,*,#48092,.F.);
#67505=ORIENTED_EDGE('',*,*,#48089,.T.);
#67506=ORIENTED_EDGE('',*,*,#48081,.F.);
#67507=ORIENTED_EDGE('',*,*,#48085,.F.);
#67508=ORIENTED_EDGE('',*,*,#48080,.F.);
#67509=ORIENTED_EDGE('',*,*,#48075,.T.);
#67510=ORIENTED_EDGE('',*,*,#48069,.F.);
#67511=ORIENTED_EDGE('',*,*,#48076,.F.);
#67512=ORIENTED_EDGE('',*,*,#48068,.F.);
#67513=ORIENTED_EDGE('',*,*,#48065,.T.);
#67514=ORIENTED_EDGE('',*,*,#48057,.F.);
#67515=ORIENTED_EDGE('',*,*,#48061,.F.);
#67516=ORIENTED_EDGE('',*,*,#48056,.F.);
#67517=ORIENTED_EDGE('',*,*,#48051,.T.);
#67518=ORIENTED_EDGE('',*,*,#48045,.F.);
#67519=ORIENTED_EDGE('',*,*,#48052,.F.);
#67520=ORIENTED_EDGE('',*,*,#48044,.F.);
#67521=ORIENTED_EDGE('',*,*,#48041,.T.);
#67522=ORIENTED_EDGE('',*,*,#48033,.F.);
#67523=ORIENTED_EDGE('',*,*,#48037,.F.);
#67524=ORIENTED_EDGE('',*,*,#48032,.F.);
#67525=ORIENTED_EDGE('',*,*,#48027,.T.);
#67526=ORIENTED_EDGE('',*,*,#48021,.F.);
#67527=ORIENTED_EDGE('',*,*,#48028,.F.);
#67528=ORIENTED_EDGE('',*,*,#48020,.F.);
#67529=ORIENTED_EDGE('',*,*,#48017,.T.);
#67530=ORIENTED_EDGE('',*,*,#48009,.F.);
#67531=ORIENTED_EDGE('',*,*,#48013,.F.);
#67532=ORIENTED_EDGE('',*,*,#48008,.F.);
#67533=ORIENTED_EDGE('',*,*,#48003,.T.);
#67534=ORIENTED_EDGE('',*,*,#47997,.F.);
#67535=ORIENTED_EDGE('',*,*,#48004,.F.);
#67536=ORIENTED_EDGE('',*,*,#47996,.F.);
#67537=ORIENTED_EDGE('',*,*,#47993,.T.);
#67538=ORIENTED_EDGE('',*,*,#47985,.F.);
#67539=ORIENTED_EDGE('',*,*,#47989,.F.);
#67540=ORIENTED_EDGE('',*,*,#47984,.F.);
#67541=ORIENTED_EDGE('',*,*,#47979,.T.);
#67542=ORIENTED_EDGE('',*,*,#47973,.F.);
#67543=ORIENTED_EDGE('',*,*,#47980,.F.);
#67544=ORIENTED_EDGE('',*,*,#47972,.F.);
#67545=ORIENTED_EDGE('',*,*,#47969,.T.);
#67546=ORIENTED_EDGE('',*,*,#47961,.F.);
#67547=ORIENTED_EDGE('',*,*,#47965,.F.);
#67548=ORIENTED_EDGE('',*,*,#47960,.F.);
#67549=ORIENTED_EDGE('',*,*,#47955,.T.);
#67550=ORIENTED_EDGE('',*,*,#47949,.F.);
#67551=ORIENTED_EDGE('',*,*,#47956,.F.);
#67552=ORIENTED_EDGE('',*,*,#47948,.F.);
#67553=ORIENTED_EDGE('',*,*,#47945,.T.);
#67554=ORIENTED_EDGE('',*,*,#47937,.F.);
#67555=ORIENTED_EDGE('',*,*,#47941,.F.);
#67556=ORIENTED_EDGE('',*,*,#47936,.F.);
#67557=ORIENTED_EDGE('',*,*,#47931,.T.);
#67558=ORIENTED_EDGE('',*,*,#47925,.F.);
#67559=ORIENTED_EDGE('',*,*,#47932,.F.);
#67560=ORIENTED_EDGE('',*,*,#47924,.F.);
#67561=ORIENTED_EDGE('',*,*,#47921,.T.);
#67562=ORIENTED_EDGE('',*,*,#47913,.F.);
#67563=ORIENTED_EDGE('',*,*,#47917,.F.);
#67564=ORIENTED_EDGE('',*,*,#47912,.F.);
#67565=ORIENTED_EDGE('',*,*,#47907,.T.);
#67566=ORIENTED_EDGE('',*,*,#47901,.F.);
#67567=ORIENTED_EDGE('',*,*,#47908,.F.);
#67568=ORIENTED_EDGE('',*,*,#47900,.F.);
#67569=ORIENTED_EDGE('',*,*,#47897,.T.);
#67570=ORIENTED_EDGE('',*,*,#47889,.F.);
#67571=ORIENTED_EDGE('',*,*,#47893,.F.);
#67572=ORIENTED_EDGE('',*,*,#47888,.F.);
#67573=ORIENTED_EDGE('',*,*,#47883,.T.);
#67574=ORIENTED_EDGE('',*,*,#47877,.F.);
#67575=ORIENTED_EDGE('',*,*,#47884,.F.);
#67576=ORIENTED_EDGE('',*,*,#47876,.F.);
#67577=ORIENTED_EDGE('',*,*,#47873,.T.);
#67578=ORIENTED_EDGE('',*,*,#47864,.F.);
#67579=ORIENTED_EDGE('',*,*,#47869,.F.);
#67580=ORIENTED_EDGE('',*,*,#48379,.F.);
#67581=ORIENTED_EDGE('',*,*,#48380,.T.);
#67582=ORIENTED_EDGE('',*,*,#48381,.F.);
#67583=ORIENTED_EDGE('',*,*,#48382,.F.);
#67584=ORIENTED_EDGE('',*,*,#48383,.T.);
#67585=ORIENTED_EDGE('',*,*,#48384,.T.);
#67586=ORIENTED_EDGE('',*,*,#48379,.T.);
#67587=ORIENTED_EDGE('',*,*,#47868,.T.);
#67588=ORIENTED_EDGE('',*,*,#48385,.F.);
#67589=ORIENTED_EDGE('',*,*,#48386,.T.);
#67590=ORIENTED_EDGE('',*,*,#48387,.F.);
#67591=ORIENTED_EDGE('',*,*,#48375,.T.);
#67592=ORIENTED_EDGE('',*,*,#48378,.T.);
#67593=ORIENTED_EDGE('',*,*,#48381,.T.);
#67594=ORIENTED_EDGE('',*,*,#48388,.T.);
#67595=ORIENTED_EDGE('',*,*,#48389,.F.);
#67596=ORIENTED_EDGE('',*,*,#48390,.F.);
#67597=ORIENTED_EDGE('',*,*,#48384,.F.);
#67598=ORIENTED_EDGE('',*,*,#48391,.F.);
#67599=ORIENTED_EDGE('',*,*,#48388,.F.);
#67600=ORIENTED_EDGE('',*,*,#48380,.F.);
#67601=ORIENTED_EDGE('',*,*,#48386,.F.);
#67602=ORIENTED_EDGE('',*,*,#48382,.T.);
#67603=ORIENTED_EDGE('',*,*,#48390,.T.);
#67604=ORIENTED_EDGE('',*,*,#48392,.F.);
#67605=ORIENTED_EDGE('',*,*,#48383,.F.);
#67606=ORIENTED_EDGE('',*,*,#48393,.T.);
#67607=ORIENTED_EDGE('',*,*,#48394,.T.);
#67608=ORIENTED_EDGE('',*,*,#48393,.F.);
#67609=ORIENTED_EDGE('',*,*,#48385,.T.);
#67610=ORIENTED_EDGE('',*,*,#47870,.T.);
#67611=ORIENTED_EDGE('',*,*,#47866,.T.);
#67612=ORIENTED_EDGE('',*,*,#47872,.T.);
#67613=ORIENTED_EDGE('',*,*,#47875,.T.);
#67614=ORIENTED_EDGE('',*,*,#47885,.T.);
#67615=ORIENTED_EDGE('',*,*,#47879,.T.);
#67616=ORIENTED_EDGE('',*,*,#47882,.T.);
#67617=ORIENTED_EDGE('',*,*,#47887,.T.);
#67618=ORIENTED_EDGE('',*,*,#47894,.T.);
#67619=ORIENTED_EDGE('',*,*,#47891,.T.);
#67620=ORIENTED_EDGE('',*,*,#47896,.T.);
#67621=ORIENTED_EDGE('',*,*,#47899,.T.);
#67622=ORIENTED_EDGE('',*,*,#47909,.T.);
#67623=ORIENTED_EDGE('',*,*,#47903,.T.);
#67624=ORIENTED_EDGE('',*,*,#47906,.T.);
#67625=ORIENTED_EDGE('',*,*,#47911,.T.);
#67626=ORIENTED_EDGE('',*,*,#47918,.T.);
#67627=ORIENTED_EDGE('',*,*,#47915,.T.);
#67628=ORIENTED_EDGE('',*,*,#47920,.T.);
#67629=ORIENTED_EDGE('',*,*,#47923,.T.);
#67630=ORIENTED_EDGE('',*,*,#47933,.T.);
#67631=ORIENTED_EDGE('',*,*,#47927,.T.);
#67632=ORIENTED_EDGE('',*,*,#47930,.T.);
#67633=ORIENTED_EDGE('',*,*,#47935,.T.);
#67634=ORIENTED_EDGE('',*,*,#47942,.T.);
#67635=ORIENTED_EDGE('',*,*,#47939,.T.);
#67636=ORIENTED_EDGE('',*,*,#47944,.T.);
#67637=ORIENTED_EDGE('',*,*,#47947,.T.);
#67638=ORIENTED_EDGE('',*,*,#47957,.T.);
#67639=ORIENTED_EDGE('',*,*,#47951,.T.);
#67640=ORIENTED_EDGE('',*,*,#47954,.T.);
#67641=ORIENTED_EDGE('',*,*,#47959,.T.);
#67642=ORIENTED_EDGE('',*,*,#47966,.T.);
#67643=ORIENTED_EDGE('',*,*,#47963,.T.);
#67644=ORIENTED_EDGE('',*,*,#47968,.T.);
#67645=ORIENTED_EDGE('',*,*,#47971,.T.);
#67646=ORIENTED_EDGE('',*,*,#47981,.T.);
#67647=ORIENTED_EDGE('',*,*,#47975,.T.);
#67648=ORIENTED_EDGE('',*,*,#47978,.T.);
#67649=ORIENTED_EDGE('',*,*,#47983,.T.);
#67650=ORIENTED_EDGE('',*,*,#47990,.T.);
#67651=ORIENTED_EDGE('',*,*,#47987,.T.);
#67652=ORIENTED_EDGE('',*,*,#47992,.T.);
#67653=ORIENTED_EDGE('',*,*,#47995,.T.);
#67654=ORIENTED_EDGE('',*,*,#48005,.T.);
#67655=ORIENTED_EDGE('',*,*,#47999,.T.);
#67656=ORIENTED_EDGE('',*,*,#48002,.T.);
#67657=ORIENTED_EDGE('',*,*,#48007,.T.);
#67658=ORIENTED_EDGE('',*,*,#48014,.T.);
#67659=ORIENTED_EDGE('',*,*,#48011,.T.);
#67660=ORIENTED_EDGE('',*,*,#48016,.T.);
#67661=ORIENTED_EDGE('',*,*,#48019,.T.);
#67662=ORIENTED_EDGE('',*,*,#48029,.T.);
#67663=ORIENTED_EDGE('',*,*,#48023,.T.);
#67664=ORIENTED_EDGE('',*,*,#48026,.T.);
#67665=ORIENTED_EDGE('',*,*,#48031,.T.);
#67666=ORIENTED_EDGE('',*,*,#48038,.T.);
#67667=ORIENTED_EDGE('',*,*,#48035,.T.);
#67668=ORIENTED_EDGE('',*,*,#48040,.T.);
#67669=ORIENTED_EDGE('',*,*,#48043,.T.);
#67670=ORIENTED_EDGE('',*,*,#48053,.T.);
#67671=ORIENTED_EDGE('',*,*,#48047,.T.);
#67672=ORIENTED_EDGE('',*,*,#48050,.T.);
#67673=ORIENTED_EDGE('',*,*,#48055,.T.);
#67674=ORIENTED_EDGE('',*,*,#48062,.T.);
#67675=ORIENTED_EDGE('',*,*,#48059,.T.);
#67676=ORIENTED_EDGE('',*,*,#48064,.T.);
#67677=ORIENTED_EDGE('',*,*,#48067,.T.);
#67678=ORIENTED_EDGE('',*,*,#48077,.T.);
#67679=ORIENTED_EDGE('',*,*,#48071,.T.);
#67680=ORIENTED_EDGE('',*,*,#48074,.T.);
#67681=ORIENTED_EDGE('',*,*,#48079,.T.);
#67682=ORIENTED_EDGE('',*,*,#48086,.T.);
#67683=ORIENTED_EDGE('',*,*,#48083,.T.);
#67684=ORIENTED_EDGE('',*,*,#48088,.T.);
#67685=ORIENTED_EDGE('',*,*,#48091,.T.);
#67686=ORIENTED_EDGE('',*,*,#48101,.T.);
#67687=ORIENTED_EDGE('',*,*,#48095,.T.);
#67688=ORIENTED_EDGE('',*,*,#48098,.T.);
#67689=ORIENTED_EDGE('',*,*,#48103,.T.);
#67690=ORIENTED_EDGE('',*,*,#48110,.T.);
#67691=ORIENTED_EDGE('',*,*,#48107,.T.);
#67692=ORIENTED_EDGE('',*,*,#48112,.T.);
#67693=ORIENTED_EDGE('',*,*,#48115,.T.);
#67694=ORIENTED_EDGE('',*,*,#48125,.T.);
#67695=ORIENTED_EDGE('',*,*,#48119,.T.);
#67696=ORIENTED_EDGE('',*,*,#48122,.T.);
#67697=ORIENTED_EDGE('',*,*,#48127,.T.);
#67698=ORIENTED_EDGE('',*,*,#48134,.T.);
#67699=ORIENTED_EDGE('',*,*,#48131,.T.);
#67700=ORIENTED_EDGE('',*,*,#48136,.T.);
#67701=ORIENTED_EDGE('',*,*,#48139,.T.);
#67702=ORIENTED_EDGE('',*,*,#48149,.T.);
#67703=ORIENTED_EDGE('',*,*,#48143,.T.);
#67704=ORIENTED_EDGE('',*,*,#48146,.T.);
#67705=ORIENTED_EDGE('',*,*,#48151,.T.);
#67706=ORIENTED_EDGE('',*,*,#48158,.T.);
#67707=ORIENTED_EDGE('',*,*,#48155,.T.);
#67708=ORIENTED_EDGE('',*,*,#48160,.T.);
#67709=ORIENTED_EDGE('',*,*,#48163,.T.);
#67710=ORIENTED_EDGE('',*,*,#48173,.T.);
#67711=ORIENTED_EDGE('',*,*,#48167,.T.);
#67712=ORIENTED_EDGE('',*,*,#48170,.T.);
#67713=ORIENTED_EDGE('',*,*,#48175,.T.);
#67714=ORIENTED_EDGE('',*,*,#48182,.T.);
#67715=ORIENTED_EDGE('',*,*,#48179,.T.);
#67716=ORIENTED_EDGE('',*,*,#48184,.T.);
#67717=ORIENTED_EDGE('',*,*,#48187,.T.);
#67718=ORIENTED_EDGE('',*,*,#48197,.T.);
#67719=ORIENTED_EDGE('',*,*,#48191,.T.);
#67720=ORIENTED_EDGE('',*,*,#48194,.T.);
#67721=ORIENTED_EDGE('',*,*,#48199,.T.);
#67722=ORIENTED_EDGE('',*,*,#48206,.T.);
#67723=ORIENTED_EDGE('',*,*,#48203,.T.);
#67724=ORIENTED_EDGE('',*,*,#48208,.T.);
#67725=ORIENTED_EDGE('',*,*,#48211,.T.);
#67726=ORIENTED_EDGE('',*,*,#48221,.T.);
#67727=ORIENTED_EDGE('',*,*,#48215,.T.);
#67728=ORIENTED_EDGE('',*,*,#48218,.T.);
#67729=ORIENTED_EDGE('',*,*,#48223,.T.);
#67730=ORIENTED_EDGE('',*,*,#48230,.T.);
#67731=ORIENTED_EDGE('',*,*,#48227,.T.);
#67732=ORIENTED_EDGE('',*,*,#48232,.T.);
#67733=ORIENTED_EDGE('',*,*,#48235,.T.);
#67734=ORIENTED_EDGE('',*,*,#48245,.T.);
#67735=ORIENTED_EDGE('',*,*,#48239,.T.);
#67736=ORIENTED_EDGE('',*,*,#48242,.T.);
#67737=ORIENTED_EDGE('',*,*,#48247,.T.);
#67738=ORIENTED_EDGE('',*,*,#48254,.T.);
#67739=ORIENTED_EDGE('',*,*,#48251,.T.);
#67740=ORIENTED_EDGE('',*,*,#48256,.T.);
#67741=ORIENTED_EDGE('',*,*,#48259,.T.);
#67742=ORIENTED_EDGE('',*,*,#48269,.T.);
#67743=ORIENTED_EDGE('',*,*,#48263,.T.);
#67744=ORIENTED_EDGE('',*,*,#48266,.T.);
#67745=ORIENTED_EDGE('',*,*,#48271,.T.);
#67746=ORIENTED_EDGE('',*,*,#48278,.T.);
#67747=ORIENTED_EDGE('',*,*,#48275,.T.);
#67748=ORIENTED_EDGE('',*,*,#48280,.T.);
#67749=ORIENTED_EDGE('',*,*,#48283,.T.);
#67750=ORIENTED_EDGE('',*,*,#48293,.T.);
#67751=ORIENTED_EDGE('',*,*,#48287,.T.);
#67752=ORIENTED_EDGE('',*,*,#48290,.T.);
#67753=ORIENTED_EDGE('',*,*,#48295,.T.);
#67754=ORIENTED_EDGE('',*,*,#48302,.T.);
#67755=ORIENTED_EDGE('',*,*,#48299,.T.);
#67756=ORIENTED_EDGE('',*,*,#48304,.T.);
#67757=ORIENTED_EDGE('',*,*,#48307,.T.);
#67758=ORIENTED_EDGE('',*,*,#48317,.T.);
#67759=ORIENTED_EDGE('',*,*,#48311,.T.);
#67760=ORIENTED_EDGE('',*,*,#48314,.T.);
#67761=ORIENTED_EDGE('',*,*,#48319,.T.);
#67762=ORIENTED_EDGE('',*,*,#48326,.T.);
#67763=ORIENTED_EDGE('',*,*,#48323,.T.);
#67764=ORIENTED_EDGE('',*,*,#48328,.T.);
#67765=ORIENTED_EDGE('',*,*,#48331,.T.);
#67766=ORIENTED_EDGE('',*,*,#48341,.T.);
#67767=ORIENTED_EDGE('',*,*,#48335,.T.);
#67768=ORIENTED_EDGE('',*,*,#48338,.T.);
#67769=ORIENTED_EDGE('',*,*,#48343,.T.);
#67770=ORIENTED_EDGE('',*,*,#48350,.T.);
#67771=ORIENTED_EDGE('',*,*,#48347,.T.);
#67772=ORIENTED_EDGE('',*,*,#48352,.T.);
#67773=ORIENTED_EDGE('',*,*,#48355,.T.);
#67774=ORIENTED_EDGE('',*,*,#48365,.T.);
#67775=ORIENTED_EDGE('',*,*,#48359,.T.);
#67776=ORIENTED_EDGE('',*,*,#48362,.T.);
#67777=ORIENTED_EDGE('',*,*,#48367,.T.);
#67778=ORIENTED_EDGE('',*,*,#48374,.T.);
#67779=ORIENTED_EDGE('',*,*,#48371,.T.);
#67780=ORIENTED_EDGE('',*,*,#48376,.T.);
#67781=ORIENTED_EDGE('',*,*,#48387,.T.);
#67782=ORIENTED_EDGE('',*,*,#48392,.T.);
#67783=ORIENTED_EDGE('',*,*,#48389,.T.);
#67784=ORIENTED_EDGE('',*,*,#48391,.T.);
#67785=ORIENTED_EDGE('',*,*,#48394,.F.);
#67786=ORIENTED_EDGE('',*,*,#48395,.F.);
#67787=ORIENTED_EDGE('',*,*,#48396,.T.);
#67788=ORIENTED_EDGE('',*,*,#48397,.F.);
#67789=ORIENTED_EDGE('',*,*,#48396,.F.);
#67790=ORIENTED_EDGE('',*,*,#48398,.F.);
#67791=ORIENTED_EDGE('',*,*,#48399,.T.);
#67792=ORIENTED_EDGE('',*,*,#48400,.F.);
#67793=ORIENTED_EDGE('',*,*,#48399,.F.);
#67794=ORIENTED_EDGE('',*,*,#48400,.T.);
#67795=ORIENTED_EDGE('',*,*,#48395,.T.);
#67796=ORIENTED_EDGE('',*,*,#48401,.T.);
#67797=ORIENTED_EDGE('',*,*,#48402,.T.);
#67798=ORIENTED_EDGE('',*,*,#48403,.T.);
#67799=ORIENTED_EDGE('',*,*,#48404,.T.);
#67800=ORIENTED_EDGE('',*,*,#48405,.T.);
#67801=ORIENTED_EDGE('',*,*,#48406,.T.);
#67802=ORIENTED_EDGE('',*,*,#48407,.T.);
#67803=ORIENTED_EDGE('',*,*,#48408,.T.);
#67804=ORIENTED_EDGE('',*,*,#48409,.T.);
#67805=ORIENTED_EDGE('',*,*,#48410,.T.);
#67806=ORIENTED_EDGE('',*,*,#48411,.T.);
#67807=ORIENTED_EDGE('',*,*,#48412,.T.);
#67808=ORIENTED_EDGE('',*,*,#48413,.T.);
#67809=ORIENTED_EDGE('',*,*,#48414,.T.);
#67810=ORIENTED_EDGE('',*,*,#48415,.T.);
#67811=ORIENTED_EDGE('',*,*,#48416,.T.);
#67812=ORIENTED_EDGE('',*,*,#48417,.T.);
#67813=ORIENTED_EDGE('',*,*,#48418,.T.);
#67814=ORIENTED_EDGE('',*,*,#48419,.T.);
#67815=ORIENTED_EDGE('',*,*,#48420,.T.);
#67816=ORIENTED_EDGE('',*,*,#48421,.T.);
#67817=ORIENTED_EDGE('',*,*,#48422,.T.);
#67818=ORIENTED_EDGE('',*,*,#48423,.T.);
#67819=ORIENTED_EDGE('',*,*,#48424,.T.);
#67820=ORIENTED_EDGE('',*,*,#48425,.T.);
#67821=ORIENTED_EDGE('',*,*,#48426,.T.);
#67822=ORIENTED_EDGE('',*,*,#48427,.T.);
#67823=ORIENTED_EDGE('',*,*,#48428,.T.);
#67824=ORIENTED_EDGE('',*,*,#48429,.T.);
#67825=ORIENTED_EDGE('',*,*,#48430,.T.);
#67826=ORIENTED_EDGE('',*,*,#48431,.T.);
#67827=ORIENTED_EDGE('',*,*,#48432,.T.);
#67828=ORIENTED_EDGE('',*,*,#48433,.T.);
#67829=ORIENTED_EDGE('',*,*,#48434,.T.);
#67830=ORIENTED_EDGE('',*,*,#48435,.T.);
#67831=ORIENTED_EDGE('',*,*,#48436,.T.);
#67832=ORIENTED_EDGE('',*,*,#48437,.T.);
#67833=ORIENTED_EDGE('',*,*,#48438,.T.);
#67834=ORIENTED_EDGE('',*,*,#48439,.T.);
#67835=ORIENTED_EDGE('',*,*,#48440,.T.);
#67836=ORIENTED_EDGE('',*,*,#48441,.T.);
#67837=ORIENTED_EDGE('',*,*,#48442,.T.);
#67838=ORIENTED_EDGE('',*,*,#48443,.T.);
#67839=ORIENTED_EDGE('',*,*,#48444,.T.);
#67840=ORIENTED_EDGE('',*,*,#48445,.T.);
#67841=ORIENTED_EDGE('',*,*,#48446,.T.);
#67842=ORIENTED_EDGE('',*,*,#48447,.T.);
#67843=ORIENTED_EDGE('',*,*,#48448,.T.);
#67844=ORIENTED_EDGE('',*,*,#48449,.T.);
#67845=ORIENTED_EDGE('',*,*,#48450,.T.);
#67846=ORIENTED_EDGE('',*,*,#48451,.T.);
#67847=ORIENTED_EDGE('',*,*,#48452,.T.);
#67848=ORIENTED_EDGE('',*,*,#48453,.T.);
#67849=ORIENTED_EDGE('',*,*,#48454,.T.);
#67850=ORIENTED_EDGE('',*,*,#48455,.T.);
#67851=ORIENTED_EDGE('',*,*,#48456,.T.);
#67852=ORIENTED_EDGE('',*,*,#48457,.T.);
#67853=ORIENTED_EDGE('',*,*,#48458,.T.);
#67854=ORIENTED_EDGE('',*,*,#48459,.T.);
#67855=ORIENTED_EDGE('',*,*,#48460,.T.);
#67856=ORIENTED_EDGE('',*,*,#48461,.T.);
#67857=ORIENTED_EDGE('',*,*,#48462,.T.);
#67858=ORIENTED_EDGE('',*,*,#48463,.T.);
#67859=ORIENTED_EDGE('',*,*,#48464,.T.);
#67860=ORIENTED_EDGE('',*,*,#48465,.T.);
#67861=ORIENTED_EDGE('',*,*,#48466,.T.);
#67862=ORIENTED_EDGE('',*,*,#48467,.T.);
#67863=ORIENTED_EDGE('',*,*,#48468,.T.);
#67864=ORIENTED_EDGE('',*,*,#48469,.T.);
#67865=ORIENTED_EDGE('',*,*,#48470,.T.);
#67866=ORIENTED_EDGE('',*,*,#48471,.T.);
#67867=ORIENTED_EDGE('',*,*,#48472,.T.);
#67868=ORIENTED_EDGE('',*,*,#48473,.T.);
#67869=ORIENTED_EDGE('',*,*,#48474,.T.);
#67870=ORIENTED_EDGE('',*,*,#48475,.T.);
#67871=ORIENTED_EDGE('',*,*,#48476,.T.);
#67872=ORIENTED_EDGE('',*,*,#48477,.T.);
#67873=ORIENTED_EDGE('',*,*,#48478,.T.);
#67874=ORIENTED_EDGE('',*,*,#48479,.T.);
#67875=ORIENTED_EDGE('',*,*,#48480,.T.);
#67876=ORIENTED_EDGE('',*,*,#48481,.T.);
#67877=ORIENTED_EDGE('',*,*,#48482,.T.);
#67878=ORIENTED_EDGE('',*,*,#48483,.T.);
#67879=ORIENTED_EDGE('',*,*,#48484,.T.);
#67880=ORIENTED_EDGE('',*,*,#48485,.T.);
#67881=ORIENTED_EDGE('',*,*,#48486,.T.);
#67882=ORIENTED_EDGE('',*,*,#48487,.T.);
#67883=ORIENTED_EDGE('',*,*,#48488,.T.);
#67884=ORIENTED_EDGE('',*,*,#48489,.T.);
#67885=ORIENTED_EDGE('',*,*,#48490,.T.);
#67886=ORIENTED_EDGE('',*,*,#48491,.T.);
#67887=ORIENTED_EDGE('',*,*,#48492,.T.);
#67888=ORIENTED_EDGE('',*,*,#48493,.T.);
#67889=ORIENTED_EDGE('',*,*,#48494,.T.);
#67890=ORIENTED_EDGE('',*,*,#48495,.T.);
#67891=ORIENTED_EDGE('',*,*,#48496,.T.);
#67892=ORIENTED_EDGE('',*,*,#48497,.T.);
#67893=ORIENTED_EDGE('',*,*,#48498,.T.);
#67894=ORIENTED_EDGE('',*,*,#48499,.T.);
#67895=ORIENTED_EDGE('',*,*,#48500,.T.);
#67896=ORIENTED_EDGE('',*,*,#48501,.T.);
#67897=ORIENTED_EDGE('',*,*,#48502,.T.);
#67898=ORIENTED_EDGE('',*,*,#48503,.T.);
#67899=ORIENTED_EDGE('',*,*,#48504,.F.);
#67900=ORIENTED_EDGE('',*,*,#48505,.T.);
#67901=ORIENTED_EDGE('',*,*,#48506,.F.);
#67902=ORIENTED_EDGE('',*,*,#48505,.F.);
#67903=ORIENTED_EDGE('',*,*,#48504,.T.);
#67904=ORIENTED_EDGE('',*,*,#48398,.T.);
#67905=ORIENTED_EDGE('',*,*,#48453,.F.);
#67906=ORIENTED_EDGE('',*,*,#48507,.T.);
#67907=ORIENTED_EDGE('',*,*,#48508,.F.);
#67908=ORIENTED_EDGE('',*,*,#48509,.F.);
#67909=ORIENTED_EDGE('',*,*,#48452,.F.);
#67910=ORIENTED_EDGE('',*,*,#48510,.T.);
#67911=ORIENTED_EDGE('',*,*,#48511,.F.);
#67912=ORIENTED_EDGE('',*,*,#48507,.F.);
#67913=ORIENTED_EDGE('',*,*,#48451,.F.);
#67914=ORIENTED_EDGE('',*,*,#48512,.F.);
#67915=ORIENTED_EDGE('',*,*,#48513,.F.);
#67916=ORIENTED_EDGE('',*,*,#48510,.F.);
#67917=ORIENTED_EDGE('',*,*,#48450,.F.);
#67918=ORIENTED_EDGE('',*,*,#48514,.T.);
#67919=ORIENTED_EDGE('',*,*,#48515,.F.);
#67920=ORIENTED_EDGE('',*,*,#48512,.T.);
#67921=ORIENTED_EDGE('',*,*,#48449,.F.);
#67922=ORIENTED_EDGE('',*,*,#48516,.T.);
#67923=ORIENTED_EDGE('',*,*,#48517,.F.);
#67924=ORIENTED_EDGE('',*,*,#48514,.F.);
#67925=ORIENTED_EDGE('',*,*,#48448,.F.);
#67926=ORIENTED_EDGE('',*,*,#48518,.T.);
#67927=ORIENTED_EDGE('',*,*,#48519,.F.);
#67928=ORIENTED_EDGE('',*,*,#48516,.F.);
#67929=ORIENTED_EDGE('',*,*,#48447,.F.);
#67930=ORIENTED_EDGE('',*,*,#48520,.T.);
#67931=ORIENTED_EDGE('',*,*,#48521,.F.);
#67932=ORIENTED_EDGE('',*,*,#48518,.F.);
#67933=ORIENTED_EDGE('',*,*,#48446,.F.);
#67934=ORIENTED_EDGE('',*,*,#48522,.T.);
#67935=ORIENTED_EDGE('',*,*,#48523,.F.);
#67936=ORIENTED_EDGE('',*,*,#48520,.F.);
#67937=ORIENTED_EDGE('',*,*,#48445,.F.);
#67938=ORIENTED_EDGE('',*,*,#48524,.F.);
#67939=ORIENTED_EDGE('',*,*,#48525,.F.);
#67940=ORIENTED_EDGE('',*,*,#48522,.F.);
#67941=ORIENTED_EDGE('',*,*,#48444,.F.);
#67942=ORIENTED_EDGE('',*,*,#48526,.T.);
#67943=ORIENTED_EDGE('',*,*,#48527,.F.);
#67944=ORIENTED_EDGE('',*,*,#48524,.T.);
#67945=ORIENTED_EDGE('',*,*,#48443,.F.);
#67946=ORIENTED_EDGE('',*,*,#48528,.T.);
#67947=ORIENTED_EDGE('',*,*,#48529,.F.);
#67948=ORIENTED_EDGE('',*,*,#48526,.F.);
#67949=ORIENTED_EDGE('',*,*,#48442,.F.);
#67950=ORIENTED_EDGE('',*,*,#48530,.T.);
#67951=ORIENTED_EDGE('',*,*,#48531,.F.);
#67952=ORIENTED_EDGE('',*,*,#48528,.F.);
#67953=ORIENTED_EDGE('',*,*,#48441,.F.);
#67954=ORIENTED_EDGE('',*,*,#48532,.T.);
#67955=ORIENTED_EDGE('',*,*,#48533,.F.);
#67956=ORIENTED_EDGE('',*,*,#48530,.F.);
#67957=ORIENTED_EDGE('',*,*,#48440,.F.);
#67958=ORIENTED_EDGE('',*,*,#48534,.T.);
#67959=ORIENTED_EDGE('',*,*,#48535,.F.);
#67960=ORIENTED_EDGE('',*,*,#48532,.F.);
#67961=ORIENTED_EDGE('',*,*,#48439,.F.);
#67962=ORIENTED_EDGE('',*,*,#48536,.F.);
#67963=ORIENTED_EDGE('',*,*,#48537,.F.);
#67964=ORIENTED_EDGE('',*,*,#48534,.F.);
#67965=ORIENTED_EDGE('',*,*,#48438,.F.);
#67966=ORIENTED_EDGE('',*,*,#48538,.T.);
#67967=ORIENTED_EDGE('',*,*,#48539,.F.);
#67968=ORIENTED_EDGE('',*,*,#48536,.T.);
#67969=ORIENTED_EDGE('',*,*,#48437,.F.);
#67970=ORIENTED_EDGE('',*,*,#48540,.T.);
#67971=ORIENTED_EDGE('',*,*,#48541,.F.);
#67972=ORIENTED_EDGE('',*,*,#48538,.F.);
#67973=ORIENTED_EDGE('',*,*,#48540,.F.);
#67974=ORIENTED_EDGE('',*,*,#48436,.F.);
#67975=ORIENTED_EDGE('',*,*,#48542,.T.);
#67976=ORIENTED_EDGE('',*,*,#48543,.F.);
#67977=ORIENTED_EDGE('',*,*,#48435,.F.);
#67978=ORIENTED_EDGE('',*,*,#48544,.T.);
#67979=ORIENTED_EDGE('',*,*,#48545,.F.);
#67980=ORIENTED_EDGE('',*,*,#48542,.F.);
#67981=ORIENTED_EDGE('',*,*,#48434,.F.);
#67982=ORIENTED_EDGE('',*,*,#48546,.T.);
#67983=ORIENTED_EDGE('',*,*,#48547,.F.);
#67984=ORIENTED_EDGE('',*,*,#48544,.F.);
#67985=ORIENTED_EDGE('',*,*,#48433,.F.);
#67986=ORIENTED_EDGE('',*,*,#48548,.F.);
#67987=ORIENTED_EDGE('',*,*,#48549,.F.);
#67988=ORIENTED_EDGE('',*,*,#48546,.F.);
#67989=ORIENTED_EDGE('',*,*,#48432,.F.);
#67990=ORIENTED_EDGE('',*,*,#48550,.T.);
#67991=ORIENTED_EDGE('',*,*,#48551,.F.);
#67992=ORIENTED_EDGE('',*,*,#48548,.T.);
#67993=ORIENTED_EDGE('',*,*,#48431,.F.);
#67994=ORIENTED_EDGE('',*,*,#48552,.T.);
#67995=ORIENTED_EDGE('',*,*,#48553,.F.);
#67996=ORIENTED_EDGE('',*,*,#48550,.F.);
#67997=ORIENTED_EDGE('',*,*,#48430,.F.);
#67998=ORIENTED_EDGE('',*,*,#48554,.T.);
#67999=ORIENTED_EDGE('',*,*,#48555,.F.);
#68000=ORIENTED_EDGE('',*,*,#48552,.F.);
#68001=ORIENTED_EDGE('',*,*,#48429,.F.);
#68002=ORIENTED_EDGE('',*,*,#48556,.T.);
#68003=ORIENTED_EDGE('',*,*,#48557,.F.);
#68004=ORIENTED_EDGE('',*,*,#48554,.F.);
#68005=ORIENTED_EDGE('',*,*,#48428,.F.);
#68006=ORIENTED_EDGE('',*,*,#48558,.T.);
#68007=ORIENTED_EDGE('',*,*,#48559,.F.);
#68008=ORIENTED_EDGE('',*,*,#48556,.F.);
#68009=ORIENTED_EDGE('',*,*,#48427,.F.);
#68010=ORIENTED_EDGE('',*,*,#48560,.F.);
#68011=ORIENTED_EDGE('',*,*,#48561,.F.);
#68012=ORIENTED_EDGE('',*,*,#48558,.F.);
#68013=ORIENTED_EDGE('',*,*,#48426,.F.);
#68014=ORIENTED_EDGE('',*,*,#48562,.T.);
#68015=ORIENTED_EDGE('',*,*,#48563,.F.);
#68016=ORIENTED_EDGE('',*,*,#48560,.T.);
#68017=ORIENTED_EDGE('',*,*,#48425,.F.);
#68018=ORIENTED_EDGE('',*,*,#48564,.T.);
#68019=ORIENTED_EDGE('',*,*,#48565,.F.);
#68020=ORIENTED_EDGE('',*,*,#48562,.F.);
#68021=ORIENTED_EDGE('',*,*,#48424,.F.);
#68022=ORIENTED_EDGE('',*,*,#48566,.T.);
#68023=ORIENTED_EDGE('',*,*,#48567,.F.);
#68024=ORIENTED_EDGE('',*,*,#48564,.F.);
#68025=ORIENTED_EDGE('',*,*,#48423,.F.);
#68026=ORIENTED_EDGE('',*,*,#48568,.T.);
#68027=ORIENTED_EDGE('',*,*,#48569,.F.);
#68028=ORIENTED_EDGE('',*,*,#48566,.F.);
#68029=ORIENTED_EDGE('',*,*,#48422,.F.);
#68030=ORIENTED_EDGE('',*,*,#48570,.T.);
#68031=ORIENTED_EDGE('',*,*,#48571,.F.);
#68032=ORIENTED_EDGE('',*,*,#48568,.F.);
#68033=ORIENTED_EDGE('',*,*,#48421,.F.);
#68034=ORIENTED_EDGE('',*,*,#48572,.F.);
#68035=ORIENTED_EDGE('',*,*,#48573,.F.);
#68036=ORIENTED_EDGE('',*,*,#48570,.F.);
#68037=ORIENTED_EDGE('',*,*,#48420,.F.);
#68038=ORIENTED_EDGE('',*,*,#48574,.T.);
#68039=ORIENTED_EDGE('',*,*,#48575,.F.);
#68040=ORIENTED_EDGE('',*,*,#48572,.T.);
#68041=ORIENTED_EDGE('',*,*,#48419,.F.);
#68042=ORIENTED_EDGE('',*,*,#48576,.T.);
#68043=ORIENTED_EDGE('',*,*,#48577,.F.);
#68044=ORIENTED_EDGE('',*,*,#48574,.F.);
#68045=ORIENTED_EDGE('',*,*,#48418,.F.);
#68046=ORIENTED_EDGE('',*,*,#48578,.T.);
#68047=ORIENTED_EDGE('',*,*,#48579,.F.);
#68048=ORIENTED_EDGE('',*,*,#48576,.F.);
#68049=ORIENTED_EDGE('',*,*,#48417,.F.);
#68050=ORIENTED_EDGE('',*,*,#48580,.T.);
#68051=ORIENTED_EDGE('',*,*,#48581,.F.);
#68052=ORIENTED_EDGE('',*,*,#48578,.F.);
#68053=ORIENTED_EDGE('',*,*,#48416,.F.);
#68054=ORIENTED_EDGE('',*,*,#48582,.T.);
#68055=ORIENTED_EDGE('',*,*,#48583,.F.);
#68056=ORIENTED_EDGE('',*,*,#48580,.F.);
#68057=ORIENTED_EDGE('',*,*,#48415,.F.);
#68058=ORIENTED_EDGE('',*,*,#48584,.F.);
#68059=ORIENTED_EDGE('',*,*,#48585,.F.);
#68060=ORIENTED_EDGE('',*,*,#48582,.F.);
#68061=ORIENTED_EDGE('',*,*,#48414,.F.);
#68062=ORIENTED_EDGE('',*,*,#48586,.T.);
#68063=ORIENTED_EDGE('',*,*,#48587,.F.);
#68064=ORIENTED_EDGE('',*,*,#48584,.T.);
#68065=ORIENTED_EDGE('',*,*,#48413,.F.);
#68066=ORIENTED_EDGE('',*,*,#48588,.T.);
#68067=ORIENTED_EDGE('',*,*,#48589,.F.);
#68068=ORIENTED_EDGE('',*,*,#48586,.F.);
#68069=ORIENTED_EDGE('',*,*,#48412,.F.);
#68070=ORIENTED_EDGE('',*,*,#48590,.T.);
#68071=ORIENTED_EDGE('',*,*,#48591,.F.);
#68072=ORIENTED_EDGE('',*,*,#48588,.F.);
#68073=ORIENTED_EDGE('',*,*,#48411,.F.);
#68074=ORIENTED_EDGE('',*,*,#48592,.T.);
#68075=ORIENTED_EDGE('',*,*,#48593,.F.);
#68076=ORIENTED_EDGE('',*,*,#48590,.F.);
#68077=ORIENTED_EDGE('',*,*,#48410,.F.);
#68078=ORIENTED_EDGE('',*,*,#48594,.T.);
#68079=ORIENTED_EDGE('',*,*,#48595,.F.);
#68080=ORIENTED_EDGE('',*,*,#48592,.F.);
#68081=ORIENTED_EDGE('',*,*,#48409,.F.);
#68082=ORIENTED_EDGE('',*,*,#48596,.F.);
#68083=ORIENTED_EDGE('',*,*,#48597,.F.);
#68084=ORIENTED_EDGE('',*,*,#48594,.F.);
#68085=ORIENTED_EDGE('',*,*,#48408,.F.);
#68086=ORIENTED_EDGE('',*,*,#48598,.T.);
#68087=ORIENTED_EDGE('',*,*,#48599,.F.);
#68088=ORIENTED_EDGE('',*,*,#48596,.T.);
#68089=ORIENTED_EDGE('',*,*,#48407,.F.);
#68090=ORIENTED_EDGE('',*,*,#48600,.T.);
#68091=ORIENTED_EDGE('',*,*,#48601,.F.);
#68092=ORIENTED_EDGE('',*,*,#48598,.F.);
#68093=ORIENTED_EDGE('',*,*,#48406,.F.);
#68094=ORIENTED_EDGE('',*,*,#48602,.T.);
#68095=ORIENTED_EDGE('',*,*,#48603,.F.);
#68096=ORIENTED_EDGE('',*,*,#48600,.F.);
#68097=ORIENTED_EDGE('',*,*,#48405,.F.);
#68098=ORIENTED_EDGE('',*,*,#48604,.T.);
#68099=ORIENTED_EDGE('',*,*,#48605,.F.);
#68100=ORIENTED_EDGE('',*,*,#48602,.F.);
#68101=ORIENTED_EDGE('',*,*,#48404,.F.);
#68102=ORIENTED_EDGE('',*,*,#48606,.T.);
#68103=ORIENTED_EDGE('',*,*,#48607,.F.);
#68104=ORIENTED_EDGE('',*,*,#48604,.F.);
#68105=ORIENTED_EDGE('',*,*,#48403,.F.);
#68106=ORIENTED_EDGE('',*,*,#48608,.F.);
#68107=ORIENTED_EDGE('',*,*,#48609,.F.);
#68108=ORIENTED_EDGE('',*,*,#48606,.F.);
#68109=ORIENTED_EDGE('',*,*,#48543,.T.);
#68110=ORIENTED_EDGE('',*,*,#48545,.T.);
#68111=ORIENTED_EDGE('',*,*,#48547,.T.);
#68112=ORIENTED_EDGE('',*,*,#48549,.T.);
#68113=ORIENTED_EDGE('',*,*,#48551,.T.);
#68114=ORIENTED_EDGE('',*,*,#48553,.T.);
#68115=ORIENTED_EDGE('',*,*,#48555,.T.);
#68116=ORIENTED_EDGE('',*,*,#48557,.T.);
#68117=ORIENTED_EDGE('',*,*,#48559,.T.);
#68118=ORIENTED_EDGE('',*,*,#48561,.T.);
#68119=ORIENTED_EDGE('',*,*,#48563,.T.);
#68120=ORIENTED_EDGE('',*,*,#48565,.T.);
#68121=ORIENTED_EDGE('',*,*,#48567,.T.);
#68122=ORIENTED_EDGE('',*,*,#48569,.T.);
#68123=ORIENTED_EDGE('',*,*,#48571,.T.);
#68124=ORIENTED_EDGE('',*,*,#48573,.T.);
#68125=ORIENTED_EDGE('',*,*,#48575,.T.);
#68126=ORIENTED_EDGE('',*,*,#48577,.T.);
#68127=ORIENTED_EDGE('',*,*,#48579,.T.);
#68128=ORIENTED_EDGE('',*,*,#48581,.T.);
#68129=ORIENTED_EDGE('',*,*,#48583,.T.);
#68130=ORIENTED_EDGE('',*,*,#48585,.T.);
#68131=ORIENTED_EDGE('',*,*,#48587,.T.);
#68132=ORIENTED_EDGE('',*,*,#48589,.T.);
#68133=ORIENTED_EDGE('',*,*,#48591,.T.);
#68134=ORIENTED_EDGE('',*,*,#48593,.T.);
#68135=ORIENTED_EDGE('',*,*,#48595,.T.);
#68136=ORIENTED_EDGE('',*,*,#48597,.T.);
#68137=ORIENTED_EDGE('',*,*,#48599,.T.);
#68138=ORIENTED_EDGE('',*,*,#48601,.T.);
#68139=ORIENTED_EDGE('',*,*,#48603,.T.);
#68140=ORIENTED_EDGE('',*,*,#48605,.T.);
#68141=ORIENTED_EDGE('',*,*,#48607,.T.);
#68142=ORIENTED_EDGE('',*,*,#48609,.T.);
#68143=ORIENTED_EDGE('',*,*,#48610,.T.);
#68144=ORIENTED_EDGE('',*,*,#48611,.T.);
#68145=ORIENTED_EDGE('',*,*,#48612,.T.);
#68146=ORIENTED_EDGE('',*,*,#48613,.T.);
#68147=ORIENTED_EDGE('',*,*,#48614,.T.);
#68148=ORIENTED_EDGE('',*,*,#48615,.T.);
#68149=ORIENTED_EDGE('',*,*,#48616,.T.);
#68150=ORIENTED_EDGE('',*,*,#48617,.T.);
#68151=ORIENTED_EDGE('',*,*,#48618,.T.);
#68152=ORIENTED_EDGE('',*,*,#48619,.T.);
#68153=ORIENTED_EDGE('',*,*,#48620,.T.);
#68154=ORIENTED_EDGE('',*,*,#48621,.T.);
#68155=ORIENTED_EDGE('',*,*,#48622,.T.);
#68156=ORIENTED_EDGE('',*,*,#48623,.T.);
#68157=ORIENTED_EDGE('',*,*,#48624,.T.);
#68158=ORIENTED_EDGE('',*,*,#48625,.T.);
#68159=ORIENTED_EDGE('',*,*,#48626,.T.);
#68160=ORIENTED_EDGE('',*,*,#48627,.T.);
#68161=ORIENTED_EDGE('',*,*,#48628,.T.);
#68162=ORIENTED_EDGE('',*,*,#48629,.T.);
#68163=ORIENTED_EDGE('',*,*,#48630,.T.);
#68164=ORIENTED_EDGE('',*,*,#48631,.T.);
#68165=ORIENTED_EDGE('',*,*,#48632,.T.);
#68166=ORIENTED_EDGE('',*,*,#48633,.T.);
#68167=ORIENTED_EDGE('',*,*,#48634,.T.);
#68168=ORIENTED_EDGE('',*,*,#48635,.T.);
#68169=ORIENTED_EDGE('',*,*,#48636,.T.);
#68170=ORIENTED_EDGE('',*,*,#48637,.T.);
#68171=ORIENTED_EDGE('',*,*,#48638,.T.);
#68172=ORIENTED_EDGE('',*,*,#48639,.T.);
#68173=ORIENTED_EDGE('',*,*,#48640,.T.);
#68174=ORIENTED_EDGE('',*,*,#48641,.T.);
#68175=ORIENTED_EDGE('',*,*,#48642,.T.);
#68176=ORIENTED_EDGE('',*,*,#48643,.T.);
#68177=ORIENTED_EDGE('',*,*,#48644,.T.);
#68178=ORIENTED_EDGE('',*,*,#48645,.T.);
#68179=ORIENTED_EDGE('',*,*,#48646,.T.);
#68180=ORIENTED_EDGE('',*,*,#48647,.T.);
#68181=ORIENTED_EDGE('',*,*,#48648,.T.);
#68182=ORIENTED_EDGE('',*,*,#48649,.T.);
#68183=ORIENTED_EDGE('',*,*,#48650,.T.);
#68184=ORIENTED_EDGE('',*,*,#48651,.T.);
#68185=ORIENTED_EDGE('',*,*,#48652,.T.);
#68186=ORIENTED_EDGE('',*,*,#48653,.T.);
#68187=ORIENTED_EDGE('',*,*,#48654,.T.);
#68188=ORIENTED_EDGE('',*,*,#48655,.T.);
#68189=ORIENTED_EDGE('',*,*,#48656,.T.);
#68190=ORIENTED_EDGE('',*,*,#48657,.T.);
#68191=ORIENTED_EDGE('',*,*,#48658,.T.);
#68192=ORIENTED_EDGE('',*,*,#48659,.T.);
#68193=ORIENTED_EDGE('',*,*,#48660,.T.);
#68194=ORIENTED_EDGE('',*,*,#48508,.T.);
#68195=ORIENTED_EDGE('',*,*,#48511,.T.);
#68196=ORIENTED_EDGE('',*,*,#48513,.T.);
#68197=ORIENTED_EDGE('',*,*,#48515,.T.);
#68198=ORIENTED_EDGE('',*,*,#48517,.T.);
#68199=ORIENTED_EDGE('',*,*,#48519,.T.);
#68200=ORIENTED_EDGE('',*,*,#48521,.T.);
#68201=ORIENTED_EDGE('',*,*,#48523,.T.);
#68202=ORIENTED_EDGE('',*,*,#48525,.T.);
#68203=ORIENTED_EDGE('',*,*,#48527,.T.);
#68204=ORIENTED_EDGE('',*,*,#48529,.T.);
#68205=ORIENTED_EDGE('',*,*,#48531,.T.);
#68206=ORIENTED_EDGE('',*,*,#48533,.T.);
#68207=ORIENTED_EDGE('',*,*,#48535,.T.);
#68208=ORIENTED_EDGE('',*,*,#48537,.T.);
#68209=ORIENTED_EDGE('',*,*,#48539,.T.);
#68210=ORIENTED_EDGE('',*,*,#48541,.T.);
#68211=ORIENTED_EDGE('',*,*,#48506,.T.);
#68212=ORIENTED_EDGE('',*,*,#48455,.F.);
#68213=ORIENTED_EDGE('',*,*,#48661,.T.);
#68214=ORIENTED_EDGE('',*,*,#48659,.F.);
#68215=ORIENTED_EDGE('',*,*,#48662,.F.);
#68216=ORIENTED_EDGE('',*,*,#48454,.F.);
#68217=ORIENTED_EDGE('',*,*,#48509,.T.);
#68218=ORIENTED_EDGE('',*,*,#48660,.F.);
#68219=ORIENTED_EDGE('',*,*,#48661,.F.);
#68220=ORIENTED_EDGE('',*,*,#48456,.F.);
#68221=ORIENTED_EDGE('',*,*,#48662,.T.);
#68222=ORIENTED_EDGE('',*,*,#48658,.F.);
#68223=ORIENTED_EDGE('',*,*,#48663,.T.);
#68224=ORIENTED_EDGE('',*,*,#48457,.F.);
#68225=ORIENTED_EDGE('',*,*,#48663,.F.);
#68226=ORIENTED_EDGE('',*,*,#48657,.F.);
#68227=ORIENTED_EDGE('',*,*,#48664,.F.);
#68228=ORIENTED_EDGE('',*,*,#48458,.F.);
#68229=ORIENTED_EDGE('',*,*,#48664,.T.);
#68230=ORIENTED_EDGE('',*,*,#48656,.F.);
#68231=ORIENTED_EDGE('',*,*,#48665,.F.);
#68232=ORIENTED_EDGE('',*,*,#48459,.F.);
#68233=ORIENTED_EDGE('',*,*,#48665,.T.);
#68234=ORIENTED_EDGE('',*,*,#48655,.F.);
#68235=ORIENTED_EDGE('',*,*,#48666,.F.);
#68236=ORIENTED_EDGE('',*,*,#48460,.F.);
#68237=ORIENTED_EDGE('',*,*,#48666,.T.);
#68238=ORIENTED_EDGE('',*,*,#48654,.F.);
#68239=ORIENTED_EDGE('',*,*,#48667,.F.);
#68240=ORIENTED_EDGE('',*,*,#48461,.F.);
#68241=ORIENTED_EDGE('',*,*,#48667,.T.);
#68242=ORIENTED_EDGE('',*,*,#48653,.F.);
#68243=ORIENTED_EDGE('',*,*,#48668,.F.);
#68244=ORIENTED_EDGE('',*,*,#48462,.F.);
#68245=ORIENTED_EDGE('',*,*,#48668,.T.);
#68246=ORIENTED_EDGE('',*,*,#48652,.F.);
#68247=ORIENTED_EDGE('',*,*,#48669,.T.);
#68248=ORIENTED_EDGE('',*,*,#48467,.F.);
#68249=ORIENTED_EDGE('',*,*,#48670,.T.);
#68250=ORIENTED_EDGE('',*,*,#48647,.F.);
#68251=ORIENTED_EDGE('',*,*,#48671,.F.);
#68252=ORIENTED_EDGE('',*,*,#48463,.F.);
#68253=ORIENTED_EDGE('',*,*,#48669,.F.);
#68254=ORIENTED_EDGE('',*,*,#48651,.F.);
#68255=ORIENTED_EDGE('',*,*,#48672,.F.);
#68256=ORIENTED_EDGE('',*,*,#48464,.F.);
#68257=ORIENTED_EDGE('',*,*,#48672,.T.);
#68258=ORIENTED_EDGE('',*,*,#48650,.F.);
#68259=ORIENTED_EDGE('',*,*,#48673,.F.);
#68260=ORIENTED_EDGE('',*,*,#48465,.F.);
#68261=ORIENTED_EDGE('',*,*,#48673,.T.);
#68262=ORIENTED_EDGE('',*,*,#48649,.F.);
#68263=ORIENTED_EDGE('',*,*,#48674,.F.);
#68264=ORIENTED_EDGE('',*,*,#48466,.F.);
#68265=ORIENTED_EDGE('',*,*,#48674,.T.);
#68266=ORIENTED_EDGE('',*,*,#48648,.F.);
#68267=ORIENTED_EDGE('',*,*,#48670,.F.);
#68268=ORIENTED_EDGE('',*,*,#48469,.F.);
#68269=ORIENTED_EDGE('',*,*,#48675,.F.);
#68270=ORIENTED_EDGE('',*,*,#48645,.F.);
#68271=ORIENTED_EDGE('',*,*,#48676,.F.);
#68272=ORIENTED_EDGE('',*,*,#48473,.F.);
#68273=ORIENTED_EDGE('',*,*,#48677,.T.);
#68274=ORIENTED_EDGE('',*,*,#48641,.F.);
#68275=ORIENTED_EDGE('',*,*,#48678,.F.);
#68276=ORIENTED_EDGE('',*,*,#48470,.F.);
#68277=ORIENTED_EDGE('',*,*,#48676,.T.);
#68278=ORIENTED_EDGE('',*,*,#48644,.F.);
#68279=ORIENTED_EDGE('',*,*,#48679,.F.);
#68280=ORIENTED_EDGE('',*,*,#48471,.F.);
#68281=ORIENTED_EDGE('',*,*,#48679,.T.);
#68282=ORIENTED_EDGE('',*,*,#48643,.F.);
#68283=ORIENTED_EDGE('',*,*,#48680,.F.);
#68284=ORIENTED_EDGE('',*,*,#48472,.F.);
#68285=ORIENTED_EDGE('',*,*,#48680,.T.);
#68286=ORIENTED_EDGE('',*,*,#48642,.F.);
#68287=ORIENTED_EDGE('',*,*,#48677,.F.);
#68288=ORIENTED_EDGE('',*,*,#48474,.F.);
#68289=ORIENTED_EDGE('',*,*,#48678,.T.);
#68290=ORIENTED_EDGE('',*,*,#48640,.F.);
#68291=ORIENTED_EDGE('',*,*,#48681,.T.);
#68292=ORIENTED_EDGE('',*,*,#48475,.F.);
#68293=ORIENTED_EDGE('',*,*,#48681,.F.);
#68294=ORIENTED_EDGE('',*,*,#48639,.F.);
#68295=ORIENTED_EDGE('',*,*,#48682,.F.);
#68296=ORIENTED_EDGE('',*,*,#48476,.F.);
#68297=ORIENTED_EDGE('',*,*,#48682,.T.);
#68298=ORIENTED_EDGE('',*,*,#48638,.F.);
#68299=ORIENTED_EDGE('',*,*,#48683,.F.);
#68300=ORIENTED_EDGE('',*,*,#48477,.F.);
#68301=ORIENTED_EDGE('',*,*,#48683,.T.);
#68302=ORIENTED_EDGE('',*,*,#48637,.F.);
#68303=ORIENTED_EDGE('',*,*,#48684,.F.);
#68304=ORIENTED_EDGE('',*,*,#48478,.F.);
#68305=ORIENTED_EDGE('',*,*,#48684,.T.);
#68306=ORIENTED_EDGE('',*,*,#48636,.F.);
#68307=ORIENTED_EDGE('',*,*,#48685,.F.);
#68308=ORIENTED_EDGE('',*,*,#48479,.F.);
#68309=ORIENTED_EDGE('',*,*,#48685,.T.);
#68310=ORIENTED_EDGE('',*,*,#48635,.F.);
#68311=ORIENTED_EDGE('',*,*,#48686,.F.);
#68312=ORIENTED_EDGE('',*,*,#48468,.F.);
#68313=ORIENTED_EDGE('',*,*,#48671,.T.);
#68314=ORIENTED_EDGE('',*,*,#48646,.F.);
#68315=ORIENTED_EDGE('',*,*,#48675,.T.);
#68316=ORIENTED_EDGE('',*,*,#48480,.F.);
#68317=ORIENTED_EDGE('',*,*,#48686,.T.);
#68318=ORIENTED_EDGE('',*,*,#48634,.F.);
#68319=ORIENTED_EDGE('',*,*,#48687,.T.);
#68320=ORIENTED_EDGE('',*,*,#48485,.F.);
#68321=ORIENTED_EDGE('',*,*,#48688,.T.);
#68322=ORIENTED_EDGE('',*,*,#48629,.F.);
#68323=ORIENTED_EDGE('',*,*,#48689,.F.);
#68324=ORIENTED_EDGE('',*,*,#48481,.F.);
#68325=ORIENTED_EDGE('',*,*,#48687,.F.);
#68326=ORIENTED_EDGE('',*,*,#48633,.F.);
#68327=ORIENTED_EDGE('',*,*,#48690,.F.);
#68328=ORIENTED_EDGE('',*,*,#48482,.F.);
#68329=ORIENTED_EDGE('',*,*,#48690,.T.);
#68330=ORIENTED_EDGE('',*,*,#48632,.F.);
#68331=ORIENTED_EDGE('',*,*,#48691,.F.);
#68332=ORIENTED_EDGE('',*,*,#48483,.F.);
#68333=ORIENTED_EDGE('',*,*,#48691,.T.);
#68334=ORIENTED_EDGE('',*,*,#48631,.F.);
#68335=ORIENTED_EDGE('',*,*,#48692,.F.);
#68336=ORIENTED_EDGE('',*,*,#48484,.F.);
#68337=ORIENTED_EDGE('',*,*,#48692,.T.);
#68338=ORIENTED_EDGE('',*,*,#48630,.F.);
#68339=ORIENTED_EDGE('',*,*,#48688,.F.);
#68340=ORIENTED_EDGE('',*,*,#48487,.F.);
#68341=ORIENTED_EDGE('',*,*,#48693,.F.);
#68342=ORIENTED_EDGE('',*,*,#48627,.F.);
#68343=ORIENTED_EDGE('',*,*,#48694,.F.);
#68344=ORIENTED_EDGE('',*,*,#48491,.F.);
#68345=ORIENTED_EDGE('',*,*,#48695,.T.);
#68346=ORIENTED_EDGE('',*,*,#48623,.F.);
#68347=ORIENTED_EDGE('',*,*,#48696,.F.);
#68348=ORIENTED_EDGE('',*,*,#48488,.F.);
#68349=ORIENTED_EDGE('',*,*,#48694,.T.);
#68350=ORIENTED_EDGE('',*,*,#48626,.F.);
#68351=ORIENTED_EDGE('',*,*,#48697,.F.);
#68352=ORIENTED_EDGE('',*,*,#48489,.F.);
#68353=ORIENTED_EDGE('',*,*,#48697,.T.);
#68354=ORIENTED_EDGE('',*,*,#48625,.F.);
#68355=ORIENTED_EDGE('',*,*,#48698,.F.);
#68356=ORIENTED_EDGE('',*,*,#48490,.F.);
#68357=ORIENTED_EDGE('',*,*,#48698,.T.);
#68358=ORIENTED_EDGE('',*,*,#48624,.F.);
#68359=ORIENTED_EDGE('',*,*,#48695,.F.);
#68360=ORIENTED_EDGE('',*,*,#48492,.F.);
#68361=ORIENTED_EDGE('',*,*,#48696,.T.);
#68362=ORIENTED_EDGE('',*,*,#48622,.F.);
#68363=ORIENTED_EDGE('',*,*,#48699,.T.);
#68364=ORIENTED_EDGE('',*,*,#48493,.F.);
#68365=ORIENTED_EDGE('',*,*,#48699,.F.);
#68366=ORIENTED_EDGE('',*,*,#48621,.F.);
#68367=ORIENTED_EDGE('',*,*,#48700,.F.);
#68368=ORIENTED_EDGE('',*,*,#48494,.F.);
#68369=ORIENTED_EDGE('',*,*,#48700,.T.);
#68370=ORIENTED_EDGE('',*,*,#48620,.F.);
#68371=ORIENTED_EDGE('',*,*,#48701,.F.);
#68372=ORIENTED_EDGE('',*,*,#48495,.F.);
#68373=ORIENTED_EDGE('',*,*,#48701,.T.);
#68374=ORIENTED_EDGE('',*,*,#48619,.F.);
#68375=ORIENTED_EDGE('',*,*,#48702,.F.);
#68376=ORIENTED_EDGE('',*,*,#48496,.F.);
#68377=ORIENTED_EDGE('',*,*,#48702,.T.);
#68378=ORIENTED_EDGE('',*,*,#48618,.F.);
#68379=ORIENTED_EDGE('',*,*,#48703,.F.);
#68380=ORIENTED_EDGE('',*,*,#48497,.F.);
#68381=ORIENTED_EDGE('',*,*,#48703,.T.);
#68382=ORIENTED_EDGE('',*,*,#48617,.F.);
#68383=ORIENTED_EDGE('',*,*,#48704,.F.);
#68384=ORIENTED_EDGE('',*,*,#48486,.F.);
#68385=ORIENTED_EDGE('',*,*,#48689,.T.);
#68386=ORIENTED_EDGE('',*,*,#48628,.F.);
#68387=ORIENTED_EDGE('',*,*,#48693,.T.);
#68388=ORIENTED_EDGE('',*,*,#48498,.F.);
#68389=ORIENTED_EDGE('',*,*,#48704,.T.);
#68390=ORIENTED_EDGE('',*,*,#48616,.F.);
#68391=ORIENTED_EDGE('',*,*,#48705,.T.);
#68392=ORIENTED_EDGE('',*,*,#48401,.F.);
#68393=ORIENTED_EDGE('',*,*,#48706,.T.);
#68394=ORIENTED_EDGE('',*,*,#48611,.F.);
#68395=ORIENTED_EDGE('',*,*,#48707,.F.);
#68396=ORIENTED_EDGE('',*,*,#48499,.F.);
#68397=ORIENTED_EDGE('',*,*,#48705,.F.);
#68398=ORIENTED_EDGE('',*,*,#48615,.F.);
#68399=ORIENTED_EDGE('',*,*,#48708,.F.);
#68400=ORIENTED_EDGE('',*,*,#48500,.F.);
#68401=ORIENTED_EDGE('',*,*,#48708,.T.);
#68402=ORIENTED_EDGE('',*,*,#48614,.F.);
#68403=ORIENTED_EDGE('',*,*,#48709,.F.);
#68404=ORIENTED_EDGE('',*,*,#48501,.F.);
#68405=ORIENTED_EDGE('',*,*,#48709,.T.);
#68406=ORIENTED_EDGE('',*,*,#48613,.F.);
#68407=ORIENTED_EDGE('',*,*,#48710,.F.);
#68408=ORIENTED_EDGE('',*,*,#48502,.F.);
#68409=ORIENTED_EDGE('',*,*,#48710,.T.);
#68410=ORIENTED_EDGE('',*,*,#48612,.F.);
#68411=ORIENTED_EDGE('',*,*,#48706,.F.);
#68412=ORIENTED_EDGE('',*,*,#48402,.F.);
#68413=ORIENTED_EDGE('',*,*,#48707,.T.);
#68414=ORIENTED_EDGE('',*,*,#48610,.F.);
#68415=ORIENTED_EDGE('',*,*,#48608,.T.);
#68416=ORIENTED_EDGE('',*,*,#48503,.F.);
#68417=ORIENTED_EDGE('',*,*,#48711,.T.);
#68418=ORIENTED_EDGE('',*,*,#48712,.F.);
#68419=ORIENTED_EDGE('',*,*,#48711,.F.);
#68420=ORIENTED_EDGE('',*,*,#48712,.T.);
#68421=ORIENTED_EDGE('',*,*,#48397,.T.);
#87702=CYLINDRICAL_SURFACE('',#98433,11.5);
#87703=CYLINDRICAL_SURFACE('',#98436,10.375);
#87704=CYLINDRICAL_SURFACE('',#98439,11.5);
#87705=CYLINDRICAL_SURFACE('',#98442,10.375);
#87706=CYLINDRICAL_SURFACE('',#98445,11.5);
#87707=CYLINDRICAL_SURFACE('',#98448,10.375);
#87708=CYLINDRICAL_SURFACE('',#98451,11.5);
#87709=CYLINDRICAL_SURFACE('',#98454,10.375);
#87710=CYLINDRICAL_SURFACE('',#98457,11.5);
#87711=CYLINDRICAL_SURFACE('',#98460,10.375);
#87712=CYLINDRICAL_SURFACE('',#98463,11.5);
#87713=CYLINDRICAL_SURFACE('',#98466,10.375);
#87714=CYLINDRICAL_SURFACE('',#98469,11.5);
#87715=CYLINDRICAL_SURFACE('',#98472,10.375);
#87716=CYLINDRICAL_SURFACE('',#98475,11.5);
#87717=CYLINDRICAL_SURFACE('',#98478,10.375);
#87718=CYLINDRICAL_SURFACE('',#98481,11.5);
#87719=CYLINDRICAL_SURFACE('',#98484,10.375);
#87720=CYLINDRICAL_SURFACE('',#98487,11.5);
#87721=CYLINDRICAL_SURFACE('',#98490,10.375);
#87722=CYLINDRICAL_SURFACE('',#98493,11.5);
#87723=CYLINDRICAL_SURFACE('',#98496,10.375);
#87724=CYLINDRICAL_SURFACE('',#98499,11.5);
#87725=CYLINDRICAL_SURFACE('',#98502,10.375);
#87726=CYLINDRICAL_SURFACE('',#98505,11.5);
#87727=CYLINDRICAL_SURFACE('',#98508,10.375);
#87728=CYLINDRICAL_SURFACE('',#98511,11.5);
#87729=CYLINDRICAL_SURFACE('',#98514,10.375);
#87730=CYLINDRICAL_SURFACE('',#98517,11.5);
#87731=CYLINDRICAL_SURFACE('',#98520,10.375);
#87732=CYLINDRICAL_SURFACE('',#98523,11.5);
#87733=CYLINDRICAL_SURFACE('',#98526,10.375);
#87734=CYLINDRICAL_SURFACE('',#98529,11.5);
#87735=CYLINDRICAL_SURFACE('',#98532,10.375);
#87736=CYLINDRICAL_SURFACE('',#98535,11.5);
#87737=CYLINDRICAL_SURFACE('',#98538,10.375);
#87738=CYLINDRICAL_SURFACE('',#98541,11.5);
#87739=CYLINDRICAL_SURFACE('',#98544,10.375);
#87740=CYLINDRICAL_SURFACE('',#98547,11.5);
#87741=CYLINDRICAL_SURFACE('',#98550,10.375);
#87742=CYLINDRICAL_SURFACE('',#98553,11.5);
#87743=CYLINDRICAL_SURFACE('',#98556,10.375);
#87744=CYLINDRICAL_SURFACE('',#98559,11.5);
#87745=CYLINDRICAL_SURFACE('',#98562,10.375);
#87746=CYLINDRICAL_SURFACE('',#98565,11.5);
#87747=CYLINDRICAL_SURFACE('',#98568,10.375);
#87748=CYLINDRICAL_SURFACE('',#98571,11.5);
#87749=CYLINDRICAL_SURFACE('',#98574,10.375);
#87750=CYLINDRICAL_SURFACE('',#98577,11.5);
#87751=CYLINDRICAL_SURFACE('',#98580,10.375);
#87752=CYLINDRICAL_SURFACE('',#98583,11.5);
#87753=CYLINDRICAL_SURFACE('',#98586,10.375);
#87754=CYLINDRICAL_SURFACE('',#98589,11.5);
#87755=CYLINDRICAL_SURFACE('',#98592,10.375);
#87756=CYLINDRICAL_SURFACE('',#98595,11.5);
#87757=CYLINDRICAL_SURFACE('',#98598,10.375);
#87758=CYLINDRICAL_SURFACE('',#98601,11.5);
#87759=CYLINDRICAL_SURFACE('',#98604,10.375);
#87760=CYLINDRICAL_SURFACE('',#98607,11.5);
#87761=CYLINDRICAL_SURFACE('',#98610,10.375);
#87762=CYLINDRICAL_SURFACE('',#98613,11.5);
#87763=CYLINDRICAL_SURFACE('',#98616,10.375);
#87764=CYLINDRICAL_SURFACE('',#98619,11.5);
#87765=CYLINDRICAL_SURFACE('',#98622,10.375);
#87766=CYLINDRICAL_SURFACE('',#98625,11.5);
#87767=CYLINDRICAL_SURFACE('',#98628,10.375);
#87768=CYLINDRICAL_SURFACE('',#98631,11.5);
#87769=CYLINDRICAL_SURFACE('',#98634,10.375);
#87770=CYLINDRICAL_SURFACE('',#98637,11.5);
#87771=CYLINDRICAL_SURFACE('',#98640,10.375);
#87772=CYLINDRICAL_SURFACE('',#98643,11.5);
#87773=CYLINDRICAL_SURFACE('',#98646,10.375);
#87774=CYLINDRICAL_SURFACE('',#98649,11.5);
#87775=CYLINDRICAL_SURFACE('',#98652,10.375);
#87776=CYLINDRICAL_SURFACE('',#98655,11.5);
#87777=CYLINDRICAL_SURFACE('',#98658,10.375);
#87778=CYLINDRICAL_SURFACE('',#98661,11.5);
#87779=CYLINDRICAL_SURFACE('',#98664,10.375);
#87780=CYLINDRICAL_SURFACE('',#98667,11.5);
#87781=CYLINDRICAL_SURFACE('',#98670,10.375);
#87782=CYLINDRICAL_SURFACE('',#98673,11.5);
#87783=CYLINDRICAL_SURFACE('',#98676,10.375);
#87784=CYLINDRICAL_SURFACE('',#98679,11.5);
#87785=CYLINDRICAL_SURFACE('',#98682,10.375);
#87786=CYLINDRICAL_SURFACE('',#98685,11.5);
#87787=CYLINDRICAL_SURFACE('',#98693,10.375);
#87788=CYLINDRICAL_SURFACE('',#98695,10.375);
#87789=CYLINDRICAL_SURFACE('',#98697,11.5);
#87790=CYLINDRICAL_SURFACE('',#98699,3.5);
#87791=CYLINDRICAL_SURFACE('',#98702,1.5);
#87792=CYLINDRICAL_SURFACE('',#98705,1.5);
#87793=CYLINDRICAL_SURFACE('',#98746,3.);
#87794=CYLINDRICAL_SURFACE('',#98750,4.75);
#87795=CYLINDRICAL_SURFACE('',#98753,3.625);
#87796=CYLINDRICAL_SURFACE('',#98756,4.75);
#87797=CYLINDRICAL_SURFACE('',#98759,3.625);
#87798=CYLINDRICAL_SURFACE('',#98762,4.75);
#87799=CYLINDRICAL_SURFACE('',#98765,3.625);
#87800=CYLINDRICAL_SURFACE('',#98768,4.75);
#87801=CYLINDRICAL_SURFACE('',#98771,3.625);
#87802=CYLINDRICAL_SURFACE('',#98774,4.75);
#87803=CYLINDRICAL_SURFACE('',#98777,3.625);
#87804=CYLINDRICAL_SURFACE('',#98780,4.75);
#87805=CYLINDRICAL_SURFACE('',#98783,3.625);
#87806=CYLINDRICAL_SURFACE('',#98786,4.75);
#87807=CYLINDRICAL_SURFACE('',#98789,3.625);
#87808=CYLINDRICAL_SURFACE('',#98792,4.75);
#87809=CYLINDRICAL_SURFACE('',#98795,3.625);
#87810=CYLINDRICAL_SURFACE('',#98798,4.75);
#87811=CYLINDRICAL_SURFACE('',#98820,3.625);
#87812=CYLINDRICAL_SURFACE('',#98822,4.75);
#87813=CYLINDRICAL_SURFACE('',#98824,3.625);
#87814=CYLINDRICAL_SURFACE('',#98827,4.75);
#87815=CYLINDRICAL_SURFACE('',#98830,4.75);
#87816=CYLINDRICAL_SURFACE('',#98831,3.625);
#87817=CYLINDRICAL_SURFACE('',#98833,4.75);
#87818=CYLINDRICAL_SURFACE('',#98835,3.625);
#87819=CYLINDRICAL_SURFACE('',#98836,3.625);
#87820=CYLINDRICAL_SURFACE('',#98839,4.75);
#87821=CYLINDRICAL_SURFACE('',#98842,4.75);
#87822=CYLINDRICAL_SURFACE('',#98843,3.625);
#87823=CYLINDRICAL_SURFACE('',#98845,4.75);
#87824=CYLINDRICAL_SURFACE('',#98847,3.625);
#87825=CYLINDRICAL_SURFACE('',#98848,3.625);
#87826=CYLINDRICAL_SURFACE('',#98851,4.75);
#87827=CYLINDRICAL_SURFACE('',#98852,3.625);
#87828=CYLINDRICAL_SURFACE('',#98853,3.5);
#90406=ADVANCED_FACE('',(#7942),#87702,.T.);
#90407=ADVANCED_FACE('',(#7943),#6215,.T.);
#90408=ADVANCED_FACE('',(#7944),#6216,.T.);
#90409=ADVANCED_FACE('',(#7945),#87703,.T.);
#90410=ADVANCED_FACE('',(#7946),#87704,.T.);
#90411=ADVANCED_FACE('',(#7947),#6217,.T.);
#90412=ADVANCED_FACE('',(#7948),#6218,.T.);
#90413=ADVANCED_FACE('',(#7949),#87705,.T.);
#90414=ADVANCED_FACE('',(#7950),#87706,.T.);
#90415=ADVANCED_FACE('',(#7951),#6219,.T.);
#90416=ADVANCED_FACE('',(#7952),#6220,.T.);
#90417=ADVANCED_FACE('',(#7953),#87707,.T.);
#90418=ADVANCED_FACE('',(#7954),#87708,.T.);
#90419=ADVANCED_FACE('',(#7955),#6221,.T.);
#90420=ADVANCED_FACE('',(#7956),#6222,.T.);
#90421=ADVANCED_FACE('',(#7957),#87709,.T.);
#90422=ADVANCED_FACE('',(#7958),#87710,.T.);
#90423=ADVANCED_FACE('',(#7959),#6223,.T.);
#90424=ADVANCED_FACE('',(#7960),#6224,.T.);
#90425=ADVANCED_FACE('',(#7961),#87711,.T.);
#90426=ADVANCED_FACE('',(#7962),#87712,.T.);
#90427=ADVANCED_FACE('',(#7963),#6225,.T.);
#90428=ADVANCED_FACE('',(#7964),#6226,.T.);
#90429=ADVANCED_FACE('',(#7965),#87713,.T.);
#90430=ADVANCED_FACE('',(#7966),#87714,.T.);
#90431=ADVANCED_FACE('',(#7967),#6227,.T.);
#90432=ADVANCED_FACE('',(#7968),#6228,.T.);
#90433=ADVANCED_FACE('',(#7969),#87715,.T.);
#90434=ADVANCED_FACE('',(#7970),#87716,.T.);
#90435=ADVANCED_FACE('',(#7971),#6229,.T.);
#90436=ADVANCED_FACE('',(#7972),#6230,.T.);
#90437=ADVANCED_FACE('',(#7973),#87717,.T.);
#90438=ADVANCED_FACE('',(#7974),#87718,.T.);
#90439=ADVANCED_FACE('',(#7975),#6231,.T.);
#90440=ADVANCED_FACE('',(#7976),#6232,.T.);
#90441=ADVANCED_FACE('',(#7977),#87719,.T.);
#90442=ADVANCED_FACE('',(#7978),#87720,.T.);
#90443=ADVANCED_FACE('',(#7979),#6233,.T.);
#90444=ADVANCED_FACE('',(#7980),#6234,.T.);
#90445=ADVANCED_FACE('',(#7981),#87721,.T.);
#90446=ADVANCED_FACE('',(#7982),#87722,.T.);
#90447=ADVANCED_FACE('',(#7983),#6235,.T.);
#90448=ADVANCED_FACE('',(#7984),#6236,.T.);
#90449=ADVANCED_FACE('',(#7985),#87723,.T.);
#90450=ADVANCED_FACE('',(#7986),#87724,.T.);
#90451=ADVANCED_FACE('',(#7987),#6237,.T.);
#90452=ADVANCED_FACE('',(#7988),#6238,.T.);
#90453=ADVANCED_FACE('',(#7989),#87725,.T.);
#90454=ADVANCED_FACE('',(#7990),#87726,.T.);
#90455=ADVANCED_FACE('',(#7991),#6239,.T.);
#90456=ADVANCED_FACE('',(#7992),#6240,.T.);
#90457=ADVANCED_FACE('',(#7993),#87727,.T.);
#90458=ADVANCED_FACE('',(#7994),#87728,.T.);
#90459=ADVANCED_FACE('',(#7995),#6241,.T.);
#90460=ADVANCED_FACE('',(#7996),#6242,.T.);
#90461=ADVANCED_FACE('',(#7997),#87729,.T.);
#90462=ADVANCED_FACE('',(#7998),#87730,.T.);
#90463=ADVANCED_FACE('',(#7999),#6243,.T.);
#90464=ADVANCED_FACE('',(#8000),#6244,.T.);
#90465=ADVANCED_FACE('',(#8001),#87731,.T.);
#90466=ADVANCED_FACE('',(#8002),#87732,.T.);
#90467=ADVANCED_FACE('',(#8003),#6245,.T.);
#90468=ADVANCED_FACE('',(#8004),#6246,.T.);
#90469=ADVANCED_FACE('',(#8005),#87733,.T.);
#90470=ADVANCED_FACE('',(#8006),#87734,.T.);
#90471=ADVANCED_FACE('',(#8007),#6247,.T.);
#90472=ADVANCED_FACE('',(#8008),#6248,.T.);
#90473=ADVANCED_FACE('',(#8009),#87735,.T.);
#90474=ADVANCED_FACE('',(#8010),#87736,.T.);
#90475=ADVANCED_FACE('',(#8011),#6249,.T.);
#90476=ADVANCED_FACE('',(#8012),#6250,.T.);
#90477=ADVANCED_FACE('',(#8013),#87737,.T.);
#90478=ADVANCED_FACE('',(#8014),#87738,.T.);
#90479=ADVANCED_FACE('',(#8015),#6251,.T.);
#90480=ADVANCED_FACE('',(#8016),#6252,.T.);
#90481=ADVANCED_FACE('',(#8017),#87739,.T.);
#90482=ADVANCED_FACE('',(#8018),#87740,.T.);
#90483=ADVANCED_FACE('',(#8019),#6253,.T.);
#90484=ADVANCED_FACE('',(#8020),#6254,.T.);
#90485=ADVANCED_FACE('',(#8021),#87741,.T.);
#90486=ADVANCED_FACE('',(#8022),#87742,.T.);
#90487=ADVANCED_FACE('',(#8023),#6255,.T.);
#90488=ADVANCED_FACE('',(#8024),#6256,.T.);
#90489=ADVANCED_FACE('',(#8025),#87743,.T.);
#90490=ADVANCED_FACE('',(#8026),#87744,.T.);
#90491=ADVANCED_FACE('',(#8027),#6257,.T.);
#90492=ADVANCED_FACE('',(#8028),#6258,.T.);
#90493=ADVANCED_FACE('',(#8029),#87745,.T.);
#90494=ADVANCED_FACE('',(#8030),#87746,.T.);
#90495=ADVANCED_FACE('',(#8031),#6259,.T.);
#90496=ADVANCED_FACE('',(#8032),#6260,.T.);
#90497=ADVANCED_FACE('',(#8033),#87747,.T.);
#90498=ADVANCED_FACE('',(#8034),#87748,.T.);
#90499=ADVANCED_FACE('',(#8035),#6261,.T.);
#90500=ADVANCED_FACE('',(#8036),#6262,.T.);
#90501=ADVANCED_FACE('',(#8037),#87749,.T.);
#90502=ADVANCED_FACE('',(#8038),#87750,.T.);
#90503=ADVANCED_FACE('',(#8039),#6263,.T.);
#90504=ADVANCED_FACE('',(#8040),#6264,.T.);
#90505=ADVANCED_FACE('',(#8041),#87751,.T.);
#90506=ADVANCED_FACE('',(#8042),#87752,.T.);
#90507=ADVANCED_FACE('',(#8043),#6265,.T.);
#90508=ADVANCED_FACE('',(#8044),#6266,.T.);
#90509=ADVANCED_FACE('',(#8045),#87753,.T.);
#90510=ADVANCED_FACE('',(#8046),#87754,.T.);
#90511=ADVANCED_FACE('',(#8047),#6267,.T.);
#90512=ADVANCED_FACE('',(#8048),#6268,.T.);
#90513=ADVANCED_FACE('',(#8049),#87755,.T.);
#90514=ADVANCED_FACE('',(#8050),#87756,.T.);
#90515=ADVANCED_FACE('',(#8051),#6269,.T.);
#90516=ADVANCED_FACE('',(#8052),#6270,.T.);
#90517=ADVANCED_FACE('',(#8053),#87757,.T.);
#90518=ADVANCED_FACE('',(#8054),#87758,.T.);
#90519=ADVANCED_FACE('',(#8055),#6271,.T.);
#90520=ADVANCED_FACE('',(#8056),#6272,.T.);
#90521=ADVANCED_FACE('',(#8057),#87759,.T.);
#90522=ADVANCED_FACE('',(#8058),#87760,.T.);
#90523=ADVANCED_FACE('',(#8059),#6273,.T.);
#90524=ADVANCED_FACE('',(#8060),#6274,.T.);
#90525=ADVANCED_FACE('',(#8061),#87761,.T.);
#90526=ADVANCED_FACE('',(#8062),#87762,.T.);
#90527=ADVANCED_FACE('',(#8063),#6275,.T.);
#90528=ADVANCED_FACE('',(#8064),#6276,.T.);
#90529=ADVANCED_FACE('',(#8065),#87763,.T.);
#90530=ADVANCED_FACE('',(#8066),#87764,.T.);
#90531=ADVANCED_FACE('',(#8067),#6277,.T.);
#90532=ADVANCED_FACE('',(#8068),#6278,.T.);
#90533=ADVANCED_FACE('',(#8069),#87765,.T.);
#90534=ADVANCED_FACE('',(#8070),#87766,.T.);
#90535=ADVANCED_FACE('',(#8071),#6279,.T.);
#90536=ADVANCED_FACE('',(#8072),#6280,.T.);
#90537=ADVANCED_FACE('',(#8073),#87767,.T.);
#90538=ADVANCED_FACE('',(#8074),#87768,.T.);
#90539=ADVANCED_FACE('',(#8075),#6281,.T.);
#90540=ADVANCED_FACE('',(#8076),#6282,.T.);
#90541=ADVANCED_FACE('',(#8077),#87769,.T.);
#90542=ADVANCED_FACE('',(#8078),#87770,.T.);
#90543=ADVANCED_FACE('',(#8079),#6283,.T.);
#90544=ADVANCED_FACE('',(#8080),#6284,.T.);
#90545=ADVANCED_FACE('',(#8081),#87771,.T.);
#90546=ADVANCED_FACE('',(#8082),#87772,.T.);
#90547=ADVANCED_FACE('',(#8083),#6285,.T.);
#90548=ADVANCED_FACE('',(#8084),#6286,.T.);
#90549=ADVANCED_FACE('',(#8085),#87773,.T.);
#90550=ADVANCED_FACE('',(#8086),#87774,.T.);
#90551=ADVANCED_FACE('',(#8087),#6287,.T.);
#90552=ADVANCED_FACE('',(#8088),#6288,.T.);
#90553=ADVANCED_FACE('',(#8089),#87775,.T.);
#90554=ADVANCED_FACE('',(#8090),#87776,.T.);
#90555=ADVANCED_FACE('',(#8091),#6289,.T.);
#90556=ADVANCED_FACE('',(#8092),#6290,.T.);
#90557=ADVANCED_FACE('',(#8093),#87777,.T.);
#90558=ADVANCED_FACE('',(#8094),#87778,.T.);
#90559=ADVANCED_FACE('',(#8095),#6291,.T.);
#90560=ADVANCED_FACE('',(#8096),#6292,.T.);
#90561=ADVANCED_FACE('',(#8097),#87779,.T.);
#90562=ADVANCED_FACE('',(#8098),#87780,.T.);
#90563=ADVANCED_FACE('',(#8099),#6293,.T.);
#90564=ADVANCED_FACE('',(#8100),#6294,.T.);
#90565=ADVANCED_FACE('',(#8101),#87781,.T.);
#90566=ADVANCED_FACE('',(#8102),#87782,.T.);
#90567=ADVANCED_FACE('',(#8103),#6295,.T.);
#90568=ADVANCED_FACE('',(#8104),#6296,.T.);
#90569=ADVANCED_FACE('',(#8105),#87783,.T.);
#90570=ADVANCED_FACE('',(#8106),#87784,.T.);
#90571=ADVANCED_FACE('',(#8107),#6297,.T.);
#90572=ADVANCED_FACE('',(#8108),#6298,.T.);
#90573=ADVANCED_FACE('',(#8109),#87785,.T.);
#90574=ADVANCED_FACE('',(#8110),#87786,.T.);
#90575=ADVANCED_FACE('',(#8111),#6299,.T.);
#90576=ADVANCED_FACE('',(#8112),#6300,.T.);
#90577=ADVANCED_FACE('',(#8113,#5187),#5608,.F.);
#90578=ADVANCED_FACE('',(#8114),#87787,.T.);
#90579=ADVANCED_FACE('',(#8115),#87788,.T.);
#90580=ADVANCED_FACE('',(#8116),#87789,.T.);
#90581=ADVANCED_FACE('',(#8117),#6301,.T.);
#90582=ADVANCED_FACE('',(#8118),#6302,.T.);
#90583=ADVANCED_FACE('',(#8119),#87790,.F.);
#90584=ADVANCED_FACE('',(#8120,#5188),#5609,.T.);
#90585=ADVANCED_FACE('',(#8121),#87791,.T.);
#90586=ADVANCED_FACE('',(#8122),#87792,.T.);
#90587=ADVANCED_FACE('',(#8123),#5610,.F.);
#90588=ADVANCED_FACE('',(#8124),#5611,.T.);
#90589=ADVANCED_FACE('',(#8125,#5189),#5612,.T.);
#90590=ADVANCED_FACE('',(#8126),#87793,.T.);
#90591=ADVANCED_FACE('',(#8127,#5190),#5613,.T.);
#90592=ADVANCED_FACE('',(#8128),#87794,.T.);
#90593=ADVANCED_FACE('',(#8129),#6303,.T.);
#90594=ADVANCED_FACE('',(#8130),#5614,.T.);
#90595=ADVANCED_FACE('',(#8131),#87795,.T.);
#90596=ADVANCED_FACE('',(#8132),#5615,.T.);
#90597=ADVANCED_FACE('',(#8133),#6304,.T.);
#90598=ADVANCED_FACE('',(#8134),#87796,.T.);
#90599=ADVANCED_FACE('',(#8135),#6305,.T.);
#90600=ADVANCED_FACE('',(#8136),#5616,.T.);
#90601=ADVANCED_FACE('',(#8137),#87797,.T.);
#90602=ADVANCED_FACE('',(#8138),#5617,.T.);
#90603=ADVANCED_FACE('',(#8139),#6306,.T.);
#90604=ADVANCED_FACE('',(#8140),#87798,.T.);
#90605=ADVANCED_FACE('',(#8141),#6307,.T.);
#90606=ADVANCED_FACE('',(#8142),#5618,.T.);
#90607=ADVANCED_FACE('',(#8143),#87799,.T.);
#90608=ADVANCED_FACE('',(#8144),#5619,.T.);
#90609=ADVANCED_FACE('',(#8145),#6308,.T.);
#90610=ADVANCED_FACE('',(#8146),#87800,.T.);
#90611=ADVANCED_FACE('',(#8147),#6309,.T.);
#90612=ADVANCED_FACE('',(#8148),#5620,.T.);
#90613=ADVANCED_FACE('',(#8149),#87801,.T.);
#90614=ADVANCED_FACE('',(#8150),#5621,.T.);
#90615=ADVANCED_FACE('',(#8151),#6310,.T.);
#90616=ADVANCED_FACE('',(#8152),#87802,.T.);
#90617=ADVANCED_FACE('',(#8153),#6311,.T.);
#90618=ADVANCED_FACE('',(#8154),#5622,.T.);
#90619=ADVANCED_FACE('',(#8155),#87803,.T.);
#90620=ADVANCED_FACE('',(#8156),#5623,.T.);
#90621=ADVANCED_FACE('',(#8157),#6312,.T.);
#90622=ADVANCED_FACE('',(#8158),#87804,.T.);
#90623=ADVANCED_FACE('',(#8159),#6313,.T.);
#90624=ADVANCED_FACE('',(#8160),#5624,.T.);
#90625=ADVANCED_FACE('',(#8161),#87805,.T.);
#90626=ADVANCED_FACE('',(#8162),#5625,.T.);
#90627=ADVANCED_FACE('',(#8163),#6314,.T.);
#90628=ADVANCED_FACE('',(#8164),#87806,.T.);
#90629=ADVANCED_FACE('',(#8165),#6315,.T.);
#90630=ADVANCED_FACE('',(#8166),#5626,.T.);
#90631=ADVANCED_FACE('',(#8167),#87807,.T.);
#90632=ADVANCED_FACE('',(#8168),#5627,.T.);
#90633=ADVANCED_FACE('',(#8169),#6316,.T.);
#90634=ADVANCED_FACE('',(#8170),#87808,.T.);
#90635=ADVANCED_FACE('',(#8171),#6317,.T.);
#90636=ADVANCED_FACE('',(#8172),#5628,.T.);
#90637=ADVANCED_FACE('',(#8173),#87809,.T.);
#90638=ADVANCED_FACE('',(#8174),#5629,.T.);
#90639=ADVANCED_FACE('',(#8175),#6318,.T.);
#90640=ADVANCED_FACE('',(#8176),#87810,.T.);
#90641=ADVANCED_FACE('',(#8177),#6319,.T.);
#90642=ADVANCED_FACE('',(#8178),#5630,.T.);
#90643=ADVANCED_FACE('',(#8179,#5191),#5631,.T.);
#90644=ADVANCED_FACE('',(#8180),#5632,.T.);
#90645=ADVANCED_FACE('',(#8181),#6320,.T.);
#90646=ADVANCED_FACE('',(#8182),#87811,.T.);
#90647=ADVANCED_FACE('',(#8183),#5633,.T.);
#90648=ADVANCED_FACE('',(#8184),#6321,.T.);
#90649=ADVANCED_FACE('',(#8185),#87812,.T.);
#90650=ADVANCED_FACE('',(#8186),#6322,.T.);
#90651=ADVANCED_FACE('',(#8187),#5634,.T.);
#90652=ADVANCED_FACE('',(#8188),#87813,.T.);
#90653=ADVANCED_FACE('',(#8189),#5635,.T.);
#90654=ADVANCED_FACE('',(#8190),#5636,.T.);
#90655=ADVANCED_FACE('',(#8191),#6323,.T.);
#90656=ADVANCED_FACE('',(#8192),#87814,.T.);
#90657=ADVANCED_FACE('',(#8193),#6324,.T.);
#90658=ADVANCED_FACE('',(#8194),#5637,.T.);
#90659=ADVANCED_FACE('',(#8195),#5638,.T.);
#90660=ADVANCED_FACE('',(#8196),#6325,.T.);
#90661=ADVANCED_FACE('',(#8197),#87815,.T.);
#90662=ADVANCED_FACE('',(#8198),#6326,.T.);
#90663=ADVANCED_FACE('',(#8199),#87816,.T.);
#90664=ADVANCED_FACE('',(#8200),#5639,.T.);
#90665=ADVANCED_FACE('',(#8201),#6327,.T.);
#90666=ADVANCED_FACE('',(#8202),#87817,.T.);
#90667=ADVANCED_FACE('',(#8203),#6328,.T.);
#90668=ADVANCED_FACE('',(#8204),#5640,.T.);
#90669=ADVANCED_FACE('',(#8205),#87818,.T.);
#90670=ADVANCED_FACE('',(#8206),#87819,.T.);
#90671=ADVANCED_FACE('',(#8207),#5641,.T.);
#90672=ADVANCED_FACE('',(#8208),#5642,.T.);
#90673=ADVANCED_FACE('',(#8209),#6329,.T.);
#90674=ADVANCED_FACE('',(#8210),#87820,.T.);
#90675=ADVANCED_FACE('',(#8211),#6330,.T.);
#90676=ADVANCED_FACE('',(#8212),#5643,.T.);
#90677=ADVANCED_FACE('',(#8213),#5644,.T.);
#90678=ADVANCED_FACE('',(#8214),#6331,.T.);
#90679=ADVANCED_FACE('',(#8215),#87821,.T.);
#90680=ADVANCED_FACE('',(#8216),#6332,.T.);
#90681=ADVANCED_FACE('',(#8217),#87822,.T.);
#90682=ADVANCED_FACE('',(#8218),#5645,.T.);
#90683=ADVANCED_FACE('',(#8219),#6333,.T.);
#90684=ADVANCED_FACE('',(#8220),#87823,.T.);
#90685=ADVANCED_FACE('',(#8221),#6334,.T.);
#90686=ADVANCED_FACE('',(#8222),#5646,.T.);
#90687=ADVANCED_FACE('',(#8223),#87824,.T.);
#90688=ADVANCED_FACE('',(#8224),#87825,.T.);
#90689=ADVANCED_FACE('',(#8225),#5647,.T.);
#90690=ADVANCED_FACE('',(#8226),#5648,.T.);
#90691=ADVANCED_FACE('',(#8227),#6335,.T.);
#90692=ADVANCED_FACE('',(#8228),#87826,.T.);
#90693=ADVANCED_FACE('',(#8229),#6336,.T.);
#90694=ADVANCED_FACE('',(#8230),#87827,.T.);
#90695=ADVANCED_FACE('',(#8231),#87828,.T.);
#90696=ADVANCED_FACE('',(#8232,#5192),#5649,.T.);
#94634=CLOSED_SHELL('',(#90406,#90407,#90408,#90409,#90410,#90411,#90412,
#90413,#90414,#90415,#90416,#90417,#90418,#90419,#90420,#90421,#90422,#90423,
#90424,#90425,#90426,#90427,#90428,#90429,#90430,#90431,#90432,#90433,#90434,
#90435,#90436,#90437,#90438,#90439,#90440,#90441,#90442,#90443,#90444,#90445,
#90446,#90447,#90448,#90449,#90450,#90451,#90452,#90453,#90454,#90455,#90456,
#90457,#90458,#90459,#90460,#90461,#90462,#90463,#90464,#90465,#90466,#90467,
#90468,#90469,#90470,#90471,#90472,#90473,#90474,#90475,#90476,#90477,#90478,
#90479,#90480,#90481,#90482,#90483,#90484,#90485,#90486,#90487,#90488,#90489,
#90490,#90491,#90492,#90493,#90494,#90495,#90496,#90497,#90498,#90499,#90500,
#90501,#90502,#90503,#90504,#90505,#90506,#90507,#90508,#90509,#90510,#90511,
#90512,#90513,#90514,#90515,#90516,#90517,#90518,#90519,#90520,#90521,#90522,
#90523,#90524,#90525,#90526,#90527,#90528,#90529,#90530,#90531,#90532,#90533,
#90534,#90535,#90536,#90537,#90538,#90539,#90540,#90541,#90542,#90543,#90544,
#90545,#90546,#90547,#90548,#90549,#90550,#90551,#90552,#90553,#90554,#90555,
#90556,#90557,#90558,#90559,#90560,#90561,#90562,#90563,#90564,#90565,#90566,
#90567,#90568,#90569,#90570,#90571,#90572,#90573,#90574,#90575,#90576,#90577,
#90578,#90579,#90580,#90581,#90582,#90583,#90584));
#94635=CLOSED_SHELL('',(#90585,#90586,#90587,#90588,#90589,#90590,#90591,
#90592,#90593,#90594,#90595,#90596,#90597,#90598,#90599,#90600,#90601,#90602,
#90603,#90604,#90605,#90606,#90607,#90608,#90609,#90610,#90611,#90612,#90613,
#90614,#90615,#90616,#90617,#90618,#90619,#90620,#90621,#90622,#90623,#90624,
#90625,#90626,#90627,#90628,#90629,#90630,#90631,#90632,#90633,#90634,#90635,
#90636,#90637,#90638,#90639,#90640,#90641,#90642,#90643,#90644,#90645,#90646,
#90647,#90648,#90649,#90650,#90651,#90652,#90653,#90654,#90655,#90656,#90657,
#90658,#90659,#90660,#90661,#90662,#90663,#90664,#90665,#90666,#90667,#90668,
#90669,#90670,#90671,#90672,#90673,#90674,#90675,#90676,#90677,#90678,#90679,
#90680,#90681,#90682,#90683,#90684,#90685,#90686,#90687,#90688,#90689,#90690,
#90691,#90692,#90693,#90694,#90695,#90696));
#98432=AXIS2_PLACEMENT_3D('',#153537,#114071,#114072);
#98433=AXIS2_PLACEMENT_3D('',#153538,#114073,#114074);
#98434=AXIS2_PLACEMENT_3D('',#153541,#114075,#114076);
#98435=AXIS2_PLACEMENT_3D('',#153545,#114078,#114079);
#98436=AXIS2_PLACEMENT_3D('',#157327,#114083,#114084);
#98437=AXIS2_PLACEMENT_3D('',#157331,#114086,#114087);
#98438=AXIS2_PLACEMENT_3D('',#157332,#114088,#114089);
#98439=AXIS2_PLACEMENT_3D('',#157333,#114090,#114091);
#98440=AXIS2_PLACEMENT_3D('',#157336,#114092,#114093);
#98441=AXIS2_PLACEMENT_3D('',#157340,#114095,#114096);
#98442=AXIS2_PLACEMENT_3D('',#160815,#114099,#114100);
#98443=AXIS2_PLACEMENT_3D('',#160819,#114102,#114103);
#98444=AXIS2_PLACEMENT_3D('',#160820,#114104,#114105);
#98445=AXIS2_PLACEMENT_3D('',#160821,#114106,#114107);
#98446=AXIS2_PLACEMENT_3D('',#160824,#114108,#114109);
#98447=AXIS2_PLACEMENT_3D('',#160828,#114111,#114112);
#98448=AXIS2_PLACEMENT_3D('',#164015,#114115,#114116);
#98449=AXIS2_PLACEMENT_3D('',#164019,#114118,#114119);
#98450=AXIS2_PLACEMENT_3D('',#164020,#114120,#114121);
#98451=AXIS2_PLACEMENT_3D('',#164021,#114122,#114123);
#98452=AXIS2_PLACEMENT_3D('',#164024,#114124,#114125);
#98453=AXIS2_PLACEMENT_3D('',#164028,#114127,#114128);
#98454=AXIS2_PLACEMENT_3D('',#167215,#114131,#114132);
#98455=AXIS2_PLACEMENT_3D('',#167219,#114134,#114135);
#98456=AXIS2_PLACEMENT_3D('',#167220,#114136,#114137);
#98457=AXIS2_PLACEMENT_3D('',#167221,#114138,#114139);
#98458=AXIS2_PLACEMENT_3D('',#167224,#114140,#114141);
#98459=AXIS2_PLACEMENT_3D('',#167228,#114143,#114144);
#98460=AXIS2_PLACEMENT_3D('',#171009,#114147,#114148);
#98461=AXIS2_PLACEMENT_3D('',#171013,#114150,#114151);
#98462=AXIS2_PLACEMENT_3D('',#171014,#114152,#114153);
#98463=AXIS2_PLACEMENT_3D('',#171015,#114154,#114155);
#98464=AXIS2_PLACEMENT_3D('',#171018,#114156,#114157);
#98465=AXIS2_PLACEMENT_3D('',#171022,#114159,#114160);
#98466=AXIS2_PLACEMENT_3D('',#174497,#114163,#114164);
#98467=AXIS2_PLACEMENT_3D('',#174501,#114166,#114167);
#98468=AXIS2_PLACEMENT_3D('',#174502,#114168,#114169);
#98469=AXIS2_PLACEMENT_3D('',#174503,#114170,#114171);
#98470=AXIS2_PLACEMENT_3D('',#174506,#114172,#114173);
#98471=AXIS2_PLACEMENT_3D('',#174510,#114175,#114176);
#98472=AXIS2_PLACEMENT_3D('',#177706,#114179,#114180);
#98473=AXIS2_PLACEMENT_3D('',#177710,#114182,#114183);
#98474=AXIS2_PLACEMENT_3D('',#177711,#114184,#114185);
#98475=AXIS2_PLACEMENT_3D('',#177712,#114186,#114187);
#98476=AXIS2_PLACEMENT_3D('',#177715,#114188,#114189);
#98477=AXIS2_PLACEMENT_3D('',#177719,#114191,#114192);
#98478=AXIS2_PLACEMENT_3D('',#181197,#114195,#114196);
#98479=AXIS2_PLACEMENT_3D('',#181201,#114198,#114199);
#98480=AXIS2_PLACEMENT_3D('',#181202,#114200,#114201);
#98481=AXIS2_PLACEMENT_3D('',#181203,#114202,#114203);
#98482=AXIS2_PLACEMENT_3D('',#181206,#114204,#114205);
#98483=AXIS2_PLACEMENT_3D('',#181210,#114207,#114208);
#98484=AXIS2_PLACEMENT_3D('',#184679,#114211,#114212);
#98485=AXIS2_PLACEMENT_3D('',#184683,#114214,#114215);
#98486=AXIS2_PLACEMENT_3D('',#184684,#114216,#114217);
#98487=AXIS2_PLACEMENT_3D('',#184685,#114218,#114219);
#98488=AXIS2_PLACEMENT_3D('',#184688,#114220,#114221);
#98489=AXIS2_PLACEMENT_3D('',#184692,#114223,#114224);
#98490=AXIS2_PLACEMENT_3D('',#187867,#114227,#114228);
#98491=AXIS2_PLACEMENT_3D('',#187871,#114230,#114231);
#98492=AXIS2_PLACEMENT_3D('',#187872,#114232,#114233);
#98493=AXIS2_PLACEMENT_3D('',#187873,#114234,#114235);
#98494=AXIS2_PLACEMENT_3D('',#187876,#114236,#114237);
#98495=AXIS2_PLACEMENT_3D('',#187880,#114239,#114240);
#98496=AXIS2_PLACEMENT_3D('',#191001,#114243,#114244);
#98497=AXIS2_PLACEMENT_3D('',#191005,#114246,#114247);
#98498=AXIS2_PLACEMENT_3D('',#191006,#114248,#114249);
#98499=AXIS2_PLACEMENT_3D('',#191007,#114250,#114251);
#98500=AXIS2_PLACEMENT_3D('',#191010,#114252,#114253);
#98501=AXIS2_PLACEMENT_3D('',#191014,#114255,#114256);
#98502=AXIS2_PLACEMENT_3D('',#194469,#114259,#114260);
#98503=AXIS2_PLACEMENT_3D('',#194473,#114262,#114263);
#98504=AXIS2_PLACEMENT_3D('',#194474,#114264,#114265);
#98505=AXIS2_PLACEMENT_3D('',#194475,#114266,#114267);
#98506=AXIS2_PLACEMENT_3D('',#194478,#114268,#114269);
#98507=AXIS2_PLACEMENT_3D('',#194482,#114271,#114272);
#98508=AXIS2_PLACEMENT_3D('',#197945,#114275,#114276);
#98509=AXIS2_PLACEMENT_3D('',#197949,#114278,#114279);
#98510=AXIS2_PLACEMENT_3D('',#197950,#114280,#114281);
#98511=AXIS2_PLACEMENT_3D('',#197951,#114282,#114283);
#98512=AXIS2_PLACEMENT_3D('',#197954,#114284,#114285);
#98513=AXIS2_PLACEMENT_3D('',#197958,#114287,#114288);
#98514=AXIS2_PLACEMENT_3D('',#201103,#114291,#114292);
#98515=AXIS2_PLACEMENT_3D('',#201107,#114294,#114295);
#98516=AXIS2_PLACEMENT_3D('',#201108,#114296,#114297);
#98517=AXIS2_PLACEMENT_3D('',#201109,#114298,#114299);
#98518=AXIS2_PLACEMENT_3D('',#201112,#114300,#114301);
#98519=AXIS2_PLACEMENT_3D('',#201116,#114303,#114304);
#98520=AXIS2_PLACEMENT_3D('',#204279,#114307,#114308);
#98521=AXIS2_PLACEMENT_3D('',#204283,#114310,#114311);
#98522=AXIS2_PLACEMENT_3D('',#204284,#114312,#114313);
#98523=AXIS2_PLACEMENT_3D('',#204285,#114314,#114315);
#98524=AXIS2_PLACEMENT_3D('',#204288,#114316,#114317);
#98525=AXIS2_PLACEMENT_3D('',#204292,#114319,#114320);
#98526=AXIS2_PLACEMENT_3D('',#207431,#114323,#114324);
#98527=AXIS2_PLACEMENT_3D('',#207435,#114326,#114327);
#98528=AXIS2_PLACEMENT_3D('',#207436,#114328,#114329);
#98529=AXIS2_PLACEMENT_3D('',#207437,#114330,#114331);
#98530=AXIS2_PLACEMENT_3D('',#207440,#114332,#114333);
#98531=AXIS2_PLACEMENT_3D('',#207444,#114335,#114336);
#98532=AXIS2_PLACEMENT_3D('',#210610,#114339,#114340);
#98533=AXIS2_PLACEMENT_3D('',#210614,#114342,#114343);
#98534=AXIS2_PLACEMENT_3D('',#210615,#114344,#114345);
#98535=AXIS2_PLACEMENT_3D('',#210616,#114346,#114347);
#98536=AXIS2_PLACEMENT_3D('',#210619,#114348,#114349);
#98537=AXIS2_PLACEMENT_3D('',#210623,#114351,#114352);
#98538=AXIS2_PLACEMENT_3D('',#213774,#114355,#114356);
#98539=AXIS2_PLACEMENT_3D('',#213778,#114358,#114359);
#98540=AXIS2_PLACEMENT_3D('',#213779,#114360,#114361);
#98541=AXIS2_PLACEMENT_3D('',#213780,#114362,#114363);
#98542=AXIS2_PLACEMENT_3D('',#213783,#114364,#114365);
#98543=AXIS2_PLACEMENT_3D('',#213787,#114367,#114368);
#98544=AXIS2_PLACEMENT_3D('',#216941,#114371,#114372);
#98545=AXIS2_PLACEMENT_3D('',#216945,#114374,#114375);
#98546=AXIS2_PLACEMENT_3D('',#216946,#114376,#114377);
#98547=AXIS2_PLACEMENT_3D('',#216947,#114378,#114379);
#98548=AXIS2_PLACEMENT_3D('',#216950,#114380,#114381);
#98549=AXIS2_PLACEMENT_3D('',#216954,#114383,#114384);
#98550=AXIS2_PLACEMENT_3D('',#220406,#114387,#114388);
#98551=AXIS2_PLACEMENT_3D('',#220410,#114390,#114391);
#98552=AXIS2_PLACEMENT_3D('',#220411,#114392,#114393);
#98553=AXIS2_PLACEMENT_3D('',#220412,#114394,#114395);
#98554=AXIS2_PLACEMENT_3D('',#220415,#114396,#114397);
#98555=AXIS2_PLACEMENT_3D('',#220419,#114399,#114400);
#98556=AXIS2_PLACEMENT_3D('',#223549,#114403,#114404);
#98557=AXIS2_PLACEMENT_3D('',#223553,#114406,#114407);
#98558=AXIS2_PLACEMENT_3D('',#223554,#114408,#114409);
#98559=AXIS2_PLACEMENT_3D('',#223555,#114410,#114411);
#98560=AXIS2_PLACEMENT_3D('',#223558,#114412,#114413);
#98561=AXIS2_PLACEMENT_3D('',#223562,#114415,#114416);
#98562=AXIS2_PLACEMENT_3D('',#226993,#114419,#114420);
#98563=AXIS2_PLACEMENT_3D('',#226997,#114422,#114423);
#98564=AXIS2_PLACEMENT_3D('',#226998,#114424,#114425);
#98565=AXIS2_PLACEMENT_3D('',#226999,#114426,#114427);
#98566=AXIS2_PLACEMENT_3D('',#227002,#114428,#114429);
#98567=AXIS2_PLACEMENT_3D('',#227006,#114431,#114432);
#98568=AXIS2_PLACEMENT_3D('',#230133,#114435,#114436);
#98569=AXIS2_PLACEMENT_3D('',#230137,#114438,#114439);
#98570=AXIS2_PLACEMENT_3D('',#230138,#114440,#114441);
#98571=AXIS2_PLACEMENT_3D('',#230139,#114442,#114443);
#98572=AXIS2_PLACEMENT_3D('',#230142,#114444,#114445);
#98573=AXIS2_PLACEMENT_3D('',#230146,#114447,#114448);
#98574=AXIS2_PLACEMENT_3D('',#233273,#114451,#114452);
#98575=AXIS2_PLACEMENT_3D('',#233277,#114454,#114455);
#98576=AXIS2_PLACEMENT_3D('',#233278,#114456,#114457);
#98577=AXIS2_PLACEMENT_3D('',#233279,#114458,#114459);
#98578=AXIS2_PLACEMENT_3D('',#233282,#114460,#114461);
#98579=AXIS2_PLACEMENT_3D('',#233286,#114463,#114464);
#98580=AXIS2_PLACEMENT_3D('',#236431,#114467,#114468);
#98581=AXIS2_PLACEMENT_3D('',#236435,#114470,#114471);
#98582=AXIS2_PLACEMENT_3D('',#236436,#114472,#114473);
#98583=AXIS2_PLACEMENT_3D('',#236437,#114474,#114475);
#98584=AXIS2_PLACEMENT_3D('',#236440,#114476,#114477);
#98585=AXIS2_PLACEMENT_3D('',#236444,#114479,#114480);
#98586=AXIS2_PLACEMENT_3D('',#239601,#114483,#114484);
#98587=AXIS2_PLACEMENT_3D('',#239605,#114486,#114487);
#98588=AXIS2_PLACEMENT_3D('',#239606,#114488,#114489);
#98589=AXIS2_PLACEMENT_3D('',#239607,#114490,#114491);
#98590=AXIS2_PLACEMENT_3D('',#239610,#114492,#114493);
#98591=AXIS2_PLACEMENT_3D('',#239614,#114495,#114496);
#98592=AXIS2_PLACEMENT_3D('',#242768,#114499,#114500);
#98593=AXIS2_PLACEMENT_3D('',#242772,#114502,#114503);
#98594=AXIS2_PLACEMENT_3D('',#242773,#114504,#114505);
#98595=AXIS2_PLACEMENT_3D('',#242774,#114506,#114507);
#98596=AXIS2_PLACEMENT_3D('',#242777,#114508,#114509);
#98597=AXIS2_PLACEMENT_3D('',#242781,#114511,#114512);
#98598=AXIS2_PLACEMENT_3D('',#246250,#114515,#114516);
#98599=AXIS2_PLACEMENT_3D('',#246254,#114518,#114519);
#98600=AXIS2_PLACEMENT_3D('',#246255,#114520,#114521);
#98601=AXIS2_PLACEMENT_3D('',#246256,#114522,#114523);
#98602=AXIS2_PLACEMENT_3D('',#246259,#114524,#114525);
#98603=AXIS2_PLACEMENT_3D('',#246263,#114527,#114528);
#98604=AXIS2_PLACEMENT_3D('',#249423,#114531,#114532);
#98605=AXIS2_PLACEMENT_3D('',#249427,#114534,#114535);
#98606=AXIS2_PLACEMENT_3D('',#249428,#114536,#114537);
#98607=AXIS2_PLACEMENT_3D('',#249429,#114538,#114539);
#98608=AXIS2_PLACEMENT_3D('',#249432,#114540,#114541);
#98609=AXIS2_PLACEMENT_3D('',#249436,#114543,#114544);
#98610=AXIS2_PLACEMENT_3D('',#252596,#114547,#114548);
#98611=AXIS2_PLACEMENT_3D('',#252600,#114550,#114551);
#98612=AXIS2_PLACEMENT_3D('',#252601,#114552,#114553);
#98613=AXIS2_PLACEMENT_3D('',#252602,#114554,#114555);
#98614=AXIS2_PLACEMENT_3D('',#252605,#114556,#114557);
#98615=AXIS2_PLACEMENT_3D('',#252609,#114559,#114560);
#98616=AXIS2_PLACEMENT_3D('',#255748,#114563,#114564);
#98617=AXIS2_PLACEMENT_3D('',#255752,#114566,#114567);
#98618=AXIS2_PLACEMENT_3D('',#255753,#114568,#114569);
#98619=AXIS2_PLACEMENT_3D('',#255754,#114570,#114571);
#98620=AXIS2_PLACEMENT_3D('',#255757,#114572,#114573);
#98621=AXIS2_PLACEMENT_3D('',#255761,#114575,#114576);
#98622=AXIS2_PLACEMENT_3D('',#258897,#114579,#114580);
#98623=AXIS2_PLACEMENT_3D('',#258901,#114582,#114583);
#98624=AXIS2_PLACEMENT_3D('',#258902,#114584,#114585);
#98625=AXIS2_PLACEMENT_3D('',#258903,#114586,#114587);
#98626=AXIS2_PLACEMENT_3D('',#258906,#114588,#114589);
#98627=AXIS2_PLACEMENT_3D('',#258910,#114591,#114592);
#98628=AXIS2_PLACEMENT_3D('',#262689,#114595,#114596);
#98629=AXIS2_PLACEMENT_3D('',#262693,#114598,#114599);
#98630=AXIS2_PLACEMENT_3D('',#262694,#114600,#114601);
#98631=AXIS2_PLACEMENT_3D('',#262695,#114602,#114603);
#98632=AXIS2_PLACEMENT_3D('',#262698,#114604,#114605);
#98633=AXIS2_PLACEMENT_3D('',#262702,#114607,#114608);
#98634=AXIS2_PLACEMENT_3D('',#266143,#114611,#114612);
#98635=AXIS2_PLACEMENT_3D('',#266147,#114614,#114615);
#98636=AXIS2_PLACEMENT_3D('',#266148,#114616,#114617);
#98637=AXIS2_PLACEMENT_3D('',#266149,#114618,#114619);
#98638=AXIS2_PLACEMENT_3D('',#266152,#114620,#114621);
#98639=AXIS2_PLACEMENT_3D('',#266156,#114623,#114624);
#98640=AXIS2_PLACEMENT_3D('',#269632,#114627,#114628);
#98641=AXIS2_PLACEMENT_3D('',#269636,#114630,#114631);
#98642=AXIS2_PLACEMENT_3D('',#269637,#114632,#114633);
#98643=AXIS2_PLACEMENT_3D('',#269638,#114634,#114635);
#98644=AXIS2_PLACEMENT_3D('',#269641,#114636,#114637);
#98645=AXIS2_PLACEMENT_3D('',#269645,#114639,#114640);
#98646=AXIS2_PLACEMENT_3D('',#272829,#114643,#114644);
#98647=AXIS2_PLACEMENT_3D('',#272833,#114646,#114647);
#98648=AXIS2_PLACEMENT_3D('',#272834,#114648,#114649);
#98649=AXIS2_PLACEMENT_3D('',#272835,#114650,#114651);
#98650=AXIS2_PLACEMENT_3D('',#272838,#114652,#114653);
#98651=AXIS2_PLACEMENT_3D('',#272842,#114655,#114656);
#98652=AXIS2_PLACEMENT_3D('',#276032,#114659,#114660);
#98653=AXIS2_PLACEMENT_3D('',#276036,#114662,#114663);
#98654=AXIS2_PLACEMENT_3D('',#276037,#114664,#114665);
#98655=AXIS2_PLACEMENT_3D('',#276038,#114666,#114667);
#98656=AXIS2_PLACEMENT_3D('',#276041,#114668,#114669);
#98657=AXIS2_PLACEMENT_3D('',#276045,#114671,#114672);
#98658=AXIS2_PLACEMENT_3D('',#279527,#114675,#114676);
#98659=AXIS2_PLACEMENT_3D('',#279531,#114678,#114679);
#98660=AXIS2_PLACEMENT_3D('',#279532,#114680,#114681);
#98661=AXIS2_PLACEMENT_3D('',#279533,#114682,#114683);
#98662=AXIS2_PLACEMENT_3D('',#279536,#114684,#114685);
#98663=AXIS2_PLACEMENT_3D('',#279540,#114687,#114688);
#98664=AXIS2_PLACEMENT_3D('',#282736,#114691,#114692);
#98665=AXIS2_PLACEMENT_3D('',#282740,#114694,#114695);
#98666=AXIS2_PLACEMENT_3D('',#282741,#114696,#114697);
#98667=AXIS2_PLACEMENT_3D('',#282742,#114698,#114699);
#98668=AXIS2_PLACEMENT_3D('',#282745,#114700,#114701);
#98669=AXIS2_PLACEMENT_3D('',#282749,#114703,#114704);
#98670=AXIS2_PLACEMENT_3D('',#286530,#114707,#114708);
#98671=AXIS2_PLACEMENT_3D('',#286534,#114710,#114711);
#98672=AXIS2_PLACEMENT_3D('',#286535,#114712,#114713);
#98673=AXIS2_PLACEMENT_3D('',#286536,#114714,#114715);
#98674=AXIS2_PLACEMENT_3D('',#286539,#114716,#114717);
#98675=AXIS2_PLACEMENT_3D('',#286543,#114719,#114720);
#98676=AXIS2_PLACEMENT_3D('',#290025,#114723,#114724);
#98677=AXIS2_PLACEMENT_3D('',#290029,#114726,#114727);
#98678=AXIS2_PLACEMENT_3D('',#290030,#114728,#114729);
#98679=AXIS2_PLACEMENT_3D('',#290031,#114730,#114731);
#98680=AXIS2_PLACEMENT_3D('',#290034,#114732,#114733);
#98681=AXIS2_PLACEMENT_3D('',#290038,#114735,#114736);
#98682=AXIS2_PLACEMENT_3D('',#293213,#114739,#114740);
#98683=AXIS2_PLACEMENT_3D('',#293217,#114742,#114743);
#98684=AXIS2_PLACEMENT_3D('',#293218,#114744,#114745);
#98685=AXIS2_PLACEMENT_3D('',#293219,#114746,#114747);
#98686=AXIS2_PLACEMENT_3D('',#293222,#114748,#114749);
#98687=AXIS2_PLACEMENT_3D('',#293226,#114751,#114752);
#98688=AXIS2_PLACEMENT_3D('',#296698,#114755,#114756);
#98689=AXIS2_PLACEMENT_3D('',#296700,#114757,#114758);
#98690=AXIS2_PLACEMENT_3D('',#296702,#114759,#114760);
#98691=AXIS2_PLACEMENT_3D('',#297176,#114761,#114762);
#98692=AXIS2_PLACEMENT_3D('',#297500,#114763,#114764);
#98693=AXIS2_PLACEMENT_3D('',#297501,#114765,#114766);
#98694=AXIS2_PLACEMENT_3D('',#297504,#114768,#114769);
#98695=AXIS2_PLACEMENT_3D('',#297505,#114770,#114771);
#98696=AXIS2_PLACEMENT_3D('',#297508,#114773,#114774);
#98697=AXIS2_PLACEMENT_3D('',#297509,#114775,#114776);
#98698=AXIS2_PLACEMENT_3D('',#297513,#114778,#114779);
#98699=AXIS2_PLACEMENT_3D('',#300196,#114781,#114782);
#98700=AXIS2_PLACEMENT_3D('',#300199,#114784,#114785);
#98701=AXIS2_PLACEMENT_3D('',#300200,#114786,#114787);
#98702=AXIS2_PLACEMENT_3D('',#300201,#114788,#114789);
#98703=AXIS2_PLACEMENT_3D('',#300203,#114790,#114791);
#98704=AXIS2_PLACEMENT_3D('',#300206,#114793,#114794);
#98705=AXIS2_PLACEMENT_3D('',#300207,#114795,#114796);
#98706=AXIS2_PLACEMENT_3D('',#300209,#114797,#114798);
#98707=AXIS2_PLACEMENT_3D('',#300212,#114800,#114801);
#98708=AXIS2_PLACEMENT_3D('',#300213,#114802,#114803);
#98709=AXIS2_PLACEMENT_3D('',#300214,#114804,#114805);
#98710=AXIS2_PLACEMENT_3D('',#300215,#114806,#114807);
#98711=AXIS2_PLACEMENT_3D('',#300220,#114809,#114810);
#98712=AXIS2_PLACEMENT_3D('',#300239,#114812,#114813);
#98713=AXIS2_PLACEMENT_3D('',#300287,#114815,#114816);
#98714=AXIS2_PLACEMENT_3D('',#300308,#114818,#114819);
#98715=AXIS2_PLACEMENT_3D('',#300359,#114821,#114822);
#98716=AXIS2_PLACEMENT_3D('',#300380,#114824,#114825);
#98717=AXIS2_PLACEMENT_3D('',#300431,#114827,#114828);
#98718=AXIS2_PLACEMENT_3D('',#300452,#114830,#114831);
#98719=AXIS2_PLACEMENT_3D('',#300503,#114833,#114834);
#98720=AXIS2_PLACEMENT_3D('',#300522,#114836,#114837);
#98721=AXIS2_PLACEMENT_3D('',#300570,#114839,#114840);
#98722=AXIS2_PLACEMENT_3D('',#300591,#114842,#114843);
#98723=AXIS2_PLACEMENT_3D('',#300612,#114845,#114846);
#98724=AXIS2_PLACEMENT_3D('',#300633,#114848,#114849);
#98725=AXIS2_PLACEMENT_3D('',#300684,#114851,#114852);
#98726=AXIS2_PLACEMENT_3D('',#300705,#114854,#114855);
#98727=AXIS2_PLACEMENT_3D('',#300720,#114857,#114858);
#98728=AXIS2_PLACEMENT_3D('',#300741,#114860,#114861);
#98729=AXIS2_PLACEMENT_3D('',#300789,#114863,#114864);
#98730=AXIS2_PLACEMENT_3D('',#300810,#114866,#114867);
#98731=AXIS2_PLACEMENT_3D('',#300858,#114869,#114870);
#98732=AXIS2_PLACEMENT_3D('',#300879,#114872,#114873);
#98733=AXIS2_PLACEMENT_3D('',#300900,#114875,#114876);
#98734=AXIS2_PLACEMENT_3D('',#300921,#114878,#114879);
#98735=AXIS2_PLACEMENT_3D('',#300969,#114881,#114882);
#98736=AXIS2_PLACEMENT_3D('',#300990,#114884,#114885);
#98737=AXIS2_PLACEMENT_3D('',#301011,#114887,#114888);
#98738=AXIS2_PLACEMENT_3D('',#301032,#114890,#114891);
#98739=AXIS2_PLACEMENT_3D('',#301080,#114893,#114894);
#98740=AXIS2_PLACEMENT_3D('',#301101,#114896,#114897);
#98741=AXIS2_PLACEMENT_3D('',#301149,#114899,#114900);
#98742=AXIS2_PLACEMENT_3D('',#301168,#114902,#114903);
#98743=AXIS2_PLACEMENT_3D('',#301216,#114905,#114906);
#98744=AXIS2_PLACEMENT_3D('',#301237,#114908,#114909);
#98745=AXIS2_PLACEMENT_3D('',#301282,#114910,#114911);
#98746=AXIS2_PLACEMENT_3D('',#301283,#114912,#114913);
#98747=AXIS2_PLACEMENT_3D('',#301285,#114914,#114915);
#98748=AXIS2_PLACEMENT_3D('',#301288,#114917,#114918);
#98749=AXIS2_PLACEMENT_3D('',#301289,#114919,#114920);
#98750=AXIS2_PLACEMENT_3D('',#301290,#114921,#114922);
#98751=AXIS2_PLACEMENT_3D('',#301294,#114924,#114925);
#98752=AXIS2_PLACEMENT_3D('',#302956,#114928,#114929);
#98753=AXIS2_PLACEMENT_3D('',#302960,#114932,#114933);
#98754=AXIS2_PLACEMENT_3D('',#302963,#114935,#114936);
#98755=AXIS2_PLACEMENT_3D('',#302964,#114937,#114938);
#98756=AXIS2_PLACEMENT_3D('',#304631,#114942,#114943);
#98757=AXIS2_PLACEMENT_3D('',#304634,#114945,#114946);
#98758=AXIS2_PLACEMENT_3D('',#306295,#114948,#114949);
#98759=AXIS2_PLACEMENT_3D('',#306299,#114952,#114953);
#98760=AXIS2_PLACEMENT_3D('',#306302,#114955,#114956);
#98761=AXIS2_PLACEMENT_3D('',#306303,#114957,#114958);
#98762=AXIS2_PLACEMENT_3D('',#307974,#114962,#114963);
#98763=AXIS2_PLACEMENT_3D('',#307977,#114965,#114966);
#98764=AXIS2_PLACEMENT_3D('',#309638,#114968,#114969);
#98765=AXIS2_PLACEMENT_3D('',#309642,#114972,#114973);
#98766=AXIS2_PLACEMENT_3D('',#309645,#114975,#114976);
#98767=AXIS2_PLACEMENT_3D('',#309646,#114977,#114978);
#98768=AXIS2_PLACEMENT_3D('',#311314,#114982,#114983);
#98769=AXIS2_PLACEMENT_3D('',#311317,#114985,#114986);
#98770=AXIS2_PLACEMENT_3D('',#312978,#114988,#114989);
#98771=AXIS2_PLACEMENT_3D('',#312982,#114992,#114993);
#98772=AXIS2_PLACEMENT_3D('',#312985,#114995,#114996);
#98773=AXIS2_PLACEMENT_3D('',#312986,#114997,#114998);
#98774=AXIS2_PLACEMENT_3D('',#314661,#115002,#115003);
#98775=AXIS2_PLACEMENT_3D('',#314664,#115005,#115006);
#98776=AXIS2_PLACEMENT_3D('',#316325,#115008,#115009);
#98777=AXIS2_PLACEMENT_3D('',#316329,#115012,#115013);
#98778=AXIS2_PLACEMENT_3D('',#316332,#115015,#115016);
#98779=AXIS2_PLACEMENT_3D('',#316333,#115017,#115018);
#98780=AXIS2_PLACEMENT_3D('',#318008,#115022,#115023);
#98781=AXIS2_PLACEMENT_3D('',#318011,#115025,#115026);
#98782=AXIS2_PLACEMENT_3D('',#319672,#115028,#115029);
#98783=AXIS2_PLACEMENT_3D('',#319676,#115032,#115033);
#98784=AXIS2_PLACEMENT_3D('',#319679,#115035,#115036);
#98785=AXIS2_PLACEMENT_3D('',#319680,#115037,#115038);
#98786=AXIS2_PLACEMENT_3D('',#321355,#115042,#115043);
#98787=AXIS2_PLACEMENT_3D('',#321358,#115045,#115046);
#98788=AXIS2_PLACEMENT_3D('',#323019,#115048,#115049);
#98789=AXIS2_PLACEMENT_3D('',#323023,#115052,#115053);
#98790=AXIS2_PLACEMENT_3D('',#323026,#115055,#115056);
#98791=AXIS2_PLACEMENT_3D('',#323027,#115057,#115058);
#98792=AXIS2_PLACEMENT_3D('',#324702,#115062,#115063);
#98793=AXIS2_PLACEMENT_3D('',#324705,#115065,#115066);
#98794=AXIS2_PLACEMENT_3D('',#326366,#115068,#115069);
#98795=AXIS2_PLACEMENT_3D('',#326370,#115072,#115073);
#98796=AXIS2_PLACEMENT_3D('',#326373,#115075,#115076);
#98797=AXIS2_PLACEMENT_3D('',#326374,#115077,#115078);
#98798=AXIS2_PLACEMENT_3D('',#328045,#115082,#115083);
#98799=AXIS2_PLACEMENT_3D('',#328048,#115085,#115086);
#98800=AXIS2_PLACEMENT_3D('',#329709,#115088,#115089);
#98801=AXIS2_PLACEMENT_3D('',#329713,#115092,#115093);
#98802=AXIS2_PLACEMENT_3D('',#329715,#115094,#115095);
#98803=AXIS2_PLACEMENT_3D('',#329736,#115097,#115098);
#98804=AXIS2_PLACEMENT_3D('',#329749,#115100,#115101);
#98805=AXIS2_PLACEMENT_3D('',#329770,#115103,#115104);
#98806=AXIS2_PLACEMENT_3D('',#329783,#115106,#115107);
#98807=AXIS2_PLACEMENT_3D('',#329804,#115109,#115110);
#98808=AXIS2_PLACEMENT_3D('',#329817,#115112,#115113);
#98809=AXIS2_PLACEMENT_3D('',#329834,#115115,#115116);
#98810=AXIS2_PLACEMENT_3D('',#329847,#115118,#115119);
#98811=AXIS2_PLACEMENT_3D('',#329868,#115121,#115122);
#98812=AXIS2_PLACEMENT_3D('',#329881,#115124,#115125);
#98813=AXIS2_PLACEMENT_3D('',#329902,#115127,#115128);
#98814=AXIS2_PLACEMENT_3D('',#329915,#115130,#115131);
#98815=AXIS2_PLACEMENT_3D('',#329936,#115133,#115134);
#98816=AXIS2_PLACEMENT_3D('',#329949,#115136,#115137);
#98817=AXIS2_PLACEMENT_3D('',#329968,#115139,#115140);
#98818=AXIS2_PLACEMENT_3D('',#329981,#115142,#115143);
#98819=AXIS2_PLACEMENT_3D('',#329994,#115145,#115146);
#98820=AXIS2_PLACEMENT_3D('',#331650,#115149,#115150);
#98821=AXIS2_PLACEMENT_3D('',#331652,#115152,#115153);
#98822=AXIS2_PLACEMENT_3D('',#333305,#115156,#115157);
#98823=AXIS2_PLACEMENT_3D('',#334961,#115160,#115161);
#98824=AXIS2_PLACEMENT_3D('',#334963,#115163,#115164);
#98825=AXIS2_PLACEMENT_3D('',#334965,#115166,#115167);
#98826=AXIS2_PLACEMENT_3D('',#334968,#115170,#115171);
#98827=AXIS2_PLACEMENT_3D('',#336621,#115174,#115175);
#98828=AXIS2_PLACEMENT_3D('',#338276,#115177,#115178);
#98829=AXIS2_PLACEMENT_3D('',#338279,#115181,#115182);
#98830=AXIS2_PLACEMENT_3D('',#339933,#115186,#115187);
#98831=AXIS2_PLACEMENT_3D('',#341588,#115189,#115190);
#98832=AXIS2_PLACEMENT_3D('',#341590,#115192,#115193);
#98833=AXIS2_PLACEMENT_3D('',#343243,#115196,#115197);
#98834=AXIS2_PLACEMENT_3D('',#344899,#115200,#115201);
#98835=AXIS2_PLACEMENT_3D('',#344901,#115203,#115204);
#98836=AXIS2_PLACEMENT_3D('',#344902,#115205,#115206);
#98837=AXIS2_PLACEMENT_3D('',#344904,#115208,#115209);
#98838=AXIS2_PLACEMENT_3D('',#344907,#115212,#115213);
#98839=AXIS2_PLACEMENT_3D('',#346560,#115216,#115217);
#98840=AXIS2_PLACEMENT_3D('',#348215,#115219,#115220);
#98841=AXIS2_PLACEMENT_3D('',#348218,#115223,#115224);
#98842=AXIS2_PLACEMENT_3D('',#349872,#115228,#115229);
#98843=AXIS2_PLACEMENT_3D('',#351527,#115231,#115232);
#98844=AXIS2_PLACEMENT_3D('',#351529,#115234,#115235);
#98845=AXIS2_PLACEMENT_3D('',#353182,#115238,#115239);
#98846=AXIS2_PLACEMENT_3D('',#354838,#115242,#115243);
#98847=AXIS2_PLACEMENT_3D('',#354840,#115245,#115246);
#98848=AXIS2_PLACEMENT_3D('',#354841,#115247,#115248);
#98849=AXIS2_PLACEMENT_3D('',#354843,#115250,#115251);
#98850=AXIS2_PLACEMENT_3D('',#354846,#115254,#115255);
#98851=AXIS2_PLACEMENT_3D('',#356499,#115258,#115259);
#98852=AXIS2_PLACEMENT_3D('',#358154,#115261,#115262);
#98853=AXIS2_PLACEMENT_3D('',#358155,#115263,#115264);
#98854=AXIS2_PLACEMENT_3D('',#358158,#115266,#115267);
#98855=AXIS2_PLACEMENT_3D('',#358159,#115268,#115269);
#114071=DIRECTION('axis',(0.,0.,1.));
#114072=DIRECTION('refdir',(1.,0.,0.));
#114073=DIRECTION('center_axis',(5.13675726285535E-34,-1.,-1.22464674570954E-16));
#114074=DIRECTION('ref_axis',(0.0618200639786049,1.22230437692711E-16,-0.998087310654575));
#114075=DIRECTION('center_axis',(5.13675726285535E-34,-1.,-1.22464674570954E-16));
#114076=DIRECTION('ref_axis',(-0.93969262091562,4.18853855054451E-17,-0.342020142969288));
#114077=DIRECTION('',(5.13675726285535E-34,-1.,-1.22464674570954E-16));
#114078=DIRECTION('center_axis',(5.13675726285535E-34,-1.,-1.22464674570954E-16));
#114079=DIRECTION('ref_axis',(-0.93969262091562,4.18853855054451E-17,-0.342020142969288));
#114080=DIRECTION('',(5.13675726285535E-34,-1.,-1.22464674570954E-16));
#114081=DIRECTION('',(5.13675726285535E-34,-1.,-1.22464674570954E-16));
#114082=DIRECTION('',(-5.13675726285535E-34,1.,1.22464674570954E-16));
#114083=DIRECTION('center_axis',(5.13675726285535E-34,-1.,-1.22464674570954E-16));
#114084=DIRECTION('ref_axis',(0.0784590959774507,1.22087156847365E-16,-0.996917333713484));
#114085=DIRECTION('',(5.13675726285535E-34,-1.,-1.22464674570954E-16));
#114086=DIRECTION('center_axis',(5.13675726285535E-34,-1.,-1.22464674570954E-16));
#114087=DIRECTION('ref_axis',(-0.93969262091562,4.18853855054451E-17,-0.342020142969288));
#114088=DIRECTION('center_axis',(5.13675726285535E-34,-1.,-1.22464674570954E-16));
#114089=DIRECTION('ref_axis',(-0.93969262091562,4.18853855054451E-17,-0.342020142969288));
#114090=DIRECTION('center_axis',(5.13675726285535E-34,-1.,-1.22464674570954E-16));
#114091=DIRECTION('ref_axis',(0.203233458912656,1.1990887460271E-16,-0.979130308579199));
#114092=DIRECTION('center_axis',(5.13675726285535E-34,-1.,-1.22464674570954E-16));
#114093=DIRECTION('ref_axis',(-0.93969262091562,4.18853855054451E-17,-0.342020142969288));
#114094=DIRECTION('',(5.13675726285535E-34,-1.,-1.22464674570954E-16));
#114095=DIRECTION('center_axis',(5.13675726285535E-34,-1.,-1.22464674570954E-16));
#114096=DIRECTION('ref_axis',(-0.93969262091562,4.18853855054451E-17,-0.342020142969288));
#114097=DIRECTION('',(5.13675726285535E-34,-1.,-1.22464674570954E-16));
#114098=DIRECTION('',(-5.13675726285535E-34,1.,1.22464674570954E-16));
#114099=DIRECTION('center_axis',(5.13675726285535E-34,-1.,-1.22464674570954E-16));
#114100=DIRECTION('ref_axis',(0.0784590959774507,1.22087156847365E-16,-0.996917333713484));
#114101=DIRECTION('',(5.13675726285535E-34,-1.,-1.22464674570954E-16));
#114102=DIRECTION('center_axis',(5.13675726285535E-34,-1.,-1.22464674570954E-16));
#114103=DIRECTION('ref_axis',(-0.93969262091562,4.18853855054451E-17,-0.342020142969288));
#114104=DIRECTION('center_axis',(5.13675726285535E-34,-1.,-1.22464674570954E-16));
#114105=DIRECTION('ref_axis',(-0.93969262091562,4.18853855054451E-17,-0.342020142969288));
#114106=DIRECTION('center_axis',(5.13675726285535E-34,-1.,-1.22464674570954E-16));
#114107=DIRECTION('ref_axis',(0.340509606979888,1.1514631260766E-16,-0.940241036944465));
#114108=DIRECTION('center_axis',(5.13675726285535E-34,-1.,-1.22464674570954E-16));
#114109=DIRECTION('ref_axis',(-0.93969262091562,4.18853855054451E-17,-0.342020142969288));
#114110=DIRECTION('',(5.13675726285535E-34,-1.,-1.22464674570954E-16));
#114111=DIRECTION('center_axis',(5.13675726285535E-34,-1.,-1.22464674570954E-16));
#114112=DIRECTION('ref_axis',(-0.93969262091562,4.18853855054451E-17,-0.342020142969288));
#114113=DIRECTION('',(5.13675726285535E-34,-1.,-1.22464674570954E-16));
#114114=DIRECTION('',(-5.13675726285535E-34,1.,1.22464674570954E-16));
#114115=DIRECTION('center_axis',(5.13675726285535E-34,-1.,-1.22464674570954E-16));
#114116=DIRECTION('ref_axis',(0.0784590959774507,1.22087156847365E-16,-0.996917333713484));
#114117=DIRECTION('',(5.13675726285535E-34,-1.,-1.22464674570954E-16));
#114118=DIRECTION('center_axis',(5.13675726285535E-34,-1.,-1.22464674570954E-16));
#114119=DIRECTION('ref_axis',(-0.93969262091562,4.18853855054451E-17,-0.342020142969288));
#114120=DIRECTION('center_axis',(5.13675726285535E-34,-1.,-1.22464674570954E-16));
#114121=DIRECTION('ref_axis',(-0.93969262091562,4.18853855054451E-17,-0.342020142969288));
#114122=DIRECTION('center_axis',(5.13675726285535E-34,-1.,-1.22464674570954E-16));
#114123=DIRECTION('ref_axis',(0.470853961165332,1.08039703752382E-16,-0.882211169309773));
#114124=DIRECTION('center_axis',(5.13675726285535E-34,-1.,-1.22464674570954E-16));
#114125=DIRECTION('ref_axis',(-0.93969262091562,4.18853855054451E-17,-0.342020142969288));
#114126=DIRECTION('',(5.13675726285535E-34,-1.,-1.22464674570954E-16));
#114127=DIRECTION('center_axis',(5.13675726285535E-34,-1.,-1.22464674570954E-16));
#114128=DIRECTION('ref_axis',(-0.93969262091562,4.18853855054451E-17,-0.342020142969288));
#114129=DIRECTION('',(5.13675726285535E-34,-1.,-1.22464674570954E-16));
#114130=DIRECTION('',(-5.13675726285535E-34,1.,1.22464674570954E-16));
#114131=DIRECTION('center_axis',(5.13675726285535E-34,-1.,-1.22464674570954E-16));
#114132=DIRECTION('ref_axis',(0.0784590959774507,1.22087156847365E-16,-0.996917333713484));
#114133=DIRECTION('',(5.13675726285535E-34,-1.,-1.22464674570954E-16));
#114134=DIRECTION('center_axis',(5.13675726285535E-34,-1.,-1.22464674570954E-16));
#114135=DIRECTION('ref_axis',(-0.93969262091562,4.18853855054451E-17,-0.342020142969288));
#114136=DIRECTION('center_axis',(5.13675726285535E-34,-1.,-1.22464674570954E-16));
#114137=DIRECTION('ref_axis',(-0.93969262091562,4.18853855054451E-17,-0.342020142969288));
#114138=DIRECTION('center_axis',(5.13675726285535E-34,-1.,-1.22464674570954E-16));
#114139=DIRECTION('ref_axis',(0.591613087024489,9.87337180501123E-17,-0.806222026033372));
#114140=DIRECTION('center_axis',(5.13675726285535E-34,-1.,-1.22464674570954E-16));
#114141=DIRECTION('ref_axis',(-0.93969262091562,4.18853855054451E-17,-0.342020142969288));
#114142=DIRECTION('',(5.13675726285535E-34,-1.,-1.22464674570954E-16));
#114143=DIRECTION('center_axis',(5.13675726285535E-34,-1.,-1.22464674570954E-16));
#114144=DIRECTION('ref_axis',(-0.93969262091562,4.18853855054451E-17,-0.342020142969288));
#114145=DIRECTION('',(5.13675726285535E-34,-1.,-1.22464674570954E-16));
#114146=DIRECTION('',(-5.13675726285535E-34,1.,1.22464674570954E-16));
#114147=DIRECTION('center_axis',(5.13675726285535E-34,-1.,-1.22464674570954E-16));
#114148=DIRECTION('ref_axis',(0.0784590959774507,1.22087156847365E-16,-0.996917333713484));
#114149=DIRECTION('',(5.13675726285535E-34,-1.,-1.22464674570954E-16));
#114150=DIRECTION('center_axis',(5.13675726285535E-34,-1.,-1.22464674570954E-16));
#114151=DIRECTION('ref_axis',(-0.93969262091562,4.18853855054451E-17,-0.342020142969288));
#114152=DIRECTION('center_axis',(5.13675726285535E-34,-1.,-1.22464674570954E-16));
#114153=DIRECTION('ref_axis',(-0.93969262091562,4.18853855054451E-17,-0.342020142969288));
#114154=DIRECTION('center_axis',(5.13675726285535E-34,-1.,-1.22464674570954E-16));
#114155=DIRECTION('ref_axis',(0.700328675782159,8.74177986363949E-17,-0.713820527777962));
#114156=DIRECTION('center_axis',(5.13675726285535E-34,-1.,-1.22464674570954E-16));
#114157=DIRECTION('ref_axis',(-0.93969262091562,4.18853855054451E-17,-0.342020142969288));
#114158=DIRECTION('',(5.13675726285535E-34,-1.,-1.22464674570954E-16));
#114159=DIRECTION('center_axis',(5.13675726285535E-34,-1.,-1.22464674570954E-16));
#114160=DIRECTION('ref_axis',(-0.93969262091562,4.18853855054451E-17,-0.342020142969288));
#114161=DIRECTION('',(5.13675726285535E-34,-1.,-1.22464674570954E-16));
#114162=DIRECTION('',(-5.13675726285535E-34,1.,1.22464674570954E-16));
#114163=DIRECTION('center_axis',(5.13675726285535E-34,-1.,-1.22464674570954E-16));
#114164=DIRECTION('ref_axis',(0.0784590959774507,1.22087156847365E-16,-0.996917333713484));
#114165=DIRECTION('',(5.13675726285535E-34,-1.,-1.22464674570954E-16));
#114166=DIRECTION('center_axis',(5.13675726285535E-34,-1.,-1.22464674570954E-16));
#114167=DIRECTION('ref_axis',(-0.93969262091562,4.18853855054451E-17,-0.342020142969288));
#114168=DIRECTION('center_axis',(5.13675726285535E-34,-1.,-1.22464674570954E-16));
#114169=DIRECTION('ref_axis',(-0.93969262091562,4.18853855054451E-17,-0.342020142969288));
#114170=DIRECTION('center_axis',(5.13675726285535E-34,-1.,-1.22464674570954E-16));
#114171=DIRECTION('ref_axis',(0.794787592671922,7.4322304895865E-17,-0.606887701749485));
#114172=DIRECTION('center_axis',(5.13675726285535E-34,-1.,-1.22464674570954E-16));
#114173=DIRECTION('ref_axis',(-0.93969262091562,4.18853855054451E-17,-0.342020142969288));
#114174=DIRECTION('',(5.13675726285535E-34,-1.,-1.22464674570954E-16));
#114175=DIRECTION('center_axis',(5.13675726285535E-34,-1.,-1.22464674570954E-16));
#114176=DIRECTION('ref_axis',(-0.93969262091562,4.18853855054451E-17,-0.342020142969288));
#114177=DIRECTION('',(5.13675726285535E-34,-1.,-1.22464674570954E-16));
#114178=DIRECTION('',(-5.13675726285535E-34,1.,1.22464674570954E-16));
#114179=DIRECTION('center_axis',(5.13675726285535E-34,-1.,-1.22464674570954E-16));
#114180=DIRECTION('ref_axis',(0.0784590959774507,1.22087156847365E-16,-0.996917333713484));
#114181=DIRECTION('',(5.13675726285535E-34,-1.,-1.22464674570954E-16));
#114182=DIRECTION('center_axis',(5.13675726285535E-34,-1.,-1.22464674570954E-16));
#114183=DIRECTION('ref_axis',(-0.93969262091562,4.18853855054451E-17,-0.342020142969288));
#114184=DIRECTION('center_axis',(5.13675726285535E-34,-1.,-1.22464674570954E-16));
#114185=DIRECTION('ref_axis',(-0.93969262091562,4.18853855054451E-17,-0.342020142969288));
#114186=DIRECTION('center_axis',(5.13675726285535E-34,-1.,-1.22464674570954E-16));
#114187=DIRECTION('ref_axis',(0.87306692619485,5.97138233402766E-17,-0.487600392108822));
#114188=DIRECTION('center_axis',(5.13675726285535E-34,-1.,-1.22464674570954E-16));
#114189=DIRECTION('ref_axis',(-0.93969262091562,4.18853855054451E-17,-0.342020142969288));
#114190=DIRECTION('',(5.13675726285535E-34,-1.,-1.22464674570954E-16));
#114191=DIRECTION('center_axis',(5.13675726285535E-34,-1.,-1.22464674570954E-16));
#114192=DIRECTION('ref_axis',(-0.93969262091562,4.18853855054451E-17,-0.342020142969288));
#114193=DIRECTION('',(5.13675726285535E-34,-1.,-1.22464674570954E-16));
#114194=DIRECTION('',(-5.13675726285535E-34,1.,1.22464674570954E-16));
#114195=DIRECTION('center_axis',(5.13675726285535E-34,-1.,-1.22464674570954E-16));
#114196=DIRECTION('ref_axis',(0.0784590959774507,1.22087156847365E-16,-0.996917333713484));
#114197=DIRECTION('',(5.13675726285535E-34,-1.,-1.22464674570954E-16));
#114198=DIRECTION('center_axis',(5.13675726285535E-34,-1.,-1.22464674570954E-16));
#114199=DIRECTION('ref_axis',(-0.93969262091562,4.18853855054451E-17,-0.342020142969288));
#114200=DIRECTION('center_axis',(5.13675726285535E-34,-1.,-1.22464674570954E-16));
#114201=DIRECTION('ref_axis',(-0.93969262091562,4.18853855054451E-17,-0.342020142969288));
#114202=DIRECTION('center_axis',(5.13675726285535E-34,-1.,-1.22464674570954E-16));
#114203=DIRECTION('ref_axis',(0.933573134654503,4.38897405736607E-17,-0.358386944867368));
#114204=DIRECTION('center_axis',(5.13675726285535E-34,-1.,-1.22464674570954E-16));
#114205=DIRECTION('ref_axis',(-0.93969262091562,4.18853855054451E-17,-0.342020142969288));
#114206=DIRECTION('',(5.13675726285535E-34,-1.,-1.22464674570954E-16));
#114207=DIRECTION('center_axis',(5.13675726285535E-34,-1.,-1.22464674570954E-16));
#114208=DIRECTION('ref_axis',(-0.93969262091562,4.18853855054451E-17,-0.342020142969288));
#114209=DIRECTION('',(5.13675726285535E-34,-1.,-1.22464674570954E-16));
#114210=DIRECTION('',(-5.13675726285535E-34,1.,1.22464674570954E-16));
#114211=DIRECTION('center_axis',(5.13675726285535E-34,-1.,-1.22464674570954E-16));
#114212=DIRECTION('ref_axis',(0.0784590959774507,1.22087156847365E-16,-0.996917333713484));
#114213=DIRECTION('',(5.13675726285535E-34,-1.,-1.22464674570954E-16));
#114214=DIRECTION('center_axis',(5.13675726285535E-34,-1.,-1.22464674570954E-16));
#114215=DIRECTION('ref_axis',(-0.93969262091562,4.18853855054451E-17,-0.342020142969288));
#114216=DIRECTION('center_axis',(5.13675726285535E-34,-1.,-1.22464674570954E-16));
#114217=DIRECTION('ref_axis',(-0.93969262091562,4.18853855054451E-17,-0.342020142969288));
#114218=DIRECTION('center_axis',(5.13675726285535E-34,-1.,-1.22464674570954E-16));
#114219=DIRECTION('ref_axis',(0.975074486292716,2.71721892731301E-17,-0.221877773066607));
#114220=DIRECTION('center_axis',(5.13675726285535E-34,-1.,-1.22464674570954E-16));
#114221=DIRECTION('ref_axis',(-0.93969262091562,4.18853855054451E-17,-0.342020142969288));
#114222=DIRECTION('',(5.13675726285535E-34,-1.,-1.22464674570954E-16));
#114223=DIRECTION('center_axis',(5.13675726285535E-34,-1.,-1.22464674570954E-16));
#114224=DIRECTION('ref_axis',(-0.93969262091562,4.18853855054451E-17,-0.342020142969288));
#114225=DIRECTION('',(5.13675726285535E-34,-1.,-1.22464674570954E-16));
#114226=DIRECTION('',(-5.13675726285535E-34,1.,1.22464674570954E-16));
#114227=DIRECTION('center_axis',(5.13675726285535E-34,-1.,-1.22464674570954E-16));
#114228=DIRECTION('ref_axis',(0.0784590959774507,1.22087156847365E-16,-0.996917333713484));
#114229=DIRECTION('',(5.13675726285535E-34,-1.,-1.22464674570954E-16));
#114230=DIRECTION('center_axis',(5.13675726285535E-34,-1.,-1.22464674570954E-16));
#114231=DIRECTION('ref_axis',(-0.93969262091562,4.18853855054451E-17,-0.342020142969288));
#114232=DIRECTION('center_axis',(5.13675726285535E-34,-1.,-1.22464674570954E-16));
#114233=DIRECTION('ref_axis',(-0.93969262091562,4.18853855054451E-17,-0.342020142969288));
#114234=DIRECTION('center_axis',(5.13675726285535E-34,-1.,-1.22464674570954E-16));
#114235=DIRECTION('ref_axis',(0.996726133306289,9.9014906031653E-18,-0.0808518100248454));
#114236=DIRECTION('center_axis',(5.13675726285535E-34,-1.,-1.22464674570954E-16));
#114237=DIRECTION('ref_axis',(-0.93969262091562,4.18853855054451E-17,-0.342020142969288));
#114238=DIRECTION('',(5.13675726285535E-34,-1.,-1.22464674570954E-16));
#114239=DIRECTION('center_axis',(5.13675726285535E-34,-1.,-1.22464674570954E-16));
#114240=DIRECTION('ref_axis',(-0.93969262091562,4.18853855054451E-17,-0.342020142969288));
#114241=DIRECTION('',(5.13675726285535E-34,-1.,-1.22464674570954E-16));
#114242=DIRECTION('',(-5.13675726285535E-34,1.,1.22464674570954E-16));
#114243=DIRECTION('center_axis',(5.13675726285535E-34,-1.,-1.22464674570954E-16));
#114244=DIRECTION('ref_axis',(0.0784590959774507,1.22087156847365E-16,-0.996917333713484));
#114245=DIRECTION('',(5.13675726285535E-34,-1.,-1.22464674570954E-16));
#114246=DIRECTION('center_axis',(5.13675726285535E-34,-1.,-1.22464674570954E-16));
#114247=DIRECTION('ref_axis',(-0.93969262091562,4.18853855054451E-17,-0.342020142969288));
#114248=DIRECTION('center_axis',(5.13675726285535E-34,-1.,-1.22464674570954E-16));
#114249=DIRECTION('ref_axis',(-0.93969262091562,4.18853855054451E-17,-0.342020142969288));
#114250=DIRECTION('center_axis',(5.13675726285535E-34,-1.,-1.22464674570954E-16));
#114251=DIRECTION('ref_axis',(0.998087310654575,-7.57077401709542E-18,0.0618200639786049));
#114252=DIRECTION('center_axis',(5.13675726285535E-34,-1.,-1.22464674570954E-16));
#114253=DIRECTION('ref_axis',(-0.93969262091562,4.18853855054451E-17,-0.342020142969288));
#114254=DIRECTION('',(5.13675726285535E-34,-1.,-1.22464674570954E-16));
#114255=DIRECTION('center_axis',(5.13675726285535E-34,-1.,-1.22464674570954E-16));
#114256=DIRECTION('ref_axis',(-0.93969262091562,4.18853855054451E-17,-0.342020142969288));
#114257=DIRECTION('',(5.13675726285535E-34,-1.,-1.22464674570954E-16));
#114258=DIRECTION('',(-5.13675726285535E-34,1.,1.22464674570954E-16));
#114259=DIRECTION('center_axis',(5.13675726285535E-34,-1.,-1.22464674570954E-16));
#114260=DIRECTION('ref_axis',(0.0784590959774507,1.22087156847365E-16,-0.996917333713484));
#114261=DIRECTION('',(5.13675726285535E-34,-1.,-1.22464674570954E-16));
#114262=DIRECTION('center_axis',(5.13675726285535E-34,-1.,-1.22464674570954E-16));
#114263=DIRECTION('ref_axis',(-0.93969262091562,4.18853855054451E-17,-0.342020142969288));
#114264=DIRECTION('center_axis',(5.13675726285535E-34,-1.,-1.22464674570954E-16));
#114265=DIRECTION('ref_axis',(-0.93969262091562,4.18853855054451E-17,-0.342020142969288));
#114266=DIRECTION('center_axis',(5.13675726285535E-34,-1.,-1.22464674570954E-16));
#114267=DIRECTION('ref_axis',(0.979130308579199,-2.48889194076679E-17,0.203233458912656));
#114268=DIRECTION('center_axis',(5.13675726285535E-34,-1.,-1.22464674570954E-16));
#114269=DIRECTION('ref_axis',(-0.93969262091562,4.18853855054451E-17,-0.342020142969288));
#114270=DIRECTION('',(5.13675726285535E-34,-1.,-1.22464674570954E-16));
#114271=DIRECTION('center_axis',(5.13675726285535E-34,-1.,-1.22464674570954E-16));
#114272=DIRECTION('ref_axis',(-0.93969262091562,4.18853855054451E-17,-0.342020142969288));
#114273=DIRECTION('',(5.13675726285535E-34,-1.,-1.22464674570954E-16));
#114274=DIRECTION('',(-5.13675726285535E-34,1.,1.22464674570954E-16));
#114275=DIRECTION('center_axis',(5.13675726285535E-34,-1.,-1.22464674570954E-16));
#114276=DIRECTION('ref_axis',(0.0784590959774507,1.22087156847365E-16,-0.996917333713484));
#114277=DIRECTION('',(5.13675726285535E-34,-1.,-1.22464674570954E-16));
#114278=DIRECTION('center_axis',(5.13675726285535E-34,-1.,-1.22464674570954E-16));
#114279=DIRECTION('ref_axis',(-0.93969262091562,4.18853855054451E-17,-0.342020142969288));
#114280=DIRECTION('center_axis',(5.13675726285535E-34,-1.,-1.22464674570954E-16));
#114281=DIRECTION('ref_axis',(-0.93969262091562,4.18853855054451E-17,-0.342020142969288));
#114282=DIRECTION('center_axis',(5.13675726285535E-34,-1.,-1.22464674570954E-16));
#114283=DIRECTION('ref_axis',(0.940241036944465,-4.17003982070755E-17,0.340509606979888));
#114284=DIRECTION('center_axis',(5.13675726285535E-34,-1.,-1.22464674570954E-16));
#114285=DIRECTION('ref_axis',(-0.93969262091562,4.18853855054451E-17,-0.342020142969288));
#114286=DIRECTION('',(5.13675726285535E-34,-1.,-1.22464674570954E-16));
#114287=DIRECTION('center_axis',(5.13675726285535E-34,-1.,-1.22464674570954E-16));
#114288=DIRECTION('ref_axis',(-0.93969262091562,4.18853855054451E-17,-0.342020142969288));
#114289=DIRECTION('',(5.13675726285535E-34,-1.,-1.22464674570954E-16));
#114290=DIRECTION('',(-5.13675726285535E-34,1.,1.22464674570954E-16));
#114291=DIRECTION('center_axis',(5.13675726285535E-34,-1.,-1.22464674570954E-16));
#114292=DIRECTION('ref_axis',(0.0784590959774507,1.22087156847365E-16,-0.996917333713484));
#114293=DIRECTION('',(5.13675726285535E-34,-1.,-1.22464674570954E-16));
#114294=DIRECTION('center_axis',(5.13675726285535E-34,-1.,-1.22464674570954E-16));
#114295=DIRECTION('ref_axis',(-0.93969262091562,4.18853855054451E-17,-0.342020142969288));
#114296=DIRECTION('center_axis',(5.13675726285535E-34,-1.,-1.22464674570954E-16));
#114297=DIRECTION('ref_axis',(-0.93969262091562,4.18853855054451E-17,-0.342020142969288));
#114298=DIRECTION('center_axis',(5.13675726285535E-34,-1.,-1.22464674570954E-16));
#114299=DIRECTION('ref_axis',(0.882211169309773,-5.76629771245571E-17,0.470853961165332));
#114300=DIRECTION('center_axis',(5.13675726285535E-34,-1.,-1.22464674570954E-16));
#114301=DIRECTION('ref_axis',(-0.93969262091562,4.18853855054451E-17,-0.342020142969288));
#114302=DIRECTION('',(5.13675726285535E-34,-1.,-1.22464674570954E-16));
#114303=DIRECTION('center_axis',(5.13675726285535E-34,-1.,-1.22464674570954E-16));
#114304=DIRECTION('ref_axis',(-0.93969262091562,4.18853855054451E-17,-0.342020142969288));
#114305=DIRECTION('',(5.13675726285535E-34,-1.,-1.22464674570954E-16));
#114306=DIRECTION('',(-5.13675726285535E-34,1.,1.22464674570954E-16));
#114307=DIRECTION('center_axis',(5.13675726285535E-34,-1.,-1.22464674570954E-16));
#114308=DIRECTION('ref_axis',(0.0784590959774507,1.22087156847365E-16,-0.996917333713484));
#114309=DIRECTION('',(5.13675726285535E-34,-1.,-1.22464674570954E-16));
#114310=DIRECTION('center_axis',(5.13675726285535E-34,-1.,-1.22464674570954E-16));
#114311=DIRECTION('ref_axis',(-0.93969262091562,4.18853855054451E-17,-0.342020142969288));
#114312=DIRECTION('center_axis',(5.13675726285535E-34,-1.,-1.22464674570954E-16));
#114313=DIRECTION('ref_axis',(-0.93969262091562,4.18853855054451E-17,-0.342020142969288));
#114314=DIRECTION('center_axis',(5.13675726285535E-34,-1.,-1.22464674570954E-16));
#114315=DIRECTION('ref_axis',(0.806222026033372,-7.24517041743716E-17,0.591613087024489));
#114316=DIRECTION('center_axis',(5.13675726285535E-34,-1.,-1.22464674570954E-16));
#114317=DIRECTION('ref_axis',(-0.93969262091562,4.18853855054451E-17,-0.342020142969288));
#114318=DIRECTION('',(5.13675726285535E-34,-1.,-1.22464674570954E-16));
#114319=DIRECTION('center_axis',(5.13675726285535E-34,-1.,-1.22464674570954E-16));
#114320=DIRECTION('ref_axis',(-0.93969262091562,4.18853855054451E-17,-0.342020142969288));
#114321=DIRECTION('',(5.13675726285535E-34,-1.,-1.22464674570954E-16));
#114322=DIRECTION('',(-5.13675726285535E-34,1.,1.22464674570954E-16));
#114323=DIRECTION('center_axis',(5.13675726285535E-34,-1.,-1.22464674570954E-16));
#114324=DIRECTION('ref_axis',(0.0784590959774507,1.22087156847365E-16,-0.996917333713484));
#114325=DIRECTION('',(5.13675726285535E-34,-1.,-1.22464674570954E-16));
#114326=DIRECTION('center_axis',(5.13675726285535E-34,-1.,-1.22464674570954E-16));
#114327=DIRECTION('ref_axis',(-0.93969262091562,4.18853855054451E-17,-0.342020142969288));
#114328=DIRECTION('center_axis',(5.13675726285535E-34,-1.,-1.22464674570954E-16));
#114329=DIRECTION('ref_axis',(-0.93969262091562,4.18853855054451E-17,-0.342020142969288));
#114330=DIRECTION('center_axis',(5.13675726285535E-34,-1.,-1.22464674570954E-16));
#114331=DIRECTION('ref_axis',(0.713820527777962,-8.57655233723694E-17,0.700328675782159));
#114332=DIRECTION('center_axis',(5.13675726285535E-34,-1.,-1.22464674570954E-16));
#114333=DIRECTION('ref_axis',(-0.93969262091562,4.18853855054451E-17,-0.342020142969288));
#114334=DIRECTION('',(5.13675726285535E-34,-1.,-1.22464674570954E-16));
#114335=DIRECTION('center_axis',(5.13675726285535E-34,-1.,-1.22464674570954E-16));
#114336=DIRECTION('ref_axis',(-0.93969262091562,4.18853855054451E-17,-0.342020142969288));
#114337=DIRECTION('',(5.13675726285535E-34,-1.,-1.22464674570954E-16));
#114338=DIRECTION('',(-5.13675726285535E-34,1.,1.22464674570954E-16));
#114339=DIRECTION('center_axis',(5.13675726285535E-34,-1.,-1.22464674570954E-16));
#114340=DIRECTION('ref_axis',(0.0784590959774507,1.22087156847365E-16,-0.996917333713484));
#114341=DIRECTION('',(5.13675726285535E-34,-1.,-1.22464674570954E-16));
#114342=DIRECTION('center_axis',(5.13675726285535E-34,-1.,-1.22464674570954E-16));
#114343=DIRECTION('ref_axis',(-0.93969262091562,4.18853855054451E-17,-0.342020142969288));
#114344=DIRECTION('center_axis',(5.13675726285535E-34,-1.,-1.22464674570954E-16));
#114345=DIRECTION('ref_axis',(-0.93969262091562,4.18853855054451E-17,-0.342020142969288));
#114346=DIRECTION('center_axis',(5.13675726285535E-34,-1.,-1.22464674570954E-16));
#114347=DIRECTION('ref_axis',(0.606887701749485,-9.73334038895991E-17,0.794787592671922));
#114348=DIRECTION('center_axis',(5.13675726285535E-34,-1.,-1.22464674570954E-16));
#114349=DIRECTION('ref_axis',(-0.93969262091562,4.18853855054451E-17,-0.342020142969288));
#114350=DIRECTION('',(5.13675726285535E-34,-1.,-1.22464674570954E-16));
#114351=DIRECTION('center_axis',(5.13675726285535E-34,-1.,-1.22464674570954E-16));
#114352=DIRECTION('ref_axis',(-0.93969262091562,4.18853855054451E-17,-0.342020142969288));
#114353=DIRECTION('',(5.13675726285535E-34,-1.,-1.22464674570954E-16));
#114354=DIRECTION('',(-5.13675726285535E-34,1.,1.22464674570954E-16));
#114355=DIRECTION('center_axis',(5.13675726285535E-34,-1.,-1.22464674570954E-16));
#114356=DIRECTION('ref_axis',(0.0784590959774507,1.22087156847365E-16,-0.996917333713484));
#114357=DIRECTION('',(5.13675726285535E-34,-1.,-1.22464674570954E-16));
#114358=DIRECTION('center_axis',(5.13675726285535E-34,-1.,-1.22464674570954E-16));
#114359=DIRECTION('ref_axis',(-0.93969262091562,4.18853855054451E-17,-0.342020142969288));
#114360=DIRECTION('center_axis',(5.13675726285535E-34,-1.,-1.22464674570954E-16));
#114361=DIRECTION('ref_axis',(-0.93969262091562,4.18853855054451E-17,-0.342020142969288));
#114362=DIRECTION('center_axis',(5.13675726285535E-34,-1.,-1.22464674570954E-16));
#114363=DIRECTION('ref_axis',(0.487600392108822,-1.06919856995116E-16,0.87306692619485));
#114364=DIRECTION('center_axis',(5.13675726285535E-34,-1.,-1.22464674570954E-16));
#114365=DIRECTION('ref_axis',(-0.93969262091562,4.18853855054451E-17,-0.342020142969288));
#114366=DIRECTION('',(5.13675726285535E-34,-1.,-1.22464674570954E-16));
#114367=DIRECTION('center_axis',(5.13675726285535E-34,-1.,-1.22464674570954E-16));
#114368=DIRECTION('ref_axis',(-0.93969262091562,4.18853855054451E-17,-0.342020142969288));
#114369=DIRECTION('',(5.13675726285535E-34,-1.,-1.22464674570954E-16));
#114370=DIRECTION('',(-5.13675726285535E-34,1.,1.22464674570954E-16));
#114371=DIRECTION('center_axis',(5.13675726285535E-34,-1.,-1.22464674570954E-16));
#114372=DIRECTION('ref_axis',(0.0784590959774507,1.22087156847365E-16,-0.996917333713484));
#114373=DIRECTION('',(5.13675726285535E-34,-1.,-1.22464674570954E-16));
#114374=DIRECTION('center_axis',(5.13675726285535E-34,-1.,-1.22464674570954E-16));
#114375=DIRECTION('ref_axis',(-0.93969262091562,4.18853855054451E-17,-0.342020142969288));
#114376=DIRECTION('center_axis',(5.13675726285535E-34,-1.,-1.22464674570954E-16));
#114377=DIRECTION('ref_axis',(-0.93969262091562,4.18853855054451E-17,-0.342020142969288));
#114378=DIRECTION('center_axis',(5.13675726285535E-34,-1.,-1.22464674570954E-16));
#114379=DIRECTION('ref_axis',(0.358386944867368,-1.14329730123649E-16,0.933573134654503));
#114380=DIRECTION('center_axis',(5.13675726285535E-34,-1.,-1.22464674570954E-16));
#114381=DIRECTION('ref_axis',(-0.93969262091562,4.18853855054451E-17,-0.342020142969288));
#114382=DIRECTION('',(5.13675726285535E-34,-1.,-1.22464674570954E-16));
#114383=DIRECTION('center_axis',(5.13675726285535E-34,-1.,-1.22464674570954E-16));
#114384=DIRECTION('ref_axis',(-0.93969262091562,4.18853855054451E-17,-0.342020142969288));
#114385=DIRECTION('',(5.13675726285535E-34,-1.,-1.22464674570954E-16));
#114386=DIRECTION('',(-5.13675726285535E-34,1.,1.22464674570954E-16));
#114387=DIRECTION('center_axis',(5.13675726285535E-34,-1.,-1.22464674570954E-16));
#114388=DIRECTION('ref_axis',(0.0784590959774507,1.22087156847365E-16,-0.996917333713484));
#114389=DIRECTION('',(5.13675726285535E-34,-1.,-1.22464674570954E-16));
#114390=DIRECTION('center_axis',(5.13675726285535E-34,-1.,-1.22464674570954E-16));
#114391=DIRECTION('ref_axis',(-0.93969262091562,4.18853855054451E-17,-0.342020142969288));
#114392=DIRECTION('center_axis',(5.13675726285535E-34,-1.,-1.22464674570954E-16));
#114393=DIRECTION('ref_axis',(-0.93969262091562,4.18853855054451E-17,-0.342020142969288));
#114394=DIRECTION('center_axis',(5.13675726285535E-34,-1.,-1.22464674570954E-16));
#114395=DIRECTION('ref_axis',(0.221877773066607,-1.19412179646278E-16,0.975074486292716));
#114396=DIRECTION('center_axis',(5.13675726285535E-34,-1.,-1.22464674570954E-16));
#114397=DIRECTION('ref_axis',(-0.93969262091562,4.18853855054451E-17,-0.342020142969288));
#114398=DIRECTION('',(5.13675726285535E-34,-1.,-1.22464674570954E-16));
#114399=DIRECTION('center_axis',(5.13675726285535E-34,-1.,-1.22464674570954E-16));
#114400=DIRECTION('ref_axis',(-0.93969262091562,4.18853855054451E-17,-0.342020142969288));
#114401=DIRECTION('',(5.13675726285535E-34,-1.,-1.22464674570954E-16));
#114402=DIRECTION('',(-5.13675726285535E-34,1.,1.22464674570954E-16));
#114403=DIRECTION('center_axis',(5.13675726285535E-34,-1.,-1.22464674570954E-16));
#114404=DIRECTION('ref_axis',(0.0784590959774507,1.22087156847365E-16,-0.996917333713484));
#114405=DIRECTION('',(5.13675726285535E-34,-1.,-1.22464674570954E-16));
#114406=DIRECTION('center_axis',(5.13675726285535E-34,-1.,-1.22464674570954E-16));
#114407=DIRECTION('ref_axis',(-0.93969262091562,4.18853855054451E-17,-0.342020142969288));
#114408=DIRECTION('center_axis',(5.13675726285535E-34,-1.,-1.22464674570954E-16));
#114409=DIRECTION('ref_axis',(-0.93969262091562,4.18853855054451E-17,-0.342020142969288));
#114410=DIRECTION('center_axis',(5.13675726285535E-34,-1.,-1.22464674570954E-16));
#114411=DIRECTION('ref_axis',(0.0808518100248454,-1.2206374155172E-16,0.996726133306289));
#114412=DIRECTION('center_axis',(5.13675726285535E-34,-1.,-1.22464674570954E-16));
#114413=DIRECTION('ref_axis',(-0.93969262091562,4.18853855054451E-17,-0.342020142969288));
#114414=DIRECTION('',(5.13675726285535E-34,-1.,-1.22464674570954E-16));
#114415=DIRECTION('center_axis',(5.13675726285535E-34,-1.,-1.22464674570954E-16));
#114416=DIRECTION('ref_axis',(-0.93969262091562,4.18853855054451E-17,-0.342020142969288));
#114417=DIRECTION('',(5.13675726285535E-34,-1.,-1.22464674570954E-16));
#114418=DIRECTION('',(-5.13675726285535E-34,1.,1.22464674570954E-16));
#114419=DIRECTION('center_axis',(5.13675726285535E-34,-1.,-1.22464674570954E-16));
#114420=DIRECTION('ref_axis',(0.0784590959774507,1.22087156847365E-16,-0.996917333713484));
#114421=DIRECTION('',(5.13675726285535E-34,-1.,-1.22464674570954E-16));
#114422=DIRECTION('center_axis',(5.13675726285535E-34,-1.,-1.22464674570954E-16));
#114423=DIRECTION('ref_axis',(-0.93969262091562,4.18853855054451E-17,-0.342020142969288));
#114424=DIRECTION('center_axis',(5.13675726285535E-34,-1.,-1.22464674570954E-16));
#114425=DIRECTION('ref_axis',(-0.93969262091562,4.18853855054451E-17,-0.342020142969288));
#114426=DIRECTION('center_axis',(5.13675726285535E-34,-1.,-1.22464674570954E-16));
#114427=DIRECTION('ref_axis',(-0.0618200639786049,-1.22230437692711E-16,
0.998087310654575));
#114428=DIRECTION('center_axis',(5.13675726285535E-34,-1.,-1.22464674570954E-16));
#114429=DIRECTION('ref_axis',(-0.93969262091562,4.18853855054451E-17,-0.342020142969288));
#114430=DIRECTION('',(5.13675726285535E-34,-1.,-1.22464674570954E-16));
#114431=DIRECTION('center_axis',(5.13675726285535E-34,-1.,-1.22464674570954E-16));
#114432=DIRECTION('ref_axis',(-0.93969262091562,4.18853855054451E-17,-0.342020142969288));
#114433=DIRECTION('',(5.13675726285535E-34,-1.,-1.22464674570954E-16));
#114434=DIRECTION('',(-5.13675726285535E-34,1.,1.22464674570954E-16));
#114435=DIRECTION('center_axis',(5.13675726285535E-34,-1.,-1.22464674570954E-16));
#114436=DIRECTION('ref_axis',(0.0784590959774507,1.22087156847365E-16,-0.996917333713484));
#114437=DIRECTION('',(5.13675726285535E-34,-1.,-1.22464674570954E-16));
#114438=DIRECTION('center_axis',(5.13675726285535E-34,-1.,-1.22464674570954E-16));
#114439=DIRECTION('ref_axis',(-0.93969262091562,4.18853855054451E-17,-0.342020142969288));
#114440=DIRECTION('center_axis',(5.13675726285535E-34,-1.,-1.22464674570954E-16));
#114441=DIRECTION('ref_axis',(-0.93969262091562,4.18853855054451E-17,-0.342020142969288));
#114442=DIRECTION('center_axis',(5.13675726285535E-34,-1.,-1.22464674570954E-16));
#114443=DIRECTION('ref_axis',(-0.203233458912656,-1.1990887460271E-16,0.979130308579199));
#114444=DIRECTION('center_axis',(5.13675726285535E-34,-1.,-1.22464674570954E-16));
#114445=DIRECTION('ref_axis',(-0.93969262091562,4.18853855054451E-17,-0.342020142969288));
#114446=DIRECTION('',(5.13675726285535E-34,-1.,-1.22464674570954E-16));
#114447=DIRECTION('center_axis',(5.13675726285535E-34,-1.,-1.22464674570954E-16));
#114448=DIRECTION('ref_axis',(-0.93969262091562,4.18853855054451E-17,-0.342020142969288));
#114449=DIRECTION('',(5.13675726285535E-34,-1.,-1.22464674570954E-16));
#114450=DIRECTION('',(-5.13675726285535E-34,1.,1.22464674570954E-16));
#114451=DIRECTION('center_axis',(5.13675726285535E-34,-1.,-1.22464674570954E-16));
#114452=DIRECTION('ref_axis',(0.0784590959774507,1.22087156847365E-16,-0.996917333713484));
#114453=DIRECTION('',(5.13675726285535E-34,-1.,-1.22464674570954E-16));
#114454=DIRECTION('center_axis',(5.13675726285535E-34,-1.,-1.22464674570954E-16));
#114455=DIRECTION('ref_axis',(-0.93969262091562,4.18853855054451E-17,-0.342020142969288));
#114456=DIRECTION('center_axis',(5.13675726285535E-34,-1.,-1.22464674570954E-16));
#114457=DIRECTION('ref_axis',(-0.93969262091562,4.18853855054451E-17,-0.342020142969288));
#114458=DIRECTION('center_axis',(5.13675726285535E-34,-1.,-1.22464674570954E-16));
#114459=DIRECTION('ref_axis',(-0.340509606979888,-1.1514631260766E-16,0.940241036944465));
#114460=DIRECTION('center_axis',(5.13675726285535E-34,-1.,-1.22464674570954E-16));
#114461=DIRECTION('ref_axis',(-0.93969262091562,4.18853855054451E-17,-0.342020142969288));
#114462=DIRECTION('',(5.13675726285535E-34,-1.,-1.22464674570954E-16));
#114463=DIRECTION('center_axis',(5.13675726285535E-34,-1.,-1.22464674570954E-16));
#114464=DIRECTION('ref_axis',(-0.93969262091562,4.18853855054451E-17,-0.342020142969288));
#114465=DIRECTION('',(5.13675726285535E-34,-1.,-1.22464674570954E-16));
#114466=DIRECTION('',(-5.13675726285535E-34,1.,1.22464674570954E-16));
#114467=DIRECTION('center_axis',(5.13675726285535E-34,-1.,-1.22464674570954E-16));
#114468=DIRECTION('ref_axis',(0.0784590959774507,1.22087156847365E-16,-0.996917333713484));
#114469=DIRECTION('',(5.13675726285535E-34,-1.,-1.22464674570954E-16));
#114470=DIRECTION('center_axis',(5.13675726285535E-34,-1.,-1.22464674570954E-16));
#114471=DIRECTION('ref_axis',(-0.93969262091562,4.18853855054451E-17,-0.342020142969288));
#114472=DIRECTION('center_axis',(5.13675726285535E-34,-1.,-1.22464674570954E-16));
#114473=DIRECTION('ref_axis',(-0.93969262091562,4.18853855054451E-17,-0.342020142969288));
#114474=DIRECTION('center_axis',(5.13675726285535E-34,-1.,-1.22464674570954E-16));
#114475=DIRECTION('ref_axis',(-0.470853961165332,-1.08039703752382E-16,
0.882211169309773));
#114476=DIRECTION('center_axis',(5.13675726285535E-34,-1.,-1.22464674570954E-16));
#114477=DIRECTION('ref_axis',(-0.93969262091562,4.18853855054451E-17,-0.342020142969288));
#114478=DIRECTION('',(5.13675726285535E-34,-1.,-1.22464674570954E-16));
#114479=DIRECTION('center_axis',(5.13675726285535E-34,-1.,-1.22464674570954E-16));
#114480=DIRECTION('ref_axis',(-0.93969262091562,4.18853855054451E-17,-0.342020142969288));
#114481=DIRECTION('',(5.13675726285535E-34,-1.,-1.22464674570954E-16));
#114482=DIRECTION('',(-5.13675726285535E-34,1.,1.22464674570954E-16));
#114483=DIRECTION('center_axis',(5.13675726285535E-34,-1.,-1.22464674570954E-16));
#114484=DIRECTION('ref_axis',(0.0784590959774507,1.22087156847365E-16,-0.996917333713484));
#114485=DIRECTION('',(5.13675726285535E-34,-1.,-1.22464674570954E-16));
#114486=DIRECTION('center_axis',(5.13675726285535E-34,-1.,-1.22464674570954E-16));
#114487=DIRECTION('ref_axis',(-0.93969262091562,4.18853855054451E-17,-0.342020142969288));
#114488=DIRECTION('center_axis',(5.13675726285535E-34,-1.,-1.22464674570954E-16));
#114489=DIRECTION('ref_axis',(-0.93969262091562,4.18853855054451E-17,-0.342020142969288));
#114490=DIRECTION('center_axis',(5.13675726285535E-34,-1.,-1.22464674570954E-16));
#114491=DIRECTION('ref_axis',(-0.591613087024489,-9.87337180501123E-17,
0.806222026033372));
#114492=DIRECTION('center_axis',(5.13675726285535E-34,-1.,-1.22464674570954E-16));
#114493=DIRECTION('ref_axis',(-0.93969262091562,4.18853855054451E-17,-0.342020142969288));
#114494=DIRECTION('',(5.13675726285535E-34,-1.,-1.22464674570954E-16));
#114495=DIRECTION('center_axis',(5.13675726285535E-34,-1.,-1.22464674570954E-16));
#114496=DIRECTION('ref_axis',(-0.93969262091562,4.18853855054451E-17,-0.342020142969288));
#114497=DIRECTION('',(5.13675726285535E-34,-1.,-1.22464674570954E-16));
#114498=DIRECTION('',(-5.13675726285535E-34,1.,1.22464674570954E-16));
#114499=DIRECTION('center_axis',(5.13675726285535E-34,-1.,-1.22464674570954E-16));
#114500=DIRECTION('ref_axis',(0.0784590959774507,1.22087156847365E-16,-0.996917333713484));
#114501=DIRECTION('',(5.13675726285535E-34,-1.,-1.22464674570954E-16));
#114502=DIRECTION('center_axis',(5.13675726285535E-34,-1.,-1.22464674570954E-16));
#114503=DIRECTION('ref_axis',(-0.93969262091562,4.18853855054451E-17,-0.342020142969288));
#114504=DIRECTION('center_axis',(5.13675726285535E-34,-1.,-1.22464674570954E-16));
#114505=DIRECTION('ref_axis',(-0.93969262091562,4.18853855054451E-17,-0.342020142969288));
#114506=DIRECTION('center_axis',(5.13675726285535E-34,-1.,-1.22464674570954E-16));
#114507=DIRECTION('ref_axis',(-0.700328675782159,-8.74177986363949E-17,
0.713820527777962));
#114508=DIRECTION('center_axis',(5.13675726285535E-34,-1.,-1.22464674570954E-16));
#114509=DIRECTION('ref_axis',(-0.93969262091562,4.18853855054451E-17,-0.342020142969288));
#114510=DIRECTION('',(5.13675726285535E-34,-1.,-1.22464674570954E-16));
#114511=DIRECTION('center_axis',(5.13675726285535E-34,-1.,-1.22464674570954E-16));
#114512=DIRECTION('ref_axis',(-0.93969262091562,4.18853855054451E-17,-0.342020142969288));
#114513=DIRECTION('',(5.13675726285535E-34,-1.,-1.22464674570954E-16));
#114514=DIRECTION('',(-5.13675726285535E-34,1.,1.22464674570954E-16));
#114515=DIRECTION('center_axis',(5.13675726285535E-34,-1.,-1.22464674570954E-16));
#114516=DIRECTION('ref_axis',(0.0784590959774507,1.22087156847365E-16,-0.996917333713484));
#114517=DIRECTION('',(5.13675726285535E-34,-1.,-1.22464674570954E-16));
#114518=DIRECTION('center_axis',(5.13675726285535E-34,-1.,-1.22464674570954E-16));
#114519=DIRECTION('ref_axis',(-0.93969262091562,4.18853855054451E-17,-0.342020142969288));
#114520=DIRECTION('center_axis',(5.13675726285535E-34,-1.,-1.22464674570954E-16));
#114521=DIRECTION('ref_axis',(-0.93969262091562,4.18853855054451E-17,-0.342020142969288));
#114522=DIRECTION('center_axis',(5.13675726285535E-34,-1.,-1.22464674570954E-16));
#114523=DIRECTION('ref_axis',(-0.794787592671922,-7.4322304895865E-17,0.606887701749485));
#114524=DIRECTION('center_axis',(5.13675726285535E-34,-1.,-1.22464674570954E-16));
#114525=DIRECTION('ref_axis',(-0.93969262091562,4.18853855054451E-17,-0.342020142969288));
#114526=DIRECTION('',(5.13675726285535E-34,-1.,-1.22464674570954E-16));
#114527=DIRECTION('center_axis',(5.13675726285535E-34,-1.,-1.22464674570954E-16));
#114528=DIRECTION('ref_axis',(-0.93969262091562,4.18853855054451E-17,-0.342020142969288));
#114529=DIRECTION('',(5.13675726285535E-34,-1.,-1.22464674570954E-16));
#114530=DIRECTION('',(-5.13675726285535E-34,1.,1.22464674570954E-16));
#114531=DIRECTION('center_axis',(5.13675726285535E-34,-1.,-1.22464674570954E-16));
#114532=DIRECTION('ref_axis',(0.0784590959774507,1.22087156847365E-16,-0.996917333713484));
#114533=DIRECTION('',(5.13675726285535E-34,-1.,-1.22464674570954E-16));
#114534=DIRECTION('center_axis',(5.13675726285535E-34,-1.,-1.22464674570954E-16));
#114535=DIRECTION('ref_axis',(-0.93969262091562,4.18853855054451E-17,-0.342020142969288));
#114536=DIRECTION('center_axis',(5.13675726285535E-34,-1.,-1.22464674570954E-16));
#114537=DIRECTION('ref_axis',(-0.93969262091562,4.18853855054451E-17,-0.342020142969288));
#114538=DIRECTION('center_axis',(5.13675726285535E-34,-1.,-1.22464674570954E-16));
#114539=DIRECTION('ref_axis',(-0.87306692619485,-5.97138233402766E-17,0.487600392108822));
#114540=DIRECTION('center_axis',(5.13675726285535E-34,-1.,-1.22464674570954E-16));
#114541=DIRECTION('ref_axis',(-0.93969262091562,4.18853855054451E-17,-0.342020142969288));
#114542=DIRECTION('',(5.13675726285535E-34,-1.,-1.22464674570954E-16));
#114543=DIRECTION('center_axis',(5.13675726285535E-34,-1.,-1.22464674570954E-16));
#114544=DIRECTION('ref_axis',(-0.93969262091562,4.18853855054451E-17,-0.342020142969288));
#114545=DIRECTION('',(5.13675726285535E-34,-1.,-1.22464674570954E-16));
#114546=DIRECTION('',(-5.13675726285535E-34,1.,1.22464674570954E-16));
#114547=DIRECTION('center_axis',(5.13675726285535E-34,-1.,-1.22464674570954E-16));
#114548=DIRECTION('ref_axis',(0.0784590959774507,1.22087156847365E-16,-0.996917333713484));
#114549=DIRECTION('',(5.13675726285535E-34,-1.,-1.22464674570954E-16));
#114550=DIRECTION('center_axis',(5.13675726285535E-34,-1.,-1.22464674570954E-16));
#114551=DIRECTION('ref_axis',(-0.93969262091562,4.18853855054451E-17,-0.342020142969288));
#114552=DIRECTION('center_axis',(5.13675726285535E-34,-1.,-1.22464674570954E-16));
#114553=DIRECTION('ref_axis',(-0.93969262091562,4.18853855054451E-17,-0.342020142969288));
#114554=DIRECTION('center_axis',(5.13675726285535E-34,-1.,-1.22464674570954E-16));
#114555=DIRECTION('ref_axis',(-0.933573134654503,-4.38897405736607E-17,
0.358386944867368));
#114556=DIRECTION('center_axis',(5.13675726285535E-34,-1.,-1.22464674570954E-16));
#114557=DIRECTION('ref_axis',(-0.93969262091562,4.18853855054451E-17,-0.342020142969288));
#114558=DIRECTION('',(5.13675726285535E-34,-1.,-1.22464674570954E-16));
#114559=DIRECTION('center_axis',(5.13675726285535E-34,-1.,-1.22464674570954E-16));
#114560=DIRECTION('ref_axis',(-0.93969262091562,4.18853855054451E-17,-0.342020142969288));
#114561=DIRECTION('',(5.13675726285535E-34,-1.,-1.22464674570954E-16));
#114562=DIRECTION('',(-5.13675726285535E-34,1.,1.22464674570954E-16));
#114563=DIRECTION('center_axis',(5.13675726285535E-34,-1.,-1.22464674570954E-16));
#114564=DIRECTION('ref_axis',(0.0784590959774507,1.22087156847365E-16,-0.996917333713484));
#114565=DIRECTION('',(5.13675726285535E-34,-1.,-1.22464674570954E-16));
#114566=DIRECTION('center_axis',(5.13675726285535E-34,-1.,-1.22464674570954E-16));
#114567=DIRECTION('ref_axis',(-0.93969262091562,4.18853855054451E-17,-0.342020142969288));
#114568=DIRECTION('center_axis',(5.13675726285535E-34,-1.,-1.22464674570954E-16));
#114569=DIRECTION('ref_axis',(-0.93969262091562,4.18853855054451E-17,-0.342020142969288));
#114570=DIRECTION('center_axis',(5.13675726285535E-34,-1.,-1.22464674570954E-16));
#114571=DIRECTION('ref_axis',(-0.975074486292716,-2.71721892731301E-17,
0.221877773066607));
#114572=DIRECTION('center_axis',(5.13675726285535E-34,-1.,-1.22464674570954E-16));
#114573=DIRECTION('ref_axis',(-0.93969262091562,4.18853855054451E-17,-0.342020142969288));
#114574=DIRECTION('',(5.13675726285535E-34,-1.,-1.22464674570954E-16));
#114575=DIRECTION('center_axis',(5.13675726285535E-34,-1.,-1.22464674570954E-16));
#114576=DIRECTION('ref_axis',(-0.93969262091562,4.18853855054451E-17,-0.342020142969288));
#114577=DIRECTION('',(5.13675726285535E-34,-1.,-1.22464674570954E-16));
#114578=DIRECTION('',(-5.13675726285535E-34,1.,1.22464674570954E-16));
#114579=DIRECTION('center_axis',(5.13675726285535E-34,-1.,-1.22464674570954E-16));
#114580=DIRECTION('ref_axis',(0.0784590959774507,1.22087156847365E-16,-0.996917333713484));
#114581=DIRECTION('',(5.13675726285535E-34,-1.,-1.22464674570954E-16));
#114582=DIRECTION('center_axis',(5.13675726285535E-34,-1.,-1.22464674570954E-16));
#114583=DIRECTION('ref_axis',(-0.93969262091562,4.18853855054451E-17,-0.342020142969288));
#114584=DIRECTION('center_axis',(5.13675726285535E-34,-1.,-1.22464674570954E-16));
#114585=DIRECTION('ref_axis',(-0.93969262091562,4.18853855054451E-17,-0.342020142969288));
#114586=DIRECTION('center_axis',(5.13675726285535E-34,-1.,-1.22464674570954E-16));
#114587=DIRECTION('ref_axis',(-0.996726133306289,-9.9014906031653E-18,0.0808518100248454));
#114588=DIRECTION('center_axis',(5.13675726285535E-34,-1.,-1.22464674570954E-16));
#114589=DIRECTION('ref_axis',(-0.93969262091562,4.18853855054451E-17,-0.342020142969288));
#114590=DIRECTION('',(5.13675726285535E-34,-1.,-1.22464674570954E-16));
#114591=DIRECTION('center_axis',(5.13675726285535E-34,-1.,-1.22464674570954E-16));
#114592=DIRECTION('ref_axis',(-0.93969262091562,4.18853855054451E-17,-0.342020142969288));
#114593=DIRECTION('',(5.13675726285535E-34,-1.,-1.22464674570954E-16));
#114594=DIRECTION('',(-5.13675726285535E-34,1.,1.22464674570954E-16));
#114595=DIRECTION('center_axis',(5.13675726285535E-34,-1.,-1.22464674570954E-16));
#114596=DIRECTION('ref_axis',(0.0784590959774507,1.22087156847365E-16,-0.996917333713484));
#114597=DIRECTION('',(5.13675726285535E-34,-1.,-1.22464674570954E-16));
#114598=DIRECTION('center_axis',(5.13675726285535E-34,-1.,-1.22464674570954E-16));
#114599=DIRECTION('ref_axis',(-0.93969262091562,4.18853855054451E-17,-0.342020142969288));
#114600=DIRECTION('center_axis',(5.13675726285535E-34,-1.,-1.22464674570954E-16));
#114601=DIRECTION('ref_axis',(-0.93969262091562,4.18853855054451E-17,-0.342020142969288));
#114602=DIRECTION('center_axis',(5.13675726285535E-34,-1.,-1.22464674570954E-16));
#114603=DIRECTION('ref_axis',(-0.998087310654575,7.57077401709542E-18,-0.0618200639786049));
#114604=DIRECTION('center_axis',(5.13675726285535E-34,-1.,-1.22464674570954E-16));
#114605=DIRECTION('ref_axis',(-0.93969262091562,4.18853855054451E-17,-0.342020142969288));
#114606=DIRECTION('',(5.13675726285535E-34,-1.,-1.22464674570954E-16));
#114607=DIRECTION('center_axis',(5.13675726285535E-34,-1.,-1.22464674570954E-16));
#114608=DIRECTION('ref_axis',(-0.93969262091562,4.18853855054451E-17,-0.342020142969288));
#114609=DIRECTION('',(5.13675726285535E-34,-1.,-1.22464674570954E-16));
#114610=DIRECTION('',(-5.13675726285535E-34,1.,1.22464674570954E-16));
#114611=DIRECTION('center_axis',(5.13675726285535E-34,-1.,-1.22464674570954E-16));
#114612=DIRECTION('ref_axis',(0.0784590959774507,1.22087156847365E-16,-0.996917333713484));
#114613=DIRECTION('',(5.13675726285535E-34,-1.,-1.22464674570954E-16));
#114614=DIRECTION('center_axis',(5.13675726285535E-34,-1.,-1.22464674570954E-16));
#114615=DIRECTION('ref_axis',(-0.93969262091562,4.18853855054451E-17,-0.342020142969288));
#114616=DIRECTION('center_axis',(5.13675726285535E-34,-1.,-1.22464674570954E-16));
#114617=DIRECTION('ref_axis',(-0.93969262091562,4.18853855054451E-17,-0.342020142969288));
#114618=DIRECTION('center_axis',(5.13675726285535E-34,-1.,-1.22464674570954E-16));
#114619=DIRECTION('ref_axis',(-0.979130308579199,2.48889194076679E-17,-0.203233458912656));
#114620=DIRECTION('center_axis',(5.13675726285535E-34,-1.,-1.22464674570954E-16));
#114621=DIRECTION('ref_axis',(-0.93969262091562,4.18853855054451E-17,-0.342020142969288));
#114622=DIRECTION('',(5.13675726285535E-34,-1.,-1.22464674570954E-16));
#114623=DIRECTION('center_axis',(5.13675726285535E-34,-1.,-1.22464674570954E-16));
#114624=DIRECTION('ref_axis',(-0.93969262091562,4.18853855054451E-17,-0.342020142969288));
#114625=DIRECTION('',(5.13675726285535E-34,-1.,-1.22464674570954E-16));
#114626=DIRECTION('',(-5.13675726285535E-34,1.,1.22464674570954E-16));
#114627=DIRECTION('center_axis',(5.13675726285535E-34,-1.,-1.22464674570954E-16));
#114628=DIRECTION('ref_axis',(0.0784590959774507,1.22087156847365E-16,-0.996917333713484));
#114629=DIRECTION('',(5.13675726285535E-34,-1.,-1.22464674570954E-16));
#114630=DIRECTION('center_axis',(5.13675726285535E-34,-1.,-1.22464674570954E-16));
#114631=DIRECTION('ref_axis',(-0.93969262091562,4.18853855054451E-17,-0.342020142969288));
#114632=DIRECTION('center_axis',(5.13675726285535E-34,-1.,-1.22464674570954E-16));
#114633=DIRECTION('ref_axis',(-0.93969262091562,4.18853855054451E-17,-0.342020142969288));
#114634=DIRECTION('center_axis',(5.13675726285535E-34,-1.,-1.22464674570954E-16));
#114635=DIRECTION('ref_axis',(-0.940241036944465,4.17003982070755E-17,-0.340509606979888));
#114636=DIRECTION('center_axis',(5.13675726285535E-34,-1.,-1.22464674570954E-16));
#114637=DIRECTION('ref_axis',(-0.93969262091562,4.18853855054451E-17,-0.342020142969288));
#114638=DIRECTION('',(5.13675726285535E-34,-1.,-1.22464674570954E-16));
#114639=DIRECTION('center_axis',(5.13675726285535E-34,-1.,-1.22464674570954E-16));
#114640=DIRECTION('ref_axis',(-0.93969262091562,4.18853855054451E-17,-0.342020142969288));
#114641=DIRECTION('',(5.13675726285535E-34,-1.,-1.22464674570954E-16));
#114642=DIRECTION('',(-5.13675726285535E-34,1.,1.22464674570954E-16));
#114643=DIRECTION('center_axis',(5.13675726285535E-34,-1.,-1.22464674570954E-16));
#114644=DIRECTION('ref_axis',(0.0784590959774507,1.22087156847365E-16,-0.996917333713484));
#114645=DIRECTION('',(5.13675726285535E-34,-1.,-1.22464674570954E-16));
#114646=DIRECTION('center_axis',(5.13675726285535E-34,-1.,-1.22464674570954E-16));
#114647=DIRECTION('ref_axis',(-0.93969262091562,4.18853855054451E-17,-0.342020142969288));
#114648=DIRECTION('center_axis',(5.13675726285535E-34,-1.,-1.22464674570954E-16));
#114649=DIRECTION('ref_axis',(-0.93969262091562,4.18853855054451E-17,-0.342020142969288));
#114650=DIRECTION('center_axis',(5.13675726285535E-34,-1.,-1.22464674570954E-16));
#114651=DIRECTION('ref_axis',(-0.882211169309773,5.76629771245571E-17,-0.470853961165332));
#114652=DIRECTION('center_axis',(5.13675726285535E-34,-1.,-1.22464674570954E-16));
#114653=DIRECTION('ref_axis',(-0.93969262091562,4.18853855054451E-17,-0.342020142969288));
#114654=DIRECTION('',(5.13675726285535E-34,-1.,-1.22464674570954E-16));
#114655=DIRECTION('center_axis',(5.13675726285535E-34,-1.,-1.22464674570954E-16));
#114656=DIRECTION('ref_axis',(-0.93969262091562,4.18853855054451E-17,-0.342020142969288));
#114657=DIRECTION('',(5.13675726285535E-34,-1.,-1.22464674570954E-16));
#114658=DIRECTION('',(-5.13675726285535E-34,1.,1.22464674570954E-16));
#114659=DIRECTION('center_axis',(5.13675726285535E-34,-1.,-1.22464674570954E-16));
#114660=DIRECTION('ref_axis',(0.0784590959774507,1.22087156847365E-16,-0.996917333713484));
#114661=DIRECTION('',(5.13675726285535E-34,-1.,-1.22464674570954E-16));
#114662=DIRECTION('center_axis',(5.13675726285535E-34,-1.,-1.22464674570954E-16));
#114663=DIRECTION('ref_axis',(-0.93969262091562,4.18853855054451E-17,-0.342020142969288));
#114664=DIRECTION('center_axis',(5.13675726285535E-34,-1.,-1.22464674570954E-16));
#114665=DIRECTION('ref_axis',(-0.93969262091562,4.18853855054451E-17,-0.342020142969288));
#114666=DIRECTION('center_axis',(5.13675726285535E-34,-1.,-1.22464674570954E-16));
#114667=DIRECTION('ref_axis',(-0.806222026033372,7.24517041743716E-17,-0.591613087024489));
#114668=DIRECTION('center_axis',(5.13675726285535E-34,-1.,-1.22464674570954E-16));
#114669=DIRECTION('ref_axis',(-0.93969262091562,4.18853855054451E-17,-0.342020142969288));
#114670=DIRECTION('',(5.13675726285535E-34,-1.,-1.22464674570954E-16));
#114671=DIRECTION('center_axis',(5.13675726285535E-34,-1.,-1.22464674570954E-16));
#114672=DIRECTION('ref_axis',(-0.93969262091562,4.18853855054451E-17,-0.342020142969288));
#114673=DIRECTION('',(5.13675726285535E-34,-1.,-1.22464674570954E-16));
#114674=DIRECTION('',(-5.13675726285535E-34,1.,1.22464674570954E-16));
#114675=DIRECTION('center_axis',(5.13675726285535E-34,-1.,-1.22464674570954E-16));
#114676=DIRECTION('ref_axis',(0.0784590959774507,1.22087156847365E-16,-0.996917333713484));
#114677=DIRECTION('',(5.13675726285535E-34,-1.,-1.22464674570954E-16));
#114678=DIRECTION('center_axis',(5.13675726285535E-34,-1.,-1.22464674570954E-16));
#114679=DIRECTION('ref_axis',(-0.93969262091562,4.18853855054451E-17,-0.342020142969288));
#114680=DIRECTION('center_axis',(5.13675726285535E-34,-1.,-1.22464674570954E-16));
#114681=DIRECTION('ref_axis',(-0.93969262091562,4.18853855054451E-17,-0.342020142969288));
#114682=DIRECTION('center_axis',(5.13675726285535E-34,-1.,-1.22464674570954E-16));
#114683=DIRECTION('ref_axis',(-0.713820527777962,8.57655233723694E-17,-0.700328675782159));
#114684=DIRECTION('center_axis',(5.13675726285535E-34,-1.,-1.22464674570954E-16));
#114685=DIRECTION('ref_axis',(-0.93969262091562,4.18853855054451E-17,-0.342020142969288));
#114686=DIRECTION('',(5.13675726285535E-34,-1.,-1.22464674570954E-16));
#114687=DIRECTION('center_axis',(5.13675726285535E-34,-1.,-1.22464674570954E-16));
#114688=DIRECTION('ref_axis',(-0.93969262091562,4.18853855054451E-17,-0.342020142969288));
#114689=DIRECTION('',(5.13675726285535E-34,-1.,-1.22464674570954E-16));
#114690=DIRECTION('',(-5.13675726285535E-34,1.,1.22464674570954E-16));
#114691=DIRECTION('center_axis',(5.13675726285535E-34,-1.,-1.22464674570954E-16));
#114692=DIRECTION('ref_axis',(0.0784590959774507,1.22087156847365E-16,-0.996917333713484));
#114693=DIRECTION('',(5.13675726285535E-34,-1.,-1.22464674570954E-16));
#114694=DIRECTION('center_axis',(5.13675726285535E-34,-1.,-1.22464674570954E-16));
#114695=DIRECTION('ref_axis',(-0.93969262091562,4.18853855054451E-17,-0.342020142969288));
#114696=DIRECTION('center_axis',(5.13675726285535E-34,-1.,-1.22464674570954E-16));
#114697=DIRECTION('ref_axis',(-0.93969262091562,4.18853855054451E-17,-0.342020142969288));
#114698=DIRECTION('center_axis',(5.13675726285535E-34,-1.,-1.22464674570954E-16));
#114699=DIRECTION('ref_axis',(-0.606887701749485,9.73334038895991E-17,-0.794787592671922));
#114700=DIRECTION('center_axis',(5.13675726285535E-34,-1.,-1.22464674570954E-16));
#114701=DIRECTION('ref_axis',(-0.93969262091562,4.18853855054451E-17,-0.342020142969288));
#114702=DIRECTION('',(5.13675726285535E-34,-1.,-1.22464674570954E-16));
#114703=DIRECTION('center_axis',(5.13675726285535E-34,-1.,-1.22464674570954E-16));
#114704=DIRECTION('ref_axis',(-0.93969262091562,4.18853855054451E-17,-0.342020142969288));
#114705=DIRECTION('',(5.13675726285535E-34,-1.,-1.22464674570954E-16));
#114706=DIRECTION('',(-5.13675726285535E-34,1.,1.22464674570954E-16));
#114707=DIRECTION('center_axis',(5.13675726285535E-34,-1.,-1.22464674570954E-16));
#114708=DIRECTION('ref_axis',(0.0784590959774507,1.22087156847365E-16,-0.996917333713484));
#114709=DIRECTION('',(5.13675726285535E-34,-1.,-1.22464674570954E-16));
#114710=DIRECTION('center_axis',(5.13675726285535E-34,-1.,-1.22464674570954E-16));
#114711=DIRECTION('ref_axis',(-0.93969262091562,4.18853855054451E-17,-0.342020142969288));
#114712=DIRECTION('center_axis',(5.13675726285535E-34,-1.,-1.22464674570954E-16));
#114713=DIRECTION('ref_axis',(-0.93969262091562,4.18853855054451E-17,-0.342020142969288));
#114714=DIRECTION('center_axis',(5.13675726285535E-34,-1.,-1.22464674570954E-16));
#114715=DIRECTION('ref_axis',(-0.487600392108822,1.06919856995116E-16,-0.87306692619485));
#114716=DIRECTION('center_axis',(5.13675726285535E-34,-1.,-1.22464674570954E-16));
#114717=DIRECTION('ref_axis',(-0.93969262091562,4.18853855054451E-17,-0.342020142969288));
#114718=DIRECTION('',(5.13675726285535E-34,-1.,-1.22464674570954E-16));
#114719=DIRECTION('center_axis',(5.13675726285535E-34,-1.,-1.22464674570954E-16));
#114720=DIRECTION('ref_axis',(-0.93969262091562,4.18853855054451E-17,-0.342020142969288));
#114721=DIRECTION('',(5.13675726285535E-34,-1.,-1.22464674570954E-16));
#114722=DIRECTION('',(-5.13675726285535E-34,1.,1.22464674570954E-16));
#114723=DIRECTION('center_axis',(5.13675726285535E-34,-1.,-1.22464674570954E-16));
#114724=DIRECTION('ref_axis',(0.0784590959774507,1.22087156847365E-16,-0.996917333713484));
#114725=DIRECTION('',(5.13675726285535E-34,-1.,-1.22464674570954E-16));
#114726=DIRECTION('center_axis',(5.13675726285535E-34,-1.,-1.22464674570954E-16));
#114727=DIRECTION('ref_axis',(-0.93969262091562,4.18853855054451E-17,-0.342020142969288));
#114728=DIRECTION('center_axis',(5.13675726285535E-34,-1.,-1.22464674570954E-16));
#114729=DIRECTION('ref_axis',(-0.93969262091562,4.18853855054451E-17,-0.342020142969288));
#114730=DIRECTION('center_axis',(5.13675726285535E-34,-1.,-1.22464674570954E-16));
#114731=DIRECTION('ref_axis',(-0.358386944867368,1.14329730123649E-16,-0.933573134654503));
#114732=DIRECTION('center_axis',(5.13675726285535E-34,-1.,-1.22464674570954E-16));
#114733=DIRECTION('ref_axis',(-0.93969262091562,4.18853855054451E-17,-0.342020142969288));
#114734=DIRECTION('',(5.13675726285535E-34,-1.,-1.22464674570954E-16));
#114735=DIRECTION('center_axis',(5.13675726285535E-34,-1.,-1.22464674570954E-16));
#114736=DIRECTION('ref_axis',(-0.93969262091562,4.18853855054451E-17,-0.342020142969288));
#114737=DIRECTION('',(5.13675726285535E-34,-1.,-1.22464674570954E-16));
#114738=DIRECTION('',(-5.13675726285535E-34,1.,1.22464674570954E-16));
#114739=DIRECTION('center_axis',(5.13675726285535E-34,-1.,-1.22464674570954E-16));
#114740=DIRECTION('ref_axis',(0.0784590959774507,1.22087156847365E-16,-0.996917333713484));
#114741=DIRECTION('',(5.13675726285535E-34,-1.,-1.22464674570954E-16));
#114742=DIRECTION('center_axis',(5.13675726285535E-34,-1.,-1.22464674570954E-16));
#114743=DIRECTION('ref_axis',(-0.93969262091562,4.18853855054451E-17,-0.342020142969288));
#114744=DIRECTION('center_axis',(5.13675726285535E-34,-1.,-1.22464674570954E-16));
#114745=DIRECTION('ref_axis',(-0.93969262091562,4.18853855054451E-17,-0.342020142969288));
#114746=DIRECTION('center_axis',(5.13675726285535E-34,-1.,-1.22464674570954E-16));
#114747=DIRECTION('ref_axis',(-0.221877773066607,1.19412179646278E-16,-0.975074486292716));
#114748=DIRECTION('center_axis',(5.13675726285535E-34,-1.,-1.22464674570954E-16));
#114749=DIRECTION('ref_axis',(-0.93969262091562,4.18853855054451E-17,-0.342020142969288));
#114750=DIRECTION('',(5.13675726285535E-34,-1.,-1.22464674570954E-16));
#114751=DIRECTION('center_axis',(5.13675726285535E-34,-1.,-1.22464674570954E-16));
#114752=DIRECTION('ref_axis',(-0.93969262091562,4.18853855054451E-17,-0.342020142969288));
#114753=DIRECTION('',(5.13675726285535E-34,-1.,-1.22464674570954E-16));
#114754=DIRECTION('',(-5.13675726285535E-34,1.,1.22464674570954E-16));
#114755=DIRECTION('center_axis',(5.13675726285535E-34,-1.,-1.22464674570954E-16));
#114756=DIRECTION('ref_axis',(0.0784590959774507,1.22087156847365E-16,-0.996917333713484));
#114757=DIRECTION('center_axis',(5.13675726285535E-34,-1.,-1.22464674570954E-16));
#114758=DIRECTION('ref_axis',(-0.93969262091562,4.18853855054451E-17,-0.342020142969288));
#114759=DIRECTION('center_axis',(5.13675726285535E-34,-1.,-1.22464674570954E-16));
#114760=DIRECTION('ref_axis',(-0.93969262091562,4.18853855054451E-17,-0.342020142969288));
#114761=DIRECTION('center_axis',(5.13675726285535E-34,-1.,-1.22464674570954E-16));
#114762=DIRECTION('ref_axis',(-0.93969262091562,4.18853855054451E-17,-0.342020142969288));
#114763=DIRECTION('center_axis',(5.13675726285535E-34,-1.,-1.22464674570954E-16));
#114764=DIRECTION('ref_axis',(0.93969262091562,-4.18853855054451E-17,0.342020142969288));
#114765=DIRECTION('center_axis',(5.13675726285535E-34,-1.,-1.22464674570954E-16));
#114766=DIRECTION('ref_axis',(0.0784590959774507,1.22087156847365E-16,-0.996917333713484));
#114767=DIRECTION('',(-5.13675726285535E-34,1.,1.22464674570954E-16));
#114768=DIRECTION('center_axis',(5.13675726285535E-34,-1.,-1.22464674570954E-16));
#114769=DIRECTION('ref_axis',(-0.93969262091562,4.18853855054451E-17,-0.342020142969288));
#114770=DIRECTION('center_axis',(5.13675726285535E-34,-1.,-1.22464674570954E-16));
#114771=DIRECTION('ref_axis',(0.0784590959774507,1.22087156847365E-16,-0.996917333713484));
#114772=DIRECTION('',(5.13675726285535E-34,-1.,-1.22464674570954E-16));
#114773=DIRECTION('center_axis',(5.13675726285535E-34,-1.,-1.22464674570954E-16));
#114774=DIRECTION('ref_axis',(-0.93969262091562,4.18853855054451E-17,-0.342020142969288));
#114775=DIRECTION('center_axis',(5.13675726285535E-34,-1.,-1.22464674570954E-16));
#114776=DIRECTION('ref_axis',(-0.0808518100248454,1.2206374155172E-16,-0.996726133306289));
#114777=DIRECTION('',(5.13675726285535E-34,-1.,-1.22464674570954E-16));
#114778=DIRECTION('center_axis',(5.13675726285535E-34,-1.,-1.22464674570954E-16));
#114779=DIRECTION('ref_axis',(-0.93969262091562,4.18853855054451E-17,-0.342020142969288));
#114780=DIRECTION('',(5.13675726285535E-34,-1.,-1.22464674570954E-16));
#114781=DIRECTION('center_axis',(5.13675726285535E-34,-1.,-1.22464674570954E-16));
#114782=DIRECTION('ref_axis',(0.93969262091562,-4.18853855054451E-17,0.342020142969288));
#114783=DIRECTION('',(5.13675726285535E-34,-1.,-1.22464674570954E-16));
#114784=DIRECTION('center_axis',(5.13675726285535E-34,-1.,-1.22464674570954E-16));
#114785=DIRECTION('ref_axis',(0.93969262091562,-4.18853855054451E-17,0.342020142969288));
#114786=DIRECTION('center_axis',(5.13675726285535E-34,-1.,-1.22464674570954E-16));
#114787=DIRECTION('ref_axis',(-1.5735453877384E-50,1.22464674570954E-16,
-1.));
#114788=DIRECTION('center_axis',(4.44089209850063E-16,1.,1.22464674570954E-16));
#114789=DIRECTION('ref_axis',(-1.,4.44089209850063E-16,-2.07165259840883E-30));
#114790=DIRECTION('center_axis',(5.55111512312577E-16,1.,1.22464679914736E-16));
#114791=DIRECTION('ref_axis',(-1.,5.55111512312577E-16,-2.05805628826764E-30));
#114792=DIRECTION('',(-4.44089209850063E-16,-1.,-1.22464674570954E-16));
#114793=DIRECTION('center_axis',(-1.56641358065672E-32,-1.,-1.22464674570954E-16));
#114794=DIRECTION('ref_axis',(-0.0784590959774507,-1.22087156847365E-16,
0.996917333713484));
#114795=DIRECTION('center_axis',(4.44089209850063E-16,1.,1.22464674570954E-16));
#114796=DIRECTION('ref_axis',(-1.,4.44089209850063E-16,-2.07165259840883E-30));
#114797=DIRECTION('center_axis',(-1.56641358065672E-32,-1.,-1.22464674570954E-16));
#114798=DIRECTION('ref_axis',(-1.,4.44089209850063E-16,-2.07165259840883E-30));
#114799=DIRECTION('',(-4.44089209850063E-16,-1.,-1.22464674570954E-16));
#114800=DIRECTION('center_axis',(-5.55111512312577E-16,-1.,-1.22464679914736E-16));
#114801=DIRECTION('ref_axis',(-1.,5.55111512312577E-16,-2.05805628826764E-30));
#114802=DIRECTION('center_axis',(5.55111512312577E-16,1.,1.22464679914736E-16));
#114803=DIRECTION('ref_axis',(-1.,5.55111512312577E-16,-2.05805628826764E-30));
#114804=DIRECTION('center_axis',(5.55111512312577E-16,1.,1.22464679914736E-16));
#114805=DIRECTION('ref_axis',(-1.,5.55111512312577E-16,-2.05805628826764E-30));
#114806=DIRECTION('center_axis',(1.56641358065672E-32,1.,1.22464674570954E-16));
#114807=DIRECTION('ref_axis',(0.0784590959774507,1.22087156847365E-16,-0.996917333713484));
#114808=DIRECTION('',(-0.334274317935853,-1.15419995177468E-16,0.942475824819141));
#114809=DIRECTION('center_axis',(1.56641358065672E-32,1.,1.22464674570954E-16));
#114810=DIRECTION('ref_axis',(-0.93969262091562,4.18853855054452E-17,-0.342020142969288));
#114811=DIRECTION('',(0.184775606034611,1.20355923031387E-16,-0.98278073618409));
#114812=DIRECTION('center_axis',(1.56641358065672E-32,1.,1.22464674570954E-16));
#114813=DIRECTION('ref_axis',(-0.93969262091562,4.18853855054451E-17,-0.342020142969288));
#114814=DIRECTION('',(0.0287600210011737,-1.2241401645099E-16,0.999586345040793));
#114815=DIRECTION('center_axis',(1.56641358065672E-32,1.,1.22464674570954E-16));
#114816=DIRECTION('ref_axis',(-0.93969262091562,4.18853855054452E-17,-0.342020142969288));
#114817=DIRECTION('',(-0.182723229956296,1.20402907287232E-16,-0.983164391764845));
#114818=DIRECTION('center_axis',(1.56641358065672E-32,1.,1.22464674570954E-16));
#114819=DIRECTION('ref_axis',(-0.93969262091562,4.18853855054451E-17,-0.342020142969288));
#114820=DIRECTION('',(0.387910159064799,-1.12875346322704E-16,0.921697189153966));
#114821=DIRECTION('center_axis',(1.56641358065672E-32,1.,1.22464674570954E-16));
#114822=DIRECTION('ref_axis',(-0.93969262091562,4.18853855054452E-17,-0.342020142969288));
#114823=DIRECTION('',(-0.525544280992694,1.04188811695823E-16,-0.850766247988172));
#114824=DIRECTION('center_axis',(1.56641358065672E-32,1.,1.22464674570954E-16));
#114825=DIRECTION('ref_axis',(-0.93969262091562,4.18853855054451E-17,-0.342020142969288));
#114826=DIRECTION('',(0.694670879902617,-8.80922351273172E-17,0.71932771989916));
#114827=DIRECTION('center_axis',(1.56641358065672E-32,1.,1.22464674570954E-16));
#114828=DIRECTION('ref_axis',(-0.93969262091562,4.18853855054452E-17,-0.342020142969288));
#114829=DIRECTION('',(-0.797387662985364,7.39034399784702E-17,-0.603467409988924));
#114830=DIRECTION('center_axis',(1.56641358065672E-32,1.,1.22464674570954E-16));
#114831=DIRECTION('ref_axis',(-0.93969262091562,4.18853855054451E-17,-0.342020142969288));
#114832=DIRECTION('',(0.907612447952903,-5.14117795447764E-17,0.419809056978216));
#114833=DIRECTION('center_axis',(1.56641358065672E-32,1.,1.22464674570954E-16));
#114834=DIRECTION('ref_axis',(-0.93969262091562,4.18853855054452E-17,-0.342020142969288));
#114835=DIRECTION('',(-0.961539424227938,3.36369991449791E-17,-0.274666954065111));
#114836=DIRECTION('center_axis',(1.56641358065672E-32,1.,1.22464674570954E-16));
#114837=DIRECTION('ref_axis',(-0.93969262091562,4.18853855054451E-17,-0.342020142969288));
#114838=DIRECTION('',(0.997975925895315,-7.78787841426065E-18,0.0635928559933293));
#114839=DIRECTION('center_axis',(1.56641358065672E-32,1.,1.22464674570954E-16));
#114840=DIRECTION('ref_axis',(-0.93969262091562,4.18853855054452E-17,-0.342020142969288));
#114841=DIRECTION('',(-0.995829958489319,-1.11723051865237E-17,0.0912287990448269));
#114842=DIRECTION('center_axis',(1.56641358065672E-32,1.,1.22464674570954E-16));
#114843=DIRECTION('ref_axis',(-0.93969262091562,4.18853855054451E-17,-0.342020142969288));
#114844=DIRECTION('',(0.953557225147758,3.68878192755495E-17,-0.301211916046674));
#114845=DIRECTION('center_axis',(1.56641358065672E-32,1.,1.22464674570954E-16));
#114846=DIRECTION('ref_axis',(-0.93969262091562,4.18853855054452E-17,-0.342020142969288));
#114847=DIRECTION('',(-0.895628138133327,-5.44727275177746E-17,0.444803595066215));
#114848=DIRECTION('center_axis',(1.56641358065672E-32,1.,1.22464674570954E-16));
#114849=DIRECTION('ref_axis',(-0.93969262091562,4.18853855054451E-17,-0.342020142969288));
#114850=DIRECTION('',(0.780355338322394,7.65816121419183E-17,-0.62533634625835));
#114851=DIRECTION('center_axis',(1.56641358065672E-32,1.,1.22464674570954E-16));
#114852=DIRECTION('ref_axis',(-0.93969262091562,4.18853855054452E-17,-0.342020142969288));
#114853=DIRECTION('',(-0.674466775907303,-9.04163060396167E-17,0.738305199898529));
#114854=DIRECTION('center_axis',(1.56641358065672E-32,1.,1.22464674570954E-16));
#114855=DIRECTION('ref_axis',(-0.93969262091562,4.18853855054451E-17,-0.342020142969288));
#114856=DIRECTION('',(0.501762135978649,1.05932634322597E-16,-0.865005640963193));
#114857=DIRECTION('center_axis',(1.56641358065672E-32,1.,1.22464674570954E-16));
#114858=DIRECTION('ref_axis',(-0.93969262091562,4.18853855054452E-17,-0.342020142969288));
#114859=DIRECTION('',(-0.362214936962566,-1.14148661601617E-16,0.93209459790367));
#114860=DIRECTION('center_axis',(1.56641358065672E-32,1.,1.22464674570954E-16));
#114861=DIRECTION('ref_axis',(-0.93969262091562,4.18853855054451E-17,-0.342020142969288));
#114862=DIRECTION('',(0.15540318800344,1.20976866795283E-16,-0.987851127021864));
#114863=DIRECTION('center_axis',(1.56641358065672E-32,1.,1.22464674570954E-16));
#114864=DIRECTION('ref_axis',(-0.93969262091562,4.18853855054452E-17,-0.342020142969288));
#114865=DIRECTION('',(-0.00104396100007576,-1.22464607836593E-16,0.999999455072567));
#114866=DIRECTION('center_axis',(1.56641358065672E-32,1.,1.22464674570954E-16));
#114867=DIRECTION('ref_axis',(-0.93969262091562,4.18853855054451E-17,-0.342020142969288));
#114868=DIRECTION('',(-0.211943832922472,1.19682503558106E-16,-0.977281848642515));
#114869=DIRECTION('center_axis',(1.56641358065672E-32,1.,1.22464674570954E-16));
#114870=DIRECTION('ref_axis',(-0.93969262091562,4.18853855054452E-17,-0.342020142969288));
#114871=DIRECTION('',(0.360268003917448,-1.14241030078174E-16,0.932848843786247));
#114872=DIRECTION('center_axis',(1.56641358065672E-32,1.,1.22464674570954E-16));
#114873=DIRECTION('ref_axis',(-0.93969262091562,4.18853855054451E-17,-0.342020142969288));
#114874=DIRECTION('',(-0.550666659981411,1.0222435511424E-16,-0.834725241971822));
#114875=DIRECTION('center_axis',(1.56641358065672E-32,1.,1.22464674570954E-16));
#114876=DIRECTION('ref_axis',(-0.93969262091562,4.18853855054452E-17,-0.342020142969288));
#114877=DIRECTION('',(0.672923776631946,-9.05885684876879E-17,0.739711829595417));
#114878=DIRECTION('center_axis',(1.56641358065672E-32,1.,1.22464674570954E-16));
#114879=DIRECTION('ref_axis',(-0.93969262091562,4.18853855054451E-17,-0.342020142969288));
#114880=DIRECTION('',(-0.815018905804237,7.09602409279082E-17,-0.579434364860823));
#114881=DIRECTION('center_axis',(1.56641358065672E-32,1.,1.22464674570954E-16));
#114882=DIRECTION('ref_axis',(-0.93969262091562,4.18853855054452E-17,-0.342020142969288));
#114883=DIRECTION('',(0.894697468857086,-5.47016183864292E-17,0.446672630928651));
#114884=DIRECTION('center_axis',(1.56641358065672E-32,1.,1.22464674570954E-16));
#114885=DIRECTION('ref_axis',(-0.93969262091562,4.18853855054451E-17,-0.342020142969288));
#114886=DIRECTION('',(-0.969298331894766,3.01125528719676E-17,-0.245887664973305));
#114887=DIRECTION('center_axis',(1.56641358065672E-32,1.,1.22464674570954E-16));
#114888=DIRECTION('ref_axis',(-0.93969262091562,4.18853855054452E-17,-0.342020142969288));
#114889=DIRECTION('',(0.995637308827798,-1.14269118092488E-17,0.0933078199838617));
#114890=DIRECTION('center_axis',(1.56641358065672E-32,1.,1.22464674570954E-16));
#114891=DIRECTION('ref_axis',(-0.93969262091562,4.18853855054451E-17,-0.342020142969288));
#114892=DIRECTION('',(-0.992668646322072,-1.48020021201242E-17,0.120867525039216));
#114893=DIRECTION('center_axis',(1.56641358065672E-32,1.,1.22464674570954E-16));
#114894=DIRECTION('ref_axis',(-0.93969262091562,4.18853855054452E-17,-0.342020142969288));
#114895=DIRECTION('',(0.96211081236153,3.3391063018321E-17,-0.272658733102456));
#114896=DIRECTION('center_axis',(1.56641358065672E-32,1.,1.22464674570954E-16));
#114897=DIRECTION('ref_axis',(-0.93969262091562,4.18853855054451E-17,-0.342020142969288));
#114898=DIRECTION('',(-0.881973559148804,-5.77174648318459E-17,0.471298887079516));
#114899=DIRECTION('center_axis',(1.56641358065672E-32,1.,1.22464674570954E-16));
#114900=DIRECTION('ref_axis',(-0.93969262091562,4.18853855054452E-17,-0.342020142969288));
#114901=DIRECTION('',(0.798645919725862,7.36993891912942E-17,-0.601801208793429));
#114902=DIRECTION('center_axis',(1.56641358065672E-32,1.,1.22464674570954E-16));
#114903=DIRECTION('ref_axis',(-0.93969262091562,4.18853855054451E-17,-0.342020142969288));
#114904=DIRECTION('',(-0.652163056951551,-9.28378638595332E-17,0.758078720943682));
#114905=DIRECTION('center_axis',(1.56641358065672E-32,1.,1.22464674570954E-16));
#114906=DIRECTION('ref_axis',(-0.93969262091562,4.18853855054452E-17,-0.342020142969288));
#114907=DIRECTION('',(0.527319471663896,1.0405420446143E-16,-0.849667096458437));
#114908=DIRECTION('center_axis',(1.56641358065672E-32,1.,1.22464674570954E-16));
#114909=DIRECTION('ref_axis',(-0.93969262091562,4.18853855054451E-17,-0.342020142969288));
#114910=DIRECTION('center_axis',(-1.56641358065672E-32,-1.,-1.22464674570954E-16));
#114911=DIRECTION('ref_axis',(0.93969262091562,-4.18853855054452E-17,0.342020142969288));
#114912=DIRECTION('center_axis',(-1.56641358065672E-32,-1.,-1.22464674570954E-16));
#114913=DIRECTION('ref_axis',(-0.0784590959774507,-1.22087156847365E-16,
0.996917333713484));
#114914=DIRECTION('center_axis',(1.56641358065672E-32,1.,1.22464674570954E-16));
#114915=DIRECTION('ref_axis',(-0.0784590959774507,-1.22087156847365E-16,
0.996917333713484));
#114916=DIRECTION('',(1.56641358065672E-32,1.,1.22464674570954E-16));
#114917=DIRECTION('center_axis',(1.56641358065672E-32,1.,1.22464674570954E-16));
#114918=DIRECTION('ref_axis',(-0.0784590959774507,-1.22087156847365E-16,
0.996917333713484));
#114919=DIRECTION('center_axis',(-1.56641358065672E-32,-1.,-1.22464674570954E-16));
#114920=DIRECTION('ref_axis',(-0.0784590959774507,-1.22087156847365E-16,
0.996917333713484));
#114921=DIRECTION('center_axis',(-1.56641358065672E-32,-1.,-1.22464674570954E-16));
#114922=DIRECTION('ref_axis',(-0.225894875006821,-1.19299169089874E-16,
0.974151685029417));
#114923=DIRECTION('',(-1.56641358065672E-32,-1.,-1.22464674570954E-16));
#114924=DIRECTION('center_axis',(-1.56641358065672E-32,-1.,-1.22464674570954E-16));
#114925=DIRECTION('ref_axis',(-0.225894875006821,-1.19299169089874E-16,
0.974151685029417));
#114926=DIRECTION('',(-1.56641358065672E-32,-1.,-1.22464674570954E-16));
#114927=DIRECTION('',(-1.56641358065672E-32,-1.,-1.22464674570954E-16));
#114928=DIRECTION('center_axis',(-0.932094434249406,4.4358585953941E-17,
-0.36221535809692));
#114929=DIRECTION('ref_axis',(0.36221535809692,1.14148641559751E-16,-0.932094434249406));
#114930=DIRECTION('',(1.56641358065672E-32,1.,1.22464674570954E-16));
#114931=DIRECTION('',(0.36221535809692,1.14148641559751E-16,-0.932094434249406));
#114932=DIRECTION('center_axis',(-1.56641358065672E-32,-1.,-1.22464674570954E-16));
#114933=DIRECTION('ref_axis',(0.0784590959774507,1.22087156847365E-16,-0.996917333713484));
#114934=DIRECTION('',(-1.56641358065672E-32,-1.,-1.22464674570954E-16));
#114935=DIRECTION('center_axis',(-1.56641358065672E-32,-1.,-1.22464674570954E-16));
#114936=DIRECTION('ref_axis',(0.0784590959774507,1.22087156847365E-16,-0.996917333713484));
#114937=DIRECTION('center_axis',(0.865005821949093,-6.14480984846721E-17,
0.501761823970471));
#114938=DIRECTION('ref_axis',(-0.501761823970471,-1.05932656486976E-16,
0.865005821949093));
#114939=DIRECTION('',(-1.56641358065672E-32,-1.,-1.22464674570954E-16));
#114940=DIRECTION('',(-0.501761823970471,-1.05932656486976E-16,0.865005821949093));
#114941=DIRECTION('',(-1.56641358065672E-32,-1.,-1.22464674570954E-16));
#114942=DIRECTION('center_axis',(-1.56641358065672E-32,-1.,-1.22464674570954E-16));
#114943=DIRECTION('ref_axis',(-0.562544874928296,-1.01249721339324E-16,
0.826766752894617));
#114944=DIRECTION('',(-1.56641358065672E-32,-1.,-1.22464674570954E-16));
#114945=DIRECTION('center_axis',(-1.56641358065672E-32,-1.,-1.22464674570954E-16));
#114946=DIRECTION('ref_axis',(-0.562544874928296,-1.01249721339324E-16,
0.826766752894617));
#114947=DIRECTION('',(-1.56641358065672E-32,-1.,-1.22464674570954E-16));
#114948=DIRECTION('center_axis',(-0.738304895785748,8.25983949885278E-17,
-0.674467108804273));
#114949=DIRECTION('ref_axis',(0.674467108804273,9.04162687965439E-17,-0.738304895785748));
#114950=DIRECTION('',(1.56641358065672E-32,1.,1.22464674570954E-16));
#114951=DIRECTION('',(0.674467108804273,9.04162687965439E-17,-0.738304895785748));
#114952=DIRECTION('center_axis',(-1.56641358065672E-32,-1.,-1.22464674570954E-16));
#114953=DIRECTION('ref_axis',(0.0784590959774507,1.22087156847365E-16,-0.996917333713484));
#114954=DIRECTION('',(-1.56641358065672E-32,-1.,-1.22464674570954E-16));
#114955=DIRECTION('center_axis',(-1.56641358065672E-32,-1.,-1.22464674570954E-16));
#114956=DIRECTION('ref_axis',(0.0784590959774507,1.22087156847365E-16,-0.996917333713484));
#114957=DIRECTION('center_axis',(0.625336629973868,-9.55659347144022E-17,
0.780355110967389));
#114958=DIRECTION('ref_axis',(-0.780355110967389,-7.65816468870469E-17,
0.625336629973867));
#114959=DIRECTION('',(-1.56641358065672E-32,-1.,-1.22464674570954E-16));
#114960=DIRECTION('',(-0.780355110967389,-7.65816468870469E-17,0.625336629973867));
#114961=DIRECTION('',(-1.56641358065672E-32,-1.,-1.22464674570954E-16));
#114962=DIRECTION('center_axis',(-1.56641358065672E-32,-1.,-1.22464674570954E-16));
#114963=DIRECTION('ref_axis',(-0.823220073969957,-6.95259374905277E-17,
0.567722387979282));
#114964=DIRECTION('',(-1.56641358065672E-32,-1.,-1.22464674570954E-16));
#114965=DIRECTION('center_axis',(-1.56641358065672E-32,-1.,-1.22464674570954E-16));
#114966=DIRECTION('ref_axis',(-0.823220073969957,-6.95259374905277E-17,
0.567722387979282));
#114967=DIRECTION('',(-1.56641358065672E-32,-1.,-1.22464674570954E-16));
#114968=DIRECTION('center_axis',(-0.444803189723036,1.09682833126328E-16,
-0.895628339442323));
#114969=DIRECTION('ref_axis',(0.895628339442323,5.4472677877554E-17,-0.444803189723036));
#114970=DIRECTION('',(1.56641358065672E-32,1.,1.22464674570954E-16));
#114971=DIRECTION('',(0.895628339442323,5.4472677877554E-17,-0.444803189723036));
#114972=DIRECTION('center_axis',(-1.56641358065672E-32,-1.,-1.22464674570954E-16));
#114973=DIRECTION('ref_axis',(0.0784590959774507,1.22087156847365E-16,-0.996917333713484));
#114974=DIRECTION('',(-1.56641358065672E-32,-1.,-1.22464674570954E-16));
#114975=DIRECTION('center_axis',(-1.56641358065672E-32,-1.,-1.22464674570954E-16));
#114976=DIRECTION('ref_axis',(0.0784590959774507,1.22087156847365E-16,-0.996917333713484));
#114977=DIRECTION('center_axis',(0.301212261052566,-1.16777061916137E-16,
0.95355711616641));
#114978=DIRECTION('ref_axis',(-0.95355711616641,-3.68878615265838E-17,0.301212261052566));
#114979=DIRECTION('',(-1.56641358065672E-32,-1.,-1.22464674570954E-16));
#114980=DIRECTION('',(-0.95355711616641,-3.68878615265838E-17,0.301212261052566));
#114981=DIRECTION('',(-1.56641358065672E-32,-1.,-1.22464674570954E-16));
#114982=DIRECTION('center_axis',(-1.56641358065672E-32,-1.,-1.22464674570954E-16));
#114983=DIRECTION('ref_axis',(-0.972714838948175,-2.84122906837056E-17,
0.232003969987639));
#114984=DIRECTION('',(-1.56641358065672E-32,-1.,-1.22464674570954E-16));
#114985=DIRECTION('center_axis',(-1.56641358065672E-32,-1.,-1.22464674570954E-16));
#114986=DIRECTION('ref_axis',(-0.972714838948175,-2.84122906837056E-17,
0.232003969987639));
#114987=DIRECTION('',(-1.56641358065672E-32,-1.,-1.22464674570954E-16));
#114988=DIRECTION('center_axis',(-0.0912283479827209,1.21953996854895E-16,
-0.995829999811385));
#114989=DIRECTION('ref_axis',(0.995829999811385,1.11722499473497E-17,-0.091228347982721));
#114990=DIRECTION('',(1.56641358065672E-32,1.,1.22464674570954E-16));
#114991=DIRECTION('',(0.995829999811385,1.11722499473497E-17,-0.0912283479827209));
#114992=DIRECTION('center_axis',(-1.56641358065672E-32,-1.,-1.22464674570954E-16));
#114993=DIRECTION('ref_axis',(0.0784590959774507,1.22087156847365E-16,-0.996917333713484));
#114994=DIRECTION('',(-1.56641358065672E-32,-1.,-1.22464674570954E-16));
#114995=DIRECTION('center_axis',(-1.56641358065672E-32,-1.,-1.22464674570954E-16));
#114996=DIRECTION('ref_axis',(0.0784590959774507,1.22087156847365E-16,-0.996917333713484));
#114997=DIRECTION('center_axis',(-0.0635924930016405,-1.22216799827077E-16,
0.997975949025745));
#114998=DIRECTION('ref_axis',(-0.997975949025745,7.78783396060161E-18,-0.0635924930016405));
#114999=DIRECTION('',(-1.56641358065672E-32,-1.,-1.22464674570954E-16));
#115000=DIRECTION('',(-0.997975949025745,7.78783396060161E-18,-0.0635924930016405));
#115001=DIRECTION('',(-1.56641358065672E-32,-1.,-1.22464674570954E-16));
#115002=DIRECTION('center_axis',(-1.56641358065672E-32,-1.,-1.22464674570954E-16));
#115003=DIRECTION('ref_axis',(-0.990839075129605,1.65385934532139E-17,-0.135047870017665));
#115004=DIRECTION('',(-1.56641358065672E-32,-1.,-1.22464674570954E-16));
#115005=DIRECTION('center_axis',(-1.56641358065672E-32,-1.,-1.22464674570954E-16));
#115006=DIRECTION('ref_axis',(-0.990839075129605,1.65385934532139E-17,-0.135047870017665));
#115007=DIRECTION('',(-1.56641358065672E-32,-1.,-1.22464674570954E-16));
#115008=DIRECTION('center_axis',(0.274667386883407,1.17754597534162E-16,
-0.961539300591838));
#115009=DIRECTION('ref_axis',(0.961539300591838,-3.36370521499308E-17,0.274667386883407));
#115010=DIRECTION('',(1.56641358065672E-32,1.,1.22464674570954E-16));
#115011=DIRECTION('',(0.961539300591838,-3.36370521499308E-17,0.274667386883407));
#115012=DIRECTION('center_axis',(-1.56641358065672E-32,-1.,-1.22464674570954E-16));
#115013=DIRECTION('ref_axis',(0.0784590959774507,1.22087156847365E-16,-0.996917333713484));
#115014=DIRECTION('',(-1.56641358065672E-32,-1.,-1.22464674570954E-16));
#115015=DIRECTION('center_axis',(-1.56641358065672E-32,-1.,-1.22464674570954E-16));
#115016=DIRECTION('ref_axis',(0.0784590959774507,1.22087156847365E-16,-0.996917333713484));
#115017=DIRECTION('center_axis',(-0.419808728869155,-1.11150481660855E-16,
0.907612599717117));
#115018=DIRECTION('ref_axis',(-0.907612599717117,5.1411739363007E-17,-0.419808728869155));
#115019=DIRECTION('',(-1.56641358065672E-32,-1.,-1.22464674570954E-16));
#115020=DIRECTION('',(-0.907612599717117,5.1411739363007E-17,-0.419808728869155));
#115021=DIRECTION('',(-1.56641358065672E-32,-1.,-1.22464674570954E-16));
#115022=DIRECTION('center_axis',(-1.56641358065672E-32,-1.,-1.22464674570954E-16));
#115023=DIRECTION('ref_axis',(-0.875145004198729,5.92558488100051E-17,-0.483860746109876));
#115024=DIRECTION('',(-1.56641358065672E-32,-1.,-1.22464674570954E-16));
#115025=DIRECTION('center_axis',(-1.56641358065672E-32,-1.,-1.22464674570954E-16));
#115026=DIRECTION('ref_axis',(-0.875145004198729,5.92558488100051E-17,-0.483860746109876));
#115027=DIRECTION('',(-1.56641358065672E-32,-1.,-1.22464674570954E-16));
#115028=DIRECTION('center_axis',(0.603467769136497,9.76517873678849E-17,
-0.797387391180359));
#115029=DIRECTION('ref_axis',(0.79738739118036,-7.39034839613609E-17,0.603467769136497));
#115030=DIRECTION('',(1.56641358065672E-32,1.,1.22464674570954E-16));
#115031=DIRECTION('',(0.797387391180359,-7.39034839613609E-17,0.603467769136497));
#115032=DIRECTION('center_axis',(-1.56641358065672E-32,-1.,-1.22464674570954E-16));
#115033=DIRECTION('ref_axis',(0.0784590959774507,1.22087156847365E-16,-0.996917333713484));
#115034=DIRECTION('',(-1.56641358065672E-32,-1.,-1.22464674570954E-16));
#115035=DIRECTION('center_axis',(-1.56641358065672E-32,-1.,-1.22464674570954E-16));
#115036=DIRECTION('ref_axis',(0.0784590959774507,1.22087156847365E-16,-0.996917333713484));
#115037=DIRECTION('center_axis',(-0.719327468371104,-8.50726751378232E-17,
0.694671140358384));
#115038=DIRECTION('ref_axis',(-0.694671140358384,8.80922043240157E-17,-0.719327468371104));
#115039=DIRECTION('',(-1.56641358065672E-32,-1.,-1.22464674570954E-16));
#115040=DIRECTION('',(-0.694671140358384,8.80922043240157E-17,-0.719327468371104));
#115041=DIRECTION('',(-1.56641358065672E-32,-1.,-1.22464674570954E-16));
#115042=DIRECTION('center_axis',(-1.56641358065672E-32,-1.,-1.22464674570954E-16));
#115043=DIRECTION('ref_axis',(-0.641257749973319,9.3970273644354E-17,-0.767325548968074));
#115044=DIRECTION('',(-1.56641358065672E-32,-1.,-1.22464674570954E-16));
#115045=DIRECTION('center_axis',(-1.56641358065672E-32,-1.,-1.22464674570954E-16));
#115046=DIRECTION('ref_axis',(-0.641257749973319,9.3970273644354E-17,-0.767325548968074));
#115047=DIRECTION('',(-1.56641358065672E-32,-1.,-1.22464674570954E-16));
#115048=DIRECTION('center_axis',(0.850766486309441,6.4360562097336E-17,
-0.525543895191151));
#115049=DIRECTION('ref_axis',(0.525543895191151,-1.0418884088176E-16,0.850766486309441));
#115050=DIRECTION('',(1.56641358065672E-32,1.,1.22464674570954E-16));
#115051=DIRECTION('',(0.525543895191151,-1.0418884088176E-16,0.850766486309441));
#115052=DIRECTION('center_axis',(-1.56641358065672E-32,-1.,-1.22464674570954E-16));
#115053=DIRECTION('ref_axis',(0.0784590959774507,1.22087156847365E-16,-0.996917333713484));
#115054=DIRECTION('',(-1.56641358065672E-32,-1.,-1.22464674570954E-16));
#115055=DIRECTION('center_axis',(-1.56641358065672E-32,-1.,-1.22464674570954E-16));
#115056=DIRECTION('ref_axis',(0.0784590959774507,1.22087156847365E-16,-0.996917333713484));
#115057=DIRECTION('center_axis',(-0.92169704816257,-4.75053324187471E-17,
0.38791049406842));
#115058=DIRECTION('ref_axis',(-0.38791049406842,1.12875329056238E-16,-0.92169704816257));
#115059=DIRECTION('',(-1.56641358065672E-32,-1.,-1.22464674570954E-16));
#115060=DIRECTION('',(-0.38791049406842,1.12875329056238E-16,-0.92169704816257));
#115061=DIRECTION('',(-1.56641358065672E-32,-1.,-1.22464674570954E-16));
#115062=DIRECTION('center_axis',(-1.56641358065672E-32,-1.,-1.22464674570954E-16));
#115063=DIRECTION('ref_axis',(-0.320765085004956,1.15993492128908E-16,-0.947158783014634));
#115064=DIRECTION('',(-1.56641358065672E-32,-1.,-1.22464674570954E-16));
#115065=DIRECTION('center_axis',(-1.56641358065672E-32,-1.,-1.22464674570954E-16));
#115066=DIRECTION('ref_axis',(-0.320765085004956,1.15993492128908E-16,-0.947158783014634));
#115067=DIRECTION('',(-1.56641358065672E-32,-1.,-1.22464674570954E-16));
#115068=DIRECTION('center_axis',(0.983164474478833,2.23770863898615E-17,
-0.18272278490314));
#115069=DIRECTION('ref_axis',(0.18272278490314,-1.20402917416774E-16,0.983164474478834));
#115070=DIRECTION('',(1.56641358065672E-32,1.,1.22464674570954E-16));
#115071=DIRECTION('',(0.18272278490314,-1.20402917416774E-16,0.983164474478833));
#115072=DIRECTION('center_axis',(-1.56641358065672E-32,-1.,-1.22464674570954E-16));
#115073=DIRECTION('ref_axis',(0.0784590959774507,1.22087156847365E-16,-0.996917333713484));
#115074=DIRECTION('',(-1.56641358065672E-32,-1.,-1.22464674570954E-16));
#115075=DIRECTION('center_axis',(-1.56641358065672E-32,-1.,-1.22464674570954E-16));
#115076=DIRECTION('ref_axis',(0.0784590959774507,1.22087156847365E-16,-0.996917333713484));
#115077=DIRECTION('center_axis',(-0.999586334568139,-3.52213118803864E-18,
0.0287603849875744));
#115078=DIRECTION('ref_axis',(-0.0287603849875744,1.2241401516846E-16,-0.999586334568139));
#115079=DIRECTION('',(-1.56641358065672E-32,-1.,-1.22464674570954E-16));
#115080=DIRECTION('',(-0.0287603849875744,1.2241401516846E-16,-0.999586334568139));
#115081=DIRECTION('',(-1.56641358065672E-32,-1.,-1.22464674570954E-16));
#115082=DIRECTION('center_axis',(-1.56641358065672E-32,-1.,-1.22464674570954E-16));
#115083=DIRECTION('ref_axis',(0.0430486839877822,1.2235114684375E-16,-0.999072975716449));
#115084=DIRECTION('',(-1.56641358065672E-32,-1.,-1.22464674570954E-16));
#115085=DIRECTION('center_axis',(-1.56641358065672E-32,-1.,-1.22464674570954E-16));
#115086=DIRECTION('ref_axis',(0.0430486839877822,1.2235114684375E-16,-0.999072975716449));
#115087=DIRECTION('',(-1.56641358065672E-32,-1.,-1.22464674570954E-16));
#115088=DIRECTION('center_axis',(0.982780652540913,-2.26285389436506E-17,
0.184776050913685));
#115089=DIRECTION('ref_axis',(-0.184776050913685,-1.20355912788053E-16,
0.982780652540913));
#115090=DIRECTION('',(1.56641358065672E-32,1.,1.22464674570954E-16));
#115091=DIRECTION('',(-0.184776050913685,-1.20355912788053E-16,0.982780652540913));
#115092=DIRECTION('center_axis',(-1.56641358065672E-32,-1.,-1.22464674570954E-16));
#115093=DIRECTION('ref_axis',(0.0784590959774507,1.22087156847365E-16,-0.996917333713484));
#115094=DIRECTION('center_axis',(-1.56641358065672E-32,-1.,-1.22464674570954E-16));
#115095=DIRECTION('ref_axis',(0.0784590959774507,1.22087156847365E-16,-0.996917333713484));
#115096=DIRECTION('',(0.33427397305035,1.15420010157692E-16,-0.94247594714196));
#115097=DIRECTION('center_axis',(-1.56641358065672E-32,-1.,-1.22464674570954E-16));
#115098=DIRECTION('ref_axis',(0.401048487995911,1.12184601205912E-16,-0.916056826990659));
#115099=DIRECTION('',(-0.52731985596956,-1.04054175252689E-16,0.849666857950952));
#115100=DIRECTION('center_axis',(-1.56641358065672E-32,-1.,-1.22464674570954E-16));
#115101=DIRECTION('ref_axis',(0.0784590959774507,1.22087156847365E-16,-0.996917333713484));
#115102=DIRECTION('',(0.652162777961028,9.28378932524043E-17,-0.758078960954699));
#115103=DIRECTION('center_axis',(-1.56641358065672E-32,-1.,-1.22464674570954E-16));
#115104=DIRECTION('ref_axis',(0.704884471951656,8.68669035655391E-17,-0.709322127951352));
#115105=DIRECTION('',(-0.798646193064008,-7.36993447678216E-17,0.601800846048232));
#115106=DIRECTION('center_axis',(-1.56641358065672E-32,-1.,-1.22464674570954E-16));
#115107=DIRECTION('ref_axis',(0.0784590959774507,1.22087156847365E-16,-0.996917333713484));
#115108=DIRECTION('',(0.881973386681221,5.77175043573365E-17,-0.471299209829655));
#115109=DIRECTION('center_axis',(-1.56641358065672E-32,-1.,-1.22464674570954E-16));
#115110=DIRECTION('ref_axis',(0.913521902831698,4.98173491156488E-17,-0.406789543925055));
#115111=DIRECTION('',(-0.962110936816233,-3.33910092374037E-17,0.272658293947921));
#115112=DIRECTION('center_axis',(-1.56641358065672E-32,-1.,-1.22464674570954E-16));
#115113=DIRECTION('ref_axis',(0.0784590959774507,1.22087156847365E-16,-0.996917333713484));
#115114=DIRECTION('',(0.992668602005981,1.48020466925524E-17,-0.120867889000728));
#115115=DIRECTION('center_axis',(-1.56641358065672E-32,-1.,-1.22464674570954E-16));
#115116=DIRECTION('ref_axis',(0.998783137960738,6.03968575555981E-18,-0.0493177789980613));
#115117=DIRECTION('',(-0.995637266656693,1.14269669163886E-17,-0.0933082699678263));
#115118=DIRECTION('center_axis',(-1.56641358065672E-32,-1.,-1.22464674570954E-16));
#115119=DIRECTION('ref_axis',(0.0784590959774507,1.22087156847365E-16,-0.996917333713484));
#115120=DIRECTION('',(0.969298422184675,-3.01125092835498E-17,0.245887309046847));
#115121=DIRECTION('center_axis',(-1.56641358065672E-32,-1.,-1.22464674570954E-16));
#115122=DIRECTION('ref_axis',(0.949153176178072,-3.85536706080351E-17,0.314814625059063));
#115123=DIRECTION('',(-0.894697266701741,5.47016679751246E-17,-0.446673035851096));
#115124=DIRECTION('center_axis',(-1.56641358065672E-32,-1.,-1.22464674570954E-16));
#115125=DIRECTION('ref_axis',(0.0784590959774507,1.22087156847365E-16,-0.996917333713484));
#115126=DIRECTION('',(0.815019118992681,-7.09602042049129E-17,0.579434064994797));
#115127=DIRECTION('center_axis',(-1.56641358065672E-32,-1.,-1.22464674570954E-16));
#115128=DIRECTION('ref_axis',(0.771334818374299,-7.79401402152037E-17,0.636429570308834));
#115129=DIRECTION('',(-0.67292344359886,9.05886055900302E-17,-0.739712132559046));
#115130=DIRECTION('center_axis',(-1.56641358065672E-32,-1.,-1.22464674570954E-16));
#115131=DIRECTION('ref_axis',(0.0784590959774507,1.22087156847365E-16,-0.996917333713484));
#115132=DIRECTION('',(0.550666967895411,-1.02224330237946E-16,0.834725038841459));
#115133=DIRECTION('center_axis',(-1.56641358065672E-32,-1.,-1.22464674570954E-16));
#115134=DIRECTION('ref_axis',(0.489343419188033,-1.06800361983615E-16,0.872091175335105));
#115135=DIRECTION('',(-0.360267580169336,1.14241050119789E-16,-0.932849007438466));
#115136=DIRECTION('center_axis',(-1.56641358065672E-32,-1.,-1.22464674570954E-16));
#115137=DIRECTION('ref_axis',(0.0784590959774507,1.22087156847365E-16,-0.996917333713484));
#115138=DIRECTION('',(0.211944190997081,-1.19682494047993E-16,0.977281770986542));
#115139=DIRECTION('center_axis',(-1.56641358065672E-32,-1.,-1.22464674570954E-16));
#115140=DIRECTION('ref_axis',(0.141263479938992,-1.21236603048261E-16,0.989972034572455));
#115141=DIRECTION('',(0.00104441599957958,1.2246460777841E-16,-0.999999454597461));
#115142=DIRECTION('center_axis',(-1.56641358065672E-32,-1.,-1.22464674570954E-16));
#115143=DIRECTION('ref_axis',(-0.0784590959774507,-1.22087156847365E-16,
0.996917333713484));
#115144=DIRECTION('',(-0.155402821938502,-1.20976873847682E-16,0.987851184609074));
#115145=DIRECTION('center_axis',(0.987851184609074,-1.90313560161066E-17,
0.155402821938502));
#115146=DIRECTION('ref_axis',(-0.155402821938502,-1.20976873847682E-16,
0.987851184609074));
#115147=DIRECTION('',(-1.56641358065672E-32,-1.,-1.22464674570954E-16));
#115148=DIRECTION('',(-1.56641358065672E-32,-1.,-1.22464674570954E-16));
#115149=DIRECTION('center_axis',(-1.56641358065672E-32,-1.,-1.22464674570954E-16));
#115150=DIRECTION('ref_axis',(-0.0784590959774507,-1.22087156847365E-16,
0.996917333713484));
#115151=DIRECTION('',(1.56641358065672E-32,1.,1.22464674570954E-16));
#115152=DIRECTION('center_axis',(-0.999999454597461,1.27904065505227E-19,
-0.00104441599957958));
#115153=DIRECTION('ref_axis',(0.00104441599957958,1.2246460777841E-16,-0.999999454597461));
#115154=DIRECTION('',(-1.56641358065672E-32,-1.,-1.22464674570954E-16));
#115155=DIRECTION('',(-1.56641358065672E-32,-1.,-1.22464674570954E-16));
#115156=DIRECTION('center_axis',(-1.56641358065672E-32,-1.,-1.22464674570954E-16));
#115157=DIRECTION('ref_axis',(0.141263479938992,-1.21236603048261E-16,0.989972034572455));
#115158=DIRECTION('',(-1.56641358065672E-32,-1.,-1.22464674570954E-16));
#115159=DIRECTION('',(-1.56641358065672E-32,-1.,-1.22464674570954E-16));
#115160=DIRECTION('center_axis',(0.977281770986542,2.59556763776617E-17,
-0.211944190997081));
#115161=DIRECTION('ref_axis',(0.211944190997081,-1.19682494047993E-16,0.977281770986542));
#115162=DIRECTION('',(-1.56641358065672E-32,-1.,-1.22464674570954E-16));
#115163=DIRECTION('center_axis',(-1.56641358065672E-32,-1.,-1.22464674570954E-16));
#115164=DIRECTION('ref_axis',(0.0784590959774507,1.22087156847365E-16,-0.996917333713484));
#115165=DIRECTION('',(1.56641358065672E-32,1.,1.22464674570954E-16));
#115166=DIRECTION('center_axis',(0.834725038841459,6.74372510202856E-17,
-0.550666967895411));
#115167=DIRECTION('ref_axis',(0.550666967895411,-1.02224330237946E-16,0.834725038841459));
#115168=DIRECTION('',(-1.56641358065672E-32,-1.,-1.22464674570954E-16));
#115169=DIRECTION('',(-1.56641358065672E-32,-1.,-1.22464674570954E-16));
#115170=DIRECTION('center_axis',(-0.932849007438466,-4.41200519639029E-17,
0.360267580169336));
#115171=DIRECTION('ref_axis',(-0.360267580169336,1.14241050119789E-16,-0.932849007438466));
#115172=DIRECTION('',(-1.56641358065672E-32,-1.,-1.22464674570954E-16));
#115173=DIRECTION('',(-1.56641358065672E-32,-1.,-1.22464674570954E-16));
#115174=DIRECTION('center_axis',(-1.56641358065672E-32,-1.,-1.22464674570954E-16));
#115175=DIRECTION('ref_axis',(0.489343419188033,-1.06800361983615E-16,0.872091175335105));
#115176=DIRECTION('',(-1.56641358065672E-32,-1.,-1.22464674570954E-16));
#115177=DIRECTION('center_axis',(-0.739712132559046,-8.24093505315003E-17,
0.67292344359886));
#115178=DIRECTION('ref_axis',(-0.67292344359886,9.05886055900302E-17,-0.739712132559046));
#115179=DIRECTION('',(1.56641358065672E-32,1.,1.22464674570954E-16));
#115180=DIRECTION('',(-1.56641358065672E-32,-1.,-1.22464674570954E-16));
#115181=DIRECTION('center_axis',(0.579434064994797,9.98110511765445E-17,
-0.815019118992681));
#115182=DIRECTION('ref_axis',(0.815019118992681,-7.09602042049129E-17,0.579434064994797));
#115183=DIRECTION('',(-1.56641358065672E-32,-1.,-1.22464674570954E-16));
#115184=DIRECTION('',(-1.56641358065672E-32,-1.,-1.22464674570954E-16));
#115185=DIRECTION('',(-1.56641358065672E-32,-1.,-1.22464674570954E-16));
#115186=DIRECTION('center_axis',(-1.56641358065672E-32,-1.,-1.22464674570954E-16));
#115187=DIRECTION('ref_axis',(0.771334818374299,-7.79401402152037E-17,0.636429570308834));
#115188=DIRECTION('',(-1.56641358065672E-32,-1.,-1.22464674570954E-16));
#115189=DIRECTION('center_axis',(-1.56641358065672E-32,-1.,-1.22464674570954E-16));
#115190=DIRECTION('ref_axis',(0.0784590959774507,1.22087156847365E-16,-0.996917333713484));
#115191=DIRECTION('',(1.56641358065672E-32,1.,1.22464674570954E-16));
#115192=DIRECTION('center_axis',(-0.446673035851096,-1.09568809606151E-16,
0.894697266701741));
#115193=DIRECTION('ref_axis',(-0.894697266701741,5.47016679751246E-17,-0.446673035851096));
#115194=DIRECTION('',(-1.56641358065672E-32,-1.,-1.22464674570954E-16));
#115195=DIRECTION('',(-1.56641358065672E-32,-1.,-1.22464674570954E-16));
#115196=DIRECTION('center_axis',(-1.56641358065672E-32,-1.,-1.22464674570954E-16));
#115197=DIRECTION('ref_axis',(0.949153176178072,-3.85536706080351E-17,0.314814625059063));
#115198=DIRECTION('',(-1.56641358065672E-32,-1.,-1.22464674570954E-16));
#115199=DIRECTION('',(-1.56641358065672E-32,-1.,-1.22464674570954E-16));
#115200=DIRECTION('center_axis',(0.245887309046847,1.18704815834986E-16,
-0.969298422184675));
#115201=DIRECTION('ref_axis',(0.969298422184675,-3.01125092835499E-17,0.245887309046847));
#115202=DIRECTION('',(-1.56641358065672E-32,-1.,-1.22464674570954E-16));
#115203=DIRECTION('center_axis',(-1.56641358065672E-32,-1.,-1.22464674570954E-16));
#115204=DIRECTION('ref_axis',(0.0784590959774507,1.22087156847365E-16,-0.996917333713484));
#115205=DIRECTION('center_axis',(-1.56641358065672E-32,-1.,-1.22464674570954E-16));
#115206=DIRECTION('ref_axis',(0.0784590959774507,1.22087156847365E-16,-0.996917333713484));
#115207=DIRECTION('',(1.56641358065672E-32,1.,1.22464674570954E-16));
#115208=DIRECTION('center_axis',(-0.120867889000728,1.21566837301467E-16,
-0.992668602005981));
#115209=DIRECTION('ref_axis',(0.992668602005981,1.48020466925524E-17,-0.120867889000728));
#115210=DIRECTION('',(-1.56641358065672E-32,-1.,-1.22464674570954E-16));
#115211=DIRECTION('',(-1.56641358065672E-32,-1.,-1.22464674570954E-16));
#115212=DIRECTION('center_axis',(-0.0933082699678263,-1.21930393851826E-16,
0.995637266656693));
#115213=DIRECTION('ref_axis',(-0.995637266656693,1.14269669163886E-17,-0.0933082699678263));
#115214=DIRECTION('',(-1.56641358065672E-32,-1.,-1.22464674570954E-16));
#115215=DIRECTION('',(-1.56641358065672E-32,-1.,-1.22464674570954E-16));
#115216=DIRECTION('center_axis',(-1.56641358065672E-32,-1.,-1.22464674570954E-16));
#115217=DIRECTION('ref_axis',(0.998783137960738,6.03968575555981E-18,-0.0493177789980613));
#115218=DIRECTION('',(-1.56641358065672E-32,-1.,-1.22464674570954E-16));
#115219=DIRECTION('center_axis',(0.272658293947921,-1.17824602778356E-16,
0.962110936816233));
#115220=DIRECTION('ref_axis',(-0.962110936816233,-3.33910092374037E-17,
0.272658293947921));
#115221=DIRECTION('',(1.56641358065672E-32,1.,1.22464674570954E-16));
#115222=DIRECTION('',(-1.56641358065672E-32,-1.,-1.22464674570954E-16));
#115223=DIRECTION('center_axis',(-0.471299209829655,1.08010583780158E-16,
-0.881973386681221));
#115224=DIRECTION('ref_axis',(0.881973386681221,5.77175043573365E-17,-0.471299209829655));
#115225=DIRECTION('',(-1.56641358065672E-32,-1.,-1.22464674570954E-16));
#115226=DIRECTION('',(-1.56641358065672E-32,-1.,-1.22464674570954E-16));
#115227=DIRECTION('',(-1.56641358065672E-32,-1.,-1.22464674570954E-16));
#115228=DIRECTION('center_axis',(-1.56641358065672E-32,-1.,-1.22464674570954E-16));
#115229=DIRECTION('ref_axis',(0.913521902831698,4.98173491156488E-17,-0.406789543925055));
#115230=DIRECTION('',(-1.56641358065672E-32,-1.,-1.22464674570954E-16));
#115231=DIRECTION('center_axis',(-1.56641358065672E-32,-1.,-1.22464674570954E-16));
#115232=DIRECTION('ref_axis',(0.0784590959774507,1.22087156847365E-16,-0.996917333713484));
#115233=DIRECTION('',(1.56641358065672E-32,1.,1.22464674570954E-16));
#115234=DIRECTION('center_axis',(0.601800846048232,-9.78059461309152E-17,
0.798646193064008));
#115235=DIRECTION('ref_axis',(-0.798646193064008,-7.36993447678216E-17,
0.601800846048232));
#115236=DIRECTION('',(-1.56641358065672E-32,-1.,-1.22464674570954E-16));
#115237=DIRECTION('',(-1.56641358065672E-32,-1.,-1.22464674570954E-16));
#115238=DIRECTION('center_axis',(-1.56641358065672E-32,-1.,-1.22464674570954E-16));
#115239=DIRECTION('ref_axis',(0.704884471951656,8.68669035655391E-17,-0.709322127951352));
#115240=DIRECTION('',(-1.56641358065672E-32,-1.,-1.22464674570954E-16));
#115241=DIRECTION('',(-1.56641358065672E-32,-1.,-1.22464674570954E-16));
#115242=DIRECTION('center_axis',(-0.758078960954699,7.98669023702868E-17,
-0.652162777961028));
#115243=DIRECTION('ref_axis',(0.652162777961028,9.28378932524043E-17,-0.758078960954699));
#115244=DIRECTION('',(-1.56641358065672E-32,-1.,-1.22464674570954E-16));
#115245=DIRECTION('center_axis',(-1.56641358065672E-32,-1.,-1.22464674570954E-16));
#115246=DIRECTION('ref_axis',(0.0784590959774507,1.22087156847365E-16,-0.996917333713484));
#115247=DIRECTION('center_axis',(-1.56641358065672E-32,-1.,-1.22464674570954E-16));
#115248=DIRECTION('ref_axis',(0.0784590959774507,1.22087156847365E-16,-0.996917333713484));
#115249=DIRECTION('',(1.56641358065672E-32,1.,1.22464674570954E-16));
#115250=DIRECTION('center_axis',(-0.94247594714196,4.0936753327151E-17,
-0.33427397305035));
#115251=DIRECTION('ref_axis',(0.33427397305035,1.15420010157692E-16,-0.94247594714196));
#115252=DIRECTION('',(-1.56641358065672E-32,-1.,-1.22464674570954E-16));
#115253=DIRECTION('',(-1.56641358065672E-32,-1.,-1.22464674570954E-16));
#115254=DIRECTION('center_axis',(0.849666857950952,-6.45780545561146E-17,
0.52731985596956));
#115255=DIRECTION('ref_axis',(-0.52731985596956,-1.04054175252689E-16,0.849666857950952));
#115256=DIRECTION('',(-1.56641358065672E-32,-1.,-1.22464674570954E-16));
#115257=DIRECTION('',(-1.56641358065672E-32,-1.,-1.22464674570954E-16));
#115258=DIRECTION('center_axis',(-1.56641358065672E-32,-1.,-1.22464674570954E-16));
#115259=DIRECTION('ref_axis',(0.401048487995911,1.12184601205912E-16,-0.916056826990659));
#115260=DIRECTION('',(-1.56641358065672E-32,-1.,-1.22464674570954E-16));
#115261=DIRECTION('center_axis',(-1.56641358065672E-32,-1.,-1.22464674570954E-16));
#115262=DIRECTION('ref_axis',(0.0784590959774507,1.22087156847365E-16,-0.996917333713484));
#115263=DIRECTION('center_axis',(-1.56641358065672E-32,-1.,-1.22464674570954E-16));
#115264=DIRECTION('ref_axis',(0.93969262091562,-4.18853855054452E-17,0.342020142969288));
#115265=DIRECTION('',(1.56641358065672E-32,1.,1.22464674570954E-16));
#115266=DIRECTION('center_axis',(1.56641358065672E-32,1.,1.22464674570954E-16));
#115267=DIRECTION('ref_axis',(0.93969262091562,-4.18853855054452E-17,0.342020142969288));
#115268=DIRECTION('center_axis',(1.56641358065672E-32,1.,1.22464674570954E-16));
#115269=DIRECTION('ref_axis',(0.0784590959774507,1.22087156847365E-16,-0.996917333713484));
#153537=CARTESIAN_POINT('',(0.,0.,0.));
#153538=CARTESIAN_POINT('Origin',(-5.66257110645729E-14,15.2,-1.77635683940025E-14));
#153539=CARTESIAN_POINT('',(0.710930733999944,15.2,-11.478004072));
#153540=CARTESIAN_POINT('',(1.09337742899994,15.2,-11.447904865));
#153541=CARTESIAN_POINT('Origin',(-5.66257110645729E-14,15.2,-1.77635683940025E-14));
#153542=CARTESIAN_POINT('',(1.09337742899994,12.2,-11.447904865));
#153543=CARTESIAN_POINT('',(1.09337742899994,15.2,-11.447904865));
#153544=CARTESIAN_POINT('',(0.710930733999944,12.2,-11.478004072));
#153545=CARTESIAN_POINT('Origin',(-5.66257110645729E-14,12.2,-1.77635683940025E-14));
#153546=CARTESIAN_POINT('',(0.710930733999944,15.2,-11.478004072));
#153547=CARTESIAN_POINT('Ctrl Pts',(0.292001928999944,15.2,-10.370890023));
#153548=CARTESIAN_POINT('Ctrl Pts',(0.292001928999944,11.6,-10.370890023));
#153549=CARTESIAN_POINT('Ctrl Pts',(0.292021795999944,15.2,-10.371063246));
#153550=CARTESIAN_POINT('Ctrl Pts',(0.292021795999944,11.6,-10.371063246));
#153551=CARTESIAN_POINT('Ctrl Pts',(0.292062308999944,15.2,-10.371415731));
#153552=CARTESIAN_POINT('Ctrl Pts',(0.292062308999944,11.6,-10.371415731));
#153553=CARTESIAN_POINT('Ctrl Pts',(0.292123960999945,15.2,-10.371949799));
#153554=CARTESIAN_POINT('Ctrl Pts',(0.292123960999945,11.6,-10.371949799));
#153555=CARTESIAN_POINT('Ctrl Pts',(0.292207546999944,15.2,-10.372669176));
#153556=CARTESIAN_POINT('Ctrl Pts',(0.292207546999944,11.6,-10.372669176));
#153557=CARTESIAN_POINT('Ctrl Pts',(0.292314179999943,15.2,-10.373578975));
#153558=CARTESIAN_POINT('Ctrl Pts',(0.292314179999943,11.6,-10.373578975));
#153559=CARTESIAN_POINT('Ctrl Pts',(0.292423468999944,15.2,-10.374503411));
#153560=CARTESIAN_POINT('Ctrl Pts',(0.292423468999944,11.6,-10.374503411));
#153561=CARTESIAN_POINT('Ctrl Pts',(0.292534811999945,15.2,-10.375437184));
#153562=CARTESIAN_POINT('Ctrl Pts',(0.292534811999945,11.6,-10.375437184));
#153563=CARTESIAN_POINT('Ctrl Pts',(0.292648222999944,15.2,-10.376380266));
#153564=CARTESIAN_POINT('Ctrl Pts',(0.292648222999944,11.6,-10.376380266));
#153565=CARTESIAN_POINT('Ctrl Pts',(0.292763716999945,15.2,-10.377332627));
#153566=CARTESIAN_POINT('Ctrl Pts',(0.292763716999945,11.6,-10.377332627));
#153567=CARTESIAN_POINT('Ctrl Pts',(0.292881308999944,15.2,-10.378294239));
#153568=CARTESIAN_POINT('Ctrl Pts',(0.292881308999944,11.6,-10.378294239));
#153569=CARTESIAN_POINT('Ctrl Pts',(0.293001014999945,15.2,-10.379265074));
#153570=CARTESIAN_POINT('Ctrl Pts',(0.293001014999945,11.6,-10.379265074));
#153571=CARTESIAN_POINT('Ctrl Pts',(0.293122845999945,15.2,-10.380245102));
#153572=CARTESIAN_POINT('Ctrl Pts',(0.293122845999945,11.6,-10.380245102));
#153573=CARTESIAN_POINT('Ctrl Pts',(0.293246819999944,15.2,-10.381234297));
#153574=CARTESIAN_POINT('Ctrl Pts',(0.293246819999944,11.6,-10.381234297));
#153575=CARTESIAN_POINT('Ctrl Pts',(0.293372948999944,15.2,-10.382232628));
#153576=CARTESIAN_POINT('Ctrl Pts',(0.293372948999944,11.6,-10.382232628));
#153577=CARTESIAN_POINT('Ctrl Pts',(0.293501248999943,15.2,-10.383240069));
#153578=CARTESIAN_POINT('Ctrl Pts',(0.293501248999943,11.6,-10.383240069));
#153579=CARTESIAN_POINT('Ctrl Pts',(0.293631731999945,15.2,-10.384256592));
#153580=CARTESIAN_POINT('Ctrl Pts',(0.293631731999945,11.6,-10.384256592));
#153581=CARTESIAN_POINT('Ctrl Pts',(0.293764412999945,15.2,-10.385282168));
#153582=CARTESIAN_POINT('Ctrl Pts',(0.293764412999945,11.6,-10.385282168));
#153583=CARTESIAN_POINT('Ctrl Pts',(0.293899306999944,15.2,-10.38631677));
#153584=CARTESIAN_POINT('Ctrl Pts',(0.293899306999944,11.6,-10.38631677));
#153585=CARTESIAN_POINT('Ctrl Pts',(0.294036426999943,15.2,-10.387360371));
#153586=CARTESIAN_POINT('Ctrl Pts',(0.294036426999943,11.6,-10.387360371));
#153587=CARTESIAN_POINT('Ctrl Pts',(0.294175786999944,15.2,-10.388412945));
#153588=CARTESIAN_POINT('Ctrl Pts',(0.294175786999944,11.6,-10.388412945));
#153589=CARTESIAN_POINT('Ctrl Pts',(0.294317400999944,15.2,-10.389474461));
#153590=CARTESIAN_POINT('Ctrl Pts',(0.294317400999944,11.6,-10.389474461));
#153591=CARTESIAN_POINT('Ctrl Pts',(0.294461281999944,15.2,-10.390544895));
#153592=CARTESIAN_POINT('Ctrl Pts',(0.294461281999944,11.6,-10.390544895));
#153593=CARTESIAN_POINT('Ctrl Pts',(0.294607443999944,15.2,-10.391624218));
#153594=CARTESIAN_POINT('Ctrl Pts',(0.294607443999944,11.6,-10.391624218));
#153595=CARTESIAN_POINT('Ctrl Pts',(0.294755900999943,15.2,-10.392712404));
#153596=CARTESIAN_POINT('Ctrl Pts',(0.294755900999943,11.6,-10.392712404));
#153597=CARTESIAN_POINT('Ctrl Pts',(0.294906665999944,15.2,-10.393809427));
#153598=CARTESIAN_POINT('Ctrl Pts',(0.294906665999944,11.6,-10.393809427));
#153599=CARTESIAN_POINT('Ctrl Pts',(0.295059751999943,15.2,-10.394915259));
#153600=CARTESIAN_POINT('Ctrl Pts',(0.295059751999943,11.6,-10.394915259));
#153601=CARTESIAN_POINT('Ctrl Pts',(0.295215172999944,15.2,-10.396029875));
#153602=CARTESIAN_POINT('Ctrl Pts',(0.295215172999944,11.6,-10.396029875));
#153603=CARTESIAN_POINT('Ctrl Pts',(0.295372941999944,15.2,-10.397153247));
#153604=CARTESIAN_POINT('Ctrl Pts',(0.295372941999944,11.6,-10.397153247));
#153605=CARTESIAN_POINT('Ctrl Pts',(0.295533071999945,15.2,-10.39828535));
#153606=CARTESIAN_POINT('Ctrl Pts',(0.295533071999945,11.6,-10.39828535));
#153607=CARTESIAN_POINT('Ctrl Pts',(0.295695575999944,15.2,-10.399426157));
#153608=CARTESIAN_POINT('Ctrl Pts',(0.295695575999944,11.6,-10.399426157));
#153609=CARTESIAN_POINT('Ctrl Pts',(0.295860466999944,15.2,-10.400575642));
#153610=CARTESIAN_POINT('Ctrl Pts',(0.295860466999944,11.6,-10.400575642));
#153611=CARTESIAN_POINT('Ctrl Pts',(0.296027758999945,15.2,-10.401733778));
#153612=CARTESIAN_POINT('Ctrl Pts',(0.296027758999945,11.6,-10.401733778));
#153613=CARTESIAN_POINT('Ctrl Pts',(0.296197462999944,15.2,-10.402900542));
#153614=CARTESIAN_POINT('Ctrl Pts',(0.296197462999944,11.6,-10.402900542));
#153615=CARTESIAN_POINT('Ctrl Pts',(0.296369592999944,15.2,-10.404075906));
#153616=CARTESIAN_POINT('Ctrl Pts',(0.296369592999944,11.6,-10.404075906));
#153617=CARTESIAN_POINT('Ctrl Pts',(0.296544161999943,15.2,-10.405259845));
#153618=CARTESIAN_POINT('Ctrl Pts',(0.296544161999943,11.6,-10.405259845));
#153619=CARTESIAN_POINT('Ctrl Pts',(0.296721181999944,15.2,-10.406452335));
#153620=CARTESIAN_POINT('Ctrl Pts',(0.296721181999944,11.6,-10.406452335));
#153621=CARTESIAN_POINT('Ctrl Pts',(0.296900663999944,15.2,-10.407653347));
#153622=CARTESIAN_POINT('Ctrl Pts',(0.296900663999944,11.6,-10.407653347));
#153623=CARTESIAN_POINT('Ctrl Pts',(0.297082623999945,15.2,-10.408862859));
#153624=CARTESIAN_POINT('Ctrl Pts',(0.297082623999945,11.6,-10.408862859));
#153625=CARTESIAN_POINT('Ctrl Pts',(0.297267072999944,15.2,-10.410080845));
#153626=CARTESIAN_POINT('Ctrl Pts',(0.297267072999944,11.6,-10.410080845));
#153627=CARTESIAN_POINT('Ctrl Pts',(0.297454020999943,15.2,-10.411307279));
#153628=CARTESIAN_POINT('Ctrl Pts',(0.297454020999943,11.6,-10.411307279));
#153629=CARTESIAN_POINT('Ctrl Pts',(0.297643483999943,15.2,-10.412542137));
#153630=CARTESIAN_POINT('Ctrl Pts',(0.297643483999943,11.6,-10.412542137));
#153631=CARTESIAN_POINT('Ctrl Pts',(0.297835472999944,15.2,-10.413785393));
#153632=CARTESIAN_POINT('Ctrl Pts',(0.297835472999944,11.6,-10.413785393));
#153633=CARTESIAN_POINT('Ctrl Pts',(0.298029997999943,15.2,-10.415037024));
#153634=CARTESIAN_POINT('Ctrl Pts',(0.298029997999943,11.6,-10.415037024));
#153635=CARTESIAN_POINT('Ctrl Pts',(0.298227073999945,15.2,-10.416297005));
#153636=CARTESIAN_POINT('Ctrl Pts',(0.298227073999945,11.6,-10.416297005));
#153637=CARTESIAN_POINT('Ctrl Pts',(0.298426710999945,15.2,-10.41756531));
#153638=CARTESIAN_POINT('Ctrl Pts',(0.298426710999945,11.6,-10.41756531));
#153639=CARTESIAN_POINT('Ctrl Pts',(0.298628921999944,15.2,-10.418841915));
#153640=CARTESIAN_POINT('Ctrl Pts',(0.298628921999944,11.6,-10.418841915));
#153641=CARTESIAN_POINT('Ctrl Pts',(0.298833718999945,15.2,-10.420126796));
#153642=CARTESIAN_POINT('Ctrl Pts',(0.298833718999945,11.6,-10.420126796));
#153643=CARTESIAN_POINT('Ctrl Pts',(0.299041113999945,15.2,-10.421419931));
#153644=CARTESIAN_POINT('Ctrl Pts',(0.299041113999945,11.6,-10.421419931));
#153645=CARTESIAN_POINT('Ctrl Pts',(0.299251117999945,15.2,-10.422721292));
#153646=CARTESIAN_POINT('Ctrl Pts',(0.299251117999945,11.6,-10.422721292));
#153647=CARTESIAN_POINT('Ctrl Pts',(0.299463742999944,15.2,-10.424030856));
#153648=CARTESIAN_POINT('Ctrl Pts',(0.299463742999944,11.6,-10.424030856));
#153649=CARTESIAN_POINT('Ctrl Pts',(0.299679000999945,15.2,-10.425348601));
#153650=CARTESIAN_POINT('Ctrl Pts',(0.299679000999945,11.6,-10.425348601));
#153651=CARTESIAN_POINT('Ctrl Pts',(0.299896902999944,15.2,-10.426674502));
#153652=CARTESIAN_POINT('Ctrl Pts',(0.299896902999944,11.6,-10.426674502));
#153653=CARTESIAN_POINT('Ctrl Pts',(0.300117460999945,15.2,-10.428008535));
#153654=CARTESIAN_POINT('Ctrl Pts',(0.300117460999945,11.6,-10.428008535));
#153655=CARTESIAN_POINT('Ctrl Pts',(0.300340685999944,15.2,-10.429350676));
#153656=CARTESIAN_POINT('Ctrl Pts',(0.300340685999944,11.6,-10.429350676));
#153657=CARTESIAN_POINT('Ctrl Pts',(0.300566589999944,15.2,-10.430700902));
#153658=CARTESIAN_POINT('Ctrl Pts',(0.300566589999944,11.6,-10.430700902));
#153659=CARTESIAN_POINT('Ctrl Pts',(0.300795183999943,15.2,-10.43205919));
#153660=CARTESIAN_POINT('Ctrl Pts',(0.300795183999943,11.6,-10.43205919));
#153661=CARTESIAN_POINT('Ctrl Pts',(0.301026478999944,15.2,-10.433425516));
#153662=CARTESIAN_POINT('Ctrl Pts',(0.301026478999944,11.6,-10.433425516));
#153663=CARTESIAN_POINT('Ctrl Pts',(0.301260486999944,15.2,-10.434799858));
#153664=CARTESIAN_POINT('Ctrl Pts',(0.301260486999944,11.6,-10.434799858));
#153665=CARTESIAN_POINT('Ctrl Pts',(0.301497219999945,15.2,-10.43618219));
#153666=CARTESIAN_POINT('Ctrl Pts',(0.301497219999945,11.6,-10.43618219));
#153667=CARTESIAN_POINT('Ctrl Pts',(0.301736685999944,15.2,-10.437572491));
#153668=CARTESIAN_POINT('Ctrl Pts',(0.301736685999944,11.6,-10.437572491));
#153669=CARTESIAN_POINT('Ctrl Pts',(0.301978897999945,15.2,-10.438970738));
#153670=CARTESIAN_POINT('Ctrl Pts',(0.301978897999945,11.6,-10.438970738));
#153671=CARTESIAN_POINT('Ctrl Pts',(0.302223867999943,15.2,-10.440376907));
#153672=CARTESIAN_POINT('Ctrl Pts',(0.302223867999943,11.6,-10.440376907));
#153673=CARTESIAN_POINT('Ctrl Pts',(0.302471604999944,15.2,-10.441790977));
#153674=CARTESIAN_POINT('Ctrl Pts',(0.302471604999944,11.6,-10.441790977));
#153675=CARTESIAN_POINT('Ctrl Pts',(0.302722120999944,15.2,-10.443212923));
#153676=CARTESIAN_POINT('Ctrl Pts',(0.302722120999944,11.6,-10.443212923));
#153677=CARTESIAN_POINT('Ctrl Pts',(0.302975424999945,15.2,-10.444642725));
#153678=CARTESIAN_POINT('Ctrl Pts',(0.302975424999945,11.6,-10.444642725));
#153679=CARTESIAN_POINT('Ctrl Pts',(0.303231531999945,15.2,-10.446080357));
#153680=CARTESIAN_POINT('Ctrl Pts',(0.303231531999945,11.6,-10.446080357));
#153681=CARTESIAN_POINT('Ctrl Pts',(0.303490447999945,15.2,-10.447525799));
#153682=CARTESIAN_POINT('Ctrl Pts',(0.303490447999945,11.6,-10.447525799));
#153683=CARTESIAN_POINT('Ctrl Pts',(0.303752185999944,15.2,-10.448979029));
#153684=CARTESIAN_POINT('Ctrl Pts',(0.303752185999944,11.6,-10.448979029));
#153685=CARTESIAN_POINT('Ctrl Pts',(0.304016755999944,15.2,-10.450440023));
#153686=CARTESIAN_POINT('Ctrl Pts',(0.304016755999944,11.6,-10.450440023));
#153687=CARTESIAN_POINT('Ctrl Pts',(0.304284168999944,15.2,-10.451908761));
#153688=CARTESIAN_POINT('Ctrl Pts',(0.304284168999944,11.6,-10.451908761));
#153689=CARTESIAN_POINT('Ctrl Pts',(0.304554434999943,15.2,-10.453385218));
#153690=CARTESIAN_POINT('Ctrl Pts',(0.304554434999943,11.6,-10.453385218));
#153691=CARTESIAN_POINT('Ctrl Pts',(0.304827565999943,15.2,-10.454869375));
#153692=CARTESIAN_POINT('Ctrl Pts',(0.304827565999943,11.6,-10.454869375));
#153693=CARTESIAN_POINT('Ctrl Pts',(0.305103568999944,15.2,-10.456361208));
#153694=CARTESIAN_POINT('Ctrl Pts',(0.305103568999944,11.6,-10.456361208));
#153695=CARTESIAN_POINT('Ctrl Pts',(0.305382456999944,15.2,-10.457860694));
#153696=CARTESIAN_POINT('Ctrl Pts',(0.305382456999944,11.6,-10.457860694));
#153697=CARTESIAN_POINT('Ctrl Pts',(0.305664239999944,15.2,-10.459367814));
#153698=CARTESIAN_POINT('Ctrl Pts',(0.305664239999944,11.6,-10.459367814));
#153699=CARTESIAN_POINT('Ctrl Pts',(0.305948927999945,15.2,-10.460882546));
#153700=CARTESIAN_POINT('Ctrl Pts',(0.305948927999945,11.6,-10.460882546));
#153701=CARTESIAN_POINT('Ctrl Pts',(0.306236529999945,15.2,-10.462404866));
#153702=CARTESIAN_POINT('Ctrl Pts',(0.306236529999945,11.6,-10.462404866));
#153703=CARTESIAN_POINT('Ctrl Pts',(0.306527057999944,15.2,-10.463934755));
#153704=CARTESIAN_POINT('Ctrl Pts',(0.306527057999944,11.6,-10.463934755));
#153705=CARTESIAN_POINT('Ctrl Pts',(0.306820520999944,15.2,-10.46547219));
#153706=CARTESIAN_POINT('Ctrl Pts',(0.306820520999944,11.6,-10.46547219));
#153707=CARTESIAN_POINT('Ctrl Pts',(0.307116928999944,15.2,-10.46701715));
#153708=CARTESIAN_POINT('Ctrl Pts',(0.307116928999944,11.6,-10.46701715));
#153709=CARTESIAN_POINT('Ctrl Pts',(0.307416291999945,15.2,-10.468569615));
#153710=CARTESIAN_POINT('Ctrl Pts',(0.307416291999945,11.6,-10.468569615));
#153711=CARTESIAN_POINT('Ctrl Pts',(0.307718619999945,15.2,-10.470129561));
#153712=CARTESIAN_POINT('Ctrl Pts',(0.307718619999945,11.6,-10.470129561));
#153713=CARTESIAN_POINT('Ctrl Pts',(0.308023921999944,15.2,-10.47169697));
#153714=CARTESIAN_POINT('Ctrl Pts',(0.308023921999944,11.6,-10.47169697));
#153715=CARTESIAN_POINT('Ctrl Pts',(0.308332209999945,15.2,-10.473271818));
#153716=CARTESIAN_POINT('Ctrl Pts',(0.308332209999945,11.6,-10.473271818));
#153717=CARTESIAN_POINT('Ctrl Pts',(0.308643490999945,15.2,-10.474854086));
#153718=CARTESIAN_POINT('Ctrl Pts',(0.308643490999945,11.6,-10.474854086));
#153719=CARTESIAN_POINT('Ctrl Pts',(0.308957776999945,15.2,-10.476443753));
#153720=CARTESIAN_POINT('Ctrl Pts',(0.308957776999945,11.6,-10.476443753));
#153721=CARTESIAN_POINT('Ctrl Pts',(0.309275075999944,15.2,-10.478040796));
#153722=CARTESIAN_POINT('Ctrl Pts',(0.309275075999944,11.6,-10.478040796));
#153723=CARTESIAN_POINT('Ctrl Pts',(0.309595398999944,15.2,-10.479645198));
#153724=CARTESIAN_POINT('Ctrl Pts',(0.309595398999944,11.6,-10.479645198));
#153725=CARTESIAN_POINT('Ctrl Pts',(0.309918754999944,15.2,-10.481256934));
#153726=CARTESIAN_POINT('Ctrl Pts',(0.309918754999944,11.6,-10.481256934));
#153727=CARTESIAN_POINT('Ctrl Pts',(0.310245152999944,15.2,-10.482875987));
#153728=CARTESIAN_POINT('Ctrl Pts',(0.310245152999944,11.6,-10.482875987));
#153729=CARTESIAN_POINT('Ctrl Pts',(0.310574601999944,15.2,-10.484502335));
#153730=CARTESIAN_POINT('Ctrl Pts',(0.310574601999944,11.6,-10.484502335));
#153731=CARTESIAN_POINT('Ctrl Pts',(0.310907112999944,15.2,-10.486135957));
#153732=CARTESIAN_POINT('Ctrl Pts',(0.310907112999944,11.6,-10.486135957));
#153733=CARTESIAN_POINT('Ctrl Pts',(0.311242694999944,15.2,-10.487776833));
#153734=CARTESIAN_POINT('Ctrl Pts',(0.311242694999944,11.6,-10.487776833));
#153735=CARTESIAN_POINT('Ctrl Pts',(0.311581355999945,15.2,-10.489424943));
#153736=CARTESIAN_POINT('Ctrl Pts',(0.311581355999945,11.6,-10.489424943));
#153737=CARTESIAN_POINT('Ctrl Pts',(0.311923106999944,15.2,-10.491080266));
#153738=CARTESIAN_POINT('Ctrl Pts',(0.311923106999944,11.6,-10.491080266));
#153739=CARTESIAN_POINT('Ctrl Pts',(0.312267955999944,15.2,-10.492742782));
#153740=CARTESIAN_POINT('Ctrl Pts',(0.312267955999944,11.6,-10.492742782));
#153741=CARTESIAN_POINT('Ctrl Pts',(0.312615911999944,15.2,-10.494412473));
#153742=CARTESIAN_POINT('Ctrl Pts',(0.312615911999944,11.6,-10.494412473));
#153743=CARTESIAN_POINT('Ctrl Pts',(0.312966985999944,15.2,-10.496089316));
#153744=CARTESIAN_POINT('Ctrl Pts',(0.312966985999944,11.6,-10.496089316));
#153745=CARTESIAN_POINT('Ctrl Pts',(0.313321185999945,15.2,-10.497773293));
#153746=CARTESIAN_POINT('Ctrl Pts',(0.313321185999945,11.6,-10.497773293));
#153747=CARTESIAN_POINT('Ctrl Pts',(0.313678518999945,15.2,-10.499464382));
#153748=CARTESIAN_POINT('Ctrl Pts',(0.313678518999945,11.6,-10.499464382));
#153749=CARTESIAN_POINT('Ctrl Pts',(0.314038995999945,15.2,-10.501162565));
#153750=CARTESIAN_POINT('Ctrl Pts',(0.314038995999945,11.6,-10.501162565));
#153751=CARTESIAN_POINT('Ctrl Pts',(0.314402626999944,15.2,-10.502867822));
#153752=CARTESIAN_POINT('Ctrl Pts',(0.314402626999944,11.6,-10.502867822));
#153753=CARTESIAN_POINT('Ctrl Pts',(0.314769418999944,15.2,-10.504580133));
#153754=CARTESIAN_POINT('Ctrl Pts',(0.314769418999944,11.6,-10.504580133));
#153755=CARTESIAN_POINT('Ctrl Pts',(0.315139380999945,15.2,-10.506299478));
#153756=CARTESIAN_POINT('Ctrl Pts',(0.315139380999945,11.6,-10.506299478));
#153757=CARTESIAN_POINT('Ctrl Pts',(0.315512523999945,15.2,-10.508025838));
#153758=CARTESIAN_POINT('Ctrl Pts',(0.315512523999945,11.6,-10.508025838));
#153759=CARTESIAN_POINT('Ctrl Pts',(0.315888853999944,15.2,-10.509759194));
#153760=CARTESIAN_POINT('Ctrl Pts',(0.315888853999944,11.6,-10.509759194));
#153761=CARTESIAN_POINT('Ctrl Pts',(0.316268379999943,15.2,-10.511499525));
#153762=CARTESIAN_POINT('Ctrl Pts',(0.316268379999943,11.6,-10.511499525));
#153763=CARTESIAN_POINT('Ctrl Pts',(0.316651111999944,15.2,-10.513246812));
#153764=CARTESIAN_POINT('Ctrl Pts',(0.316651111999944,11.6,-10.513246812));
#153765=CARTESIAN_POINT('Ctrl Pts',(0.317037058999944,15.2,-10.515001037));
#153766=CARTESIAN_POINT('Ctrl Pts',(0.317037058999944,11.6,-10.515001037));
#153767=CARTESIAN_POINT('Ctrl Pts',(0.317426227999944,15.2,-10.516762179));
#153768=CARTESIAN_POINT('Ctrl Pts',(0.317426227999944,11.6,-10.516762179));
#153769=CARTESIAN_POINT('Ctrl Pts',(0.317818627999945,15.2,-10.518530222));
#153770=CARTESIAN_POINT('Ctrl Pts',(0.317818627999945,11.6,-10.518530222));
#153771=CARTESIAN_POINT('Ctrl Pts',(0.318214267999943,15.2,-10.520305143));
#153772=CARTESIAN_POINT('Ctrl Pts',(0.318214267999943,11.6,-10.520305143));
#153773=CARTESIAN_POINT('Ctrl Pts',(0.318613155999945,15.2,-10.522086924));
#153774=CARTESIAN_POINT('Ctrl Pts',(0.318613155999945,11.6,-10.522086924));
#153775=CARTESIAN_POINT('Ctrl Pts',(0.319015301999944,15.2,-10.523875548));
#153776=CARTESIAN_POINT('Ctrl Pts',(0.319015301999944,11.6,-10.523875548));
#153777=CARTESIAN_POINT('Ctrl Pts',(0.319420711999945,15.2,-10.525670994));
#153778=CARTESIAN_POINT('Ctrl Pts',(0.319420711999945,11.6,-10.525670994));
#153779=CARTESIAN_POINT('Ctrl Pts',(0.319829394999944,15.2,-10.527473244));
#153780=CARTESIAN_POINT('Ctrl Pts',(0.319829394999944,11.6,-10.527473244));
#153781=CARTESIAN_POINT('Ctrl Pts',(0.320241359999944,15.2,-10.529282279));
#153782=CARTESIAN_POINT('Ctrl Pts',(0.320241359999944,11.6,-10.529282279));
#153783=CARTESIAN_POINT('Ctrl Pts',(0.320656615999945,15.2,-10.53109808));
#153784=CARTESIAN_POINT('Ctrl Pts',(0.320656615999945,11.6,-10.53109808));
#153785=CARTESIAN_POINT('Ctrl Pts',(0.321075168999944,15.2,-10.532920629));
#153786=CARTESIAN_POINT('Ctrl Pts',(0.321075168999944,11.6,-10.532920629));
#153787=CARTESIAN_POINT('Ctrl Pts',(0.321497027999945,15.2,-10.534749907));
#153788=CARTESIAN_POINT('Ctrl Pts',(0.321497027999945,11.6,-10.534749907));
#153789=CARTESIAN_POINT('Ctrl Pts',(0.321922202999945,15.2,-10.536585896));
#153790=CARTESIAN_POINT('Ctrl Pts',(0.321922202999945,11.6,-10.536585896));
#153791=CARTESIAN_POINT('Ctrl Pts',(0.322350699999945,15.2,-10.538428576));
#153792=CARTESIAN_POINT('Ctrl Pts',(0.322350699999945,11.6,-10.538428576));
#153793=CARTESIAN_POINT('Ctrl Pts',(0.322782527999944,15.2,-10.54027793));
#153794=CARTESIAN_POINT('Ctrl Pts',(0.322782527999944,11.6,-10.54027793));
#153795=CARTESIAN_POINT('Ctrl Pts',(0.323217693999943,15.2,-10.54213394));
#153796=CARTESIAN_POINT('Ctrl Pts',(0.323217693999943,11.6,-10.54213394));
#153797=CARTESIAN_POINT('Ctrl Pts',(0.323656205999944,15.2,-10.543996587));
#153798=CARTESIAN_POINT('Ctrl Pts',(0.323656205999944,11.6,-10.543996587));
#153799=CARTESIAN_POINT('Ctrl Pts',(0.324098074999943,15.2,-10.545865852));
#153800=CARTESIAN_POINT('Ctrl Pts',(0.324098074999943,11.6,-10.545865852));
#153801=CARTESIAN_POINT('Ctrl Pts',(0.324543303999943,15.2,-10.547741717));
#153802=CARTESIAN_POINT('Ctrl Pts',(0.324543303999943,11.6,-10.547741717));
#153803=CARTESIAN_POINT('Ctrl Pts',(0.324991904999944,15.2,-10.549624165));
#153804=CARTESIAN_POINT('Ctrl Pts',(0.324991904999944,11.6,-10.549624165));
#153805=CARTESIAN_POINT('Ctrl Pts',(0.325443882999944,15.2,-10.551513176));
#153806=CARTESIAN_POINT('Ctrl Pts',(0.325443882999944,11.6,-10.551513176));
#153807=CARTESIAN_POINT('Ctrl Pts',(0.325899247999945,15.2,-10.553408734));
#153808=CARTESIAN_POINT('Ctrl Pts',(0.325899247999945,11.6,-10.553408734));
#153809=CARTESIAN_POINT('Ctrl Pts',(0.326358006999945,15.2,-10.555310821));
#153810=CARTESIAN_POINT('Ctrl Pts',(0.326358006999945,11.6,-10.555310821));
#153811=CARTESIAN_POINT('Ctrl Pts',(0.326820166999945,15.2,-10.557219417));
#153812=CARTESIAN_POINT('Ctrl Pts',(0.326820166999945,11.6,-10.557219417));
#153813=CARTESIAN_POINT('Ctrl Pts',(0.327285734999944,15.2,-10.559134506));
#153814=CARTESIAN_POINT('Ctrl Pts',(0.327285734999944,11.6,-10.559134506));
#153815=CARTESIAN_POINT('Ctrl Pts',(0.327754721999945,15.2,-10.56105607));
#153816=CARTESIAN_POINT('Ctrl Pts',(0.327754721999945,11.6,-10.56105607));
#153817=CARTESIAN_POINT('Ctrl Pts',(0.328227131999944,15.2,-10.562984091));
#153818=CARTESIAN_POINT('Ctrl Pts',(0.328227131999944,11.6,-10.562984091));
#153819=CARTESIAN_POINT('Ctrl Pts',(0.328702974999944,15.2,-10.56491855));
#153820=CARTESIAN_POINT('Ctrl Pts',(0.328702974999944,11.6,-10.56491855));
#153821=CARTESIAN_POINT('Ctrl Pts',(0.329182255999945,15.2,-10.566859432));
#153822=CARTESIAN_POINT('Ctrl Pts',(0.329182255999945,11.6,-10.566859432));
#153823=CARTESIAN_POINT('Ctrl Pts',(0.329664984999944,15.2,-10.568806718));
#153824=CARTESIAN_POINT('Ctrl Pts',(0.329664984999944,11.6,-10.568806718));
#153825=CARTESIAN_POINT('Ctrl Pts',(0.330151167999944,15.2,-10.57076039));
#153826=CARTESIAN_POINT('Ctrl Pts',(0.330151167999944,11.6,-10.57076039));
#153827=CARTESIAN_POINT('Ctrl Pts',(0.330640813999944,15.2,-10.572720431));
#153828=CARTESIAN_POINT('Ctrl Pts',(0.330640813999944,11.6,-10.572720431));
#153829=CARTESIAN_POINT('Ctrl Pts',(0.331133927999945,15.2,-10.574686823));
#153830=CARTESIAN_POINT('Ctrl Pts',(0.331133927999945,11.6,-10.574686823));
#153831=CARTESIAN_POINT('Ctrl Pts',(0.331630518999945,15.2,-10.57665955));
#153832=CARTESIAN_POINT('Ctrl Pts',(0.331630518999945,11.6,-10.57665955));
#153833=CARTESIAN_POINT('Ctrl Pts',(0.332130593999944,15.2,-10.578638595));
#153834=CARTESIAN_POINT('Ctrl Pts',(0.332130593999944,11.6,-10.578638595));
#153835=CARTESIAN_POINT('Ctrl Pts',(0.332634160999945,15.2,-10.580623937));
#153836=CARTESIAN_POINT('Ctrl Pts',(0.332634160999945,11.6,-10.580623937));
#153837=CARTESIAN_POINT('Ctrl Pts',(0.333141224999943,15.2,-10.582615564));
#153838=CARTESIAN_POINT('Ctrl Pts',(0.333141224999943,11.6,-10.582615564));
#153839=CARTESIAN_POINT('Ctrl Pts',(0.333651795999945,15.2,-10.584613455));
#153840=CARTESIAN_POINT('Ctrl Pts',(0.333651795999945,11.6,-10.584613455));
#153841=CARTESIAN_POINT('Ctrl Pts',(0.334165878999944,15.2,-10.586617594));
#153842=CARTESIAN_POINT('Ctrl Pts',(0.334165878999944,11.6,-10.586617594));
#153843=CARTESIAN_POINT('Ctrl Pts',(0.334683482999945,15.2,-10.588627965));
#153844=CARTESIAN_POINT('Ctrl Pts',(0.334683482999945,11.6,-10.588627965));
#153845=CARTESIAN_POINT('Ctrl Pts',(0.335204611999943,15.2,-10.59064455));
#153846=CARTESIAN_POINT('Ctrl Pts',(0.335204611999943,11.6,-10.59064455));
#153847=CARTESIAN_POINT('Ctrl Pts',(0.335729277999944,15.2,-10.592667332));
#153848=CARTESIAN_POINT('Ctrl Pts',(0.335729277999944,11.6,-10.592667332));
#153849=CARTESIAN_POINT('Ctrl Pts',(0.336257482999944,15.2,-10.594696293));
#153850=CARTESIAN_POINT('Ctrl Pts',(0.336257482999944,11.6,-10.594696293));
#153851=CARTESIAN_POINT('Ctrl Pts',(0.336789236999945,15.2,-10.59673142));
#153852=CARTESIAN_POINT('Ctrl Pts',(0.336789236999945,11.6,-10.59673142));
#153853=CARTESIAN_POINT('Ctrl Pts',(0.337324545999945,15.2,-10.598772692));
#153854=CARTESIAN_POINT('Ctrl Pts',(0.337324545999945,11.6,-10.598772692));
#153855=CARTESIAN_POINT('Ctrl Pts',(0.337863417999945,15.2,-10.600820093));
#153856=CARTESIAN_POINT('Ctrl Pts',(0.337863417999945,11.6,-10.600820093));
#153857=CARTESIAN_POINT('Ctrl Pts',(0.338405857999945,15.2,-10.602873609));
#153858=CARTESIAN_POINT('Ctrl Pts',(0.338405857999945,11.6,-10.602873609));
#153859=CARTESIAN_POINT('Ctrl Pts',(0.338951873999944,15.2,-10.60493322));
#153860=CARTESIAN_POINT('Ctrl Pts',(0.338951873999944,11.6,-10.60493322));
#153861=CARTESIAN_POINT('Ctrl Pts',(0.339501472999943,15.2,-10.606998913));
#153862=CARTESIAN_POINT('Ctrl Pts',(0.339501472999943,11.6,-10.606998913));
#153863=CARTESIAN_POINT('Ctrl Pts',(0.340054661999943,15.2,-10.609070667));
#153864=CARTESIAN_POINT('Ctrl Pts',(0.340054661999943,11.6,-10.609070667));
#153865=CARTESIAN_POINT('Ctrl Pts',(0.340611446999944,15.2,-10.611148469));
#153866=CARTESIAN_POINT('Ctrl Pts',(0.340611446999944,11.6,-10.611148469));
#153867=CARTESIAN_POINT('Ctrl Pts',(0.341171834999944,15.2,-10.613232302));
#153868=CARTESIAN_POINT('Ctrl Pts',(0.341171834999944,11.6,-10.613232302));
#153869=CARTESIAN_POINT('Ctrl Pts',(0.341735832999944,15.2,-10.615322148));
#153870=CARTESIAN_POINT('Ctrl Pts',(0.341735832999944,11.6,-10.615322148));
#153871=CARTESIAN_POINT('Ctrl Pts',(0.342303446999944,15.2,-10.617417992));
#153872=CARTESIAN_POINT('Ctrl Pts',(0.342303446999944,11.6,-10.617417992));
#153873=CARTESIAN_POINT('Ctrl Pts',(0.342874684999943,15.2,-10.619519817));
#153874=CARTESIAN_POINT('Ctrl Pts',(0.342874684999943,11.6,-10.619519817));
#153875=CARTESIAN_POINT('Ctrl Pts',(0.343449551999945,15.2,-10.621627608));
#153876=CARTESIAN_POINT('Ctrl Pts',(0.343449551999945,11.6,-10.621627608));
#153877=CARTESIAN_POINT('Ctrl Pts',(0.344028054999944,15.2,-10.623741347));
#153878=CARTESIAN_POINT('Ctrl Pts',(0.344028054999944,11.6,-10.623741347));
#153879=CARTESIAN_POINT('Ctrl Pts',(0.344610201999943,15.2,-10.625861018));
#153880=CARTESIAN_POINT('Ctrl Pts',(0.344610201999943,11.6,-10.625861018));
#153881=CARTESIAN_POINT('Ctrl Pts',(0.345195997999944,15.2,-10.627986606));
#153882=CARTESIAN_POINT('Ctrl Pts',(0.345195997999944,11.6,-10.627986606));
#153883=CARTESIAN_POINT('Ctrl Pts',(0.345785448999945,15.2,-10.630118095));
#153884=CARTESIAN_POINT('Ctrl Pts',(0.345785448999945,11.6,-10.630118095));
#153885=CARTESIAN_POINT('Ctrl Pts',(0.346378563999944,15.2,-10.632255468));
#153886=CARTESIAN_POINT('Ctrl Pts',(0.346378563999944,11.6,-10.632255468));
#153887=CARTESIAN_POINT('Ctrl Pts',(0.346975346999944,15.2,-10.634398708));
#153888=CARTESIAN_POINT('Ctrl Pts',(0.346975346999944,11.6,-10.634398708));
#153889=CARTESIAN_POINT('Ctrl Pts',(0.347575804999943,15.2,-10.636547803));
#153890=CARTESIAN_POINT('Ctrl Pts',(0.347575804999943,11.6,-10.636547803));
#153891=CARTESIAN_POINT('Ctrl Pts',(0.348179944999943,15.2,-10.638702732));
#153892=CARTESIAN_POINT('Ctrl Pts',(0.348179944999943,11.6,-10.638702732));
#153893=CARTESIAN_POINT('Ctrl Pts',(0.348787772999944,15.2,-10.640863483));
#153894=CARTESIAN_POINT('Ctrl Pts',(0.348787772999944,11.6,-10.640863483));
#153895=CARTESIAN_POINT('Ctrl Pts',(0.349399294999945,15.2,-10.643030038));
#153896=CARTESIAN_POINT('Ctrl Pts',(0.349399294999945,11.6,-10.643030038));
#153897=CARTESIAN_POINT('Ctrl Pts',(0.350014516999944,15.2,-10.645202383));
#153898=CARTESIAN_POINT('Ctrl Pts',(0.350014516999944,11.6,-10.645202383));
#153899=CARTESIAN_POINT('Ctrl Pts',(0.350633445999945,15.2,-10.647380501));
#153900=CARTESIAN_POINT('Ctrl Pts',(0.350633445999945,11.6,-10.647380501));
#153901=CARTESIAN_POINT('Ctrl Pts',(0.351256087999945,15.2,-10.649564376));
#153902=CARTESIAN_POINT('Ctrl Pts',(0.351256087999945,11.6,-10.649564376));
#153903=CARTESIAN_POINT('Ctrl Pts',(0.351882449999945,15.2,-10.651753993));
#153904=CARTESIAN_POINT('Ctrl Pts',(0.351882449999945,11.6,-10.651753993));
#153905=CARTESIAN_POINT('Ctrl Pts',(0.352512535999944,15.2,-10.653949337));
#153906=CARTESIAN_POINT('Ctrl Pts',(0.352512535999944,11.6,-10.653949337));
#153907=CARTESIAN_POINT('Ctrl Pts',(0.353146353999945,15.2,-10.656150391));
#153908=CARTESIAN_POINT('Ctrl Pts',(0.353146353999945,11.6,-10.656150391));
#153909=CARTESIAN_POINT('Ctrl Pts',(0.353783908999944,15.2,-10.658357141));
#153910=CARTESIAN_POINT('Ctrl Pts',(0.353783908999944,11.6,-10.658357141));
#153911=CARTESIAN_POINT('Ctrl Pts',(0.354425208999943,15.2,-10.660569571));
#153912=CARTESIAN_POINT('Ctrl Pts',(0.354425208999943,11.6,-10.660569571));
#153913=CARTESIAN_POINT('Ctrl Pts',(0.355070257999944,15.2,-10.662787664));
#153914=CARTESIAN_POINT('Ctrl Pts',(0.355070257999944,11.6,-10.662787664));
#153915=CARTESIAN_POINT('Ctrl Pts',(0.355719062999944,15.2,-10.665011407));
#153916=CARTESIAN_POINT('Ctrl Pts',(0.355719062999944,11.6,-10.665011407));
#153917=CARTESIAN_POINT('Ctrl Pts',(0.356371629999943,15.2,-10.667240784));
#153918=CARTESIAN_POINT('Ctrl Pts',(0.356371629999943,11.6,-10.667240784));
#153919=CARTESIAN_POINT('Ctrl Pts',(0.357027963999944,15.2,-10.669475778));
#153920=CARTESIAN_POINT('Ctrl Pts',(0.357027963999944,11.6,-10.669475778));
#153921=CARTESIAN_POINT('Ctrl Pts',(0.357688070999943,15.2,-10.671716375));
#153922=CARTESIAN_POINT('Ctrl Pts',(0.357688070999943,11.6,-10.671716375));
#153923=CARTESIAN_POINT('Ctrl Pts',(0.358351957999944,15.2,-10.673962561));
#153924=CARTESIAN_POINT('Ctrl Pts',(0.358351957999944,11.6,-10.673962561));
#153925=CARTESIAN_POINT('Ctrl Pts',(0.359019631999944,15.2,-10.676214319));
#153926=CARTESIAN_POINT('Ctrl Pts',(0.359019631999944,11.6,-10.676214319));
#153927=CARTESIAN_POINT('Ctrl Pts',(0.359691094999944,15.2,-10.678471635));
#153928=CARTESIAN_POINT('Ctrl Pts',(0.359691094999944,11.6,-10.678471635));
#153929=CARTESIAN_POINT('Ctrl Pts',(0.360366356999944,15.2,-10.680734493));
#153930=CARTESIAN_POINT('Ctrl Pts',(0.360366356999944,11.6,-10.680734493));
#153931=CARTESIAN_POINT('Ctrl Pts',(0.361045420999944,15.2,-10.683002879));
#153932=CARTESIAN_POINT('Ctrl Pts',(0.361045420999944,11.6,-10.683002879));
#153933=CARTESIAN_POINT('Ctrl Pts',(0.361728292999944,15.2,-10.685276775));
#153934=CARTESIAN_POINT('Ctrl Pts',(0.361728292999944,11.6,-10.685276775));
#153935=CARTESIAN_POINT('Ctrl Pts',(0.362414979999944,15.2,-10.687556171));
#153936=CARTESIAN_POINT('Ctrl Pts',(0.362414979999944,11.6,-10.687556171));
#153937=CARTESIAN_POINT('Ctrl Pts',(0.363105486999944,15.2,-10.689841047));
#153938=CARTESIAN_POINT('Ctrl Pts',(0.363105486999944,11.6,-10.689841047));
#153939=CARTESIAN_POINT('Ctrl Pts',(0.363799819999944,15.2,-10.692131392));
#153940=CARTESIAN_POINT('Ctrl Pts',(0.363799819999944,11.6,-10.692131392));
#153941=CARTESIAN_POINT('Ctrl Pts',(0.364497983999945,15.2,-10.69442719));
#153942=CARTESIAN_POINT('Ctrl Pts',(0.364497983999945,11.6,-10.69442719));
#153943=CARTESIAN_POINT('Ctrl Pts',(0.365199985999943,15.2,-10.696728424));
#153944=CARTESIAN_POINT('Ctrl Pts',(0.365199985999943,11.6,-10.696728424));
#153945=CARTESIAN_POINT('Ctrl Pts',(0.365905829999944,15.2,-10.699035082));
#153946=CARTESIAN_POINT('Ctrl Pts',(0.365905829999944,11.6,-10.699035082));
#153947=CARTESIAN_POINT('Ctrl Pts',(0.366615521999943,15.2,-10.701347148));
#153948=CARTESIAN_POINT('Ctrl Pts',(0.366615521999943,11.6,-10.701347148));
#153949=CARTESIAN_POINT('Ctrl Pts',(0.367329068999943,15.2,-10.703664607));
#153950=CARTESIAN_POINT('Ctrl Pts',(0.367329068999943,11.6,-10.703664607));
#153951=CARTESIAN_POINT('Ctrl Pts',(0.368046474999945,15.2,-10.705987445));
#153952=CARTESIAN_POINT('Ctrl Pts',(0.368046474999945,11.6,-10.705987445));
#153953=CARTESIAN_POINT('Ctrl Pts',(0.368767745999945,15.2,-10.708315648));
#153954=CARTESIAN_POINT('Ctrl Pts',(0.368767745999945,11.6,-10.708315648));
#153955=CARTESIAN_POINT('Ctrl Pts',(0.369492886999945,15.2,-10.710649199));
#153956=CARTESIAN_POINT('Ctrl Pts',(0.369492886999945,11.6,-10.710649199));
#153957=CARTESIAN_POINT('Ctrl Pts',(0.370221902999944,15.2,-10.712988086));
#153958=CARTESIAN_POINT('Ctrl Pts',(0.370221902999944,11.6,-10.712988086));
#153959=CARTESIAN_POINT('Ctrl Pts',(0.370954801999943,15.2,-10.715332293));
#153960=CARTESIAN_POINT('Ctrl Pts',(0.370954801999943,11.6,-10.715332293));
#153961=CARTESIAN_POINT('Ctrl Pts',(0.371691585999944,15.2,-10.717681807));
#153962=CARTESIAN_POINT('Ctrl Pts',(0.371691585999944,11.6,-10.717681807));
#153963=CARTESIAN_POINT('Ctrl Pts',(0.372432262999943,15.2,-10.720036612));
#153964=CARTESIAN_POINT('Ctrl Pts',(0.372432262999943,11.6,-10.720036612));
#153965=CARTESIAN_POINT('Ctrl Pts',(0.373176837999944,15.2,-10.722396693));
#153966=CARTESIAN_POINT('Ctrl Pts',(0.373176837999944,11.6,-10.722396693));
#153967=CARTESIAN_POINT('Ctrl Pts',(0.373925314999944,15.2,-10.724762038));
#153968=CARTESIAN_POINT('Ctrl Pts',(0.373925314999944,11.6,-10.724762038));
#153969=CARTESIAN_POINT('Ctrl Pts',(0.374677699999945,15.2,-10.72713263));
#153970=CARTESIAN_POINT('Ctrl Pts',(0.374677699999945,11.6,-10.72713263));
#153971=CARTESIAN_POINT('Ctrl Pts',(0.375433997999943,15.2,-10.729508457));
#153972=CARTESIAN_POINT('Ctrl Pts',(0.375433997999943,11.6,-10.729508457));
#153973=CARTESIAN_POINT('Ctrl Pts',(0.376194214999943,15.2,-10.731889504));
#153974=CARTESIAN_POINT('Ctrl Pts',(0.376194214999943,11.6,-10.731889504));
#153975=CARTESIAN_POINT('Ctrl Pts',(0.376958354999944,15.2,-10.734275757));
#153976=CARTESIAN_POINT('Ctrl Pts',(0.376958354999944,11.6,-10.734275757));
#153977=CARTESIAN_POINT('Ctrl Pts',(0.377726424999943,15.2,-10.7366672));
#153978=CARTESIAN_POINT('Ctrl Pts',(0.377726424999943,11.6,-10.7366672));
#153979=CARTESIAN_POINT('Ctrl Pts',(0.378498428999944,15.2,-10.73906382));
#153980=CARTESIAN_POINT('Ctrl Pts',(0.378498428999944,11.6,-10.73906382));
#153981=CARTESIAN_POINT('Ctrl Pts',(0.379274372999945,15.2,-10.741465604));
#153982=CARTESIAN_POINT('Ctrl Pts',(0.379274372999945,11.6,-10.741465604));
#153983=CARTESIAN_POINT('Ctrl Pts',(0.380054259999945,15.2,-10.743872536));
#153984=CARTESIAN_POINT('Ctrl Pts',(0.380054259999945,11.6,-10.743872536));
#153985=CARTESIAN_POINT('Ctrl Pts',(0.380838096999945,15.2,-10.746284604));
#153986=CARTESIAN_POINT('Ctrl Pts',(0.380838096999945,11.6,-10.746284604));
#153987=CARTESIAN_POINT('Ctrl Pts',(0.381625889999944,15.2,-10.748701792));
#153988=CARTESIAN_POINT('Ctrl Pts',(0.381625889999944,11.6,-10.748701792));
#153989=CARTESIAN_POINT('Ctrl Pts',(0.382417640999944,15.2,-10.751124087));
#153990=CARTESIAN_POINT('Ctrl Pts',(0.382417640999944,11.6,-10.751124087));
#153991=CARTESIAN_POINT('Ctrl Pts',(0.383213356999944,15.2,-10.753551475));
#153992=CARTESIAN_POINT('Ctrl Pts',(0.383213356999944,11.6,-10.753551475));
#153993=CARTESIAN_POINT('Ctrl Pts',(0.384013043999945,15.2,-10.755983942));
#153994=CARTESIAN_POINT('Ctrl Pts',(0.384013043999945,11.6,-10.755983942));
#153995=CARTESIAN_POINT('Ctrl Pts',(0.384816703999944,15.2,-10.758421474));
#153996=CARTESIAN_POINT('Ctrl Pts',(0.384816703999944,11.6,-10.758421474));
#153997=CARTESIAN_POINT('Ctrl Pts',(0.385624345999943,15.2,-10.760864057));
#153998=CARTESIAN_POINT('Ctrl Pts',(0.385624345999943,11.6,-10.760864057));
#153999=CARTESIAN_POINT('Ctrl Pts',(0.386435970999944,15.2,-10.763311678));
#154000=CARTESIAN_POINT('Ctrl Pts',(0.386435970999944,11.6,-10.763311678));
#154001=CARTESIAN_POINT('Ctrl Pts',(0.387251585999945,15.2,-10.765764322));
#154002=CARTESIAN_POINT('Ctrl Pts',(0.387251585999945,11.6,-10.765764322));
#154003=CARTESIAN_POINT('Ctrl Pts',(0.388071194999944,15.2,-10.768221976));
#154004=CARTESIAN_POINT('Ctrl Pts',(0.388071194999944,11.6,-10.768221976));
#154005=CARTESIAN_POINT('Ctrl Pts',(0.388894804999945,15.2,-10.770684626));
#154006=CARTESIAN_POINT('Ctrl Pts',(0.388894804999945,11.6,-10.770684626));
#154007=CARTESIAN_POINT('Ctrl Pts',(0.389722417999945,15.2,-10.773152259));
#154008=CARTESIAN_POINT('Ctrl Pts',(0.389722417999945,11.6,-10.773152259));
#154009=CARTESIAN_POINT('Ctrl Pts',(0.390554040999945,15.2,-10.77562486));
#154010=CARTESIAN_POINT('Ctrl Pts',(0.390554040999945,11.6,-10.77562486));
#154011=CARTESIAN_POINT('Ctrl Pts',(0.391389675999945,15.2,-10.778102417));
#154012=CARTESIAN_POINT('Ctrl Pts',(0.391389675999945,11.6,-10.778102417));
#154013=CARTESIAN_POINT('Ctrl Pts',(0.392229331999945,15.2,-10.780584915));
#154014=CARTESIAN_POINT('Ctrl Pts',(0.392229331999945,11.6,-10.780584915));
#154015=CARTESIAN_POINT('Ctrl Pts',(0.393073008999943,15.2,-10.78307234));
#154016=CARTESIAN_POINT('Ctrl Pts',(0.393073008999943,11.6,-10.78307234));
#154017=CARTESIAN_POINT('Ctrl Pts',(0.393920715999944,15.2,-10.785564681));
#154018=CARTESIAN_POINT('Ctrl Pts',(0.393920715999944,11.6,-10.785564681));
#154019=CARTESIAN_POINT('Ctrl Pts',(0.394772454999943,15.2,-10.788061922));
#154020=CARTESIAN_POINT('Ctrl Pts',(0.394772454999943,11.6,-10.788061922));
#154021=CARTESIAN_POINT('Ctrl Pts',(0.395628231999944,15.2,-10.790564051));
#154022=CARTESIAN_POINT('Ctrl Pts',(0.395628231999944,11.6,-10.790564051));
#154023=CARTESIAN_POINT('Ctrl Pts',(0.396488050999944,15.2,-10.793071054));
#154024=CARTESIAN_POINT('Ctrl Pts',(0.396488050999944,11.6,-10.793071054));
#154025=CARTESIAN_POINT('Ctrl Pts',(0.397351916999943,15.2,-10.795582918));
#154026=CARTESIAN_POINT('Ctrl Pts',(0.397351916999943,11.6,-10.795582918));
#154027=CARTESIAN_POINT('Ctrl Pts',(0.398219834999944,15.2,-10.798099629));
#154028=CARTESIAN_POINT('Ctrl Pts',(0.398219834999944,11.6,-10.798099629));
#154029=CARTESIAN_POINT('Ctrl Pts',(0.399091808999945,15.2,-10.800621174));
#154030=CARTESIAN_POINT('Ctrl Pts',(0.399091808999945,11.6,-10.800621174));
#154031=CARTESIAN_POINT('Ctrl Pts',(0.399967842999944,15.2,-10.80314754));
#154032=CARTESIAN_POINT('Ctrl Pts',(0.399967842999944,11.6,-10.80314754));
#154033=CARTESIAN_POINT('Ctrl Pts',(0.400847942999943,15.2,-10.805678712));
#154034=CARTESIAN_POINT('Ctrl Pts',(0.400847942999943,11.6,-10.805678712));
#154035=CARTESIAN_POINT('Ctrl Pts',(0.401732111999945,15.2,-10.808214679));
#154036=CARTESIAN_POINT('Ctrl Pts',(0.401732111999945,11.6,-10.808214679));
#154037=CARTESIAN_POINT('Ctrl Pts',(0.402620355999943,15.2,-10.810755427));
#154038=CARTESIAN_POINT('Ctrl Pts',(0.402620355999943,11.6,-10.810755427));
#154039=CARTESIAN_POINT('Ctrl Pts',(0.403512678999943,15.2,-10.813300943));
#154040=CARTESIAN_POINT('Ctrl Pts',(0.403512678999943,11.6,-10.813300943));
#154041=CARTESIAN_POINT('Ctrl Pts',(0.404409085999945,15.2,-10.815851213));
#154042=CARTESIAN_POINT('Ctrl Pts',(0.404409085999945,11.6,-10.815851213));
#154043=CARTESIAN_POINT('Ctrl Pts',(0.405309579999944,15.2,-10.818406225));
#154044=CARTESIAN_POINT('Ctrl Pts',(0.405309579999944,11.6,-10.818406225));
#154045=CARTESIAN_POINT('Ctrl Pts',(0.406214165999945,15.2,-10.820965964));
#154046=CARTESIAN_POINT('Ctrl Pts',(0.406214165999945,11.6,-10.820965964));
#154047=CARTESIAN_POINT('Ctrl Pts',(0.407122848999943,15.2,-10.82353042));
#154048=CARTESIAN_POINT('Ctrl Pts',(0.407122848999943,11.6,-10.82353042));
#154049=CARTESIAN_POINT('Ctrl Pts',(0.408035631999945,15.2,-10.826099577));
#154050=CARTESIAN_POINT('Ctrl Pts',(0.408035631999945,11.6,-10.826099577));
#154051=CARTESIAN_POINT('Ctrl Pts',(0.408952521999945,15.2,-10.828673424));
#154052=CARTESIAN_POINT('Ctrl Pts',(0.408952521999945,11.6,-10.828673424));
#154053=CARTESIAN_POINT('Ctrl Pts',(0.409873521999945,15.2,-10.831251946));
#154054=CARTESIAN_POINT('Ctrl Pts',(0.409873521999945,11.6,-10.831251946));
#154055=CARTESIAN_POINT('Ctrl Pts',(0.410798634999944,15.2,-10.833835132));
#154056=CARTESIAN_POINT('Ctrl Pts',(0.410798634999944,11.6,-10.833835132));
#154057=CARTESIAN_POINT('Ctrl Pts',(0.411727865999945,15.2,-10.836422969));
#154058=CARTESIAN_POINT('Ctrl Pts',(0.411727865999945,11.6,-10.836422969));
#154059=CARTESIAN_POINT('Ctrl Pts',(0.412661221999944,15.2,-10.839015443));
#154060=CARTESIAN_POINT('Ctrl Pts',(0.412661221999944,11.6,-10.839015443));
#154061=CARTESIAN_POINT('Ctrl Pts',(0.413598702999943,15.2,-10.841612542));
#154062=CARTESIAN_POINT('Ctrl Pts',(0.413598702999943,11.6,-10.841612542));
#154063=CARTESIAN_POINT('Ctrl Pts',(0.414540315999944,15.2,-10.844214253));
#154064=CARTESIAN_POINT('Ctrl Pts',(0.414540315999944,11.6,-10.844214253));
#154065=CARTESIAN_POINT('Ctrl Pts',(0.415486064999945,15.2,-10.846820562));
#154066=CARTESIAN_POINT('Ctrl Pts',(0.415486064999945,11.6,-10.846820562));
#154067=CARTESIAN_POINT('Ctrl Pts',(0.416435952999944,15.2,-10.849431457));
#154068=CARTESIAN_POINT('Ctrl Pts',(0.416435952999944,11.6,-10.849431457));
#154069=CARTESIAN_POINT('Ctrl Pts',(0.417389984999945,15.2,-10.852046927));
#154070=CARTESIAN_POINT('Ctrl Pts',(0.417389984999945,11.6,-10.852046927));
#154071=CARTESIAN_POINT('Ctrl Pts',(0.418348164999944,15.2,-10.854666958));
#154072=CARTESIAN_POINT('Ctrl Pts',(0.418348164999944,11.6,-10.854666958));
#154073=CARTESIAN_POINT('Ctrl Pts',(0.419310496999945,15.2,-10.857291535));
#154074=CARTESIAN_POINT('Ctrl Pts',(0.419310496999945,11.6,-10.857291535));
#154075=CARTESIAN_POINT('Ctrl Pts',(0.420276985999944,15.2,-10.859920649));
#154076=CARTESIAN_POINT('Ctrl Pts',(0.420276985999944,11.6,-10.859920649));
#154077=CARTESIAN_POINT('Ctrl Pts',(0.421247635999944,15.2,-10.862554285));
#154078=CARTESIAN_POINT('Ctrl Pts',(0.421247635999944,11.6,-10.862554285));
#154079=CARTESIAN_POINT('Ctrl Pts',(0.422222449999945,15.2,-10.865192432));
#154080=CARTESIAN_POINT('Ctrl Pts',(0.422222449999945,11.6,-10.865192432));
#154081=CARTESIAN_POINT('Ctrl Pts',(0.423201432999945,15.2,-10.867835076));
#154082=CARTESIAN_POINT('Ctrl Pts',(0.423201432999945,11.6,-10.867835076));
#154083=CARTESIAN_POINT('Ctrl Pts',(0.424184586999944,15.2,-10.870482205));
#154084=CARTESIAN_POINT('Ctrl Pts',(0.424184586999944,11.6,-10.870482205));
#154085=CARTESIAN_POINT('Ctrl Pts',(0.425171919999944,15.2,-10.873133806));
#154086=CARTESIAN_POINT('Ctrl Pts',(0.425171919999944,11.6,-10.873133806));
#154087=CARTESIAN_POINT('Ctrl Pts',(0.426163432999944,15.2,-10.875789868));
#154088=CARTESIAN_POINT('Ctrl Pts',(0.426163432999944,11.6,-10.875789868));
#154089=CARTESIAN_POINT('Ctrl Pts',(0.427159130999945,15.2,-10.878450378));
#154090=CARTESIAN_POINT('Ctrl Pts',(0.427159130999945,11.6,-10.878450378));
#154091=CARTESIAN_POINT('Ctrl Pts',(0.428159016999944,15.2,-10.881115322));
#154092=CARTESIAN_POINT('Ctrl Pts',(0.428159016999944,11.6,-10.881115322));
#154093=CARTESIAN_POINT('Ctrl Pts',(0.429163096999944,15.2,-10.883784689));
#154094=CARTESIAN_POINT('Ctrl Pts',(0.429163096999944,11.6,-10.883784689));
#154095=CARTESIAN_POINT('Ctrl Pts',(0.430171372999943,15.2,-10.886458467));
#154096=CARTESIAN_POINT('Ctrl Pts',(0.430171372999943,11.6,-10.886458467));
#154097=CARTESIAN_POINT('Ctrl Pts',(0.431183849999943,15.2,-10.889136642));
#154098=CARTESIAN_POINT('Ctrl Pts',(0.431183849999943,11.6,-10.889136642));
#154099=CARTESIAN_POINT('Ctrl Pts',(0.432200529999944,15.2,-10.891819203));
#154100=CARTESIAN_POINT('Ctrl Pts',(0.432200529999944,11.6,-10.891819203));
#154101=CARTESIAN_POINT('Ctrl Pts',(0.433221419999944,15.2,-10.894506138));
#154102=CARTESIAN_POINT('Ctrl Pts',(0.433221419999944,11.6,-10.894506138));
#154103=CARTESIAN_POINT('Ctrl Pts',(0.434246522999944,15.2,-10.897197434));
#154104=CARTESIAN_POINT('Ctrl Pts',(0.434246522999944,11.6,-10.897197434));
#154105=CARTESIAN_POINT('Ctrl Pts',(0.435275840999945,15.2,-10.899893077));
#154106=CARTESIAN_POINT('Ctrl Pts',(0.435275840999945,11.6,-10.899893077));
#154107=CARTESIAN_POINT('Ctrl Pts',(0.436309378999944,15.2,-10.902593058));
#154108=CARTESIAN_POINT('Ctrl Pts',(0.436309378999944,11.6,-10.902593058));
#154109=CARTESIAN_POINT('Ctrl Pts',(0.437347139999943,15.2,-10.905297364));
#154110=CARTESIAN_POINT('Ctrl Pts',(0.437347139999943,11.6,-10.905297364));
#154111=CARTESIAN_POINT('Ctrl Pts',(0.438389128999944,15.2,-10.908005981));
#154112=CARTESIAN_POINT('Ctrl Pts',(0.438389128999944,11.6,-10.908005981));
#154113=CARTESIAN_POINT('Ctrl Pts',(0.439435350999944,15.2,-10.910718898));
#154114=CARTESIAN_POINT('Ctrl Pts',(0.439435350999944,11.6,-10.910718898));
#154115=CARTESIAN_POINT('Ctrl Pts',(0.440485805999945,15.2,-10.913436104));
#154116=CARTESIAN_POINT('Ctrl Pts',(0.440485805999945,11.6,-10.913436104));
#154117=CARTESIAN_POINT('Ctrl Pts',(0.441540500999944,15.2,-10.916157585));
#154118=CARTESIAN_POINT('Ctrl Pts',(0.441540500999944,11.6,-10.916157585));
#154119=CARTESIAN_POINT('Ctrl Pts',(0.442599438999943,15.2,-10.91888333));
#154120=CARTESIAN_POINT('Ctrl Pts',(0.442599438999943,11.6,-10.91888333));
#154121=CARTESIAN_POINT('Ctrl Pts',(0.443662621999945,15.2,-10.921613326));
#154122=CARTESIAN_POINT('Ctrl Pts',(0.443662621999945,11.6,-10.921613326));
#154123=CARTESIAN_POINT('Ctrl Pts',(0.444730055999945,15.2,-10.924347562));
#154124=CARTESIAN_POINT('Ctrl Pts',(0.444730055999945,11.6,-10.924347562));
#154125=CARTESIAN_POINT('Ctrl Pts',(0.445801742999944,15.2,-10.927086026));
#154126=CARTESIAN_POINT('Ctrl Pts',(0.445801742999944,11.6,-10.927086026));
#154127=CARTESIAN_POINT('Ctrl Pts',(0.446877687999944,15.2,-10.929828706));
#154128=CARTESIAN_POINT('Ctrl Pts',(0.446877687999944,11.6,-10.929828706));
#154129=CARTESIAN_POINT('Ctrl Pts',(0.447957893999943,15.2,-10.932575589));
#154130=CARTESIAN_POINT('Ctrl Pts',(0.447957893999943,11.6,-10.932575589));
#154131=CARTESIAN_POINT('Ctrl Pts',(0.449042363999944,15.2,-10.935326664));
#154132=CARTESIAN_POINT('Ctrl Pts',(0.449042363999944,11.6,-10.935326664));
#154133=CARTESIAN_POINT('Ctrl Pts',(0.450131101999943,15.2,-10.93808192));
#154134=CARTESIAN_POINT('Ctrl Pts',(0.450131101999943,11.6,-10.93808192));
#154135=CARTESIAN_POINT('Ctrl Pts',(0.451224112999944,15.2,-10.940841343));
#154136=CARTESIAN_POINT('Ctrl Pts',(0.451224112999944,11.6,-10.940841343));
#154137=CARTESIAN_POINT('Ctrl Pts',(0.452321397999944,15.2,-10.943604921));
#154138=CARTESIAN_POINT('Ctrl Pts',(0.452321397999944,11.6,-10.943604921));
#154139=CARTESIAN_POINT('Ctrl Pts',(0.453422961999944,15.2,-10.946372645));
#154140=CARTESIAN_POINT('Ctrl Pts',(0.453422961999944,11.6,-10.946372645));
#154141=CARTESIAN_POINT('Ctrl Pts',(0.454528808999944,15.2,-10.949144502));
#154142=CARTESIAN_POINT('Ctrl Pts',(0.454528808999944,11.6,-10.949144502));
#154143=CARTESIAN_POINT('Ctrl Pts',(0.455638941999944,15.2,-10.951920478));
#154144=CARTESIAN_POINT('Ctrl Pts',(0.455638941999944,11.6,-10.951920478));
#154145=CARTESIAN_POINT('Ctrl Pts',(0.456753363999944,15.2,-10.954700564));
#154146=CARTESIAN_POINT('Ctrl Pts',(0.456753363999944,11.6,-10.954700564));
#154147=CARTESIAN_POINT('Ctrl Pts',(0.457872078999945,15.2,-10.957484747));
#154148=CARTESIAN_POINT('Ctrl Pts',(0.457872078999945,11.6,-10.957484747));
#154149=CARTESIAN_POINT('Ctrl Pts',(0.458995090999944,15.2,-10.960273016));
#154150=CARTESIAN_POINT('Ctrl Pts',(0.458995090999944,11.6,-10.960273016));
#154151=CARTESIAN_POINT('Ctrl Pts',(0.460122400999945,15.2,-10.963065359));
#154152=CARTESIAN_POINT('Ctrl Pts',(0.460122400999945,11.6,-10.963065359));
#154153=CARTESIAN_POINT('Ctrl Pts',(0.461254015999945,15.2,-10.965861764));
#154154=CARTESIAN_POINT('Ctrl Pts',(0.461254015999945,11.6,-10.965861764));
#154155=CARTESIAN_POINT('Ctrl Pts',(0.462389937999944,15.2,-10.96866222));
#154156=CARTESIAN_POINT('Ctrl Pts',(0.462389937999944,11.6,-10.96866222));
#154157=CARTESIAN_POINT('Ctrl Pts',(0.463530168999944,15.2,-10.971466714));
#154158=CARTESIAN_POINT('Ctrl Pts',(0.463530168999944,11.6,-10.971466714));
#154159=CARTESIAN_POINT('Ctrl Pts',(0.464674712999944,15.2,-10.974275237));
#154160=CARTESIAN_POINT('Ctrl Pts',(0.464674712999944,11.6,-10.974275237));
#154161=CARTESIAN_POINT('Ctrl Pts',(0.465823575999943,15.2,-10.977087774));
#154162=CARTESIAN_POINT('Ctrl Pts',(0.465823575999943,11.6,-10.977087774));
#154163=CARTESIAN_POINT('Ctrl Pts',(0.466976756999945,15.2,-10.979904316));
#154164=CARTESIAN_POINT('Ctrl Pts',(0.466976756999945,11.6,-10.979904316));
#154165=CARTESIAN_POINT('Ctrl Pts',(0.468134261999945,15.2,-10.982724852));
#154166=CARTESIAN_POINT('Ctrl Pts',(0.468134261999945,11.6,-10.982724852));
#154167=CARTESIAN_POINT('Ctrl Pts',(0.469296094999944,15.2,-10.985549368));
#154168=CARTESIAN_POINT('Ctrl Pts',(0.469296094999944,11.6,-10.985549368));
#154169=CARTESIAN_POINT('Ctrl Pts',(0.470462256999945,15.2,-10.988377854));
#154170=CARTESIAN_POINT('Ctrl Pts',(0.470462256999945,11.6,-10.988377854));
#154171=CARTESIAN_POINT('Ctrl Pts',(0.471632752999945,15.2,-10.991210298));
#154172=CARTESIAN_POINT('Ctrl Pts',(0.471632752999945,11.6,-10.991210298));
#154173=CARTESIAN_POINT('Ctrl Pts',(0.472807584999944,15.2,-10.994046689));
#154174=CARTESIAN_POINT('Ctrl Pts',(0.472807584999944,11.6,-10.994046689));
#154175=CARTESIAN_POINT('Ctrl Pts',(0.473986757999943,15.2,-10.996887016));
#154176=CARTESIAN_POINT('Ctrl Pts',(0.473986757999943,11.6,-10.996887016));
#154177=CARTESIAN_POINT('Ctrl Pts',(0.475170271999945,15.2,-10.999731268));
#154178=CARTESIAN_POINT('Ctrl Pts',(0.475170271999945,11.6,-10.999731268));
#154179=CARTESIAN_POINT('Ctrl Pts',(0.476358134999944,15.2,-11.002579431));
#154180=CARTESIAN_POINT('Ctrl Pts',(0.476358134999944,11.6,-11.002579431));
#154181=CARTESIAN_POINT('Ctrl Pts',(0.477550345999944,15.2,-11.005431497));
#154182=CARTESIAN_POINT('Ctrl Pts',(0.477550345999944,11.6,-11.005431497));
#154183=CARTESIAN_POINT('Ctrl Pts',(0.478746909999943,15.2,-11.008287453));
#154184=CARTESIAN_POINT('Ctrl Pts',(0.478746909999943,11.6,-11.008287453));
#154185=CARTESIAN_POINT('Ctrl Pts',(0.479947829999944,15.2,-11.011147287));
#154186=CARTESIAN_POINT('Ctrl Pts',(0.479947829999944,11.6,-11.011147287));
#154187=CARTESIAN_POINT('Ctrl Pts',(0.481153109999944,15.2,-11.014010988));
#154188=CARTESIAN_POINT('Ctrl Pts',(0.481153109999944,11.6,-11.014010988));
#154189=CARTESIAN_POINT('Ctrl Pts',(0.482362750999944,15.2,-11.016878547));
#154190=CARTESIAN_POINT('Ctrl Pts',(0.482362750999944,11.6,-11.016878547));
#154191=CARTESIAN_POINT('Ctrl Pts',(0.483576757999945,15.2,-11.01974995));
#154192=CARTESIAN_POINT('Ctrl Pts',(0.483576757999945,11.6,-11.01974995));
#154193=CARTESIAN_POINT('Ctrl Pts',(0.484795132999943,15.2,-11.022625188));
#154194=CARTESIAN_POINT('Ctrl Pts',(0.484795132999943,11.6,-11.022625188));
#154195=CARTESIAN_POINT('Ctrl Pts',(0.486017879999944,15.2,-11.025504247));
#154196=CARTESIAN_POINT('Ctrl Pts',(0.486017879999944,11.6,-11.025504247));
#154197=CARTESIAN_POINT('Ctrl Pts',(0.487245001999945,15.2,-11.028387119));
#154198=CARTESIAN_POINT('Ctrl Pts',(0.487245001999945,11.6,-11.028387119));
#154199=CARTESIAN_POINT('Ctrl Pts',(0.488476501999945,15.2,-11.031273791));
#154200=CARTESIAN_POINT('Ctrl Pts',(0.488476501999945,11.6,-11.031273791));
#154201=CARTESIAN_POINT('Ctrl Pts',(0.489712381999944,15.2,-11.034164252));
#154202=CARTESIAN_POINT('Ctrl Pts',(0.489712381999944,11.6,-11.034164252));
#154203=CARTESIAN_POINT('Ctrl Pts',(0.490952645999944,15.2,-11.037058491));
#154204=CARTESIAN_POINT('Ctrl Pts',(0.490952645999944,11.6,-11.037058491));
#154205=CARTESIAN_POINT('Ctrl Pts',(0.492197297999944,15.2,-11.039956497));
#154206=CARTESIAN_POINT('Ctrl Pts',(0.492197297999944,11.6,-11.039956497));
#154207=CARTESIAN_POINT('Ctrl Pts',(0.493446337999943,15.2,-11.04285826));
#154208=CARTESIAN_POINT('Ctrl Pts',(0.493446337999943,11.6,-11.04285826));
#154209=CARTESIAN_POINT('Ctrl Pts',(0.494699771999944,15.2,-11.045763768));
#154210=CARTESIAN_POINT('Ctrl Pts',(0.494699771999944,11.6,-11.045763768));
#154211=CARTESIAN_POINT('Ctrl Pts',(0.495957600999944,15.2,-11.04867301));
#154212=CARTESIAN_POINT('Ctrl Pts',(0.495957600999944,11.6,-11.04867301));
#154213=CARTESIAN_POINT('Ctrl Pts',(0.497219829999944,15.2,-11.051585974));
#154214=CARTESIAN_POINT('Ctrl Pts',(0.497219829999944,11.6,-11.051585974));
#154215=CARTESIAN_POINT('Ctrl Pts',(0.498486459999944,15.2,-11.05450265));
#154216=CARTESIAN_POINT('Ctrl Pts',(0.498486459999944,11.6,-11.05450265));
#154217=CARTESIAN_POINT('Ctrl Pts',(0.499757494999944,15.2,-11.057423028));
#154218=CARTESIAN_POINT('Ctrl Pts',(0.499757494999944,11.6,-11.057423028));
#154219=CARTESIAN_POINT('Ctrl Pts',(0.501032935999944,15.2,-11.060347096));
#154220=CARTESIAN_POINT('Ctrl Pts',(0.501032935999944,11.6,-11.060347096));
#154221=CARTESIAN_POINT('Ctrl Pts',(0.502312788999945,15.2,-11.063274844));
#154222=CARTESIAN_POINT('Ctrl Pts',(0.502312788999945,11.6,-11.063274844));
#154223=CARTESIAN_POINT('Ctrl Pts',(0.503597054999945,15.2,-11.066206259));
#154224=CARTESIAN_POINT('Ctrl Pts',(0.503597054999945,11.6,-11.066206259));
#154225=CARTESIAN_POINT('Ctrl Pts',(0.504885736999944,15.2,-11.069141332));
#154226=CARTESIAN_POINT('Ctrl Pts',(0.504885736999944,11.6,-11.069141332));
#154227=CARTESIAN_POINT('Ctrl Pts',(0.506178838999943,15.2,-11.072080052));
#154228=CARTESIAN_POINT('Ctrl Pts',(0.506178838999943,11.6,-11.072080052));
#154229=CARTESIAN_POINT('Ctrl Pts',(0.507476362999945,15.2,-11.075022407));
#154230=CARTESIAN_POINT('Ctrl Pts',(0.507476362999945,11.6,-11.075022407));
#154231=CARTESIAN_POINT('Ctrl Pts',(0.508778309999944,15.2,-11.077968387));
#154232=CARTESIAN_POINT('Ctrl Pts',(0.508778309999944,11.6,-11.077968387));
#154233=CARTESIAN_POINT('Ctrl Pts',(0.510084685999944,15.2,-11.080917982));
#154234=CARTESIAN_POINT('Ctrl Pts',(0.510084685999944,11.6,-11.080917982));
#154235=CARTESIAN_POINT('Ctrl Pts',(0.511395492999944,15.2,-11.08387118));
#154236=CARTESIAN_POINT('Ctrl Pts',(0.511395492999944,11.6,-11.08387118));
#154237=CARTESIAN_POINT('Ctrl Pts',(0.512710730999945,15.2,-11.086827972));
#154238=CARTESIAN_POINT('Ctrl Pts',(0.512710730999945,11.6,-11.086827972));
#154239=CARTESIAN_POINT('Ctrl Pts',(0.514030406999945,15.2,-11.089788344));
#154240=CARTESIAN_POINT('Ctrl Pts',(0.514030406999945,11.6,-11.089788344));
#154241=CARTESIAN_POINT('Ctrl Pts',(0.515354519999944,15.2,-11.092752289));
#154242=CARTESIAN_POINT('Ctrl Pts',(0.515354519999944,11.6,-11.092752289));
#154243=CARTESIAN_POINT('Ctrl Pts',(0.516683075999944,15.2,-11.095719793));
#154244=CARTESIAN_POINT('Ctrl Pts',(0.516683075999944,11.6,-11.095719793));
#154245=CARTESIAN_POINT('Ctrl Pts',(0.518016074999944,15.2,-11.098690848));
#154246=CARTESIAN_POINT('Ctrl Pts',(0.518016074999944,11.6,-11.098690848));
#154247=CARTESIAN_POINT('Ctrl Pts',(0.519353520999944,15.2,-11.101665441));
#154248=CARTESIAN_POINT('Ctrl Pts',(0.519353520999944,11.6,-11.101665441));
#154249=CARTESIAN_POINT('Ctrl Pts',(0.520695416999944,15.2,-11.104643564));
#154250=CARTESIAN_POINT('Ctrl Pts',(0.520695416999944,11.6,-11.104643564));
#154251=CARTESIAN_POINT('Ctrl Pts',(0.522041764999944,15.2,-11.107625205));
#154252=CARTESIAN_POINT('Ctrl Pts',(0.522041764999944,11.6,-11.107625205));
#154253=CARTESIAN_POINT('Ctrl Pts',(0.523392567999944,15.2,-11.110610353));
#154254=CARTESIAN_POINT('Ctrl Pts',(0.523392567999944,11.6,-11.110610353));
#154255=CARTESIAN_POINT('Ctrl Pts',(0.524747828999944,15.2,-11.113598997));
#154256=CARTESIAN_POINT('Ctrl Pts',(0.524747828999944,11.6,-11.113598997));
#154257=CARTESIAN_POINT('Ctrl Pts',(0.526107550999945,15.2,-11.116591128));
#154258=CARTESIAN_POINT('Ctrl Pts',(0.526107550999945,11.6,-11.116591128));
#154259=CARTESIAN_POINT('Ctrl Pts',(0.527471734999944,15.2,-11.119586735));
#154260=CARTESIAN_POINT('Ctrl Pts',(0.527471734999944,11.6,-11.119586735));
#154261=CARTESIAN_POINT('Ctrl Pts',(0.528840383999943,15.2,-11.122585808));
#154262=CARTESIAN_POINT('Ctrl Pts',(0.528840383999943,11.6,-11.122585808));
#154263=CARTESIAN_POINT('Ctrl Pts',(0.530213500999944,15.2,-11.125588334));
#154264=CARTESIAN_POINT('Ctrl Pts',(0.530213500999944,11.6,-11.125588334));
#154265=CARTESIAN_POINT('Ctrl Pts',(0.531591089999944,15.2,-11.128594306));
#154266=CARTESIAN_POINT('Ctrl Pts',(0.531591089999944,11.6,-11.128594306));
#154267=CARTESIAN_POINT('Ctrl Pts',(0.532973150999945,15.2,-11.131603711));
#154268=CARTESIAN_POINT('Ctrl Pts',(0.532973150999945,11.6,-11.131603711));
#154269=CARTESIAN_POINT('Ctrl Pts',(0.534359687999945,15.2,-11.13461654));
#154270=CARTESIAN_POINT('Ctrl Pts',(0.534359687999945,11.6,-11.13461654));
#154271=CARTESIAN_POINT('Ctrl Pts',(0.535750703999944,15.2,-11.137632781));
#154272=CARTESIAN_POINT('Ctrl Pts',(0.535750703999944,11.6,-11.137632781));
#154273=CARTESIAN_POINT('Ctrl Pts',(0.537146200999944,15.2,-11.140652425));
#154274=CARTESIAN_POINT('Ctrl Pts',(0.537146200999944,11.6,-11.140652425));
#154275=CARTESIAN_POINT('Ctrl Pts',(0.538546180999945,15.2,-11.143675461));
#154276=CARTESIAN_POINT('Ctrl Pts',(0.538546180999945,11.6,-11.143675461));
#154277=CARTESIAN_POINT('Ctrl Pts',(0.539950646999944,15.2,-11.146701879));
#154278=CARTESIAN_POINT('Ctrl Pts',(0.539950646999944,11.6,-11.146701879));
#154279=CARTESIAN_POINT('Ctrl Pts',(0.541359600999944,15.2,-11.149731669));
#154280=CARTESIAN_POINT('Ctrl Pts',(0.541359600999944,11.6,-11.149731669));
#154281=CARTESIAN_POINT('Ctrl Pts',(0.542773046999944,15.2,-11.152764819));
#154282=CARTESIAN_POINT('Ctrl Pts',(0.542773046999944,11.6,-11.152764819));
#154283=CARTESIAN_POINT('Ctrl Pts',(0.544190985999945,15.2,-11.155801321));
#154284=CARTESIAN_POINT('Ctrl Pts',(0.544190985999945,11.6,-11.155801321));
#154285=CARTESIAN_POINT('Ctrl Pts',(0.545613420999944,15.2,-11.158841164));
#154286=CARTESIAN_POINT('Ctrl Pts',(0.545613420999944,11.6,-11.158841164));
#154287=CARTESIAN_POINT('Ctrl Pts',(0.547040353999945,15.2,-11.161884336));
#154288=CARTESIAN_POINT('Ctrl Pts',(0.547040353999945,11.6,-11.161884336));
#154289=CARTESIAN_POINT('Ctrl Pts',(0.548471787999943,15.2,-11.164930828));
#154290=CARTESIAN_POINT('Ctrl Pts',(0.548471787999943,11.6,-11.164930828));
#154291=CARTESIAN_POINT('Ctrl Pts',(0.549907724999944,15.2,-11.167980631));
#154292=CARTESIAN_POINT('Ctrl Pts',(0.549907724999944,11.6,-11.167980631));
#154293=CARTESIAN_POINT('Ctrl Pts',(0.551348166999944,15.2,-11.171033733));
#154294=CARTESIAN_POINT('Ctrl Pts',(0.551348166999944,11.6,-11.171033733));
#154295=CARTESIAN_POINT('Ctrl Pts',(0.552793118999944,15.2,-11.174090123));
#154296=CARTESIAN_POINT('Ctrl Pts',(0.552793118999944,11.6,-11.174090123));
#154297=CARTESIAN_POINT('Ctrl Pts',(0.554242579999944,15.2,-11.177149794));
#154298=CARTESIAN_POINT('Ctrl Pts',(0.554242579999944,11.6,-11.177149794));
#154299=CARTESIAN_POINT('Ctrl Pts',(0.555696552999944,15.2,-11.180212734));
#154300=CARTESIAN_POINT('Ctrl Pts',(0.555696552999944,11.6,-11.180212734));
#154301=CARTESIAN_POINT('Ctrl Pts',(0.557155042999944,15.2,-11.183278932));
#154302=CARTESIAN_POINT('Ctrl Pts',(0.557155042999944,11.6,-11.183278932));
#154303=CARTESIAN_POINT('Ctrl Pts',(0.558618047999944,15.2,-11.186348379));
#154304=CARTESIAN_POINT('Ctrl Pts',(0.558618047999944,11.6,-11.186348379));
#154305=CARTESIAN_POINT('Ctrl Pts',(0.560085574999943,15.2,-11.189421065));
#154306=CARTESIAN_POINT('Ctrl Pts',(0.560085574999943,11.6,-11.189421065));
#154307=CARTESIAN_POINT('Ctrl Pts',(0.561557623999944,15.2,-11.192496979));
#154308=CARTESIAN_POINT('Ctrl Pts',(0.561557623999944,11.6,-11.192496979));
#154309=CARTESIAN_POINT('Ctrl Pts',(0.563034195999944,15.2,-11.195576112));
#154310=CARTESIAN_POINT('Ctrl Pts',(0.563034195999944,11.6,-11.195576112));
#154311=CARTESIAN_POINT('Ctrl Pts',(0.564515294999944,15.2,-11.198658453));
#154312=CARTESIAN_POINT('Ctrl Pts',(0.564515294999944,11.6,-11.198658453));
#154313=CARTESIAN_POINT('Ctrl Pts',(0.566000922999944,15.2,-11.201743993));
#154314=CARTESIAN_POINT('Ctrl Pts',(0.566000922999944,11.6,-11.201743993));
#154315=CARTESIAN_POINT('Ctrl Pts',(0.567491082999945,15.2,-11.204832721));
#154316=CARTESIAN_POINT('Ctrl Pts',(0.567491082999945,11.6,-11.204832721));
#154317=CARTESIAN_POINT('Ctrl Pts',(0.568985775999944,15.2,-11.207924627));
#154318=CARTESIAN_POINT('Ctrl Pts',(0.568985775999944,11.6,-11.207924627));
#154319=CARTESIAN_POINT('Ctrl Pts',(0.570485004999944,15.2,-11.211019702));
#154320=CARTESIAN_POINT('Ctrl Pts',(0.570485004999944,11.6,-11.211019702));
#154321=CARTESIAN_POINT('Ctrl Pts',(0.571988771999944,15.2,-11.214117935));
#154322=CARTESIAN_POINT('Ctrl Pts',(0.571988771999944,11.6,-11.214117935));
#154323=CARTESIAN_POINT('Ctrl Pts',(0.573497078999944,15.2,-11.217219316));
#154324=CARTESIAN_POINT('Ctrl Pts',(0.573497078999944,11.6,-11.217219316));
#154325=CARTESIAN_POINT('Ctrl Pts',(0.575009928999944,15.2,-11.220323837));
#154326=CARTESIAN_POINT('Ctrl Pts',(0.575009928999944,11.6,-11.220323837));
#154327=CARTESIAN_POINT('Ctrl Pts',(0.576527321999943,15.2,-11.223431485));
#154328=CARTESIAN_POINT('Ctrl Pts',(0.576527321999943,11.6,-11.223431485));
#154329=CARTESIAN_POINT('Ctrl Pts',(0.578049262999943,15.2,-11.226542253));
#154330=CARTESIAN_POINT('Ctrl Pts',(0.578049262999943,11.6,-11.226542253));
#154331=CARTESIAN_POINT('Ctrl Pts',(0.579575752999945,15.2,-11.229656128));
#154332=CARTESIAN_POINT('Ctrl Pts',(0.579575752999945,11.6,-11.229656128));
#154333=CARTESIAN_POINT('Ctrl Pts',(0.581106792999945,15.2,-11.232773103));
#154334=CARTESIAN_POINT('Ctrl Pts',(0.581106792999945,11.6,-11.232773103));
#154335=CARTESIAN_POINT('Ctrl Pts',(0.582642387999944,15.2,-11.235893168));
#154336=CARTESIAN_POINT('Ctrl Pts',(0.582642387999944,11.6,-11.235893168));
#154337=CARTESIAN_POINT('Ctrl Pts',(0.584182536999944,15.2,-11.23901631));
#154338=CARTESIAN_POINT('Ctrl Pts',(0.584182536999944,11.6,-11.23901631));
#154339=CARTESIAN_POINT('Ctrl Pts',(0.585727243999944,15.2,-11.242142523));
#154340=CARTESIAN_POINT('Ctrl Pts',(0.585727243999944,11.6,-11.242142523));
#154341=CARTESIAN_POINT('Ctrl Pts',(0.587276510999944,15.2,-11.245271795));
#154342=CARTESIAN_POINT('Ctrl Pts',(0.587276510999944,11.6,-11.245271795));
#154343=CARTESIAN_POINT('Ctrl Pts',(0.588830339999945,15.2,-11.248404117));
#154344=CARTESIAN_POINT('Ctrl Pts',(0.588830339999945,11.6,-11.248404117));
#154345=CARTESIAN_POINT('Ctrl Pts',(0.590388730999944,15.2,-11.251539479));
#154346=CARTESIAN_POINT('Ctrl Pts',(0.590388730999944,11.6,-11.251539479));
#154347=CARTESIAN_POINT('Ctrl Pts',(0.591951689999944,15.2,-11.254677871));
#154348=CARTESIAN_POINT('Ctrl Pts',(0.591951689999944,11.6,-11.254677871));
#154349=CARTESIAN_POINT('Ctrl Pts',(0.593519214999944,15.2,-11.257819284));
#154350=CARTESIAN_POINT('Ctrl Pts',(0.593519214999944,11.6,-11.257819284));
#154351=CARTESIAN_POINT('Ctrl Pts',(0.595091311999945,15.2,-11.260963707));
#154352=CARTESIAN_POINT('Ctrl Pts',(0.595091311999945,11.6,-11.260963707));
#154353=CARTESIAN_POINT('Ctrl Pts',(0.596667979999944,15.2,-11.264111132));
#154354=CARTESIAN_POINT('Ctrl Pts',(0.596667979999944,11.6,-11.264111132));
#154355=CARTESIAN_POINT('Ctrl Pts',(0.598249221999944,15.2,-11.267261548));
#154356=CARTESIAN_POINT('Ctrl Pts',(0.598249221999944,11.6,-11.267261548));
#154357=CARTESIAN_POINT('Ctrl Pts',(0.599835039999944,15.2,-11.270414946));
#154358=CARTESIAN_POINT('Ctrl Pts',(0.599835039999944,11.6,-11.270414946));
#154359=CARTESIAN_POINT('Ctrl Pts',(0.601425436999944,15.2,-11.273571316));
#154360=CARTESIAN_POINT('Ctrl Pts',(0.601425436999944,11.6,-11.273571316));
#154361=CARTESIAN_POINT('Ctrl Pts',(0.603020412999945,15.2,-11.276730648));
#154362=CARTESIAN_POINT('Ctrl Pts',(0.603020412999945,11.6,-11.276730648));
#154363=CARTESIAN_POINT('Ctrl Pts',(0.604619971999945,15.2,-11.279892934));
#154364=CARTESIAN_POINT('Ctrl Pts',(0.604619971999945,11.6,-11.279892934));
#154365=CARTESIAN_POINT('Ctrl Pts',(0.606224114999944,15.2,-11.283058161));
#154366=CARTESIAN_POINT('Ctrl Pts',(0.606224114999944,11.6,-11.283058161));
#154367=CARTESIAN_POINT('Ctrl Pts',(0.607832842999944,15.2,-11.286226323));
#154368=CARTESIAN_POINT('Ctrl Pts',(0.607832842999944,11.6,-11.286226323));
#154369=CARTESIAN_POINT('Ctrl Pts',(0.609446159999945,15.2,-11.289397409));
#154370=CARTESIAN_POINT('Ctrl Pts',(0.609446159999945,11.6,-11.289397409));
#154371=CARTESIAN_POINT('Ctrl Pts',(0.611064066999945,15.2,-11.29257141));
#154372=CARTESIAN_POINT('Ctrl Pts',(0.611064066999945,11.6,-11.29257141));
#154373=CARTESIAN_POINT('Ctrl Pts',(0.612686564999944,15.2,-11.295748315));
#154374=CARTESIAN_POINT('Ctrl Pts',(0.612686564999944,11.6,-11.295748315));
#154375=CARTESIAN_POINT('Ctrl Pts',(0.614313656999944,15.2,-11.298928116));
#154376=CARTESIAN_POINT('Ctrl Pts',(0.614313656999944,11.6,-11.298928116));
#154377=CARTESIAN_POINT('Ctrl Pts',(0.615945344999944,15.2,-11.302110802));
#154378=CARTESIAN_POINT('Ctrl Pts',(0.615945344999944,11.6,-11.302110802));
#154379=CARTESIAN_POINT('Ctrl Pts',(0.617581629999945,15.2,-11.305296365));
#154380=CARTESIAN_POINT('Ctrl Pts',(0.617581629999945,11.6,-11.305296365));
#154381=CARTESIAN_POINT('Ctrl Pts',(0.619222514999944,15.2,-11.308484795));
#154382=CARTESIAN_POINT('Ctrl Pts',(0.619222514999944,11.6,-11.308484795));
#154383=CARTESIAN_POINT('Ctrl Pts',(0.620868000999945,15.2,-11.311676082));
#154384=CARTESIAN_POINT('Ctrl Pts',(0.620868000999945,11.6,-11.311676082));
#154385=CARTESIAN_POINT('Ctrl Pts',(0.622518089999944,15.2,-11.314870217));
#154386=CARTESIAN_POINT('Ctrl Pts',(0.622518089999944,11.6,-11.314870217));
#154387=CARTESIAN_POINT('Ctrl Pts',(0.624172783999944,15.2,-11.31806719));
#154388=CARTESIAN_POINT('Ctrl Pts',(0.624172783999944,11.6,-11.31806719));
#154389=CARTESIAN_POINT('Ctrl Pts',(0.625832085999944,15.2,-11.321266994));
#154390=CARTESIAN_POINT('Ctrl Pts',(0.625832085999944,11.6,-11.321266994));
#154391=CARTESIAN_POINT('Ctrl Pts',(0.627495994999945,15.2,-11.324469616));
#154392=CARTESIAN_POINT('Ctrl Pts',(0.627495994999945,11.6,-11.324469616));
#154393=CARTESIAN_POINT('Ctrl Pts',(0.629164515999945,15.2,-11.327675049));
#154394=CARTESIAN_POINT('Ctrl Pts',(0.629164515999945,11.6,-11.327675049));
#154395=CARTESIAN_POINT('Ctrl Pts',(0.630837647999944,15.2,-11.330883282));
#154396=CARTESIAN_POINT('Ctrl Pts',(0.630837647999944,11.6,-11.330883282));
#154397=CARTESIAN_POINT('Ctrl Pts',(0.632515393999945,15.2,-11.334094307));
#154398=CARTESIAN_POINT('Ctrl Pts',(0.632515393999945,11.6,-11.334094307));
#154399=CARTESIAN_POINT('Ctrl Pts',(0.634197756999945,15.2,-11.337308115));
#154400=CARTESIAN_POINT('Ctrl Pts',(0.634197756999945,11.6,-11.337308115));
#154401=CARTESIAN_POINT('Ctrl Pts',(0.635884736999944,15.2,-11.340524695));
#154402=CARTESIAN_POINT('Ctrl Pts',(0.635884736999944,11.6,-11.340524695));
#154403=CARTESIAN_POINT('Ctrl Pts',(0.637576336999944,15.2,-11.343744038));
#154404=CARTESIAN_POINT('Ctrl Pts',(0.637576336999944,11.6,-11.343744038));
#154405=CARTESIAN_POINT('Ctrl Pts',(0.639272556999945,15.2,-11.346966135));
#154406=CARTESIAN_POINT('Ctrl Pts',(0.639272556999945,11.6,-11.346966135));
#154407=CARTESIAN_POINT('Ctrl Pts',(0.640973400999945,15.2,-11.350190979));
#154408=CARTESIAN_POINT('Ctrl Pts',(0.640973400999945,11.6,-11.350190979));
#154409=CARTESIAN_POINT('Ctrl Pts',(0.642678868999944,15.2,-11.353418557));
#154410=CARTESIAN_POINT('Ctrl Pts',(0.642678868999944,11.6,-11.353418557));
#154411=CARTESIAN_POINT('Ctrl Pts',(0.644388963999944,15.2,-11.356648862));
#154412=CARTESIAN_POINT('Ctrl Pts',(0.644388963999944,11.6,-11.356648862));
#154413=CARTESIAN_POINT('Ctrl Pts',(0.646103685999945,15.2,-11.359881884));
#154414=CARTESIAN_POINT('Ctrl Pts',(0.646103685999945,11.6,-11.359881884));
#154415=CARTESIAN_POINT('Ctrl Pts',(0.647823038999944,15.2,-11.363117614));
#154416=CARTESIAN_POINT('Ctrl Pts',(0.647823038999944,11.6,-11.363117614));
#154417=CARTESIAN_POINT('Ctrl Pts',(0.649547021999944,15.2,-11.366356043));
#154418=CARTESIAN_POINT('Ctrl Pts',(0.649547021999944,11.6,-11.366356043));
#154419=CARTESIAN_POINT('Ctrl Pts',(0.651275639999944,15.2,-11.369597161));
#154420=CARTESIAN_POINT('Ctrl Pts',(0.651275639999944,11.6,-11.369597161));
#154421=CARTESIAN_POINT('Ctrl Pts',(0.653008890999944,15.2,-11.37284096));
#154422=CARTESIAN_POINT('Ctrl Pts',(0.653008890999944,11.6,-11.37284096));
#154423=CARTESIAN_POINT('Ctrl Pts',(0.654746778999944,15.2,-11.37608743));
#154424=CARTESIAN_POINT('Ctrl Pts',(0.654746778999944,11.6,-11.37608743));
#154425=CARTESIAN_POINT('Ctrl Pts',(0.656489305999944,15.2,-11.379336561));
#154426=CARTESIAN_POINT('Ctrl Pts',(0.656489305999944,11.6,-11.379336561));
#154427=CARTESIAN_POINT('Ctrl Pts',(0.658236471999943,15.2,-11.382588345));
#154428=CARTESIAN_POINT('Ctrl Pts',(0.658236471999943,11.6,-11.382588345));
#154429=CARTESIAN_POINT('Ctrl Pts',(0.659988278999944,15.2,-11.385842772));
#154430=CARTESIAN_POINT('Ctrl Pts',(0.659988278999944,11.6,-11.385842772));
#154431=CARTESIAN_POINT('Ctrl Pts',(0.661744729999943,15.2,-11.389099835));
#154432=CARTESIAN_POINT('Ctrl Pts',(0.661744729999943,11.6,-11.389099835));
#154433=CARTESIAN_POINT('Ctrl Pts',(0.663505824999944,15.2,-11.392359523));
#154434=CARTESIAN_POINT('Ctrl Pts',(0.663505824999944,11.6,-11.392359523));
#154435=CARTESIAN_POINT('Ctrl Pts',(0.665271565999944,15.2,-11.395621827));
#154436=CARTESIAN_POINT('Ctrl Pts',(0.665271565999944,11.6,-11.395621827));
#154437=CARTESIAN_POINT('Ctrl Pts',(0.667041954999944,15.2,-11.39888674));
#154438=CARTESIAN_POINT('Ctrl Pts',(0.667041954999944,11.6,-11.39888674));
#154439=CARTESIAN_POINT('Ctrl Pts',(0.668816992999944,15.2,-11.402154251));
#154440=CARTESIAN_POINT('Ctrl Pts',(0.668816992999944,11.6,-11.402154251));
#154441=CARTESIAN_POINT('Ctrl Pts',(0.670596681999944,15.2,-11.405424352));
#154442=CARTESIAN_POINT('Ctrl Pts',(0.670596681999944,11.6,-11.405424352));
#154443=CARTESIAN_POINT('Ctrl Pts',(0.672381022999944,15.2,-11.408697032));
#154444=CARTESIAN_POINT('Ctrl Pts',(0.672381022999944,11.6,-11.408697032));
#154445=CARTESIAN_POINT('Ctrl Pts',(0.674170018999944,15.2,-11.411972283));
#154446=CARTESIAN_POINT('Ctrl Pts',(0.674170018999944,11.6,-11.411972283));
#154447=CARTESIAN_POINT('Ctrl Pts',(0.675963669999944,15.2,-11.415250096));
#154448=CARTESIAN_POINT('Ctrl Pts',(0.675963669999944,11.6,-11.415250096));
#154449=CARTESIAN_POINT('Ctrl Pts',(0.677761977999943,15.2,-11.418530461));
#154450=CARTESIAN_POINT('Ctrl Pts',(0.677761977999943,11.6,-11.418530461));
#154451=CARTESIAN_POINT('Ctrl Pts',(0.679564944999944,15.2,-11.421813369));
#154452=CARTESIAN_POINT('Ctrl Pts',(0.679564944999944,11.6,-11.421813369));
#154453=CARTESIAN_POINT('Ctrl Pts',(0.681372572999944,15.2,-11.425098811));
#154454=CARTESIAN_POINT('Ctrl Pts',(0.681372572999944,11.6,-11.425098811));
#154455=CARTESIAN_POINT('Ctrl Pts',(0.683184861999945,15.2,-11.42838678));
#154456=CARTESIAN_POINT('Ctrl Pts',(0.683184861999945,11.6,-11.42838678));
#154457=CARTESIAN_POINT('Ctrl Pts',(0.685001812999944,15.2,-11.431677269));
#154458=CARTESIAN_POINT('Ctrl Pts',(0.685001812999944,11.6,-11.431677269));
#154459=CARTESIAN_POINT('Ctrl Pts',(0.686823428999944,15.2,-11.434970268));
#154460=CARTESIAN_POINT('Ctrl Pts',(0.686823428999944,11.6,-11.434970268));
#154461=CARTESIAN_POINT('Ctrl Pts',(0.688649710999945,15.2,-11.438265769));
#154462=CARTESIAN_POINT('Ctrl Pts',(0.688649710999945,11.6,-11.438265769));
#154463=CARTESIAN_POINT('Ctrl Pts',(0.690480658999945,15.2,-11.441563763));
#154464=CARTESIAN_POINT('Ctrl Pts',(0.690480658999945,11.6,-11.441563763));
#154465=CARTESIAN_POINT('Ctrl Pts',(0.692316276999944,15.2,-11.444864239));
#154466=CARTESIAN_POINT('Ctrl Pts',(0.692316276999944,11.6,-11.444864239));
#154467=CARTESIAN_POINT('Ctrl Pts',(0.694156563999945,15.2,-11.448167187));
#154468=CARTESIAN_POINT('Ctrl Pts',(0.694156563999945,11.6,-11.448167187));
#154469=CARTESIAN_POINT('Ctrl Pts',(0.696001524999944,15.2,-11.451472595));
#154470=CARTESIAN_POINT('Ctrl Pts',(0.696001524999944,11.6,-11.451472595));
#154471=CARTESIAN_POINT('Ctrl Pts',(0.697851158999944,15.2,-11.454780453));
#154472=CARTESIAN_POINT('Ctrl Pts',(0.697851158999944,11.6,-11.454780453));
#154473=CARTESIAN_POINT('Ctrl Pts',(0.699705468999944,15.2,-11.458090751));
#154474=CARTESIAN_POINT('Ctrl Pts',(0.699705468999944,11.6,-11.458090751));
#154475=CARTESIAN_POINT('Ctrl Pts',(0.701564455999945,15.2,-11.461403481));
#154476=CARTESIAN_POINT('Ctrl Pts',(0.701564455999945,11.6,-11.461403481));
#154477=CARTESIAN_POINT('Ctrl Pts',(0.703428120999944,15.2,-11.464718637));
#154478=CARTESIAN_POINT('Ctrl Pts',(0.703428120999944,11.6,-11.464718637));
#154479=CARTESIAN_POINT('Ctrl Pts',(0.705296462999944,15.2,-11.468036216));
#154480=CARTESIAN_POINT('Ctrl Pts',(0.705296462999944,11.6,-11.468036216));
#154481=CARTESIAN_POINT('Ctrl Pts',(0.707169485999944,15.2,-11.471356215));
#154482=CARTESIAN_POINT('Ctrl Pts',(0.707169485999944,11.6,-11.471356215));
#154483=CARTESIAN_POINT('Ctrl Pts',(0.708671644999944,15.2,-11.474014149));
#154484=CARTESIAN_POINT('Ctrl Pts',(0.708671644999944,11.6,-11.474014149));
#154485=CARTESIAN_POINT('Ctrl Pts',(0.709800370999945,15.2,-11.476008688));
#154486=CARTESIAN_POINT('Ctrl Pts',(0.709800370999945,11.6,-11.476008688));
#154487=CARTESIAN_POINT('Ctrl Pts',(0.710553790999944,15.2,-11.477338863));
#154488=CARTESIAN_POINT('Ctrl Pts',(0.710553790999944,11.6,-11.477338863));
#154489=CARTESIAN_POINT('Ctrl Pts',(0.710930733999944,15.2,-11.478004072));
#154490=CARTESIAN_POINT('Ctrl Pts',(0.710930733999944,11.6,-11.478004072));
#154491=CARTESIAN_POINT('',(0.292001928999944,15.2,-10.370890023));
#154492=CARTESIAN_POINT('',(0.292001928999944,12.2,-10.370890023));
#154493=CARTESIAN_POINT('',(0.292001928999944,15.2,-10.370890023));
#154494=CARTESIAN_POINT('Ctrl Pts',(0.292001928999944,15.2,-10.370890023));
#154495=CARTESIAN_POINT('Ctrl Pts',(0.292021795999944,15.2,-10.371063245));
#154496=CARTESIAN_POINT('Ctrl Pts',(0.292062308999944,15.2,-10.371415731));
#154497=CARTESIAN_POINT('Ctrl Pts',(0.292123960999945,15.2,-10.371949799));
#154498=CARTESIAN_POINT('Ctrl Pts',(0.292207546999944,15.2,-10.372669176));
#154499=CARTESIAN_POINT('Ctrl Pts',(0.292314179999943,15.2,-10.373578975));
#154500=CARTESIAN_POINT('Ctrl Pts',(0.292423468999944,15.2,-10.374503411));
#154501=CARTESIAN_POINT('Ctrl Pts',(0.292534811999945,15.2,-10.375437184));
#154502=CARTESIAN_POINT('Ctrl Pts',(0.292648222999944,15.2,-10.376380266));
#154503=CARTESIAN_POINT('Ctrl Pts',(0.292763716999945,15.2,-10.377332627));
#154504=CARTESIAN_POINT('Ctrl Pts',(0.292881308999944,15.2,-10.378294239));
#154505=CARTESIAN_POINT('Ctrl Pts',(0.293001014999945,15.2,-10.379265074));
#154506=CARTESIAN_POINT('Ctrl Pts',(0.293122845999945,15.2,-10.380245102));
#154507=CARTESIAN_POINT('Ctrl Pts',(0.293246819999944,15.2,-10.381234297));
#154508=CARTESIAN_POINT('Ctrl Pts',(0.293372948999944,15.2,-10.382232628));
#154509=CARTESIAN_POINT('Ctrl Pts',(0.293501248999943,15.2,-10.383240069));
#154510=CARTESIAN_POINT('Ctrl Pts',(0.293631731999945,15.2,-10.384256592));
#154511=CARTESIAN_POINT('Ctrl Pts',(0.293764412999945,15.2,-10.385282168));
#154512=CARTESIAN_POINT('Ctrl Pts',(0.293899306999944,15.2,-10.38631677));
#154513=CARTESIAN_POINT('Ctrl Pts',(0.294036426999943,15.2,-10.387360371));
#154514=CARTESIAN_POINT('Ctrl Pts',(0.294175786999944,15.2,-10.388412945));
#154515=CARTESIAN_POINT('Ctrl Pts',(0.294317400999944,15.2,-10.389474461));
#154516=CARTESIAN_POINT('Ctrl Pts',(0.294461281999944,15.2,-10.390544895));
#154517=CARTESIAN_POINT('Ctrl Pts',(0.294607443999944,15.2,-10.391624218));
#154518=CARTESIAN_POINT('Ctrl Pts',(0.294755900999943,15.2,-10.392712404));
#154519=CARTESIAN_POINT('Ctrl Pts',(0.294906665999944,15.2,-10.393809427));
#154520=CARTESIAN_POINT('Ctrl Pts',(0.295059751999943,15.2,-10.394915259));
#154521=CARTESIAN_POINT('Ctrl Pts',(0.295215172999944,15.2,-10.396029875));
#154522=CARTESIAN_POINT('Ctrl Pts',(0.295372941999944,15.2,-10.397153247));
#154523=CARTESIAN_POINT('Ctrl Pts',(0.295533071999945,15.2,-10.39828535));
#154524=CARTESIAN_POINT('Ctrl Pts',(0.295695575999944,15.2,-10.399426157));
#154525=CARTESIAN_POINT('Ctrl Pts',(0.295860466999944,15.2,-10.400575642));
#154526=CARTESIAN_POINT('Ctrl Pts',(0.296027758999945,15.2,-10.401733778));
#154527=CARTESIAN_POINT('Ctrl Pts',(0.296197462999944,15.2,-10.402900542));
#154528=CARTESIAN_POINT('Ctrl Pts',(0.296369592999944,15.2,-10.404075906));
#154529=CARTESIAN_POINT('Ctrl Pts',(0.296544161999943,15.2,-10.405259845));
#154530=CARTESIAN_POINT('Ctrl Pts',(0.296721181999944,15.2,-10.406452335));
#154531=CARTESIAN_POINT('Ctrl Pts',(0.296900663999944,15.2,-10.407653347));
#154532=CARTESIAN_POINT('Ctrl Pts',(0.297082623999945,15.2,-10.408862859));
#154533=CARTESIAN_POINT('Ctrl Pts',(0.297267072999944,15.2,-10.410080845));
#154534=CARTESIAN_POINT('Ctrl Pts',(0.297454020999943,15.2,-10.411307279));
#154535=CARTESIAN_POINT('Ctrl Pts',(0.297643483999943,15.2,-10.412542137));
#154536=CARTESIAN_POINT('Ctrl Pts',(0.297835472999944,15.2,-10.413785393));
#154537=CARTESIAN_POINT('Ctrl Pts',(0.298029997999943,15.2,-10.415037024));
#154538=CARTESIAN_POINT('Ctrl Pts',(0.298227073999945,15.2,-10.416297005));
#154539=CARTESIAN_POINT('Ctrl Pts',(0.298426710999945,15.2,-10.41756531));
#154540=CARTESIAN_POINT('Ctrl Pts',(0.298628921999944,15.2,-10.418841915));
#154541=CARTESIAN_POINT('Ctrl Pts',(0.298874678413339,15.2,-10.420383772284));
#154542=CARTESIAN_POINT('Ctrl Pts',(0.299124331804587,15.2,-10.4219380104286));
#154543=CARTESIAN_POINT('Ctrl Pts',(0.299377904195303,15.2,-10.4235045735714));
#154544=CARTESIAN_POINT('Ctrl Pts',(0.299635420609226,15.2,-10.4250834208572));
#154545=CARTESIAN_POINT('Ctrl Pts',(0.299896902999944,15.2,-10.426674502));
#154546=CARTESIAN_POINT('Ctrl Pts',(0.300117460999945,15.2,-10.428008535));
#154547=CARTESIAN_POINT('Ctrl Pts',(0.300340685999944,15.2,-10.429350676));
#154548=CARTESIAN_POINT('Ctrl Pts',(0.300566589999944,15.2,-10.430700902));
#154549=CARTESIAN_POINT('Ctrl Pts',(0.300795183999943,15.2,-10.43205919));
#154550=CARTESIAN_POINT('Ctrl Pts',(0.301026478999944,15.2,-10.433425516));
#154551=CARTESIAN_POINT('Ctrl Pts',(0.301260486999944,15.2,-10.434799858));
#154552=CARTESIAN_POINT('Ctrl Pts',(0.301497219999945,15.2,-10.43618219));
#154553=CARTESIAN_POINT('Ctrl Pts',(0.301736685999944,15.2,-10.437572491));
#154554=CARTESIAN_POINT('Ctrl Pts',(0.301978897999945,15.2,-10.438970738));
#154555=CARTESIAN_POINT('Ctrl Pts',(0.302223867999943,15.2,-10.440376907));
#154556=CARTESIAN_POINT('Ctrl Pts',(0.302471604999944,15.2,-10.441790977));
#154557=CARTESIAN_POINT('Ctrl Pts',(0.302722120999944,15.2,-10.443212923));
#154558=CARTESIAN_POINT('Ctrl Pts',(0.302975424999945,15.2,-10.444642725));
#154559=CARTESIAN_POINT('Ctrl Pts',(0.303231531999945,15.2,-10.446080357));
#154560=CARTESIAN_POINT('Ctrl Pts',(0.303490447999945,15.2,-10.447525799));
#154561=CARTESIAN_POINT('Ctrl Pts',(0.303752185999944,15.2,-10.448979029));
#154562=CARTESIAN_POINT('Ctrl Pts',(0.304016755999944,15.2,-10.450440023));
#154563=CARTESIAN_POINT('Ctrl Pts',(0.304284168999944,15.2,-10.451908761));
#154564=CARTESIAN_POINT('Ctrl Pts',(0.304554434999943,15.2,-10.453385218));
#154565=CARTESIAN_POINT('Ctrl Pts',(0.304827565999943,15.2,-10.454869375));
#154566=CARTESIAN_POINT('Ctrl Pts',(0.305103568999944,15.2,-10.456361208));
#154567=CARTESIAN_POINT('Ctrl Pts',(0.305382456999944,15.2,-10.457860694));
#154568=CARTESIAN_POINT('Ctrl Pts',(0.305664239999944,15.2,-10.459367814));
#154569=CARTESIAN_POINT('Ctrl Pts',(0.305948927999945,15.2,-10.460882546));
#154570=CARTESIAN_POINT('Ctrl Pts',(0.306236529999945,15.2,-10.462404866));
#154571=CARTESIAN_POINT('Ctrl Pts',(0.306527057999944,15.2,-10.463934755));
#154572=CARTESIAN_POINT('Ctrl Pts',(0.306820520999944,15.2,-10.46547219));
#154573=CARTESIAN_POINT('Ctrl Pts',(0.307116928999944,15.2,-10.46701715));
#154574=CARTESIAN_POINT('Ctrl Pts',(0.307416291999945,15.2,-10.468569615));
#154575=CARTESIAN_POINT('Ctrl Pts',(0.307718619999945,15.2,-10.470129561));
#154576=CARTESIAN_POINT('Ctrl Pts',(0.308023921999944,15.2,-10.47169697));
#154577=CARTESIAN_POINT('Ctrl Pts',(0.308332209999945,15.2,-10.473271818));
#154578=CARTESIAN_POINT('Ctrl Pts',(0.308643490999945,15.2,-10.474854086));
#154579=CARTESIAN_POINT('Ctrl Pts',(0.308957776999945,15.2,-10.476443753));
#154580=CARTESIAN_POINT('Ctrl Pts',(0.309275075999944,15.2,-10.478040796));
#154581=CARTESIAN_POINT('Ctrl Pts',(0.309595398999944,15.2,-10.479645198));
#154582=CARTESIAN_POINT('Ctrl Pts',(0.309918754999944,15.2,-10.481256934));
#154583=CARTESIAN_POINT('Ctrl Pts',(0.310245152999944,15.2,-10.482875987));
#154584=CARTESIAN_POINT('Ctrl Pts',(0.310574601999944,15.2,-10.484502335));
#154585=CARTESIAN_POINT('Ctrl Pts',(0.310907112999944,15.2,-10.486135957));
#154586=CARTESIAN_POINT('Ctrl Pts',(0.311242694999944,15.2,-10.487776833));
#154587=CARTESIAN_POINT('Ctrl Pts',(0.311581355999945,15.2,-10.489424943));
#154588=CARTESIAN_POINT('Ctrl Pts',(0.311923106999944,15.2,-10.491080266));
#154589=CARTESIAN_POINT('Ctrl Pts',(0.312267955999944,15.2,-10.492742782));
#154590=CARTESIAN_POINT('Ctrl Pts',(0.312615911999944,15.2,-10.494412473));
#154591=CARTESIAN_POINT('Ctrl Pts',(0.312966985999944,15.2,-10.496089316));
#154592=CARTESIAN_POINT('Ctrl Pts',(0.313321185999945,15.2,-10.497773293));
#154593=CARTESIAN_POINT('Ctrl Pts',(0.313678518999945,15.2,-10.499464382));
#154594=CARTESIAN_POINT('Ctrl Pts',(0.314038995999945,15.2,-10.501162565));
#154595=CARTESIAN_POINT('Ctrl Pts',(0.314402626999944,15.2,-10.502867822));
#154596=CARTESIAN_POINT('Ctrl Pts',(0.314769418999944,15.2,-10.504580133));
#154597=CARTESIAN_POINT('Ctrl Pts',(0.315139380999945,15.2,-10.506299478));
#154598=CARTESIAN_POINT('Ctrl Pts',(0.315512523999945,15.2,-10.508025838));
#154599=CARTESIAN_POINT('Ctrl Pts',(0.315888853999944,15.2,-10.509759194));
#154600=CARTESIAN_POINT('Ctrl Pts',(0.316268379999943,15.2,-10.511499525));
#154601=CARTESIAN_POINT('Ctrl Pts',(0.316651111999944,15.2,-10.513246812));
#154602=CARTESIAN_POINT('Ctrl Pts',(0.317037058999944,15.2,-10.515001037));
#154603=CARTESIAN_POINT('Ctrl Pts',(0.317426227999944,15.2,-10.516762179));
#154604=CARTESIAN_POINT('Ctrl Pts',(0.317818627999945,15.2,-10.518530222));
#154605=CARTESIAN_POINT('Ctrl Pts',(0.318214267999943,15.2,-10.520305143));
#154606=CARTESIAN_POINT('Ctrl Pts',(0.318613155999945,15.2,-10.522086924));
#154607=CARTESIAN_POINT('Ctrl Pts',(0.319015301999944,15.2,-10.523875548));
#154608=CARTESIAN_POINT('Ctrl Pts',(0.319420711999945,15.2,-10.525670994));
#154609=CARTESIAN_POINT('Ctrl Pts',(0.319829394999944,15.2,-10.527473244));
#154610=CARTESIAN_POINT('Ctrl Pts',(0.320241359999944,15.2,-10.529282279));
#154611=CARTESIAN_POINT('Ctrl Pts',(0.320656615999945,15.2,-10.53109808));
#154612=CARTESIAN_POINT('Ctrl Pts',(0.321075168999944,15.2,-10.532920629));
#154613=CARTESIAN_POINT('Ctrl Pts',(0.321497027999945,15.2,-10.534749907));
#154614=CARTESIAN_POINT('Ctrl Pts',(0.321922202999945,15.2,-10.536585896));
#154615=CARTESIAN_POINT('Ctrl Pts',(0.322350699999945,15.2,-10.538428576));
#154616=CARTESIAN_POINT('Ctrl Pts',(0.322782527999944,15.2,-10.54027793));
#154617=CARTESIAN_POINT('Ctrl Pts',(0.323217693999943,15.2,-10.54213394));
#154618=CARTESIAN_POINT('Ctrl Pts',(0.323656205999944,15.2,-10.543996587));
#154619=CARTESIAN_POINT('Ctrl Pts',(0.324098074999943,15.2,-10.545865852));
#154620=CARTESIAN_POINT('Ctrl Pts',(0.324543303999943,15.2,-10.547741717));
#154621=CARTESIAN_POINT('Ctrl Pts',(0.324991904999944,15.2,-10.549624165));
#154622=CARTESIAN_POINT('Ctrl Pts',(0.325443882999944,15.2,-10.551513176));
#154623=CARTESIAN_POINT('Ctrl Pts',(0.325899247999945,15.2,-10.553408734));
#154624=CARTESIAN_POINT('Ctrl Pts',(0.326358006999945,15.2,-10.555310821));
#154625=CARTESIAN_POINT('Ctrl Pts',(0.326820166999945,15.2,-10.557219417));
#154626=CARTESIAN_POINT('Ctrl Pts',(0.327285734999944,15.2,-10.559134506));
#154627=CARTESIAN_POINT('Ctrl Pts',(0.327754721999945,15.2,-10.56105607));
#154628=CARTESIAN_POINT('Ctrl Pts',(0.328227131999944,15.2,-10.562984091));
#154629=CARTESIAN_POINT('Ctrl Pts',(0.328702974999944,15.2,-10.56491855));
#154630=CARTESIAN_POINT('Ctrl Pts',(0.329182255999945,15.2,-10.566859432));
#154631=CARTESIAN_POINT('Ctrl Pts',(0.329664984999944,15.2,-10.568806718));
#154632=CARTESIAN_POINT('Ctrl Pts',(0.330151167999944,15.2,-10.57076039));
#154633=CARTESIAN_POINT('Ctrl Pts',(0.330640813999944,15.2,-10.572720431));
#154634=CARTESIAN_POINT('Ctrl Pts',(0.331133927999945,15.2,-10.574686823));
#154635=CARTESIAN_POINT('Ctrl Pts',(0.331630518999945,15.2,-10.57665955));
#154636=CARTESIAN_POINT('Ctrl Pts',(0.332130593999944,15.2,-10.578638595));
#154637=CARTESIAN_POINT('Ctrl Pts',(0.332634160999945,15.2,-10.580623937));
#154638=CARTESIAN_POINT('Ctrl Pts',(0.333141224999943,15.2,-10.582615564));
#154639=CARTESIAN_POINT('Ctrl Pts',(0.333651795999945,15.2,-10.584613455));
#154640=CARTESIAN_POINT('Ctrl Pts',(0.334165878999944,15.2,-10.586617594));
#154641=CARTESIAN_POINT('Ctrl Pts',(0.334683482999945,15.2,-10.588627965));
#154642=CARTESIAN_POINT('Ctrl Pts',(0.335204611999943,15.2,-10.59064455));
#154643=CARTESIAN_POINT('Ctrl Pts',(0.335729277999944,15.2,-10.592667332));
#154644=CARTESIAN_POINT('Ctrl Pts',(0.336257482999944,15.2,-10.594696293));
#154645=CARTESIAN_POINT('Ctrl Pts',(0.336789236999945,15.2,-10.59673142));
#154646=CARTESIAN_POINT('Ctrl Pts',(0.337324545999945,15.2,-10.598772692));
#154647=CARTESIAN_POINT('Ctrl Pts',(0.337863417999945,15.2,-10.600820093));
#154648=CARTESIAN_POINT('Ctrl Pts',(0.338405857999945,15.2,-10.602873609));
#154649=CARTESIAN_POINT('Ctrl Pts',(0.338951873999944,15.2,-10.60493322));
#154650=CARTESIAN_POINT('Ctrl Pts',(0.339501472999943,15.2,-10.606998913));
#154651=CARTESIAN_POINT('Ctrl Pts',(0.340054661999943,15.2,-10.609070667));
#154652=CARTESIAN_POINT('Ctrl Pts',(0.340611446999944,15.2,-10.611148469));
#154653=CARTESIAN_POINT('Ctrl Pts',(0.341171834999944,15.2,-10.613232302));
#154654=CARTESIAN_POINT('Ctrl Pts',(0.341735832999944,15.2,-10.615322148));
#154655=CARTESIAN_POINT('Ctrl Pts',(0.342303446999944,15.2,-10.617417992));
#154656=CARTESIAN_POINT('Ctrl Pts',(0.342874684999943,15.2,-10.619519817));
#154657=CARTESIAN_POINT('Ctrl Pts',(0.343449551999945,15.2,-10.621627608));
#154658=CARTESIAN_POINT('Ctrl Pts',(0.344028054999944,15.2,-10.623741347));
#154659=CARTESIAN_POINT('Ctrl Pts',(0.344610201999943,15.2,-10.625861018));
#154660=CARTESIAN_POINT('Ctrl Pts',(0.345195997999944,15.2,-10.627986606));
#154661=CARTESIAN_POINT('Ctrl Pts',(0.345785448999945,15.2,-10.630118095));
#154662=CARTESIAN_POINT('Ctrl Pts',(0.346378563999944,15.2,-10.632255468));
#154663=CARTESIAN_POINT('Ctrl Pts',(0.346975346999944,15.2,-10.634398708));
#154664=CARTESIAN_POINT('Ctrl Pts',(0.347575804999943,15.2,-10.636547803));
#154665=CARTESIAN_POINT('Ctrl Pts',(0.348179944999943,15.2,-10.638702732));
#154666=CARTESIAN_POINT('Ctrl Pts',(0.348787772999944,15.2,-10.640863483));
#154667=CARTESIAN_POINT('Ctrl Pts',(0.349399294999945,15.2,-10.643030038));
#154668=CARTESIAN_POINT('Ctrl Pts',(0.350014516999944,15.2,-10.645202383));
#154669=CARTESIAN_POINT('Ctrl Pts',(0.350633445999945,15.2,-10.647380501));
#154670=CARTESIAN_POINT('Ctrl Pts',(0.351256087999945,15.2,-10.649564376));
#154671=CARTESIAN_POINT('Ctrl Pts',(0.351882449999945,15.2,-10.651753993));
#154672=CARTESIAN_POINT('Ctrl Pts',(0.352512535999944,15.2,-10.653949337));
#154673=CARTESIAN_POINT('Ctrl Pts',(0.353146353999945,15.2,-10.656150391));
#154674=CARTESIAN_POINT('Ctrl Pts',(0.353783908999944,15.2,-10.658357141));
#154675=CARTESIAN_POINT('Ctrl Pts',(0.354425208999943,15.2,-10.660569571));
#154676=CARTESIAN_POINT('Ctrl Pts',(0.355070257999944,15.2,-10.662787664));
#154677=CARTESIAN_POINT('Ctrl Pts',(0.355719062999944,15.2,-10.665011407));
#154678=CARTESIAN_POINT('Ctrl Pts',(0.356371629999943,15.2,-10.667240784));
#154679=CARTESIAN_POINT('Ctrl Pts',(0.357027963999944,15.2,-10.669475778));
#154680=CARTESIAN_POINT('Ctrl Pts',(0.357688070999943,15.2,-10.671716375));
#154681=CARTESIAN_POINT('Ctrl Pts',(0.358351957999944,15.2,-10.673962561));
#154682=CARTESIAN_POINT('Ctrl Pts',(0.359019631999944,15.2,-10.676214319));
#154683=CARTESIAN_POINT('Ctrl Pts',(0.359691094999944,15.2,-10.678471635));
#154684=CARTESIAN_POINT('Ctrl Pts',(0.360366356999944,15.2,-10.680734493));
#154685=CARTESIAN_POINT('Ctrl Pts',(0.361045420999944,15.2,-10.683002879));
#154686=CARTESIAN_POINT('Ctrl Pts',(0.361728292999944,15.2,-10.685276775));
#154687=CARTESIAN_POINT('Ctrl Pts',(0.362414979999944,15.2,-10.687556171));
#154688=CARTESIAN_POINT('Ctrl Pts',(0.363105486999944,15.2,-10.689841047));
#154689=CARTESIAN_POINT('Ctrl Pts',(0.363799819999944,15.2,-10.692131392));
#154690=CARTESIAN_POINT('Ctrl Pts',(0.364497983999945,15.2,-10.69442719));
#154691=CARTESIAN_POINT('Ctrl Pts',(0.365199985999943,15.2,-10.696728424));
#154692=CARTESIAN_POINT('Ctrl Pts',(0.365905829999944,15.2,-10.699035082));
#154693=CARTESIAN_POINT('Ctrl Pts',(0.366615521999943,15.2,-10.701347148));
#154694=CARTESIAN_POINT('Ctrl Pts',(0.367329068999943,15.2,-10.703664607));
#154695=CARTESIAN_POINT('Ctrl Pts',(0.368046474999945,15.2,-10.705987445));
#154696=CARTESIAN_POINT('Ctrl Pts',(0.368767745999945,15.2,-10.708315648));
#154697=CARTESIAN_POINT('Ctrl Pts',(0.369492886999945,15.2,-10.710649199));
#154698=CARTESIAN_POINT('Ctrl Pts',(0.370221902999944,15.2,-10.712988086));
#154699=CARTESIAN_POINT('Ctrl Pts',(0.370954801999943,15.2,-10.715332293));
#154700=CARTESIAN_POINT('Ctrl Pts',(0.371691585999944,15.2,-10.717681807));
#154701=CARTESIAN_POINT('Ctrl Pts',(0.372432262999943,15.2,-10.720036612));
#154702=CARTESIAN_POINT('Ctrl Pts',(0.373176837999944,15.2,-10.722396693));
#154703=CARTESIAN_POINT('Ctrl Pts',(0.373925314999944,15.2,-10.724762038));
#154704=CARTESIAN_POINT('Ctrl Pts',(0.374677699999945,15.2,-10.72713263));
#154705=CARTESIAN_POINT('Ctrl Pts',(0.375433997999943,15.2,-10.729508457));
#154706=CARTESIAN_POINT('Ctrl Pts',(0.376194214999943,15.2,-10.731889504));
#154707=CARTESIAN_POINT('Ctrl Pts',(0.376958354999944,15.2,-10.734275757));
#154708=CARTESIAN_POINT('Ctrl Pts',(0.377726424999943,15.2,-10.7366672));
#154709=CARTESIAN_POINT('Ctrl Pts',(0.378498428999944,15.2,-10.73906382));
#154710=CARTESIAN_POINT('Ctrl Pts',(0.379274372999945,15.2,-10.741465604));
#154711=CARTESIAN_POINT('Ctrl Pts',(0.380054259999945,15.2,-10.743872536));
#154712=CARTESIAN_POINT('Ctrl Pts',(0.380838096999945,15.2,-10.746284604));
#154713=CARTESIAN_POINT('Ctrl Pts',(0.381625889999944,15.2,-10.748701792));
#154714=CARTESIAN_POINT('Ctrl Pts',(0.382417640999944,15.2,-10.751124087));
#154715=CARTESIAN_POINT('Ctrl Pts',(0.383213356999944,15.2,-10.753551475));
#154716=CARTESIAN_POINT('Ctrl Pts',(0.384013043999945,15.2,-10.755983942));
#154717=CARTESIAN_POINT('Ctrl Pts',(0.384816703999944,15.2,-10.758421474));
#154718=CARTESIAN_POINT('Ctrl Pts',(0.385624345999943,15.2,-10.760864057));
#154719=CARTESIAN_POINT('Ctrl Pts',(0.386435970999944,15.2,-10.763311678));
#154720=CARTESIAN_POINT('Ctrl Pts',(0.387251585999945,15.2,-10.765764322));
#154721=CARTESIAN_POINT('Ctrl Pts',(0.388071194999944,15.2,-10.768221976));
#154722=CARTESIAN_POINT('Ctrl Pts',(0.388894804999945,15.2,-10.770684626));
#154723=CARTESIAN_POINT('Ctrl Pts',(0.389722417999945,15.2,-10.773152259));
#154724=CARTESIAN_POINT('Ctrl Pts',(0.390554040999945,15.2,-10.77562486));
#154725=CARTESIAN_POINT('Ctrl Pts',(0.391389675999945,15.2,-10.778102417));
#154726=CARTESIAN_POINT('Ctrl Pts',(0.392229331999945,15.2,-10.780584915));
#154727=CARTESIAN_POINT('Ctrl Pts',(0.393073008999943,15.2,-10.78307234));
#154728=CARTESIAN_POINT('Ctrl Pts',(0.393920715999944,15.2,-10.785564681));
#154729=CARTESIAN_POINT('Ctrl Pts',(0.394772454999943,15.2,-10.788061922));
#154730=CARTESIAN_POINT('Ctrl Pts',(0.395628231999944,15.2,-10.790564051));
#154731=CARTESIAN_POINT('Ctrl Pts',(0.396488050999944,15.2,-10.793071054));
#154732=CARTESIAN_POINT('Ctrl Pts',(0.397351916999943,15.2,-10.795582918));
#154733=CARTESIAN_POINT('Ctrl Pts',(0.398219834999944,15.2,-10.798099629));
#154734=CARTESIAN_POINT('Ctrl Pts',(0.399091808999945,15.2,-10.800621174));
#154735=CARTESIAN_POINT('Ctrl Pts',(0.399967842999944,15.2,-10.80314754));
#154736=CARTESIAN_POINT('Ctrl Pts',(0.400847942999943,15.2,-10.805678712));
#154737=CARTESIAN_POINT('Ctrl Pts',(0.401732111999945,15.2,-10.808214679));
#154738=CARTESIAN_POINT('Ctrl Pts',(0.402620355999943,15.2,-10.810755427));
#154739=CARTESIAN_POINT('Ctrl Pts',(0.403512678999943,15.2,-10.813300943));
#154740=CARTESIAN_POINT('Ctrl Pts',(0.404409085999945,15.2,-10.815851213));
#154741=CARTESIAN_POINT('Ctrl Pts',(0.405309579999944,15.2,-10.818406225));
#154742=CARTESIAN_POINT('Ctrl Pts',(0.406214165999945,15.2,-10.820965964));
#154743=CARTESIAN_POINT('Ctrl Pts',(0.407122848999943,15.2,-10.82353042));
#154744=CARTESIAN_POINT('Ctrl Pts',(0.408035631999945,15.2,-10.826099577));
#154745=CARTESIAN_POINT('Ctrl Pts',(0.408952521999945,15.2,-10.828673424));
#154746=CARTESIAN_POINT('Ctrl Pts',(0.409873521999945,15.2,-10.831251946));
#154747=CARTESIAN_POINT('Ctrl Pts',(0.410798634999944,15.2,-10.833835132));
#154748=CARTESIAN_POINT('Ctrl Pts',(0.411727865999945,15.2,-10.836422969));
#154749=CARTESIAN_POINT('Ctrl Pts',(0.412661221999944,15.2,-10.839015443));
#154750=CARTESIAN_POINT('Ctrl Pts',(0.413598702999943,15.2,-10.841612542));
#154751=CARTESIAN_POINT('Ctrl Pts',(0.414540315999944,15.2,-10.844214253));
#154752=CARTESIAN_POINT('Ctrl Pts',(0.415486064999945,15.2,-10.846820562));
#154753=CARTESIAN_POINT('Ctrl Pts',(0.416435952999944,15.2,-10.849431457));
#154754=CARTESIAN_POINT('Ctrl Pts',(0.417389984999945,15.2,-10.852046927));
#154755=CARTESIAN_POINT('Ctrl Pts',(0.418348164999944,15.2,-10.854666958));
#154756=CARTESIAN_POINT('Ctrl Pts',(0.419310496999945,15.2,-10.857291535));
#154757=CARTESIAN_POINT('Ctrl Pts',(0.420276985999944,15.2,-10.859920649));
#154758=CARTESIAN_POINT('Ctrl Pts',(0.421247635999944,15.2,-10.862554285));
#154759=CARTESIAN_POINT('Ctrl Pts',(0.422222449999945,15.2,-10.865192432));
#154760=CARTESIAN_POINT('Ctrl Pts',(0.423201432999945,15.2,-10.867835076));
#154761=CARTESIAN_POINT('Ctrl Pts',(0.424184586999944,15.2,-10.870482205));
#154762=CARTESIAN_POINT('Ctrl Pts',(0.425171919999944,15.2,-10.873133806));
#154763=CARTESIAN_POINT('Ctrl Pts',(0.426163432999944,15.2,-10.875789868));
#154764=CARTESIAN_POINT('Ctrl Pts',(0.427159130999945,15.2,-10.878450378));
#154765=CARTESIAN_POINT('Ctrl Pts',(0.428159016999944,15.2,-10.881115322));
#154766=CARTESIAN_POINT('Ctrl Pts',(0.429163096999944,15.2,-10.883784689));
#154767=CARTESIAN_POINT('Ctrl Pts',(0.430171372999943,15.2,-10.886458467));
#154768=CARTESIAN_POINT('Ctrl Pts',(0.431183849999943,15.2,-10.889136642));
#154769=CARTESIAN_POINT('Ctrl Pts',(0.432200529999944,15.2,-10.891819203));
#154770=CARTESIAN_POINT('Ctrl Pts',(0.433221419999944,15.2,-10.894506138));
#154771=CARTESIAN_POINT('Ctrl Pts',(0.434246522999944,15.2,-10.897197434));
#154772=CARTESIAN_POINT('Ctrl Pts',(0.435275840999945,15.2,-10.899893077));
#154773=CARTESIAN_POINT('Ctrl Pts',(0.436309378999944,15.2,-10.902593058));
#154774=CARTESIAN_POINT('Ctrl Pts',(0.437347139999943,15.2,-10.905297364));
#154775=CARTESIAN_POINT('Ctrl Pts',(0.438389128999944,15.2,-10.908005981));
#154776=CARTESIAN_POINT('Ctrl Pts',(0.439435350999944,15.2,-10.910718898));
#154777=CARTESIAN_POINT('Ctrl Pts',(0.440485805999945,15.2,-10.913436104));
#154778=CARTESIAN_POINT('Ctrl Pts',(0.441540500999944,15.2,-10.916157585));
#154779=CARTESIAN_POINT('Ctrl Pts',(0.442599438999943,15.2,-10.91888333));
#154780=CARTESIAN_POINT('Ctrl Pts',(0.443662621999945,15.2,-10.921613326));
#154781=CARTESIAN_POINT('Ctrl Pts',(0.444730055999945,15.2,-10.924347562));
#154782=CARTESIAN_POINT('Ctrl Pts',(0.445801742999944,15.2,-10.927086026));
#154783=CARTESIAN_POINT('Ctrl Pts',(0.446877687999944,15.2,-10.929828706));
#154784=CARTESIAN_POINT('Ctrl Pts',(0.447957893999943,15.2,-10.932575589));
#154785=CARTESIAN_POINT('Ctrl Pts',(0.449042363999944,15.2,-10.935326664));
#154786=CARTESIAN_POINT('Ctrl Pts',(0.450131101999943,15.2,-10.93808192));
#154787=CARTESIAN_POINT('Ctrl Pts',(0.451224112999944,15.2,-10.940841343));
#154788=CARTESIAN_POINT('Ctrl Pts',(0.452321397999944,15.2,-10.943604921));
#154789=CARTESIAN_POINT('Ctrl Pts',(0.453422961999944,15.2,-10.946372645));
#154790=CARTESIAN_POINT('Ctrl Pts',(0.454528808999944,15.2,-10.949144502));
#154791=CARTESIAN_POINT('Ctrl Pts',(0.455638941999944,15.2,-10.951920478));
#154792=CARTESIAN_POINT('Ctrl Pts',(0.456753363999944,15.2,-10.954700564));
#154793=CARTESIAN_POINT('Ctrl Pts',(0.457872078999945,15.2,-10.957484747));
#154794=CARTESIAN_POINT('Ctrl Pts',(0.458995090999944,15.2,-10.960273016));
#154795=CARTESIAN_POINT('Ctrl Pts',(0.460122400999945,15.2,-10.963065359));
#154796=CARTESIAN_POINT('Ctrl Pts',(0.461254015999945,15.2,-10.965861764));
#154797=CARTESIAN_POINT('Ctrl Pts',(0.462389937999944,15.2,-10.96866222));
#154798=CARTESIAN_POINT('Ctrl Pts',(0.463530168999944,15.2,-10.971466714));
#154799=CARTESIAN_POINT('Ctrl Pts',(0.464674712999944,15.2,-10.974275237));
#154800=CARTESIAN_POINT('Ctrl Pts',(0.465823575999943,15.2,-10.977087774));
#154801=CARTESIAN_POINT('Ctrl Pts',(0.466976756999945,15.2,-10.979904316));
#154802=CARTESIAN_POINT('Ctrl Pts',(0.468134261999945,15.2,-10.982724852));
#154803=CARTESIAN_POINT('Ctrl Pts',(0.469296094999944,15.2,-10.985549368));
#154804=CARTESIAN_POINT('Ctrl Pts',(0.470462256999945,15.2,-10.988377854));
#154805=CARTESIAN_POINT('Ctrl Pts',(0.471632752999945,15.2,-10.991210298));
#154806=CARTESIAN_POINT('Ctrl Pts',(0.472807584999944,15.2,-10.994046689));
#154807=CARTESIAN_POINT('Ctrl Pts',(0.473986757999943,15.2,-10.996887016));
#154808=CARTESIAN_POINT('Ctrl Pts',(0.475170271999945,15.2,-10.999731268));
#154809=CARTESIAN_POINT('Ctrl Pts',(0.476358134999944,15.2,-11.002579431));
#154810=CARTESIAN_POINT('Ctrl Pts',(0.477550345999944,15.2,-11.005431497));
#154811=CARTESIAN_POINT('Ctrl Pts',(0.478746909999943,15.2,-11.008287453));
#154812=CARTESIAN_POINT('Ctrl Pts',(0.479947829999944,15.2,-11.011147287));
#154813=CARTESIAN_POINT('Ctrl Pts',(0.481153109999944,15.2,-11.014010988));
#154814=CARTESIAN_POINT('Ctrl Pts',(0.482362750999944,15.2,-11.016878547));
#154815=CARTESIAN_POINT('Ctrl Pts',(0.483576757999945,15.2,-11.01974995));
#154816=CARTESIAN_POINT('Ctrl Pts',(0.484795132999943,15.2,-11.022625188));
#154817=CARTESIAN_POINT('Ctrl Pts',(0.486017879999944,15.2,-11.025504247));
#154818=CARTESIAN_POINT('Ctrl Pts',(0.487245001999945,15.2,-11.028387119));
#154819=CARTESIAN_POINT('Ctrl Pts',(0.488476501999945,15.2,-11.031273791));
#154820=CARTESIAN_POINT('Ctrl Pts',(0.489712381999944,15.2,-11.034164252));
#154821=CARTESIAN_POINT('Ctrl Pts',(0.490952645999944,15.2,-11.037058491));
#154822=CARTESIAN_POINT('Ctrl Pts',(0.492197297999944,15.2,-11.039956497));
#154823=CARTESIAN_POINT('Ctrl Pts',(0.493446337999943,15.2,-11.04285826));
#154824=CARTESIAN_POINT('Ctrl Pts',(0.494699771999944,15.2,-11.045763768));
#154825=CARTESIAN_POINT('Ctrl Pts',(0.495957600999944,15.2,-11.04867301));
#154826=CARTESIAN_POINT('Ctrl Pts',(0.497219829999944,15.2,-11.051585974));
#154827=CARTESIAN_POINT('Ctrl Pts',(0.498486459999944,15.2,-11.05450265));
#154828=CARTESIAN_POINT('Ctrl Pts',(0.499757494999944,15.2,-11.057423028));
#154829=CARTESIAN_POINT('Ctrl Pts',(0.501032935999944,15.2,-11.060347096));
#154830=CARTESIAN_POINT('Ctrl Pts',(0.502312788999945,15.2,-11.063274844));
#154831=CARTESIAN_POINT('Ctrl Pts',(0.503597054999945,15.2,-11.066206259));
#154832=CARTESIAN_POINT('Ctrl Pts',(0.504885736999944,15.2,-11.069141332));
#154833=CARTESIAN_POINT('Ctrl Pts',(0.506178838999943,15.2,-11.072080052));
#154834=CARTESIAN_POINT('Ctrl Pts',(0.507476362999945,15.2,-11.075022407));
#154835=CARTESIAN_POINT('Ctrl Pts',(0.508778309999944,15.2,-11.077968387));
#154836=CARTESIAN_POINT('Ctrl Pts',(0.510084685999944,15.2,-11.080917982));
#154837=CARTESIAN_POINT('Ctrl Pts',(0.511395492999944,15.2,-11.08387118));
#154838=CARTESIAN_POINT('Ctrl Pts',(0.512710730999945,15.2,-11.086827972));
#154839=CARTESIAN_POINT('Ctrl Pts',(0.514030406999945,15.2,-11.089788344));
#154840=CARTESIAN_POINT('Ctrl Pts',(0.515354519999944,15.2,-11.092752289));
#154841=CARTESIAN_POINT('Ctrl Pts',(0.516683075999944,15.2,-11.095719793));
#154842=CARTESIAN_POINT('Ctrl Pts',(0.518016074999944,15.2,-11.098690848));
#154843=CARTESIAN_POINT('Ctrl Pts',(0.519353520999944,15.2,-11.101665441));
#154844=CARTESIAN_POINT('Ctrl Pts',(0.520695416999944,15.2,-11.104643564));
#154845=CARTESIAN_POINT('Ctrl Pts',(0.522041764999944,15.2,-11.107625205));
#154846=CARTESIAN_POINT('Ctrl Pts',(0.523392567999944,15.2,-11.110610353));
#154847=CARTESIAN_POINT('Ctrl Pts',(0.524747828999944,15.2,-11.113598997));
#154848=CARTESIAN_POINT('Ctrl Pts',(0.526107550999945,15.2,-11.116591128));
#154849=CARTESIAN_POINT('Ctrl Pts',(0.527471734999944,15.2,-11.119586735));
#154850=CARTESIAN_POINT('Ctrl Pts',(0.528840383999943,15.2,-11.122585808));
#154851=CARTESIAN_POINT('Ctrl Pts',(0.530213500999944,15.2,-11.125588334));
#154852=CARTESIAN_POINT('Ctrl Pts',(0.531591089999944,15.2,-11.128594306));
#154853=CARTESIAN_POINT('Ctrl Pts',(0.532973150999945,15.2,-11.131603711));
#154854=CARTESIAN_POINT('Ctrl Pts',(0.534359687999945,15.2,-11.13461654));
#154855=CARTESIAN_POINT('Ctrl Pts',(0.535750703999944,15.2,-11.137632781));
#154856=CARTESIAN_POINT('Ctrl Pts',(0.537146200999944,15.2,-11.140652425));
#154857=CARTESIAN_POINT('Ctrl Pts',(0.538546180999945,15.2,-11.143675461));
#154858=CARTESIAN_POINT('Ctrl Pts',(0.539950646999944,15.2,-11.146701879));
#154859=CARTESIAN_POINT('Ctrl Pts',(0.541359600999944,15.2,-11.149731669));
#154860=CARTESIAN_POINT('Ctrl Pts',(0.542773046999944,15.2,-11.152764819));
#154861=CARTESIAN_POINT('Ctrl Pts',(0.544190985999945,15.2,-11.155801321));
#154862=CARTESIAN_POINT('Ctrl Pts',(0.545613420999944,15.2,-11.158841164));
#154863=CARTESIAN_POINT('Ctrl Pts',(0.547040353999945,15.2,-11.161884336));
#154864=CARTESIAN_POINT('Ctrl Pts',(0.548471787999943,15.2,-11.164930828));
#154865=CARTESIAN_POINT('Ctrl Pts',(0.549907724999944,15.2,-11.167980631));
#154866=CARTESIAN_POINT('Ctrl Pts',(0.551348166999944,15.2,-11.171033733));
#154867=CARTESIAN_POINT('Ctrl Pts',(0.552793118999944,15.2,-11.174090123));
#154868=CARTESIAN_POINT('Ctrl Pts',(0.554242579999944,15.2,-11.177149794));
#154869=CARTESIAN_POINT('Ctrl Pts',(0.555696552999944,15.2,-11.180212734));
#154870=CARTESIAN_POINT('Ctrl Pts',(0.557155042999944,15.2,-11.183278932));
#154871=CARTESIAN_POINT('Ctrl Pts',(0.558618047999944,15.2,-11.186348379));
#154872=CARTESIAN_POINT('Ctrl Pts',(0.560085574999943,15.2,-11.189421065));
#154873=CARTESIAN_POINT('Ctrl Pts',(0.561557623999944,15.2,-11.192496979));
#154874=CARTESIAN_POINT('Ctrl Pts',(0.563034195999944,15.2,-11.195576112));
#154875=CARTESIAN_POINT('Ctrl Pts',(0.564515294999944,15.2,-11.198658453));
#154876=CARTESIAN_POINT('Ctrl Pts',(0.566000922999944,15.2,-11.201743993));
#154877=CARTESIAN_POINT('Ctrl Pts',(0.567491082999945,15.2,-11.204832721));
#154878=CARTESIAN_POINT('Ctrl Pts',(0.568985775999944,15.2,-11.207924627));
#154879=CARTESIAN_POINT('Ctrl Pts',(0.570485004999944,15.2,-11.211019702));
#154880=CARTESIAN_POINT('Ctrl Pts',(0.571988771999944,15.2,-11.214117935));
#154881=CARTESIAN_POINT('Ctrl Pts',(0.573497078999944,15.2,-11.217219316));
#154882=CARTESIAN_POINT('Ctrl Pts',(0.575009928999944,15.2,-11.220323837));
#154883=CARTESIAN_POINT('Ctrl Pts',(0.576527321999943,15.2,-11.223431485));
#154884=CARTESIAN_POINT('Ctrl Pts',(0.578049262999943,15.2,-11.226542253));
#154885=CARTESIAN_POINT('Ctrl Pts',(0.579575752999945,15.2,-11.229656128));
#154886=CARTESIAN_POINT('Ctrl Pts',(0.581106792999945,15.2,-11.232773103));
#154887=CARTESIAN_POINT('Ctrl Pts',(0.582642387999944,15.2,-11.235893168));
#154888=CARTESIAN_POINT('Ctrl Pts',(0.584182536999944,15.2,-11.23901631));
#154889=CARTESIAN_POINT('Ctrl Pts',(0.585727243999944,15.2,-11.242142523));
#154890=CARTESIAN_POINT('Ctrl Pts',(0.587276510999944,15.2,-11.245271795));
#154891=CARTESIAN_POINT('Ctrl Pts',(0.588830339999945,15.2,-11.248404117));
#154892=CARTESIAN_POINT('Ctrl Pts',(0.590388730999944,15.2,-11.251539479));
#154893=CARTESIAN_POINT('Ctrl Pts',(0.591951689999944,15.2,-11.254677871));
#154894=CARTESIAN_POINT('Ctrl Pts',(0.593519214999944,15.2,-11.257819284));
#154895=CARTESIAN_POINT('Ctrl Pts',(0.595091311999945,15.2,-11.260963707));
#154896=CARTESIAN_POINT('Ctrl Pts',(0.596667979999944,15.2,-11.264111132));
#154897=CARTESIAN_POINT('Ctrl Pts',(0.598249221999944,15.2,-11.267261548));
#154898=CARTESIAN_POINT('Ctrl Pts',(0.599835039999944,15.2,-11.270414946));
#154899=CARTESIAN_POINT('Ctrl Pts',(0.601425436999944,15.2,-11.273571316));
#154900=CARTESIAN_POINT('Ctrl Pts',(0.603020412999945,15.2,-11.276730648));
#154901=CARTESIAN_POINT('Ctrl Pts',(0.604619971999945,15.2,-11.279892934));
#154902=CARTESIAN_POINT('Ctrl Pts',(0.606224114999944,15.2,-11.283058161));
#154903=CARTESIAN_POINT('Ctrl Pts',(0.607832842999944,15.2,-11.286226323));
#154904=CARTESIAN_POINT('Ctrl Pts',(0.609446159999945,15.2,-11.289397409));
#154905=CARTESIAN_POINT('Ctrl Pts',(0.611064066999945,15.2,-11.29257141));
#154906=CARTESIAN_POINT('Ctrl Pts',(0.612686564999944,15.2,-11.295748315));
#154907=CARTESIAN_POINT('Ctrl Pts',(0.614313656999944,15.2,-11.298928116));
#154908=CARTESIAN_POINT('Ctrl Pts',(0.615945344999944,15.2,-11.302110802));
#154909=CARTESIAN_POINT('Ctrl Pts',(0.617581629999945,15.2,-11.305296365));
#154910=CARTESIAN_POINT('Ctrl Pts',(0.619222514999944,15.2,-11.308484795));
#154911=CARTESIAN_POINT('Ctrl Pts',(0.620868000999945,15.2,-11.311676082));
#154912=CARTESIAN_POINT('Ctrl Pts',(0.622518089999944,15.2,-11.314870217));
#154913=CARTESIAN_POINT('Ctrl Pts',(0.624172783999944,15.2,-11.31806719));
#154914=CARTESIAN_POINT('Ctrl Pts',(0.625832085999944,15.2,-11.321266994));
#154915=CARTESIAN_POINT('Ctrl Pts',(0.627495994999945,15.2,-11.324469616));
#154916=CARTESIAN_POINT('Ctrl Pts',(0.629164515999945,15.2,-11.327675049));
#154917=CARTESIAN_POINT('Ctrl Pts',(0.630837647999944,15.2,-11.330883282));
#154918=CARTESIAN_POINT('Ctrl Pts',(0.632515393999945,15.2,-11.334094307));
#154919=CARTESIAN_POINT('Ctrl Pts',(0.634197756999945,15.2,-11.337308115));
#154920=CARTESIAN_POINT('Ctrl Pts',(0.635884736999944,15.2,-11.340524695));
#154921=CARTESIAN_POINT('Ctrl Pts',(0.637576336999944,15.2,-11.343744038));
#154922=CARTESIAN_POINT('Ctrl Pts',(0.639272556999945,15.2,-11.346966135));
#154923=CARTESIAN_POINT('Ctrl Pts',(0.640973400999945,15.2,-11.350190979));
#154924=CARTESIAN_POINT('Ctrl Pts',(0.642678868999944,15.2,-11.353418557));
#154925=CARTESIAN_POINT('Ctrl Pts',(0.644388963999944,15.2,-11.356648862));
#154926=CARTESIAN_POINT('Ctrl Pts',(0.646103685999945,15.2,-11.359881884));
#154927=CARTESIAN_POINT('Ctrl Pts',(0.647823038999944,15.2,-11.363117614));
#154928=CARTESIAN_POINT('Ctrl Pts',(0.649547021999944,15.2,-11.366356043));
#154929=CARTESIAN_POINT('Ctrl Pts',(0.651275639999944,15.2,-11.369597161));
#154930=CARTESIAN_POINT('Ctrl Pts',(0.653008890999944,15.2,-11.37284096));
#154931=CARTESIAN_POINT('Ctrl Pts',(0.654746778999944,15.2,-11.37608743));
#154932=CARTESIAN_POINT('Ctrl Pts',(0.656489305999944,15.2,-11.379336561));
#154933=CARTESIAN_POINT('Ctrl Pts',(0.658236471999943,15.2,-11.382588345));
#154934=CARTESIAN_POINT('Ctrl Pts',(0.659988278999944,15.2,-11.385842772));
#154935=CARTESIAN_POINT('Ctrl Pts',(0.661744729999943,15.2,-11.389099835));
#154936=CARTESIAN_POINT('Ctrl Pts',(0.663505824999944,15.2,-11.392359523));
#154937=CARTESIAN_POINT('Ctrl Pts',(0.665271565999944,15.2,-11.395621827));
#154938=CARTESIAN_POINT('Ctrl Pts',(0.667041954999944,15.2,-11.39888674));
#154939=CARTESIAN_POINT('Ctrl Pts',(0.668816992999944,15.2,-11.402154251));
#154940=CARTESIAN_POINT('Ctrl Pts',(0.670596681999944,15.2,-11.405424352));
#154941=CARTESIAN_POINT('Ctrl Pts',(0.672381022999944,15.2,-11.408697032));
#154942=CARTESIAN_POINT('Ctrl Pts',(0.674170018999944,15.2,-11.411972283));
#154943=CARTESIAN_POINT('Ctrl Pts',(0.675963669999944,15.2,-11.415250096));
#154944=CARTESIAN_POINT('Ctrl Pts',(0.677761977999943,15.2,-11.418530461));
#154945=CARTESIAN_POINT('Ctrl Pts',(0.679564944999944,15.2,-11.421813369));
#154946=CARTESIAN_POINT('Ctrl Pts',(0.681372572999944,15.2,-11.425098811));
#154947=CARTESIAN_POINT('Ctrl Pts',(0.683184861999945,15.2,-11.42838678));
#154948=CARTESIAN_POINT('Ctrl Pts',(0.685001812999944,15.2,-11.431677269));
#154949=CARTESIAN_POINT('Ctrl Pts',(0.686823428999944,15.2,-11.434970268));
#154950=CARTESIAN_POINT('Ctrl Pts',(0.688649710999945,15.2,-11.438265769));
#154951=CARTESIAN_POINT('Ctrl Pts',(0.690480658999945,15.2,-11.441563763));
#154952=CARTESIAN_POINT('Ctrl Pts',(0.692316276999944,15.2,-11.444864239));
#154953=CARTESIAN_POINT('Ctrl Pts',(0.694156563999945,15.2,-11.448167187));
#154954=CARTESIAN_POINT('Ctrl Pts',(0.696001524999944,15.2,-11.451472595));
#154955=CARTESIAN_POINT('Ctrl Pts',(0.697851158999944,15.2,-11.454780453));
#154956=CARTESIAN_POINT('Ctrl Pts',(0.699705468999944,15.2,-11.458090751));
#154957=CARTESIAN_POINT('Ctrl Pts',(0.701564455999945,15.2,-11.461403481));
#154958=CARTESIAN_POINT('Ctrl Pts',(0.703428120999944,15.2,-11.464718637));
#154959=CARTESIAN_POINT('Ctrl Pts',(0.705296462999944,15.2,-11.468036216));
#154960=CARTESIAN_POINT('Ctrl Pts',(0.707169485999944,15.2,-11.471356215));
#154961=CARTESIAN_POINT('Ctrl Pts',(0.708671644999944,15.2,-11.474014149));
#154962=CARTESIAN_POINT('Ctrl Pts',(0.709800370999945,15.2,-11.476008688));
#154963=CARTESIAN_POINT('Ctrl Pts',(0.710553790999944,15.2,-11.477338863));
#154964=CARTESIAN_POINT('Ctrl Pts',(0.710930733999944,15.2,-11.478004072));
#154965=CARTESIAN_POINT('Ctrl Pts',(0.292001928999944,12.2,-10.370890023));
#154966=CARTESIAN_POINT('Ctrl Pts',(0.292021795999944,12.2,-10.371063245));
#154967=CARTESIAN_POINT('Ctrl Pts',(0.292062308999944,12.2,-10.371415731));
#154968=CARTESIAN_POINT('Ctrl Pts',(0.292123960999945,12.2,-10.371949799));
#154969=CARTESIAN_POINT('Ctrl Pts',(0.292207546999944,12.2,-10.372669176));
#154970=CARTESIAN_POINT('Ctrl Pts',(0.292314179999943,12.2,-10.373578975));
#154971=CARTESIAN_POINT('Ctrl Pts',(0.292423468999944,12.2,-10.374503411));
#154972=CARTESIAN_POINT('Ctrl Pts',(0.292534811999945,12.2,-10.375437184));
#154973=CARTESIAN_POINT('Ctrl Pts',(0.292648222999944,12.2,-10.376380266));
#154974=CARTESIAN_POINT('Ctrl Pts',(0.292763716999945,12.2,-10.377332627));
#154975=CARTESIAN_POINT('Ctrl Pts',(0.292881308999944,12.2,-10.378294239));
#154976=CARTESIAN_POINT('Ctrl Pts',(0.293001014999945,12.2,-10.379265074));
#154977=CARTESIAN_POINT('Ctrl Pts',(0.293122845999945,12.2,-10.380245102));
#154978=CARTESIAN_POINT('Ctrl Pts',(0.293246819999944,12.2,-10.381234297));
#154979=CARTESIAN_POINT('Ctrl Pts',(0.293372948999944,12.2,-10.382232628));
#154980=CARTESIAN_POINT('Ctrl Pts',(0.293501248999943,12.2,-10.383240069));
#154981=CARTESIAN_POINT('Ctrl Pts',(0.293631731999945,12.2,-10.384256592));
#154982=CARTESIAN_POINT('Ctrl Pts',(0.293764412999945,12.2,-10.385282168));
#154983=CARTESIAN_POINT('Ctrl Pts',(0.293899306999944,12.2,-10.38631677));
#154984=CARTESIAN_POINT('Ctrl Pts',(0.294036426999943,12.2,-10.387360371));
#154985=CARTESIAN_POINT('Ctrl Pts',(0.294175786999944,12.2,-10.388412945));
#154986=CARTESIAN_POINT('Ctrl Pts',(0.294317400999944,12.2,-10.389474461));
#154987=CARTESIAN_POINT('Ctrl Pts',(0.294461281999944,12.2,-10.390544895));
#154988=CARTESIAN_POINT('Ctrl Pts',(0.294607443999944,12.2,-10.391624218));
#154989=CARTESIAN_POINT('Ctrl Pts',(0.294755900999943,12.2,-10.392712404));
#154990=CARTESIAN_POINT('Ctrl Pts',(0.294906665999944,12.2,-10.393809427));
#154991=CARTESIAN_POINT('Ctrl Pts',(0.295059751999943,12.2,-10.394915259));
#154992=CARTESIAN_POINT('Ctrl Pts',(0.295215172999944,12.2,-10.396029875));
#154993=CARTESIAN_POINT('Ctrl Pts',(0.295372941999944,12.2,-10.397153247));
#154994=CARTESIAN_POINT('Ctrl Pts',(0.295533071999945,12.2,-10.39828535));
#154995=CARTESIAN_POINT('Ctrl Pts',(0.295695575999944,12.2,-10.399426157));
#154996=CARTESIAN_POINT('Ctrl Pts',(0.295860466999944,12.2,-10.400575642));
#154997=CARTESIAN_POINT('Ctrl Pts',(0.296027758999945,12.2,-10.401733778));
#154998=CARTESIAN_POINT('Ctrl Pts',(0.296197462999944,12.2,-10.402900542));
#154999=CARTESIAN_POINT('Ctrl Pts',(0.296369592999944,12.2,-10.404075906));
#155000=CARTESIAN_POINT('Ctrl Pts',(0.296544161999943,12.2,-10.405259845));
#155001=CARTESIAN_POINT('Ctrl Pts',(0.296721181999944,12.2,-10.406452335));
#155002=CARTESIAN_POINT('Ctrl Pts',(0.296900663999944,12.2,-10.407653347));
#155003=CARTESIAN_POINT('Ctrl Pts',(0.297082623999945,12.2,-10.408862859));
#155004=CARTESIAN_POINT('Ctrl Pts',(0.297267072999944,12.2,-10.410080845));
#155005=CARTESIAN_POINT('Ctrl Pts',(0.297454020999943,12.2,-10.411307279));
#155006=CARTESIAN_POINT('Ctrl Pts',(0.297643483999943,12.2,-10.412542137));
#155007=CARTESIAN_POINT('Ctrl Pts',(0.297835472999944,12.2,-10.413785393));
#155008=CARTESIAN_POINT('Ctrl Pts',(0.298029997999943,12.2,-10.415037024));
#155009=CARTESIAN_POINT('Ctrl Pts',(0.298227073999945,12.2,-10.416297005));
#155010=CARTESIAN_POINT('Ctrl Pts',(0.298426710999945,12.2,-10.41756531));
#155011=CARTESIAN_POINT('Ctrl Pts',(0.298628921999944,12.2,-10.418841915));
#155012=CARTESIAN_POINT('Ctrl Pts',(0.298874678413339,12.2,-10.420383772284));
#155013=CARTESIAN_POINT('Ctrl Pts',(0.299124331804587,12.2,-10.4219380104286));
#155014=CARTESIAN_POINT('Ctrl Pts',(0.299377904195303,12.2,-10.4235045735714));
#155015=CARTESIAN_POINT('Ctrl Pts',(0.299635420609226,12.2,-10.4250834208572));
#155016=CARTESIAN_POINT('Ctrl Pts',(0.299896902999944,12.2,-10.426674502));
#155017=CARTESIAN_POINT('Ctrl Pts',(0.300117460999945,12.2,-10.428008535));
#155018=CARTESIAN_POINT('Ctrl Pts',(0.300340685999944,12.2,-10.429350676));
#155019=CARTESIAN_POINT('Ctrl Pts',(0.300566589999944,12.2,-10.430700902));
#155020=CARTESIAN_POINT('Ctrl Pts',(0.300795183999943,12.2,-10.43205919));
#155021=CARTESIAN_POINT('Ctrl Pts',(0.301026478999944,12.2,-10.433425516));
#155022=CARTESIAN_POINT('Ctrl Pts',(0.301260486999944,12.2,-10.434799858));
#155023=CARTESIAN_POINT('Ctrl Pts',(0.301497219999945,12.2,-10.43618219));
#155024=CARTESIAN_POINT('Ctrl Pts',(0.301736685999944,12.2,-10.437572491));
#155025=CARTESIAN_POINT('Ctrl Pts',(0.301978897999945,12.2,-10.438970738));
#155026=CARTESIAN_POINT('Ctrl Pts',(0.302223867999943,12.2,-10.440376907));
#155027=CARTESIAN_POINT('Ctrl Pts',(0.302471604999944,12.2,-10.441790977));
#155028=CARTESIAN_POINT('Ctrl Pts',(0.302722120999944,12.2,-10.443212923));
#155029=CARTESIAN_POINT('Ctrl Pts',(0.302975424999945,12.2,-10.444642725));
#155030=CARTESIAN_POINT('Ctrl Pts',(0.303231531999945,12.2,-10.446080357));
#155031=CARTESIAN_POINT('Ctrl Pts',(0.303490447999945,12.2,-10.447525799));
#155032=CARTESIAN_POINT('Ctrl Pts',(0.303752185999944,12.2,-10.448979029));
#155033=CARTESIAN_POINT('Ctrl Pts',(0.304016755999944,12.2,-10.450440023));
#155034=CARTESIAN_POINT('Ctrl Pts',(0.304284168999944,12.2,-10.451908761));
#155035=CARTESIAN_POINT('Ctrl Pts',(0.304554434999943,12.2,-10.453385218));
#155036=CARTESIAN_POINT('Ctrl Pts',(0.304827565999943,12.2,-10.454869375));
#155037=CARTESIAN_POINT('Ctrl Pts',(0.305103568999944,12.2,-10.456361208));
#155038=CARTESIAN_POINT('Ctrl Pts',(0.305382456999944,12.2,-10.457860694));
#155039=CARTESIAN_POINT('Ctrl Pts',(0.305664239999944,12.2,-10.459367814));
#155040=CARTESIAN_POINT('Ctrl Pts',(0.305948927999945,12.2,-10.460882546));
#155041=CARTESIAN_POINT('Ctrl Pts',(0.306236529999945,12.2,-10.462404866));
#155042=CARTESIAN_POINT('Ctrl Pts',(0.306527057999944,12.2,-10.463934755));
#155043=CARTESIAN_POINT('Ctrl Pts',(0.306820520999944,12.2,-10.46547219));
#155044=CARTESIAN_POINT('Ctrl Pts',(0.307116928999944,12.2,-10.46701715));
#155045=CARTESIAN_POINT('Ctrl Pts',(0.307416291999945,12.2,-10.468569615));
#155046=CARTESIAN_POINT('Ctrl Pts',(0.307718619999945,12.2,-10.470129561));
#155047=CARTESIAN_POINT('Ctrl Pts',(0.308023921999944,12.2,-10.47169697));
#155048=CARTESIAN_POINT('Ctrl Pts',(0.308332209999945,12.2,-10.473271818));
#155049=CARTESIAN_POINT('Ctrl Pts',(0.308643490999945,12.2,-10.474854086));
#155050=CARTESIAN_POINT('Ctrl Pts',(0.308957776999945,12.2,-10.476443753));
#155051=CARTESIAN_POINT('Ctrl Pts',(0.309275075999944,12.2,-10.478040796));
#155052=CARTESIAN_POINT('Ctrl Pts',(0.309595398999944,12.2,-10.479645198));
#155053=CARTESIAN_POINT('Ctrl Pts',(0.309918754999944,12.2,-10.481256934));
#155054=CARTESIAN_POINT('Ctrl Pts',(0.310245152999944,12.2,-10.482875987));
#155055=CARTESIAN_POINT('Ctrl Pts',(0.310574601999944,12.2,-10.484502335));
#155056=CARTESIAN_POINT('Ctrl Pts',(0.310907112999944,12.2,-10.486135957));
#155057=CARTESIAN_POINT('Ctrl Pts',(0.311242694999944,12.2,-10.487776833));
#155058=CARTESIAN_POINT('Ctrl Pts',(0.311581355999945,12.2,-10.489424943));
#155059=CARTESIAN_POINT('Ctrl Pts',(0.311923106999944,12.2,-10.491080266));
#155060=CARTESIAN_POINT('Ctrl Pts',(0.312267955999944,12.2,-10.492742782));
#155061=CARTESIAN_POINT('Ctrl Pts',(0.312615911999944,12.2,-10.494412473));
#155062=CARTESIAN_POINT('Ctrl Pts',(0.312966985999944,12.2,-10.496089316));
#155063=CARTESIAN_POINT('Ctrl Pts',(0.313321185999945,12.2,-10.497773293));
#155064=CARTESIAN_POINT('Ctrl Pts',(0.313678518999945,12.2,-10.499464382));
#155065=CARTESIAN_POINT('Ctrl Pts',(0.314038995999945,12.2,-10.501162565));
#155066=CARTESIAN_POINT('Ctrl Pts',(0.314402626999944,12.2,-10.502867822));
#155067=CARTESIAN_POINT('Ctrl Pts',(0.314769418999944,12.2,-10.504580133));
#155068=CARTESIAN_POINT('Ctrl Pts',(0.315139380999945,12.2,-10.506299478));
#155069=CARTESIAN_POINT('Ctrl Pts',(0.315512523999945,12.2,-10.508025838));
#155070=CARTESIAN_POINT('Ctrl Pts',(0.315888853999944,12.2,-10.509759194));
#155071=CARTESIAN_POINT('Ctrl Pts',(0.316268379999943,12.2,-10.511499525));
#155072=CARTESIAN_POINT('Ctrl Pts',(0.316651111999944,12.2,-10.513246812));
#155073=CARTESIAN_POINT('Ctrl Pts',(0.317037058999944,12.2,-10.515001037));
#155074=CARTESIAN_POINT('Ctrl Pts',(0.317426227999944,12.2,-10.516762179));
#155075=CARTESIAN_POINT('Ctrl Pts',(0.317818627999945,12.2,-10.518530222));
#155076=CARTESIAN_POINT('Ctrl Pts',(0.318214267999943,12.2,-10.520305143));
#155077=CARTESIAN_POINT('Ctrl Pts',(0.318613155999945,12.2,-10.522086924));
#155078=CARTESIAN_POINT('Ctrl Pts',(0.319015301999944,12.2,-10.523875548));
#155079=CARTESIAN_POINT('Ctrl Pts',(0.319420711999945,12.2,-10.525670994));
#155080=CARTESIAN_POINT('Ctrl Pts',(0.319829394999944,12.2,-10.527473244));
#155081=CARTESIAN_POINT('Ctrl Pts',(0.320241359999944,12.2,-10.529282279));
#155082=CARTESIAN_POINT('Ctrl Pts',(0.320656615999945,12.2,-10.53109808));
#155083=CARTESIAN_POINT('Ctrl Pts',(0.321075168999944,12.2,-10.532920629));
#155084=CARTESIAN_POINT('Ctrl Pts',(0.321497027999945,12.2,-10.534749907));
#155085=CARTESIAN_POINT('Ctrl Pts',(0.321922202999945,12.2,-10.536585896));
#155086=CARTESIAN_POINT('Ctrl Pts',(0.322350699999945,12.2,-10.538428576));
#155087=CARTESIAN_POINT('Ctrl Pts',(0.322782527999944,12.2,-10.54027793));
#155088=CARTESIAN_POINT('Ctrl Pts',(0.323217693999943,12.2,-10.54213394));
#155089=CARTESIAN_POINT('Ctrl Pts',(0.323656205999944,12.2,-10.543996587));
#155090=CARTESIAN_POINT('Ctrl Pts',(0.324098074999943,12.2,-10.545865852));
#155091=CARTESIAN_POINT('Ctrl Pts',(0.324543303999943,12.2,-10.547741717));
#155092=CARTESIAN_POINT('Ctrl Pts',(0.324991904999944,12.2,-10.549624165));
#155093=CARTESIAN_POINT('Ctrl Pts',(0.325443882999944,12.2,-10.551513176));
#155094=CARTESIAN_POINT('Ctrl Pts',(0.325899247999945,12.2,-10.553408734));
#155095=CARTESIAN_POINT('Ctrl Pts',(0.326358006999945,12.2,-10.555310821));
#155096=CARTESIAN_POINT('Ctrl Pts',(0.326820166999945,12.2,-10.557219417));
#155097=CARTESIAN_POINT('Ctrl Pts',(0.327285734999944,12.2,-10.559134506));
#155098=CARTESIAN_POINT('Ctrl Pts',(0.327754721999945,12.2,-10.56105607));
#155099=CARTESIAN_POINT('Ctrl Pts',(0.328227131999944,12.2,-10.562984091));
#155100=CARTESIAN_POINT('Ctrl Pts',(0.328702974999944,12.2,-10.56491855));
#155101=CARTESIAN_POINT('Ctrl Pts',(0.329182255999945,12.2,-10.566859432));
#155102=CARTESIAN_POINT('Ctrl Pts',(0.329664984999944,12.2,-10.568806718));
#155103=CARTESIAN_POINT('Ctrl Pts',(0.330151167999944,12.2,-10.57076039));
#155104=CARTESIAN_POINT('Ctrl Pts',(0.330640813999944,12.2,-10.572720431));
#155105=CARTESIAN_POINT('Ctrl Pts',(0.331133927999945,12.2,-10.574686823));
#155106=CARTESIAN_POINT('Ctrl Pts',(0.331630518999945,12.2,-10.57665955));
#155107=CARTESIAN_POINT('Ctrl Pts',(0.332130593999944,12.2,-10.578638595));
#155108=CARTESIAN_POINT('Ctrl Pts',(0.332634160999945,12.2,-10.580623937));
#155109=CARTESIAN_POINT('Ctrl Pts',(0.333141224999943,12.2,-10.582615564));
#155110=CARTESIAN_POINT('Ctrl Pts',(0.333651795999945,12.2,-10.584613455));
#155111=CARTESIAN_POINT('Ctrl Pts',(0.334165878999944,12.2,-10.586617594));
#155112=CARTESIAN_POINT('Ctrl Pts',(0.334683482999945,12.2,-10.588627965));
#155113=CARTESIAN_POINT('Ctrl Pts',(0.335204611999943,12.2,-10.59064455));
#155114=CARTESIAN_POINT('Ctrl Pts',(0.335729277999944,12.2,-10.592667332));
#155115=CARTESIAN_POINT('Ctrl Pts',(0.336257482999944,12.2,-10.594696293));
#155116=CARTESIAN_POINT('Ctrl Pts',(0.336789236999945,12.2,-10.59673142));
#155117=CARTESIAN_POINT('Ctrl Pts',(0.337324545999945,12.2,-10.598772692));
#155118=CARTESIAN_POINT('Ctrl Pts',(0.337863417999945,12.2,-10.600820093));
#155119=CARTESIAN_POINT('Ctrl Pts',(0.338405857999945,12.2,-10.602873609));
#155120=CARTESIAN_POINT('Ctrl Pts',(0.338951873999944,12.2,-10.60493322));
#155121=CARTESIAN_POINT('Ctrl Pts',(0.339501472999943,12.2,-10.606998913));
#155122=CARTESIAN_POINT('Ctrl Pts',(0.340054661999943,12.2,-10.609070667));
#155123=CARTESIAN_POINT('Ctrl Pts',(0.340611446999944,12.2,-10.611148469));
#155124=CARTESIAN_POINT('Ctrl Pts',(0.341171834999944,12.2,-10.613232302));
#155125=CARTESIAN_POINT('Ctrl Pts',(0.341735832999944,12.2,-10.615322148));
#155126=CARTESIAN_POINT('Ctrl Pts',(0.342303446999944,12.2,-10.617417992));
#155127=CARTESIAN_POINT('Ctrl Pts',(0.342874684999943,12.2,-10.619519817));
#155128=CARTESIAN_POINT('Ctrl Pts',(0.343449551999945,12.2,-10.621627608));
#155129=CARTESIAN_POINT('Ctrl Pts',(0.344028054999944,12.2,-10.623741347));
#155130=CARTESIAN_POINT('Ctrl Pts',(0.344610201999943,12.2,-10.625861018));
#155131=CARTESIAN_POINT('Ctrl Pts',(0.345195997999944,12.2,-10.627986606));
#155132=CARTESIAN_POINT('Ctrl Pts',(0.345785448999945,12.2,-10.630118095));
#155133=CARTESIAN_POINT('Ctrl Pts',(0.346378563999944,12.2,-10.632255468));
#155134=CARTESIAN_POINT('Ctrl Pts',(0.346975346999944,12.2,-10.634398708));
#155135=CARTESIAN_POINT('Ctrl Pts',(0.347575804999943,12.2,-10.636547803));
#155136=CARTESIAN_POINT('Ctrl Pts',(0.348179944999943,12.2,-10.638702732));
#155137=CARTESIAN_POINT('Ctrl Pts',(0.348787772999944,12.2,-10.640863483));
#155138=CARTESIAN_POINT('Ctrl Pts',(0.349399294999945,12.2,-10.643030038));
#155139=CARTESIAN_POINT('Ctrl Pts',(0.350014516999944,12.2,-10.645202383));
#155140=CARTESIAN_POINT('Ctrl Pts',(0.350633445999945,12.2,-10.647380501));
#155141=CARTESIAN_POINT('Ctrl Pts',(0.351256087999945,12.2,-10.649564376));
#155142=CARTESIAN_POINT('Ctrl Pts',(0.351882449999945,12.2,-10.651753993));
#155143=CARTESIAN_POINT('Ctrl Pts',(0.352512535999944,12.2,-10.653949337));
#155144=CARTESIAN_POINT('Ctrl Pts',(0.353146353999945,12.2,-10.656150391));
#155145=CARTESIAN_POINT('Ctrl Pts',(0.353783908999944,12.2,-10.658357141));
#155146=CARTESIAN_POINT('Ctrl Pts',(0.354425208999943,12.2,-10.660569571));
#155147=CARTESIAN_POINT('Ctrl Pts',(0.355070257999944,12.2,-10.662787664));
#155148=CARTESIAN_POINT('Ctrl Pts',(0.355719062999944,12.2,-10.665011407));
#155149=CARTESIAN_POINT('Ctrl Pts',(0.356371629999943,12.2,-10.667240784));
#155150=CARTESIAN_POINT('Ctrl Pts',(0.357027963999944,12.2,-10.669475778));
#155151=CARTESIAN_POINT('Ctrl Pts',(0.357688070999943,12.2,-10.671716375));
#155152=CARTESIAN_POINT('Ctrl Pts',(0.358351957999944,12.2,-10.673962561));
#155153=CARTESIAN_POINT('Ctrl Pts',(0.359019631999944,12.2,-10.676214319));
#155154=CARTESIAN_POINT('Ctrl Pts',(0.359691094999944,12.2,-10.678471635));
#155155=CARTESIAN_POINT('Ctrl Pts',(0.360366356999944,12.2,-10.680734493));
#155156=CARTESIAN_POINT('Ctrl Pts',(0.361045420999944,12.2,-10.683002879));
#155157=CARTESIAN_POINT('Ctrl Pts',(0.361728292999944,12.2,-10.685276775));
#155158=CARTESIAN_POINT('Ctrl Pts',(0.362414979999944,12.2,-10.687556171));
#155159=CARTESIAN_POINT('Ctrl Pts',(0.363105486999944,12.2,-10.689841047));
#155160=CARTESIAN_POINT('Ctrl Pts',(0.363799819999944,12.2,-10.692131392));
#155161=CARTESIAN_POINT('Ctrl Pts',(0.364497983999945,12.2,-10.69442719));
#155162=CARTESIAN_POINT('Ctrl Pts',(0.365199985999943,12.2,-10.696728424));
#155163=CARTESIAN_POINT('Ctrl Pts',(0.365905829999944,12.2,-10.699035082));
#155164=CARTESIAN_POINT('Ctrl Pts',(0.366615521999943,12.2,-10.701347148));
#155165=CARTESIAN_POINT('Ctrl Pts',(0.367329068999943,12.2,-10.703664607));
#155166=CARTESIAN_POINT('Ctrl Pts',(0.368046474999945,12.2,-10.705987445));
#155167=CARTESIAN_POINT('Ctrl Pts',(0.368767745999945,12.2,-10.708315648));
#155168=CARTESIAN_POINT('Ctrl Pts',(0.369492886999945,12.2,-10.710649199));
#155169=CARTESIAN_POINT('Ctrl Pts',(0.370221902999944,12.2,-10.712988086));
#155170=CARTESIAN_POINT('Ctrl Pts',(0.370954801999943,12.2,-10.715332293));
#155171=CARTESIAN_POINT('Ctrl Pts',(0.371691585999944,12.2,-10.717681807));
#155172=CARTESIAN_POINT('Ctrl Pts',(0.372432262999943,12.2,-10.720036612));
#155173=CARTESIAN_POINT('Ctrl Pts',(0.373176837999944,12.2,-10.722396693));
#155174=CARTESIAN_POINT('Ctrl Pts',(0.373925314999944,12.2,-10.724762038));
#155175=CARTESIAN_POINT('Ctrl Pts',(0.374677699999945,12.2,-10.72713263));
#155176=CARTESIAN_POINT('Ctrl Pts',(0.375433997999943,12.2,-10.729508457));
#155177=CARTESIAN_POINT('Ctrl Pts',(0.376194214999943,12.2,-10.731889504));
#155178=CARTESIAN_POINT('Ctrl Pts',(0.376958354999944,12.2,-10.734275757));
#155179=CARTESIAN_POINT('Ctrl Pts',(0.377726424999943,12.2,-10.7366672));
#155180=CARTESIAN_POINT('Ctrl Pts',(0.378498428999944,12.2,-10.73906382));
#155181=CARTESIAN_POINT('Ctrl Pts',(0.379274372999945,12.2,-10.741465604));
#155182=CARTESIAN_POINT('Ctrl Pts',(0.380054259999945,12.2,-10.743872536));
#155183=CARTESIAN_POINT('Ctrl Pts',(0.380838096999945,12.2,-10.746284604));
#155184=CARTESIAN_POINT('Ctrl Pts',(0.381625889999944,12.2,-10.748701792));
#155185=CARTESIAN_POINT('Ctrl Pts',(0.382417640999944,12.2,-10.751124087));
#155186=CARTESIAN_POINT('Ctrl Pts',(0.383213356999944,12.2,-10.753551475));
#155187=CARTESIAN_POINT('Ctrl Pts',(0.384013043999945,12.2,-10.755983942));
#155188=CARTESIAN_POINT('Ctrl Pts',(0.384816703999944,12.2,-10.758421474));
#155189=CARTESIAN_POINT('Ctrl Pts',(0.385624345999943,12.2,-10.760864057));
#155190=CARTESIAN_POINT('Ctrl Pts',(0.386435970999944,12.2,-10.763311678));
#155191=CARTESIAN_POINT('Ctrl Pts',(0.387251585999945,12.2,-10.765764322));
#155192=CARTESIAN_POINT('Ctrl Pts',(0.388071194999944,12.2,-10.768221976));
#155193=CARTESIAN_POINT('Ctrl Pts',(0.388894804999945,12.2,-10.770684626));
#155194=CARTESIAN_POINT('Ctrl Pts',(0.389722417999945,12.2,-10.773152259));
#155195=CARTESIAN_POINT('Ctrl Pts',(0.390554040999945,12.2,-10.77562486));
#155196=CARTESIAN_POINT('Ctrl Pts',(0.391389675999945,12.2,-10.778102417));
#155197=CARTESIAN_POINT('Ctrl Pts',(0.392229331999945,12.2,-10.780584915));
#155198=CARTESIAN_POINT('Ctrl Pts',(0.393073008999943,12.2,-10.78307234));
#155199=CARTESIAN_POINT('Ctrl Pts',(0.393920715999944,12.2,-10.785564681));
#155200=CARTESIAN_POINT('Ctrl Pts',(0.394772454999943,12.2,-10.788061922));
#155201=CARTESIAN_POINT('Ctrl Pts',(0.395628231999944,12.2,-10.790564051));
#155202=CARTESIAN_POINT('Ctrl Pts',(0.396488050999944,12.2,-10.793071054));
#155203=CARTESIAN_POINT('Ctrl Pts',(0.397351916999943,12.2,-10.795582918));
#155204=CARTESIAN_POINT('Ctrl Pts',(0.398219834999944,12.2,-10.798099629));
#155205=CARTESIAN_POINT('Ctrl Pts',(0.399091808999945,12.2,-10.800621174));
#155206=CARTESIAN_POINT('Ctrl Pts',(0.399967842999944,12.2,-10.80314754));
#155207=CARTESIAN_POINT('Ctrl Pts',(0.400847942999943,12.2,-10.805678712));
#155208=CARTESIAN_POINT('Ctrl Pts',(0.401732111999945,12.2,-10.808214679));
#155209=CARTESIAN_POINT('Ctrl Pts',(0.402620355999943,12.2,-10.810755427));
#155210=CARTESIAN_POINT('Ctrl Pts',(0.403512678999943,12.2,-10.813300943));
#155211=CARTESIAN_POINT('Ctrl Pts',(0.404409085999945,12.2,-10.815851213));
#155212=CARTESIAN_POINT('Ctrl Pts',(0.405309579999944,12.2,-10.818406225));
#155213=CARTESIAN_POINT('Ctrl Pts',(0.406214165999945,12.2,-10.820965964));
#155214=CARTESIAN_POINT('Ctrl Pts',(0.407122848999943,12.2,-10.82353042));
#155215=CARTESIAN_POINT('Ctrl Pts',(0.408035631999945,12.2,-10.826099577));
#155216=CARTESIAN_POINT('Ctrl Pts',(0.408952521999945,12.2,-10.828673424));
#155217=CARTESIAN_POINT('Ctrl Pts',(0.409873521999945,12.2,-10.831251946));
#155218=CARTESIAN_POINT('Ctrl Pts',(0.410798634999944,12.2,-10.833835132));
#155219=CARTESIAN_POINT('Ctrl Pts',(0.411727865999945,12.2,-10.836422969));
#155220=CARTESIAN_POINT('Ctrl Pts',(0.412661221999944,12.2,-10.839015443));
#155221=CARTESIAN_POINT('Ctrl Pts',(0.413598702999943,12.2,-10.841612542));
#155222=CARTESIAN_POINT('Ctrl Pts',(0.414540315999944,12.2,-10.844214253));
#155223=CARTESIAN_POINT('Ctrl Pts',(0.415486064999945,12.2,-10.846820562));
#155224=CARTESIAN_POINT('Ctrl Pts',(0.416435952999944,12.2,-10.849431457));
#155225=CARTESIAN_POINT('Ctrl Pts',(0.417389984999945,12.2,-10.852046927));
#155226=CARTESIAN_POINT('Ctrl Pts',(0.418348164999944,12.2,-10.854666958));
#155227=CARTESIAN_POINT('Ctrl Pts',(0.419310496999945,12.2,-10.857291535));
#155228=CARTESIAN_POINT('Ctrl Pts',(0.420276985999944,12.2,-10.859920649));
#155229=CARTESIAN_POINT('Ctrl Pts',(0.421247635999944,12.2,-10.862554285));
#155230=CARTESIAN_POINT('Ctrl Pts',(0.422222449999945,12.2,-10.865192432));
#155231=CARTESIAN_POINT('Ctrl Pts',(0.423201432999945,12.2,-10.867835076));
#155232=CARTESIAN_POINT('Ctrl Pts',(0.424184586999944,12.2,-10.870482205));
#155233=CARTESIAN_POINT('Ctrl Pts',(0.425171919999944,12.2,-10.873133806));
#155234=CARTESIAN_POINT('Ctrl Pts',(0.426163432999944,12.2,-10.875789868));
#155235=CARTESIAN_POINT('Ctrl Pts',(0.427159130999945,12.2,-10.878450378));
#155236=CARTESIAN_POINT('Ctrl Pts',(0.428159016999944,12.2,-10.881115322));
#155237=CARTESIAN_POINT('Ctrl Pts',(0.429163096999944,12.2,-10.883784689));
#155238=CARTESIAN_POINT('Ctrl Pts',(0.430171372999943,12.2,-10.886458467));
#155239=CARTESIAN_POINT('Ctrl Pts',(0.431183849999943,12.2,-10.889136642));
#155240=CARTESIAN_POINT('Ctrl Pts',(0.432200529999944,12.2,-10.891819203));
#155241=CARTESIAN_POINT('Ctrl Pts',(0.433221419999944,12.2,-10.894506138));
#155242=CARTESIAN_POINT('Ctrl Pts',(0.434246522999944,12.2,-10.897197434));
#155243=CARTESIAN_POINT('Ctrl Pts',(0.435275840999945,12.2,-10.899893077));
#155244=CARTESIAN_POINT('Ctrl Pts',(0.436309378999944,12.2,-10.902593058));
#155245=CARTESIAN_POINT('Ctrl Pts',(0.437347139999943,12.2,-10.905297364));
#155246=CARTESIAN_POINT('Ctrl Pts',(0.438389128999944,12.2,-10.908005981));
#155247=CARTESIAN_POINT('Ctrl Pts',(0.439435350999944,12.2,-10.910718898));
#155248=CARTESIAN_POINT('Ctrl Pts',(0.440485805999945,12.2,-10.913436104));
#155249=CARTESIAN_POINT('Ctrl Pts',(0.441540500999944,12.2,-10.916157585));
#155250=CARTESIAN_POINT('Ctrl Pts',(0.442599438999943,12.2,-10.91888333));
#155251=CARTESIAN_POINT('Ctrl Pts',(0.443662621999945,12.2,-10.921613326));
#155252=CARTESIAN_POINT('Ctrl Pts',(0.444730055999945,12.2,-10.924347562));
#155253=CARTESIAN_POINT('Ctrl Pts',(0.445801742999944,12.2,-10.927086026));
#155254=CARTESIAN_POINT('Ctrl Pts',(0.446877687999944,12.2,-10.929828706));
#155255=CARTESIAN_POINT('Ctrl Pts',(0.447957893999943,12.2,-10.932575589));
#155256=CARTESIAN_POINT('Ctrl Pts',(0.449042363999944,12.2,-10.935326664));
#155257=CARTESIAN_POINT('Ctrl Pts',(0.450131101999943,12.2,-10.93808192));
#155258=CARTESIAN_POINT('Ctrl Pts',(0.451224112999944,12.2,-10.940841343));
#155259=CARTESIAN_POINT('Ctrl Pts',(0.452321397999944,12.2,-10.943604921));
#155260=CARTESIAN_POINT('Ctrl Pts',(0.453422961999944,12.2,-10.946372645));
#155261=CARTESIAN_POINT('Ctrl Pts',(0.454528808999944,12.2,-10.949144502));
#155262=CARTESIAN_POINT('Ctrl Pts',(0.455638941999944,12.2,-10.951920478));
#155263=CARTESIAN_POINT('Ctrl Pts',(0.456753363999944,12.2,-10.954700564));
#155264=CARTESIAN_POINT('Ctrl Pts',(0.457872078999945,12.2,-10.957484747));
#155265=CARTESIAN_POINT('Ctrl Pts',(0.458995090999944,12.2,-10.960273016));
#155266=CARTESIAN_POINT('Ctrl Pts',(0.460122400999945,12.2,-10.963065359));
#155267=CARTESIAN_POINT('Ctrl Pts',(0.461254015999945,12.2,-10.965861764));
#155268=CARTESIAN_POINT('Ctrl Pts',(0.462389937999944,12.2,-10.96866222));
#155269=CARTESIAN_POINT('Ctrl Pts',(0.463530168999944,12.2,-10.971466714));
#155270=CARTESIAN_POINT('Ctrl Pts',(0.464674712999944,12.2,-10.974275237));
#155271=CARTESIAN_POINT('Ctrl Pts',(0.465823575999943,12.2,-10.977087774));
#155272=CARTESIAN_POINT('Ctrl Pts',(0.466976756999945,12.2,-10.979904316));
#155273=CARTESIAN_POINT('Ctrl Pts',(0.468134261999945,12.2,-10.982724852));
#155274=CARTESIAN_POINT('Ctrl Pts',(0.469296094999944,12.2,-10.985549368));
#155275=CARTESIAN_POINT('Ctrl Pts',(0.470462256999945,12.2,-10.988377854));
#155276=CARTESIAN_POINT('Ctrl Pts',(0.471632752999945,12.2,-10.991210298));
#155277=CARTESIAN_POINT('Ctrl Pts',(0.472807584999944,12.2,-10.994046689));
#155278=CARTESIAN_POINT('Ctrl Pts',(0.473986757999943,12.2,-10.996887016));
#155279=CARTESIAN_POINT('Ctrl Pts',(0.475170271999945,12.2,-10.999731268));
#155280=CARTESIAN_POINT('Ctrl Pts',(0.476358134999944,12.2,-11.002579431));
#155281=CARTESIAN_POINT('Ctrl Pts',(0.477550345999944,12.2,-11.005431497));
#155282=CARTESIAN_POINT('Ctrl Pts',(0.478746909999943,12.2,-11.008287453));
#155283=CARTESIAN_POINT('Ctrl Pts',(0.479947829999944,12.2,-11.011147287));
#155284=CARTESIAN_POINT('Ctrl Pts',(0.481153109999944,12.2,-11.014010988));
#155285=CARTESIAN_POINT('Ctrl Pts',(0.482362750999944,12.2,-11.016878547));
#155286=CARTESIAN_POINT('Ctrl Pts',(0.483576757999945,12.2,-11.01974995));
#155287=CARTESIAN_POINT('Ctrl Pts',(0.484795132999943,12.2,-11.022625188));
#155288=CARTESIAN_POINT('Ctrl Pts',(0.486017879999944,12.2,-11.025504247));
#155289=CARTESIAN_POINT('Ctrl Pts',(0.487245001999945,12.2,-11.028387119));
#155290=CARTESIAN_POINT('Ctrl Pts',(0.488476501999945,12.2,-11.031273791));
#155291=CARTESIAN_POINT('Ctrl Pts',(0.489712381999944,12.2,-11.034164252));
#155292=CARTESIAN_POINT('Ctrl Pts',(0.490952645999944,12.2,-11.037058491));
#155293=CARTESIAN_POINT('Ctrl Pts',(0.492197297999944,12.2,-11.039956497));
#155294=CARTESIAN_POINT('Ctrl Pts',(0.493446337999943,12.2,-11.04285826));
#155295=CARTESIAN_POINT('Ctrl Pts',(0.494699771999944,12.2,-11.045763768));
#155296=CARTESIAN_POINT('Ctrl Pts',(0.495957600999944,12.2,-11.04867301));
#155297=CARTESIAN_POINT('Ctrl Pts',(0.497219829999944,12.2,-11.051585974));
#155298=CARTESIAN_POINT('Ctrl Pts',(0.498486459999944,12.2,-11.05450265));
#155299=CARTESIAN_POINT('Ctrl Pts',(0.499757494999944,12.2,-11.057423028));
#155300=CARTESIAN_POINT('Ctrl Pts',(0.501032935999944,12.2,-11.060347096));
#155301=CARTESIAN_POINT('Ctrl Pts',(0.502312788999945,12.2,-11.063274844));
#155302=CARTESIAN_POINT('Ctrl Pts',(0.503597054999945,12.2,-11.066206259));
#155303=CARTESIAN_POINT('Ctrl Pts',(0.504885736999944,12.2,-11.069141332));
#155304=CARTESIAN_POINT('Ctrl Pts',(0.506178838999943,12.2,-11.072080052));
#155305=CARTESIAN_POINT('Ctrl Pts',(0.507476362999945,12.2,-11.075022407));
#155306=CARTESIAN_POINT('Ctrl Pts',(0.508778309999944,12.2,-11.077968387));
#155307=CARTESIAN_POINT('Ctrl Pts',(0.510084685999944,12.2,-11.080917982));
#155308=CARTESIAN_POINT('Ctrl Pts',(0.511395492999944,12.2,-11.08387118));
#155309=CARTESIAN_POINT('Ctrl Pts',(0.512710730999945,12.2,-11.086827972));
#155310=CARTESIAN_POINT('Ctrl Pts',(0.514030406999945,12.2,-11.089788344));
#155311=CARTESIAN_POINT('Ctrl Pts',(0.515354519999944,12.2,-11.092752289));
#155312=CARTESIAN_POINT('Ctrl Pts',(0.516683075999944,12.2,-11.095719793));
#155313=CARTESIAN_POINT('Ctrl Pts',(0.518016074999944,12.2,-11.098690848));
#155314=CARTESIAN_POINT('Ctrl Pts',(0.519353520999944,12.2,-11.101665441));
#155315=CARTESIAN_POINT('Ctrl Pts',(0.520695416999944,12.2,-11.104643564));
#155316=CARTESIAN_POINT('Ctrl Pts',(0.522041764999944,12.2,-11.107625205));
#155317=CARTESIAN_POINT('Ctrl Pts',(0.523392567999944,12.2,-11.110610353));
#155318=CARTESIAN_POINT('Ctrl Pts',(0.524747828999944,12.2,-11.113598997));
#155319=CARTESIAN_POINT('Ctrl Pts',(0.526107550999945,12.2,-11.116591128));
#155320=CARTESIAN_POINT('Ctrl Pts',(0.527471734999944,12.2,-11.119586735));
#155321=CARTESIAN_POINT('Ctrl Pts',(0.528840383999943,12.2,-11.122585808));
#155322=CARTESIAN_POINT('Ctrl Pts',(0.530213500999944,12.2,-11.125588334));
#155323=CARTESIAN_POINT('Ctrl Pts',(0.531591089999944,12.2,-11.128594306));
#155324=CARTESIAN_POINT('Ctrl Pts',(0.532973150999945,12.2,-11.131603711));
#155325=CARTESIAN_POINT('Ctrl Pts',(0.534359687999945,12.2,-11.13461654));
#155326=CARTESIAN_POINT('Ctrl Pts',(0.535750703999944,12.2,-11.137632781));
#155327=CARTESIAN_POINT('Ctrl Pts',(0.537146200999944,12.2,-11.140652425));
#155328=CARTESIAN_POINT('Ctrl Pts',(0.538546180999945,12.2,-11.143675461));
#155329=CARTESIAN_POINT('Ctrl Pts',(0.539950646999944,12.2,-11.146701879));
#155330=CARTESIAN_POINT('Ctrl Pts',(0.541359600999944,12.2,-11.149731669));
#155331=CARTESIAN_POINT('Ctrl Pts',(0.542773046999944,12.2,-11.152764819));
#155332=CARTESIAN_POINT('Ctrl Pts',(0.544190985999945,12.2,-11.155801321));
#155333=CARTESIAN_POINT('Ctrl Pts',(0.545613420999944,12.2,-11.158841164));
#155334=CARTESIAN_POINT('Ctrl Pts',(0.547040353999945,12.2,-11.161884336));
#155335=CARTESIAN_POINT('Ctrl Pts',(0.548471787999943,12.2,-11.164930828));
#155336=CARTESIAN_POINT('Ctrl Pts',(0.549907724999944,12.2,-11.167980631));
#155337=CARTESIAN_POINT('Ctrl Pts',(0.551348166999944,12.2,-11.171033733));
#155338=CARTESIAN_POINT('Ctrl Pts',(0.552793118999944,12.2,-11.174090123));
#155339=CARTESIAN_POINT('Ctrl Pts',(0.554242579999944,12.2,-11.177149794));
#155340=CARTESIAN_POINT('Ctrl Pts',(0.555696552999944,12.2,-11.180212734));
#155341=CARTESIAN_POINT('Ctrl Pts',(0.557155042999944,12.2,-11.183278932));
#155342=CARTESIAN_POINT('Ctrl Pts',(0.558618047999944,12.2,-11.186348379));
#155343=CARTESIAN_POINT('Ctrl Pts',(0.560085574999943,12.2,-11.189421065));
#155344=CARTESIAN_POINT('Ctrl Pts',(0.561557623999944,12.2,-11.192496979));
#155345=CARTESIAN_POINT('Ctrl Pts',(0.563034195999944,12.2,-11.195576112));
#155346=CARTESIAN_POINT('Ctrl Pts',(0.564515294999944,12.2,-11.198658453));
#155347=CARTESIAN_POINT('Ctrl Pts',(0.566000922999944,12.2,-11.201743993));
#155348=CARTESIAN_POINT('Ctrl Pts',(0.567491082999945,12.2,-11.204832721));
#155349=CARTESIAN_POINT('Ctrl Pts',(0.568985775999944,12.2,-11.207924627));
#155350=CARTESIAN_POINT('Ctrl Pts',(0.570485004999944,12.2,-11.211019702));
#155351=CARTESIAN_POINT('Ctrl Pts',(0.571988771999944,12.2,-11.214117935));
#155352=CARTESIAN_POINT('Ctrl Pts',(0.573497078999944,12.2,-11.217219316));
#155353=CARTESIAN_POINT('Ctrl Pts',(0.575009928999944,12.2,-11.220323837));
#155354=CARTESIAN_POINT('Ctrl Pts',(0.576527321999943,12.2,-11.223431485));
#155355=CARTESIAN_POINT('Ctrl Pts',(0.578049262999943,12.2,-11.226542253));
#155356=CARTESIAN_POINT('Ctrl Pts',(0.579575752999945,12.2,-11.229656128));
#155357=CARTESIAN_POINT('Ctrl Pts',(0.581106792999945,12.2,-11.232773103));
#155358=CARTESIAN_POINT('Ctrl Pts',(0.582642387999944,12.2,-11.235893168));
#155359=CARTESIAN_POINT('Ctrl Pts',(0.584182536999944,12.2,-11.23901631));
#155360=CARTESIAN_POINT('Ctrl Pts',(0.585727243999944,12.2,-11.242142523));
#155361=CARTESIAN_POINT('Ctrl Pts',(0.587276510999944,12.2,-11.245271795));
#155362=CARTESIAN_POINT('Ctrl Pts',(0.588830339999945,12.2,-11.248404117));
#155363=CARTESIAN_POINT('Ctrl Pts',(0.590388730999944,12.2,-11.251539479));
#155364=CARTESIAN_POINT('Ctrl Pts',(0.591951689999944,12.2,-11.254677871));
#155365=CARTESIAN_POINT('Ctrl Pts',(0.593519214999944,12.2,-11.257819284));
#155366=CARTESIAN_POINT('Ctrl Pts',(0.595091311999945,12.2,-11.260963707));
#155367=CARTESIAN_POINT('Ctrl Pts',(0.596667979999944,12.2,-11.264111132));
#155368=CARTESIAN_POINT('Ctrl Pts',(0.598249221999944,12.2,-11.267261548));
#155369=CARTESIAN_POINT('Ctrl Pts',(0.599835039999944,12.2,-11.270414946));
#155370=CARTESIAN_POINT('Ctrl Pts',(0.601425436999944,12.2,-11.273571316));
#155371=CARTESIAN_POINT('Ctrl Pts',(0.603020412999945,12.2,-11.276730648));
#155372=CARTESIAN_POINT('Ctrl Pts',(0.604619971999945,12.2,-11.279892934));
#155373=CARTESIAN_POINT('Ctrl Pts',(0.606224114999944,12.2,-11.283058161));
#155374=CARTESIAN_POINT('Ctrl Pts',(0.607832842999944,12.2,-11.286226323));
#155375=CARTESIAN_POINT('Ctrl Pts',(0.609446159999945,12.2,-11.289397409));
#155376=CARTESIAN_POINT('Ctrl Pts',(0.611064066999945,12.2,-11.29257141));
#155377=CARTESIAN_POINT('Ctrl Pts',(0.612686564999944,12.2,-11.295748315));
#155378=CARTESIAN_POINT('Ctrl Pts',(0.614313656999944,12.2,-11.298928116));
#155379=CARTESIAN_POINT('Ctrl Pts',(0.615945344999944,12.2,-11.302110802));
#155380=CARTESIAN_POINT('Ctrl Pts',(0.617581629999945,12.2,-11.305296365));
#155381=CARTESIAN_POINT('Ctrl Pts',(0.619222514999944,12.2,-11.308484795));
#155382=CARTESIAN_POINT('Ctrl Pts',(0.620868000999945,12.2,-11.311676082));
#155383=CARTESIAN_POINT('Ctrl Pts',(0.622518089999944,12.2,-11.314870217));
#155384=CARTESIAN_POINT('Ctrl Pts',(0.624172783999944,12.2,-11.31806719));
#155385=CARTESIAN_POINT('Ctrl Pts',(0.625832085999944,12.2,-11.321266994));
#155386=CARTESIAN_POINT('Ctrl Pts',(0.627495994999945,12.2,-11.324469616));
#155387=CARTESIAN_POINT('Ctrl Pts',(0.629164515999945,12.2,-11.327675049));
#155388=CARTESIAN_POINT('Ctrl Pts',(0.630837647999944,12.2,-11.330883282));
#155389=CARTESIAN_POINT('Ctrl Pts',(0.632515393999945,12.2,-11.334094307));
#155390=CARTESIAN_POINT('Ctrl Pts',(0.634197756999945,12.2,-11.337308115));
#155391=CARTESIAN_POINT('Ctrl Pts',(0.635884736999944,12.2,-11.340524695));
#155392=CARTESIAN_POINT('Ctrl Pts',(0.637576336999944,12.2,-11.343744038));
#155393=CARTESIAN_POINT('Ctrl Pts',(0.639272556999945,12.2,-11.346966135));
#155394=CARTESIAN_POINT('Ctrl Pts',(0.640973400999945,12.2,-11.350190979));
#155395=CARTESIAN_POINT('Ctrl Pts',(0.642678868999944,12.2,-11.353418557));
#155396=CARTESIAN_POINT('Ctrl Pts',(0.644388963999944,12.2,-11.356648862));
#155397=CARTESIAN_POINT('Ctrl Pts',(0.646103685999945,12.2,-11.359881884));
#155398=CARTESIAN_POINT('Ctrl Pts',(0.647823038999944,12.2,-11.363117614));
#155399=CARTESIAN_POINT('Ctrl Pts',(0.649547021999944,12.2,-11.366356043));
#155400=CARTESIAN_POINT('Ctrl Pts',(0.651275639999944,12.2,-11.369597161));
#155401=CARTESIAN_POINT('Ctrl Pts',(0.653008890999944,12.2,-11.37284096));
#155402=CARTESIAN_POINT('Ctrl Pts',(0.654746778999944,12.2,-11.37608743));
#155403=CARTESIAN_POINT('Ctrl Pts',(0.656489305999944,12.2,-11.379336561));
#155404=CARTESIAN_POINT('Ctrl Pts',(0.658236471999943,12.2,-11.382588345));
#155405=CARTESIAN_POINT('Ctrl Pts',(0.659988278999944,12.2,-11.385842772));
#155406=CARTESIAN_POINT('Ctrl Pts',(0.661744729999943,12.2,-11.389099835));
#155407=CARTESIAN_POINT('Ctrl Pts',(0.663505824999944,12.2,-11.392359523));
#155408=CARTESIAN_POINT('Ctrl Pts',(0.665271565999944,12.2,-11.395621827));
#155409=CARTESIAN_POINT('Ctrl Pts',(0.667041954999944,12.2,-11.39888674));
#155410=CARTESIAN_POINT('Ctrl Pts',(0.668816992999944,12.2,-11.402154251));
#155411=CARTESIAN_POINT('Ctrl Pts',(0.670596681999944,12.2,-11.405424352));
#155412=CARTESIAN_POINT('Ctrl Pts',(0.672381022999944,12.2,-11.408697032));
#155413=CARTESIAN_POINT('Ctrl Pts',(0.674170018999944,12.2,-11.411972283));
#155414=CARTESIAN_POINT('Ctrl Pts',(0.675963669999944,12.2,-11.415250096));
#155415=CARTESIAN_POINT('Ctrl Pts',(0.677761977999943,12.2,-11.418530461));
#155416=CARTESIAN_POINT('Ctrl Pts',(0.679564944999944,12.2,-11.421813369));
#155417=CARTESIAN_POINT('Ctrl Pts',(0.681372572999944,12.2,-11.425098811));
#155418=CARTESIAN_POINT('Ctrl Pts',(0.683184861999945,12.2,-11.42838678));
#155419=CARTESIAN_POINT('Ctrl Pts',(0.685001812999944,12.2,-11.431677269));
#155420=CARTESIAN_POINT('Ctrl Pts',(0.686823428999944,12.2,-11.434970268));
#155421=CARTESIAN_POINT('Ctrl Pts',(0.688649710999945,12.2,-11.438265769));
#155422=CARTESIAN_POINT('Ctrl Pts',(0.690480658999945,12.2,-11.441563763));
#155423=CARTESIAN_POINT('Ctrl Pts',(0.692316276999944,12.2,-11.444864239));
#155424=CARTESIAN_POINT('Ctrl Pts',(0.694156563999945,12.2,-11.448167187));
#155425=CARTESIAN_POINT('Ctrl Pts',(0.696001524999944,12.2,-11.451472595));
#155426=CARTESIAN_POINT('Ctrl Pts',(0.697851158999944,12.2,-11.454780453));
#155427=CARTESIAN_POINT('Ctrl Pts',(0.699705468999944,12.2,-11.458090751));
#155428=CARTESIAN_POINT('Ctrl Pts',(0.701564455999945,12.2,-11.461403481));
#155429=CARTESIAN_POINT('Ctrl Pts',(0.703428120999944,12.2,-11.464718637));
#155430=CARTESIAN_POINT('Ctrl Pts',(0.705296462999944,12.2,-11.468036216));
#155431=CARTESIAN_POINT('Ctrl Pts',(0.707169485999944,12.2,-11.471356215));
#155432=CARTESIAN_POINT('Ctrl Pts',(0.708671644999944,12.2,-11.474014149));
#155433=CARTESIAN_POINT('Ctrl Pts',(0.709800370999945,12.2,-11.476008688));
#155434=CARTESIAN_POINT('Ctrl Pts',(0.710553790999944,12.2,-11.477338863));
#155435=CARTESIAN_POINT('Ctrl Pts',(0.710930733999944,12.2,-11.478004072));
#155436=CARTESIAN_POINT('Ctrl Pts',(1.09337742899994,15.2,-11.447904865));
#155437=CARTESIAN_POINT('Ctrl Pts',(1.09337742899994,11.6,-11.447904865));
#155438=CARTESIAN_POINT('Ctrl Pts',(1.09364566999994,15.2,-11.447188878));
#155439=CARTESIAN_POINT('Ctrl Pts',(1.09364566999994,11.6,-11.447188878));
#155440=CARTESIAN_POINT('Ctrl Pts',(1.09418172899994,15.2,-11.445757219));
#155441=CARTESIAN_POINT('Ctrl Pts',(1.09418172899994,11.6,-11.445757219));
#155442=CARTESIAN_POINT('Ctrl Pts',(1.09498454299994,15.2,-11.443610664));
#155443=CARTESIAN_POINT('Ctrl Pts',(1.09498454299994,11.6,-11.443610664));
#155444=CARTESIAN_POINT('Ctrl Pts',(1.09605241599994,15.2,-11.440750465));
#155445=CARTESIAN_POINT('Ctrl Pts',(1.09605241599994,11.6,-11.440750465));
#155446=CARTESIAN_POINT('Ctrl Pts',(1.09738301599994,15.2,-11.437178335));
#155447=CARTESIAN_POINT('Ctrl Pts',(1.09738301599994,11.6,-11.437178335));
#155448=CARTESIAN_POINT('Ctrl Pts',(1.09870937299994,15.2,-11.433609328));
#155449=CARTESIAN_POINT('Ctrl Pts',(1.09870937299994,11.6,-11.433609328));
#155450=CARTESIAN_POINT('Ctrl Pts',(1.10003148899994,15.2,-11.430043446));
#155451=CARTESIAN_POINT('Ctrl Pts',(1.10003148899994,11.6,-11.430043446));
#155452=CARTESIAN_POINT('Ctrl Pts',(1.10134936299994,15.2,-11.426480691));
#155453=CARTESIAN_POINT('Ctrl Pts',(1.10134936299994,11.6,-11.426480691));
#155454=CARTESIAN_POINT('Ctrl Pts',(1.10266299899994,15.2,-11.422921069));
#155455=CARTESIAN_POINT('Ctrl Pts',(1.10266299899994,11.6,-11.422921069));
#155456=CARTESIAN_POINT('Ctrl Pts',(1.10397239799994,15.2,-11.419364591));
#155457=CARTESIAN_POINT('Ctrl Pts',(1.10397239799994,11.6,-11.419364591));
#155458=CARTESIAN_POINT('Ctrl Pts',(1.10527756399994,15.2,-11.415811262));
#155459=CARTESIAN_POINT('Ctrl Pts',(1.10527756399994,11.6,-11.415811262));
#155460=CARTESIAN_POINT('Ctrl Pts',(1.10657849999994,15.2,-11.412261095));
#155461=CARTESIAN_POINT('Ctrl Pts',(1.10657849999994,11.6,-11.412261095));
#155462=CARTESIAN_POINT('Ctrl Pts',(1.10787520999994,15.2,-11.408714099));
#155463=CARTESIAN_POINT('Ctrl Pts',(1.10787520999994,11.6,-11.408714099));
#155464=CARTESIAN_POINT('Ctrl Pts',(1.10916769599994,15.2,-11.405170286));
#155465=CARTESIAN_POINT('Ctrl Pts',(1.10916769599994,11.6,-11.405170286));
#155466=CARTESIAN_POINT('Ctrl Pts',(1.11045596299994,15.2,-11.401629665));
#155467=CARTESIAN_POINT('Ctrl Pts',(1.11045596299994,11.6,-11.401629665));
#155468=CARTESIAN_POINT('Ctrl Pts',(1.11174001299994,15.2,-11.398092244));
#155469=CARTESIAN_POINT('Ctrl Pts',(1.11174001299994,11.6,-11.398092244));
#155470=CARTESIAN_POINT('Ctrl Pts',(1.11301984899994,15.2,-11.394558034));
#155471=CARTESIAN_POINT('Ctrl Pts',(1.11301984899994,11.6,-11.394558034));
#155472=CARTESIAN_POINT('Ctrl Pts',(1.11429547399994,15.2,-11.39102704));
#155473=CARTESIAN_POINT('Ctrl Pts',(1.11429547399994,11.6,-11.39102704));
#155474=CARTESIAN_POINT('Ctrl Pts',(1.11556688999994,15.2,-11.387499272));
#155475=CARTESIAN_POINT('Ctrl Pts',(1.11556688999994,11.6,-11.387499272));
#155476=CARTESIAN_POINT('Ctrl Pts',(1.11683409999994,15.2,-11.383974735));
#155477=CARTESIAN_POINT('Ctrl Pts',(1.11683409999994,11.6,-11.383974735));
#155478=CARTESIAN_POINT('Ctrl Pts',(1.11809710599994,15.2,-11.38045344));
#155479=CARTESIAN_POINT('Ctrl Pts',(1.11809710599994,11.6,-11.38045344));
#155480=CARTESIAN_POINT('Ctrl Pts',(1.11935591099994,15.2,-11.376935393));
#155481=CARTESIAN_POINT('Ctrl Pts',(1.11935591099994,11.6,-11.376935393));
#155482=CARTESIAN_POINT('Ctrl Pts',(1.12061051899994,15.2,-11.373420606));
#155483=CARTESIAN_POINT('Ctrl Pts',(1.12061051899994,11.6,-11.373420606));
#155484=CARTESIAN_POINT('Ctrl Pts',(1.12186093199994,15.2,-11.369909084));
#155485=CARTESIAN_POINT('Ctrl Pts',(1.12186093199994,11.6,-11.369909084));
#155486=CARTESIAN_POINT('Ctrl Pts',(1.12310715399994,15.2,-11.366400839));
#155487=CARTESIAN_POINT('Ctrl Pts',(1.12310715399994,11.6,-11.366400839));
#155488=CARTESIAN_POINT('Ctrl Pts',(1.12434918699994,15.2,-11.36289588));
#155489=CARTESIAN_POINT('Ctrl Pts',(1.12434918699994,11.6,-11.36289588));
#155490=CARTESIAN_POINT('Ctrl Pts',(1.12558703399994,15.2,-11.359394214));
#155491=CARTESIAN_POINT('Ctrl Pts',(1.12558703399994,11.6,-11.359394214));
#155492=CARTESIAN_POINT('Ctrl Pts',(1.12682069999994,15.2,-11.355895851));
#155493=CARTESIAN_POINT('Ctrl Pts',(1.12682069999994,11.6,-11.355895851));
#155494=CARTESIAN_POINT('Ctrl Pts',(1.12805018499994,15.2,-11.3524008));
#155495=CARTESIAN_POINT('Ctrl Pts',(1.12805018499994,11.6,-11.3524008));
#155496=CARTESIAN_POINT('Ctrl Pts',(1.12927549399994,15.2,-11.348909068));
#155497=CARTESIAN_POINT('Ctrl Pts',(1.12927549399994,11.6,-11.348909068));
#155498=CARTESIAN_POINT('Ctrl Pts',(1.13049662999994,15.2,-11.345420665));
#155499=CARTESIAN_POINT('Ctrl Pts',(1.13049662999994,11.6,-11.345420665));
#155500=CARTESIAN_POINT('Ctrl Pts',(1.13171359399994,15.2,-11.341935598));
#155501=CARTESIAN_POINT('Ctrl Pts',(1.13171359399994,11.6,-11.341935598));
#155502=CARTESIAN_POINT('Ctrl Pts',(1.13292639099994,15.2,-11.338453878));
#155503=CARTESIAN_POINT('Ctrl Pts',(1.13292639099994,11.6,-11.338453878));
#155504=CARTESIAN_POINT('Ctrl Pts',(1.13413502299994,15.2,-11.334975512));
#155505=CARTESIAN_POINT('Ctrl Pts',(1.13413502299994,11.6,-11.334975512));
#155506=CARTESIAN_POINT('Ctrl Pts',(1.13533949399994,15.2,-11.331500509));
#155507=CARTESIAN_POINT('Ctrl Pts',(1.13533949399994,11.6,-11.331500509));
#155508=CARTESIAN_POINT('Ctrl Pts',(1.13653980599994,15.2,-11.32802888));
#155509=CARTESIAN_POINT('Ctrl Pts',(1.13653980599994,11.6,-11.32802888));
#155510=CARTESIAN_POINT('Ctrl Pts',(1.13773596199994,15.2,-11.324560631));
#155511=CARTESIAN_POINT('Ctrl Pts',(1.13773596199994,11.6,-11.324560631));
#155512=CARTESIAN_POINT('Ctrl Pts',(1.13892796699994,15.2,-11.321095772));
#155513=CARTESIAN_POINT('Ctrl Pts',(1.13892796699994,11.6,-11.321095772));
#155514=CARTESIAN_POINT('Ctrl Pts',(1.14011582299994,15.2,-11.317634312));
#155515=CARTESIAN_POINT('Ctrl Pts',(1.14011582299994,11.6,-11.317634312));
#155516=CARTESIAN_POINT('Ctrl Pts',(1.14129953199994,15.2,-11.31417626));
#155517=CARTESIAN_POINT('Ctrl Pts',(1.14129953199994,11.6,-11.31417626));
#155518=CARTESIAN_POINT('Ctrl Pts',(1.14247909799994,15.2,-11.310721625));
#155519=CARTESIAN_POINT('Ctrl Pts',(1.14247909799994,11.6,-11.310721625));
#155520=CARTESIAN_POINT('Ctrl Pts',(1.14365452599994,15.2,-11.307270414));
#155521=CARTESIAN_POINT('Ctrl Pts',(1.14365452599994,11.6,-11.307270414));
#155522=CARTESIAN_POINT('Ctrl Pts',(1.14482581499994,15.2,-11.303822638));
#155523=CARTESIAN_POINT('Ctrl Pts',(1.14482581499994,11.6,-11.303822638));
#155524=CARTESIAN_POINT('Ctrl Pts',(1.14599297199994,15.2,-11.300378306));
#155525=CARTESIAN_POINT('Ctrl Pts',(1.14599297199994,11.6,-11.300378306));
#155526=CARTESIAN_POINT('Ctrl Pts',(1.14715599899994,15.2,-11.296937426));
#155527=CARTESIAN_POINT('Ctrl Pts',(1.14715599899994,11.6,-11.296937426));
#155528=CARTESIAN_POINT('Ctrl Pts',(1.14831489899994,15.2,-11.293500006));
#155529=CARTESIAN_POINT('Ctrl Pts',(1.14831489899994,11.6,-11.293500006));
#155530=CARTESIAN_POINT('Ctrl Pts',(1.14946967399994,15.2,-11.290066057));
#155531=CARTESIAN_POINT('Ctrl Pts',(1.14946967399994,11.6,-11.290066057));
#155532=CARTESIAN_POINT('Ctrl Pts',(1.15062032899994,15.2,-11.286635586));
#155533=CARTESIAN_POINT('Ctrl Pts',(1.15062032899994,11.6,-11.286635586));
#155534=CARTESIAN_POINT('Ctrl Pts',(1.15176686799994,15.2,-11.283208603));
#155535=CARTESIAN_POINT('Ctrl Pts',(1.15176686799994,11.6,-11.283208603));
#155536=CARTESIAN_POINT('Ctrl Pts',(1.15290929199994,15.2,-11.279785118));
#155537=CARTESIAN_POINT('Ctrl Pts',(1.15290929199994,11.6,-11.279785118));
#155538=CARTESIAN_POINT('Ctrl Pts',(1.15404760399994,15.2,-11.276365138));
#155539=CARTESIAN_POINT('Ctrl Pts',(1.15404760399994,11.6,-11.276365138));
#155540=CARTESIAN_POINT('Ctrl Pts',(1.15518180899994,15.2,-11.272948673));
#155541=CARTESIAN_POINT('Ctrl Pts',(1.15518180899994,11.6,-11.272948673));
#155542=CARTESIAN_POINT('Ctrl Pts',(1.15631190999994,15.2,-11.269535732));
#155543=CARTESIAN_POINT('Ctrl Pts',(1.15631190999994,11.6,-11.269535732));
#155544=CARTESIAN_POINT('Ctrl Pts',(1.15743790999994,15.2,-11.266126325));
#155545=CARTESIAN_POINT('Ctrl Pts',(1.15743790999994,11.6,-11.266126325));
#155546=CARTESIAN_POINT('Ctrl Pts',(1.15855981299994,15.2,-11.262720459));
#155547=CARTESIAN_POINT('Ctrl Pts',(1.15855981299994,11.6,-11.262720459));
#155548=CARTESIAN_POINT('Ctrl Pts',(1.15967762099994,15.2,-11.259318144));
#155549=CARTESIAN_POINT('Ctrl Pts',(1.15967762099994,11.6,-11.259318144));
#155550=CARTESIAN_POINT('Ctrl Pts',(1.16079133799994,15.2,-11.25591939));
#155551=CARTESIAN_POINT('Ctrl Pts',(1.16079133799994,11.6,-11.25591939));
#155552=CARTESIAN_POINT('Ctrl Pts',(1.16190096699994,15.2,-11.252524204));
#155553=CARTESIAN_POINT('Ctrl Pts',(1.16190096699994,11.6,-11.252524204));
#155554=CARTESIAN_POINT('Ctrl Pts',(1.16300651299994,15.2,-11.249132598));
#155555=CARTESIAN_POINT('Ctrl Pts',(1.16300651299994,11.6,-11.249132598));
#155556=CARTESIAN_POINT('Ctrl Pts',(1.16410797799994,15.2,-11.245744578));
#155557=CARTESIAN_POINT('Ctrl Pts',(1.16410797799994,11.6,-11.245744578));
#155558=CARTESIAN_POINT('Ctrl Pts',(1.16520536399994,15.2,-11.242360155));
#155559=CARTESIAN_POINT('Ctrl Pts',(1.16520536399994,11.6,-11.242360155));
#155560=CARTESIAN_POINT('Ctrl Pts',(1.16629867699995,15.2,-11.238979338));
#155561=CARTESIAN_POINT('Ctrl Pts',(1.16629867699995,11.6,-11.238979338));
#155562=CARTESIAN_POINT('Ctrl Pts',(1.16738791999994,15.2,-11.235602136));
#155563=CARTESIAN_POINT('Ctrl Pts',(1.16738791999994,11.6,-11.235602136));
#155564=CARTESIAN_POINT('Ctrl Pts',(1.16847309399994,15.2,-11.232228557));
#155565=CARTESIAN_POINT('Ctrl Pts',(1.16847309399994,11.6,-11.232228557));
#155566=CARTESIAN_POINT('Ctrl Pts',(1.16955420599994,15.2,-11.228858612));
#155567=CARTESIAN_POINT('Ctrl Pts',(1.16955420599994,11.6,-11.228858612));
#155568=CARTESIAN_POINT('Ctrl Pts',(1.17063125699994,15.2,-11.22549231));
#155569=CARTESIAN_POINT('Ctrl Pts',(1.17063125699994,11.6,-11.22549231));
#155570=CARTESIAN_POINT('Ctrl Pts',(1.17170425099994,15.2,-11.222129659));
#155571=CARTESIAN_POINT('Ctrl Pts',(1.17170425099994,11.6,-11.222129659));
#155572=CARTESIAN_POINT('Ctrl Pts',(1.17277319199994,15.2,-11.218770669));
#155573=CARTESIAN_POINT('Ctrl Pts',(1.17277319199994,11.6,-11.218770669));
#155574=CARTESIAN_POINT('Ctrl Pts',(1.17383808199994,15.2,-11.215415349));
#155575=CARTESIAN_POINT('Ctrl Pts',(1.17383808199994,11.6,-11.215415349));
#155576=CARTESIAN_POINT('Ctrl Pts',(1.17489892699994,15.2,-11.212063708));
#155577=CARTESIAN_POINT('Ctrl Pts',(1.17489892699994,11.6,-11.212063708));
#155578=CARTESIAN_POINT('Ctrl Pts',(1.17595572899994,15.2,-11.208715756));
#155579=CARTESIAN_POINT('Ctrl Pts',(1.17595572899994,11.6,-11.208715756));
#155580=CARTESIAN_POINT('Ctrl Pts',(1.17700849199994,15.2,-11.205371503));
#155581=CARTESIAN_POINT('Ctrl Pts',(1.17700849199994,11.6,-11.205371503));
#155582=CARTESIAN_POINT('Ctrl Pts',(1.17805721899994,15.2,-11.202030955));
#155583=CARTESIAN_POINT('Ctrl Pts',(1.17805721899994,11.6,-11.202030955));
#155584=CARTESIAN_POINT('Ctrl Pts',(1.17910191399994,15.2,-11.198694125));
#155585=CARTESIAN_POINT('Ctrl Pts',(1.17910191399994,11.6,-11.198694125));
#155586=CARTESIAN_POINT('Ctrl Pts',(1.18014258099994,15.2,-11.195361021));
#155587=CARTESIAN_POINT('Ctrl Pts',(1.18014258099994,11.6,-11.195361021));
#155588=CARTESIAN_POINT('Ctrl Pts',(1.18117922299994,15.2,-11.192031652));
#155589=CARTESIAN_POINT('Ctrl Pts',(1.18117922299994,11.6,-11.192031652));
#155590=CARTESIAN_POINT('Ctrl Pts',(1.18221184299994,15.2,-11.188706028));
#155591=CARTESIAN_POINT('Ctrl Pts',(1.18221184299994,11.6,-11.188706028));
#155592=CARTESIAN_POINT('Ctrl Pts',(1.18324044599994,15.2,-11.185384157));
#155593=CARTESIAN_POINT('Ctrl Pts',(1.18324044599994,11.6,-11.185384157));
#155594=CARTESIAN_POINT('Ctrl Pts',(1.18426503499994,15.2,-11.18206605));
#155595=CARTESIAN_POINT('Ctrl Pts',(1.18426503499994,11.6,-11.18206605));
#155596=CARTESIAN_POINT('Ctrl Pts',(1.18528561399994,15.2,-11.178751715));
#155597=CARTESIAN_POINT('Ctrl Pts',(1.18528561399994,11.6,-11.178751715));
#155598=CARTESIAN_POINT('Ctrl Pts',(1.18630218599994,15.2,-11.175441163));
#155599=CARTESIAN_POINT('Ctrl Pts',(1.18630218599994,11.6,-11.175441163));
#155600=CARTESIAN_POINT('Ctrl Pts',(1.18731475499994,15.2,-11.172134402));
#155601=CARTESIAN_POINT('Ctrl Pts',(1.18731475499994,11.6,-11.172134402));
#155602=CARTESIAN_POINT('Ctrl Pts',(1.18832332499994,15.2,-11.168831442));
#155603=CARTESIAN_POINT('Ctrl Pts',(1.18832332499994,11.6,-11.168831442));
#155604=CARTESIAN_POINT('Ctrl Pts',(1.18932789799994,15.2,-11.165532292));
#155605=CARTESIAN_POINT('Ctrl Pts',(1.18932789799994,11.6,-11.165532292));
#155606=CARTESIAN_POINT('Ctrl Pts',(1.19032848099994,15.2,-11.162236962));
#155607=CARTESIAN_POINT('Ctrl Pts',(1.19032848099994,11.6,-11.162236962));
#155608=CARTESIAN_POINT('Ctrl Pts',(1.19132507499994,15.2,-11.158945462));
#155609=CARTESIAN_POINT('Ctrl Pts',(1.19132507499994,11.6,-11.158945462));
#155610=CARTESIAN_POINT('Ctrl Pts',(1.19231768599994,15.2,-11.155657801));
#155611=CARTESIAN_POINT('Ctrl Pts',(1.19231768599994,11.6,-11.155657801));
#155612=CARTESIAN_POINT('Ctrl Pts',(1.19330631499994,15.2,-11.152373988));
#155613=CARTESIAN_POINT('Ctrl Pts',(1.19330631499994,11.6,-11.152373988));
#155614=CARTESIAN_POINT('Ctrl Pts',(1.19429096799994,15.2,-11.149094033));
#155615=CARTESIAN_POINT('Ctrl Pts',(1.19429096799994,11.6,-11.149094033));
#155616=CARTESIAN_POINT('Ctrl Pts',(1.19527164899994,15.2,-11.145817945));
#155617=CARTESIAN_POINT('Ctrl Pts',(1.19527164899994,11.6,-11.145817945));
#155618=CARTESIAN_POINT('Ctrl Pts',(1.19624835999994,15.2,-11.142545735));
#155619=CARTESIAN_POINT('Ctrl Pts',(1.19624835999994,11.6,-11.142545735));
#155620=CARTESIAN_POINT('Ctrl Pts',(1.19722110599994,15.2,-11.139277411));
#155621=CARTESIAN_POINT('Ctrl Pts',(1.19722110599994,11.6,-11.139277411));
#155622=CARTESIAN_POINT('Ctrl Pts',(1.19818989099994,15.2,-11.136012983));
#155623=CARTESIAN_POINT('Ctrl Pts',(1.19818989099994,11.6,-11.136012983));
#155624=CARTESIAN_POINT('Ctrl Pts',(1.19915471699994,15.2,-11.132752462));
#155625=CARTESIAN_POINT('Ctrl Pts',(1.19915471699994,11.6,-11.132752462));
#155626=CARTESIAN_POINT('Ctrl Pts',(1.20011559099995,15.2,-11.129495855));
#155627=CARTESIAN_POINT('Ctrl Pts',(1.20011559099995,11.6,-11.129495855));
#155628=CARTESIAN_POINT('Ctrl Pts',(1.20107251499994,15.2,-11.126243174));
#155629=CARTESIAN_POINT('Ctrl Pts',(1.20107251499994,11.6,-11.126243174));
#155630=CARTESIAN_POINT('Ctrl Pts',(1.20202549299994,15.2,-11.122994428));
#155631=CARTESIAN_POINT('Ctrl Pts',(1.20202549299994,11.6,-11.122994428));
#155632=CARTESIAN_POINT('Ctrl Pts',(1.20297452899994,15.2,-11.119749625));
#155633=CARTESIAN_POINT('Ctrl Pts',(1.20297452899994,11.6,-11.119749625));
#155634=CARTESIAN_POINT('Ctrl Pts',(1.20391962699994,15.2,-11.116508778));
#155635=CARTESIAN_POINT('Ctrl Pts',(1.20391962699994,11.6,-11.116508778));
#155636=CARTESIAN_POINT('Ctrl Pts',(1.20486078999994,15.2,-11.113271894));
#155637=CARTESIAN_POINT('Ctrl Pts',(1.20486078999994,11.6,-11.113271894));
#155638=CARTESIAN_POINT('Ctrl Pts',(1.20579802499994,15.2,-11.110038983));
#155639=CARTESIAN_POINT('Ctrl Pts',(1.20579802499994,11.6,-11.110038983));
#155640=CARTESIAN_POINT('Ctrl Pts',(1.20673133299994,15.2,-11.106810055));
#155641=CARTESIAN_POINT('Ctrl Pts',(1.20673133299994,11.6,-11.106810055));
#155642=CARTESIAN_POINT('Ctrl Pts',(1.20766071899994,15.2,-11.103585121));
#155643=CARTESIAN_POINT('Ctrl Pts',(1.20766071899994,11.6,-11.103585121));
#155644=CARTESIAN_POINT('Ctrl Pts',(1.20858618699994,15.2,-11.100364189));
#155645=CARTESIAN_POINT('Ctrl Pts',(1.20858618699994,11.6,-11.100364189));
#155646=CARTESIAN_POINT('Ctrl Pts',(1.20950774199994,15.2,-11.09714727));
#155647=CARTESIAN_POINT('Ctrl Pts',(1.20950774199994,11.6,-11.09714727));
#155648=CARTESIAN_POINT('Ctrl Pts',(1.21042538699994,15.2,-11.093934372));
#155649=CARTESIAN_POINT('Ctrl Pts',(1.21042538699994,11.6,-11.093934372));
#155650=CARTESIAN_POINT('Ctrl Pts',(1.21133912499995,15.2,-11.090725508));
#155651=CARTESIAN_POINT('Ctrl Pts',(1.21133912499995,11.6,-11.090725508));
#155652=CARTESIAN_POINT('Ctrl Pts',(1.21224896299994,15.2,-11.087520685));
#155653=CARTESIAN_POINT('Ctrl Pts',(1.21224896299994,11.6,-11.087520685));
#155654=CARTESIAN_POINT('Ctrl Pts',(1.21315490199994,15.2,-11.084319915));
#155655=CARTESIAN_POINT('Ctrl Pts',(1.21315490199994,11.6,-11.084319915));
#155656=CARTESIAN_POINT('Ctrl Pts',(1.21405694699994,15.2,-11.081123205));
#155657=CARTESIAN_POINT('Ctrl Pts',(1.21405694699994,11.6,-11.081123205));
#155658=CARTESIAN_POINT('Ctrl Pts',(1.21495510399994,15.2,-11.077930567));
#155659=CARTESIAN_POINT('Ctrl Pts',(1.21495510399994,11.6,-11.077930567));
#155660=CARTESIAN_POINT('Ctrl Pts',(1.21584937499994,15.2,-11.074742011));
#155661=CARTESIAN_POINT('Ctrl Pts',(1.21584937499994,11.6,-11.074742011));
#155662=CARTESIAN_POINT('Ctrl Pts',(1.21673976599994,15.2,-11.071557546));
#155663=CARTESIAN_POINT('Ctrl Pts',(1.21673976599994,11.6,-11.071557546));
#155664=CARTESIAN_POINT('Ctrl Pts',(1.21762627899994,15.2,-11.068377182));
#155665=CARTESIAN_POINT('Ctrl Pts',(1.21762627899994,11.6,-11.068377182));
#155666=CARTESIAN_POINT('Ctrl Pts',(1.21850891999994,15.2,-11.06520093));
#155667=CARTESIAN_POINT('Ctrl Pts',(1.21850891999994,11.6,-11.06520093));
#155668=CARTESIAN_POINT('Ctrl Pts',(1.21938769199994,15.2,-11.062028798));
#155669=CARTESIAN_POINT('Ctrl Pts',(1.21938769199994,11.6,-11.062028798));
#155670=CARTESIAN_POINT('Ctrl Pts',(1.22026259999994,15.2,-11.058860798));
#155671=CARTESIAN_POINT('Ctrl Pts',(1.22026259999994,11.6,-11.058860798));
#155672=CARTESIAN_POINT('Ctrl Pts',(1.22113364899994,15.2,-11.055696939));
#155673=CARTESIAN_POINT('Ctrl Pts',(1.22113364899994,11.6,-11.055696939));
#155674=CARTESIAN_POINT('Ctrl Pts',(1.22200084099994,15.2,-11.052537231));
#155675=CARTESIAN_POINT('Ctrl Pts',(1.22200084099994,11.6,-11.052537231));
#155676=CARTESIAN_POINT('Ctrl Pts',(1.22286418199994,15.2,-11.049381684));
#155677=CARTESIAN_POINT('Ctrl Pts',(1.22286418199994,11.6,-11.049381684));
#155678=CARTESIAN_POINT('Ctrl Pts',(1.22372367599994,15.2,-11.046230309));
#155679=CARTESIAN_POINT('Ctrl Pts',(1.22372367599994,11.6,-11.046230309));
#155680=CARTESIAN_POINT('Ctrl Pts',(1.22457932699994,15.2,-11.043083114));
#155681=CARTESIAN_POINT('Ctrl Pts',(1.22457932699994,11.6,-11.043083114));
#155682=CARTESIAN_POINT('Ctrl Pts',(1.22543113999994,15.2,-11.03994011));
#155683=CARTESIAN_POINT('Ctrl Pts',(1.22543113999994,11.6,-11.03994011));
#155684=CARTESIAN_POINT('Ctrl Pts',(1.22627911799994,15.2,-11.036801309));
#155685=CARTESIAN_POINT('Ctrl Pts',(1.22627911799994,11.6,-11.036801309));
#155686=CARTESIAN_POINT('Ctrl Pts',(1.22712326699994,15.2,-11.033666719));
#155687=CARTESIAN_POINT('Ctrl Pts',(1.22712326699994,11.6,-11.033666719));
#155688=CARTESIAN_POINT('Ctrl Pts',(1.22796359099994,15.2,-11.030536351));
#155689=CARTESIAN_POINT('Ctrl Pts',(1.22796359099994,11.6,-11.030536351));
#155690=CARTESIAN_POINT('Ctrl Pts',(1.22880009299994,15.2,-11.027410214));
#155691=CARTESIAN_POINT('Ctrl Pts',(1.22880009299994,11.6,-11.027410214));
#155692=CARTESIAN_POINT('Ctrl Pts',(1.22963277899994,15.2,-11.024288319));
#155693=CARTESIAN_POINT('Ctrl Pts',(1.22963277899994,11.6,-11.024288319));
#155694=CARTESIAN_POINT('Ctrl Pts',(1.23046165299994,15.2,-11.021170677));
#155695=CARTESIAN_POINT('Ctrl Pts',(1.23046165299994,11.6,-11.021170677));
#155696=CARTESIAN_POINT('Ctrl Pts',(1.23128671899994,15.2,-11.018057297));
#155697=CARTESIAN_POINT('Ctrl Pts',(1.23128671899994,11.6,-11.018057297));
#155698=CARTESIAN_POINT('Ctrl Pts',(1.23210798199994,15.2,-11.01494819));
#155699=CARTESIAN_POINT('Ctrl Pts',(1.23210798199994,11.6,-11.01494819));
#155700=CARTESIAN_POINT('Ctrl Pts',(1.23292544599995,15.2,-11.011843364));
#155701=CARTESIAN_POINT('Ctrl Pts',(1.23292544599995,11.6,-11.011843364));
#155702=CARTESIAN_POINT('Ctrl Pts',(1.23373911599994,15.2,-11.008742833));
#155703=CARTESIAN_POINT('Ctrl Pts',(1.23373911599994,11.6,-11.008742833));
#155704=CARTESIAN_POINT('Ctrl Pts',(1.23454899599994,15.2,-11.005646604));
#155705=CARTESIAN_POINT('Ctrl Pts',(1.23454899599994,11.6,-11.005646604));
#155706=CARTESIAN_POINT('Ctrl Pts',(1.23535509099994,15.2,-11.002554689));
#155707=CARTESIAN_POINT('Ctrl Pts',(1.23535509099994,11.6,-11.002554689));
#155708=CARTESIAN_POINT('Ctrl Pts',(1.23615740499994,15.2,-10.999467099));
#155709=CARTESIAN_POINT('Ctrl Pts',(1.23615740499994,11.6,-10.999467099));
#155710=CARTESIAN_POINT('Ctrl Pts',(1.23695594399994,15.2,-10.996383842));
#155711=CARTESIAN_POINT('Ctrl Pts',(1.23695594399994,11.6,-10.996383842));
#155712=CARTESIAN_POINT('Ctrl Pts',(1.23775071099994,15.2,-10.99330493));
#155713=CARTESIAN_POINT('Ctrl Pts',(1.23775071099994,11.6,-10.99330493));
#155714=CARTESIAN_POINT('Ctrl Pts',(1.23854171099994,15.2,-10.990230373));
#155715=CARTESIAN_POINT('Ctrl Pts',(1.23854171099994,11.6,-10.990230373));
#155716=CARTESIAN_POINT('Ctrl Pts',(1.23932894799994,15.2,-10.98716018));
#155717=CARTESIAN_POINT('Ctrl Pts',(1.23932894799994,11.6,-10.98716018));
#155718=CARTESIAN_POINT('Ctrl Pts',(1.24011242899994,15.2,-10.984094365));
#155719=CARTESIAN_POINT('Ctrl Pts',(1.24011242899994,11.6,-10.984094365));
#155720=CARTESIAN_POINT('Ctrl Pts',(1.24089215599994,15.2,-10.981032935));
#155721=CARTESIAN_POINT('Ctrl Pts',(1.24089215599994,11.6,-10.981032935));
#155722=CARTESIAN_POINT('Ctrl Pts',(1.24166813499994,15.2,-10.977975901));
#155723=CARTESIAN_POINT('Ctrl Pts',(1.24166813499994,11.6,-10.977975901));
#155724=CARTESIAN_POINT('Ctrl Pts',(1.24244037099994,15.2,-10.974923275));
#155725=CARTESIAN_POINT('Ctrl Pts',(1.24244037099994,11.6,-10.974923275));
#155726=CARTESIAN_POINT('Ctrl Pts',(1.24320886799994,15.2,-10.971875066));
#155727=CARTESIAN_POINT('Ctrl Pts',(1.24320886799994,11.6,-10.971875066));
#155728=CARTESIAN_POINT('Ctrl Pts',(1.24397362999994,15.2,-10.968831284));
#155729=CARTESIAN_POINT('Ctrl Pts',(1.24397362999994,11.6,-10.968831284));
#155730=CARTESIAN_POINT('Ctrl Pts',(1.24473466399994,15.2,-10.965791941));
#155731=CARTESIAN_POINT('Ctrl Pts',(1.24473466399994,11.6,-10.965791941));
#155732=CARTESIAN_POINT('Ctrl Pts',(1.24549197299994,15.2,-10.962757048));
#155733=CARTESIAN_POINT('Ctrl Pts',(1.24549197299994,11.6,-10.962757048));
#155734=CARTESIAN_POINT('Ctrl Pts',(1.24624556199994,15.2,-10.959726614));
#155735=CARTESIAN_POINT('Ctrl Pts',(1.24624556199994,11.6,-10.959726614));
#155736=CARTESIAN_POINT('Ctrl Pts',(1.24699543599994,15.2,-10.95670065));
#155737=CARTESIAN_POINT('Ctrl Pts',(1.24699543599994,11.6,-10.95670065));
#155738=CARTESIAN_POINT('Ctrl Pts',(1.24774159999994,15.2,-10.953679166));
#155739=CARTESIAN_POINT('Ctrl Pts',(1.24774159999994,11.6,-10.953679166));
#155740=CARTESIAN_POINT('Ctrl Pts',(1.24848405899994,15.2,-10.950662174));
#155741=CARTESIAN_POINT('Ctrl Pts',(1.24848405899994,11.6,-10.950662174));
#155742=CARTESIAN_POINT('Ctrl Pts',(1.24922281699994,15.2,-10.947649684));
#155743=CARTESIAN_POINT('Ctrl Pts',(1.24922281699994,11.6,-10.947649684));
#155744=CARTESIAN_POINT('Ctrl Pts',(1.24995787899994,15.2,-10.944641705));
#155745=CARTESIAN_POINT('Ctrl Pts',(1.24995787899994,11.6,-10.944641705));
#155746=CARTESIAN_POINT('Ctrl Pts',(1.25068925199994,15.2,-10.941638251));
#155747=CARTESIAN_POINT('Ctrl Pts',(1.25068925199994,11.6,-10.941638251));
#155748=CARTESIAN_POINT('Ctrl Pts',(1.25141693799994,15.2,-10.93863933));
#155749=CARTESIAN_POINT('Ctrl Pts',(1.25141693799994,11.6,-10.93863933));
#155750=CARTESIAN_POINT('Ctrl Pts',(1.25214094299994,15.2,-10.935644954));
#155751=CARTESIAN_POINT('Ctrl Pts',(1.25214094299994,11.6,-10.935644954));
#155752=CARTESIAN_POINT('Ctrl Pts',(1.25286127299994,15.2,-10.932655133));
#155753=CARTESIAN_POINT('Ctrl Pts',(1.25286127299994,11.6,-10.932655133));
#155754=CARTESIAN_POINT('Ctrl Pts',(1.25357793199994,15.2,-10.929669878));
#155755=CARTESIAN_POINT('Ctrl Pts',(1.25357793199994,11.6,-10.929669878));
#155756=CARTESIAN_POINT('Ctrl Pts',(1.25429092499994,15.2,-10.9266892));
#155757=CARTESIAN_POINT('Ctrl Pts',(1.25429092499994,11.6,-10.9266892));
#155758=CARTESIAN_POINT('Ctrl Pts',(1.25500025699994,15.2,-10.923713108));
#155759=CARTESIAN_POINT('Ctrl Pts',(1.25500025699994,11.6,-10.923713108));
#155760=CARTESIAN_POINT('Ctrl Pts',(1.25570593399994,15.2,-10.920741616));
#155761=CARTESIAN_POINT('Ctrl Pts',(1.25570593399994,11.6,-10.920741616));
#155762=CARTESIAN_POINT('Ctrl Pts',(1.25640795899994,15.2,-10.917774733));
#155763=CARTESIAN_POINT('Ctrl Pts',(1.25640795899994,11.6,-10.917774733));
#155764=CARTESIAN_POINT('Ctrl Pts',(1.25710633899994,15.2,-10.91481247));
#155765=CARTESIAN_POINT('Ctrl Pts',(1.25710633899994,11.6,-10.91481247));
#155766=CARTESIAN_POINT('Ctrl Pts',(1.25780107799994,15.2,-10.911854838));
#155767=CARTESIAN_POINT('Ctrl Pts',(1.25780107799994,11.6,-10.911854838));
#155768=CARTESIAN_POINT('Ctrl Pts',(1.25849218299994,15.2,-10.908901847));
#155769=CARTESIAN_POINT('Ctrl Pts',(1.25849218299994,11.6,-10.908901847));
#155770=CARTESIAN_POINT('Ctrl Pts',(1.25917965599994,15.2,-10.905953509));
#155771=CARTESIAN_POINT('Ctrl Pts',(1.25917965599994,11.6,-10.905953509));
#155772=CARTESIAN_POINT('Ctrl Pts',(1.25986350399994,15.2,-10.903009834));
#155773=CARTESIAN_POINT('Ctrl Pts',(1.25986350399994,11.6,-10.903009834));
#155774=CARTESIAN_POINT('Ctrl Pts',(1.26054373299994,15.2,-10.900070834));
#155775=CARTESIAN_POINT('Ctrl Pts',(1.26054373299994,11.6,-10.900070834));
#155776=CARTESIAN_POINT('Ctrl Pts',(1.26122034599994,15.2,-10.89713652));
#155777=CARTESIAN_POINT('Ctrl Pts',(1.26122034599994,11.6,-10.89713652));
#155778=CARTESIAN_POINT('Ctrl Pts',(1.26189334999994,15.2,-10.894206901));
#155779=CARTESIAN_POINT('Ctrl Pts',(1.26189334999994,11.6,-10.894206901));
#155780=CARTESIAN_POINT('Ctrl Pts',(1.26256274999994,15.2,-10.89128199));
#155781=CARTESIAN_POINT('Ctrl Pts',(1.26256274999994,11.6,-10.89128199));
#155782=CARTESIAN_POINT('Ctrl Pts',(1.26322855099994,15.2,-10.888361798));
#155783=CARTESIAN_POINT('Ctrl Pts',(1.26322855099994,11.6,-10.888361798));
#155784=CARTESIAN_POINT('Ctrl Pts',(1.26389075699994,15.2,-10.885446335));
#155785=CARTESIAN_POINT('Ctrl Pts',(1.26389075699994,11.6,-10.885446335));
#155786=CARTESIAN_POINT('Ctrl Pts',(1.26454937499994,15.2,-10.882535612));
#155787=CARTESIAN_POINT('Ctrl Pts',(1.26454937499994,11.6,-10.882535612));
#155788=CARTESIAN_POINT('Ctrl Pts',(1.26520440999994,15.2,-10.879629641));
#155789=CARTESIAN_POINT('Ctrl Pts',(1.26520440999994,11.6,-10.879629641));
#155790=CARTESIAN_POINT('Ctrl Pts',(1.26585586699994,15.2,-10.876728433));
#155791=CARTESIAN_POINT('Ctrl Pts',(1.26585586699994,11.6,-10.876728433));
#155792=CARTESIAN_POINT('Ctrl Pts',(1.26650375199994,15.2,-10.873831999));
#155793=CARTESIAN_POINT('Ctrl Pts',(1.26650375199994,11.6,-10.873831999));
#155794=CARTESIAN_POINT('Ctrl Pts',(1.26714806899994,15.2,-10.870940349));
#155795=CARTESIAN_POINT('Ctrl Pts',(1.26714806899994,11.6,-10.870940349));
#155796=CARTESIAN_POINT('Ctrl Pts',(1.26778882499994,15.2,-10.868053496));
#155797=CARTESIAN_POINT('Ctrl Pts',(1.26778882499994,11.6,-10.868053496));
#155798=CARTESIAN_POINT('Ctrl Pts',(1.26842602399994,15.2,-10.86517145));
#155799=CARTESIAN_POINT('Ctrl Pts',(1.26842602399994,11.6,-10.86517145));
#155800=CARTESIAN_POINT('Ctrl Pts',(1.26905967299994,15.2,-10.862294222));
#155801=CARTESIAN_POINT('Ctrl Pts',(1.26905967299994,11.6,-10.862294222));
#155802=CARTESIAN_POINT('Ctrl Pts',(1.26968977599994,15.2,-10.859421825));
#155803=CARTESIAN_POINT('Ctrl Pts',(1.26968977599994,11.6,-10.859421825));
#155804=CARTESIAN_POINT('Ctrl Pts',(1.27031633899994,15.2,-10.856554267));
#155805=CARTESIAN_POINT('Ctrl Pts',(1.27031633899994,11.6,-10.856554267));
#155806=CARTESIAN_POINT('Ctrl Pts',(1.27093936699994,15.2,-10.853691563));
#155807=CARTESIAN_POINT('Ctrl Pts',(1.27093936699994,11.6,-10.853691563));
#155808=CARTESIAN_POINT('Ctrl Pts',(1.27155886699994,15.2,-10.850833723));
#155809=CARTESIAN_POINT('Ctrl Pts',(1.27155886699994,11.6,-10.850833723));
#155810=CARTESIAN_POINT('Ctrl Pts',(1.27217484299994,15.2,-10.847980757));
#155811=CARTESIAN_POINT('Ctrl Pts',(1.27217484299994,11.6,-10.847980757));
#155812=CARTESIAN_POINT('Ctrl Pts',(1.27278730099994,15.2,-10.845132677));
#155813=CARTESIAN_POINT('Ctrl Pts',(1.27278730099994,11.6,-10.845132677));
#155814=CARTESIAN_POINT('Ctrl Pts',(1.27339624799994,15.2,-10.842289496));
#155815=CARTESIAN_POINT('Ctrl Pts',(1.27339624799994,11.6,-10.842289496));
#155816=CARTESIAN_POINT('Ctrl Pts',(1.27400168799994,15.2,-10.839451223));
#155817=CARTESIAN_POINT('Ctrl Pts',(1.27400168799994,11.6,-10.839451223));
#155818=CARTESIAN_POINT('Ctrl Pts',(1.27460362599994,15.2,-10.83661787));
#155819=CARTESIAN_POINT('Ctrl Pts',(1.27460362599994,11.6,-10.83661787));
#155820=CARTESIAN_POINT('Ctrl Pts',(1.27520206999994,15.2,-10.833789449));
#155821=CARTESIAN_POINT('Ctrl Pts',(1.27520206999994,11.6,-10.833789449));
#155822=CARTESIAN_POINT('Ctrl Pts',(1.27579702299994,15.2,-10.830965973));
#155823=CARTESIAN_POINT('Ctrl Pts',(1.27579702299994,11.6,-10.830965973));
#155824=CARTESIAN_POINT('Ctrl Pts',(1.27638849299994,15.2,-10.828147449));
#155825=CARTESIAN_POINT('Ctrl Pts',(1.27638849299994,11.6,-10.828147449));
#155826=CARTESIAN_POINT('Ctrl Pts',(1.27697648499994,15.2,-10.825333894));
#155827=CARTESIAN_POINT('Ctrl Pts',(1.27697648499994,11.6,-10.825333894));
#155828=CARTESIAN_POINT('Ctrl Pts',(1.27756100499994,15.2,-10.822525316));
#155829=CARTESIAN_POINT('Ctrl Pts',(1.27756100499994,11.6,-10.822525316));
#155830=CARTESIAN_POINT('Ctrl Pts',(1.27814205599994,15.2,-10.819721726));
#155831=CARTESIAN_POINT('Ctrl Pts',(1.27814205599994,11.6,-10.819721726));
#155832=CARTESIAN_POINT('Ctrl Pts',(1.27871964799994,15.2,-10.816923139));
#155833=CARTESIAN_POINT('Ctrl Pts',(1.27871964799994,11.6,-10.816923139));
#155834=CARTESIAN_POINT('Ctrl Pts',(1.27929378499994,15.2,-10.814129563));
#155835=CARTESIAN_POINT('Ctrl Pts',(1.27929378499994,11.6,-10.814129563));
#155836=CARTESIAN_POINT('Ctrl Pts',(1.27986447099994,15.2,-10.811341012));
#155837=CARTESIAN_POINT('Ctrl Pts',(1.27986447099994,11.6,-10.811341012));
#155838=CARTESIAN_POINT('Ctrl Pts',(1.28043171499994,15.2,-10.808557497));
#155839=CARTESIAN_POINT('Ctrl Pts',(1.28043171499994,11.6,-10.808557497));
#155840=CARTESIAN_POINT('Ctrl Pts',(1.28099552199994,15.2,-10.805779028));
#155841=CARTESIAN_POINT('Ctrl Pts',(1.28099552199994,11.6,-10.805779028));
#155842=CARTESIAN_POINT('Ctrl Pts',(1.28155589699994,15.2,-10.80300562));
#155843=CARTESIAN_POINT('Ctrl Pts',(1.28155589699994,11.6,-10.80300562));
#155844=CARTESIAN_POINT('Ctrl Pts',(1.28211284599994,15.2,-10.800237282));
#155845=CARTESIAN_POINT('Ctrl Pts',(1.28211284599994,11.6,-10.800237282));
#155846=CARTESIAN_POINT('Ctrl Pts',(1.28266637399994,15.2,-10.797474026));
#155847=CARTESIAN_POINT('Ctrl Pts',(1.28266637399994,11.6,-10.797474026));
#155848=CARTESIAN_POINT('Ctrl Pts',(1.28321648999994,15.2,-10.794715865));
#155849=CARTESIAN_POINT('Ctrl Pts',(1.28321648999994,11.6,-10.794715865));
#155850=CARTESIAN_POINT('Ctrl Pts',(1.28376319699994,15.2,-10.791962811));
#155851=CARTESIAN_POINT('Ctrl Pts',(1.28376319699994,11.6,-10.791962811));
#155852=CARTESIAN_POINT('Ctrl Pts',(1.28430650299994,15.2,-10.789214873));
#155853=CARTESIAN_POINT('Ctrl Pts',(1.28430650299994,11.6,-10.789214873));
#155854=CARTESIAN_POINT('Ctrl Pts',(1.28484641299994,15.2,-10.786472067));
#155855=CARTESIAN_POINT('Ctrl Pts',(1.28484641299994,11.6,-10.786472067));
#155856=CARTESIAN_POINT('Ctrl Pts',(1.28538293299994,15.2,-10.7837344));
#155857=CARTESIAN_POINT('Ctrl Pts',(1.28538293299994,11.6,-10.7837344));
#155858=CARTESIAN_POINT('Ctrl Pts',(1.28591606999994,15.2,-10.781001888));
#155859=CARTESIAN_POINT('Ctrl Pts',(1.28591606999994,11.6,-10.781001888));
#155860=CARTESIAN_POINT('Ctrl Pts',(1.28644582999994,15.2,-10.778274541));
#155861=CARTESIAN_POINT('Ctrl Pts',(1.28644582999994,11.6,-10.778274541));
#155862=CARTESIAN_POINT('Ctrl Pts',(1.28697221699994,15.2,-10.775552372));
#155863=CARTESIAN_POINT('Ctrl Pts',(1.28697221699994,11.6,-10.775552372));
#155864=CARTESIAN_POINT('Ctrl Pts',(1.28749524099994,15.2,-10.772835393));
#155865=CARTESIAN_POINT('Ctrl Pts',(1.28749524099994,11.6,-10.772835393));
#155866=CARTESIAN_POINT('Ctrl Pts',(1.28801490399994,15.2,-10.770123614));
#155867=CARTESIAN_POINT('Ctrl Pts',(1.28801490399994,11.6,-10.770123614));
#155868=CARTESIAN_POINT('Ctrl Pts',(1.28853121599994,15.2,-10.767417049));
#155869=CARTESIAN_POINT('Ctrl Pts',(1.28853121599994,11.6,-10.767417049));
#155870=CARTESIAN_POINT('Ctrl Pts',(1.28904418099994,15.2,-10.764715709));
#155871=CARTESIAN_POINT('Ctrl Pts',(1.28904418099994,11.6,-10.764715709));
#155872=CARTESIAN_POINT('Ctrl Pts',(1.28955380499994,15.2,-10.762019607));
#155873=CARTESIAN_POINT('Ctrl Pts',(1.28955380499994,11.6,-10.762019607));
#155874=CARTESIAN_POINT('Ctrl Pts',(1.29006009599994,15.2,-10.759328754));
#155875=CARTESIAN_POINT('Ctrl Pts',(1.29006009599994,11.6,-10.759328754));
#155876=CARTESIAN_POINT('Ctrl Pts',(1.29056305799994,15.2,-10.756643162));
#155877=CARTESIAN_POINT('Ctrl Pts',(1.29056305799994,11.6,-10.756643162));
#155878=CARTESIAN_POINT('Ctrl Pts',(1.29106269899994,15.2,-10.753962844));
#155879=CARTESIAN_POINT('Ctrl Pts',(1.29106269899994,11.6,-10.753962844));
#155880=CARTESIAN_POINT('Ctrl Pts',(1.29155902499994,15.2,-10.751287813));
#155881=CARTESIAN_POINT('Ctrl Pts',(1.29155902499994,11.6,-10.751287813));
#155882=CARTESIAN_POINT('Ctrl Pts',(1.29205204299994,15.2,-10.748618079));
#155883=CARTESIAN_POINT('Ctrl Pts',(1.29205204299994,11.6,-10.748618079));
#155884=CARTESIAN_POINT('Ctrl Pts',(1.29254175999994,15.2,-10.745953656));
#155885=CARTESIAN_POINT('Ctrl Pts',(1.29254175999994,11.6,-10.745953656));
#155886=CARTESIAN_POINT('Ctrl Pts',(1.29302817899994,15.2,-10.743294554));
#155887=CARTESIAN_POINT('Ctrl Pts',(1.29302817899994,11.6,-10.743294554));
#155888=CARTESIAN_POINT('Ctrl Pts',(1.29351130999994,15.2,-10.740640788));
#155889=CARTESIAN_POINT('Ctrl Pts',(1.29351130999994,11.6,-10.740640788));
#155890=CARTESIAN_POINT('Ctrl Pts',(1.29399115799994,15.2,-10.737992369));
#155891=CARTESIAN_POINT('Ctrl Pts',(1.29399115799994,11.6,-10.737992369));
#155892=CARTESIAN_POINT('Ctrl Pts',(1.29446772899994,15.2,-10.73534931));
#155893=CARTESIAN_POINT('Ctrl Pts',(1.29446772899994,11.6,-10.73534931));
#155894=CARTESIAN_POINT('Ctrl Pts',(1.29494102999994,15.2,-10.732711622));
#155895=CARTESIAN_POINT('Ctrl Pts',(1.29494102999994,11.6,-10.732711622));
#155896=CARTESIAN_POINT('Ctrl Pts',(1.29541106899994,15.2,-10.730079319));
#155897=CARTESIAN_POINT('Ctrl Pts',(1.29541106899994,11.6,-10.730079319));
#155898=CARTESIAN_POINT('Ctrl Pts',(1.29587784999994,15.2,-10.727452411));
#155899=CARTESIAN_POINT('Ctrl Pts',(1.29587784999994,11.6,-10.727452411));
#155900=CARTESIAN_POINT('Ctrl Pts',(1.29634138199994,15.2,-10.724830913));
#155901=CARTESIAN_POINT('Ctrl Pts',(1.29634138199994,11.6,-10.724830913));
#155902=CARTESIAN_POINT('Ctrl Pts',(1.29680167099994,15.2,-10.722214836));
#155903=CARTESIAN_POINT('Ctrl Pts',(1.29680167099994,11.6,-10.722214836));
#155904=CARTESIAN_POINT('Ctrl Pts',(1.29725872199994,15.2,-10.719604194));
#155905=CARTESIAN_POINT('Ctrl Pts',(1.29725872199994,11.6,-10.719604194));
#155906=CARTESIAN_POINT('Ctrl Pts',(1.29771254399994,15.2,-10.716998997));
#155907=CARTESIAN_POINT('Ctrl Pts',(1.29771254399994,11.6,-10.716998997));
#155908=CARTESIAN_POINT('Ctrl Pts',(1.29816314199994,15.2,-10.714399259));
#155909=CARTESIAN_POINT('Ctrl Pts',(1.29816314199994,11.6,-10.714399259));
#155910=CARTESIAN_POINT('Ctrl Pts',(1.29861052399994,15.2,-10.711804993));
#155911=CARTESIAN_POINT('Ctrl Pts',(1.29861052399994,11.6,-10.711804993));
#155912=CARTESIAN_POINT('Ctrl Pts',(1.29905469599994,15.2,-10.70921621));
#155913=CARTESIAN_POINT('Ctrl Pts',(1.29905469599994,11.6,-10.70921621));
#155914=CARTESIAN_POINT('Ctrl Pts',(1.29949566599994,15.2,-10.706632926));
#155915=CARTESIAN_POINT('Ctrl Pts',(1.29949566599994,11.6,-10.706632926));
#155916=CARTESIAN_POINT('Ctrl Pts',(1.29993343799994,15.2,-10.70405515));
#155917=CARTESIAN_POINT('Ctrl Pts',(1.29993343799994,11.6,-10.70405515));
#155918=CARTESIAN_POINT('Ctrl Pts',(1.30036802199994,15.2,-10.701482895));
#155919=CARTESIAN_POINT('Ctrl Pts',(1.30036802199994,11.6,-10.701482895));
#155920=CARTESIAN_POINT('Ctrl Pts',(1.30079942299994,15.2,-10.698916176));
#155921=CARTESIAN_POINT('Ctrl Pts',(1.30079942299994,11.6,-10.698916176));
#155922=CARTESIAN_POINT('Ctrl Pts',(1.30122764799994,15.2,-10.696355005));
#155923=CARTESIAN_POINT('Ctrl Pts',(1.30122764799994,11.6,-10.696355005));
#155924=CARTESIAN_POINT('Ctrl Pts',(1.30165270499994,15.2,-10.693799393));
#155925=CARTESIAN_POINT('Ctrl Pts',(1.30165270499994,11.6,-10.693799393));
#155926=CARTESIAN_POINT('Ctrl Pts',(1.30207460099994,15.2,-10.691249355));
#155927=CARTESIAN_POINT('Ctrl Pts',(1.30207460099994,11.6,-10.691249355));
#155928=CARTESIAN_POINT('Ctrl Pts',(1.30249334099994,15.2,-10.688704902));
#155929=CARTESIAN_POINT('Ctrl Pts',(1.30249334099994,11.6,-10.688704902));
#155930=CARTESIAN_POINT('Ctrl Pts',(1.30290893499994,15.2,-10.686166048));
#155931=CARTESIAN_POINT('Ctrl Pts',(1.30290893499994,11.6,-10.686166048));
#155932=CARTESIAN_POINT('Ctrl Pts',(1.30332138799994,15.2,-10.683632806));
#155933=CARTESIAN_POINT('Ctrl Pts',(1.30332138799994,11.6,-10.683632806));
#155934=CARTESIAN_POINT('Ctrl Pts',(1.30373070599994,15.2,-10.681105188));
#155935=CARTESIAN_POINT('Ctrl Pts',(1.30373070599994,11.6,-10.681105188));
#155936=CARTESIAN_POINT('Ctrl Pts',(1.30413689999994,15.2,-10.678583208));
#155937=CARTESIAN_POINT('Ctrl Pts',(1.30413689999994,11.6,-10.678583208));
#155938=CARTESIAN_POINT('Ctrl Pts',(1.30453997299994,15.2,-10.676066879));
#155939=CARTESIAN_POINT('Ctrl Pts',(1.30453997299994,11.6,-10.676066879));
#155940=CARTESIAN_POINT('Ctrl Pts',(1.30493993399994,15.2,-10.673556212));
#155941=CARTESIAN_POINT('Ctrl Pts',(1.30493993399994,11.6,-10.673556212));
#155942=CARTESIAN_POINT('Ctrl Pts',(1.30533679099994,15.2,-10.671051222));
#155943=CARTESIAN_POINT('Ctrl Pts',(1.30533679099994,11.6,-10.671051222));
#155944=CARTESIAN_POINT('Ctrl Pts',(1.30573054999994,15.2,-10.668551921));
#155945=CARTESIAN_POINT('Ctrl Pts',(1.30573054999994,11.6,-10.668551921));
#155946=CARTESIAN_POINT('Ctrl Pts',(1.30612121799994,15.2,-10.666058323));
#155947=CARTESIAN_POINT('Ctrl Pts',(1.30612121799994,11.6,-10.666058323));
#155948=CARTESIAN_POINT('Ctrl Pts',(1.30650880299994,15.2,-10.663570441));
#155949=CARTESIAN_POINT('Ctrl Pts',(1.30650880299994,11.6,-10.663570441));
#155950=CARTESIAN_POINT('Ctrl Pts',(1.30689331299994,15.2,-10.661088288));
#155951=CARTESIAN_POINT('Ctrl Pts',(1.30689331299994,11.6,-10.661088288));
#155952=CARTESIAN_POINT('Ctrl Pts',(1.30727475299994,15.2,-10.658611877));
#155953=CARTESIAN_POINT('Ctrl Pts',(1.30727475299994,11.6,-10.658611877));
#155954=CARTESIAN_POINT('Ctrl Pts',(1.30765313299994,15.2,-10.65614122));
#155955=CARTESIAN_POINT('Ctrl Pts',(1.30765313299994,11.6,-10.65614122));
#155956=CARTESIAN_POINT('Ctrl Pts',(1.30802845799994,15.2,-10.653676332));
#155957=CARTESIAN_POINT('Ctrl Pts',(1.30802845799994,11.6,-10.653676332));
#155958=CARTESIAN_POINT('Ctrl Pts',(1.30840073799994,15.2,-10.651217227));
#155959=CARTESIAN_POINT('Ctrl Pts',(1.30840073799994,11.6,-10.651217227));
#155960=CARTESIAN_POINT('Ctrl Pts',(1.30876997899994,15.2,-10.648763916));
#155961=CARTESIAN_POINT('Ctrl Pts',(1.30876997899994,11.6,-10.648763916));
#155962=CARTESIAN_POINT('Ctrl Pts',(1.30913618799994,15.2,-10.646316414));
#155963=CARTESIAN_POINT('Ctrl Pts',(1.30913618799994,11.6,-10.646316414));
#155964=CARTESIAN_POINT('Ctrl Pts',(1.30949937299994,15.2,-10.643874733));
#155965=CARTESIAN_POINT('Ctrl Pts',(1.30949937299994,11.6,-10.643874733));
#155966=CARTESIAN_POINT('Ctrl Pts',(1.30985954199994,15.2,-10.641438888));
#155967=CARTESIAN_POINT('Ctrl Pts',(1.30985954199994,11.6,-10.641438888));
#155968=CARTESIAN_POINT('Ctrl Pts',(1.31021670199994,15.2,-10.639008891));
#155969=CARTESIAN_POINT('Ctrl Pts',(1.31021670199994,11.6,-10.639008891));
#155970=CARTESIAN_POINT('Ctrl Pts',(1.31057086099994,15.2,-10.636584756));
#155971=CARTESIAN_POINT('Ctrl Pts',(1.31057086099994,11.6,-10.636584756));
#155972=CARTESIAN_POINT('Ctrl Pts',(1.31092202599994,15.2,-10.634166498));
#155973=CARTESIAN_POINT('Ctrl Pts',(1.31092202599994,11.6,-10.634166498));
#155974=CARTESIAN_POINT('Ctrl Pts',(1.31127020599994,15.2,-10.631754128));
#155975=CARTESIAN_POINT('Ctrl Pts',(1.31127020599994,11.6,-10.631754128));
#155976=CARTESIAN_POINT('Ctrl Pts',(1.31161540699994,15.2,-10.629347661));
#155977=CARTESIAN_POINT('Ctrl Pts',(1.31161540699994,11.6,-10.629347661));
#155978=CARTESIAN_POINT('Ctrl Pts',(1.31195763899994,15.2,-10.62694711));
#155979=CARTESIAN_POINT('Ctrl Pts',(1.31195763899994,11.6,-10.62694711));
#155980=CARTESIAN_POINT('Ctrl Pts',(1.31229690599994,15.2,-10.62455249));
#155981=CARTESIAN_POINT('Ctrl Pts',(1.31229690599994,11.6,-10.62455249));
#155982=CARTESIAN_POINT('Ctrl Pts',(1.31263321999994,15.2,-10.622163812));
#155983=CARTESIAN_POINT('Ctrl Pts',(1.31263321999994,11.6,-10.622163812));
#155984=CARTESIAN_POINT('Ctrl Pts',(1.31296658599994,15.2,-10.619781092));
#155985=CARTESIAN_POINT('Ctrl Pts',(1.31296658599994,11.6,-10.619781092));
#155986=CARTESIAN_POINT('Ctrl Pts',(1.31329701299994,15.2,-10.617404343));
#155987=CARTESIAN_POINT('Ctrl Pts',(1.31329701299994,11.6,-10.617404343));
#155988=CARTESIAN_POINT('Ctrl Pts',(1.31362450899994,15.2,-10.615033578));
#155989=CARTESIAN_POINT('Ctrl Pts',(1.31362450899994,11.6,-10.615033578));
#155990=CARTESIAN_POINT('Ctrl Pts',(1.31394908099994,15.2,-10.612668813));
#155991=CARTESIAN_POINT('Ctrl Pts',(1.31394908099994,11.6,-10.612668813));
#155992=CARTESIAN_POINT('Ctrl Pts',(1.31427073799994,15.2,-10.61031006));
#155993=CARTESIAN_POINT('Ctrl Pts',(1.31427073799994,11.6,-10.61031006));
#155994=CARTESIAN_POINT('Ctrl Pts',(1.31458948699994,15.2,-10.607957333));
#155995=CARTESIAN_POINT('Ctrl Pts',(1.31458948699994,11.6,-10.607957333));
#155996=CARTESIAN_POINT('Ctrl Pts',(1.31490533699994,15.2,-10.605610646));
#155997=CARTESIAN_POINT('Ctrl Pts',(1.31490533699994,11.6,-10.605610646));
#155998=CARTESIAN_POINT('Ctrl Pts',(1.31521829599994,15.2,-10.603270013));
#155999=CARTESIAN_POINT('Ctrl Pts',(1.31521829599994,11.6,-10.603270013));
#156000=CARTESIAN_POINT('Ctrl Pts',(1.31552837099994,15.2,-10.600935449));
#156001=CARTESIAN_POINT('Ctrl Pts',(1.31552837099994,11.6,-10.600935449));
#156002=CARTESIAN_POINT('Ctrl Pts',(1.31583557099994,15.2,-10.598606966));
#156003=CARTESIAN_POINT('Ctrl Pts',(1.31583557099994,11.6,-10.598606966));
#156004=CARTESIAN_POINT('Ctrl Pts',(1.31613990399994,15.2,-10.59628458));
#156005=CARTESIAN_POINT('Ctrl Pts',(1.31613990399994,11.6,-10.59628458));
#156006=CARTESIAN_POINT('Ctrl Pts',(1.31644137799994,15.2,-10.593968305));
#156007=CARTESIAN_POINT('Ctrl Pts',(1.31644137799994,11.6,-10.593968305));
#156008=CARTESIAN_POINT('Ctrl Pts',(1.31674000099994,15.2,-10.591658153));
#156009=CARTESIAN_POINT('Ctrl Pts',(1.31674000099994,11.6,-10.591658153));
#156010=CARTESIAN_POINT('Ctrl Pts',(1.31703578199994,15.2,-10.58935414));
#156011=CARTESIAN_POINT('Ctrl Pts',(1.31703578199994,11.6,-10.58935414));
#156012=CARTESIAN_POINT('Ctrl Pts',(1.31732872999994,15.2,-10.58705628));
#156013=CARTESIAN_POINT('Ctrl Pts',(1.31732872999994,11.6,-10.58705628));
#156014=CARTESIAN_POINT('Ctrl Pts',(1.31761885099994,15.2,-10.584764587));
#156015=CARTESIAN_POINT('Ctrl Pts',(1.31761885099994,11.6,-10.584764587));
#156016=CARTESIAN_POINT('Ctrl Pts',(1.31790615399994,15.2,-10.582479074));
#156017=CARTESIAN_POINT('Ctrl Pts',(1.31790615399994,11.6,-10.582479074));
#156018=CARTESIAN_POINT('Ctrl Pts',(1.31819064899994,15.2,-10.580199758));
#156019=CARTESIAN_POINT('Ctrl Pts',(1.31819064899994,11.6,-10.580199758));
#156020=CARTESIAN_POINT('Ctrl Pts',(1.31847234299994,15.2,-10.577926652));
#156021=CARTESIAN_POINT('Ctrl Pts',(1.31847234299994,11.6,-10.577926652));
#156022=CARTESIAN_POINT('Ctrl Pts',(1.31875124399994,15.2,-10.575659769));
#156023=CARTESIAN_POINT('Ctrl Pts',(1.31875124399994,11.6,-10.575659769));
#156024=CARTESIAN_POINT('Ctrl Pts',(1.31902736199994,15.2,-10.573399125));
#156025=CARTESIAN_POINT('Ctrl Pts',(1.31902736199994,11.6,-10.573399125));
#156026=CARTESIAN_POINT('Ctrl Pts',(1.31930070599994,15.2,-10.571144734));
#156027=CARTESIAN_POINT('Ctrl Pts',(1.31930070599994,11.6,-10.571144734));
#156028=CARTESIAN_POINT('Ctrl Pts',(1.31957128199994,15.2,-10.56889661));
#156029=CARTESIAN_POINT('Ctrl Pts',(1.31957128199994,11.6,-10.56889661));
#156030=CARTESIAN_POINT('Ctrl Pts',(1.31983910099994,15.2,-10.566654769));
#156031=CARTESIAN_POINT('Ctrl Pts',(1.31983910099994,11.6,-10.566654769));
#156032=CARTESIAN_POINT('Ctrl Pts',(1.32010416999994,15.2,-10.564419224));
#156033=CARTESIAN_POINT('Ctrl Pts',(1.32010416999994,11.6,-10.564419224));
#156034=CARTESIAN_POINT('Ctrl Pts',(1.32036649799994,15.2,-10.562189991));
#156035=CARTESIAN_POINT('Ctrl Pts',(1.32036649799994,11.6,-10.562189991));
#156036=CARTESIAN_POINT('Ctrl Pts',(1.32062609499994,15.2,-10.559967084));
#156037=CARTESIAN_POINT('Ctrl Pts',(1.32062609499994,11.6,-10.559967084));
#156038=CARTESIAN_POINT('Ctrl Pts',(1.32088296799994,15.2,-10.557750517));
#156039=CARTESIAN_POINT('Ctrl Pts',(1.32088296799994,11.6,-10.557750517));
#156040=CARTESIAN_POINT('Ctrl Pts',(1.32113712699994,15.2,-10.555540305));
#156041=CARTESIAN_POINT('Ctrl Pts',(1.32113712699994,11.6,-10.555540305));
#156042=CARTESIAN_POINT('Ctrl Pts',(1.32138857999994,15.2,-10.553336463));
#156043=CARTESIAN_POINT('Ctrl Pts',(1.32138857999994,11.6,-10.553336463));
#156044=CARTESIAN_POINT('Ctrl Pts',(1.32163733599994,15.2,-10.551139007));
#156045=CARTESIAN_POINT('Ctrl Pts',(1.32163733599994,11.6,-10.551139007));
#156046=CARTESIAN_POINT('Ctrl Pts',(1.32188340499994,15.2,-10.548947949));
#156047=CARTESIAN_POINT('Ctrl Pts',(1.32188340499994,11.6,-10.548947949));
#156048=CARTESIAN_POINT('Ctrl Pts',(1.32212679399994,15.2,-10.546763306));
#156049=CARTESIAN_POINT('Ctrl Pts',(1.32212679399994,11.6,-10.546763306));
#156050=CARTESIAN_POINT('Ctrl Pts',(1.32236751399994,15.2,-10.544585093));
#156051=CARTESIAN_POINT('Ctrl Pts',(1.32236751399994,11.6,-10.544585093));
#156052=CARTESIAN_POINT('Ctrl Pts',(1.32260557299994,15.2,-10.542413324));
#156053=CARTESIAN_POINT('Ctrl Pts',(1.32260557299994,11.6,-10.542413324));
#156054=CARTESIAN_POINT('Ctrl Pts',(1.32284097899994,15.2,-10.540248014));
#156055=CARTESIAN_POINT('Ctrl Pts',(1.32284097899994,11.6,-10.540248014));
#156056=CARTESIAN_POINT('Ctrl Pts',(1.32307374299994,15.2,-10.53808918));
#156057=CARTESIAN_POINT('Ctrl Pts',(1.32307374299994,11.6,-10.53808918));
#156058=CARTESIAN_POINT('Ctrl Pts',(1.32330387399994,15.2,-10.535936834));
#156059=CARTESIAN_POINT('Ctrl Pts',(1.32330387399994,11.6,-10.535936834));
#156060=CARTESIAN_POINT('Ctrl Pts',(1.32353137899994,15.2,-10.533790993));
#156061=CARTESIAN_POINT('Ctrl Pts',(1.32353137899994,11.6,-10.533790993));
#156062=CARTESIAN_POINT('Ctrl Pts',(1.32375626899994,15.2,-10.531651672));
#156063=CARTESIAN_POINT('Ctrl Pts',(1.32375626899994,11.6,-10.531651672));
#156064=CARTESIAN_POINT('Ctrl Pts',(1.32397855299994,15.2,-10.529518885));
#156065=CARTESIAN_POINT('Ctrl Pts',(1.32397855299994,11.6,-10.529518885));
#156066=CARTESIAN_POINT('Ctrl Pts',(1.32419823999994,15.2,-10.52739265));
#156067=CARTESIAN_POINT('Ctrl Pts',(1.32419823999994,11.6,-10.52739265));
#156068=CARTESIAN_POINT('Ctrl Pts',(1.32441533999994,15.2,-10.52527298));
#156069=CARTESIAN_POINT('Ctrl Pts',(1.32441533999994,11.6,-10.52527298));
#156070=CARTESIAN_POINT('Ctrl Pts',(1.32462986099994,15.2,-10.523159891));
#156071=CARTESIAN_POINT('Ctrl Pts',(1.32462986099994,11.6,-10.523159891));
#156072=CARTESIAN_POINT('Ctrl Pts',(1.32484181499994,15.2,-10.521053397));
#156073=CARTESIAN_POINT('Ctrl Pts',(1.32484181499994,11.6,-10.521053397));
#156074=CARTESIAN_POINT('Ctrl Pts',(1.32505120699994,15.2,-10.518953515));
#156075=CARTESIAN_POINT('Ctrl Pts',(1.32505120699994,11.6,-10.518953515));
#156076=CARTESIAN_POINT('Ctrl Pts',(1.32525805199994,15.2,-10.516860261));
#156077=CARTESIAN_POINT('Ctrl Pts',(1.32525805199994,11.6,-10.516860261));
#156078=CARTESIAN_POINT('Ctrl Pts',(1.32546235399994,15.2,-10.514773649));
#156079=CARTESIAN_POINT('Ctrl Pts',(1.32546235399994,11.6,-10.514773649));
#156080=CARTESIAN_POINT('Ctrl Pts',(1.32566412699994,15.2,-10.512693695));
#156081=CARTESIAN_POINT('Ctrl Pts',(1.32566412699994,11.6,-10.512693695));
#156082=CARTESIAN_POINT('Ctrl Pts',(1.32586337699994,15.2,-10.510620415));
#156083=CARTESIAN_POINT('Ctrl Pts',(1.32586337699994,11.6,-10.510620415));
#156084=CARTESIAN_POINT('Ctrl Pts',(1.32606011699994,15.2,-10.508553825));
#156085=CARTESIAN_POINT('Ctrl Pts',(1.32606011699994,11.6,-10.508553825));
#156086=CARTESIAN_POINT('Ctrl Pts',(1.32625435399994,15.2,-10.506493939));
#156087=CARTESIAN_POINT('Ctrl Pts',(1.32625435399994,11.6,-10.506493939));
#156088=CARTESIAN_POINT('Ctrl Pts',(1.32644609999994,15.2,-10.504440774));
#156089=CARTESIAN_POINT('Ctrl Pts',(1.32644609999994,11.6,-10.504440774));
#156090=CARTESIAN_POINT('Ctrl Pts',(1.32663536199994,15.2,-10.502394346));
#156091=CARTESIAN_POINT('Ctrl Pts',(1.32663536199994,11.6,-10.502394346));
#156092=CARTESIAN_POINT('Ctrl Pts',(1.32682215299994,15.2,-10.500354671));
#156093=CARTESIAN_POINT('Ctrl Pts',(1.32682215299994,11.6,-10.500354671));
#156094=CARTESIAN_POINT('Ctrl Pts',(1.32700648099994,15.2,-10.498321763));
#156095=CARTESIAN_POINT('Ctrl Pts',(1.32700648099994,11.6,-10.498321763));
#156096=CARTESIAN_POINT('Ctrl Pts',(1.32718835599994,15.2,-10.49629564));
#156097=CARTESIAN_POINT('Ctrl Pts',(1.32718835599994,11.6,-10.49629564));
#156098=CARTESIAN_POINT('Ctrl Pts',(1.32736778799994,15.2,-10.494276317));
#156099=CARTESIAN_POINT('Ctrl Pts',(1.32736778799994,11.6,-10.494276317));
#156100=CARTESIAN_POINT('Ctrl Pts',(1.32754478699994,15.2,-10.49226381));
#156101=CARTESIAN_POINT('Ctrl Pts',(1.32754478699994,11.6,-10.49226381));
#156102=CARTESIAN_POINT('Ctrl Pts',(1.32771936299994,15.2,-10.490258135));
#156103=CARTESIAN_POINT('Ctrl Pts',(1.32771936299994,11.6,-10.490258135));
#156104=CARTESIAN_POINT('Ctrl Pts',(1.32789152599994,15.2,-10.488259308));
#156105=CARTESIAN_POINT('Ctrl Pts',(1.32789152599994,11.6,-10.488259308));
#156106=CARTESIAN_POINT('Ctrl Pts',(1.32806128599994,15.2,-10.486267346));
#156107=CARTESIAN_POINT('Ctrl Pts',(1.32806128599994,11.6,-10.486267346));
#156108=CARTESIAN_POINT('Ctrl Pts',(1.32822865399994,15.2,-10.484282264));
#156109=CARTESIAN_POINT('Ctrl Pts',(1.32822865399994,11.6,-10.484282264));
#156110=CARTESIAN_POINT('Ctrl Pts',(1.32839363899994,15.2,-10.48230408));
#156111=CARTESIAN_POINT('Ctrl Pts',(1.32839363899994,11.6,-10.48230408));
#156112=CARTESIAN_POINT('Ctrl Pts',(1.32855625199994,15.2,-10.480332808));
#156113=CARTESIAN_POINT('Ctrl Pts',(1.32855625199994,11.6,-10.480332808));
#156114=CARTESIAN_POINT('Ctrl Pts',(1.32871650299994,15.2,-10.478368465));
#156115=CARTESIAN_POINT('Ctrl Pts',(1.32871650299994,11.6,-10.478368465));
#156116=CARTESIAN_POINT('Ctrl Pts',(1.32887440299994,15.2,-10.476411069));
#156117=CARTESIAN_POINT('Ctrl Pts',(1.32887440299994,11.6,-10.476411069));
#156118=CARTESIAN_POINT('Ctrl Pts',(1.32902996199994,15.2,-10.474460635));
#156119=CARTESIAN_POINT('Ctrl Pts',(1.32902996199994,11.6,-10.474460635));
#156120=CARTESIAN_POINT('Ctrl Pts',(1.32918318899994,15.2,-10.47251718));
#156121=CARTESIAN_POINT('Ctrl Pts',(1.32918318899994,11.6,-10.47251718));
#156122=CARTESIAN_POINT('Ctrl Pts',(1.32933409699994,15.2,-10.47058072));
#156123=CARTESIAN_POINT('Ctrl Pts',(1.32933409699994,11.6,-10.47058072));
#156124=CARTESIAN_POINT('Ctrl Pts',(1.32948269399994,15.2,-10.468651272));
#156125=CARTESIAN_POINT('Ctrl Pts',(1.32948269399994,11.6,-10.468651272));
#156126=CARTESIAN_POINT('Ctrl Pts',(1.32962899299994,15.2,-10.466728852));
#156127=CARTESIAN_POINT('Ctrl Pts',(1.32962899299994,11.6,-10.466728852));
#156128=CARTESIAN_POINT('Ctrl Pts',(1.32977300299994,15.2,-10.464813477));
#156129=CARTESIAN_POINT('Ctrl Pts',(1.32977300299994,11.6,-10.464813477));
#156130=CARTESIAN_POINT('Ctrl Pts',(1.32991473499994,15.2,-10.462905165));
#156131=CARTESIAN_POINT('Ctrl Pts',(1.32991473499994,11.6,-10.462905165));
#156132=CARTESIAN_POINT('Ctrl Pts',(1.33005419999994,15.2,-10.461003932));
#156133=CARTESIAN_POINT('Ctrl Pts',(1.33005419999994,11.6,-10.461003932));
#156134=CARTESIAN_POINT('Ctrl Pts',(1.33019140799994,15.2,-10.459109793));
#156135=CARTESIAN_POINT('Ctrl Pts',(1.33019140799994,11.6,-10.459109793));
#156136=CARTESIAN_POINT('Ctrl Pts',(1.33032637099994,15.2,-10.457222766));
#156137=CARTESIAN_POINT('Ctrl Pts',(1.33032637099994,11.6,-10.457222766));
#156138=CARTESIAN_POINT('Ctrl Pts',(1.33045909799994,15.2,-10.45534287));
#156139=CARTESIAN_POINT('Ctrl Pts',(1.33045909799994,11.6,-10.45534287));
#156140=CARTESIAN_POINT('Ctrl Pts',(1.33058960299994,15.2,-10.453470121));
#156141=CARTESIAN_POINT('Ctrl Pts',(1.33058960299994,11.6,-10.453470121));
#156142=CARTESIAN_POINT('Ctrl Pts',(1.33071789299994,15.2,-10.451604534));
#156143=CARTESIAN_POINT('Ctrl Pts',(1.33071789299994,11.6,-10.451604534));
#156144=CARTESIAN_POINT('Ctrl Pts',(1.33084398199994,15.2,-10.449746128));
#156145=CARTESIAN_POINT('Ctrl Pts',(1.33084398199994,11.6,-10.449746128));
#156146=CARTESIAN_POINT('Ctrl Pts',(1.33096787999994,15.2,-10.447894919));
#156147=CARTESIAN_POINT('Ctrl Pts',(1.33096787999994,11.6,-10.447894919));
#156148=CARTESIAN_POINT('Ctrl Pts',(1.33108959799994,15.2,-10.446050926));
#156149=CARTESIAN_POINT('Ctrl Pts',(1.33108959799994,11.6,-10.446050926));
#156150=CARTESIAN_POINT('Ctrl Pts',(1.33120914699994,15.2,-10.444214164));
#156151=CARTESIAN_POINT('Ctrl Pts',(1.33120914699994,11.6,-10.444214164));
#156152=CARTESIAN_POINT('Ctrl Pts',(1.33132653899994,15.2,-10.442384652));
#156153=CARTESIAN_POINT('Ctrl Pts',(1.33132653899994,11.6,-10.442384652));
#156154=CARTESIAN_POINT('Ctrl Pts',(1.33144178299994,15.2,-10.440562407));
#156155=CARTESIAN_POINT('Ctrl Pts',(1.33144178299994,11.6,-10.440562407));
#156156=CARTESIAN_POINT('Ctrl Pts',(1.33155489399994,15.2,-10.438747447));
#156157=CARTESIAN_POINT('Ctrl Pts',(1.33155489399994,11.6,-10.438747447));
#156158=CARTESIAN_POINT('Ctrl Pts',(1.33166587999994,15.2,-10.436939788));
#156159=CARTESIAN_POINT('Ctrl Pts',(1.33166587999994,11.6,-10.436939788));
#156160=CARTESIAN_POINT('Ctrl Pts',(1.33177475499994,15.2,-10.435139448));
#156161=CARTESIAN_POINT('Ctrl Pts',(1.33177475499994,11.6,-10.435139448));
#156162=CARTESIAN_POINT('Ctrl Pts',(1.33188152799994,15.2,-10.433346446));
#156163=CARTESIAN_POINT('Ctrl Pts',(1.33188152799994,11.6,-10.433346446));
#156164=CARTESIAN_POINT('Ctrl Pts',(1.33198621199994,15.2,-10.431560797));
#156165=CARTESIAN_POINT('Ctrl Pts',(1.33198621199994,11.6,-10.431560797));
#156166=CARTESIAN_POINT('Ctrl Pts',(1.33208881899994,15.2,-10.429782521));
#156167=CARTESIAN_POINT('Ctrl Pts',(1.33208881899994,11.6,-10.429782521));
#156168=CARTESIAN_POINT('Ctrl Pts',(1.33218935899994,15.2,-10.428011636));
#156169=CARTESIAN_POINT('Ctrl Pts',(1.33218935899994,11.6,-10.428011636));
#156170=CARTESIAN_POINT('Ctrl Pts',(1.33228784499994,15.2,-10.426248158));
#156171=CARTESIAN_POINT('Ctrl Pts',(1.33228784499994,11.6,-10.426248158));
#156172=CARTESIAN_POINT('Ctrl Pts',(1.33238428799994,15.2,-10.424492106));
#156173=CARTESIAN_POINT('Ctrl Pts',(1.33238428799994,11.6,-10.424492106));
#156174=CARTESIAN_POINT('Ctrl Pts',(1.33247869999994,15.2,-10.422743497));
#156175=CARTESIAN_POINT('Ctrl Pts',(1.33247869999994,11.6,-10.422743497));
#156176=CARTESIAN_POINT('Ctrl Pts',(1.33257109199994,15.2,-10.421002351));
#156177=CARTESIAN_POINT('Ctrl Pts',(1.33257109199994,11.6,-10.421002351));
#156178=CARTESIAN_POINT('Ctrl Pts',(1.33266147799994,15.2,-10.419268684));
#156179=CARTESIAN_POINT('Ctrl Pts',(1.33266147799994,11.6,-10.419268684));
#156180=CARTESIAN_POINT('Ctrl Pts',(1.33274986699994,15.2,-10.417542515));
#156181=CARTESIAN_POINT('Ctrl Pts',(1.33274986699994,11.6,-10.417542515));
#156182=CARTESIAN_POINT('Ctrl Pts',(1.33283627399994,15.2,-10.415823863));
#156183=CARTESIAN_POINT('Ctrl Pts',(1.33283627399994,11.6,-10.415823863));
#156184=CARTESIAN_POINT('Ctrl Pts',(1.33292070899994,15.2,-10.414112744));
#156185=CARTESIAN_POINT('Ctrl Pts',(1.33292070899994,11.6,-10.414112744));
#156186=CARTESIAN_POINT('Ctrl Pts',(1.33300318399994,15.2,-10.412409178));
#156187=CARTESIAN_POINT('Ctrl Pts',(1.33300318399994,11.6,-10.412409178));
#156188=CARTESIAN_POINT('Ctrl Pts',(1.33308371299994,15.2,-10.410713184));
#156189=CARTESIAN_POINT('Ctrl Pts',(1.33308371299994,11.6,-10.410713184));
#156190=CARTESIAN_POINT('Ctrl Pts',(1.33316230599994,15.2,-10.409024778));
#156191=CARTESIAN_POINT('Ctrl Pts',(1.33316230599994,11.6,-10.409024778));
#156192=CARTESIAN_POINT('Ctrl Pts',(1.33323897699994,15.2,-10.40734398));
#156193=CARTESIAN_POINT('Ctrl Pts',(1.33323897699994,11.6,-10.40734398));
#156194=CARTESIAN_POINT('Ctrl Pts',(1.33331373699994,15.2,-10.405670811));
#156195=CARTESIAN_POINT('Ctrl Pts',(1.33331373699994,11.6,-10.405670811));
#156196=CARTESIAN_POINT('Ctrl Pts',(1.33338659999994,15.2,-10.404005285));
#156197=CARTESIAN_POINT('Ctrl Pts',(1.33338659999994,11.6,-10.404005285));
#156198=CARTESIAN_POINT('Ctrl Pts',(1.33345757699994,15.2,-10.402347423));
#156199=CARTESIAN_POINT('Ctrl Pts',(1.33345757699994,11.6,-10.402347423));
#156200=CARTESIAN_POINT('Ctrl Pts',(1.33352668099994,15.2,-10.400697244));
#156201=CARTESIAN_POINT('Ctrl Pts',(1.33352668099994,11.6,-10.400697244));
#156202=CARTESIAN_POINT('Ctrl Pts',(1.33359392399994,15.2,-10.399054766));
#156203=CARTESIAN_POINT('Ctrl Pts',(1.33359392399994,11.6,-10.399054766));
#156204=CARTESIAN_POINT('Ctrl Pts',(1.33365931999994,15.2,-10.397420008));
#156205=CARTESIAN_POINT('Ctrl Pts',(1.33365931999994,11.6,-10.397420008));
#156206=CARTESIAN_POINT('Ctrl Pts',(1.33372287999994,15.2,-10.39579299));
#156207=CARTESIAN_POINT('Ctrl Pts',(1.33372287999994,11.6,-10.39579299));
#156208=CARTESIAN_POINT('Ctrl Pts',(1.33378461799994,15.2,-10.39417373));
#156209=CARTESIAN_POINT('Ctrl Pts',(1.33378461799994,11.6,-10.39417373));
#156210=CARTESIAN_POINT('Ctrl Pts',(1.33384454499994,15.2,-10.392562248));
#156211=CARTESIAN_POINT('Ctrl Pts',(1.33384454499994,11.6,-10.392562248));
#156212=CARTESIAN_POINT('Ctrl Pts',(1.33390267699994,15.2,-10.39095856));
#156213=CARTESIAN_POINT('Ctrl Pts',(1.33390267699994,11.6,-10.39095856));
#156214=CARTESIAN_POINT('Ctrl Pts',(1.33395902399994,15.2,-10.38936269));
#156215=CARTESIAN_POINT('Ctrl Pts',(1.33395902399994,11.6,-10.38936269));
#156216=CARTESIAN_POINT('Ctrl Pts',(1.33401359999994,15.2,-10.387774654));
#156217=CARTESIAN_POINT('Ctrl Pts',(1.33401359999994,11.6,-10.387774654));
#156218=CARTESIAN_POINT('Ctrl Pts',(1.33406641799994,15.2,-10.386194473));
#156219=CARTESIAN_POINT('Ctrl Pts',(1.33406641799994,11.6,-10.386194473));
#156220=CARTESIAN_POINT('Ctrl Pts',(1.33411749199994,15.2,-10.384622165));
#156221=CARTESIAN_POINT('Ctrl Pts',(1.33411749199994,11.6,-10.384622165));
#156222=CARTESIAN_POINT('Ctrl Pts',(1.33416683399994,15.2,-10.383057751));
#156223=CARTESIAN_POINT('Ctrl Pts',(1.33416683399994,11.6,-10.383057751));
#156224=CARTESIAN_POINT('Ctrl Pts',(1.33421445699994,15.2,-10.381501249));
#156225=CARTESIAN_POINT('Ctrl Pts',(1.33421445699994,11.6,-10.381501249));
#156226=CARTESIAN_POINT('Ctrl Pts',(1.33426037499994,15.2,-10.379952679));
#156227=CARTESIAN_POINT('Ctrl Pts',(1.33426037499994,11.6,-10.379952679));
#156228=CARTESIAN_POINT('Ctrl Pts',(1.33430460199994,15.2,-10.378412062));
#156229=CARTESIAN_POINT('Ctrl Pts',(1.33430460199994,11.6,-10.378412062));
#156230=CARTESIAN_POINT('Ctrl Pts',(1.33434714999994,15.2,-10.376879417));
#156231=CARTESIAN_POINT('Ctrl Pts',(1.33434714999994,11.6,-10.376879417));
#156232=CARTESIAN_POINT('Ctrl Pts',(1.33438803299994,15.2,-10.375354763));
#156233=CARTESIAN_POINT('Ctrl Pts',(1.33438803299994,11.6,-10.375354763));
#156234=CARTESIAN_POINT('Ctrl Pts',(1.33442726499994,15.2,-10.373838121));
#156235=CARTESIAN_POINT('Ctrl Pts',(1.33442726499994,11.6,-10.373838121));
#156236=CARTESIAN_POINT('Ctrl Pts',(1.33446485899994,15.2,-10.37232951));
#156237=CARTESIAN_POINT('Ctrl Pts',(1.33446485899994,11.6,-10.37232951));
#156238=CARTESIAN_POINT('Ctrl Pts',(1.33450082899994,15.2,-10.370828951));
#156239=CARTESIAN_POINT('Ctrl Pts',(1.33450082899994,11.6,-10.370828951));
#156240=CARTESIAN_POINT('Ctrl Pts',(1.33453518799994,15.2,-10.369336464));
#156241=CARTESIAN_POINT('Ctrl Pts',(1.33453518799994,11.6,-10.369336464));
#156242=CARTESIAN_POINT('Ctrl Pts',(1.33456795099994,15.2,-10.367852069));
#156243=CARTESIAN_POINT('Ctrl Pts',(1.33456795099994,11.6,-10.367852069));
#156244=CARTESIAN_POINT('Ctrl Pts',(1.33459913199994,15.2,-10.366375787));
#156245=CARTESIAN_POINT('Ctrl Pts',(1.33459913199994,11.6,-10.366375787));
#156246=CARTESIAN_POINT('Ctrl Pts',(1.33462874399994,15.2,-10.364907637));
#156247=CARTESIAN_POINT('Ctrl Pts',(1.33462874399994,11.6,-10.364907637));
#156248=CARTESIAN_POINT('Ctrl Pts',(1.33465680099994,15.2,-10.363447639));
#156249=CARTESIAN_POINT('Ctrl Pts',(1.33465680099994,11.6,-10.363447639));
#156250=CARTESIAN_POINT('Ctrl Pts',(1.33468331799994,15.2,-10.361995816));
#156251=CARTESIAN_POINT('Ctrl Pts',(1.33468331799994,11.6,-10.361995816));
#156252=CARTESIAN_POINT('Ctrl Pts',(1.33470830799994,15.2,-10.360552186));
#156253=CARTESIAN_POINT('Ctrl Pts',(1.33470830799994,11.6,-10.360552186));
#156254=CARTESIAN_POINT('Ctrl Pts',(1.33473178599994,15.2,-10.359116771));
#156255=CARTESIAN_POINT('Ctrl Pts',(1.33473178599994,11.6,-10.359116771));
#156256=CARTESIAN_POINT('Ctrl Pts',(1.33475376599994,15.2,-10.357689593));
#156257=CARTESIAN_POINT('Ctrl Pts',(1.33475376599994,11.6,-10.357689593));
#156258=CARTESIAN_POINT('Ctrl Pts',(1.33477426199994,15.2,-10.356270671));
#156259=CARTESIAN_POINT('Ctrl Pts',(1.33477426199994,11.6,-10.356270671));
#156260=CARTESIAN_POINT('Ctrl Pts',(1.33479328899994,15.2,-10.354860026));
#156261=CARTESIAN_POINT('Ctrl Pts',(1.33479328899994,11.6,-10.354860026));
#156262=CARTESIAN_POINT('Ctrl Pts',(1.33481086199994,15.2,-10.353457679));
#156263=CARTESIAN_POINT('Ctrl Pts',(1.33481086199994,11.6,-10.353457679));
#156264=CARTESIAN_POINT('Ctrl Pts',(1.33482699499994,15.2,-10.352063652));
#156265=CARTESIAN_POINT('Ctrl Pts',(1.33482699499994,11.6,-10.352063652));
#156266=CARTESIAN_POINT('Ctrl Pts',(1.33484170199994,15.2,-10.350677965));
#156267=CARTESIAN_POINT('Ctrl Pts',(1.33484170199994,11.6,-10.350677965));
#156268=CARTESIAN_POINT('Ctrl Pts',(1.33485499899994,15.2,-10.34930064));
#156269=CARTESIAN_POINT('Ctrl Pts',(1.33485499899994,11.6,-10.34930064));
#156270=CARTESIAN_POINT('Ctrl Pts',(1.33486689899994,15.2,-10.347931697));
#156271=CARTESIAN_POINT('Ctrl Pts',(1.33486689899994,11.6,-10.347931697));
#156272=CARTESIAN_POINT('Ctrl Pts',(1.33487741999994,15.2,-10.34657116));
#156273=CARTESIAN_POINT('Ctrl Pts',(1.33487741999994,11.6,-10.34657116));
#156274=CARTESIAN_POINT('Ctrl Pts',(1.33488657299994,15.2,-10.345219049));
#156275=CARTESIAN_POINT('Ctrl Pts',(1.33488657299994,11.6,-10.345219049));
#156276=CARTESIAN_POINT('Ctrl Pts',(1.33489437599994,15.2,-10.343875384));
#156277=CARTESIAN_POINT('Ctrl Pts',(1.33489437599994,11.6,-10.343875384));
#156278=CARTESIAN_POINT('Ctrl Pts',(1.33490084299994,15.2,-10.342540189));
#156279=CARTESIAN_POINT('Ctrl Pts',(1.33490084299994,11.6,-10.342540189));
#156280=CARTESIAN_POINT('Ctrl Pts',(1.33490598899994,15.2,-10.341213485));
#156281=CARTESIAN_POINT('Ctrl Pts',(1.33490598899994,11.6,-10.341213485));
#156282=CARTESIAN_POINT('Ctrl Pts',(1.33490982999994,15.2,-10.339895294));
#156283=CARTESIAN_POINT('Ctrl Pts',(1.33490982999994,11.6,-10.339895294));
#156284=CARTESIAN_POINT('Ctrl Pts',(1.33491238099994,15.2,-10.338585637));
#156285=CARTESIAN_POINT('Ctrl Pts',(1.33491238099994,11.6,-10.338585637));
#156286=CARTESIAN_POINT('Ctrl Pts',(1.33491365599994,15.2,-10.337284537));
#156287=CARTESIAN_POINT('Ctrl Pts',(1.33491365599994,11.6,-10.337284537));
#156288=CARTESIAN_POINT('Ctrl Pts',(1.33491367299994,15.2,-10.335992016));
#156289=CARTESIAN_POINT('Ctrl Pts',(1.33491367299994,11.6,-10.335992016));
#156290=CARTESIAN_POINT('Ctrl Pts',(1.33491244599994,15.2,-10.334708096));
#156291=CARTESIAN_POINT('Ctrl Pts',(1.33491244599994,11.6,-10.334708096));
#156292=CARTESIAN_POINT('Ctrl Pts',(1.33490999099994,15.2,-10.333432799));
#156293=CARTESIAN_POINT('Ctrl Pts',(1.33490999099994,11.6,-10.333432799));
#156294=CARTESIAN_POINT('Ctrl Pts',(1.33490632299994,15.2,-10.332166147));
#156295=CARTESIAN_POINT('Ctrl Pts',(1.33490632299994,11.6,-10.332166147));
#156296=CARTESIAN_POINT('Ctrl Pts',(1.33490145899994,15.2,-10.330908163));
#156297=CARTESIAN_POINT('Ctrl Pts',(1.33490145899994,11.6,-10.330908163));
#156298=CARTESIAN_POINT('Ctrl Pts',(1.33489541499994,15.2,-10.32965887));
#156299=CARTESIAN_POINT('Ctrl Pts',(1.33489541499994,11.6,-10.32965887));
#156300=CARTESIAN_POINT('Ctrl Pts',(1.33488820599994,15.2,-10.32841829));
#156301=CARTESIAN_POINT('Ctrl Pts',(1.33488820599994,11.6,-10.32841829));
#156302=CARTESIAN_POINT('Ctrl Pts',(1.33487984899994,15.2,-10.327186447));
#156303=CARTESIAN_POINT('Ctrl Pts',(1.33487984899994,11.6,-10.327186447));
#156304=CARTESIAN_POINT('Ctrl Pts',(1.33487035799994,15.2,-10.32596336));
#156305=CARTESIAN_POINT('Ctrl Pts',(1.33487035799994,11.6,-10.32596336));
#156306=CARTESIAN_POINT('Ctrl Pts',(1.33485975199994,15.2,-10.324749056));
#156307=CARTESIAN_POINT('Ctrl Pts',(1.33485975199994,11.6,-10.324749056));
#156308=CARTESIAN_POINT('Ctrl Pts',(1.33484804599994,15.2,-10.323543558));
#156309=CARTESIAN_POINT('Ctrl Pts',(1.33484804599994,11.6,-10.323543558));
#156310=CARTESIAN_POINT('Ctrl Pts',(1.33483525599994,15.2,-10.322346886));
#156311=CARTESIAN_POINT('Ctrl Pts',(1.33483525599994,11.6,-10.322346886));
#156312=CARTESIAN_POINT('Ctrl Pts',(1.33482139999994,15.2,-10.321159066));
#156313=CARTESIAN_POINT('Ctrl Pts',(1.33482139999994,11.6,-10.321159066));
#156314=CARTESIAN_POINT('Ctrl Pts',(1.33480649299994,15.2,-10.319980119));
#156315=CARTESIAN_POINT('Ctrl Pts',(1.33480649299994,11.6,-10.319980119));
#156316=CARTESIAN_POINT('Ctrl Pts',(1.33479055199994,15.2,-10.318810071));
#156317=CARTESIAN_POINT('Ctrl Pts',(1.33479055199994,11.6,-10.318810071));
#156318=CARTESIAN_POINT('Ctrl Pts',(1.33477359399994,15.2,-10.317648943));
#156319=CARTESIAN_POINT('Ctrl Pts',(1.33477359399994,11.6,-10.317648943));
#156320=CARTESIAN_POINT('Ctrl Pts',(1.33475563599994,15.2,-10.31649676));
#156321=CARTESIAN_POINT('Ctrl Pts',(1.33475563599994,11.6,-10.31649676));
#156322=CARTESIAN_POINT('Ctrl Pts',(1.33473669499994,15.2,-10.315353546));
#156323=CARTESIAN_POINT('Ctrl Pts',(1.33473669499994,11.6,-10.315353546));
#156324=CARTESIAN_POINT('Ctrl Pts',(1.33471678699994,15.2,-10.314219324));
#156325=CARTESIAN_POINT('Ctrl Pts',(1.33471678699994,11.6,-10.314219324));
#156326=CARTESIAN_POINT('Ctrl Pts',(1.33469592999994,15.2,-10.313094118));
#156327=CARTESIAN_POINT('Ctrl Pts',(1.33469592999994,11.6,-10.313094118));
#156328=CARTESIAN_POINT('Ctrl Pts',(1.33467414199994,15.2,-10.311977952));
#156329=CARTESIAN_POINT('Ctrl Pts',(1.33467414199994,11.6,-10.311977952));
#156330=CARTESIAN_POINT('Ctrl Pts',(1.33465143899994,15.2,-10.310870851));
#156331=CARTESIAN_POINT('Ctrl Pts',(1.33465143899994,11.6,-10.310870851));
#156332=CARTESIAN_POINT('Ctrl Pts',(1.33462783799994,15.2,-10.309772837));
#156333=CARTESIAN_POINT('Ctrl Pts',(1.33462783799994,11.6,-10.309772837));
#156334=CARTESIAN_POINT('Ctrl Pts',(1.33460335699994,15.2,-10.308683938));
#156335=CARTESIAN_POINT('Ctrl Pts',(1.33460335699994,11.6,-10.308683938));
#156336=CARTESIAN_POINT('Ctrl Pts',(1.33457801399994,15.2,-10.307604175));
#156337=CARTESIAN_POINT('Ctrl Pts',(1.33457801399994,11.6,-10.307604175));
#156338=CARTESIAN_POINT('Ctrl Pts',(1.33455182599994,15.2,-10.306533574));
#156339=CARTESIAN_POINT('Ctrl Pts',(1.33455182599994,11.6,-10.306533574));
#156340=CARTESIAN_POINT('Ctrl Pts',(1.33452481199994,15.2,-10.30547216));
#156341=CARTESIAN_POINT('Ctrl Pts',(1.33452481199994,11.6,-10.30547216));
#156342=CARTESIAN_POINT('Ctrl Pts',(1.33449698899994,15.2,-10.304419957));
#156343=CARTESIAN_POINT('Ctrl Pts',(1.33449698899994,11.6,-10.304419957));
#156344=CARTESIAN_POINT('Ctrl Pts',(1.33446837399994,15.2,-10.30337699));
#156345=CARTESIAN_POINT('Ctrl Pts',(1.33446837399994,11.6,-10.30337699));
#156346=CARTESIAN_POINT('Ctrl Pts',(1.33443898699994,15.2,-10.302343284));
#156347=CARTESIAN_POINT('Ctrl Pts',(1.33443898699994,11.6,-10.302343284));
#156348=CARTESIAN_POINT('Ctrl Pts',(1.33440884499994,15.2,-10.301318864));
#156349=CARTESIAN_POINT('Ctrl Pts',(1.33440884499994,11.6,-10.301318864));
#156350=CARTESIAN_POINT('Ctrl Pts',(1.33437796499994,15.2,-10.300303756));
#156351=CARTESIAN_POINT('Ctrl Pts',(1.33437796499994,11.6,-10.300303756));
#156352=CARTESIAN_POINT('Ctrl Pts',(1.33434636799994,15.2,-10.299297985));
#156353=CARTESIAN_POINT('Ctrl Pts',(1.33434636799994,11.6,-10.299297985));
#156354=CARTESIAN_POINT('Ctrl Pts',(1.33431407099994,15.2,-10.298301576));
#156355=CARTESIAN_POINT('Ctrl Pts',(1.33431407099994,11.6,-10.298301576));
#156356=CARTESIAN_POINT('Ctrl Pts',(1.33428109299994,15.2,-10.297314555));
#156357=CARTESIAN_POINT('Ctrl Pts',(1.33428109299994,11.6,-10.297314555));
#156358=CARTESIAN_POINT('Ctrl Pts',(1.33424745199994,15.2,-10.296336946));
#156359=CARTESIAN_POINT('Ctrl Pts',(1.33424745199994,11.6,-10.296336946));
#156360=CARTESIAN_POINT('Ctrl Pts',(1.33421316699994,15.2,-10.295368778));
#156361=CARTESIAN_POINT('Ctrl Pts',(1.33421316699994,11.6,-10.295368778));
#156362=CARTESIAN_POINT('Ctrl Pts',(1.33417825799994,15.2,-10.294410075));
#156363=CARTESIAN_POINT('Ctrl Pts',(1.33417825799994,11.6,-10.294410075));
#156364=CARTESIAN_POINT('Ctrl Pts',(1.33414274299994,15.2,-10.293460862));
#156365=CARTESIAN_POINT('Ctrl Pts',(1.33414274299994,11.6,-10.293460862));
#156366=CARTESIAN_POINT('Ctrl Pts',(1.33410663999994,15.2,-10.292521167));
#156367=CARTESIAN_POINT('Ctrl Pts',(1.33410663999994,11.6,-10.292521167));
#156368=CARTESIAN_POINT('Ctrl Pts',(1.33406996899994,15.2,-10.291591017));
#156369=CARTESIAN_POINT('Ctrl Pts',(1.33406996899994,11.6,-10.291591017));
#156370=CARTESIAN_POINT('Ctrl Pts',(1.33403296599994,15.2,-10.290675738));
#156371=CARTESIAN_POINT('Ctrl Pts',(1.33403296599994,11.6,-10.290675738));
#156372=CARTESIAN_POINT('Ctrl Pts',(1.33400298699994,15.2,-10.289952142));
#156373=CARTESIAN_POINT('Ctrl Pts',(1.33400298699994,11.6,-10.289952142));
#156374=CARTESIAN_POINT('Ctrl Pts',(1.33398033299994,15.2,-10.289415004));
#156375=CARTESIAN_POINT('Ctrl Pts',(1.33398033299994,11.6,-10.289415004));
#156376=CARTESIAN_POINT('Ctrl Pts',(1.33396520799994,15.2,-10.289060521));
#156377=CARTESIAN_POINT('Ctrl Pts',(1.33396520799994,11.6,-10.289060521));
#156378=CARTESIAN_POINT('Ctrl Pts',(1.33395773199994,15.2,-10.288886323));
#156379=CARTESIAN_POINT('Ctrl Pts',(1.33395773199994,11.6,-10.288886323));
#156380=CARTESIAN_POINT('',(1.33395773199994,12.2,-10.288886323));
#156381=CARTESIAN_POINT('',(1.33395773199994,15.2,-10.288886323));
#156382=CARTESIAN_POINT('',(1.33395773199994,12.2,-10.288886323));
#156383=CARTESIAN_POINT('Ctrl Pts',(1.09337742899994,12.2,-11.447904865));
#156384=CARTESIAN_POINT('Ctrl Pts',(1.09364566999994,12.2,-11.447188878));
#156385=CARTESIAN_POINT('Ctrl Pts',(1.09418172899994,12.2,-11.445757219));
#156386=CARTESIAN_POINT('Ctrl Pts',(1.09498454299994,12.2,-11.443610664));
#156387=CARTESIAN_POINT('Ctrl Pts',(1.09605241599994,12.2,-11.440750465));
#156388=CARTESIAN_POINT('Ctrl Pts',(1.09738301599994,12.2,-11.437178335));
#156389=CARTESIAN_POINT('Ctrl Pts',(1.09870937299994,12.2,-11.433609328));
#156390=CARTESIAN_POINT('Ctrl Pts',(1.10003148899994,12.2,-11.430043446));
#156391=CARTESIAN_POINT('Ctrl Pts',(1.10134936299994,12.2,-11.426480691));
#156392=CARTESIAN_POINT('Ctrl Pts',(1.10266299899994,12.2,-11.422921069));
#156393=CARTESIAN_POINT('Ctrl Pts',(1.10397239799994,12.2,-11.419364591));
#156394=CARTESIAN_POINT('Ctrl Pts',(1.10527756399994,12.2,-11.415811262));
#156395=CARTESIAN_POINT('Ctrl Pts',(1.10657849999994,12.2,-11.412261095));
#156396=CARTESIAN_POINT('Ctrl Pts',(1.10787520999994,12.2,-11.408714099));
#156397=CARTESIAN_POINT('Ctrl Pts',(1.10916769599994,12.2,-11.405170286));
#156398=CARTESIAN_POINT('Ctrl Pts',(1.11045596299994,12.2,-11.401629665));
#156399=CARTESIAN_POINT('Ctrl Pts',(1.11174001299994,12.2,-11.398092244));
#156400=CARTESIAN_POINT('Ctrl Pts',(1.11301984899994,12.2,-11.394558034));
#156401=CARTESIAN_POINT('Ctrl Pts',(1.11429547399994,12.2,-11.39102704));
#156402=CARTESIAN_POINT('Ctrl Pts',(1.11556688999994,12.2,-11.387499272));
#156403=CARTESIAN_POINT('Ctrl Pts',(1.11683409999994,12.2,-11.383974735));
#156404=CARTESIAN_POINT('Ctrl Pts',(1.11809710599994,12.2,-11.38045344));
#156405=CARTESIAN_POINT('Ctrl Pts',(1.11935591099994,12.2,-11.376935393));
#156406=CARTESIAN_POINT('Ctrl Pts',(1.12061051899994,12.2,-11.373420606));
#156407=CARTESIAN_POINT('Ctrl Pts',(1.12186093199994,12.2,-11.369909084));
#156408=CARTESIAN_POINT('Ctrl Pts',(1.12310715399994,12.2,-11.366400839));
#156409=CARTESIAN_POINT('Ctrl Pts',(1.12434918699994,12.2,-11.36289588));
#156410=CARTESIAN_POINT('Ctrl Pts',(1.12558703399994,12.2,-11.359394214));
#156411=CARTESIAN_POINT('Ctrl Pts',(1.12682069999994,12.2,-11.355895851));
#156412=CARTESIAN_POINT('Ctrl Pts',(1.12805018499994,12.2,-11.3524008));
#156413=CARTESIAN_POINT('Ctrl Pts',(1.12927549399994,12.2,-11.348909068));
#156414=CARTESIAN_POINT('Ctrl Pts',(1.13049662999994,12.2,-11.345420665));
#156415=CARTESIAN_POINT('Ctrl Pts',(1.13171359399994,12.2,-11.341935598));
#156416=CARTESIAN_POINT('Ctrl Pts',(1.13292639099994,12.2,-11.338453878));
#156417=CARTESIAN_POINT('Ctrl Pts',(1.13413502299994,12.2,-11.334975512));
#156418=CARTESIAN_POINT('Ctrl Pts',(1.13533949399994,12.2,-11.331500509));
#156419=CARTESIAN_POINT('Ctrl Pts',(1.13653980599994,12.2,-11.32802888));
#156420=CARTESIAN_POINT('Ctrl Pts',(1.13773596199994,12.2,-11.324560631));
#156421=CARTESIAN_POINT('Ctrl Pts',(1.13892796699994,12.2,-11.321095772));
#156422=CARTESIAN_POINT('Ctrl Pts',(1.14011582299994,12.2,-11.317634312));
#156423=CARTESIAN_POINT('Ctrl Pts',(1.14129953199994,12.2,-11.31417626));
#156424=CARTESIAN_POINT('Ctrl Pts',(1.14247909799994,12.2,-11.310721625));
#156425=CARTESIAN_POINT('Ctrl Pts',(1.14365452599994,12.2,-11.307270414));
#156426=CARTESIAN_POINT('Ctrl Pts',(1.14482581499994,12.2,-11.303822638));
#156427=CARTESIAN_POINT('Ctrl Pts',(1.14599297199994,12.2,-11.300378306));
#156428=CARTESIAN_POINT('Ctrl Pts',(1.14715599899994,12.2,-11.296937426));
#156429=CARTESIAN_POINT('Ctrl Pts',(1.14831489899994,12.2,-11.293500006));
#156430=CARTESIAN_POINT('Ctrl Pts',(1.14946967399994,12.2,-11.290066057));
#156431=CARTESIAN_POINT('Ctrl Pts',(1.15062032899994,12.2,-11.286635586));
#156432=CARTESIAN_POINT('Ctrl Pts',(1.15176686799994,12.2,-11.283208603));
#156433=CARTESIAN_POINT('Ctrl Pts',(1.15290929199994,12.2,-11.279785118));
#156434=CARTESIAN_POINT('Ctrl Pts',(1.15404760399994,12.2,-11.276365138));
#156435=CARTESIAN_POINT('Ctrl Pts',(1.15518180899994,12.2,-11.272948673));
#156436=CARTESIAN_POINT('Ctrl Pts',(1.15631190999994,12.2,-11.269535732));
#156437=CARTESIAN_POINT('Ctrl Pts',(1.15743790999994,12.2,-11.266126325));
#156438=CARTESIAN_POINT('Ctrl Pts',(1.15855981299994,12.2,-11.262720459));
#156439=CARTESIAN_POINT('Ctrl Pts',(1.15967762099994,12.2,-11.259318144));
#156440=CARTESIAN_POINT('Ctrl Pts',(1.16079133799994,12.2,-11.25591939));
#156441=CARTESIAN_POINT('Ctrl Pts',(1.16190096699994,12.2,-11.252524204));
#156442=CARTESIAN_POINT('Ctrl Pts',(1.16300651299994,12.2,-11.249132598));
#156443=CARTESIAN_POINT('Ctrl Pts',(1.16410797799994,12.2,-11.245744578));
#156444=CARTESIAN_POINT('Ctrl Pts',(1.16520536399994,12.2,-11.242360155));
#156445=CARTESIAN_POINT('Ctrl Pts',(1.16629867699995,12.2,-11.238979338));
#156446=CARTESIAN_POINT('Ctrl Pts',(1.16738791999994,12.2,-11.235602136));
#156447=CARTESIAN_POINT('Ctrl Pts',(1.16847309399994,12.2,-11.232228557));
#156448=CARTESIAN_POINT('Ctrl Pts',(1.16955420599994,12.2,-11.228858612));
#156449=CARTESIAN_POINT('Ctrl Pts',(1.17063125699994,12.2,-11.22549231));
#156450=CARTESIAN_POINT('Ctrl Pts',(1.17170425099994,12.2,-11.222129659));
#156451=CARTESIAN_POINT('Ctrl Pts',(1.17277319199994,12.2,-11.218770669));
#156452=CARTESIAN_POINT('Ctrl Pts',(1.17383808199994,12.2,-11.215415349));
#156453=CARTESIAN_POINT('Ctrl Pts',(1.17489892699994,12.2,-11.212063708));
#156454=CARTESIAN_POINT('Ctrl Pts',(1.17595572899994,12.2,-11.208715756));
#156455=CARTESIAN_POINT('Ctrl Pts',(1.17700849199994,12.2,-11.205371503));
#156456=CARTESIAN_POINT('Ctrl Pts',(1.17805721899994,12.2,-11.202030955));
#156457=CARTESIAN_POINT('Ctrl Pts',(1.17910191399994,12.2,-11.198694125));
#156458=CARTESIAN_POINT('Ctrl Pts',(1.18014258099994,12.2,-11.195361021));
#156459=CARTESIAN_POINT('Ctrl Pts',(1.18117922299994,12.2,-11.192031652));
#156460=CARTESIAN_POINT('Ctrl Pts',(1.18221184299994,12.2,-11.188706028));
#156461=CARTESIAN_POINT('Ctrl Pts',(1.18324044599994,12.2,-11.185384157));
#156462=CARTESIAN_POINT('Ctrl Pts',(1.18426503499994,12.2,-11.18206605));
#156463=CARTESIAN_POINT('Ctrl Pts',(1.18528561399994,12.2,-11.178751715));
#156464=CARTESIAN_POINT('Ctrl Pts',(1.18630218599994,12.2,-11.175441163));
#156465=CARTESIAN_POINT('Ctrl Pts',(1.18731475499994,12.2,-11.172134402));
#156466=CARTESIAN_POINT('Ctrl Pts',(1.18832332499994,12.2,-11.168831442));
#156467=CARTESIAN_POINT('Ctrl Pts',(1.18932789799994,12.2,-11.165532292));
#156468=CARTESIAN_POINT('Ctrl Pts',(1.19032848099994,12.2,-11.162236962));
#156469=CARTESIAN_POINT('Ctrl Pts',(1.19132507499994,12.2,-11.158945462));
#156470=CARTESIAN_POINT('Ctrl Pts',(1.19231768599994,12.2,-11.155657801));
#156471=CARTESIAN_POINT('Ctrl Pts',(1.19330631499994,12.2,-11.152373988));
#156472=CARTESIAN_POINT('Ctrl Pts',(1.19429096799994,12.2,-11.149094033));
#156473=CARTESIAN_POINT('Ctrl Pts',(1.19527164899994,12.2,-11.145817945));
#156474=CARTESIAN_POINT('Ctrl Pts',(1.19624835999994,12.2,-11.142545735));
#156475=CARTESIAN_POINT('Ctrl Pts',(1.19722110599994,12.2,-11.139277411));
#156476=CARTESIAN_POINT('Ctrl Pts',(1.19818989099994,12.2,-11.136012983));
#156477=CARTESIAN_POINT('Ctrl Pts',(1.19915471699994,12.2,-11.132752462));
#156478=CARTESIAN_POINT('Ctrl Pts',(1.20011559099995,12.2,-11.129495855));
#156479=CARTESIAN_POINT('Ctrl Pts',(1.20107251499994,12.2,-11.126243174));
#156480=CARTESIAN_POINT('Ctrl Pts',(1.20202549299994,12.2,-11.122994428));
#156481=CARTESIAN_POINT('Ctrl Pts',(1.20297452899994,12.2,-11.119749625));
#156482=CARTESIAN_POINT('Ctrl Pts',(1.20391962699994,12.2,-11.116508778));
#156483=CARTESIAN_POINT('Ctrl Pts',(1.20486078999994,12.2,-11.113271894));
#156484=CARTESIAN_POINT('Ctrl Pts',(1.20579802499994,12.2,-11.110038983));
#156485=CARTESIAN_POINT('Ctrl Pts',(1.20673133299994,12.2,-11.106810055));
#156486=CARTESIAN_POINT('Ctrl Pts',(1.20766071899994,12.2,-11.103585121));
#156487=CARTESIAN_POINT('Ctrl Pts',(1.20858618699994,12.2,-11.100364189));
#156488=CARTESIAN_POINT('Ctrl Pts',(1.20950774199994,12.2,-11.09714727));
#156489=CARTESIAN_POINT('Ctrl Pts',(1.21042538699994,12.2,-11.093934372));
#156490=CARTESIAN_POINT('Ctrl Pts',(1.21133912499995,12.2,-11.090725508));
#156491=CARTESIAN_POINT('Ctrl Pts',(1.21224896299994,12.2,-11.087520685));
#156492=CARTESIAN_POINT('Ctrl Pts',(1.21315490199994,12.2,-11.084319915));
#156493=CARTESIAN_POINT('Ctrl Pts',(1.21405694699994,12.2,-11.081123205));
#156494=CARTESIAN_POINT('Ctrl Pts',(1.21495510399994,12.2,-11.077930567));
#156495=CARTESIAN_POINT('Ctrl Pts',(1.21584937499994,12.2,-11.074742011));
#156496=CARTESIAN_POINT('Ctrl Pts',(1.21673976599994,12.2,-11.071557546));
#156497=CARTESIAN_POINT('Ctrl Pts',(1.21762627899994,12.2,-11.068377182));
#156498=CARTESIAN_POINT('Ctrl Pts',(1.21850891999994,12.2,-11.06520093));
#156499=CARTESIAN_POINT('Ctrl Pts',(1.21938769199994,12.2,-11.062028798));
#156500=CARTESIAN_POINT('Ctrl Pts',(1.22026259999994,12.2,-11.058860798));
#156501=CARTESIAN_POINT('Ctrl Pts',(1.22113364899994,12.2,-11.055696939));
#156502=CARTESIAN_POINT('Ctrl Pts',(1.22200084099994,12.2,-11.052537231));
#156503=CARTESIAN_POINT('Ctrl Pts',(1.22286418199994,12.2,-11.049381684));
#156504=CARTESIAN_POINT('Ctrl Pts',(1.22372367599994,12.2,-11.046230309));
#156505=CARTESIAN_POINT('Ctrl Pts',(1.22457932699994,12.2,-11.043083114));
#156506=CARTESIAN_POINT('Ctrl Pts',(1.22543113999994,12.2,-11.03994011));
#156507=CARTESIAN_POINT('Ctrl Pts',(1.22627911799994,12.2,-11.036801309));
#156508=CARTESIAN_POINT('Ctrl Pts',(1.22712326699994,12.2,-11.033666719));
#156509=CARTESIAN_POINT('Ctrl Pts',(1.22796359099994,12.2,-11.030536351));
#156510=CARTESIAN_POINT('Ctrl Pts',(1.22880009299994,12.2,-11.027410214));
#156511=CARTESIAN_POINT('Ctrl Pts',(1.22963277899994,12.2,-11.024288319));
#156512=CARTESIAN_POINT('Ctrl Pts',(1.23046165299994,12.2,-11.021170677));
#156513=CARTESIAN_POINT('Ctrl Pts',(1.23128671899994,12.2,-11.018057297));
#156514=CARTESIAN_POINT('Ctrl Pts',(1.23210798199994,12.2,-11.01494819));
#156515=CARTESIAN_POINT('Ctrl Pts',(1.23292544599995,12.2,-11.011843364));
#156516=CARTESIAN_POINT('Ctrl Pts',(1.23373911599994,12.2,-11.008742833));
#156517=CARTESIAN_POINT('Ctrl Pts',(1.23454899599994,12.2,-11.005646604));
#156518=CARTESIAN_POINT('Ctrl Pts',(1.23535509099994,12.2,-11.002554689));
#156519=CARTESIAN_POINT('Ctrl Pts',(1.23615740499994,12.2,-10.999467099));
#156520=CARTESIAN_POINT('Ctrl Pts',(1.23695594399994,12.2,-10.996383842));
#156521=CARTESIAN_POINT('Ctrl Pts',(1.23775071099994,12.2,-10.99330493));
#156522=CARTESIAN_POINT('Ctrl Pts',(1.23854171099994,12.2,-10.990230373));
#156523=CARTESIAN_POINT('Ctrl Pts',(1.23932894799994,12.2,-10.98716018));
#156524=CARTESIAN_POINT('Ctrl Pts',(1.24011242899994,12.2,-10.984094365));
#156525=CARTESIAN_POINT('Ctrl Pts',(1.24089215599994,12.2,-10.981032935));
#156526=CARTESIAN_POINT('Ctrl Pts',(1.24166813499994,12.2,-10.977975901));
#156527=CARTESIAN_POINT('Ctrl Pts',(1.24244037099994,12.2,-10.974923275));
#156528=CARTESIAN_POINT('Ctrl Pts',(1.24320886799994,12.2,-10.971875066));
#156529=CARTESIAN_POINT('Ctrl Pts',(1.24397362999994,12.2,-10.968831284));
#156530=CARTESIAN_POINT('Ctrl Pts',(1.24473466399994,12.2,-10.965791941));
#156531=CARTESIAN_POINT('Ctrl Pts',(1.24549197299994,12.2,-10.962757048));
#156532=CARTESIAN_POINT('Ctrl Pts',(1.24624556199994,12.2,-10.959726614));
#156533=CARTESIAN_POINT('Ctrl Pts',(1.24699543599994,12.2,-10.95670065));
#156534=CARTESIAN_POINT('Ctrl Pts',(1.24774159999994,12.2,-10.953679166));
#156535=CARTESIAN_POINT('Ctrl Pts',(1.24848405899994,12.2,-10.950662174));
#156536=CARTESIAN_POINT('Ctrl Pts',(1.24922281699994,12.2,-10.947649684));
#156537=CARTESIAN_POINT('Ctrl Pts',(1.24995787899994,12.2,-10.944641705));
#156538=CARTESIAN_POINT('Ctrl Pts',(1.25068925199994,12.2,-10.941638251));
#156539=CARTESIAN_POINT('Ctrl Pts',(1.25141693799994,12.2,-10.93863933));
#156540=CARTESIAN_POINT('Ctrl Pts',(1.25214094299994,12.2,-10.935644954));
#156541=CARTESIAN_POINT('Ctrl Pts',(1.25286127299994,12.2,-10.932655133));
#156542=CARTESIAN_POINT('Ctrl Pts',(1.25357793199994,12.2,-10.929669878));
#156543=CARTESIAN_POINT('Ctrl Pts',(1.25429092499994,12.2,-10.9266892));
#156544=CARTESIAN_POINT('Ctrl Pts',(1.25500025699994,12.2,-10.923713108));
#156545=CARTESIAN_POINT('Ctrl Pts',(1.25570593399994,12.2,-10.920741616));
#156546=CARTESIAN_POINT('Ctrl Pts',(1.25640795899994,12.2,-10.917774733));
#156547=CARTESIAN_POINT('Ctrl Pts',(1.25710633899994,12.2,-10.91481247));
#156548=CARTESIAN_POINT('Ctrl Pts',(1.25780107799994,12.2,-10.911854838));
#156549=CARTESIAN_POINT('Ctrl Pts',(1.25849218299994,12.2,-10.908901847));
#156550=CARTESIAN_POINT('Ctrl Pts',(1.25917965599994,12.2,-10.905953509));
#156551=CARTESIAN_POINT('Ctrl Pts',(1.25986350399994,12.2,-10.903009834));
#156552=CARTESIAN_POINT('Ctrl Pts',(1.26054373299994,12.2,-10.900070834));
#156553=CARTESIAN_POINT('Ctrl Pts',(1.26122034599994,12.2,-10.89713652));
#156554=CARTESIAN_POINT('Ctrl Pts',(1.26189334999994,12.2,-10.894206901));
#156555=CARTESIAN_POINT('Ctrl Pts',(1.26256274999994,12.2,-10.89128199));
#156556=CARTESIAN_POINT('Ctrl Pts',(1.26322855099994,12.2,-10.888361798));
#156557=CARTESIAN_POINT('Ctrl Pts',(1.26389075699994,12.2,-10.885446335));
#156558=CARTESIAN_POINT('Ctrl Pts',(1.26454937499994,12.2,-10.882535612));
#156559=CARTESIAN_POINT('Ctrl Pts',(1.26520440999994,12.2,-10.879629641));
#156560=CARTESIAN_POINT('Ctrl Pts',(1.26585586699994,12.2,-10.876728433));
#156561=CARTESIAN_POINT('Ctrl Pts',(1.26650375199994,12.2,-10.873831999));
#156562=CARTESIAN_POINT('Ctrl Pts',(1.26714806899994,12.2,-10.870940349));
#156563=CARTESIAN_POINT('Ctrl Pts',(1.26778882499994,12.2,-10.868053496));
#156564=CARTESIAN_POINT('Ctrl Pts',(1.26842602399994,12.2,-10.86517145));
#156565=CARTESIAN_POINT('Ctrl Pts',(1.26905967299994,12.2,-10.862294222));
#156566=CARTESIAN_POINT('Ctrl Pts',(1.26968977599994,12.2,-10.859421825));
#156567=CARTESIAN_POINT('Ctrl Pts',(1.27031633899994,12.2,-10.856554267));
#156568=CARTESIAN_POINT('Ctrl Pts',(1.27093936699994,12.2,-10.853691563));
#156569=CARTESIAN_POINT('Ctrl Pts',(1.27155886699994,12.2,-10.850833723));
#156570=CARTESIAN_POINT('Ctrl Pts',(1.27217484299994,12.2,-10.847980757));
#156571=CARTESIAN_POINT('Ctrl Pts',(1.27278730099994,12.2,-10.845132677));
#156572=CARTESIAN_POINT('Ctrl Pts',(1.27339624799994,12.2,-10.842289496));
#156573=CARTESIAN_POINT('Ctrl Pts',(1.27400168799994,12.2,-10.839451223));
#156574=CARTESIAN_POINT('Ctrl Pts',(1.27460362599994,12.2,-10.83661787));
#156575=CARTESIAN_POINT('Ctrl Pts',(1.27520206999994,12.2,-10.833789449));
#156576=CARTESIAN_POINT('Ctrl Pts',(1.27579702299994,12.2,-10.830965973));
#156577=CARTESIAN_POINT('Ctrl Pts',(1.27638849299994,12.2,-10.828147449));
#156578=CARTESIAN_POINT('Ctrl Pts',(1.27697648499994,12.2,-10.825333894));
#156579=CARTESIAN_POINT('Ctrl Pts',(1.27756100499994,12.2,-10.822525316));
#156580=CARTESIAN_POINT('Ctrl Pts',(1.27814205599994,12.2,-10.819721726));
#156581=CARTESIAN_POINT('Ctrl Pts',(1.27871964799994,12.2,-10.816923139));
#156582=CARTESIAN_POINT('Ctrl Pts',(1.27929378499994,12.2,-10.814129563));
#156583=CARTESIAN_POINT('Ctrl Pts',(1.27986447099994,12.2,-10.811341012));
#156584=CARTESIAN_POINT('Ctrl Pts',(1.28043171499994,12.2,-10.808557497));
#156585=CARTESIAN_POINT('Ctrl Pts',(1.28099552199994,12.2,-10.805779028));
#156586=CARTESIAN_POINT('Ctrl Pts',(1.28155589699994,12.2,-10.80300562));
#156587=CARTESIAN_POINT('Ctrl Pts',(1.28211284599994,12.2,-10.800237282));
#156588=CARTESIAN_POINT('Ctrl Pts',(1.28266637399994,12.2,-10.797474026));
#156589=CARTESIAN_POINT('Ctrl Pts',(1.28321648999994,12.2,-10.794715865));
#156590=CARTESIAN_POINT('Ctrl Pts',(1.28376319699994,12.2,-10.791962811));
#156591=CARTESIAN_POINT('Ctrl Pts',(1.28430650299994,12.2,-10.789214873));
#156592=CARTESIAN_POINT('Ctrl Pts',(1.28484641299994,12.2,-10.786472067));
#156593=CARTESIAN_POINT('Ctrl Pts',(1.28538293299994,12.2,-10.7837344));
#156594=CARTESIAN_POINT('Ctrl Pts',(1.28591606999994,12.2,-10.781001888));
#156595=CARTESIAN_POINT('Ctrl Pts',(1.28644582999994,12.2,-10.778274541));
#156596=CARTESIAN_POINT('Ctrl Pts',(1.28697221699994,12.2,-10.775552372));
#156597=CARTESIAN_POINT('Ctrl Pts',(1.28749524099994,12.2,-10.772835393));
#156598=CARTESIAN_POINT('Ctrl Pts',(1.28801490399994,12.2,-10.770123614));
#156599=CARTESIAN_POINT('Ctrl Pts',(1.28853121599994,12.2,-10.767417049));
#156600=CARTESIAN_POINT('Ctrl Pts',(1.28904418099994,12.2,-10.764715709));
#156601=CARTESIAN_POINT('Ctrl Pts',(1.28955380499994,12.2,-10.762019607));
#156602=CARTESIAN_POINT('Ctrl Pts',(1.29006009599994,12.2,-10.759328754));
#156603=CARTESIAN_POINT('Ctrl Pts',(1.29056305799994,12.2,-10.756643162));
#156604=CARTESIAN_POINT('Ctrl Pts',(1.29106269899994,12.2,-10.753962844));
#156605=CARTESIAN_POINT('Ctrl Pts',(1.29155902499994,12.2,-10.751287813));
#156606=CARTESIAN_POINT('Ctrl Pts',(1.29205204299994,12.2,-10.748618079));
#156607=CARTESIAN_POINT('Ctrl Pts',(1.29254175999994,12.2,-10.745953656));
#156608=CARTESIAN_POINT('Ctrl Pts',(1.29302817899994,12.2,-10.743294554));
#156609=CARTESIAN_POINT('Ctrl Pts',(1.29351130999994,12.2,-10.740640788));
#156610=CARTESIAN_POINT('Ctrl Pts',(1.29399115799994,12.2,-10.737992369));
#156611=CARTESIAN_POINT('Ctrl Pts',(1.29446772899994,12.2,-10.73534931));
#156612=CARTESIAN_POINT('Ctrl Pts',(1.29494102999994,12.2,-10.732711622));
#156613=CARTESIAN_POINT('Ctrl Pts',(1.29541106899994,12.2,-10.730079319));
#156614=CARTESIAN_POINT('Ctrl Pts',(1.29587784999994,12.2,-10.727452411));
#156615=CARTESIAN_POINT('Ctrl Pts',(1.29634138199994,12.2,-10.724830913));
#156616=CARTESIAN_POINT('Ctrl Pts',(1.29680167099994,12.2,-10.722214836));
#156617=CARTESIAN_POINT('Ctrl Pts',(1.29725872199994,12.2,-10.719604194));
#156618=CARTESIAN_POINT('Ctrl Pts',(1.29771254399994,12.2,-10.716998997));
#156619=CARTESIAN_POINT('Ctrl Pts',(1.29816314199994,12.2,-10.714399259));
#156620=CARTESIAN_POINT('Ctrl Pts',(1.29861052399994,12.2,-10.711804993));
#156621=CARTESIAN_POINT('Ctrl Pts',(1.29905469599994,12.2,-10.70921621));
#156622=CARTESIAN_POINT('Ctrl Pts',(1.29949566599994,12.2,-10.706632926));
#156623=CARTESIAN_POINT('Ctrl Pts',(1.29993343799994,12.2,-10.70405515));
#156624=CARTESIAN_POINT('Ctrl Pts',(1.30036802199994,12.2,-10.701482895));
#156625=CARTESIAN_POINT('Ctrl Pts',(1.30079942299994,12.2,-10.698916176));
#156626=CARTESIAN_POINT('Ctrl Pts',(1.30122764799994,12.2,-10.696355005));
#156627=CARTESIAN_POINT('Ctrl Pts',(1.30165270499994,12.2,-10.693799393));
#156628=CARTESIAN_POINT('Ctrl Pts',(1.30207460099994,12.2,-10.691249355));
#156629=CARTESIAN_POINT('Ctrl Pts',(1.30249334099994,12.2,-10.688704902));
#156630=CARTESIAN_POINT('Ctrl Pts',(1.30290893499994,12.2,-10.686166048));
#156631=CARTESIAN_POINT('Ctrl Pts',(1.30332138799994,12.2,-10.683632806));
#156632=CARTESIAN_POINT('Ctrl Pts',(1.30373070599994,12.2,-10.681105188));
#156633=CARTESIAN_POINT('Ctrl Pts',(1.30413689999994,12.2,-10.678583208));
#156634=CARTESIAN_POINT('Ctrl Pts',(1.30453997299994,12.2,-10.676066879));
#156635=CARTESIAN_POINT('Ctrl Pts',(1.30493993399994,12.2,-10.673556212));
#156636=CARTESIAN_POINT('Ctrl Pts',(1.30533679099994,12.2,-10.671051222));
#156637=CARTESIAN_POINT('Ctrl Pts',(1.30573054999994,12.2,-10.668551921));
#156638=CARTESIAN_POINT('Ctrl Pts',(1.30612121799994,12.2,-10.666058323));
#156639=CARTESIAN_POINT('Ctrl Pts',(1.30650880299994,12.2,-10.663570441));
#156640=CARTESIAN_POINT('Ctrl Pts',(1.30689331299994,12.2,-10.661088288));
#156641=CARTESIAN_POINT('Ctrl Pts',(1.30727475299994,12.2,-10.658611877));
#156642=CARTESIAN_POINT('Ctrl Pts',(1.30765313299994,12.2,-10.65614122));
#156643=CARTESIAN_POINT('Ctrl Pts',(1.30802845799994,12.2,-10.653676332));
#156644=CARTESIAN_POINT('Ctrl Pts',(1.30840073799994,12.2,-10.651217227));
#156645=CARTESIAN_POINT('Ctrl Pts',(1.30876997899994,12.2,-10.648763916));
#156646=CARTESIAN_POINT('Ctrl Pts',(1.30913618799994,12.2,-10.646316414));
#156647=CARTESIAN_POINT('Ctrl Pts',(1.30949937299994,12.2,-10.643874733));
#156648=CARTESIAN_POINT('Ctrl Pts',(1.30985954199994,12.2,-10.641438888));
#156649=CARTESIAN_POINT('Ctrl Pts',(1.31021670199994,12.2,-10.639008891));
#156650=CARTESIAN_POINT('Ctrl Pts',(1.31057086099994,12.2,-10.636584756));
#156651=CARTESIAN_POINT('Ctrl Pts',(1.31092202599994,12.2,-10.634166498));
#156652=CARTESIAN_POINT('Ctrl Pts',(1.31127020599994,12.2,-10.631754128));
#156653=CARTESIAN_POINT('Ctrl Pts',(1.31161540699994,12.2,-10.629347661));
#156654=CARTESIAN_POINT('Ctrl Pts',(1.31195763899994,12.2,-10.62694711));
#156655=CARTESIAN_POINT('Ctrl Pts',(1.31229690599994,12.2,-10.62455249));
#156656=CARTESIAN_POINT('Ctrl Pts',(1.31263321999994,12.2,-10.622163812));
#156657=CARTESIAN_POINT('Ctrl Pts',(1.31296658599994,12.2,-10.619781092));
#156658=CARTESIAN_POINT('Ctrl Pts',(1.31329701299994,12.2,-10.617404343));
#156659=CARTESIAN_POINT('Ctrl Pts',(1.31362450899994,12.2,-10.615033578));
#156660=CARTESIAN_POINT('Ctrl Pts',(1.31394908099994,12.2,-10.612668813));
#156661=CARTESIAN_POINT('Ctrl Pts',(1.31427073799994,12.2,-10.61031006));
#156662=CARTESIAN_POINT('Ctrl Pts',(1.31458948699994,12.2,-10.607957333));
#156663=CARTESIAN_POINT('Ctrl Pts',(1.31490533699994,12.2,-10.605610646));
#156664=CARTESIAN_POINT('Ctrl Pts',(1.31521829599994,12.2,-10.603270013));
#156665=CARTESIAN_POINT('Ctrl Pts',(1.31552837099994,12.2,-10.600935449));
#156666=CARTESIAN_POINT('Ctrl Pts',(1.31583557099994,12.2,-10.598606966));
#156667=CARTESIAN_POINT('Ctrl Pts',(1.31613990399994,12.2,-10.59628458));
#156668=CARTESIAN_POINT('Ctrl Pts',(1.31644137799994,12.2,-10.593968305));
#156669=CARTESIAN_POINT('Ctrl Pts',(1.31674000099994,12.2,-10.591658153));
#156670=CARTESIAN_POINT('Ctrl Pts',(1.31703578199994,12.2,-10.58935414));
#156671=CARTESIAN_POINT('Ctrl Pts',(1.31732872999994,12.2,-10.58705628));
#156672=CARTESIAN_POINT('Ctrl Pts',(1.31761885099994,12.2,-10.584764587));
#156673=CARTESIAN_POINT('Ctrl Pts',(1.31790615399994,12.2,-10.582479074));
#156674=CARTESIAN_POINT('Ctrl Pts',(1.31819064899994,12.2,-10.580199758));
#156675=CARTESIAN_POINT('Ctrl Pts',(1.31847234299994,12.2,-10.577926652));
#156676=CARTESIAN_POINT('Ctrl Pts',(1.31875124399994,12.2,-10.575659769));
#156677=CARTESIAN_POINT('Ctrl Pts',(1.31902736199994,12.2,-10.573399125));
#156678=CARTESIAN_POINT('Ctrl Pts',(1.31930070599994,12.2,-10.571144734));
#156679=CARTESIAN_POINT('Ctrl Pts',(1.31957128199994,12.2,-10.56889661));
#156680=CARTESIAN_POINT('Ctrl Pts',(1.31983910099994,12.2,-10.566654769));
#156681=CARTESIAN_POINT('Ctrl Pts',(1.32010416999994,12.2,-10.564419224));
#156682=CARTESIAN_POINT('Ctrl Pts',(1.32036649799994,12.2,-10.562189991));
#156683=CARTESIAN_POINT('Ctrl Pts',(1.32062609499994,12.2,-10.559967084));
#156684=CARTESIAN_POINT('Ctrl Pts',(1.32088296799994,12.2,-10.557750517));
#156685=CARTESIAN_POINT('Ctrl Pts',(1.32113712699994,12.2,-10.555540305));
#156686=CARTESIAN_POINT('Ctrl Pts',(1.32138857999994,12.2,-10.553336463));
#156687=CARTESIAN_POINT('Ctrl Pts',(1.32163733599994,12.2,-10.551139007));
#156688=CARTESIAN_POINT('Ctrl Pts',(1.32188340499994,12.2,-10.548947949));
#156689=CARTESIAN_POINT('Ctrl Pts',(1.32212679399994,12.2,-10.546763306));
#156690=CARTESIAN_POINT('Ctrl Pts',(1.32236751399994,12.2,-10.544585093));
#156691=CARTESIAN_POINT('Ctrl Pts',(1.32260557299994,12.2,-10.542413324));
#156692=CARTESIAN_POINT('Ctrl Pts',(1.32284097899994,12.2,-10.540248014));
#156693=CARTESIAN_POINT('Ctrl Pts',(1.32307374299994,12.2,-10.53808918));
#156694=CARTESIAN_POINT('Ctrl Pts',(1.32330387399994,12.2,-10.535936834));
#156695=CARTESIAN_POINT('Ctrl Pts',(1.32353137899994,12.2,-10.533790993));
#156696=CARTESIAN_POINT('Ctrl Pts',(1.32375626899994,12.2,-10.531651672));
#156697=CARTESIAN_POINT('Ctrl Pts',(1.32397855299994,12.2,-10.529518885));
#156698=CARTESIAN_POINT('Ctrl Pts',(1.32419823999994,12.2,-10.52739265));
#156699=CARTESIAN_POINT('Ctrl Pts',(1.32441533999994,12.2,-10.52527298));
#156700=CARTESIAN_POINT('Ctrl Pts',(1.32462986099994,12.2,-10.523159891));
#156701=CARTESIAN_POINT('Ctrl Pts',(1.32484181499994,12.2,-10.521053397));
#156702=CARTESIAN_POINT('Ctrl Pts',(1.32505120699994,12.2,-10.518953515));
#156703=CARTESIAN_POINT('Ctrl Pts',(1.32525805199994,12.2,-10.516860261));
#156704=CARTESIAN_POINT('Ctrl Pts',(1.32546235399994,12.2,-10.514773649));
#156705=CARTESIAN_POINT('Ctrl Pts',(1.32566412699994,12.2,-10.512693695));
#156706=CARTESIAN_POINT('Ctrl Pts',(1.32586337699994,12.2,-10.510620415));
#156707=CARTESIAN_POINT('Ctrl Pts',(1.32606011699994,12.2,-10.508553825));
#156708=CARTESIAN_POINT('Ctrl Pts',(1.32625435399994,12.2,-10.506493939));
#156709=CARTESIAN_POINT('Ctrl Pts',(1.32644609999994,12.2,-10.504440774));
#156710=CARTESIAN_POINT('Ctrl Pts',(1.32663536199994,12.2,-10.502394346));
#156711=CARTESIAN_POINT('Ctrl Pts',(1.32682215299994,12.2,-10.500354671));
#156712=CARTESIAN_POINT('Ctrl Pts',(1.32700648099994,12.2,-10.498321763));
#156713=CARTESIAN_POINT('Ctrl Pts',(1.32718835599994,12.2,-10.49629564));
#156714=CARTESIAN_POINT('Ctrl Pts',(1.32736778799994,12.2,-10.494276317));
#156715=CARTESIAN_POINT('Ctrl Pts',(1.32754478699994,12.2,-10.49226381));
#156716=CARTESIAN_POINT('Ctrl Pts',(1.32771936299994,12.2,-10.490258135));
#156717=CARTESIAN_POINT('Ctrl Pts',(1.32789152599994,12.2,-10.488259308));
#156718=CARTESIAN_POINT('Ctrl Pts',(1.32806128599994,12.2,-10.486267346));
#156719=CARTESIAN_POINT('Ctrl Pts',(1.32822865399994,12.2,-10.484282264));
#156720=CARTESIAN_POINT('Ctrl Pts',(1.32839363899994,12.2,-10.48230408));
#156721=CARTESIAN_POINT('Ctrl Pts',(1.32855625199994,12.2,-10.480332808));
#156722=CARTESIAN_POINT('Ctrl Pts',(1.32871650299994,12.2,-10.478368465));
#156723=CARTESIAN_POINT('Ctrl Pts',(1.32887440299994,12.2,-10.476411069));
#156724=CARTESIAN_POINT('Ctrl Pts',(1.32902996199994,12.2,-10.474460635));
#156725=CARTESIAN_POINT('Ctrl Pts',(1.32918318899994,12.2,-10.47251718));
#156726=CARTESIAN_POINT('Ctrl Pts',(1.32933409699994,12.2,-10.47058072));
#156727=CARTESIAN_POINT('Ctrl Pts',(1.32948269399994,12.2,-10.468651272));
#156728=CARTESIAN_POINT('Ctrl Pts',(1.32962899299994,12.2,-10.466728852));
#156729=CARTESIAN_POINT('Ctrl Pts',(1.32977300299994,12.2,-10.464813477));
#156730=CARTESIAN_POINT('Ctrl Pts',(1.32991473499994,12.2,-10.462905165));
#156731=CARTESIAN_POINT('Ctrl Pts',(1.33005419999994,12.2,-10.461003932));
#156732=CARTESIAN_POINT('Ctrl Pts',(1.33019140799994,12.2,-10.459109793));
#156733=CARTESIAN_POINT('Ctrl Pts',(1.33032637099994,12.2,-10.457222766));
#156734=CARTESIAN_POINT('Ctrl Pts',(1.33045909799994,12.2,-10.45534287));
#156735=CARTESIAN_POINT('Ctrl Pts',(1.33058960299994,12.2,-10.453470121));
#156736=CARTESIAN_POINT('Ctrl Pts',(1.33071789299994,12.2,-10.451604534));
#156737=CARTESIAN_POINT('Ctrl Pts',(1.33084398199994,12.2,-10.449746128));
#156738=CARTESIAN_POINT('Ctrl Pts',(1.33096787999994,12.2,-10.447894919));
#156739=CARTESIAN_POINT('Ctrl Pts',(1.33108959799994,12.2,-10.446050926));
#156740=CARTESIAN_POINT('Ctrl Pts',(1.33120914699994,12.2,-10.444214164));
#156741=CARTESIAN_POINT('Ctrl Pts',(1.33132653899994,12.2,-10.442384652));
#156742=CARTESIAN_POINT('Ctrl Pts',(1.33144178299994,12.2,-10.440562407));
#156743=CARTESIAN_POINT('Ctrl Pts',(1.33155489399994,12.2,-10.438747447));
#156744=CARTESIAN_POINT('Ctrl Pts',(1.33166587999994,12.2,-10.436939788));
#156745=CARTESIAN_POINT('Ctrl Pts',(1.33177475499994,12.2,-10.435139448));
#156746=CARTESIAN_POINT('Ctrl Pts',(1.33188152799994,12.2,-10.433346446));
#156747=CARTESIAN_POINT('Ctrl Pts',(1.33198621199994,12.2,-10.431560797));
#156748=CARTESIAN_POINT('Ctrl Pts',(1.33208881899994,12.2,-10.429782521));
#156749=CARTESIAN_POINT('Ctrl Pts',(1.33218935899994,12.2,-10.428011636));
#156750=CARTESIAN_POINT('Ctrl Pts',(1.33228784499994,12.2,-10.426248158));
#156751=CARTESIAN_POINT('Ctrl Pts',(1.33238428799994,12.2,-10.424492106));
#156752=CARTESIAN_POINT('Ctrl Pts',(1.33247869999994,12.2,-10.422743497));
#156753=CARTESIAN_POINT('Ctrl Pts',(1.33257109199994,12.2,-10.421002351));
#156754=CARTESIAN_POINT('Ctrl Pts',(1.33266147799994,12.2,-10.419268684));
#156755=CARTESIAN_POINT('Ctrl Pts',(1.33274986699994,12.2,-10.417542515));
#156756=CARTESIAN_POINT('Ctrl Pts',(1.33283627399994,12.2,-10.415823863));
#156757=CARTESIAN_POINT('Ctrl Pts',(1.33292070899994,12.2,-10.414112744));
#156758=CARTESIAN_POINT('Ctrl Pts',(1.33300318399994,12.2,-10.412409178));
#156759=CARTESIAN_POINT('Ctrl Pts',(1.33308371299994,12.2,-10.410713184));
#156760=CARTESIAN_POINT('Ctrl Pts',(1.33316230599994,12.2,-10.409024778));
#156761=CARTESIAN_POINT('Ctrl Pts',(1.33323897699994,12.2,-10.40734398));
#156762=CARTESIAN_POINT('Ctrl Pts',(1.33331373699994,12.2,-10.405670811));
#156763=CARTESIAN_POINT('Ctrl Pts',(1.33338659999994,12.2,-10.404005285));
#156764=CARTESIAN_POINT('Ctrl Pts',(1.33345757699994,12.2,-10.402347423));
#156765=CARTESIAN_POINT('Ctrl Pts',(1.33352668099994,12.2,-10.400697244));
#156766=CARTESIAN_POINT('Ctrl Pts',(1.33359392399994,12.2,-10.399054766));
#156767=CARTESIAN_POINT('Ctrl Pts',(1.33365931999994,12.2,-10.397420008));
#156768=CARTESIAN_POINT('Ctrl Pts',(1.33372287999994,12.2,-10.39579299));
#156769=CARTESIAN_POINT('Ctrl Pts',(1.33378461799994,12.2,-10.39417373));
#156770=CARTESIAN_POINT('Ctrl Pts',(1.33384454499994,12.2,-10.392562248));
#156771=CARTESIAN_POINT('Ctrl Pts',(1.33390267699994,12.2,-10.39095856));
#156772=CARTESIAN_POINT('Ctrl Pts',(1.33395902399994,12.2,-10.38936269));
#156773=CARTESIAN_POINT('Ctrl Pts',(1.33401359999994,12.2,-10.387774654));
#156774=CARTESIAN_POINT('Ctrl Pts',(1.33406641799994,12.2,-10.386194473));
#156775=CARTESIAN_POINT('Ctrl Pts',(1.33411749199994,12.2,-10.384622165));
#156776=CARTESIAN_POINT('Ctrl Pts',(1.33416683399994,12.2,-10.383057751));
#156777=CARTESIAN_POINT('Ctrl Pts',(1.33421445699994,12.2,-10.381501249));
#156778=CARTESIAN_POINT('Ctrl Pts',(1.33426037499994,12.2,-10.379952679));
#156779=CARTESIAN_POINT('Ctrl Pts',(1.33430460199994,12.2,-10.378412062));
#156780=CARTESIAN_POINT('Ctrl Pts',(1.33434714999994,12.2,-10.376879417));
#156781=CARTESIAN_POINT('Ctrl Pts',(1.33438803299994,12.2,-10.375354763));
#156782=CARTESIAN_POINT('Ctrl Pts',(1.33442726499994,12.2,-10.373838121));
#156783=CARTESIAN_POINT('Ctrl Pts',(1.33446485899994,12.2,-10.37232951));
#156784=CARTESIAN_POINT('Ctrl Pts',(1.33450082899994,12.2,-10.370828951));
#156785=CARTESIAN_POINT('Ctrl Pts',(1.33453518799994,12.2,-10.369336464));
#156786=CARTESIAN_POINT('Ctrl Pts',(1.33456795099994,12.2,-10.367852069));
#156787=CARTESIAN_POINT('Ctrl Pts',(1.33459913199994,12.2,-10.366375787));
#156788=CARTESIAN_POINT('Ctrl Pts',(1.33462874399994,12.2,-10.364907637));
#156789=CARTESIAN_POINT('Ctrl Pts',(1.33465680099994,12.2,-10.363447639));
#156790=CARTESIAN_POINT('Ctrl Pts',(1.33468331799994,12.2,-10.361995816));
#156791=CARTESIAN_POINT('Ctrl Pts',(1.33470830799994,12.2,-10.360552186));
#156792=CARTESIAN_POINT('Ctrl Pts',(1.33473178599994,12.2,-10.359116771));
#156793=CARTESIAN_POINT('Ctrl Pts',(1.33475376599994,12.2,-10.357689593));
#156794=CARTESIAN_POINT('Ctrl Pts',(1.33477426199994,12.2,-10.356270671));
#156795=CARTESIAN_POINT('Ctrl Pts',(1.33479328899994,12.2,-10.354860026));
#156796=CARTESIAN_POINT('Ctrl Pts',(1.33481086199994,12.2,-10.353457679));
#156797=CARTESIAN_POINT('Ctrl Pts',(1.33482699499994,12.2,-10.352063652));
#156798=CARTESIAN_POINT('Ctrl Pts',(1.33484170199994,12.2,-10.350677965));
#156799=CARTESIAN_POINT('Ctrl Pts',(1.33485499899994,12.2,-10.34930064));
#156800=CARTESIAN_POINT('Ctrl Pts',(1.33486689899994,12.2,-10.347931697));
#156801=CARTESIAN_POINT('Ctrl Pts',(1.33487741999994,12.2,-10.34657116));
#156802=CARTESIAN_POINT('Ctrl Pts',(1.33488657299994,12.2,-10.345219049));
#156803=CARTESIAN_POINT('Ctrl Pts',(1.33489437599994,12.2,-10.343875384));
#156804=CARTESIAN_POINT('Ctrl Pts',(1.33490084299994,12.2,-10.342540189));
#156805=CARTESIAN_POINT('Ctrl Pts',(1.33490598899994,12.2,-10.341213485));
#156806=CARTESIAN_POINT('Ctrl Pts',(1.33490982999994,12.2,-10.339895294));
#156807=CARTESIAN_POINT('Ctrl Pts',(1.33491238099994,12.2,-10.338585637));
#156808=CARTESIAN_POINT('Ctrl Pts',(1.33491365599994,12.2,-10.337284537));
#156809=CARTESIAN_POINT('Ctrl Pts',(1.33491367299994,12.2,-10.335992016));
#156810=CARTESIAN_POINT('Ctrl Pts',(1.33491244599994,12.2,-10.334708096));
#156811=CARTESIAN_POINT('Ctrl Pts',(1.33490999099994,12.2,-10.333432799));
#156812=CARTESIAN_POINT('Ctrl Pts',(1.33490632299994,12.2,-10.332166147));
#156813=CARTESIAN_POINT('Ctrl Pts',(1.33490145899994,12.2,-10.330908163));
#156814=CARTESIAN_POINT('Ctrl Pts',(1.33489541499994,12.2,-10.32965887));
#156815=CARTESIAN_POINT('Ctrl Pts',(1.33488820599994,12.2,-10.32841829));
#156816=CARTESIAN_POINT('Ctrl Pts',(1.33487984899994,12.2,-10.327186447));
#156817=CARTESIAN_POINT('Ctrl Pts',(1.33487035799994,12.2,-10.32596336));
#156818=CARTESIAN_POINT('Ctrl Pts',(1.33485975199994,12.2,-10.324749056));
#156819=CARTESIAN_POINT('Ctrl Pts',(1.33484804599994,12.2,-10.323543558));
#156820=CARTESIAN_POINT('Ctrl Pts',(1.33483525599994,12.2,-10.322346886));
#156821=CARTESIAN_POINT('Ctrl Pts',(1.33482139999994,12.2,-10.321159066));
#156822=CARTESIAN_POINT('Ctrl Pts',(1.33480649299994,12.2,-10.319980119));
#156823=CARTESIAN_POINT('Ctrl Pts',(1.33479055199994,12.2,-10.318810071));
#156824=CARTESIAN_POINT('Ctrl Pts',(1.33477359399994,12.2,-10.317648943));
#156825=CARTESIAN_POINT('Ctrl Pts',(1.33475563599994,12.2,-10.31649676));
#156826=CARTESIAN_POINT('Ctrl Pts',(1.33473669499994,12.2,-10.315353546));
#156827=CARTESIAN_POINT('Ctrl Pts',(1.33471678699994,12.2,-10.314219324));
#156828=CARTESIAN_POINT('Ctrl Pts',(1.33469592999994,12.2,-10.313094118));
#156829=CARTESIAN_POINT('Ctrl Pts',(1.33467414199994,12.2,-10.311977952));
#156830=CARTESIAN_POINT('Ctrl Pts',(1.33465143899994,12.2,-10.310870851));
#156831=CARTESIAN_POINT('Ctrl Pts',(1.33462783799994,12.2,-10.309772837));
#156832=CARTESIAN_POINT('Ctrl Pts',(1.33460335699994,12.2,-10.308683938));
#156833=CARTESIAN_POINT('Ctrl Pts',(1.33457801399994,12.2,-10.307604175));
#156834=CARTESIAN_POINT('Ctrl Pts',(1.33455182599994,12.2,-10.306533574));
#156835=CARTESIAN_POINT('Ctrl Pts',(1.33452481199994,12.2,-10.30547216));
#156836=CARTESIAN_POINT('Ctrl Pts',(1.33449698899994,12.2,-10.304419957));
#156837=CARTESIAN_POINT('Ctrl Pts',(1.33446837399994,12.2,-10.30337699));
#156838=CARTESIAN_POINT('Ctrl Pts',(1.33443898699994,12.2,-10.302343284));
#156839=CARTESIAN_POINT('Ctrl Pts',(1.33440884499994,12.2,-10.301318864));
#156840=CARTESIAN_POINT('Ctrl Pts',(1.33437796499994,12.2,-10.300303756));
#156841=CARTESIAN_POINT('Ctrl Pts',(1.33434636799994,12.2,-10.299297985));
#156842=CARTESIAN_POINT('Ctrl Pts',(1.33431407099994,12.2,-10.298301576));
#156843=CARTESIAN_POINT('Ctrl Pts',(1.33428109299994,12.2,-10.297314555));
#156844=CARTESIAN_POINT('Ctrl Pts',(1.33424745199994,12.2,-10.296336946));
#156845=CARTESIAN_POINT('Ctrl Pts',(1.33421316699994,12.2,-10.295368778));
#156846=CARTESIAN_POINT('Ctrl Pts',(1.33417825799994,12.2,-10.294410075));
#156847=CARTESIAN_POINT('Ctrl Pts',(1.33414274299994,12.2,-10.293460862));
#156848=CARTESIAN_POINT('Ctrl Pts',(1.33410663999994,12.2,-10.292521167));
#156849=CARTESIAN_POINT('Ctrl Pts',(1.33406996899994,12.2,-10.291591017));
#156850=CARTESIAN_POINT('Ctrl Pts',(1.33403296599994,12.2,-10.290675738));
#156851=CARTESIAN_POINT('Ctrl Pts',(1.33400298699994,12.2,-10.289952142));
#156852=CARTESIAN_POINT('Ctrl Pts',(1.33398033299994,12.2,-10.289415004));
#156853=CARTESIAN_POINT('Ctrl Pts',(1.33396520799994,12.2,-10.289060521));
#156854=CARTESIAN_POINT('Ctrl Pts',(1.33395773199994,12.2,-10.288886323));
#156855=CARTESIAN_POINT('Ctrl Pts',(1.33395773199994,15.2,-10.288886323));
#156856=CARTESIAN_POINT('Ctrl Pts',(1.33396520799994,15.2,-10.289060521));
#156857=CARTESIAN_POINT('Ctrl Pts',(1.33398033299994,15.2,-10.289415004));
#156858=CARTESIAN_POINT('Ctrl Pts',(1.33400298699994,15.2,-10.289952142));
#156859=CARTESIAN_POINT('Ctrl Pts',(1.33403296599994,15.2,-10.290675738));
#156860=CARTESIAN_POINT('Ctrl Pts',(1.33406996899994,15.2,-10.291591017));
#156861=CARTESIAN_POINT('Ctrl Pts',(1.33410663999994,15.2,-10.292521167));
#156862=CARTESIAN_POINT('Ctrl Pts',(1.33414274299994,15.2,-10.293460862));
#156863=CARTESIAN_POINT('Ctrl Pts',(1.33417825799994,15.2,-10.294410075));
#156864=CARTESIAN_POINT('Ctrl Pts',(1.33421316699994,15.2,-10.295368778));
#156865=CARTESIAN_POINT('Ctrl Pts',(1.33424745199994,15.2,-10.296336946));
#156866=CARTESIAN_POINT('Ctrl Pts',(1.33428109299994,15.2,-10.297314555));
#156867=CARTESIAN_POINT('Ctrl Pts',(1.33431407099994,15.2,-10.298301576));
#156868=CARTESIAN_POINT('Ctrl Pts',(1.33434636799994,15.2,-10.299297985));
#156869=CARTESIAN_POINT('Ctrl Pts',(1.33437796499994,15.2,-10.300303756));
#156870=CARTESIAN_POINT('Ctrl Pts',(1.33440884499994,15.2,-10.301318864));
#156871=CARTESIAN_POINT('Ctrl Pts',(1.33443898699994,15.2,-10.302343284));
#156872=CARTESIAN_POINT('Ctrl Pts',(1.33446837399994,15.2,-10.30337699));
#156873=CARTESIAN_POINT('Ctrl Pts',(1.33449698899994,15.2,-10.304419957));
#156874=CARTESIAN_POINT('Ctrl Pts',(1.33452481199994,15.2,-10.30547216));
#156875=CARTESIAN_POINT('Ctrl Pts',(1.33455182599994,15.2,-10.306533574));
#156876=CARTESIAN_POINT('Ctrl Pts',(1.33457801399994,15.2,-10.307604175));
#156877=CARTESIAN_POINT('Ctrl Pts',(1.33460335699994,15.2,-10.308683938));
#156878=CARTESIAN_POINT('Ctrl Pts',(1.33462783799994,15.2,-10.309772837));
#156879=CARTESIAN_POINT('Ctrl Pts',(1.33465143899994,15.2,-10.310870851));
#156880=CARTESIAN_POINT('Ctrl Pts',(1.33467414199994,15.2,-10.311977952));
#156881=CARTESIAN_POINT('Ctrl Pts',(1.33469592999994,15.2,-10.313094118));
#156882=CARTESIAN_POINT('Ctrl Pts',(1.33471678699994,15.2,-10.314219324));
#156883=CARTESIAN_POINT('Ctrl Pts',(1.33473669499994,15.2,-10.315353546));
#156884=CARTESIAN_POINT('Ctrl Pts',(1.33475563599994,15.2,-10.31649676));
#156885=CARTESIAN_POINT('Ctrl Pts',(1.33477359399994,15.2,-10.317648943));
#156886=CARTESIAN_POINT('Ctrl Pts',(1.33479055199994,15.2,-10.318810071));
#156887=CARTESIAN_POINT('Ctrl Pts',(1.33480649299994,15.2,-10.319980119));
#156888=CARTESIAN_POINT('Ctrl Pts',(1.33482139999994,15.2,-10.321159066));
#156889=CARTESIAN_POINT('Ctrl Pts',(1.33483525599994,15.2,-10.322346886));
#156890=CARTESIAN_POINT('Ctrl Pts',(1.33484804599994,15.2,-10.323543558));
#156891=CARTESIAN_POINT('Ctrl Pts',(1.33485975199994,15.2,-10.324749056));
#156892=CARTESIAN_POINT('Ctrl Pts',(1.33487035799994,15.2,-10.32596336));
#156893=CARTESIAN_POINT('Ctrl Pts',(1.33487984899994,15.2,-10.327186447));
#156894=CARTESIAN_POINT('Ctrl Pts',(1.33488820599994,15.2,-10.32841829));
#156895=CARTESIAN_POINT('Ctrl Pts',(1.33489541499994,15.2,-10.32965887));
#156896=CARTESIAN_POINT('Ctrl Pts',(1.33490145899994,15.2,-10.330908163));
#156897=CARTESIAN_POINT('Ctrl Pts',(1.33490632299994,15.2,-10.332166147));
#156898=CARTESIAN_POINT('Ctrl Pts',(1.33490999099994,15.2,-10.333432799));
#156899=CARTESIAN_POINT('Ctrl Pts',(1.33491244599994,15.2,-10.334708096));
#156900=CARTESIAN_POINT('Ctrl Pts',(1.33491367299994,15.2,-10.335992016));
#156901=CARTESIAN_POINT('Ctrl Pts',(1.33491365599994,15.2,-10.337284537));
#156902=CARTESIAN_POINT('Ctrl Pts',(1.33491238099994,15.2,-10.338585637));
#156903=CARTESIAN_POINT('Ctrl Pts',(1.33490982999994,15.2,-10.339895294));
#156904=CARTESIAN_POINT('Ctrl Pts',(1.33490598899994,15.2,-10.341213485));
#156905=CARTESIAN_POINT('Ctrl Pts',(1.33490084299994,15.2,-10.342540189));
#156906=CARTESIAN_POINT('Ctrl Pts',(1.33489437599994,15.2,-10.343875384));
#156907=CARTESIAN_POINT('Ctrl Pts',(1.33488657299994,15.2,-10.345219049));
#156908=CARTESIAN_POINT('Ctrl Pts',(1.33487741999994,15.2,-10.34657116));
#156909=CARTESIAN_POINT('Ctrl Pts',(1.33486689899994,15.2,-10.347931697));
#156910=CARTESIAN_POINT('Ctrl Pts',(1.33485499899994,15.2,-10.34930064));
#156911=CARTESIAN_POINT('Ctrl Pts',(1.33484170199994,15.2,-10.350677965));
#156912=CARTESIAN_POINT('Ctrl Pts',(1.33482699499994,15.2,-10.352063652));
#156913=CARTESIAN_POINT('Ctrl Pts',(1.33481086199994,15.2,-10.353457679));
#156914=CARTESIAN_POINT('Ctrl Pts',(1.33479328899994,15.2,-10.354860026));
#156915=CARTESIAN_POINT('Ctrl Pts',(1.33477426199994,15.2,-10.356270671));
#156916=CARTESIAN_POINT('Ctrl Pts',(1.33475376599994,15.2,-10.357689593));
#156917=CARTESIAN_POINT('Ctrl Pts',(1.33473178599994,15.2,-10.359116771));
#156918=CARTESIAN_POINT('Ctrl Pts',(1.33470830799994,15.2,-10.360552186));
#156919=CARTESIAN_POINT('Ctrl Pts',(1.33468331799994,15.2,-10.361995816));
#156920=CARTESIAN_POINT('Ctrl Pts',(1.33465680099994,15.2,-10.363447639));
#156921=CARTESIAN_POINT('Ctrl Pts',(1.33462874399994,15.2,-10.364907637));
#156922=CARTESIAN_POINT('Ctrl Pts',(1.33459913199994,15.2,-10.366375787));
#156923=CARTESIAN_POINT('Ctrl Pts',(1.33456795099994,15.2,-10.367852069));
#156924=CARTESIAN_POINT('Ctrl Pts',(1.33453518799994,15.2,-10.369336464));
#156925=CARTESIAN_POINT('Ctrl Pts',(1.33450082899994,15.2,-10.370828951));
#156926=CARTESIAN_POINT('Ctrl Pts',(1.33446485899994,15.2,-10.37232951));
#156927=CARTESIAN_POINT('Ctrl Pts',(1.33442726499994,15.2,-10.373838121));
#156928=CARTESIAN_POINT('Ctrl Pts',(1.33438803299994,15.2,-10.375354763));
#156929=CARTESIAN_POINT('Ctrl Pts',(1.33434714999994,15.2,-10.376879417));
#156930=CARTESIAN_POINT('Ctrl Pts',(1.33430460199994,15.2,-10.378412062));
#156931=CARTESIAN_POINT('Ctrl Pts',(1.33426037499994,15.2,-10.379952679));
#156932=CARTESIAN_POINT('Ctrl Pts',(1.33421445699994,15.2,-10.381501249));
#156933=CARTESIAN_POINT('Ctrl Pts',(1.33416683399994,15.2,-10.383057751));
#156934=CARTESIAN_POINT('Ctrl Pts',(1.33411749199994,15.2,-10.384622165));
#156935=CARTESIAN_POINT('Ctrl Pts',(1.33406641799994,15.2,-10.386194473));
#156936=CARTESIAN_POINT('Ctrl Pts',(1.33401359999994,15.2,-10.387774654));
#156937=CARTESIAN_POINT('Ctrl Pts',(1.33395902399994,15.2,-10.38936269));
#156938=CARTESIAN_POINT('Ctrl Pts',(1.33390267699994,15.2,-10.39095856));
#156939=CARTESIAN_POINT('Ctrl Pts',(1.33384454499994,15.2,-10.392562248));
#156940=CARTESIAN_POINT('Ctrl Pts',(1.33378461799994,15.2,-10.39417373));
#156941=CARTESIAN_POINT('Ctrl Pts',(1.33372287999994,15.2,-10.39579299));
#156942=CARTESIAN_POINT('Ctrl Pts',(1.33365931999994,15.2,-10.397420008));
#156943=CARTESIAN_POINT('Ctrl Pts',(1.33359392399994,15.2,-10.399054766));
#156944=CARTESIAN_POINT('Ctrl Pts',(1.33352668099994,15.2,-10.400697244));
#156945=CARTESIAN_POINT('Ctrl Pts',(1.33345757699994,15.2,-10.402347423));
#156946=CARTESIAN_POINT('Ctrl Pts',(1.33338659999994,15.2,-10.404005285));
#156947=CARTESIAN_POINT('Ctrl Pts',(1.33331373699994,15.2,-10.405670811));
#156948=CARTESIAN_POINT('Ctrl Pts',(1.33323897699994,15.2,-10.40734398));
#156949=CARTESIAN_POINT('Ctrl Pts',(1.33316230599994,15.2,-10.409024778));
#156950=CARTESIAN_POINT('Ctrl Pts',(1.33308371299994,15.2,-10.410713184));
#156951=CARTESIAN_POINT('Ctrl Pts',(1.33300318399994,15.2,-10.412409178));
#156952=CARTESIAN_POINT('Ctrl Pts',(1.33292070899994,15.2,-10.414112744));
#156953=CARTESIAN_POINT('Ctrl Pts',(1.33283627399994,15.2,-10.415823863));
#156954=CARTESIAN_POINT('Ctrl Pts',(1.33274986699994,15.2,-10.417542515));
#156955=CARTESIAN_POINT('Ctrl Pts',(1.33266147799994,15.2,-10.419268684));
#156956=CARTESIAN_POINT('Ctrl Pts',(1.33257109199994,15.2,-10.421002351));
#156957=CARTESIAN_POINT('Ctrl Pts',(1.33247869999994,15.2,-10.422743497));
#156958=CARTESIAN_POINT('Ctrl Pts',(1.33238428799994,15.2,-10.424492106));
#156959=CARTESIAN_POINT('Ctrl Pts',(1.33228784499994,15.2,-10.426248158));
#156960=CARTESIAN_POINT('Ctrl Pts',(1.33218935899994,15.2,-10.428011636));
#156961=CARTESIAN_POINT('Ctrl Pts',(1.33208881899994,15.2,-10.429782521));
#156962=CARTESIAN_POINT('Ctrl Pts',(1.33198621199994,15.2,-10.431560797));
#156963=CARTESIAN_POINT('Ctrl Pts',(1.33188152799994,15.2,-10.433346446));
#156964=CARTESIAN_POINT('Ctrl Pts',(1.33177475499994,15.2,-10.435139448));
#156965=CARTESIAN_POINT('Ctrl Pts',(1.33166587999994,15.2,-10.436939788));
#156966=CARTESIAN_POINT('Ctrl Pts',(1.33155489399994,15.2,-10.438747447));
#156967=CARTESIAN_POINT('Ctrl Pts',(1.33144178299994,15.2,-10.440562407));
#156968=CARTESIAN_POINT('Ctrl Pts',(1.33132653899994,15.2,-10.442384652));
#156969=CARTESIAN_POINT('Ctrl Pts',(1.33120914699994,15.2,-10.444214164));
#156970=CARTESIAN_POINT('Ctrl Pts',(1.33108959799994,15.2,-10.446050926));
#156971=CARTESIAN_POINT('Ctrl Pts',(1.33096787999994,15.2,-10.447894919));
#156972=CARTESIAN_POINT('Ctrl Pts',(1.33084398199994,15.2,-10.449746128));
#156973=CARTESIAN_POINT('Ctrl Pts',(1.33071789299994,15.2,-10.451604534));
#156974=CARTESIAN_POINT('Ctrl Pts',(1.33058960299994,15.2,-10.453470121));
#156975=CARTESIAN_POINT('Ctrl Pts',(1.33045909799994,15.2,-10.45534287));
#156976=CARTESIAN_POINT('Ctrl Pts',(1.33032637099994,15.2,-10.457222766));
#156977=CARTESIAN_POINT('Ctrl Pts',(1.33019140799994,15.2,-10.459109793));
#156978=CARTESIAN_POINT('Ctrl Pts',(1.33005419999994,15.2,-10.461003932));
#156979=CARTESIAN_POINT('Ctrl Pts',(1.32991473499994,15.2,-10.462905165));
#156980=CARTESIAN_POINT('Ctrl Pts',(1.32977300299994,15.2,-10.464813477));
#156981=CARTESIAN_POINT('Ctrl Pts',(1.32962899299994,15.2,-10.466728852));
#156982=CARTESIAN_POINT('Ctrl Pts',(1.32948269399994,15.2,-10.468651272));
#156983=CARTESIAN_POINT('Ctrl Pts',(1.32933409699994,15.2,-10.47058072));
#156984=CARTESIAN_POINT('Ctrl Pts',(1.32918318899994,15.2,-10.47251718));
#156985=CARTESIAN_POINT('Ctrl Pts',(1.32902996199994,15.2,-10.474460635));
#156986=CARTESIAN_POINT('Ctrl Pts',(1.32887440299994,15.2,-10.476411069));
#156987=CARTESIAN_POINT('Ctrl Pts',(1.32871650299994,15.2,-10.478368465));
#156988=CARTESIAN_POINT('Ctrl Pts',(1.32855625199994,15.2,-10.480332808));
#156989=CARTESIAN_POINT('Ctrl Pts',(1.32839363899994,15.2,-10.48230408));
#156990=CARTESIAN_POINT('Ctrl Pts',(1.32822865399994,15.2,-10.484282264));
#156991=CARTESIAN_POINT('Ctrl Pts',(1.32806128599994,15.2,-10.486267346));
#156992=CARTESIAN_POINT('Ctrl Pts',(1.32789152599994,15.2,-10.488259308));
#156993=CARTESIAN_POINT('Ctrl Pts',(1.32771936299994,15.2,-10.490258135));
#156994=CARTESIAN_POINT('Ctrl Pts',(1.32754478699994,15.2,-10.49226381));
#156995=CARTESIAN_POINT('Ctrl Pts',(1.32736778799994,15.2,-10.494276317));
#156996=CARTESIAN_POINT('Ctrl Pts',(1.32718835599994,15.2,-10.49629564));
#156997=CARTESIAN_POINT('Ctrl Pts',(1.32700648099994,15.2,-10.498321763));
#156998=CARTESIAN_POINT('Ctrl Pts',(1.32682215299994,15.2,-10.500354671));
#156999=CARTESIAN_POINT('Ctrl Pts',(1.32663536199994,15.2,-10.502394346));
#157000=CARTESIAN_POINT('Ctrl Pts',(1.32644609999994,15.2,-10.504440774));
#157001=CARTESIAN_POINT('Ctrl Pts',(1.32625435399994,15.2,-10.506493939));
#157002=CARTESIAN_POINT('Ctrl Pts',(1.32606011699994,15.2,-10.508553825));
#157003=CARTESIAN_POINT('Ctrl Pts',(1.32586337699994,15.2,-10.510620415));
#157004=CARTESIAN_POINT('Ctrl Pts',(1.32566412699994,15.2,-10.512693695));
#157005=CARTESIAN_POINT('Ctrl Pts',(1.32546235399994,15.2,-10.514773649));
#157006=CARTESIAN_POINT('Ctrl Pts',(1.32525805199994,15.2,-10.516860261));
#157007=CARTESIAN_POINT('Ctrl Pts',(1.32505120699994,15.2,-10.518953515));
#157008=CARTESIAN_POINT('Ctrl Pts',(1.32484181499994,15.2,-10.521053397));
#157009=CARTESIAN_POINT('Ctrl Pts',(1.32462986099994,15.2,-10.523159891));
#157010=CARTESIAN_POINT('Ctrl Pts',(1.32441533999994,15.2,-10.52527298));
#157011=CARTESIAN_POINT('Ctrl Pts',(1.32419823999994,15.2,-10.52739265));
#157012=CARTESIAN_POINT('Ctrl Pts',(1.32397855299994,15.2,-10.529518885));
#157013=CARTESIAN_POINT('Ctrl Pts',(1.32375626899994,15.2,-10.531651672));
#157014=CARTESIAN_POINT('Ctrl Pts',(1.32353137899994,15.2,-10.533790993));
#157015=CARTESIAN_POINT('Ctrl Pts',(1.32330387399994,15.2,-10.535936834));
#157016=CARTESIAN_POINT('Ctrl Pts',(1.32307374299994,15.2,-10.53808918));
#157017=CARTESIAN_POINT('Ctrl Pts',(1.32284097899994,15.2,-10.540248014));
#157018=CARTESIAN_POINT('Ctrl Pts',(1.32260557299994,15.2,-10.542413324));
#157019=CARTESIAN_POINT('Ctrl Pts',(1.32236751399994,15.2,-10.544585093));
#157020=CARTESIAN_POINT('Ctrl Pts',(1.32212679399994,15.2,-10.546763306));
#157021=CARTESIAN_POINT('Ctrl Pts',(1.32188340499994,15.2,-10.548947949));
#157022=CARTESIAN_POINT('Ctrl Pts',(1.32163733599994,15.2,-10.551139007));
#157023=CARTESIAN_POINT('Ctrl Pts',(1.32138857999994,15.2,-10.553336463));
#157024=CARTESIAN_POINT('Ctrl Pts',(1.32113712699994,15.2,-10.555540305));
#157025=CARTESIAN_POINT('Ctrl Pts',(1.32088296799994,15.2,-10.557750517));
#157026=CARTESIAN_POINT('Ctrl Pts',(1.32062609499994,15.2,-10.559967084));
#157027=CARTESIAN_POINT('Ctrl Pts',(1.32036649799994,15.2,-10.562189991));
#157028=CARTESIAN_POINT('Ctrl Pts',(1.32010416999994,15.2,-10.564419224));
#157029=CARTESIAN_POINT('Ctrl Pts',(1.31983910099994,15.2,-10.566654769));
#157030=CARTESIAN_POINT('Ctrl Pts',(1.31957128199994,15.2,-10.56889661));
#157031=CARTESIAN_POINT('Ctrl Pts',(1.31930070599994,15.2,-10.571144734));
#157032=CARTESIAN_POINT('Ctrl Pts',(1.31902736199994,15.2,-10.573399125));
#157033=CARTESIAN_POINT('Ctrl Pts',(1.31875124399994,15.2,-10.575659769));
#157034=CARTESIAN_POINT('Ctrl Pts',(1.31847234299994,15.2,-10.577926652));
#157035=CARTESIAN_POINT('Ctrl Pts',(1.31819064899994,15.2,-10.580199758));
#157036=CARTESIAN_POINT('Ctrl Pts',(1.31790615399994,15.2,-10.582479074));
#157037=CARTESIAN_POINT('Ctrl Pts',(1.31761885099994,15.2,-10.584764587));
#157038=CARTESIAN_POINT('Ctrl Pts',(1.31732872999994,15.2,-10.58705628));
#157039=CARTESIAN_POINT('Ctrl Pts',(1.31703578199994,15.2,-10.58935414));
#157040=CARTESIAN_POINT('Ctrl Pts',(1.31674000099994,15.2,-10.591658153));
#157041=CARTESIAN_POINT('Ctrl Pts',(1.31644137799994,15.2,-10.593968305));
#157042=CARTESIAN_POINT('Ctrl Pts',(1.31613990399994,15.2,-10.59628458));
#157043=CARTESIAN_POINT('Ctrl Pts',(1.31583557099994,15.2,-10.598606966));
#157044=CARTESIAN_POINT('Ctrl Pts',(1.31552837099994,15.2,-10.600935449));
#157045=CARTESIAN_POINT('Ctrl Pts',(1.31521829599994,15.2,-10.603270013));
#157046=CARTESIAN_POINT('Ctrl Pts',(1.31490533699994,15.2,-10.605610646));
#157047=CARTESIAN_POINT('Ctrl Pts',(1.31458948699994,15.2,-10.607957333));
#157048=CARTESIAN_POINT('Ctrl Pts',(1.31427073799994,15.2,-10.61031006));
#157049=CARTESIAN_POINT('Ctrl Pts',(1.31394908099994,15.2,-10.612668813));
#157050=CARTESIAN_POINT('Ctrl Pts',(1.31362450899994,15.2,-10.615033578));
#157051=CARTESIAN_POINT('Ctrl Pts',(1.31329701299994,15.2,-10.617404343));
#157052=CARTESIAN_POINT('Ctrl Pts',(1.31296658599994,15.2,-10.619781092));
#157053=CARTESIAN_POINT('Ctrl Pts',(1.31263321999994,15.2,-10.622163812));
#157054=CARTESIAN_POINT('Ctrl Pts',(1.31229690599994,15.2,-10.62455249));
#157055=CARTESIAN_POINT('Ctrl Pts',(1.31195763899994,15.2,-10.62694711));
#157056=CARTESIAN_POINT('Ctrl Pts',(1.31161540699994,15.2,-10.629347661));
#157057=CARTESIAN_POINT('Ctrl Pts',(1.31127020599994,15.2,-10.631754128));
#157058=CARTESIAN_POINT('Ctrl Pts',(1.31092202599994,15.2,-10.634166498));
#157059=CARTESIAN_POINT('Ctrl Pts',(1.31057086099994,15.2,-10.636584756));
#157060=CARTESIAN_POINT('Ctrl Pts',(1.31021670199994,15.2,-10.639008891));
#157061=CARTESIAN_POINT('Ctrl Pts',(1.30985954199994,15.2,-10.641438888));
#157062=CARTESIAN_POINT('Ctrl Pts',(1.30949937299994,15.2,-10.643874733));
#157063=CARTESIAN_POINT('Ctrl Pts',(1.30913618799994,15.2,-10.646316414));
#157064=CARTESIAN_POINT('Ctrl Pts',(1.30876997899994,15.2,-10.648763916));
#157065=CARTESIAN_POINT('Ctrl Pts',(1.30840073799994,15.2,-10.651217227));
#157066=CARTESIAN_POINT('Ctrl Pts',(1.30802845799994,15.2,-10.653676332));
#157067=CARTESIAN_POINT('Ctrl Pts',(1.30765313299994,15.2,-10.65614122));
#157068=CARTESIAN_POINT('Ctrl Pts',(1.30727475299994,15.2,-10.658611877));
#157069=CARTESIAN_POINT('Ctrl Pts',(1.30689331299994,15.2,-10.661088288));
#157070=CARTESIAN_POINT('Ctrl Pts',(1.30650880299994,15.2,-10.663570441));
#157071=CARTESIAN_POINT('Ctrl Pts',(1.30612121799994,15.2,-10.666058323));
#157072=CARTESIAN_POINT('Ctrl Pts',(1.30573054999994,15.2,-10.668551921));
#157073=CARTESIAN_POINT('Ctrl Pts',(1.30533679099994,15.2,-10.671051222));
#157074=CARTESIAN_POINT('Ctrl Pts',(1.30493993399994,15.2,-10.673556212));
#157075=CARTESIAN_POINT('Ctrl Pts',(1.30453997299994,15.2,-10.676066879));
#157076=CARTESIAN_POINT('Ctrl Pts',(1.30413689999994,15.2,-10.678583208));
#157077=CARTESIAN_POINT('Ctrl Pts',(1.30373070599994,15.2,-10.681105188));
#157078=CARTESIAN_POINT('Ctrl Pts',(1.30332138799994,15.2,-10.683632806));
#157079=CARTESIAN_POINT('Ctrl Pts',(1.30290893499994,15.2,-10.686166048));
#157080=CARTESIAN_POINT('Ctrl Pts',(1.30249334099994,15.2,-10.688704902));
#157081=CARTESIAN_POINT('Ctrl Pts',(1.30207460099994,15.2,-10.691249355));
#157082=CARTESIAN_POINT('Ctrl Pts',(1.30165270499994,15.2,-10.693799393));
#157083=CARTESIAN_POINT('Ctrl Pts',(1.30122764799994,15.2,-10.696355005));
#157084=CARTESIAN_POINT('Ctrl Pts',(1.30079942299994,15.2,-10.698916176));
#157085=CARTESIAN_POINT('Ctrl Pts',(1.30036802199994,15.2,-10.701482895));
#157086=CARTESIAN_POINT('Ctrl Pts',(1.29993343799994,15.2,-10.70405515));
#157087=CARTESIAN_POINT('Ctrl Pts',(1.29949566599994,15.2,-10.706632926));
#157088=CARTESIAN_POINT('Ctrl Pts',(1.29905469599994,15.2,-10.70921621));
#157089=CARTESIAN_POINT('Ctrl Pts',(1.29861052399994,15.2,-10.711804993));
#157090=CARTESIAN_POINT('Ctrl Pts',(1.29816314199994,15.2,-10.714399259));
#157091=CARTESIAN_POINT('Ctrl Pts',(1.29771254399994,15.2,-10.716998997));
#157092=CARTESIAN_POINT('Ctrl Pts',(1.29725872199994,15.2,-10.719604194));
#157093=CARTESIAN_POINT('Ctrl Pts',(1.29680167099994,15.2,-10.722214836));
#157094=CARTESIAN_POINT('Ctrl Pts',(1.29634138199994,15.2,-10.724830913));
#157095=CARTESIAN_POINT('Ctrl Pts',(1.29587784999994,15.2,-10.727452411));
#157096=CARTESIAN_POINT('Ctrl Pts',(1.29541106899994,15.2,-10.730079319));
#157097=CARTESIAN_POINT('Ctrl Pts',(1.29494102999994,15.2,-10.732711622));
#157098=CARTESIAN_POINT('Ctrl Pts',(1.29446772899994,15.2,-10.73534931));
#157099=CARTESIAN_POINT('Ctrl Pts',(1.29399115799994,15.2,-10.737992369));
#157100=CARTESIAN_POINT('Ctrl Pts',(1.29351130999994,15.2,-10.740640788));
#157101=CARTESIAN_POINT('Ctrl Pts',(1.29302817899994,15.2,-10.743294554));
#157102=CARTESIAN_POINT('Ctrl Pts',(1.29254175999994,15.2,-10.745953656));
#157103=CARTESIAN_POINT('Ctrl Pts',(1.29205204299994,15.2,-10.748618079));
#157104=CARTESIAN_POINT('Ctrl Pts',(1.29155902499994,15.2,-10.751287813));
#157105=CARTESIAN_POINT('Ctrl Pts',(1.29106269899994,15.2,-10.753962844));
#157106=CARTESIAN_POINT('Ctrl Pts',(1.29056305799994,15.2,-10.756643162));
#157107=CARTESIAN_POINT('Ctrl Pts',(1.29006009599994,15.2,-10.759328754));
#157108=CARTESIAN_POINT('Ctrl Pts',(1.28955380499994,15.2,-10.762019607));
#157109=CARTESIAN_POINT('Ctrl Pts',(1.28904418099994,15.2,-10.764715709));
#157110=CARTESIAN_POINT('Ctrl Pts',(1.28853121599994,15.2,-10.767417049));
#157111=CARTESIAN_POINT('Ctrl Pts',(1.28801490399994,15.2,-10.770123614));
#157112=CARTESIAN_POINT('Ctrl Pts',(1.28749524099994,15.2,-10.772835393));
#157113=CARTESIAN_POINT('Ctrl Pts',(1.28697221699994,15.2,-10.775552372));
#157114=CARTESIAN_POINT('Ctrl Pts',(1.28644582999994,15.2,-10.778274541));
#157115=CARTESIAN_POINT('Ctrl Pts',(1.28591606999994,15.2,-10.781001888));
#157116=CARTESIAN_POINT('Ctrl Pts',(1.28538293299994,15.2,-10.7837344));
#157117=CARTESIAN_POINT('Ctrl Pts',(1.28484641299994,15.2,-10.786472067));
#157118=CARTESIAN_POINT('Ctrl Pts',(1.28430650299994,15.2,-10.789214873));
#157119=CARTESIAN_POINT('Ctrl Pts',(1.28376319699994,15.2,-10.791962811));
#157120=CARTESIAN_POINT('Ctrl Pts',(1.28321648999994,15.2,-10.794715865));
#157121=CARTESIAN_POINT('Ctrl Pts',(1.28266637399994,15.2,-10.797474026));
#157122=CARTESIAN_POINT('Ctrl Pts',(1.28211284599994,15.2,-10.800237282));
#157123=CARTESIAN_POINT('Ctrl Pts',(1.28155589699994,15.2,-10.80300562));
#157124=CARTESIAN_POINT('Ctrl Pts',(1.28099552199994,15.2,-10.805779028));
#157125=CARTESIAN_POINT('Ctrl Pts',(1.28043171499994,15.2,-10.808557497));
#157126=CARTESIAN_POINT('Ctrl Pts',(1.27986447099994,15.2,-10.811341012));
#157127=CARTESIAN_POINT('Ctrl Pts',(1.27929378499994,15.2,-10.814129563));
#157128=CARTESIAN_POINT('Ctrl Pts',(1.27871964799994,15.2,-10.816923139));
#157129=CARTESIAN_POINT('Ctrl Pts',(1.27814205599994,15.2,-10.819721726));
#157130=CARTESIAN_POINT('Ctrl Pts',(1.27756100499994,15.2,-10.822525316));
#157131=CARTESIAN_POINT('Ctrl Pts',(1.27697648499994,15.2,-10.825333894));
#157132=CARTESIAN_POINT('Ctrl Pts',(1.27638849299994,15.2,-10.828147449));
#157133=CARTESIAN_POINT('Ctrl Pts',(1.27579702299994,15.2,-10.830965973));
#157134=CARTESIAN_POINT('Ctrl Pts',(1.27520206999994,15.2,-10.833789449));
#157135=CARTESIAN_POINT('Ctrl Pts',(1.27460362599994,15.2,-10.83661787));
#157136=CARTESIAN_POINT('Ctrl Pts',(1.27400168799994,15.2,-10.839451223));
#157137=CARTESIAN_POINT('Ctrl Pts',(1.27339624799994,15.2,-10.842289496));
#157138=CARTESIAN_POINT('Ctrl Pts',(1.27278730099994,15.2,-10.845132677));
#157139=CARTESIAN_POINT('Ctrl Pts',(1.27217484299994,15.2,-10.847980757));
#157140=CARTESIAN_POINT('Ctrl Pts',(1.27155886699994,15.2,-10.850833723));
#157141=CARTESIAN_POINT('Ctrl Pts',(1.27093936699994,15.2,-10.853691563));
#157142=CARTESIAN_POINT('Ctrl Pts',(1.27031633899994,15.2,-10.856554267));
#157143=CARTESIAN_POINT('Ctrl Pts',(1.26968977599994,15.2,-10.859421825));
#157144=CARTESIAN_POINT('Ctrl Pts',(1.26905967299994,15.2,-10.862294222));
#157145=CARTESIAN_POINT('Ctrl Pts',(1.26842602399994,15.2,-10.86517145));
#157146=CARTESIAN_POINT('Ctrl Pts',(1.26778882499994,15.2,-10.868053496));
#157147=CARTESIAN_POINT('Ctrl Pts',(1.26714806899994,15.2,-10.870940349));
#157148=CARTESIAN_POINT('Ctrl Pts',(1.26650375199994,15.2,-10.873831999));
#157149=CARTESIAN_POINT('Ctrl Pts',(1.26585586699994,15.2,-10.876728433));
#157150=CARTESIAN_POINT('Ctrl Pts',(1.26520440999994,15.2,-10.879629641));
#157151=CARTESIAN_POINT('Ctrl Pts',(1.26454937499994,15.2,-10.882535612));
#157152=CARTESIAN_POINT('Ctrl Pts',(1.26389075699994,15.2,-10.885446335));
#157153=CARTESIAN_POINT('Ctrl Pts',(1.26322855099994,15.2,-10.888361798));
#157154=CARTESIAN_POINT('Ctrl Pts',(1.26256274999994,15.2,-10.89128199));
#157155=CARTESIAN_POINT('Ctrl Pts',(1.26189334999994,15.2,-10.894206901));
#157156=CARTESIAN_POINT('Ctrl Pts',(1.26122034599994,15.2,-10.89713652));
#157157=CARTESIAN_POINT('Ctrl Pts',(1.26054373299994,15.2,-10.900070834));
#157158=CARTESIAN_POINT('Ctrl Pts',(1.25986350399994,15.2,-10.903009834));
#157159=CARTESIAN_POINT('Ctrl Pts',(1.25917965599994,15.2,-10.905953509));
#157160=CARTESIAN_POINT('Ctrl Pts',(1.25849218299994,15.2,-10.908901847));
#157161=CARTESIAN_POINT('Ctrl Pts',(1.25780107799994,15.2,-10.911854838));
#157162=CARTESIAN_POINT('Ctrl Pts',(1.25710633899994,15.2,-10.91481247));
#157163=CARTESIAN_POINT('Ctrl Pts',(1.25640795899994,15.2,-10.917774733));
#157164=CARTESIAN_POINT('Ctrl Pts',(1.25570593399994,15.2,-10.920741616));
#157165=CARTESIAN_POINT('Ctrl Pts',(1.25500025699994,15.2,-10.923713108));
#157166=CARTESIAN_POINT('Ctrl Pts',(1.25429092499994,15.2,-10.9266892));
#157167=CARTESIAN_POINT('Ctrl Pts',(1.25357793199994,15.2,-10.929669878));
#157168=CARTESIAN_POINT('Ctrl Pts',(1.25286127299994,15.2,-10.932655133));
#157169=CARTESIAN_POINT('Ctrl Pts',(1.25214094299994,15.2,-10.935644954));
#157170=CARTESIAN_POINT('Ctrl Pts',(1.25141693799994,15.2,-10.93863933));
#157171=CARTESIAN_POINT('Ctrl Pts',(1.25068925199994,15.2,-10.941638251));
#157172=CARTESIAN_POINT('Ctrl Pts',(1.24995787899994,15.2,-10.944641705));
#157173=CARTESIAN_POINT('Ctrl Pts',(1.24922281699994,15.2,-10.947649684));
#157174=CARTESIAN_POINT('Ctrl Pts',(1.24848405899994,15.2,-10.950662174));
#157175=CARTESIAN_POINT('Ctrl Pts',(1.24774159999994,15.2,-10.953679166));
#157176=CARTESIAN_POINT('Ctrl Pts',(1.24699543599994,15.2,-10.95670065));
#157177=CARTESIAN_POINT('Ctrl Pts',(1.24624556199994,15.2,-10.959726614));
#157178=CARTESIAN_POINT('Ctrl Pts',(1.24549197299994,15.2,-10.962757048));
#157179=CARTESIAN_POINT('Ctrl Pts',(1.24473466399994,15.2,-10.965791941));
#157180=CARTESIAN_POINT('Ctrl Pts',(1.24397362999994,15.2,-10.968831284));
#157181=CARTESIAN_POINT('Ctrl Pts',(1.24320886799994,15.2,-10.971875066));
#157182=CARTESIAN_POINT('Ctrl Pts',(1.24244037099994,15.2,-10.974923275));
#157183=CARTESIAN_POINT('Ctrl Pts',(1.24166813499994,15.2,-10.977975901));
#157184=CARTESIAN_POINT('Ctrl Pts',(1.24089215599994,15.2,-10.981032935));
#157185=CARTESIAN_POINT('Ctrl Pts',(1.24011242899994,15.2,-10.984094365));
#157186=CARTESIAN_POINT('Ctrl Pts',(1.23932894799994,15.2,-10.98716018));
#157187=CARTESIAN_POINT('Ctrl Pts',(1.23854171099994,15.2,-10.990230373));
#157188=CARTESIAN_POINT('Ctrl Pts',(1.23775071099994,15.2,-10.99330493));
#157189=CARTESIAN_POINT('Ctrl Pts',(1.23695594399994,15.2,-10.996383842));
#157190=CARTESIAN_POINT('Ctrl Pts',(1.23615740499994,15.2,-10.999467099));
#157191=CARTESIAN_POINT('Ctrl Pts',(1.23535509099994,15.2,-11.002554689));
#157192=CARTESIAN_POINT('Ctrl Pts',(1.23454899599994,15.2,-11.005646604));
#157193=CARTESIAN_POINT('Ctrl Pts',(1.23373911599994,15.2,-11.008742833));
#157194=CARTESIAN_POINT('Ctrl Pts',(1.23292544599995,15.2,-11.011843364));
#157195=CARTESIAN_POINT('Ctrl Pts',(1.23210798199994,15.2,-11.01494819));
#157196=CARTESIAN_POINT('Ctrl Pts',(1.23128671899994,15.2,-11.018057297));
#157197=CARTESIAN_POINT('Ctrl Pts',(1.23046165299994,15.2,-11.021170677));
#157198=CARTESIAN_POINT('Ctrl Pts',(1.22963277899994,15.2,-11.024288319));
#157199=CARTESIAN_POINT('Ctrl Pts',(1.22880009299994,15.2,-11.027410214));
#157200=CARTESIAN_POINT('Ctrl Pts',(1.22796359099994,15.2,-11.030536351));
#157201=CARTESIAN_POINT('Ctrl Pts',(1.22712326699994,15.2,-11.033666719));
#157202=CARTESIAN_POINT('Ctrl Pts',(1.22627911799994,15.2,-11.036801309));
#157203=CARTESIAN_POINT('Ctrl Pts',(1.22543113999994,15.2,-11.03994011));
#157204=CARTESIAN_POINT('Ctrl Pts',(1.22457932699994,15.2,-11.043083114));
#157205=CARTESIAN_POINT('Ctrl Pts',(1.22372367599994,15.2,-11.046230309));
#157206=CARTESIAN_POINT('Ctrl Pts',(1.22286418199994,15.2,-11.049381684));
#157207=CARTESIAN_POINT('Ctrl Pts',(1.22200084099994,15.2,-11.052537231));
#157208=CARTESIAN_POINT('Ctrl Pts',(1.22113364899994,15.2,-11.055696939));
#157209=CARTESIAN_POINT('Ctrl Pts',(1.22026259999994,15.2,-11.058860798));
#157210=CARTESIAN_POINT('Ctrl Pts',(1.21938769199994,15.2,-11.062028798));
#157211=CARTESIAN_POINT('Ctrl Pts',(1.21850891999994,15.2,-11.06520093));
#157212=CARTESIAN_POINT('Ctrl Pts',(1.21762627899994,15.2,-11.068377182));
#157213=CARTESIAN_POINT('Ctrl Pts',(1.21673976599994,15.2,-11.071557546));
#157214=CARTESIAN_POINT('Ctrl Pts',(1.21584937499994,15.2,-11.074742011));
#157215=CARTESIAN_POINT('Ctrl Pts',(1.21495510399994,15.2,-11.077930567));
#157216=CARTESIAN_POINT('Ctrl Pts',(1.21405694699994,15.2,-11.081123205));
#157217=CARTESIAN_POINT('Ctrl Pts',(1.21315490199994,15.2,-11.084319915));
#157218=CARTESIAN_POINT('Ctrl Pts',(1.21224896299994,15.2,-11.087520685));
#157219=CARTESIAN_POINT('Ctrl Pts',(1.21133912499995,15.2,-11.090725508));
#157220=CARTESIAN_POINT('Ctrl Pts',(1.21042538699994,15.2,-11.093934372));
#157221=CARTESIAN_POINT('Ctrl Pts',(1.20950774199994,15.2,-11.09714727));
#157222=CARTESIAN_POINT('Ctrl Pts',(1.20858618699994,15.2,-11.100364189));
#157223=CARTESIAN_POINT('Ctrl Pts',(1.20766071899994,15.2,-11.103585121));
#157224=CARTESIAN_POINT('Ctrl Pts',(1.20673133299994,15.2,-11.106810055));
#157225=CARTESIAN_POINT('Ctrl Pts',(1.20579802499994,15.2,-11.110038983));
#157226=CARTESIAN_POINT('Ctrl Pts',(1.20486078999994,15.2,-11.113271894));
#157227=CARTESIAN_POINT('Ctrl Pts',(1.20391962699994,15.2,-11.116508778));
#157228=CARTESIAN_POINT('Ctrl Pts',(1.20297452899994,15.2,-11.119749625));
#157229=CARTESIAN_POINT('Ctrl Pts',(1.20202549299994,15.2,-11.122994428));
#157230=CARTESIAN_POINT('Ctrl Pts',(1.20107251499994,15.2,-11.126243174));
#157231=CARTESIAN_POINT('Ctrl Pts',(1.20011559099995,15.2,-11.129495855));
#157232=CARTESIAN_POINT('Ctrl Pts',(1.19915471699994,15.2,-11.132752462));
#157233=CARTESIAN_POINT('Ctrl Pts',(1.19818989099994,15.2,-11.136012983));
#157234=CARTESIAN_POINT('Ctrl Pts',(1.19722110599994,15.2,-11.139277411));
#157235=CARTESIAN_POINT('Ctrl Pts',(1.19624835999994,15.2,-11.142545735));
#157236=CARTESIAN_POINT('Ctrl Pts',(1.19527164899994,15.2,-11.145817945));
#157237=CARTESIAN_POINT('Ctrl Pts',(1.19429096799994,15.2,-11.149094033));
#157238=CARTESIAN_POINT('Ctrl Pts',(1.19330631499994,15.2,-11.152373988));
#157239=CARTESIAN_POINT('Ctrl Pts',(1.19231768599994,15.2,-11.155657801));
#157240=CARTESIAN_POINT('Ctrl Pts',(1.19132507499994,15.2,-11.158945462));
#157241=CARTESIAN_POINT('Ctrl Pts',(1.19032848099994,15.2,-11.162236962));
#157242=CARTESIAN_POINT('Ctrl Pts',(1.18932789799994,15.2,-11.165532292));
#157243=CARTESIAN_POINT('Ctrl Pts',(1.18832332499994,15.2,-11.168831442));
#157244=CARTESIAN_POINT('Ctrl Pts',(1.18731475499994,15.2,-11.172134402));
#157245=CARTESIAN_POINT('Ctrl Pts',(1.18630218599994,15.2,-11.175441163));
#157246=CARTESIAN_POINT('Ctrl Pts',(1.18528561399994,15.2,-11.178751715));
#157247=CARTESIAN_POINT('Ctrl Pts',(1.18426503499994,15.2,-11.18206605));
#157248=CARTESIAN_POINT('Ctrl Pts',(1.18324044599994,15.2,-11.185384157));
#157249=CARTESIAN_POINT('Ctrl Pts',(1.18221184299994,15.2,-11.188706028));
#157250=CARTESIAN_POINT('Ctrl Pts',(1.18117922299994,15.2,-11.192031652));
#157251=CARTESIAN_POINT('Ctrl Pts',(1.18014258099994,15.2,-11.195361021));
#157252=CARTESIAN_POINT('Ctrl Pts',(1.17910191399994,15.2,-11.198694125));
#157253=CARTESIAN_POINT('Ctrl Pts',(1.17805721899994,15.2,-11.202030955));
#157254=CARTESIAN_POINT('Ctrl Pts',(1.17700849199994,15.2,-11.205371503));
#157255=CARTESIAN_POINT('Ctrl Pts',(1.17595572899994,15.2,-11.208715756));
#157256=CARTESIAN_POINT('Ctrl Pts',(1.17489892699994,15.2,-11.212063708));
#157257=CARTESIAN_POINT('Ctrl Pts',(1.17383808199994,15.2,-11.215415349));
#157258=CARTESIAN_POINT('Ctrl Pts',(1.17277319199994,15.2,-11.218770669));
#157259=CARTESIAN_POINT('Ctrl Pts',(1.17170425099994,15.2,-11.222129659));
#157260=CARTESIAN_POINT('Ctrl Pts',(1.17063125699994,15.2,-11.22549231));
#157261=CARTESIAN_POINT('Ctrl Pts',(1.16955420599994,15.2,-11.228858612));
#157262=CARTESIAN_POINT('Ctrl Pts',(1.16847309399994,15.2,-11.232228557));
#157263=CARTESIAN_POINT('Ctrl Pts',(1.16738791999994,15.2,-11.235602136));
#157264=CARTESIAN_POINT('Ctrl Pts',(1.16629867699995,15.2,-11.238979338));
#157265=CARTESIAN_POINT('Ctrl Pts',(1.16520536399994,15.2,-11.242360155));
#157266=CARTESIAN_POINT('Ctrl Pts',(1.16410797799994,15.2,-11.245744578));
#157267=CARTESIAN_POINT('Ctrl Pts',(1.16300651299994,15.2,-11.249132598));
#157268=CARTESIAN_POINT('Ctrl Pts',(1.16190096699994,15.2,-11.252524204));
#157269=CARTESIAN_POINT('Ctrl Pts',(1.16079133799994,15.2,-11.25591939));
#157270=CARTESIAN_POINT('Ctrl Pts',(1.15967762099994,15.2,-11.259318144));
#157271=CARTESIAN_POINT('Ctrl Pts',(1.15855981299994,15.2,-11.262720459));
#157272=CARTESIAN_POINT('Ctrl Pts',(1.15743790999994,15.2,-11.266126325));
#157273=CARTESIAN_POINT('Ctrl Pts',(1.15631190999994,15.2,-11.269535732));
#157274=CARTESIAN_POINT('Ctrl Pts',(1.15518180899994,15.2,-11.272948673));
#157275=CARTESIAN_POINT('Ctrl Pts',(1.15404760399994,15.2,-11.276365138));
#157276=CARTESIAN_POINT('Ctrl Pts',(1.15290929199994,15.2,-11.279785118));
#157277=CARTESIAN_POINT('Ctrl Pts',(1.15176686799994,15.2,-11.283208603));
#157278=CARTESIAN_POINT('Ctrl Pts',(1.15062032899994,15.2,-11.286635586));
#157279=CARTESIAN_POINT('Ctrl Pts',(1.14946967399994,15.2,-11.290066057));
#157280=CARTESIAN_POINT('Ctrl Pts',(1.14831489899994,15.2,-11.293500006));
#157281=CARTESIAN_POINT('Ctrl Pts',(1.14715599899994,15.2,-11.296937426));
#157282=CARTESIAN_POINT('Ctrl Pts',(1.14599297199994,15.2,-11.300378306));
#157283=CARTESIAN_POINT('Ctrl Pts',(1.14482581499994,15.2,-11.303822638));
#157284=CARTESIAN_POINT('Ctrl Pts',(1.14365452599994,15.2,-11.307270414));
#157285=CARTESIAN_POINT('Ctrl Pts',(1.14247909799994,15.2,-11.310721625));
#157286=CARTESIAN_POINT('Ctrl Pts',(1.14129953199994,15.2,-11.31417626));
#157287=CARTESIAN_POINT('Ctrl Pts',(1.14011582299994,15.2,-11.317634312));
#157288=CARTESIAN_POINT('Ctrl Pts',(1.13892796699994,15.2,-11.321095772));
#157289=CARTESIAN_POINT('Ctrl Pts',(1.13773596199994,15.2,-11.324560631));
#157290=CARTESIAN_POINT('Ctrl Pts',(1.13653980599994,15.2,-11.32802888));
#157291=CARTESIAN_POINT('Ctrl Pts',(1.13533949399994,15.2,-11.331500509));
#157292=CARTESIAN_POINT('Ctrl Pts',(1.13413502299994,15.2,-11.334975512));
#157293=CARTESIAN_POINT('Ctrl Pts',(1.13292639099994,15.2,-11.338453878));
#157294=CARTESIAN_POINT('Ctrl Pts',(1.13171359399994,15.2,-11.341935598));
#157295=CARTESIAN_POINT('Ctrl Pts',(1.13049662999994,15.2,-11.345420665));
#157296=CARTESIAN_POINT('Ctrl Pts',(1.12927549399994,15.2,-11.348909068));
#157297=CARTESIAN_POINT('Ctrl Pts',(1.12805018499994,15.2,-11.3524008));
#157298=CARTESIAN_POINT('Ctrl Pts',(1.12682069999994,15.2,-11.355895851));
#157299=CARTESIAN_POINT('Ctrl Pts',(1.12558703399994,15.2,-11.359394214));
#157300=CARTESIAN_POINT('Ctrl Pts',(1.12434918699994,15.2,-11.36289588));
#157301=CARTESIAN_POINT('Ctrl Pts',(1.12310715399994,15.2,-11.366400839));
#157302=CARTESIAN_POINT('Ctrl Pts',(1.12186093199994,15.2,-11.369909084));
#157303=CARTESIAN_POINT('Ctrl Pts',(1.12061051899994,15.2,-11.373420606));
#157304=CARTESIAN_POINT('Ctrl Pts',(1.11935591099994,15.2,-11.376935393));
#157305=CARTESIAN_POINT('Ctrl Pts',(1.11809710599994,15.2,-11.38045344));
#157306=CARTESIAN_POINT('Ctrl Pts',(1.11683409999994,15.2,-11.383974735));
#157307=CARTESIAN_POINT('Ctrl Pts',(1.11556688999994,15.2,-11.387499272));
#157308=CARTESIAN_POINT('Ctrl Pts',(1.11429547399994,15.2,-11.39102704));
#157309=CARTESIAN_POINT('Ctrl Pts',(1.11301984899994,15.2,-11.394558034));
#157310=CARTESIAN_POINT('Ctrl Pts',(1.11174001299994,15.2,-11.398092244));
#157311=CARTESIAN_POINT('Ctrl Pts',(1.11045596299994,15.2,-11.401629665));
#157312=CARTESIAN_POINT('Ctrl Pts',(1.10916769599994,15.2,-11.405170286));
#157313=CARTESIAN_POINT('Ctrl Pts',(1.10787520999994,15.2,-11.408714099));
#157314=CARTESIAN_POINT('Ctrl Pts',(1.10657849999994,15.2,-11.412261095));
#157315=CARTESIAN_POINT('Ctrl Pts',(1.10527756399994,15.2,-11.415811262));
#157316=CARTESIAN_POINT('Ctrl Pts',(1.10397239799994,15.2,-11.419364591));
#157317=CARTESIAN_POINT('Ctrl Pts',(1.10266299899994,15.2,-11.422921069));
#157318=CARTESIAN_POINT('Ctrl Pts',(1.10134936299994,15.2,-11.426480691));
#157319=CARTESIAN_POINT('Ctrl Pts',(1.10003148899994,15.2,-11.430043446));
#157320=CARTESIAN_POINT('Ctrl Pts',(1.09870937299994,15.2,-11.433609328));
#157321=CARTESIAN_POINT('Ctrl Pts',(1.09738301599994,15.2,-11.437178335));
#157322=CARTESIAN_POINT('Ctrl Pts',(1.09605241599994,15.2,-11.440750465));
#157323=CARTESIAN_POINT('Ctrl Pts',(1.09498454299994,15.2,-11.443610664));
#157324=CARTESIAN_POINT('Ctrl Pts',(1.09418172899994,15.2,-11.445757219));
#157325=CARTESIAN_POINT('Ctrl Pts',(1.09364566999994,15.2,-11.447188878));
#157326=CARTESIAN_POINT('Ctrl Pts',(1.09337742899994,15.2,-11.447904865));
#157327=CARTESIAN_POINT('Origin',(-5.66257110645729E-14,15.2,-1.77635683940025E-14));
#157328=CARTESIAN_POINT('',(1.76496130699994,15.2,-10.223773109));
#157329=CARTESIAN_POINT('',(1.76496130699994,12.2,-10.223773109));
#157330=CARTESIAN_POINT('',(1.76496130699994,15.2,-10.223773109));
#157331=CARTESIAN_POINT('Origin',(-5.66257110645729E-14,12.2,-1.77635683940025E-14));
#157332=CARTESIAN_POINT('Origin',(-5.66257110645729E-14,15.2,-1.77635683940025E-14));
#157333=CARTESIAN_POINT('Origin',(-5.66257110645729E-14,15.2,-1.77635683940025E-14));
#157334=CARTESIAN_POINT('',(2.33718477799994,15.2,-11.259998548));
#157335=CARTESIAN_POINT('',(2.71145515299994,15.2,-11.175777867));
#157336=CARTESIAN_POINT('Origin',(-5.66257110645729E-14,15.2,-1.77635683940025E-14));
#157337=CARTESIAN_POINT('',(2.71145515299994,12.2,-11.175777867));
#157338=CARTESIAN_POINT('',(2.71145515299994,15.2,-11.175777867));
#157339=CARTESIAN_POINT('',(2.33718477799994,12.2,-11.259998548));
#157340=CARTESIAN_POINT('Origin',(-5.66257110645729E-14,12.2,-1.77635683940025E-14));
#157341=CARTESIAN_POINT('',(2.33718477799994,15.2,-11.259998548));
#157342=CARTESIAN_POINT('Ctrl Pts',(2.71145515299994,15.2,-11.175777867));
#157343=CARTESIAN_POINT('Ctrl Pts',(2.71145515299994,11.6,-11.175777867));
#157344=CARTESIAN_POINT('Ctrl Pts',(2.71161876799995,15.2,-11.175030995));
#157345=CARTESIAN_POINT('Ctrl Pts',(2.71161876799995,11.6,-11.175030995));
#157346=CARTESIAN_POINT('Ctrl Pts',(2.71194562399995,15.2,-11.173537618));
#157347=CARTESIAN_POINT('Ctrl Pts',(2.71194562399995,11.6,-11.173537618));
#157348=CARTESIAN_POINT('Ctrl Pts',(2.71243477999994,15.2,-11.17129866));
#157349=CARTESIAN_POINT('Ctrl Pts',(2.71243477999994,11.6,-11.17129866));
#157350=CARTESIAN_POINT('Ctrl Pts',(2.71308473599994,15.2,-11.168315598));
#157351=CARTESIAN_POINT('Ctrl Pts',(2.71308473599994,11.6,-11.168315598));
#157352=CARTESIAN_POINT('Ctrl Pts',(2.71389342499994,15.2,-11.164590464));
#157353=CARTESIAN_POINT('Ctrl Pts',(2.71389342499994,11.6,-11.164590464));
#157354=CARTESIAN_POINT('Ctrl Pts',(2.71469835899994,15.2,-11.160869024));
#157355=CARTESIAN_POINT('Ctrl Pts',(2.71469835899994,11.6,-11.160869024));
#157356=CARTESIAN_POINT('Ctrl Pts',(2.71549953799994,15.2,-11.15715128));
#157357=CARTESIAN_POINT('Ctrl Pts',(2.71549953799994,11.6,-11.15715128));
#157358=CARTESIAN_POINT('Ctrl Pts',(2.71629696599994,15.2,-11.153437236));
#157359=CARTESIAN_POINT('Ctrl Pts',(2.71629696599994,11.6,-11.153437236));
#157360=CARTESIAN_POINT('Ctrl Pts',(2.71709064399994,15.2,-11.149726897));
#157361=CARTESIAN_POINT('Ctrl Pts',(2.71709064399994,11.6,-11.149726897));
#157362=CARTESIAN_POINT('Ctrl Pts',(2.71788057599994,15.2,-11.146020271));
#157363=CARTESIAN_POINT('Ctrl Pts',(2.71788057599994,11.6,-11.146020271));
#157364=CARTESIAN_POINT('Ctrl Pts',(2.71866676599994,15.2,-11.142317365));
#157365=CARTESIAN_POINT('Ctrl Pts',(2.71866676599994,11.6,-11.142317365));
#157366=CARTESIAN_POINT('Ctrl Pts',(2.71944921799995,15.2,-11.138618191));
#157367=CARTESIAN_POINT('Ctrl Pts',(2.71944921799995,11.6,-11.138618191));
#157368=CARTESIAN_POINT('Ctrl Pts',(2.72022793899994,15.2,-11.134922758));
#157369=CARTESIAN_POINT('Ctrl Pts',(2.72022793899994,11.6,-11.134922758));
#157370=CARTESIAN_POINT('Ctrl Pts',(2.72100293299995,15.2,-11.131231076));
#157371=CARTESIAN_POINT('Ctrl Pts',(2.72100293299995,11.6,-11.131231076));
#157372=CARTESIAN_POINT('Ctrl Pts',(2.72177420399994,15.2,-11.127543154));
#157373=CARTESIAN_POINT('Ctrl Pts',(2.72177420399994,11.6,-11.127543154));
#157374=CARTESIAN_POINT('Ctrl Pts',(2.72254175699994,15.2,-11.123859));
#157375=CARTESIAN_POINT('Ctrl Pts',(2.72254175699994,11.6,-11.123859));
#157376=CARTESIAN_POINT('Ctrl Pts',(2.72330559599995,15.2,-11.120178623));
#157377=CARTESIAN_POINT('Ctrl Pts',(2.72330559599995,11.6,-11.120178623));
#157378=CARTESIAN_POINT('Ctrl Pts',(2.72406572399994,15.2,-11.11650203));
#157379=CARTESIAN_POINT('Ctrl Pts',(2.72406572399994,11.6,-11.11650203));
#157380=CARTESIAN_POINT('Ctrl Pts',(2.72482214499994,15.2,-11.112829226));
#157381=CARTESIAN_POINT('Ctrl Pts',(2.72482214499994,11.6,-11.112829226));
#157382=CARTESIAN_POINT('Ctrl Pts',(2.72557486199994,15.2,-11.109160223));
#157383=CARTESIAN_POINT('Ctrl Pts',(2.72557486199994,11.6,-11.109160223));
#157384=CARTESIAN_POINT('Ctrl Pts',(2.72632387999994,15.2,-11.105495024));
#157385=CARTESIAN_POINT('Ctrl Pts',(2.72632387999994,11.6,-11.105495024));
#157386=CARTESIAN_POINT('Ctrl Pts',(2.72706920299994,15.2,-11.10183364));
#157387=CARTESIAN_POINT('Ctrl Pts',(2.72706920299994,11.6,-11.10183364));
#157388=CARTESIAN_POINT('Ctrl Pts',(2.72781083399994,15.2,-11.098176078));
#157389=CARTESIAN_POINT('Ctrl Pts',(2.72781083399994,11.6,-11.098176078));
#157390=CARTESIAN_POINT('Ctrl Pts',(2.72854877799994,15.2,-11.094522347));
#157391=CARTESIAN_POINT('Ctrl Pts',(2.72854877799994,11.6,-11.094522347));
#157392=CARTESIAN_POINT('Ctrl Pts',(2.72928303999994,15.2,-11.090872455));
#157393=CARTESIAN_POINT('Ctrl Pts',(2.72928303999994,11.6,-11.090872455));
#157394=CARTESIAN_POINT('Ctrl Pts',(2.73001362299994,15.2,-11.087226412));
#157395=CARTESIAN_POINT('Ctrl Pts',(2.73001362299994,11.6,-11.087226412));
#157396=CARTESIAN_POINT('Ctrl Pts',(2.73074053199994,15.2,-11.083584223));
#157397=CARTESIAN_POINT('Ctrl Pts',(2.73074053199994,11.6,-11.083584223));
#157398=CARTESIAN_POINT('Ctrl Pts',(2.73146377099994,15.2,-11.079945899));
#157399=CARTESIAN_POINT('Ctrl Pts',(2.73146377099994,11.6,-11.079945899));
#157400=CARTESIAN_POINT('Ctrl Pts',(2.73218334399994,15.2,-11.076311448));
#157401=CARTESIAN_POINT('Ctrl Pts',(2.73218334399994,11.6,-11.076311448));
#157402=CARTESIAN_POINT('Ctrl Pts',(2.73289925699994,15.2,-11.072680878));
#157403=CARTESIAN_POINT('Ctrl Pts',(2.73289925699994,11.6,-11.072680878));
#157404=CARTESIAN_POINT('Ctrl Pts',(2.73361150999994,15.2,-11.069054196));
#157405=CARTESIAN_POINT('Ctrl Pts',(2.73361150999994,11.6,-11.069054196));
#157406=CARTESIAN_POINT('Ctrl Pts',(2.73432011199994,15.2,-11.06543141));
#157407=CARTESIAN_POINT('Ctrl Pts',(2.73432011199994,11.6,-11.06543141));
#157408=CARTESIAN_POINT('Ctrl Pts',(2.73502506399995,15.2,-11.06181253));
#157409=CARTESIAN_POINT('Ctrl Pts',(2.73502506399995,11.6,-11.06181253));
#157410=CARTESIAN_POINT('Ctrl Pts',(2.73572636999994,15.2,-11.058197563));
#157411=CARTESIAN_POINT('Ctrl Pts',(2.73572636999994,11.6,-11.058197563));
#157412=CARTESIAN_POINT('Ctrl Pts',(2.73642403699994,15.2,-11.054586516));
#157413=CARTESIAN_POINT('Ctrl Pts',(2.73642403699994,11.6,-11.054586516));
#157414=CARTESIAN_POINT('Ctrl Pts',(2.73711806699994,15.2,-11.050979401));
#157415=CARTESIAN_POINT('Ctrl Pts',(2.73711806699994,11.6,-11.050979401));
#157416=CARTESIAN_POINT('Ctrl Pts',(2.73780846499994,15.2,-11.047376223));
#157417=CARTESIAN_POINT('Ctrl Pts',(2.73780846499994,11.6,-11.047376223));
#157418=CARTESIAN_POINT('Ctrl Pts',(2.73849523599994,15.2,-11.043776991));
#157419=CARTESIAN_POINT('Ctrl Pts',(2.73849523599994,11.6,-11.043776991));
#157420=CARTESIAN_POINT('Ctrl Pts',(2.73917838399994,15.2,-11.040181714));
#157421=CARTESIAN_POINT('Ctrl Pts',(2.73917838399994,11.6,-11.040181714));
#157422=CARTESIAN_POINT('Ctrl Pts',(2.73985791299994,15.2,-11.036590401));
#157423=CARTESIAN_POINT('Ctrl Pts',(2.73985791299994,11.6,-11.036590401));
#157424=CARTESIAN_POINT('Ctrl Pts',(2.74053382699994,15.2,-11.033003059));
#157425=CARTESIAN_POINT('Ctrl Pts',(2.74053382699994,11.6,-11.033003059));
#157426=CARTESIAN_POINT('Ctrl Pts',(2.74120613199994,15.2,-11.029419697));
#157427=CARTESIAN_POINT('Ctrl Pts',(2.74120613199994,11.6,-11.029419697));
#157428=CARTESIAN_POINT('Ctrl Pts',(2.74187482999994,15.2,-11.025840322));
#157429=CARTESIAN_POINT('Ctrl Pts',(2.74187482999994,11.6,-11.025840322));
#157430=CARTESIAN_POINT('Ctrl Pts',(2.74253992699995,15.2,-11.022264944));
#157431=CARTESIAN_POINT('Ctrl Pts',(2.74253992699995,11.6,-11.022264944));
#157432=CARTESIAN_POINT('Ctrl Pts',(2.74320142799994,15.2,-11.018693571));
#157433=CARTESIAN_POINT('Ctrl Pts',(2.74320142799994,11.6,-11.018693571));
#157434=CARTESIAN_POINT('Ctrl Pts',(2.74385933599994,15.2,-11.015126211));
#157435=CARTESIAN_POINT('Ctrl Pts',(2.74385933599994,11.6,-11.015126211));
#157436=CARTESIAN_POINT('Ctrl Pts',(2.74451365599994,15.2,-11.011562873));
#157437=CARTESIAN_POINT('Ctrl Pts',(2.74451365599994,11.6,-11.011562873));
#157438=CARTESIAN_POINT('Ctrl Pts',(2.74516439099994,15.2,-11.008003563));
#157439=CARTESIAN_POINT('Ctrl Pts',(2.74516439099994,11.6,-11.008003563));
#157440=CARTESIAN_POINT('Ctrl Pts',(2.74581154899994,15.2,-11.004448293));
#157441=CARTESIAN_POINT('Ctrl Pts',(2.74581154899994,11.6,-11.004448293));
#157442=CARTESIAN_POINT('Ctrl Pts',(2.74645513199994,15.2,-11.00089707));
#157443=CARTESIAN_POINT('Ctrl Pts',(2.74645513199994,11.6,-11.00089707));
#157444=CARTESIAN_POINT('Ctrl Pts',(2.74709514399994,15.2,-10.997349902));
#157445=CARTESIAN_POINT('Ctrl Pts',(2.74709514399994,11.6,-10.997349902));
#157446=CARTESIAN_POINT('Ctrl Pts',(2.74773159199994,15.2,-10.993806797));
#157447=CARTESIAN_POINT('Ctrl Pts',(2.74773159199994,11.6,-10.993806797));
#157448=CARTESIAN_POINT('Ctrl Pts',(2.74836447799994,15.2,-10.990267766));
#157449=CARTESIAN_POINT('Ctrl Pts',(2.74836447799994,11.6,-10.990267766));
#157450=CARTESIAN_POINT('Ctrl Pts',(2.74899380799994,15.2,-10.986732814));
#157451=CARTESIAN_POINT('Ctrl Pts',(2.74899380799994,11.6,-10.986732814));
#157452=CARTESIAN_POINT('Ctrl Pts',(2.74961958599994,15.2,-10.983201952));
#157453=CARTESIAN_POINT('Ctrl Pts',(2.74961958599994,11.6,-10.983201952));
#157454=CARTESIAN_POINT('Ctrl Pts',(2.75024181599994,15.2,-10.979675187));
#157455=CARTESIAN_POINT('Ctrl Pts',(2.75024181599994,11.6,-10.979675187));
#157456=CARTESIAN_POINT('Ctrl Pts',(2.75086050399994,15.2,-10.976152529));
#157457=CARTESIAN_POINT('Ctrl Pts',(2.75086050399994,11.6,-10.976152529));
#157458=CARTESIAN_POINT('Ctrl Pts',(2.75147565299994,15.2,-10.972633984));
#157459=CARTESIAN_POINT('Ctrl Pts',(2.75147565299994,11.6,-10.972633984));
#157460=CARTESIAN_POINT('Ctrl Pts',(2.75208726999994,15.2,-10.969119563));
#157461=CARTESIAN_POINT('Ctrl Pts',(2.75208726999994,11.6,-10.969119563));
#157462=CARTESIAN_POINT('Ctrl Pts',(2.75269535799994,15.2,-10.965609275));
#157463=CARTESIAN_POINT('Ctrl Pts',(2.75269535799994,11.6,-10.965609275));
#157464=CARTESIAN_POINT('Ctrl Pts',(2.75329991999994,15.2,-10.962103125));
#157465=CARTESIAN_POINT('Ctrl Pts',(2.75329991999994,11.6,-10.962103125));
#157466=CARTESIAN_POINT('Ctrl Pts',(2.75390096499994,15.2,-10.958601125));
#157467=CARTESIAN_POINT('Ctrl Pts',(2.75390096499994,11.6,-10.958601125));
#157468=CARTESIAN_POINT('Ctrl Pts',(2.75449849399994,15.2,-10.955103283));
#157469=CARTESIAN_POINT('Ctrl Pts',(2.75449849399994,11.6,-10.955103283));
#157470=CARTESIAN_POINT('Ctrl Pts',(2.75509251299995,15.2,-10.951609607));
#157471=CARTESIAN_POINT('Ctrl Pts',(2.75509251299995,11.6,-10.951609607));
#157472=CARTESIAN_POINT('Ctrl Pts',(2.75568302799994,15.2,-10.948120104));
#157473=CARTESIAN_POINT('Ctrl Pts',(2.75568302799994,11.6,-10.948120104));
#157474=CARTESIAN_POINT('Ctrl Pts',(2.75627004099994,15.2,-10.944634786));
#157475=CARTESIAN_POINT('Ctrl Pts',(2.75627004099994,11.6,-10.944634786));
#157476=CARTESIAN_POINT('Ctrl Pts',(2.75685355899994,15.2,-10.941153659));
#157477=CARTESIAN_POINT('Ctrl Pts',(2.75685355899994,11.6,-10.941153659));
#157478=CARTESIAN_POINT('Ctrl Pts',(2.75743358399994,15.2,-10.937676732));
#157479=CARTESIAN_POINT('Ctrl Pts',(2.75743358399994,11.6,-10.937676732));
#157480=CARTESIAN_POINT('Ctrl Pts',(2.75801012499994,15.2,-10.934204015));
#157481=CARTESIAN_POINT('Ctrl Pts',(2.75801012499994,11.6,-10.934204015));
#157482=CARTESIAN_POINT('Ctrl Pts',(2.75858318399994,15.2,-10.930735515));
#157483=CARTESIAN_POINT('Ctrl Pts',(2.75858318399994,11.6,-10.930735515));
#157484=CARTESIAN_POINT('Ctrl Pts',(2.75915276499994,15.2,-10.927271242));
#157485=CARTESIAN_POINT('Ctrl Pts',(2.75915276499994,11.6,-10.927271242));
#157486=CARTESIAN_POINT('Ctrl Pts',(2.75971887499994,15.2,-10.923811204));
#157487=CARTESIAN_POINT('Ctrl Pts',(2.75971887499994,11.6,-10.923811204));
#157488=CARTESIAN_POINT('Ctrl Pts',(2.76028151899995,15.2,-10.92035541));
#157489=CARTESIAN_POINT('Ctrl Pts',(2.76028151899995,11.6,-10.92035541));
#157490=CARTESIAN_POINT('Ctrl Pts',(2.76084070099994,15.2,-10.916903868));
#157491=CARTESIAN_POINT('Ctrl Pts',(2.76084070099994,11.6,-10.916903868));
#157492=CARTESIAN_POINT('Ctrl Pts',(2.76139642499994,15.2,-10.913456588));
#157493=CARTESIAN_POINT('Ctrl Pts',(2.76139642499994,11.6,-10.913456588));
#157494=CARTESIAN_POINT('Ctrl Pts',(2.76194869599995,15.2,-10.910013578));
#157495=CARTESIAN_POINT('Ctrl Pts',(2.76194869599995,11.6,-10.910013578));
#157496=CARTESIAN_POINT('Ctrl Pts',(2.76249751999994,15.2,-10.906574846));
#157497=CARTESIAN_POINT('Ctrl Pts',(2.76249751999994,11.6,-10.906574846));
#157498=CARTESIAN_POINT('Ctrl Pts',(2.76304290199994,15.2,-10.903140401));
#157499=CARTESIAN_POINT('Ctrl Pts',(2.76304290199994,11.6,-10.903140401));
#157500=CARTESIAN_POINT('Ctrl Pts',(2.76358484599994,15.2,-10.899710254));
#157501=CARTESIAN_POINT('Ctrl Pts',(2.76358484599994,11.6,-10.899710254));
#157502=CARTESIAN_POINT('Ctrl Pts',(2.76412335699994,15.2,-10.896284411));
#157503=CARTESIAN_POINT('Ctrl Pts',(2.76412335699994,11.6,-10.896284411));
#157504=CARTESIAN_POINT('Ctrl Pts',(2.76465844099994,15.2,-10.892862882));
#157505=CARTESIAN_POINT('Ctrl Pts',(2.76465844099994,11.6,-10.892862882));
#157506=CARTESIAN_POINT('Ctrl Pts',(2.76519010299995,15.2,-10.889445675));
#157507=CARTESIAN_POINT('Ctrl Pts',(2.76519010299995,11.6,-10.889445675));
#157508=CARTESIAN_POINT('Ctrl Pts',(2.76571834699994,15.2,-10.8860328));
#157509=CARTESIAN_POINT('Ctrl Pts',(2.76571834699994,11.6,-10.8860328));
#157510=CARTESIAN_POINT('Ctrl Pts',(2.76624317799994,15.2,-10.882624265));
#157511=CARTESIAN_POINT('Ctrl Pts',(2.76624317799994,11.6,-10.882624265));
#157512=CARTESIAN_POINT('Ctrl Pts',(2.76676460199994,15.2,-10.87922008));
#157513=CARTESIAN_POINT('Ctrl Pts',(2.76676460199994,11.6,-10.87922008));
#157514=CARTESIAN_POINT('Ctrl Pts',(2.76728262299994,15.2,-10.875820251));
#157515=CARTESIAN_POINT('Ctrl Pts',(2.76728262299994,11.6,-10.875820251));
#157516=CARTESIAN_POINT('Ctrl Pts',(2.76779724699994,15.2,-10.872424791));
#157517=CARTESIAN_POINT('Ctrl Pts',(2.76779724699994,11.6,-10.872424791));
#157518=CARTESIAN_POINT('Ctrl Pts',(2.76830847799994,15.2,-10.869033706));
#157519=CARTESIAN_POINT('Ctrl Pts',(2.76830847799994,11.6,-10.869033706));
#157520=CARTESIAN_POINT('Ctrl Pts',(2.76881632299995,15.2,-10.865647005));
#157521=CARTESIAN_POINT('Ctrl Pts',(2.76881632299995,11.6,-10.865647005));
#157522=CARTESIAN_POINT('Ctrl Pts',(2.76932078499994,15.2,-10.862264698));
#157523=CARTESIAN_POINT('Ctrl Pts',(2.76932078499994,11.6,-10.862264698));
#157524=CARTESIAN_POINT('Ctrl Pts',(2.76982187099994,15.2,-10.858886794));
#157525=CARTESIAN_POINT('Ctrl Pts',(2.76982187099994,11.6,-10.858886794));
#157526=CARTESIAN_POINT('Ctrl Pts',(2.77031958499995,15.2,-10.8555133));
#157527=CARTESIAN_POINT('Ctrl Pts',(2.77031958499995,11.6,-10.8555133));
#157528=CARTESIAN_POINT('Ctrl Pts',(2.77081393199994,15.2,-10.852144228));
#157529=CARTESIAN_POINT('Ctrl Pts',(2.77081393199994,11.6,-10.852144228));
#157530=CARTESIAN_POINT('Ctrl Pts',(2.77130491799995,15.2,-10.848779584));
#157531=CARTESIAN_POINT('Ctrl Pts',(2.77130491799995,11.6,-10.848779584));
#157532=CARTESIAN_POINT('Ctrl Pts',(2.77179254699994,15.2,-10.845419378));
#157533=CARTESIAN_POINT('Ctrl Pts',(2.77179254699994,11.6,-10.845419378));
#157534=CARTESIAN_POINT('Ctrl Pts',(2.77227682599994,15.2,-10.84206362));
#157535=CARTESIAN_POINT('Ctrl Pts',(2.77227682599994,11.6,-10.84206362));
#157536=CARTESIAN_POINT('Ctrl Pts',(2.77275775999994,15.2,-10.838712319));
#157537=CARTESIAN_POINT('Ctrl Pts',(2.77275775999994,11.6,-10.838712319));
#157538=CARTESIAN_POINT('Ctrl Pts',(2.77323535199994,15.2,-10.835365482));
#157539=CARTESIAN_POINT('Ctrl Pts',(2.77323535199994,11.6,-10.835365482));
#157540=CARTESIAN_POINT('Ctrl Pts',(2.77370960899994,15.2,-10.83202312));
#157541=CARTESIAN_POINT('Ctrl Pts',(2.77370960899994,11.6,-10.83202312));
#157542=CARTESIAN_POINT('Ctrl Pts',(2.77418053799994,15.2,-10.828685241));
#157543=CARTESIAN_POINT('Ctrl Pts',(2.77418053799994,11.6,-10.828685241));
#157544=CARTESIAN_POINT('Ctrl Pts',(2.77464813999994,15.2,-10.825351854));
#157545=CARTESIAN_POINT('Ctrl Pts',(2.77464813999994,11.6,-10.825351854));
#157546=CARTESIAN_POINT('Ctrl Pts',(2.77511242499994,15.2,-10.822022969));
#157547=CARTESIAN_POINT('Ctrl Pts',(2.77511242499994,11.6,-10.822022969));
#157548=CARTESIAN_POINT('Ctrl Pts',(2.77557339499995,15.2,-10.818698595));
#157549=CARTESIAN_POINT('Ctrl Pts',(2.77557339499995,11.6,-10.818698595));
#157550=CARTESIAN_POINT('Ctrl Pts',(2.77603105699994,15.2,-10.815378739));
#157551=CARTESIAN_POINT('Ctrl Pts',(2.77603105699994,11.6,-10.815378739));
#157552=CARTESIAN_POINT('Ctrl Pts',(2.77648541599994,15.2,-10.812063413));
#157553=CARTESIAN_POINT('Ctrl Pts',(2.77648541599994,11.6,-10.812063413));
#157554=CARTESIAN_POINT('Ctrl Pts',(2.77693647799994,15.2,-10.808752624));
#157555=CARTESIAN_POINT('Ctrl Pts',(2.77693647799994,11.6,-10.808752624));
#157556=CARTESIAN_POINT('Ctrl Pts',(2.77738424599994,15.2,-10.805446382));
#157557=CARTESIAN_POINT('Ctrl Pts',(2.77738424599994,11.6,-10.805446382));
#157558=CARTESIAN_POINT('Ctrl Pts',(2.77782872899994,15.2,-10.802144697));
#157559=CARTESIAN_POINT('Ctrl Pts',(2.77782872899994,11.6,-10.802144697));
#157560=CARTESIAN_POINT('Ctrl Pts',(2.77826992999994,15.2,-10.798847577));
#157561=CARTESIAN_POINT('Ctrl Pts',(2.77826992999994,11.6,-10.798847577));
#157562=CARTESIAN_POINT('Ctrl Pts',(2.77870785499994,15.2,-10.795555031));
#157563=CARTESIAN_POINT('Ctrl Pts',(2.77870785499994,11.6,-10.795555031));
#157564=CARTESIAN_POINT('Ctrl Pts',(2.77914250899994,15.2,-10.792267068));
#157565=CARTESIAN_POINT('Ctrl Pts',(2.77914250899994,11.6,-10.792267068));
#157566=CARTESIAN_POINT('Ctrl Pts',(2.77957389999994,15.2,-10.788983698));
#157567=CARTESIAN_POINT('Ctrl Pts',(2.77957389999994,11.6,-10.788983698));
#157568=CARTESIAN_POINT('Ctrl Pts',(2.78000203099994,15.2,-10.785704931));
#157569=CARTESIAN_POINT('Ctrl Pts',(2.78000203099994,11.6,-10.785704931));
#157570=CARTESIAN_POINT('Ctrl Pts',(2.78042690799994,15.2,-10.782430775));
#157571=CARTESIAN_POINT('Ctrl Pts',(2.78042690799994,11.6,-10.782430775));
#157572=CARTESIAN_POINT('Ctrl Pts',(2.78084853699994,15.2,-10.779161239));
#157573=CARTESIAN_POINT('Ctrl Pts',(2.78084853699994,11.6,-10.779161239));
#157574=CARTESIAN_POINT('Ctrl Pts',(2.78126692299994,15.2,-10.775896332));
#157575=CARTESIAN_POINT('Ctrl Pts',(2.78126692299994,11.6,-10.775896332));
#157576=CARTESIAN_POINT('Ctrl Pts',(2.78168207299994,15.2,-10.772636066));
#157577=CARTESIAN_POINT('Ctrl Pts',(2.78168207299994,11.6,-10.772636066));
#157578=CARTESIAN_POINT('Ctrl Pts',(2.78209398999994,15.2,-10.769380447));
#157579=CARTESIAN_POINT('Ctrl Pts',(2.78209398999994,11.6,-10.769380447));
#157580=CARTESIAN_POINT('Ctrl Pts',(2.78250268299994,15.2,-10.766129486));
#157581=CARTESIAN_POINT('Ctrl Pts',(2.78250268299994,11.6,-10.766129486));
#157582=CARTESIAN_POINT('Ctrl Pts',(2.78290815499994,15.2,-10.762883192));
#157583=CARTESIAN_POINT('Ctrl Pts',(2.78290815499994,11.6,-10.762883192));
#157584=CARTESIAN_POINT('Ctrl Pts',(2.78331041399994,15.2,-10.759641574));
#157585=CARTESIAN_POINT('Ctrl Pts',(2.78331041399994,11.6,-10.759641574));
#157586=CARTESIAN_POINT('Ctrl Pts',(2.78370946199994,15.2,-10.756404642));
#157587=CARTESIAN_POINT('Ctrl Pts',(2.78370946199994,11.6,-10.756404642));
#157588=CARTESIAN_POINT('Ctrl Pts',(2.78410530899994,15.2,-10.753172404));
#157589=CARTESIAN_POINT('Ctrl Pts',(2.78410530899994,11.6,-10.753172404));
#157590=CARTESIAN_POINT('Ctrl Pts',(2.78449795899995,15.2,-10.74994487));
#157591=CARTESIAN_POINT('Ctrl Pts',(2.78449795899995,11.6,-10.74994487));
#157592=CARTESIAN_POINT('Ctrl Pts',(2.78488741699995,15.2,-10.746722051));
#157593=CARTESIAN_POINT('Ctrl Pts',(2.78488741699995,11.6,-10.746722051));
#157594=CARTESIAN_POINT('Ctrl Pts',(2.78527368899995,15.2,-10.743503955));
#157595=CARTESIAN_POINT('Ctrl Pts',(2.78527368899995,11.6,-10.743503955));
#157596=CARTESIAN_POINT('Ctrl Pts',(2.78565678099994,15.2,-10.740290592));
#157597=CARTESIAN_POINT('Ctrl Pts',(2.78565678099994,11.6,-10.740290592));
#157598=CARTESIAN_POINT('Ctrl Pts',(2.78603669999994,15.2,-10.737081969));
#157599=CARTESIAN_POINT('Ctrl Pts',(2.78603669999994,11.6,-10.737081969));
#157600=CARTESIAN_POINT('Ctrl Pts',(2.78641344899994,15.2,-10.733878099));
#157601=CARTESIAN_POINT('Ctrl Pts',(2.78641344899994,11.6,-10.733878099));
#157602=CARTESIAN_POINT('Ctrl Pts',(2.78678703799994,15.2,-10.73067899));
#157603=CARTESIAN_POINT('Ctrl Pts',(2.78678703799994,11.6,-10.73067899));
#157604=CARTESIAN_POINT('Ctrl Pts',(2.78715746899994,15.2,-10.72748465));
#157605=CARTESIAN_POINT('Ctrl Pts',(2.78715746899994,11.6,-10.72748465));
#157606=CARTESIAN_POINT('Ctrl Pts',(2.78752474999994,15.2,-10.724295091));
#157607=CARTESIAN_POINT('Ctrl Pts',(2.78752474999994,11.6,-10.724295091));
#157608=CARTESIAN_POINT('Ctrl Pts',(2.78788888599995,15.2,-10.721110321));
#157609=CARTESIAN_POINT('Ctrl Pts',(2.78788888599995,11.6,-10.721110321));
#157610=CARTESIAN_POINT('Ctrl Pts',(2.78824988299994,15.2,-10.71793035));
#157611=CARTESIAN_POINT('Ctrl Pts',(2.78824988299994,11.6,-10.71793035));
#157612=CARTESIAN_POINT('Ctrl Pts',(2.78860774899994,15.2,-10.714755187));
#157613=CARTESIAN_POINT('Ctrl Pts',(2.78860774899994,11.6,-10.714755187));
#157614=CARTESIAN_POINT('Ctrl Pts',(2.78896248599994,15.2,-10.711584842));
#157615=CARTESIAN_POINT('Ctrl Pts',(2.78896248599994,11.6,-10.711584842));
#157616=CARTESIAN_POINT('Ctrl Pts',(2.78931410399994,15.2,-10.708419325));
#157617=CARTESIAN_POINT('Ctrl Pts',(2.78931410399994,11.6,-10.708419325));
#157618=CARTESIAN_POINT('Ctrl Pts',(2.78966260699994,15.2,-10.705258645));
#157619=CARTESIAN_POINT('Ctrl Pts',(2.78966260699994,11.6,-10.705258645));
#157620=CARTESIAN_POINT('Ctrl Pts',(2.79000799999995,15.2,-10.702102811));
#157621=CARTESIAN_POINT('Ctrl Pts',(2.79000799999995,11.6,-10.702102811));
#157622=CARTESIAN_POINT('Ctrl Pts',(2.79035029199994,15.2,-10.698951833));
#157623=CARTESIAN_POINT('Ctrl Pts',(2.79035029199994,11.6,-10.698951833));
#157624=CARTESIAN_POINT('Ctrl Pts',(2.79068948599994,15.2,-10.695805722));
#157625=CARTESIAN_POINT('Ctrl Pts',(2.79068948599994,11.6,-10.695805722));
#157626=CARTESIAN_POINT('Ctrl Pts',(2.79102558999994,15.2,-10.692664486));
#157627=CARTESIAN_POINT('Ctrl Pts',(2.79102558999994,11.6,-10.692664486));
#157628=CARTESIAN_POINT('Ctrl Pts',(2.79135860899994,15.2,-10.689528135));
#157629=CARTESIAN_POINT('Ctrl Pts',(2.79135860899994,11.6,-10.689528135));
#157630=CARTESIAN_POINT('Ctrl Pts',(2.79168855099994,15.2,-10.686396679));
#157631=CARTESIAN_POINT('Ctrl Pts',(2.79168855099994,11.6,-10.686396679));
#157632=CARTESIAN_POINT('Ctrl Pts',(2.79201541999994,15.2,-10.683270128));
#157633=CARTESIAN_POINT('Ctrl Pts',(2.79201541999994,11.6,-10.683270128));
#157634=CARTESIAN_POINT('Ctrl Pts',(2.79233922299994,15.2,-10.680148491));
#157635=CARTESIAN_POINT('Ctrl Pts',(2.79233922299994,11.6,-10.680148491));
#157636=CARTESIAN_POINT('Ctrl Pts',(2.79265996699994,15.2,-10.677031779));
#157637=CARTESIAN_POINT('Ctrl Pts',(2.79265996699994,11.6,-10.677031779));
#157638=CARTESIAN_POINT('Ctrl Pts',(2.79297765699994,15.2,-10.673919999));
#157639=CARTESIAN_POINT('Ctrl Pts',(2.79297765699994,11.6,-10.673919999));
#157640=CARTESIAN_POINT('Ctrl Pts',(2.79329229999994,15.2,-10.670813164));
#157641=CARTESIAN_POINT('Ctrl Pts',(2.79329229999994,11.6,-10.670813164));
#157642=CARTESIAN_POINT('Ctrl Pts',(2.79360390099994,15.2,-10.667711281));
#157643=CARTESIAN_POINT('Ctrl Pts',(2.79360390099994,11.6,-10.667711281));
#157644=CARTESIAN_POINT('Ctrl Pts',(2.79391246799995,15.2,-10.664614362));
#157645=CARTESIAN_POINT('Ctrl Pts',(2.79391246799995,11.6,-10.664614362));
#157646=CARTESIAN_POINT('Ctrl Pts',(2.79421800799994,15.2,-10.661522415));
#157647=CARTESIAN_POINT('Ctrl Pts',(2.79421800799994,11.6,-10.661522415));
#157648=CARTESIAN_POINT('Ctrl Pts',(2.79452052399995,15.2,-10.658435452));
#157649=CARTESIAN_POINT('Ctrl Pts',(2.79452052399995,11.6,-10.658435452));
#157650=CARTESIAN_POINT('Ctrl Pts',(2.79482002399994,15.2,-10.65535348));
#157651=CARTESIAN_POINT('Ctrl Pts',(2.79482002399994,11.6,-10.65535348));
#157652=CARTESIAN_POINT('Ctrl Pts',(2.79511651699994,15.2,-10.652276511));
#157653=CARTESIAN_POINT('Ctrl Pts',(2.79511651699994,11.6,-10.652276511));
#157654=CARTESIAN_POINT('Ctrl Pts',(2.79541000499994,15.2,-10.649204554));
#157655=CARTESIAN_POINT('Ctrl Pts',(2.79541000499994,11.6,-10.649204554));
#157656=CARTESIAN_POINT('Ctrl Pts',(2.79570049699994,15.2,-10.646137621));
#157657=CARTESIAN_POINT('Ctrl Pts',(2.79570049699994,11.6,-10.646137621));
#157658=CARTESIAN_POINT('Ctrl Pts',(2.79598799899994,15.2,-10.643075718));
#157659=CARTESIAN_POINT('Ctrl Pts',(2.79598799899994,11.6,-10.643075718));
#157660=CARTESIAN_POINT('Ctrl Pts',(2.79627251799994,15.2,-10.640018857));
#157661=CARTESIAN_POINT('Ctrl Pts',(2.79627251799994,11.6,-10.640018857));
#157662=CARTESIAN_POINT('Ctrl Pts',(2.79655405799994,15.2,-10.636967048));
#157663=CARTESIAN_POINT('Ctrl Pts',(2.79655405799994,11.6,-10.636967048));
#157664=CARTESIAN_POINT('Ctrl Pts',(2.79683262799994,15.2,-10.633920301));
#157665=CARTESIAN_POINT('Ctrl Pts',(2.79683262799994,11.6,-10.633920301));
#157666=CARTESIAN_POINT('Ctrl Pts',(2.79710823499994,15.2,-10.630878627));
#157667=CARTESIAN_POINT('Ctrl Pts',(2.79710823499994,11.6,-10.630878627));
#157668=CARTESIAN_POINT('Ctrl Pts',(2.79738088299994,15.2,-10.627842034));
#157669=CARTESIAN_POINT('Ctrl Pts',(2.79738088299994,11.6,-10.627842034));
#157670=CARTESIAN_POINT('Ctrl Pts',(2.79765057999994,15.2,-10.624810532));
#157671=CARTESIAN_POINT('Ctrl Pts',(2.79765057999994,11.6,-10.624810532));
#157672=CARTESIAN_POINT('Ctrl Pts',(2.79791733399994,15.2,-10.621784132));
#157673=CARTESIAN_POINT('Ctrl Pts',(2.79791733399994,11.6,-10.621784132));
#157674=CARTESIAN_POINT('Ctrl Pts',(2.79818114799995,15.2,-10.618762844));
#157675=CARTESIAN_POINT('Ctrl Pts',(2.79818114799995,11.6,-10.618762844));
#157676=CARTESIAN_POINT('Ctrl Pts',(2.79844203199994,15.2,-10.615746678));
#157677=CARTESIAN_POINT('Ctrl Pts',(2.79844203199994,11.6,-10.615746678));
#157678=CARTESIAN_POINT('Ctrl Pts',(2.79869999199994,15.2,-10.612735644));
#157679=CARTESIAN_POINT('Ctrl Pts',(2.79869999199994,11.6,-10.612735644));
#157680=CARTESIAN_POINT('Ctrl Pts',(2.79895503299994,15.2,-10.609729752));
#157681=CARTESIAN_POINT('Ctrl Pts',(2.79895503299994,11.6,-10.609729752));
#157682=CARTESIAN_POINT('Ctrl Pts',(2.79920716299995,15.2,-10.606729012));
#157683=CARTESIAN_POINT('Ctrl Pts',(2.79920716299995,11.6,-10.606729012));
#157684=CARTESIAN_POINT('Ctrl Pts',(2.79945638899994,15.2,-10.603733434));
#157685=CARTESIAN_POINT('Ctrl Pts',(2.79945638899994,11.6,-10.603733434));
#157686=CARTESIAN_POINT('Ctrl Pts',(2.79970271699994,15.2,-10.60074303));
#157687=CARTESIAN_POINT('Ctrl Pts',(2.79970271699994,11.6,-10.60074303));
#157688=CARTESIAN_POINT('Ctrl Pts',(2.79994615399994,15.2,-10.597757808));
#157689=CARTESIAN_POINT('Ctrl Pts',(2.79994615399994,11.6,-10.597757808));
#157690=CARTESIAN_POINT('Ctrl Pts',(2.80018670699994,15.2,-10.594777778));
#157691=CARTESIAN_POINT('Ctrl Pts',(2.80018670699994,11.6,-10.594777778));
#157692=CARTESIAN_POINT('Ctrl Pts',(2.80042438199994,15.2,-10.591802951));
#157693=CARTESIAN_POINT('Ctrl Pts',(2.80042438199994,11.6,-10.591802951));
#157694=CARTESIAN_POINT('Ctrl Pts',(2.80065918599994,15.2,-10.588833338));
#157695=CARTESIAN_POINT('Ctrl Pts',(2.80065918599994,11.6,-10.588833338));
#157696=CARTESIAN_POINT('Ctrl Pts',(2.80089112799994,15.2,-10.585868947));
#157697=CARTESIAN_POINT('Ctrl Pts',(2.80089112799994,11.6,-10.585868947));
#157698=CARTESIAN_POINT('Ctrl Pts',(2.80112021199994,15.2,-10.582909791));
#157699=CARTESIAN_POINT('Ctrl Pts',(2.80112021199994,11.6,-10.582909791));
#157700=CARTESIAN_POINT('Ctrl Pts',(2.80134644599995,15.2,-10.579955879));
#157701=CARTESIAN_POINT('Ctrl Pts',(2.80134644599995,11.6,-10.579955879));
#157702=CARTESIAN_POINT('Ctrl Pts',(2.80156983799994,15.2,-10.57700722));
#157703=CARTESIAN_POINT('Ctrl Pts',(2.80156983799994,11.6,-10.57700722));
#157704=CARTESIAN_POINT('Ctrl Pts',(2.80179039399994,15.2,-10.574063826));
#157705=CARTESIAN_POINT('Ctrl Pts',(2.80179039399994,11.6,-10.574063826));
#157706=CARTESIAN_POINT('Ctrl Pts',(2.80200812099995,15.2,-10.571125707));
#157707=CARTESIAN_POINT('Ctrl Pts',(2.80200812099995,11.6,-10.571125707));
#157708=CARTESIAN_POINT('Ctrl Pts',(2.80222302499994,15.2,-10.568192873));
#157709=CARTESIAN_POINT('Ctrl Pts',(2.80222302499994,11.6,-10.568192873));
#157710=CARTESIAN_POINT('Ctrl Pts',(2.80243511399994,15.2,-10.565265335));
#157711=CARTESIAN_POINT('Ctrl Pts',(2.80243511399994,11.6,-10.565265335));
#157712=CARTESIAN_POINT('Ctrl Pts',(2.80264439599994,15.2,-10.562343102));
#157713=CARTESIAN_POINT('Ctrl Pts',(2.80264439599994,11.6,-10.562343102));
#157714=CARTESIAN_POINT('Ctrl Pts',(2.80285087799995,15.2,-10.559426187));
#157715=CARTESIAN_POINT('Ctrl Pts',(2.80285087799995,11.6,-10.559426187));
#157716=CARTESIAN_POINT('Ctrl Pts',(2.80305456399994,15.2,-10.556514598));
#157717=CARTESIAN_POINT('Ctrl Pts',(2.80305456399994,11.6,-10.556514598));
#157718=CARTESIAN_POINT('Ctrl Pts',(2.80325546499995,15.2,-10.553608345));
#157719=CARTESIAN_POINT('Ctrl Pts',(2.80325546499995,11.6,-10.553608345));
#157720=CARTESIAN_POINT('Ctrl Pts',(2.80345358699994,15.2,-10.550707441));
#157721=CARTESIAN_POINT('Ctrl Pts',(2.80345358699994,11.6,-10.550707441));
#157722=CARTESIAN_POINT('Ctrl Pts',(2.80364893499994,15.2,-10.547811895));
#157723=CARTESIAN_POINT('Ctrl Pts',(2.80364893499994,11.6,-10.547811895));
#157724=CARTESIAN_POINT('Ctrl Pts',(2.80384151799994,15.2,-10.544921716));
#157725=CARTESIAN_POINT('Ctrl Pts',(2.80384151799994,11.6,-10.544921716));
#157726=CARTESIAN_POINT('Ctrl Pts',(2.80403134499994,15.2,-10.542036918));
#157727=CARTESIAN_POINT('Ctrl Pts',(2.80403134499994,11.6,-10.542036918));
#157728=CARTESIAN_POINT('Ctrl Pts',(2.80421841999994,15.2,-10.539157509));
#157729=CARTESIAN_POINT('Ctrl Pts',(2.80421841999994,11.6,-10.539157509));
#157730=CARTESIAN_POINT('Ctrl Pts',(2.80440275199994,15.2,-10.5362835));
#157731=CARTESIAN_POINT('Ctrl Pts',(2.80440275199994,11.6,-10.5362835));
#157732=CARTESIAN_POINT('Ctrl Pts',(2.80458434799994,15.2,-10.533414902));
#157733=CARTESIAN_POINT('Ctrl Pts',(2.80458434799994,11.6,-10.533414902));
#157734=CARTESIAN_POINT('Ctrl Pts',(2.80476321499994,15.2,-10.530551725));
#157735=CARTESIAN_POINT('Ctrl Pts',(2.80476321499994,11.6,-10.530551725));
#157736=CARTESIAN_POINT('Ctrl Pts',(2.80493936099994,15.2,-10.52769398));
#157737=CARTESIAN_POINT('Ctrl Pts',(2.80493936099994,11.6,-10.52769398));
#157738=CARTESIAN_POINT('Ctrl Pts',(2.80511279299994,15.2,-10.524841678));
#157739=CARTESIAN_POINT('Ctrl Pts',(2.80511279299994,11.6,-10.524841678));
#157740=CARTESIAN_POINT('Ctrl Pts',(2.80528351799994,15.2,-10.521994829));
#157741=CARTESIAN_POINT('Ctrl Pts',(2.80528351799994,11.6,-10.521994829));
#157742=CARTESIAN_POINT('Ctrl Pts',(2.80545154499994,15.2,-10.519153444));
#157743=CARTESIAN_POINT('Ctrl Pts',(2.80545154499994,11.6,-10.519153444));
#157744=CARTESIAN_POINT('Ctrl Pts',(2.80561687899994,15.2,-10.516317533));
#157745=CARTESIAN_POINT('Ctrl Pts',(2.80561687899994,11.6,-10.516317533));
#157746=CARTESIAN_POINT('Ctrl Pts',(2.80577952899994,15.2,-10.513487108));
#157747=CARTESIAN_POINT('Ctrl Pts',(2.80577952899994,11.6,-10.513487108));
#157748=CARTESIAN_POINT('Ctrl Pts',(2.80593950199994,15.2,-10.510662179));
#157749=CARTESIAN_POINT('Ctrl Pts',(2.80593950199994,11.6,-10.510662179));
#157750=CARTESIAN_POINT('Ctrl Pts',(2.80609680699994,15.2,-10.507842756));
#157751=CARTESIAN_POINT('Ctrl Pts',(2.80609680699994,11.6,-10.507842756));
#157752=CARTESIAN_POINT('Ctrl Pts',(2.80625144999994,15.2,-10.505028852));
#157753=CARTESIAN_POINT('Ctrl Pts',(2.80625144999994,11.6,-10.505028852));
#157754=CARTESIAN_POINT('Ctrl Pts',(2.80640343799994,15.2,-10.502220475));
#157755=CARTESIAN_POINT('Ctrl Pts',(2.80640343799994,11.6,-10.502220475));
#157756=CARTESIAN_POINT('Ctrl Pts',(2.80655278099994,15.2,-10.499417637));
#157757=CARTESIAN_POINT('Ctrl Pts',(2.80655278099994,11.6,-10.499417637));
#157758=CARTESIAN_POINT('Ctrl Pts',(2.80669948499995,15.2,-10.49662035));
#157759=CARTESIAN_POINT('Ctrl Pts',(2.80669948499995,11.6,-10.49662035));
#157760=CARTESIAN_POINT('Ctrl Pts',(2.80684355699994,15.2,-10.493828624));
#157761=CARTESIAN_POINT('Ctrl Pts',(2.80684355699994,11.6,-10.493828624));
#157762=CARTESIAN_POINT('Ctrl Pts',(2.80698500599994,15.2,-10.491042469));
#157763=CARTESIAN_POINT('Ctrl Pts',(2.80698500599994,11.6,-10.491042469));
#157764=CARTESIAN_POINT('Ctrl Pts',(2.80712383899994,15.2,-10.488261896));
#157765=CARTESIAN_POINT('Ctrl Pts',(2.80712383899994,11.6,-10.488261896));
#157766=CARTESIAN_POINT('Ctrl Pts',(2.80726006499994,15.2,-10.485486918));
#157767=CARTESIAN_POINT('Ctrl Pts',(2.80726006499994,11.6,-10.485486918));
#157768=CARTESIAN_POINT('Ctrl Pts',(2.80739368899994,15.2,-10.482717544));
#157769=CARTESIAN_POINT('Ctrl Pts',(2.80739368899994,11.6,-10.482717544));
#157770=CARTESIAN_POINT('Ctrl Pts',(2.80752472199994,15.2,-10.479953785));
#157771=CARTESIAN_POINT('Ctrl Pts',(2.80752472199994,11.6,-10.479953785));
#157772=CARTESIAN_POINT('Ctrl Pts',(2.80765316999994,15.2,-10.477195652));
#157773=CARTESIAN_POINT('Ctrl Pts',(2.80765316999994,11.6,-10.477195652));
#157774=CARTESIAN_POINT('Ctrl Pts',(2.80777904199994,15.2,-10.474443157));
#157775=CARTESIAN_POINT('Ctrl Pts',(2.80777904199994,11.6,-10.474443157));
#157776=CARTESIAN_POINT('Ctrl Pts',(2.80790234399994,15.2,-10.471696311));
#157777=CARTESIAN_POINT('Ctrl Pts',(2.80790234399994,11.6,-10.471696311));
#157778=CARTESIAN_POINT('Ctrl Pts',(2.80802308699994,15.2,-10.468955124));
#157779=CARTESIAN_POINT('Ctrl Pts',(2.80802308699994,11.6,-10.468955124));
#157780=CARTESIAN_POINT('Ctrl Pts',(2.80814127599994,15.2,-10.466219607));
#157781=CARTESIAN_POINT('Ctrl Pts',(2.80814127599994,11.6,-10.466219607));
#157782=CARTESIAN_POINT('Ctrl Pts',(2.80825691899994,15.2,-10.463489771));
#157783=CARTESIAN_POINT('Ctrl Pts',(2.80825691899994,11.6,-10.463489771));
#157784=CARTESIAN_POINT('Ctrl Pts',(2.80837002599994,15.2,-10.460765629));
#157785=CARTESIAN_POINT('Ctrl Pts',(2.80837002599994,11.6,-10.460765629));
#157786=CARTESIAN_POINT('Ctrl Pts',(2.80848060399994,15.2,-10.458047191));
#157787=CARTESIAN_POINT('Ctrl Pts',(2.80848060399994,11.6,-10.458047191));
#157788=CARTESIAN_POINT('Ctrl Pts',(2.80858866099994,15.2,-10.455334468));
#157789=CARTESIAN_POINT('Ctrl Pts',(2.80858866099994,11.6,-10.455334468));
#157790=CARTESIAN_POINT('Ctrl Pts',(2.80869420399994,15.2,-10.45262747));
#157791=CARTESIAN_POINT('Ctrl Pts',(2.80869420399994,11.6,-10.45262747));
#157792=CARTESIAN_POINT('Ctrl Pts',(2.80879724399994,15.2,-10.44992621));
#157793=CARTESIAN_POINT('Ctrl Pts',(2.80879724399994,11.6,-10.44992621));
#157794=CARTESIAN_POINT('Ctrl Pts',(2.80889778599994,15.2,-10.4472307));
#157795=CARTESIAN_POINT('Ctrl Pts',(2.80889778599994,11.6,-10.4472307));
#157796=CARTESIAN_POINT('Ctrl Pts',(2.80899583999994,15.2,-10.444540948));
#157797=CARTESIAN_POINT('Ctrl Pts',(2.80899583999994,11.6,-10.444540948));
#157798=CARTESIAN_POINT('Ctrl Pts',(2.80909141499994,15.2,-10.441856967));
#157799=CARTESIAN_POINT('Ctrl Pts',(2.80909141499994,11.6,-10.441856967));
#157800=CARTESIAN_POINT('Ctrl Pts',(2.80918451699995,15.2,-10.439178769));
#157801=CARTESIAN_POINT('Ctrl Pts',(2.80918451699995,11.6,-10.439178769));
#157802=CARTESIAN_POINT('Ctrl Pts',(2.80927515499994,15.2,-10.436506365));
#157803=CARTESIAN_POINT('Ctrl Pts',(2.80927515499994,11.6,-10.436506365));
#157804=CARTESIAN_POINT('Ctrl Pts',(2.80936333799994,15.2,-10.433839767));
#157805=CARTESIAN_POINT('Ctrl Pts',(2.80936333799994,11.6,-10.433839767));
#157806=CARTESIAN_POINT('Ctrl Pts',(2.80944907299994,15.2,-10.431178984));
#157807=CARTESIAN_POINT('Ctrl Pts',(2.80944907299994,11.6,-10.431178984));
#157808=CARTESIAN_POINT('Ctrl Pts',(2.80953236999995,15.2,-10.428524029));
#157809=CARTESIAN_POINT('Ctrl Pts',(2.80953236999995,11.6,-10.428524029));
#157810=CARTESIAN_POINT('Ctrl Pts',(2.80961323599994,15.2,-10.425874914));
#157811=CARTESIAN_POINT('Ctrl Pts',(2.80961323599994,11.6,-10.425874914));
#157812=CARTESIAN_POINT('Ctrl Pts',(2.80969167999995,15.2,-10.423231648));
#157813=CARTESIAN_POINT('Ctrl Pts',(2.80969167999995,11.6,-10.423231648));
#157814=CARTESIAN_POINT('Ctrl Pts',(2.80976771099994,15.2,-10.420594246));
#157815=CARTESIAN_POINT('Ctrl Pts',(2.80976771099994,11.6,-10.420594246));
#157816=CARTESIAN_POINT('Ctrl Pts',(2.80984133599994,15.2,-10.417962716));
#157817=CARTESIAN_POINT('Ctrl Pts',(2.80984133599994,11.6,-10.417962716));
#157818=CARTESIAN_POINT('Ctrl Pts',(2.80991256599994,15.2,-10.415337072));
#157819=CARTESIAN_POINT('Ctrl Pts',(2.80991256599994,11.6,-10.415337072));
#157820=CARTESIAN_POINT('Ctrl Pts',(2.80998140599994,15.2,-10.412717325));
#157821=CARTESIAN_POINT('Ctrl Pts',(2.80998140599994,11.6,-10.412717325));
#157822=CARTESIAN_POINT('Ctrl Pts',(2.81004786699994,15.2,-10.410103485));
#157823=CARTESIAN_POINT('Ctrl Pts',(2.81004786699994,11.6,-10.410103485));
#157824=CARTESIAN_POINT('Ctrl Pts',(2.81011195699994,15.2,-10.407495565));
#157825=CARTESIAN_POINT('Ctrl Pts',(2.81011195699994,11.6,-10.407495565));
#157826=CARTESIAN_POINT('Ctrl Pts',(2.81017368499994,15.2,-10.404893577));
#157827=CARTESIAN_POINT('Ctrl Pts',(2.81017368499994,11.6,-10.404893577));
#157828=CARTESIAN_POINT('Ctrl Pts',(2.81023305899994,15.2,-10.402297532));
#157829=CARTESIAN_POINT('Ctrl Pts',(2.81023305899994,11.6,-10.402297532));
#157830=CARTESIAN_POINT('Ctrl Pts',(2.81029008899994,15.2,-10.39970744));
#157831=CARTESIAN_POINT('Ctrl Pts',(2.81029008899994,11.6,-10.39970744));
#157832=CARTESIAN_POINT('Ctrl Pts',(2.81034478199994,15.2,-10.397123316));
#157833=CARTESIAN_POINT('Ctrl Pts',(2.81034478199994,11.6,-10.397123316));
#157834=CARTESIAN_POINT('Ctrl Pts',(2.81039714699994,15.2,-10.394545169));
#157835=CARTESIAN_POINT('Ctrl Pts',(2.81039714699994,11.6,-10.394545169));
#157836=CARTESIAN_POINT('Ctrl Pts',(2.81044719399994,15.2,-10.391973012));
#157837=CARTESIAN_POINT('Ctrl Pts',(2.81044719399994,11.6,-10.391973012));
#157838=CARTESIAN_POINT('Ctrl Pts',(2.81049492999994,15.2,-10.389406856));
#157839=CARTESIAN_POINT('Ctrl Pts',(2.81049492999994,11.6,-10.389406856));
#157840=CARTESIAN_POINT('Ctrl Pts',(2.81054036499994,15.2,-10.386846714));
#157841=CARTESIAN_POINT('Ctrl Pts',(2.81054036499994,11.6,-10.386846714));
#157842=CARTESIAN_POINT('Ctrl Pts',(2.81058350899994,15.2,-10.384292597));
#157843=CARTESIAN_POINT('Ctrl Pts',(2.81058350899994,11.6,-10.384292597));
#157844=CARTESIAN_POINT('Ctrl Pts',(2.81062436799994,15.2,-10.381744516));
#157845=CARTESIAN_POINT('Ctrl Pts',(2.81062436799994,11.6,-10.381744516));
#157846=CARTESIAN_POINT('Ctrl Pts',(2.81066295399994,15.2,-10.379202483));
#157847=CARTESIAN_POINT('Ctrl Pts',(2.81066295399994,11.6,-10.379202483));
#157848=CARTESIAN_POINT('Ctrl Pts',(2.81069927399995,15.2,-10.376666512));
#157849=CARTESIAN_POINT('Ctrl Pts',(2.81069927399995,11.6,-10.376666512));
#157850=CARTESIAN_POINT('Ctrl Pts',(2.81073333699994,15.2,-10.374136614));
#157851=CARTESIAN_POINT('Ctrl Pts',(2.81073333699994,11.6,-10.374136614));
#157852=CARTESIAN_POINT('Ctrl Pts',(2.81076515299994,15.2,-10.371612798));
#157853=CARTESIAN_POINT('Ctrl Pts',(2.81076515299994,11.6,-10.371612798));
#157854=CARTESIAN_POINT('Ctrl Pts',(2.81079472999994,15.2,-10.36909508));
#157855=CARTESIAN_POINT('Ctrl Pts',(2.81079472999994,11.6,-10.36909508));
#157856=CARTESIAN_POINT('Ctrl Pts',(2.81082207799995,15.2,-10.366583471));
#157857=CARTESIAN_POINT('Ctrl Pts',(2.81082207799995,11.6,-10.366583471));
#157858=CARTESIAN_POINT('Ctrl Pts',(2.81084720699994,15.2,-10.364077981));
#157859=CARTESIAN_POINT('Ctrl Pts',(2.81084720699994,11.6,-10.364077981));
#157860=CARTESIAN_POINT('Ctrl Pts',(2.81087012399994,15.2,-10.361578623));
#157861=CARTESIAN_POINT('Ctrl Pts',(2.81087012399994,11.6,-10.361578623));
#157862=CARTESIAN_POINT('Ctrl Pts',(2.81089083899994,15.2,-10.35908541));
#157863=CARTESIAN_POINT('Ctrl Pts',(2.81089083899994,11.6,-10.35908541));
#157864=CARTESIAN_POINT('Ctrl Pts',(2.81090936199994,15.2,-10.356598354));
#157865=CARTESIAN_POINT('Ctrl Pts',(2.81090936199994,11.6,-10.356598354));
#157866=CARTESIAN_POINT('Ctrl Pts',(2.81092570199994,15.2,-10.354117466));
#157867=CARTESIAN_POINT('Ctrl Pts',(2.81092570199994,11.6,-10.354117466));
#157868=CARTESIAN_POINT('Ctrl Pts',(2.81093986699994,15.2,-10.351642759));
#157869=CARTESIAN_POINT('Ctrl Pts',(2.81093986699994,11.6,-10.351642759));
#157870=CARTESIAN_POINT('Ctrl Pts',(2.81095186899994,15.2,-10.349174244));
#157871=CARTESIAN_POINT('Ctrl Pts',(2.81095186899994,11.6,-10.349174244));
#157872=CARTESIAN_POINT('Ctrl Pts',(2.81096171499994,15.2,-10.346711935));
#157873=CARTESIAN_POINT('Ctrl Pts',(2.81096171499994,11.6,-10.346711935));
#157874=CARTESIAN_POINT('Ctrl Pts',(2.81096941499994,15.2,-10.344255843));
#157875=CARTESIAN_POINT('Ctrl Pts',(2.81096941499994,11.6,-10.344255843));
#157876=CARTESIAN_POINT('Ctrl Pts',(2.81097497899994,15.2,-10.34180598));
#157877=CARTESIAN_POINT('Ctrl Pts',(2.81097497899994,11.6,-10.34180598));
#157878=CARTESIAN_POINT('Ctrl Pts',(2.81097841599995,15.2,-10.339362359));
#157879=CARTESIAN_POINT('Ctrl Pts',(2.81097841599995,11.6,-10.339362359));
#157880=CARTESIAN_POINT('Ctrl Pts',(2.81097973499994,15.2,-10.336924993));
#157881=CARTESIAN_POINT('Ctrl Pts',(2.81097973499994,11.6,-10.336924993));
#157882=CARTESIAN_POINT('Ctrl Pts',(2.81097894699994,15.2,-10.334493893));
#157883=CARTESIAN_POINT('Ctrl Pts',(2.81097894699994,11.6,-10.334493893));
#157884=CARTESIAN_POINT('Ctrl Pts',(2.81097606099994,15.2,-10.332069072));
#157885=CARTESIAN_POINT('Ctrl Pts',(2.81097606099994,11.6,-10.332069072));
#157886=CARTESIAN_POINT('Ctrl Pts',(2.81097108599994,15.2,-10.329650541));
#157887=CARTESIAN_POINT('Ctrl Pts',(2.81097108599994,11.6,-10.329650541));
#157888=CARTESIAN_POINT('Ctrl Pts',(2.81096403099995,15.2,-10.327238315));
#157889=CARTESIAN_POINT('Ctrl Pts',(2.81096403099995,11.6,-10.327238315));
#157890=CARTESIAN_POINT('Ctrl Pts',(2.81095490899995,15.2,-10.324832405));
#157891=CARTESIAN_POINT('Ctrl Pts',(2.81095490899995,11.6,-10.324832405));
#157892=CARTESIAN_POINT('Ctrl Pts',(2.81094372499994,15.2,-10.322432824));
#157893=CARTESIAN_POINT('Ctrl Pts',(2.81094372499994,11.6,-10.322432824));
#157894=CARTESIAN_POINT('Ctrl Pts',(2.81093049199994,15.2,-10.320039582));
#157895=CARTESIAN_POINT('Ctrl Pts',(2.81093049199994,11.6,-10.320039582));
#157896=CARTESIAN_POINT('Ctrl Pts',(2.81091521999994,15.2,-10.317652696));
#157897=CARTESIAN_POINT('Ctrl Pts',(2.81091521999994,11.6,-10.317652696));
#157898=CARTESIAN_POINT('Ctrl Pts',(2.81089791699995,15.2,-10.315272175));
#157899=CARTESIAN_POINT('Ctrl Pts',(2.81089791699995,11.6,-10.315272175));
#157900=CARTESIAN_POINT('Ctrl Pts',(2.81087859399994,15.2,-10.312898032));
#157901=CARTESIAN_POINT('Ctrl Pts',(2.81087859399994,11.6,-10.312898032));
#157902=CARTESIAN_POINT('Ctrl Pts',(2.81085726099994,15.2,-10.310530281));
#157903=CARTESIAN_POINT('Ctrl Pts',(2.81085726099994,11.6,-10.310530281));
#157904=CARTESIAN_POINT('Ctrl Pts',(2.81083392699994,15.2,-10.308168934));
#157905=CARTESIAN_POINT('Ctrl Pts',(2.81083392699994,11.6,-10.308168934));
#157906=CARTESIAN_POINT('Ctrl Pts',(2.81080860299994,15.2,-10.305814005));
#157907=CARTESIAN_POINT('Ctrl Pts',(2.81080860299994,11.6,-10.305814005));
#157908=CARTESIAN_POINT('Ctrl Pts',(2.81078129899994,15.2,-10.303465503));
#157909=CARTESIAN_POINT('Ctrl Pts',(2.81078129899994,11.6,-10.303465503));
#157910=CARTESIAN_POINT('Ctrl Pts',(2.81075202399995,15.2,-10.301123444));
#157911=CARTESIAN_POINT('Ctrl Pts',(2.81075202399995,11.6,-10.301123444));
#157912=CARTESIAN_POINT('Ctrl Pts',(2.81072078899995,15.2,-10.298787841));
#157913=CARTESIAN_POINT('Ctrl Pts',(2.81072078899995,11.6,-10.298787841));
#157914=CARTESIAN_POINT('Ctrl Pts',(2.81068760399994,15.2,-10.296458705));
#157915=CARTESIAN_POINT('Ctrl Pts',(2.81068760399994,11.6,-10.296458705));
#157916=CARTESIAN_POINT('Ctrl Pts',(2.81065247899994,15.2,-10.294136049));
#157917=CARTESIAN_POINT('Ctrl Pts',(2.81065247899994,11.6,-10.294136049));
#157918=CARTESIAN_POINT('Ctrl Pts',(2.81061542499994,15.2,-10.291819888));
#157919=CARTESIAN_POINT('Ctrl Pts',(2.81061542499994,11.6,-10.291819888));
#157920=CARTESIAN_POINT('Ctrl Pts',(2.81057645099994,15.2,-10.289510231));
#157921=CARTESIAN_POINT('Ctrl Pts',(2.81057645099994,11.6,-10.289510231));
#157922=CARTESIAN_POINT('Ctrl Pts',(2.81053556799994,15.2,-10.287207095));
#157923=CARTESIAN_POINT('Ctrl Pts',(2.81053556799994,11.6,-10.287207095));
#157924=CARTESIAN_POINT('Ctrl Pts',(2.81049278599995,15.2,-10.284910491));
#157925=CARTESIAN_POINT('Ctrl Pts',(2.81049278599995,11.6,-10.284910491));
#157926=CARTESIAN_POINT('Ctrl Pts',(2.81044811599994,15.2,-10.282620432));
#157927=CARTESIAN_POINT('Ctrl Pts',(2.81044811599994,11.6,-10.282620432));
#157928=CARTESIAN_POINT('Ctrl Pts',(2.81040156799994,15.2,-10.280336931));
#157929=CARTESIAN_POINT('Ctrl Pts',(2.81040156799994,11.6,-10.280336931));
#157930=CARTESIAN_POINT('Ctrl Pts',(2.81035315299994,15.2,-10.278060001));
#157931=CARTESIAN_POINT('Ctrl Pts',(2.81035315299994,11.6,-10.278060001));
#157932=CARTESIAN_POINT('Ctrl Pts',(2.81030287999994,15.2,-10.275789656));
#157933=CARTESIAN_POINT('Ctrl Pts',(2.81030287999994,11.6,-10.275789656));
#157934=CARTESIAN_POINT('Ctrl Pts',(2.81025076099994,15.2,-10.273525908));
#157935=CARTESIAN_POINT('Ctrl Pts',(2.81025076099994,11.6,-10.273525908));
#157936=CARTESIAN_POINT('Ctrl Pts',(2.81019680699994,15.2,-10.271268771));
#157937=CARTESIAN_POINT('Ctrl Pts',(2.81019680699994,11.6,-10.271268771));
#157938=CARTESIAN_POINT('Ctrl Pts',(2.81014102599995,15.2,-10.269018258));
#157939=CARTESIAN_POINT('Ctrl Pts',(2.81014102599995,11.6,-10.269018258));
#157940=CARTESIAN_POINT('Ctrl Pts',(2.81008343199994,15.2,-10.266774381));
#157941=CARTESIAN_POINT('Ctrl Pts',(2.81008343199994,11.6,-10.266774381));
#157942=CARTESIAN_POINT('Ctrl Pts',(2.81002403299994,15.2,-10.264537156));
#157943=CARTESIAN_POINT('Ctrl Pts',(2.81002403299994,11.6,-10.264537156));
#157944=CARTESIAN_POINT('Ctrl Pts',(2.80996284099994,15.2,-10.262306593));
#157945=CARTESIAN_POINT('Ctrl Pts',(2.80996284099994,11.6,-10.262306593));
#157946=CARTESIAN_POINT('Ctrl Pts',(2.80989986699994,15.2,-10.260082708));
#157947=CARTESIAN_POINT('Ctrl Pts',(2.80989986699994,11.6,-10.260082708));
#157948=CARTESIAN_POINT('Ctrl Pts',(2.80983512099994,15.2,-10.257865513));
#157949=CARTESIAN_POINT('Ctrl Pts',(2.80983512099994,11.6,-10.257865513));
#157950=CARTESIAN_POINT('Ctrl Pts',(2.80976861499994,15.2,-10.25565502));
#157951=CARTESIAN_POINT('Ctrl Pts',(2.80976861499994,11.6,-10.25565502));
#157952=CARTESIAN_POINT('Ctrl Pts',(2.80970035899994,15.2,-10.253451247));
#157953=CARTESIAN_POINT('Ctrl Pts',(2.80970035899994,11.6,-10.253451247));
#157954=CARTESIAN_POINT('Ctrl Pts',(2.80963036399994,15.2,-10.251254202));
#157955=CARTESIAN_POINT('Ctrl Pts',(2.80963036399994,11.6,-10.251254202));
#157956=CARTESIAN_POINT('Ctrl Pts',(2.80955864199994,15.2,-10.249063901));
#157957=CARTESIAN_POINT('Ctrl Pts',(2.80955864199994,11.6,-10.249063901));
#157958=CARTESIAN_POINT('Ctrl Pts',(2.80948520299994,15.2,-10.246880359));
#157959=CARTESIAN_POINT('Ctrl Pts',(2.80948520299994,11.6,-10.246880359));
#157960=CARTESIAN_POINT('Ctrl Pts',(2.80941005699994,15.2,-10.244703587));
#157961=CARTESIAN_POINT('Ctrl Pts',(2.80941005699994,11.6,-10.244703587));
#157962=CARTESIAN_POINT('Ctrl Pts',(2.80933321799994,15.2,-10.242533601));
#157963=CARTESIAN_POINT('Ctrl Pts',(2.80933321799994,11.6,-10.242533601));
#157964=CARTESIAN_POINT('Ctrl Pts',(2.80925469499994,15.2,-10.240370412));
#157965=CARTESIAN_POINT('Ctrl Pts',(2.80925469499994,11.6,-10.240370412));
#157966=CARTESIAN_POINT('Ctrl Pts',(2.80917449899994,15.2,-10.238214035));
#157967=CARTESIAN_POINT('Ctrl Pts',(2.80917449899994,11.6,-10.238214035));
#157968=CARTESIAN_POINT('Ctrl Pts',(2.80909264299994,15.2,-10.236064484));
#157969=CARTESIAN_POINT('Ctrl Pts',(2.80909264299994,11.6,-10.236064484));
#157970=CARTESIAN_POINT('Ctrl Pts',(2.80900913699994,15.2,-10.233921772));
#157971=CARTESIAN_POINT('Ctrl Pts',(2.80900913699994,11.6,-10.233921772));
#157972=CARTESIAN_POINT('Ctrl Pts',(2.80892399399994,15.2,-10.231785914));
#157973=CARTESIAN_POINT('Ctrl Pts',(2.80892399399994,11.6,-10.231785914));
#157974=CARTESIAN_POINT('Ctrl Pts',(2.80883722299994,15.2,-10.229656922));
#157975=CARTESIAN_POINT('Ctrl Pts',(2.80883722299994,11.6,-10.229656922));
#157976=CARTESIAN_POINT('Ctrl Pts',(2.80874883699994,15.2,-10.227534811));
#157977=CARTESIAN_POINT('Ctrl Pts',(2.80874883699994,11.6,-10.227534811));
#157978=CARTESIAN_POINT('Ctrl Pts',(2.80865884799995,15.2,-10.225419595));
#157979=CARTESIAN_POINT('Ctrl Pts',(2.80865884799995,11.6,-10.225419595));
#157980=CARTESIAN_POINT('Ctrl Pts',(2.80856726499994,15.2,-10.223311288));
#157981=CARTESIAN_POINT('Ctrl Pts',(2.80856726499994,11.6,-10.223311288));
#157982=CARTESIAN_POINT('Ctrl Pts',(2.80847410199994,15.2,-10.221209902));
#157983=CARTESIAN_POINT('Ctrl Pts',(2.80847410199994,11.6,-10.221209902));
#157984=CARTESIAN_POINT('Ctrl Pts',(2.80837936999994,15.2,-10.219115454));
#157985=CARTESIAN_POINT('Ctrl Pts',(2.80837936999994,11.6,-10.219115454));
#157986=CARTESIAN_POINT('Ctrl Pts',(2.80828307999994,15.2,-10.217027955));
#157987=CARTESIAN_POINT('Ctrl Pts',(2.80828307999994,11.6,-10.217027955));
#157988=CARTESIAN_POINT('Ctrl Pts',(2.80818524499994,15.2,-10.214947422));
#157989=CARTESIAN_POINT('Ctrl Pts',(2.80818524499994,11.6,-10.214947422));
#157990=CARTESIAN_POINT('Ctrl Pts',(2.80808587499994,15.2,-10.212873867));
#157991=CARTESIAN_POINT('Ctrl Pts',(2.80808587499994,11.6,-10.212873867));
#157992=CARTESIAN_POINT('Ctrl Pts',(2.80798498399994,15.2,-10.210807306));
#157993=CARTESIAN_POINT('Ctrl Pts',(2.80798498399994,11.6,-10.210807306));
#157994=CARTESIAN_POINT('Ctrl Pts',(2.80788258099995,15.2,-10.208747752));
#157995=CARTESIAN_POINT('Ctrl Pts',(2.80788258099995,11.6,-10.208747752));
#157996=CARTESIAN_POINT('Ctrl Pts',(2.80777868099995,15.2,-10.206695218));
#157997=CARTESIAN_POINT('Ctrl Pts',(2.80777868099995,11.6,-10.206695218));
#157998=CARTESIAN_POINT('Ctrl Pts',(2.80767329399994,15.2,-10.204649721));
#157999=CARTESIAN_POINT('Ctrl Pts',(2.80767329399994,11.6,-10.204649721));
#158000=CARTESIAN_POINT('Ctrl Pts',(2.80756643199994,15.2,-10.202611272));
#158001=CARTESIAN_POINT('Ctrl Pts',(2.80756643199994,11.6,-10.202611272));
#158002=CARTESIAN_POINT('Ctrl Pts',(2.80745810799994,15.2,-10.200579889));
#158003=CARTESIAN_POINT('Ctrl Pts',(2.80745810799994,11.6,-10.200579889));
#158004=CARTESIAN_POINT('Ctrl Pts',(2.80734833399995,15.2,-10.198555583));
#158005=CARTESIAN_POINT('Ctrl Pts',(2.80734833399995,11.6,-10.198555583));
#158006=CARTESIAN_POINT('Ctrl Pts',(2.80723712199995,15.2,-10.196538371));
#158007=CARTESIAN_POINT('Ctrl Pts',(2.80723712199995,11.6,-10.196538371));
#158008=CARTESIAN_POINT('Ctrl Pts',(2.80712448299994,15.2,-10.194528266));
#158009=CARTESIAN_POINT('Ctrl Pts',(2.80712448299994,11.6,-10.194528266));
#158010=CARTESIAN_POINT('Ctrl Pts',(2.80701043199994,15.2,-10.192525284));
#158011=CARTESIAN_POINT('Ctrl Pts',(2.80701043199994,11.6,-10.192525284));
#158012=CARTESIAN_POINT('Ctrl Pts',(2.80689497799994,15.2,-10.190529437));
#158013=CARTESIAN_POINT('Ctrl Pts',(2.80689497799994,11.6,-10.190529437));
#158014=CARTESIAN_POINT('Ctrl Pts',(2.80677813599994,15.2,-10.188540742));
#158015=CARTESIAN_POINT('Ctrl Pts',(2.80677813599994,11.6,-10.188540742));
#158016=CARTESIAN_POINT('Ctrl Pts',(2.80665991699995,15.2,-10.186559213));
#158017=CARTESIAN_POINT('Ctrl Pts',(2.80665991699995,11.6,-10.186559213));
#158018=CARTESIAN_POINT('Ctrl Pts',(2.80654033399995,15.2,-10.184584863));
#158019=CARTESIAN_POINT('Ctrl Pts',(2.80654033399995,11.6,-10.184584863));
#158020=CARTESIAN_POINT('Ctrl Pts',(2.80641939899994,15.2,-10.182617709));
#158021=CARTESIAN_POINT('Ctrl Pts',(2.80641939899994,11.6,-10.182617709));
#158022=CARTESIAN_POINT('Ctrl Pts',(2.80629712399994,15.2,-10.180657764));
#158023=CARTESIAN_POINT('Ctrl Pts',(2.80629712399994,11.6,-10.180657764));
#158024=CARTESIAN_POINT('Ctrl Pts',(2.80617352399994,15.2,-10.178705045));
#158025=CARTESIAN_POINT('Ctrl Pts',(2.80617352399994,11.6,-10.178705045));
#158026=CARTESIAN_POINT('Ctrl Pts',(2.80604860999994,15.2,-10.176759564));
#158027=CARTESIAN_POINT('Ctrl Pts',(2.80604860999994,11.6,-10.176759564));
#158028=CARTESIAN_POINT('Ctrl Pts',(2.80592239399994,15.2,-10.174821338));
#158029=CARTESIAN_POINT('Ctrl Pts',(2.80592239399994,11.6,-10.174821338));
#158030=CARTESIAN_POINT('Ctrl Pts',(2.80579489099994,15.2,-10.172890382));
#158031=CARTESIAN_POINT('Ctrl Pts',(2.80579489099994,11.6,-10.172890382));
#158032=CARTESIAN_POINT('Ctrl Pts',(2.80566611099994,15.2,-10.170966708));
#158033=CARTESIAN_POINT('Ctrl Pts',(2.80566611099994,11.6,-10.170966708));
#158034=CARTESIAN_POINT('Ctrl Pts',(2.80553606899994,15.2,-10.169050335));
#158035=CARTESIAN_POINT('Ctrl Pts',(2.80553606899994,11.6,-10.169050335));
#158036=CARTESIAN_POINT('Ctrl Pts',(2.80540477699994,15.2,-10.167141276));
#158037=CARTESIAN_POINT('Ctrl Pts',(2.80540477699994,11.6,-10.167141276));
#158038=CARTESIAN_POINT('Ctrl Pts',(2.80527224899994,15.2,-10.165239546));
#158039=CARTESIAN_POINT('Ctrl Pts',(2.80527224899994,11.6,-10.165239546));
#158040=CARTESIAN_POINT('Ctrl Pts',(2.80513849599994,15.2,-10.163345161));
#158041=CARTESIAN_POINT('Ctrl Pts',(2.80513849599994,11.6,-10.163345161));
#158042=CARTESIAN_POINT('Ctrl Pts',(2.80500353299994,15.2,-10.161458135));
#158043=CARTESIAN_POINT('Ctrl Pts',(2.80500353299994,11.6,-10.161458135));
#158044=CARTESIAN_POINT('Ctrl Pts',(2.80486737299994,15.2,-10.159578484));
#158045=CARTESIAN_POINT('Ctrl Pts',(2.80486737299994,11.6,-10.159578484));
#158046=CARTESIAN_POINT('Ctrl Pts',(2.80473002899994,15.2,-10.157706223));
#158047=CARTESIAN_POINT('Ctrl Pts',(2.80473002899994,11.6,-10.157706223));
#158048=CARTESIAN_POINT('Ctrl Pts',(2.80459151299994,15.2,-10.155841368));
#158049=CARTESIAN_POINT('Ctrl Pts',(2.80459151299994,11.6,-10.155841368));
#158050=CARTESIAN_POINT('Ctrl Pts',(2.80445183999994,15.2,-10.153983933));
#158051=CARTESIAN_POINT('Ctrl Pts',(2.80445183999994,11.6,-10.153983933));
#158052=CARTESIAN_POINT('Ctrl Pts',(2.80431102199994,15.2,-10.152133935));
#158053=CARTESIAN_POINT('Ctrl Pts',(2.80431102199994,11.6,-10.152133935));
#158054=CARTESIAN_POINT('Ctrl Pts',(2.80416907299994,15.2,-10.150291388));
#158055=CARTESIAN_POINT('Ctrl Pts',(2.80416907299994,11.6,-10.150291388));
#158056=CARTESIAN_POINT('Ctrl Pts',(2.80402600699994,15.2,-10.148456309));
#158057=CARTESIAN_POINT('Ctrl Pts',(2.80402600699994,11.6,-10.148456309));
#158058=CARTESIAN_POINT('Ctrl Pts',(2.80388183699994,15.2,-10.146628712));
#158059=CARTESIAN_POINT('Ctrl Pts',(2.80388183699994,11.6,-10.146628712));
#158060=CARTESIAN_POINT('Ctrl Pts',(2.80373657699994,15.2,-10.144808614));
#158061=CARTESIAN_POINT('Ctrl Pts',(2.80373657699994,11.6,-10.144808614));
#158062=CARTESIAN_POINT('Ctrl Pts',(2.80359023999994,15.2,-10.14299603));
#158063=CARTESIAN_POINT('Ctrl Pts',(2.80359023999994,11.6,-10.14299603));
#158064=CARTESIAN_POINT('Ctrl Pts',(2.80344283999994,15.2,-10.141190975));
#158065=CARTESIAN_POINT('Ctrl Pts',(2.80344283999994,11.6,-10.141190975));
#158066=CARTESIAN_POINT('Ctrl Pts',(2.80329439099994,15.2,-10.139393466));
#158067=CARTESIAN_POINT('Ctrl Pts',(2.80329439099994,11.6,-10.139393466));
#158068=CARTESIAN_POINT('Ctrl Pts',(2.80314490699995,15.2,-10.137603518));
#158069=CARTESIAN_POINT('Ctrl Pts',(2.80314490699995,11.6,-10.137603518));
#158070=CARTESIAN_POINT('Ctrl Pts',(2.80299440199994,15.2,-10.135821147));
#158071=CARTESIAN_POINT('Ctrl Pts',(2.80299440199994,11.6,-10.135821147));
#158072=CARTESIAN_POINT('Ctrl Pts',(2.80284288899994,15.2,-10.134046369));
#158073=CARTESIAN_POINT('Ctrl Pts',(2.80284288899994,11.6,-10.134046369));
#158074=CARTESIAN_POINT('Ctrl Pts',(2.80269038199994,15.2,-10.1322792));
#158075=CARTESIAN_POINT('Ctrl Pts',(2.80269038199994,11.6,-10.1322792));
#158076=CARTESIAN_POINT('Ctrl Pts',(2.80253689599995,15.2,-10.130519656));
#158077=CARTESIAN_POINT('Ctrl Pts',(2.80253689599995,11.6,-10.130519656));
#158078=CARTESIAN_POINT('Ctrl Pts',(2.80238244499994,15.2,-10.128767753));
#158079=CARTESIAN_POINT('Ctrl Pts',(2.80238244499994,11.6,-10.128767753));
#158080=CARTESIAN_POINT('Ctrl Pts',(2.80222704299995,15.2,-10.127023507));
#158081=CARTESIAN_POINT('Ctrl Pts',(2.80222704299995,11.6,-10.127023507));
#158082=CARTESIAN_POINT('Ctrl Pts',(2.80207070399995,15.2,-10.125286934));
#158083=CARTESIAN_POINT('Ctrl Pts',(2.80207070399995,11.6,-10.125286934));
#158084=CARTESIAN_POINT('Ctrl Pts',(2.80191344299995,15.2,-10.12355805));
#158085=CARTESIAN_POINT('Ctrl Pts',(2.80191344299995,11.6,-10.12355805));
#158086=CARTESIAN_POINT('Ctrl Pts',(2.80175527299994,15.2,-10.121836872));
#158087=CARTESIAN_POINT('Ctrl Pts',(2.80175527299994,11.6,-10.121836872));
#158088=CARTESIAN_POINT('Ctrl Pts',(2.80159621099994,15.2,-10.120123415));
#158089=CARTESIAN_POINT('Ctrl Pts',(2.80159621099994,11.6,-10.120123415));
#158090=CARTESIAN_POINT('Ctrl Pts',(2.80143626799994,15.2,-10.118417698));
#158091=CARTESIAN_POINT('Ctrl Pts',(2.80143626799994,11.6,-10.118417698));
#158092=CARTESIAN_POINT('Ctrl Pts',(2.80127546199994,15.2,-10.116719734));
#158093=CARTESIAN_POINT('Ctrl Pts',(2.80127546199994,11.6,-10.116719734));
#158094=CARTESIAN_POINT('Ctrl Pts',(2.80111380599994,15.2,-10.115029541));
#158095=CARTESIAN_POINT('Ctrl Pts',(2.80111380599994,11.6,-10.115029541));
#158096=CARTESIAN_POINT('Ctrl Pts',(2.80095131399994,15.2,-10.113347137));
#158097=CARTESIAN_POINT('Ctrl Pts',(2.80095131399994,11.6,-10.113347137));
#158098=CARTESIAN_POINT('Ctrl Pts',(2.80078800199994,15.2,-10.111672536));
#158099=CARTESIAN_POINT('Ctrl Pts',(2.80078800199994,11.6,-10.111672536));
#158100=CARTESIAN_POINT('Ctrl Pts',(2.80062388399994,15.2,-10.110005756));
#158101=CARTESIAN_POINT('Ctrl Pts',(2.80062388399994,11.6,-10.110005756));
#158102=CARTESIAN_POINT('Ctrl Pts',(2.80045897599994,15.2,-10.108346814));
#158103=CARTESIAN_POINT('Ctrl Pts',(2.80045897599994,11.6,-10.108346814));
#158104=CARTESIAN_POINT('Ctrl Pts',(2.80029329299994,15.2,-10.106695726));
#158105=CARTESIAN_POINT('Ctrl Pts',(2.80029329299994,11.6,-10.106695726));
#158106=CARTESIAN_POINT('Ctrl Pts',(2.80012684799994,15.2,-10.105052508));
#158107=CARTESIAN_POINT('Ctrl Pts',(2.80012684799994,11.6,-10.105052508));
#158108=CARTESIAN_POINT('Ctrl Pts',(2.79995965799994,15.2,-10.103417179));
#158109=CARTESIAN_POINT('Ctrl Pts',(2.79995965799994,11.6,-10.103417179));
#158110=CARTESIAN_POINT('Ctrl Pts',(2.79979173699994,15.2,-10.101789754));
#158111=CARTESIAN_POINT('Ctrl Pts',(2.79979173699994,11.6,-10.101789754));
#158112=CARTESIAN_POINT('Ctrl Pts',(2.79962310199994,15.2,-10.10017025));
#158113=CARTESIAN_POINT('Ctrl Pts',(2.79962310199994,11.6,-10.10017025));
#158114=CARTESIAN_POINT('Ctrl Pts',(2.79945376599994,15.2,-10.098558686));
#158115=CARTESIAN_POINT('Ctrl Pts',(2.79945376599994,11.6,-10.098558686));
#158116=CARTESIAN_POINT('Ctrl Pts',(2.79928374699994,15.2,-10.096955077));
#158117=CARTESIAN_POINT('Ctrl Pts',(2.79928374699994,11.6,-10.096955077));
#158118=CARTESIAN_POINT('Ctrl Pts',(2.79911305799994,15.2,-10.095359442));
#158119=CARTESIAN_POINT('Ctrl Pts',(2.79911305799994,11.6,-10.095359442));
#158120=CARTESIAN_POINT('Ctrl Pts',(2.79894171499994,15.2,-10.093771795));
#158121=CARTESIAN_POINT('Ctrl Pts',(2.79894171499994,11.6,-10.093771795));
#158122=CARTESIAN_POINT('Ctrl Pts',(2.79876973499994,15.2,-10.092192156));
#158123=CARTESIAN_POINT('Ctrl Pts',(2.79876973499994,11.6,-10.092192156));
#158124=CARTESIAN_POINT('Ctrl Pts',(2.79859713199994,15.2,-10.090620542));
#158125=CARTESIAN_POINT('Ctrl Pts',(2.79859713199994,11.6,-10.090620542));
#158126=CARTESIAN_POINT('Ctrl Pts',(2.79842392399994,15.2,-10.08905697));
#158127=CARTESIAN_POINT('Ctrl Pts',(2.79842392399994,11.6,-10.08905697));
#158128=CARTESIAN_POINT('Ctrl Pts',(2.79825012299994,15.2,-10.087501457));
#158129=CARTESIAN_POINT('Ctrl Pts',(2.79825012299994,11.6,-10.087501457));
#158130=CARTESIAN_POINT('Ctrl Pts',(2.79807574899994,15.2,-10.085954021));
#158131=CARTESIAN_POINT('Ctrl Pts',(2.79807574899994,11.6,-10.085954021));
#158132=CARTESIAN_POINT('Ctrl Pts',(2.79790081499995,15.2,-10.084414678));
#158133=CARTESIAN_POINT('Ctrl Pts',(2.79790081499995,11.6,-10.084414678));
#158134=CARTESIAN_POINT('Ctrl Pts',(2.79772533899994,15.2,-10.082883448));
#158135=CARTESIAN_POINT('Ctrl Pts',(2.79772533899994,11.6,-10.082883448));
#158136=CARTESIAN_POINT('Ctrl Pts',(2.79754933499994,15.2,-10.081360347));
#158137=CARTESIAN_POINT('Ctrl Pts',(2.79754933499994,11.6,-10.081360347));
#158138=CARTESIAN_POINT('Ctrl Pts',(2.79737282199994,15.2,-10.079845395));
#158139=CARTESIAN_POINT('Ctrl Pts',(2.79737282199994,11.6,-10.079845395));
#158140=CARTESIAN_POINT('Ctrl Pts',(2.79719581399994,15.2,-10.078338606));
#158141=CARTESIAN_POINT('Ctrl Pts',(2.79719581399994,11.6,-10.078338606));
#158142=CARTESIAN_POINT('Ctrl Pts',(2.79701832699994,15.2,-10.076840001));
#158143=CARTESIAN_POINT('Ctrl Pts',(2.79701832699994,11.6,-10.076840001));
#158144=CARTESIAN_POINT('Ctrl Pts',(2.79684037999994,15.2,-10.075349597));
#158145=CARTESIAN_POINT('Ctrl Pts',(2.79684037999994,11.6,-10.075349597));
#158146=CARTESIAN_POINT('Ctrl Pts',(2.79666198699994,15.2,-10.073867411));
#158147=CARTESIAN_POINT('Ctrl Pts',(2.79666198699994,11.6,-10.073867411));
#158148=CARTESIAN_POINT('Ctrl Pts',(2.79648316399994,15.2,-10.072393462));
#158149=CARTESIAN_POINT('Ctrl Pts',(2.79648316399994,11.6,-10.072393462));
#158150=CARTESIAN_POINT('Ctrl Pts',(2.79630393099994,15.2,-10.070927768));
#158151=CARTESIAN_POINT('Ctrl Pts',(2.79630393099994,11.6,-10.070927768));
#158152=CARTESIAN_POINT('Ctrl Pts',(2.79612430199994,15.2,-10.069470348));
#158153=CARTESIAN_POINT('Ctrl Pts',(2.79612430199994,11.6,-10.069470348));
#158154=CARTESIAN_POINT('Ctrl Pts',(2.79594429399994,15.2,-10.068021218));
#158155=CARTESIAN_POINT('Ctrl Pts',(2.79594429399994,11.6,-10.068021218));
#158156=CARTESIAN_POINT('Ctrl Pts',(2.79576392499994,15.2,-10.066580399));
#158157=CARTESIAN_POINT('Ctrl Pts',(2.79576392499994,11.6,-10.066580399));
#158158=CARTESIAN_POINT('Ctrl Pts',(2.79558320999994,15.2,-10.065147907));
#158159=CARTESIAN_POINT('Ctrl Pts',(2.79558320999994,11.6,-10.065147907));
#158160=CARTESIAN_POINT('Ctrl Pts',(2.79540216899994,15.2,-10.063723761));
#158161=CARTESIAN_POINT('Ctrl Pts',(2.79540216899994,11.6,-10.063723761));
#158162=CARTESIAN_POINT('Ctrl Pts',(2.79522081599994,15.2,-10.062307982));
#158163=CARTESIAN_POINT('Ctrl Pts',(2.79522081599994,11.6,-10.062307982));
#158164=CARTESIAN_POINT('Ctrl Pts',(2.79503916999994,15.2,-10.060900585));
#158165=CARTESIAN_POINT('Ctrl Pts',(2.79503916999994,11.6,-10.060900585));
#158166=CARTESIAN_POINT('Ctrl Pts',(2.79485724799994,15.2,-10.05950159));
#158167=CARTESIAN_POINT('Ctrl Pts',(2.79485724799994,11.6,-10.05950159));
#158168=CARTESIAN_POINT('Ctrl Pts',(2.79467506699994,15.2,-10.058111016));
#158169=CARTESIAN_POINT('Ctrl Pts',(2.79467506699994,11.6,-10.058111016));
#158170=CARTESIAN_POINT('Ctrl Pts',(2.79449264499994,15.2,-10.056728882));
#158171=CARTESIAN_POINT('Ctrl Pts',(2.79449264499994,11.6,-10.056728882));
#158172=CARTESIAN_POINT('Ctrl Pts',(2.79430999899994,15.2,-10.055355207));
#158173=CARTESIAN_POINT('Ctrl Pts',(2.79430999899994,11.6,-10.055355207));
#158174=CARTESIAN_POINT('Ctrl Pts',(2.79412714599995,15.2,-10.053990009));
#158175=CARTESIAN_POINT('Ctrl Pts',(2.79412714599995,11.6,-10.053990009));
#158176=CARTESIAN_POINT('Ctrl Pts',(2.79394410499994,15.2,-10.052633306));
#158177=CARTESIAN_POINT('Ctrl Pts',(2.79394410499994,11.6,-10.052633306));
#158178=CARTESIAN_POINT('Ctrl Pts',(2.79376089299994,15.2,-10.05128512));
#158179=CARTESIAN_POINT('Ctrl Pts',(2.79376089299994,11.6,-10.05128512));
#158180=CARTESIAN_POINT('Ctrl Pts',(2.79357752899994,15.2,-10.049945468));
#158181=CARTESIAN_POINT('Ctrl Pts',(2.79357752899994,11.6,-10.049945468));
#158182=CARTESIAN_POINT('Ctrl Pts',(2.79339402799994,15.2,-10.04861437));
#158183=CARTESIAN_POINT('Ctrl Pts',(2.79339402799994,11.6,-10.04861437));
#158184=CARTESIAN_POINT('Ctrl Pts',(2.79321041199994,15.2,-10.047291846));
#158185=CARTESIAN_POINT('Ctrl Pts',(2.79321041199994,11.6,-10.047291846));
#158186=CARTESIAN_POINT('Ctrl Pts',(2.79302669599995,15.2,-10.045977913));
#158187=CARTESIAN_POINT('Ctrl Pts',(2.79302669599995,11.6,-10.045977913));
#158188=CARTESIAN_POINT('Ctrl Pts',(2.79284289899994,15.2,-10.044672592));
#158189=CARTESIAN_POINT('Ctrl Pts',(2.79284289899994,11.6,-10.044672592));
#158190=CARTESIAN_POINT('Ctrl Pts',(2.79265904099995,15.2,-10.043375903));
#158191=CARTESIAN_POINT('Ctrl Pts',(2.79265904099995,11.6,-10.043375903));
#158192=CARTESIAN_POINT('Ctrl Pts',(2.79247513699994,15.2,-10.042087865));
#158193=CARTESIAN_POINT('Ctrl Pts',(2.79247513699994,11.6,-10.042087865));
#158194=CARTESIAN_POINT('Ctrl Pts',(2.79229120899994,15.2,-10.040808498));
#158195=CARTESIAN_POINT('Ctrl Pts',(2.79229120899994,11.6,-10.040808498));
#158196=CARTESIAN_POINT('Ctrl Pts',(2.79210727299994,15.2,-10.03953782));
#158197=CARTESIAN_POINT('Ctrl Pts',(2.79210727299994,11.6,-10.03953782));
#158198=CARTESIAN_POINT('Ctrl Pts',(2.79192334899995,15.2,-10.038275853));
#158199=CARTESIAN_POINT('Ctrl Pts',(2.79192334899995,11.6,-10.038275853));
#158200=CARTESIAN_POINT('Ctrl Pts',(2.79173945599994,15.2,-10.037022616));
#158201=CARTESIAN_POINT('Ctrl Pts',(2.79173945599994,11.6,-10.037022616));
#158202=CARTESIAN_POINT('Ctrl Pts',(2.79155561199994,15.2,-10.035778129));
#158203=CARTESIAN_POINT('Ctrl Pts',(2.79155561199994,11.6,-10.035778129));
#158204=CARTESIAN_POINT('Ctrl Pts',(2.79137183599994,15.2,-10.034542413));
#158205=CARTESIAN_POINT('Ctrl Pts',(2.79137183599994,11.6,-10.034542413));
#158206=CARTESIAN_POINT('Ctrl Pts',(2.79118814699994,15.2,-10.033315485));
#158207=CARTESIAN_POINT('Ctrl Pts',(2.79118814699994,11.6,-10.033315485));
#158208=CARTESIAN_POINT('Ctrl Pts',(2.79100456599994,15.2,-10.032097369));
#158209=CARTESIAN_POINT('Ctrl Pts',(2.79100456599994,11.6,-10.032097369));
#158210=CARTESIAN_POINT('Ctrl Pts',(2.79082110899994,15.2,-10.030888083));
#158211=CARTESIAN_POINT('Ctrl Pts',(2.79082110899994,11.6,-10.030888083));
#158212=CARTESIAN_POINT('Ctrl Pts',(2.79063779699994,15.2,-10.029687649));
#158213=CARTESIAN_POINT('Ctrl Pts',(2.79063779699994,11.6,-10.029687649));
#158214=CARTESIAN_POINT('Ctrl Pts',(2.79045464899994,15.2,-10.028496086));
#158215=CARTESIAN_POINT('Ctrl Pts',(2.79045464899994,11.6,-10.028496086));
#158216=CARTESIAN_POINT('Ctrl Pts',(2.79027168599994,15.2,-10.027313415));
#158217=CARTESIAN_POINT('Ctrl Pts',(2.79027168599994,11.6,-10.027313415));
#158218=CARTESIAN_POINT('Ctrl Pts',(2.79008892599995,15.2,-10.026139656));
#158219=CARTESIAN_POINT('Ctrl Pts',(2.79008892599995,11.6,-10.026139656));
#158220=CARTESIAN_POINT('Ctrl Pts',(2.78990638899994,15.2,-10.024974831));
#158221=CARTESIAN_POINT('Ctrl Pts',(2.78990638899994,11.6,-10.024974831));
#158222=CARTESIAN_POINT('Ctrl Pts',(2.78972409599994,15.2,-10.023818961));
#158223=CARTESIAN_POINT('Ctrl Pts',(2.78972409599994,11.6,-10.023818961));
#158224=CARTESIAN_POINT('Ctrl Pts',(2.78954206499994,15.2,-10.022672066));
#158225=CARTESIAN_POINT('Ctrl Pts',(2.78954206499994,11.6,-10.022672066));
#158226=CARTESIAN_POINT('Ctrl Pts',(2.78936031599994,15.2,-10.021534166));
#158227=CARTESIAN_POINT('Ctrl Pts',(2.78936031599994,11.6,-10.021534166));
#158228=CARTESIAN_POINT('Ctrl Pts',(2.78917887099994,15.2,-10.020405284));
#158229=CARTESIAN_POINT('Ctrl Pts',(2.78917887099994,11.6,-10.020405284));
#158230=CARTESIAN_POINT('Ctrl Pts',(2.78899774999994,15.2,-10.019285439));
#158231=CARTESIAN_POINT('Ctrl Pts',(2.78899774999994,11.6,-10.019285439));
#158232=CARTESIAN_POINT('Ctrl Pts',(2.78881697199994,15.2,-10.018174655));
#158233=CARTESIAN_POINT('Ctrl Pts',(2.78881697199994,11.6,-10.018174655));
#158234=CARTESIAN_POINT('Ctrl Pts',(2.78863655799995,15.2,-10.01707295));
#158235=CARTESIAN_POINT('Ctrl Pts',(2.78863655799995,11.6,-10.01707295));
#158236=CARTESIAN_POINT('Ctrl Pts',(2.78845652899995,15.2,-10.015980349));
#158237=CARTESIAN_POINT('Ctrl Pts',(2.78845652899995,11.6,-10.015980349));
#158238=CARTESIAN_POINT('Ctrl Pts',(2.78827690499994,15.2,-10.014896871));
#158239=CARTESIAN_POINT('Ctrl Pts',(2.78827690499994,11.6,-10.014896871));
#158240=CARTESIAN_POINT('Ctrl Pts',(2.78809770599994,15.2,-10.013822539));
#158241=CARTESIAN_POINT('Ctrl Pts',(2.78809770599994,11.6,-10.013822539));
#158242=CARTESIAN_POINT('Ctrl Pts',(2.78791895499995,15.2,-10.012757373));
#158243=CARTESIAN_POINT('Ctrl Pts',(2.78791895499995,11.6,-10.012757373));
#158244=CARTESIAN_POINT('Ctrl Pts',(2.78774067099994,15.2,-10.011701396));
#158245=CARTESIAN_POINT('Ctrl Pts',(2.78774067099994,11.6,-10.011701396));
#158246=CARTESIAN_POINT('Ctrl Pts',(2.78756287699994,15.2,-10.01065463));
#158247=CARTESIAN_POINT('Ctrl Pts',(2.78756287699994,11.6,-10.01065463));
#158248=CARTESIAN_POINT('Ctrl Pts',(2.78738559299994,15.2,-10.009617097));
#158249=CARTESIAN_POINT('Ctrl Pts',(2.78738559299994,11.6,-10.009617097));
#158250=CARTESIAN_POINT('Ctrl Pts',(2.78720883999994,15.2,-10.008588818));
#158251=CARTESIAN_POINT('Ctrl Pts',(2.78720883999994,11.6,-10.008588818));
#158252=CARTESIAN_POINT('Ctrl Pts',(2.78703263999994,15.2,-10.007569815));
#158253=CARTESIAN_POINT('Ctrl Pts',(2.78703263999994,11.6,-10.007569815));
#158254=CARTESIAN_POINT('Ctrl Pts',(2.78685701499994,15.2,-10.006560112));
#158255=CARTESIAN_POINT('Ctrl Pts',(2.78685701499994,11.6,-10.006560112));
#158256=CARTESIAN_POINT('Ctrl Pts',(2.78668198499994,15.2,-10.005559732));
#158257=CARTESIAN_POINT('Ctrl Pts',(2.78668198499994,11.6,-10.005559732));
#158258=CARTESIAN_POINT('Ctrl Pts',(2.78650757299994,15.2,-10.004568694));
#158259=CARTESIAN_POINT('Ctrl Pts',(2.78650757299994,11.6,-10.004568694));
#158260=CARTESIAN_POINT('Ctrl Pts',(2.78633380099994,15.2,-10.003587024));
#158261=CARTESIAN_POINT('Ctrl Pts',(2.78633380099994,11.6,-10.003587024));
#158262=CARTESIAN_POINT('Ctrl Pts',(2.78616069099995,15.2,-10.002614742));
#158263=CARTESIAN_POINT('Ctrl Pts',(2.78616069099995,11.6,-10.002614742));
#158264=CARTESIAN_POINT('Ctrl Pts',(2.78598826499994,15.2,-10.001651872));
#158265=CARTESIAN_POINT('Ctrl Pts',(2.78598826499994,11.6,-10.001651872));
#158266=CARTESIAN_POINT('Ctrl Pts',(2.78581654299995,15.2,-10.000698437));
#158267=CARTESIAN_POINT('Ctrl Pts',(2.78581654299995,11.6,-10.000698437));
#158268=CARTESIAN_POINT('Ctrl Pts',(2.78564555099994,15.2,-9.99975446000001));
#158269=CARTESIAN_POINT('Ctrl Pts',(2.78564555099994,11.6,-9.99975446000001));
#158270=CARTESIAN_POINT('Ctrl Pts',(2.78547531099994,15.2,-9.99881996400001));
#158271=CARTESIAN_POINT('Ctrl Pts',(2.78547531099994,11.6,-9.99881996400001));
#158272=CARTESIAN_POINT('Ctrl Pts',(2.78530584299994,15.2,-9.99789497200001));
#158273=CARTESIAN_POINT('Ctrl Pts',(2.78530584299994,11.6,-9.99789497200001));
#158274=CARTESIAN_POINT('Ctrl Pts',(2.78513717099994,15.2,-9.99697950700001));
#158275=CARTESIAN_POINT('Ctrl Pts',(2.78513717099994,11.6,-9.99697950700001));
#158276=CARTESIAN_POINT('Ctrl Pts',(2.78497028699995,15.2,-9.99607881000001));
#158277=CARTESIAN_POINT('Ctrl Pts',(2.78497028699995,11.6,-9.99607881000001));
#158278=CARTESIAN_POINT('Ctrl Pts',(2.78483763599994,15.2,-9.99536684600001));
#158279=CARTESIAN_POINT('Ctrl Pts',(2.78483763599994,11.6,-9.99536684600001));
#158280=CARTESIAN_POINT('Ctrl Pts',(2.78473876899994,15.2,-9.99483840000001));
#158281=CARTESIAN_POINT('Ctrl Pts',(2.78473876899994,11.6,-9.99483840000001));
#158282=CARTESIAN_POINT('Ctrl Pts',(2.78467334899994,15.2,-9.99448967800001));
#158283=CARTESIAN_POINT('Ctrl Pts',(2.78467334899994,11.6,-9.99448967800001));
#158284=CARTESIAN_POINT('Ctrl Pts',(2.78464115899994,15.2,-9.99431831700001));
#158285=CARTESIAN_POINT('Ctrl Pts',(2.78464115899994,11.6,-9.99431831700001));
#158286=CARTESIAN_POINT('',(2.78464115833177,12.2,-9.99431831666127));
#158287=CARTESIAN_POINT('',(2.78464115833177,15.2,-9.99431831666127));
#158288=CARTESIAN_POINT('',(2.78464115799995,12.2,-9.99431831600001));
#158289=CARTESIAN_POINT('Ctrl Pts',(2.71145515299994,12.2,-11.175777867));
#158290=CARTESIAN_POINT('Ctrl Pts',(2.71227322814856,12.2,-11.1720435063216));
#158291=CARTESIAN_POINT('Ctrl Pts',(2.71308567464298,12.2,-11.1683146746693));
#158292=CARTESIAN_POINT('Ctrl Pts',(2.71389248615398,12.2,-11.1645913879167));
#158293=CARTESIAN_POINT('Ctrl Pts',(2.71469929766498,12.2,-11.1608681011642));
#158294=CARTESIAN_POINT('Ctrl Pts',(2.71550047515118,12.2,-11.1571503540028));
#158295=CARTESIAN_POINT('Ctrl Pts',(2.71629602837101,12.2,-11.1534381629932));
#158296=CARTESIAN_POINT('Ctrl Pts',(2.71709158159084,12.2,-11.1497259719837));
#158297=CARTESIAN_POINT('Ctrl Pts',(2.7178815099234,12.2,-11.1460193377731));
#158298=CARTESIAN_POINT('Ctrl Pts',(2.718665831354,12.2,-11.1423182987818));
#158299=CARTESIAN_POINT('Ctrl Pts',(2.71945015292708,12.2,-11.1386172591182));
#158300=CARTESIAN_POINT('Ctrl Pts',(2.72022886944025,12.2,-11.1349218170144));
#158301=CARTESIAN_POINT('Ctrl Pts',(2.72100200242686,12.2,-11.1312320151873));
#158302=CARTESIAN_POINT('Ctrl Pts',(2.72229055721726,12.2,-11.1250823463691));
#158303=CARTESIAN_POINT('Ctrl Pts',(2.72356360362685,12.2,-11.1189483468318));
#158304=CARTESIAN_POINT('Ctrl Pts',(2.72482121918114,12.2,-11.1128301753747));
#158305=CARTESIAN_POINT('Ctrl Pts',(2.7255757884863,12.2,-11.1091592726339));
#158306=CARTESIAN_POINT('Ctrl Pts',(2.72632480281762,12.2,-11.1054940671912));
#158307=CARTESIAN_POINT('Ctrl Pts',(2.72706828016044,12.2,-11.1018345948087));
#158308=CARTESIAN_POINT('Ctrl Pts',(2.72781175750326,12.2,-11.0981751224262));
#158309=CARTESIAN_POINT('Ctrl Pts',(2.72854969754015,12.2,-11.0945213835527));
#158310=CARTESIAN_POINT('Ctrl Pts',(2.72928212034639,12.2,-11.0908734168108));
#158311=CARTESIAN_POINT('Ctrl Pts',(2.73001454315263,12.2,-11.0872254500688));
#158312=CARTESIAN_POINT('Ctrl Pts',(2.7307414481262,12.2,-11.0835832539512));
#158313=CARTESIAN_POINT('Ctrl Pts',(2.73146285451665,12.2,-11.07994686725));
#158314=CARTESIAN_POINT('Ctrl Pts',(2.73218426090711,12.2,-11.0763104805487));
#158315=CARTESIAN_POINT('Ctrl Pts',(2.73290016921445,12.2,-11.0726799035306));
#158316=CARTESIAN_POINT('Ctrl Pts',(2.73361059710579,12.2,-11.0690551704118));
#158317=CARTESIAN_POINT('Ctrl Pts',(2.73432102499712,12.2,-11.065430437293));
#158318=CARTESIAN_POINT('Ctrl Pts',(2.73502597318777,12.2,-11.0618115499989));
#158319=CARTESIAN_POINT('Ctrl Pts',(2.73572546007293,12.2,-11.0581985437407));
#158320=CARTESIAN_POINT('Ctrl Pts',(2.73642494695809,12.2,-11.0545855374825));
#158321=CARTESIAN_POINT('Ctrl Pts',(2.73711897324081,12.2,-11.050978414405));
#158322=CARTESIAN_POINT('Ctrl Pts',(2.73780755809153,12.2,-11.047377210285));
#158323=CARTESIAN_POINT('Ctrl Pts',(2.73849614306735,12.2,-11.0437760055109));
#158324=CARTESIAN_POINT('Ctrl Pts',(2.73917928739996,12.2,-11.0401807203383));
#158325=CARTESIAN_POINT('Ctrl Pts',(2.73985700941439,12.2,-11.0365913929842));
#158326=CARTESIAN_POINT('Ctrl Pts',(2.74053473130569,12.2,-11.0330020662821));
#158327=CARTESIAN_POINT('Ctrl Pts',(2.74120703188062,12.2,-11.029418696463));
#158328=CARTESIAN_POINT('Ctrl Pts',(2.74187392981425,12.2,-11.0258413208435));
#158329=CARTESIAN_POINT('Ctrl Pts',(2.74254082774788,12.2,-11.022263945224));
#158330=CARTESIAN_POINT('Ctrl Pts',(2.74320232467146,12.2,-11.0186925647334));
#158331=CARTESIAN_POINT('Ctrl Pts',(2.74385843898391,12.2,-11.0151272164717));
#158332=CARTESIAN_POINT('Ctrl Pts',(2.74451455329636,12.2,-11.0115618682101));
#158333=CARTESIAN_POINT('Ctrl Pts',(2.74516528453655,12.2,-11.0080025505236));
#158334=CARTESIAN_POINT('Ctrl Pts',(2.74581065526606,12.2,-11.0044493047615));
#158335=CARTESIAN_POINT('Ctrl Pts',(2.74645602599557,12.2,-11.0008960589995));
#158336=CARTESIAN_POINT('Ctrl Pts',(2.74709603415331,12.2,-10.9973488830412));
#158337=CARTESIAN_POINT('Ctrl Pts',(2.74773070146405,12.2,-10.9938078158361));
#158338=CARTESIAN_POINT('Ctrl Pts',(2.74836536877479,12.2,-10.9902667486308));
#158339=CARTESIAN_POINT('Ctrl Pts',(2.7489946944859,12.2,-10.9867317897085));
#158340=CARTESIAN_POINT('Ctrl Pts',(2.74961869888061,12.2,-10.9832029770443));
#158341=CARTESIAN_POINT('Ctrl Pts',(2.75024270338869,12.2,-10.9796741637389));
#158342=CARTESIAN_POINT('Ctrl Pts',(2.75086138659527,12.2,-10.9761514968936));
#158343=CARTESIAN_POINT('Ctrl Pts',(2.75147477010036,12.2,-10.9726350142167));
#158344=CARTESIAN_POINT('Ctrl Pts',(2.75208815349402,12.2,-10.9691185321786));
#158345=CARTESIAN_POINT('Ctrl Pts',(2.75269623685462,12.2,-10.9656082361236));
#158346=CARTESIAN_POINT('Ctrl Pts',(2.75329904074893,12.2,-10.9621041620848));
#158347=CARTESIAN_POINT('Ctrl Pts',(2.75390184464324,12.2,-10.958600088046));
#158348=CARTESIAN_POINT('Ctrl Pts',(2.75449936965271,12.2,-10.9551022388858));
#158349=CARTESIAN_POINT('Ctrl Pts',(2.75509163696718,12.2,-10.9516106502885));
#158350=CARTESIAN_POINT('Ctrl Pts',(2.75568390428166,12.2,-10.9481190616912));
#158351=CARTESIAN_POINT('Ctrl Pts',(2.75627091386792,12.2,-10.9446337351092));
#158352=CARTESIAN_POINT('Ctrl Pts',(2.75685268580778,12.2,-10.9411547090115));
#158353=CARTESIAN_POINT('Ctrl Pts',(2.75743445774765,12.2,-10.9376756829137));
#158354=CARTESIAN_POINT('Ctrl Pts',(2.75801099402459,12.2,-10.9342029577358));
#158355=CARTESIAN_POINT('Ctrl Pts',(2.75858231446262,12.2,-10.9307365721112));
#158356=CARTESIAN_POINT('Ctrl Pts',(2.75934407511585,12.2,-10.926114724192));
#158357=CARTESIAN_POINT('Ctrl Pts',(2.76009656536241,12.2,-10.921504147024));
#158358=CARTESIAN_POINT('Ctrl Pts',(2.76083983656899,12.2,-10.9169049331074));
#158359=CARTESIAN_POINT('Ctrl Pts',(2.76139728992328,12.2,-10.9134555229833));
#158360=CARTESIAN_POINT('Ctrl Pts',(2.76194955613456,12.2,-10.9100125053209));
#158361=CARTESIAN_POINT('Ctrl Pts',(2.76249665949214,12.2,-10.9065759177635));
#158362=CARTESIAN_POINT('Ctrl Pts',(2.76304376284973,12.2,-10.9031393302061));
#158363=CARTESIAN_POINT('Ctrl Pts',(2.76358570229987,12.2,-10.8997091746276));
#158364=CARTESIAN_POINT('Ctrl Pts',(2.76412250024116,12.2,-10.8962854894864));
#158365=CARTESIAN_POINT('Ctrl Pts',(2.76483823089456,12.2,-10.8917205755502));
#158366=CARTESIAN_POINT('Ctrl Pts',(2.76554482242137,12.2,-10.8871671644149));
#158367=CARTESIAN_POINT('Ctrl Pts',(2.76624232634735,12.2,-10.8826253517241));
#158368=CARTESIAN_POINT('Ctrl Pts',(2.76693983017829,12.2,-10.8780835396521));
#158369=CARTESIAN_POINT('Ctrl Pts',(2.76762824691041,12.2,-10.8735533249536));
#158370=CARTESIAN_POINT('Ctrl Pts',(2.76830763141102,12.2,-10.8690348023778));
#158371=CARTESIAN_POINT('Ctrl Pts',(2.76881716980962,12.2,-10.865645910292));
#158372=CARTESIAN_POINT('Ctrl Pts',(2.76932162752925,12.2,-10.8622635954499));
#158373=CARTESIAN_POINT('Ctrl Pts',(2.76982102791164,12.2,-10.8588878971948));
#158374=CARTESIAN_POINT('Ctrl Pts',(2.77032042829403,12.2,-10.8555121989397));
#158375=CARTESIAN_POINT('Ctrl Pts',(2.77081477072707,12.2,-10.8521431182784));
#158376=CARTESIAN_POINT('Ctrl Pts',(2.77130407866831,12.2,-10.848780694233));
#158377=CARTESIAN_POINT('Ctrl Pts',(2.77179338669844,12.2,-10.8454182695768));
#158378=CARTESIAN_POINT('Ctrl Pts',(2.77227766115215,12.2,-10.842062503039));
#158379=CARTESIAN_POINT('Ctrl Pts',(2.77275692463779,12.2,-10.8387134343032));
#158380=CARTESIAN_POINT('Ctrl Pts',(2.77323618803636,12.2,-10.8353643661758));
#158381=CARTESIAN_POINT('Ctrl Pts',(2.7737104404352,12.2,-10.8320219957314));
#158382=CARTESIAN_POINT('Ctrl Pts',(2.77417970637604,12.2,-10.8286863636448));
#158383=CARTESIAN_POINT('Ctrl Pts',(2.77464897231689,12.2,-10.8253507315583));
#158384=CARTESIAN_POINT('Ctrl Pts',(2.77511325149836,12.2,-10.8220218386413));
#158385=CARTESIAN_POINT('Ctrl Pts',(2.77557256798373,12.2,-10.8186997245386));
#158386=CARTESIAN_POINT('Ctrl Pts',(2.77603188446911,12.2,-10.8153776104359));
#158387=CARTESIAN_POINT('Ctrl Pts',(2.77648623906383,12.2,-10.8120622753145));
#158388=CARTESIAN_POINT('Ctrl Pts',(2.77693565454957,12.2,-10.808753760753));
#158389=CARTESIAN_POINT('Ctrl Pts',(2.77753487525164,12.2,-10.8043424076036));
#158390=CARTESIAN_POINT('Ctrl Pts',(2.77812531728372,12.2,-10.7999431812233));
#158391=CARTESIAN_POINT('Ctrl Pts',(2.77870703737009,12.2,-10.795556176041));
#158392=CARTESIAN_POINT('Ctrl Pts',(2.7792887573772,12.2,-10.7911691714565));
#158393=CARTESIAN_POINT('Ctrl Pts',(2.77986175804655,12.2,-10.7867943903342));
#158394=CARTESIAN_POINT('Ctrl Pts',(2.78042609594543,12.2,-10.7824319303567));
#158395=CARTESIAN_POINT('Ctrl Pts',(2.78099043392119,12.2,-10.7780694697848));
#158396=CARTESIAN_POINT('Ctrl Pts',(2.78154610997291,12.2,-10.7737193301949));
#158397=CARTESIAN_POINT('Ctrl Pts',(2.78209318402931,12.2,-10.7693816108539));
#158398=CARTESIAN_POINT('Ctrl Pts',(2.78264025801118,12.2,-10.765043892104));
#158399=CARTESIAN_POINT('Ctrl Pts',(2.78317873092156,12.2,-10.7607185945176));
#158400=CARTESIAN_POINT('Ctrl Pts',(2.78370866165657,12.2,-10.7564058158693));
#158401=CARTESIAN_POINT('Ctrl Pts',(2.78423859246379,12.2,-10.7520930366335));
#158402=CARTESIAN_POINT('Ctrl Pts',(2.78475998396721,12.2,-10.7477927764963));
#158403=CARTESIAN_POINT('Ctrl Pts',(2.78527289405016,12.2,-10.7435051378746));
#158404=CARTESIAN_POINT('Ctrl Pts',(2.78578580406323,12.2,-10.739217499837));
#158405=CARTESIAN_POINT('Ctrl Pts',(2.78629023460411,12.2,-10.7349424809897));
#158406=CARTESIAN_POINT('Ctrl Pts',(2.78678624847796,12.2,-10.7306801829019));
#158407=CARTESIAN_POINT('Ctrl Pts',(2.78728226241939,12.2,-10.7264178842333));
#158408=CARTESIAN_POINT('Ctrl Pts',(2.78776985765795,12.2,-10.7221683068366));
#158409=CARTESIAN_POINT('Ctrl Pts',(2.78824910023908,12.2,-10.7179315516621));
#158410=CARTESIAN_POINT('Ctrl Pts',(2.78872834275491,12.2,-10.7136947970648));
#158411=CARTESIAN_POINT('Ctrl Pts',(2.78919923138353,12.2,-10.7094708651316));
#158412=CARTESIAN_POINT('Ctrl Pts',(2.78966182945767,12.2,-10.7052598571968));
#158413=CARTESIAN_POINT('Ctrl Pts',(2.79024007709762,12.2,-10.6999960968479));
#158414=CARTESIAN_POINT('Ctrl Pts',(2.79080537129064,12.2,-10.6947525307299));
#158415=CARTESIAN_POINT('Ctrl Pts',(2.79135783965246,12.2,-10.6895293593564));
#158416=CARTESIAN_POINT('Ctrl Pts',(2.79179981436601,12.2,-10.6853508220298));
#158417=CARTESIAN_POINT('Ctrl Pts',(2.79223358019536,12.2,-10.681185338825));
#158418=CARTESIAN_POINT('Ctrl Pts',(2.79265920355136,12.2,-10.6770330117106));
#158419=CARTESIAN_POINT('Ctrl Pts',(2.79308482684937,12.2,-10.6728806851621));
#158420=CARTESIAN_POINT('Ctrl Pts',(2.79350230596012,12.2,-10.6687415149275));
#158421=CARTESIAN_POINT('Ctrl Pts',(2.7939117111497,12.2,-10.6646156057079));
#158422=CARTESIAN_POINT('Ctrl Pts',(2.79432111639506,12.2,-10.6604896959261));
#158423=CARTESIAN_POINT('Ctrl Pts',(2.7947224445076,12.2,-10.6563770470975));
#158424=CARTESIAN_POINT('Ctrl Pts',(2.79511576580858,12.2,-10.6522777640222));
#158425=CARTESIAN_POINT('Ctrl Pts',(2.79550908705596,12.2,-10.6481784815054));
#158426=CARTESIAN_POINT('Ctrl Pts',(2.79589439987109,12.2,-10.6440925658898));
#158427=CARTESIAN_POINT('Ctrl Pts',(2.79627177322994,12.2,-10.6400201206658));
#158428=CARTESIAN_POINT('Ctrl Pts',(2.7966491466402,12.2,-10.635947674887));
#158429=CARTESIAN_POINT('Ctrl Pts',(2.79701858100805,12.2,-10.6318887024788));
#158430=CARTESIAN_POINT('Ctrl Pts',(2.79738014524998,12.2,-10.6278433067583));
#158431=CARTESIAN_POINT('Ctrl Pts',(2.79774170949191,12.2,-10.6237979110378));
#158432=CARTESIAN_POINT('Ctrl Pts',(2.79809540441903,12.2,-10.6197660927828));
#158433=CARTESIAN_POINT('Ctrl Pts',(2.79844130104819,12.2,-10.615747960343));
#158434=CARTESIAN_POINT('Ctrl Pts',(2.79878719763023,12.2,-10.6117298284506));
#158435=CARTESIAN_POINT('Ctrl Pts',(2.79912529445218,12.2,-10.6077253810232));
#158436=CARTESIAN_POINT('Ctrl Pts',(2.79945566448123,12.2,-10.603734727793));
#158437=CARTESIAN_POINT('Ctrl Pts',(2.79995121954731,12.2,-10.5977487476758));
#158438=CARTESIAN_POINT('Ctrl Pts',(2.80042938649863,12.2,-10.5917938013158));
#158439=CARTESIAN_POINT('Ctrl Pts',(2.80089041348305,12.2,-10.5858702563623));
#158440=CARTESIAN_POINT('Ctrl Pts',(2.80119776483392,12.2,-10.5819212260345));
#158441=CARTESIAN_POINT('Ctrl Pts',(2.80149749733683,12.2,-10.5779861525192));
#158442=CARTESIAN_POINT('Ctrl Pts',(2.80178968674164,12.2,-10.57406514475));
#158443=CARTESIAN_POINT('Ctrl Pts',(2.80208187614646,12.2,-10.5701441369807));
#158444=CARTESIAN_POINT('Ctrl Pts',(2.80236651939483,12.2,-10.5662371951992));
#158445=CARTESIAN_POINT('Ctrl Pts',(2.80264369602029,12.2,-10.5623444308218));
#158446=CARTESIAN_POINT('Ctrl Pts',(2.80292087260798,12.2,-10.5584516669749));
#158447=CARTESIAN_POINT('Ctrl Pts',(2.80319057944224,12.2,-10.5545730792043));
#158448=CARTESIAN_POINT('Ctrl Pts',(2.80345289353313,12.2,-10.5507087805026));
#158449=CARTESIAN_POINT('Ctrl Pts',(2.80371520765975,12.2,-10.5468444812744));
#158450=CARTESIAN_POINT('Ctrl Pts',(2.80397012870549,12.2,-10.5429944693582));
#158451=CARTESIAN_POINT('Ctrl Pts',(2.80421773427379,12.2,-10.5391588583728));
#158452=CARTESIAN_POINT('Ctrl Pts',(2.80446533980835,12.2,-10.5353232479101));
#158453=CARTESIAN_POINT('Ctrl Pts',(2.80470562972165,12.2,-10.531502037576));
#158454=CARTESIAN_POINT('Ctrl Pts',(2.80493868248085,12.2,-10.527695341053));
#158455=CARTESIAN_POINT('Ctrl Pts',(2.80528826163553,12.2,-10.521985296009));
#158456=CARTESIAN_POINT('Ctrl Pts',(2.80562155570082,12.2,-10.5163079060207));
#158457=CARTESIAN_POINT('Ctrl Pts',(2.80593883494039,12.2,-10.5106635561402));
#158458=CARTESIAN_POINT('Ctrl Pts',(2.80615035445264,12.2,-10.5069006558781));
#158459=CARTESIAN_POINT('Ctrl Pts',(2.80635475585866,12.2,-10.5031524403812));
#158460=CARTESIAN_POINT('Ctrl Pts',(2.80655212125831,12.2,-10.4994190247333));
#158461=CARTESIAN_POINT('Ctrl Pts',(2.80674948665795,12.2,-10.4956856090854));
#158462=CARTESIAN_POINT('Ctrl Pts',(2.80693981379289,12.2,-10.4919669937559));
#158463=CARTESIAN_POINT('Ctrl Pts',(2.80712318724662,12.2,-10.4882632941111));
#158464=CARTESIAN_POINT('Ctrl Pts',(2.80730656067536,12.2,-10.4845595949709));
#158465=CARTESIAN_POINT('Ctrl Pts',(2.80748297848792,12.2,-10.4808708119328));
#158466=CARTESIAN_POINT('Ctrl Pts',(2.80765252597485,12.2,-10.4771970614941));
#158467=CARTESIAN_POINT('Ctrl Pts',(2.80782207348489,12.2,-10.4735233105549));
#158468=CARTESIAN_POINT('Ctrl Pts',(2.80798475053432,12.2,-10.4698645942013));
#158469=CARTESIAN_POINT('Ctrl Pts',(2.80814063954212,12.2,-10.4662210266709));
#158470=CARTESIAN_POINT('Ctrl Pts',(2.80829652852868,12.2,-10.462577459637));
#158471=CARTESIAN_POINT('Ctrl Pts',(2.8084456315328,12.2,-10.4589490453316));
#158472=CARTESIAN_POINT('Ctrl Pts',(2.8085880325216,12.2,-10.4553358995705));
#158473=CARTESIAN_POINT('Ctrl Pts',(2.8087304335298,12.2,-10.451722753317));
#158474=CARTESIAN_POINT('Ctrl Pts',(2.80886613339742,12.2,-10.4481248778725));
#158475=CARTESIAN_POINT('Ctrl Pts',(2.80899522024367,12.2,-10.4445423902219));
#158476=CARTESIAN_POINT('Ctrl Pts',(2.80912430707232,12.2,-10.4409599030593));
#158477=CARTESIAN_POINT('Ctrl Pts',(2.8092467797467,12.2,-10.4373928068956));
#158478=CARTESIAN_POINT('Ctrl Pts',(2.80936272601543,12.2,-10.4338412210738));
#158479=CARTESIAN_POINT('Ctrl Pts',(2.80947867229995,12.2,-10.4302896347681));
#158480=CARTESIAN_POINT('Ctrl Pts',(2.80958809251425,12.2,-10.4267535579004));
#158481=CARTESIAN_POINT('Ctrl Pts',(2.80969107674166,12.2,-10.423233113654));
#158482=CARTESIAN_POINT('Ctrl Pts',(2.80979406095505,12.2,-10.4197126698872));
#158483=CARTESIAN_POINT('Ctrl Pts',(2.80989060949194,12.2,-10.416207858894));
#158484=CARTESIAN_POINT('Ctrl Pts',(2.80998081121185,12.2,-10.4127188022813));
#158485=CARTESIAN_POINT('Ctrl Pts',(2.81007101294404,12.2,-10.4092297451933));
#158486=CARTESIAN_POINT('Ctrl Pts',(2.81015486936632,12.2,-10.4057564434743));
#158487=CARTESIAN_POINT('Ctrl Pts',(2.81023247298125,12.2,-10.4022990200091));
#158488=CARTESIAN_POINT('Ctrl Pts',(2.81031007658561,12.2,-10.398841597015));
#158489=CARTESIAN_POINT('Ctrl Pts',(2.8103814266579,12.2,-10.395400053215));
#158490=CARTESIAN_POINT('Ctrl Pts',(2.81044661626431,12.2,-10.3919745128267));
#158491=CARTESIAN_POINT('Ctrl Pts',(2.8105118058796,12.2,-10.3885489719717));
#158492=CARTESIAN_POINT('Ctrl Pts',(2.81057083531634,12.2,-10.3851394361035));
#158493=CARTESIAN_POINT('Ctrl Pts',(2.81062379970834,12.2,-10.3817460280143));
#158494=CARTESIAN_POINT('Ctrl Pts',(2.81069000519472,12.2,-10.377504268134));
#158495=CARTESIAN_POINT('Ctrl Pts',(2.81074673386461,12.2,-10.3732877113413));
#158496=CARTESIAN_POINT('Ctrl Pts',(2.81079417275301,12.2,-10.3690966069677));
#158497=CARTESIAN_POINT('Ctrl Pts',(2.81084161164142,12.2,-10.364905502594));
#158498=CARTESIAN_POINT('Ctrl Pts',(2.8108797625634,12.2,-10.3607398474113));
#158499=CARTESIAN_POINT('Ctrl Pts',(2.81090881624348,12.2,-10.356599895746));
#158500=CARTESIAN_POINT('Ctrl Pts',(2.81093786992356,12.2,-10.3524599440807));
#158501=CARTESIAN_POINT('Ctrl Pts',(2.81095782634017,12.2,-10.3483456940834));
#158502=CARTESIAN_POINT('Ctrl Pts',(2.81096888099288,12.2,-10.3442573997838));
#158503=CARTESIAN_POINT('Ctrl Pts',(2.8109799356456,12.2,-10.3401691054842));
#158504=CARTESIAN_POINT('Ctrl Pts',(2.81098208833315,12.2,-10.3361067688644));
#158505=CARTESIAN_POINT('Ctrl Pts',(2.81097553874911,12.2,-10.3320706440054));
#158506=CARTESIAN_POINT('Ctrl Pts',(2.81096898916506,12.2,-10.3280345191464));
#158507=CARTESIAN_POINT('Ctrl Pts',(2.81095373514755,12.2,-10.3240246086045));
#158508=CARTESIAN_POINT('Ctrl Pts',(2.81092998223019,12.2,-10.3200411704123));
#158509=CARTESIAN_POINT('Ctrl Pts',(2.81090622931283,12.2,-10.31605773222));
#158510=CARTESIAN_POINT('Ctrl Pts',(2.81087397636201,12.2,-10.3121007663448));
#158511=CARTESIAN_POINT('Ctrl Pts',(2.81083342948633,12.2,-10.3081705379442));
#158512=CARTESIAN_POINT('Ctrl Pts',(2.81079288261507,12.2,-10.304240309972));
#158513=CARTESIAN_POINT('Ctrl Pts',(2.81074404255054,12.2,-10.3003368164922));
#158514=CARTESIAN_POINT('Ctrl Pts',(2.81068711901574,12.2,-10.2964603255237));
#158515=CARTESIAN_POINT('Ctrl Pts',(2.81063019547474,12.2,-10.2925838341326));
#158516=CARTESIAN_POINT('Ctrl Pts',(2.81056518920885,12.2,-10.2887343451133));
#158517=CARTESIAN_POINT('Ctrl Pts',(2.81049231400116,12.2,-10.2849121277499));
#158518=CARTESIAN_POINT('Ctrl Pts',(2.81041943879347,12.2,-10.2810899103866));
#158519=CARTESIAN_POINT('Ctrl Pts',(2.81033869508631,12.2,-10.2772949636608));
#158520=CARTESIAN_POINT('Ctrl Pts',(2.8102503022352,12.2,-10.2735275611791));
#158521=CARTESIAN_POINT('Ctrl Pts',(2.81016190938409,12.2,-10.2697601586973));
#158522=CARTESIAN_POINT('Ctrl Pts',(2.8100658657063,12.2,-10.2660203007665));
#158523=CARTESIAN_POINT('Ctrl Pts',(2.80996239549835,12.2,-10.2623082627095));
#158524=CARTESIAN_POINT('Ctrl Pts',(2.80985892529041,12.2,-10.2585962246525));
#158525=CARTESIAN_POINT('Ctrl Pts',(2.80974802821282,12.2,-10.2549120077462));
#158526=CARTESIAN_POINT('Ctrl Pts',(2.80962993224098,12.2,-10.2512558882309));
#158527=CARTESIAN_POINT('Ctrl Pts',(2.80951183626913,12.2,-10.2475997687155));
#158528=CARTESIAN_POINT('Ctrl Pts',(2.80938654093395,12.2,-10.2439717513294));
#158529=CARTESIAN_POINT('Ctrl Pts',(2.8092542767667,12.2,-10.2403721149936));
#158530=CARTESIAN_POINT('Ctrl Pts',(2.80912201259945,12.2,-10.2367724786577));
#158531=CARTESIAN_POINT('Ctrl Pts',(2.80898278167219,12.2,-10.233201226061));
#158532=CARTESIAN_POINT('Ctrl Pts',(2.80883681924163,12.2,-10.2296586422416));
#158533=CARTESIAN_POINT('Ctrl Pts',(2.80869085681107,12.2,-10.2261160584222));
#158534=CARTESIAN_POINT('Ctrl Pts',(2.80853816385061,12.2,-10.2226021452027));
#158535=CARTESIAN_POINT('Ctrl Pts',(2.80837898051654,12.2,-10.219117191298));
#158536=CARTESIAN_POINT('Ctrl Pts',(2.80821979718247,12.2,-10.2156322373934));
#158537=CARTESIAN_POINT('Ctrl Pts',(2.80805412412789,12.2,-10.2121762447245));
#158538=CARTESIAN_POINT('Ctrl Pts',(2.80788220669701,12.2,-10.2087495068093));
#158539=CARTESIAN_POINT('Ctrl Pts',(2.80771028926613,12.2,-10.2053227688942));
#158540=CARTESIAN_POINT('Ctrl Pts',(2.80753212788264,12.2,-10.2019252858283));
#158541=CARTESIAN_POINT('Ctrl Pts',(2.80734797447955,12.2,-10.1985573562465));
#158542=CARTESIAN_POINT('Ctrl Pts',(2.80716382107645,12.2,-10.1951894266647));
#158543=CARTESIAN_POINT('Ctrl Pts',(2.80697367425405,12.2,-10.1918510513959));
#158544=CARTESIAN_POINT('Ctrl Pts',(2.80677779174387,12.2,-10.1885425331076));
#158545=CARTESIAN_POINT('Ctrl Pts',(2.8065035562467,12.2,-10.1839106077926));
#158546=CARTESIAN_POINT('Ctrl Pts',(2.80621807528634,12.2,-10.1793371986607));
#158547=CARTESIAN_POINT('Ctrl Pts',(2.80592207223594,12.2,-10.1748231558967));
#158548=CARTESIAN_POINT('Ctrl Pts',(2.80566835530597,12.2,-10.1709539759328));
#158549=CARTESIAN_POINT('Ctrl Pts',(2.80540690715243,12.2,-10.1671284092933));
#158550=CARTESIAN_POINT('Ctrl Pts',(2.80513819345728,12.2,-10.1633470004009));
#158551=CARTESIAN_POINT('Ctrl Pts',(2.80486947978653,12.2,-10.159565591852));
#158552=CARTESIAN_POINT('Ctrl Pts',(2.80459350390635,12.2,-10.1558283400574));
#158553=CARTESIAN_POINT('Ctrl Pts',(2.80431073924996,12.2,-10.1521357977749));
#158554=CARTESIAN_POINT('Ctrl Pts',(2.80402797459357,12.2,-10.1484432554925));
#158555=CARTESIAN_POINT('Ctrl Pts',(2.8037384244489,12.2,-10.1447954232169));
#158556=CARTESIAN_POINT('Ctrl Pts',(2.80344257777856,12.2,-10.1411928618319));
#158557=CARTESIAN_POINT('Ctrl Pts',(2.80314673108135,12.2,-10.1375903001196));
#158558=CARTESIAN_POINT('Ctrl Pts',(2.80284458940023,12.2,-10.1340330103888));
#158559=CARTESIAN_POINT('Ctrl Pts',(2.80253665471639,12.2,-10.1305215658672));
#158560=CARTESIAN_POINT('Ctrl Pts',(2.80222872006052,12.2,-10.1270101216646));
#158561=CARTESIAN_POINT('Ctrl Pts',(2.80191499338134,12.2,-10.1235445211729));
#158562=CARTESIAN_POINT('Ctrl Pts',(2.80159599080814,12.2,-10.1201253499484));
#158563=CARTESIAN_POINT('Ctrl Pts',(2.80127698823494,12.2,-10.1167061787239));
#158564=CARTESIAN_POINT('Ctrl Pts',(2.80095270991403,12.2,-10.1133334348042));
#158565=CARTESIAN_POINT('Ctrl Pts',(2.80062368650953,12.2,-10.110007715673));
#158566=CARTESIAN_POINT('Ctrl Pts',(2.80029466307514,12.2,-10.1066819962398));
#158567=CARTESIAN_POINT('Ctrl Pts',(2.79996089519015,12.2,-10.1034032999539));
#158568=CARTESIAN_POINT('Ctrl Pts',(2.79962292675478,12.2,-10.1001722346144));
#158569=CARTESIAN_POINT('Ctrl Pts',(2.79928495835011,12.2,-10.0969411695684));
#158570=CARTESIAN_POINT('Ctrl Pts',(2.79894278918881,12.2,-10.0937577355654));
#158571=CARTESIAN_POINT('Ctrl Pts',(2.79859698069979,12.2,-10.0906225524985));
#158572=CARTESIAN_POINT('Ctrl Pts',(2.79825117221078,12.2,-10.0874873694316));
#158573=CARTESIAN_POINT('Ctrl Pts',(2.79790172196454,12.2,-10.0844004344241));
#158574=CARTESIAN_POINT('Ctrl Pts',(2.79754920772748,12.2,-10.0813623843657));
#158575=CARTESIAN_POINT('Ctrl Pts',(2.7971966934584,12.2,-10.0783243340313));
#158576=CARTESIAN_POINT('Ctrl Pts',(2.79684111459727,12.2,-10.0753351655114));
#158577=CARTESIAN_POINT('Ctrl Pts',(2.79648306141092,12.2,-10.0723955254378));
#158578=CARTESIAN_POINT('Ctrl Pts',(2.79612500825709,12.2,-10.0694558856314));
#158579=CARTESIAN_POINT('Ctrl Pts',(2.79576448225877,12.2,-10.06656577444));
#158580=CARTESIAN_POINT('Ctrl Pts',(2.79540209102186,12.2,-10.0637258525454));
#158581=CARTESIAN_POINT('Ctrl Pts',(2.79503969978494,12.2,-10.0608859306507));
#158582=CARTESIAN_POINT('Ctrl Pts',(2.79467544327319,12.2,-10.0580961963021));
#158583=CARTESIAN_POINT('Ctrl Pts',(2.79430994728653,12.2,-10.0553573263994));
#158584=CARTESIAN_POINT('Ctrl Pts',(2.79394445129987,12.2,-10.0526184564967));
#158585=CARTESIAN_POINT('Ctrl Pts',(2.79357771622659,12.2,-10.0499304478117));
#158586=CARTESIAN_POINT('Ctrl Pts',(2.79321038707332,12.2,-10.0472939940706));
#158587=CARTESIAN_POINT('Ctrl Pts',(2.79284305788667,12.2,-10.0446575400901));
#158588=CARTESIAN_POINT('Ctrl Pts',(2.79247513274161,12.2,-10.0420726393062));
#158589=CARTESIAN_POINT('Ctrl Pts',(2.79210727597156,12.2,-10.0395399975871));
#158590=CARTESIAN_POINT('Ctrl Pts',(2.79173941923493,12.2,-10.0370073560981));
#158591=CARTESIAN_POINT('Ctrl Pts',(2.79137163194678,12.2,-10.034526975124));
#158592=CARTESIAN_POINT('Ctrl Pts',(2.79100459704178,12.2,-10.0320995765344));
#158593=CARTESIAN_POINT('Ctrl Pts',(2.79063756213678,12.2,-10.0296721779447));
#158594=CARTESIAN_POINT('Ctrl Pts',(2.79027127675155,12.2,-10.0272977614972));
#158595=CARTESIAN_POINT('Ctrl Pts',(2.78990645001471,12.2,-10.0249770699946));
#158596=CARTESIAN_POINT('Ctrl Pts',(2.78954162324473,12.2,-10.0226563782811));
#158597=CARTESIAN_POINT('Ctrl Pts',(2.78917825150261,12.2,-10.020389410239));
#158598=CARTESIAN_POINT('Ctrl Pts',(2.78881706296501,12.2,-10.0181769245944));
#158599=CARTESIAN_POINT('Ctrl Pts',(2.78845587446021,12.2,-10.0159644391507));
#158600=CARTESIAN_POINT('Ctrl Pts',(2.78809686787867,12.2,-10.0138064380068));
#158601=CARTESIAN_POINT('Ctrl Pts',(2.78774079347494,12.2,-10.0117036987499));
#158602=CARTESIAN_POINT('Ctrl Pts',(2.78738471907121,12.2,-10.009600959493));
#158603=CARTESIAN_POINT('Ctrl Pts',(2.78703157778039,12.2,-10.0075534820314));
#158604=CARTESIAN_POINT('Ctrl Pts',(2.78668213952542,12.2,-10.005562067751));
#158605=CARTESIAN_POINT('Ctrl Pts',(2.7863327012387,12.2,-10.0035706532898));
#158606=CARTESIAN_POINT('Ctrl Pts',(2.78598696746437,12.2,-10.0016352993104));
#158607=CARTESIAN_POINT('Ctrl Pts',(2.78564573894608,12.2,-9.99975683004517));
#158608=CARTESIAN_POINT('Ctrl Pts',(2.78530614810647,12.2,-9.99788737623124));
#158609=CARTESIAN_POINT('Ctrl Pts',(2.78497101114222,12.2,-9.99607425962044));
#158610=CARTESIAN_POINT('Ctrl Pts',(2.78464115899994,12.2,-9.99431831700001));
#158611=CARTESIAN_POINT('Ctrl Pts',(2.78464115899994,15.2,-9.99431831700001));
#158612=CARTESIAN_POINT('Ctrl Pts',(2.78497101114222,15.2,-9.99607425962044));
#158613=CARTESIAN_POINT('Ctrl Pts',(2.78530614810647,15.2,-9.99788737623122));
#158614=CARTESIAN_POINT('Ctrl Pts',(2.78564573894608,15.2,-9.99975683004517));
#158615=CARTESIAN_POINT('Ctrl Pts',(2.78598696746438,15.2,-10.0016352993104));
#158616=CARTESIAN_POINT('Ctrl Pts',(2.7863327012387,15.2,-10.0035706532898));
#158617=CARTESIAN_POINT('Ctrl Pts',(2.78668213952542,15.2,-10.005562067751));
#158618=CARTESIAN_POINT('Ctrl Pts',(2.78703157778039,15.2,-10.0075534820314));
#158619=CARTESIAN_POINT('Ctrl Pts',(2.78738471907121,15.2,-10.009600959493));
#158620=CARTESIAN_POINT('Ctrl Pts',(2.78774079347494,15.2,-10.0117036987499));
#158621=CARTESIAN_POINT('Ctrl Pts',(2.78809686787867,15.2,-10.0138064380068));
#158622=CARTESIAN_POINT('Ctrl Pts',(2.78845587446022,15.2,-10.0159644391507));
#158623=CARTESIAN_POINT('Ctrl Pts',(2.78881706296501,15.2,-10.0181769245944));
#158624=CARTESIAN_POINT('Ctrl Pts',(2.7891782515026,15.2,-10.0203894102389));
#158625=CARTESIAN_POINT('Ctrl Pts',(2.78954162324472,15.2,-10.0226563782811));
#158626=CARTESIAN_POINT('Ctrl Pts',(2.78990645001471,15.2,-10.0249770699945));
#158627=CARTESIAN_POINT('Ctrl Pts',(2.79027127675155,15.2,-10.0272977614972));
#158628=CARTESIAN_POINT('Ctrl Pts',(2.79063756213678,15.2,-10.0296721779447));
#158629=CARTESIAN_POINT('Ctrl Pts',(2.79100459704178,15.2,-10.0320995765344));
#158630=CARTESIAN_POINT('Ctrl Pts',(2.79137163194678,15.2,-10.034526975124));
#158631=CARTESIAN_POINT('Ctrl Pts',(2.79173941923493,15.2,-10.0370073560981));
#158632=CARTESIAN_POINT('Ctrl Pts',(2.79210727597156,15.2,-10.0395399975871));
#158633=CARTESIAN_POINT('Ctrl Pts',(2.79247513274161,15.2,-10.0420726393062));
#158634=CARTESIAN_POINT('Ctrl Pts',(2.79284305788667,15.2,-10.0446575400901));
#158635=CARTESIAN_POINT('Ctrl Pts',(2.79321038707332,15.2,-10.0472939940706));
#158636=CARTESIAN_POINT('Ctrl Pts',(2.79357771622659,15.2,-10.0499304478117));
#158637=CARTESIAN_POINT('Ctrl Pts',(2.79394445129986,15.2,-10.0526184564967));
#158638=CARTESIAN_POINT('Ctrl Pts',(2.79430994728653,15.2,-10.0553573263994));
#158639=CARTESIAN_POINT('Ctrl Pts',(2.79467544327319,15.2,-10.0580961963021));
#158640=CARTESIAN_POINT('Ctrl Pts',(2.79503969978494,15.2,-10.0608859306507));
#158641=CARTESIAN_POINT('Ctrl Pts',(2.79540209102186,15.2,-10.0637258525454));
#158642=CARTESIAN_POINT('Ctrl Pts',(2.79576448225877,15.2,-10.06656577444));
#158643=CARTESIAN_POINT('Ctrl Pts',(2.79612500825709,15.2,-10.0694558856313));
#158644=CARTESIAN_POINT('Ctrl Pts',(2.79648306141092,15.2,-10.0723955254378));
#158645=CARTESIAN_POINT('Ctrl Pts',(2.79684111459727,15.2,-10.0753351655114));
#158646=CARTESIAN_POINT('Ctrl Pts',(2.7971966934584,15.2,-10.0783243340313));
#158647=CARTESIAN_POINT('Ctrl Pts',(2.79754920772748,15.2,-10.0813623843657));
#158648=CARTESIAN_POINT('Ctrl Pts',(2.79790172196454,15.2,-10.0844004344241));
#158649=CARTESIAN_POINT('Ctrl Pts',(2.79825117221078,15.2,-10.0874873694316));
#158650=CARTESIAN_POINT('Ctrl Pts',(2.79859698069979,15.2,-10.0906225524985));
#158651=CARTESIAN_POINT('Ctrl Pts',(2.79894278918881,15.2,-10.0937577355654));
#158652=CARTESIAN_POINT('Ctrl Pts',(2.79928495835011,15.2,-10.0969411695684));
#158653=CARTESIAN_POINT('Ctrl Pts',(2.79962292675478,15.2,-10.1001722346144));
#158654=CARTESIAN_POINT('Ctrl Pts',(2.80001722324736,15.2,-10.1039418106971));
#158655=CARTESIAN_POINT('Ctrl Pts',(2.80040580174256,15.2,-10.1077762165708));
#158656=CARTESIAN_POINT('Ctrl Pts',(2.80078780049875,15.2,-10.1116744910597));
#158657=CARTESIAN_POINT('Ctrl Pts',(2.80111522798707,15.2,-10.1150158690196));
#158658=CARTESIAN_POINT('Ctrl Pts',(2.80143782025987,15.2,-10.1184041698702));
#158659=CARTESIAN_POINT('Ctrl Pts',(2.80175504991537,15.2,-10.1218388019089));
#158660=CARTESIAN_POINT('Ctrl Pts',(2.80207227959969,15.2,-10.1252734342596));
#158661=CARTESIAN_POINT('Ctrl Pts',(2.80238414665852,15.2,-10.1287543959148));
#158662=CARTESIAN_POINT('Ctrl Pts',(2.80269013725827,15.2,-10.1322811064423));
#158663=CARTESIAN_POINT('Ctrl Pts',(2.80299612783023,15.2,-10.1358078166495));
#158664=CARTESIAN_POINT('Ctrl Pts',(2.80329623959247,15.2,-10.1393802760467));
#158665=CARTESIAN_POINT('Ctrl Pts',(2.80358997424982,15.2,-10.142997912265));
#158666=CARTESIAN_POINT('Ctrl Pts',(2.80388370890717,15.2,-10.1466155484832));
#158667=CARTESIAN_POINT('Ctrl Pts',(2.80417106491244,15.2,-10.1502783615419));
#158668=CARTESIAN_POINT('Ctrl Pts',(2.80445155373605,15.2,-10.1539857918208));
#158669=CARTESIAN_POINT('Ctrl Pts',(2.80473204258513,15.2,-10.1576932224365));
#158670=CARTESIAN_POINT('Ctrl Pts',(2.80500566394831,15.2,-10.1614452697015));
#158671=CARTESIAN_POINT('Ctrl Pts',(2.80527194280903,15.2,-10.1652413826006));
#158672=CARTESIAN_POINT('Ctrl Pts',(2.80558260144359,15.2,-10.1696701804656));
#158673=CARTESIAN_POINT('Ctrl Pts',(2.80588326473474,15.2,-10.1741589572228));
#158674=CARTESIAN_POINT('Ctrl Pts',(2.8061731954812,15.2,-10.1787068541167));
#158675=CARTESIAN_POINT('Ctrl Pts',(2.80646312625024,15.2,-10.1832547513646));
#158676=CARTESIAN_POINT('Ctrl Pts',(2.80674232779444,15.2,-10.1878617700155));
#158677=CARTESIAN_POINT('Ctrl Pts',(2.80701008129985,15.2,-10.1925270677898));
#158678=CARTESIAN_POINT('Ctrl Pts',(2.80720133380074,15.2,-10.1958594232909));
#158679=CARTESIAN_POINT('Ctrl Pts',(2.80738674656107,15.2,-10.1992215137888));
#158680=CARTESIAN_POINT('Ctrl Pts',(2.80756606649163,15.2,-10.2026130384416));
#158681=CARTESIAN_POINT('Ctrl Pts',(2.80778125040047,15.2,-10.2066828678771));
#158682=CARTESIAN_POINT('Ctrl Pts',(2.80798765826097,15.2,-10.2107950804107));
#158683=CARTESIAN_POINT('Ctrl Pts',(2.80818486126419,15.2,-10.2149491661315));
#158684=CARTESIAN_POINT('Ctrl Pts',(2.80834919710618,15.2,-10.218410904358));
#158685=CARTESIAN_POINT('Ctrl Pts',(2.80850714112857,15.2,-10.2219017213103));
#158686=CARTESIAN_POINT('Ctrl Pts',(2.80865844953169,15.2,-10.2254213220033));
#158687=CARTESIAN_POINT('Ctrl Pts',(2.80880975793482,15.2,-10.2289409226962));
#158688=CARTESIAN_POINT('Ctrl Pts',(2.8089544304461,15.2,-10.2324893096455));
#158689=CARTESIAN_POINT('Ctrl Pts',(2.80909223051591,15.2,-10.2360661935328));
#158690=CARTESIAN_POINT('Ctrl Pts',(2.80923003058571,15.2,-10.2396430774202));
#158691=CARTESIAN_POINT('Ctrl Pts',(2.80936095711598,15.2,-10.2432484583982));
#158692=CARTESIAN_POINT('Ctrl Pts',(2.80948477628323,15.2,-10.2468820515396));
#158693=CARTESIAN_POINT('Ctrl Pts',(2.80960859545047,15.2,-10.2505156446811));
#158694=CARTESIAN_POINT('Ctrl Pts',(2.80972530584441,15.2,-10.2541774506333));
#158695=CARTESIAN_POINT('Ctrl Pts',(2.8098346809833,15.2,-10.2578671885499));
#158696=CARTESIAN_POINT('Ctrl Pts',(2.80994405612218,15.2,-10.2615569264666));
#158697=CARTESIAN_POINT('Ctrl Pts',(2.81004609506072,15.2,-10.2652745939627));
#158698=CARTESIAN_POINT('Ctrl Pts',(2.81014057270001,15.2,-10.2690199170353));
#158699=CARTESIAN_POINT('Ctrl Pts',(2.81023505033931,15.2,-10.2727652401079));
#158700=CARTESIAN_POINT('Ctrl Pts',(2.81032196679439,15.2,-10.2765382167139));
#158701=CARTESIAN_POINT('Ctrl Pts',(2.81040110123842,15.2,-10.280338574007));
#158702=CARTESIAN_POINT('Ctrl Pts',(2.81048023568246,15.2,-10.2841389313001));
#158703=CARTESIAN_POINT('Ctrl Pts',(2.81055158974336,15.2,-10.2879666677897));
#158704=CARTESIAN_POINT('Ctrl Pts',(2.81061494502073,15.2,-10.2918215143189));
#158705=CARTESIAN_POINT('Ctrl Pts',(2.81067830029809,15.2,-10.2956763608481));
#158706=CARTESIAN_POINT('Ctrl Pts',(2.81073365849251,15.2,-10.2995583151622));
#158707=CARTESIAN_POINT('Ctrl Pts',(2.81078080627208,15.2,-10.3034671141788));
#158708=CARTESIAN_POINT('Ctrl Pts',(2.81082795405164,15.2,-10.3073759131954));
#158709=CARTESIAN_POINT('Ctrl Pts',(2.81086689178798,15.2,-10.3113115518994));
#158710=CARTESIAN_POINT('Ctrl Pts',(2.81089741199562,15.2,-10.3152737700265));
#158711=CARTESIAN_POINT('Ctrl Pts',(2.81092793220327,15.2,-10.3192359881537));
#158712=CARTESIAN_POINT('Ctrl Pts',(2.81095003460243,15.2,-10.323224782873));
#158713=CARTESIAN_POINT('Ctrl Pts',(2.81096351418506,15.2,-10.3272398945418));
#158714=CARTESIAN_POINT('Ctrl Pts',(2.81097968968363,15.2,-10.3320580283693));
#158715=CARTESIAN_POINT('Ctrl Pts',(2.81098344974971,15.2,-10.3369140588243));
#158716=CARTESIAN_POINT('Ctrl Pts',(2.81097444724996,15.2,-10.3418075405022));
#158717=CARTESIAN_POINT('Ctrl Pts',(2.81096544475022,15.2,-10.34670102218));
#158718=CARTESIAN_POINT('Ctrl Pts',(2.81094368065831,15.2,-10.3516319539281));
#158719=CARTESIAN_POINT('Ctrl Pts',(2.81090881624348,15.2,-10.356599895746));
#158720=CARTESIAN_POINT('Ctrl Pts',(2.8108797625634,15.2,-10.3607398474113));
#158721=CARTESIAN_POINT('Ctrl Pts',(2.81084161164142,15.2,-10.364905502594));
#158722=CARTESIAN_POINT('Ctrl Pts',(2.81079417275301,15.2,-10.3690966069677));
#158723=CARTESIAN_POINT('Ctrl Pts',(2.81075622164022,15.2,-10.3724494906494));
#158724=CARTESIAN_POINT('Ctrl Pts',(2.81071232573732,15.2,-10.3758186640001));
#158725=CARTESIAN_POINT('Ctrl Pts',(2.81066238750935,15.2,-10.3792039989663));
#158726=CARTESIAN_POINT('Ctrl Pts',(2.8106124492882,15.2,-10.3825893334712));
#158727=CARTESIAN_POINT('Ctrl Pts',(2.81055646986062,15.2,-10.3859908288178));
#158728=CARTESIAN_POINT('Ctrl Pts',(2.81049435475499,15.2,-10.3894083592041));
#158729=CARTESIAN_POINT('Ctrl Pts',(2.8104167108666,15.2,-10.3936802725361));
#158730=CARTESIAN_POINT('Ctrl Pts',(2.81032947749463,15.2,-10.3979772409132));
#158731=CARTESIAN_POINT('Ctrl Pts',(2.81023247298125,15.2,-10.4022990200091));
#158732=CARTESIAN_POINT('Ctrl Pts',(2.81015486936632,15.2,-10.4057564434743));
#158733=CARTESIAN_POINT('Ctrl Pts',(2.81007101294404,15.2,-10.4092297451933));
#158734=CARTESIAN_POINT('Ctrl Pts',(2.80998081121184,15.2,-10.4127188022813));
#158735=CARTESIAN_POINT('Ctrl Pts',(2.80989060949194,15.2,-10.416207858894));
#158736=CARTESIAN_POINT('Ctrl Pts',(2.80979406095505,15.2,-10.4197126698872));
#158737=CARTESIAN_POINT('Ctrl Pts',(2.80969107674166,15.2,-10.423233113654));
#158738=CARTESIAN_POINT('Ctrl Pts',(2.80958809251425,15.2,-10.4267535579004));
#158739=CARTESIAN_POINT('Ctrl Pts',(2.80947867229995,15.2,-10.4302896347681));
#158740=CARTESIAN_POINT('Ctrl Pts',(2.80936272601543,15.2,-10.4338412210738));
#158741=CARTESIAN_POINT('Ctrl Pts',(2.8092467797467,15.2,-10.4373928068955));
#158742=CARTESIAN_POINT('Ctrl Pts',(2.80912430707232,15.2,-10.4409599030593));
#158743=CARTESIAN_POINT('Ctrl Pts',(2.80899522024367,15.2,-10.4445423902219));
#158744=CARTESIAN_POINT('Ctrl Pts',(2.80886613339742,15.2,-10.4481248778725));
#158745=CARTESIAN_POINT('Ctrl Pts',(2.8087304335298,15.2,-10.451722753317));
#158746=CARTESIAN_POINT('Ctrl Pts',(2.8085880325216,15.2,-10.4553358995705));
#158747=CARTESIAN_POINT('Ctrl Pts',(2.8084456315328,15.2,-10.4589490453316));
#158748=CARTESIAN_POINT('Ctrl Pts',(2.80829652852868,15.2,-10.462577459637));
#158749=CARTESIAN_POINT('Ctrl Pts',(2.80814063954212,15.2,-10.4662210266709));
#158750=CARTESIAN_POINT('Ctrl Pts',(2.80798475053432,15.2,-10.4698645942013));
#158751=CARTESIAN_POINT('Ctrl Pts',(2.80782207348489,15.2,-10.473523310555));
#158752=CARTESIAN_POINT('Ctrl Pts',(2.80765252597486,15.2,-10.4771970614941));
#158753=CARTESIAN_POINT('Ctrl Pts',(2.80748297848792,15.2,-10.4808708119328));
#158754=CARTESIAN_POINT('Ctrl Pts',(2.80730656067536,15.2,-10.4845595949709));
#158755=CARTESIAN_POINT('Ctrl Pts',(2.80712318724662,15.2,-10.4882632941111));
#158756=CARTESIAN_POINT('Ctrl Pts',(2.80693981379289,15.2,-10.4919669937559));
#158757=CARTESIAN_POINT('Ctrl Pts',(2.80674948665795,15.2,-10.4956856090854));
#158758=CARTESIAN_POINT('Ctrl Pts',(2.80655212125831,15.2,-10.4994190247333));
#158759=CARTESIAN_POINT('Ctrl Pts',(2.80635475585866,15.2,-10.5031524403812));
#158760=CARTESIAN_POINT('Ctrl Pts',(2.80615035445264,15.2,-10.5069006558781));
#158761=CARTESIAN_POINT('Ctrl Pts',(2.80593883494039,15.2,-10.5106635561402));
#158762=CARTESIAN_POINT('Ctrl Pts',(2.80572731545695,15.2,-10.5144264558896));
#158763=CARTESIAN_POINT('Ctrl Pts',(2.80550867889378,15.2,-10.5182040404485));
#158764=CARTESIAN_POINT('Ctrl Pts',(2.80528284346679,15.2,-10.521996194989));
#158765=CARTESIAN_POINT('Ctrl Pts',(2.80505700800904,15.2,-10.5257883500462));
#158766=CARTESIAN_POINT('Ctrl Pts',(2.80482397523285,15.2,-10.5295950755067));
#158767=CARTESIAN_POINT('Ctrl Pts',(2.80458366571901,15.2,-10.5334162578831));
#158768=CARTESIAN_POINT('Ctrl Pts',(2.80434335623791,15.2,-10.5372374397388));
#158769=CARTESIAN_POINT('Ctrl Pts',(2.80409576967998,15.2,-10.5410730777566));
#158770=CARTESIAN_POINT('Ctrl Pts',(2.80384082897908,15.2,-10.5449230608854));
#158771=CARTESIAN_POINT('Ctrl Pts',(2.80358588824344,15.2,-10.5487730445387));
#158772=CARTESIAN_POINT('Ctrl Pts',(2.80332359330906,15.2,-10.5526373721259));
#158773=CARTESIAN_POINT('Ctrl Pts',(2.80305386766913,15.2,-10.5565159325878));
#158774=CARTESIAN_POINT('Ctrl Pts',(2.80278414206595,15.2,-10.5603944925213));
#158775=CARTESIAN_POINT('Ctrl Pts',(2.8025069841383,15.2,-10.5642872834288));
#158776=CARTESIAN_POINT('Ctrl Pts',(2.80222232127317,15.2,-10.568194196664));
#158777=CARTESIAN_POINT('Ctrl Pts',(2.80193765836926,15.2,-10.5721011104316));
#158778=CARTESIAN_POINT('Ctrl Pts',(2.80164548692001,15.2,-10.5760221462147));
#158779=CARTESIAN_POINT('Ctrl Pts',(2.80134573545873,15.2,-10.5799571925968));
#158780=CARTESIAN_POINT('Ctrl Pts',(2.8010459840383,15.2,-10.5838922384427));
#158781=CARTESIAN_POINT('Ctrl Pts',(2.80073865119051,15.2,-10.5878412950827));
#158782=CARTESIAN_POINT('Ctrl Pts',(2.80042366431231,15.2,-10.5918042539));
#158783=CARTESIAN_POINT('Ctrl Pts',(2.80002993068235,15.2,-10.5967579528265));
#158784=CARTESIAN_POINT('Ctrl Pts',(2.79962423458771,15.2,-10.6017333720522));
#158785=CARTESIAN_POINT('Ctrl Pts',(2.79920643701889,15.2,-10.60673030219));
#158786=CARTESIAN_POINT('Ctrl Pts',(2.79878863945008,15.2,-10.6117272323277));
#158787=CARTESIAN_POINT('Ctrl Pts',(2.79835873998929,15.2,-10.6167456710605));
#158788=CARTESIAN_POINT('Ctrl Pts',(2.79791659908715,15.2,-10.6217854096705));
#158789=CARTESIAN_POINT('Ctrl Pts',(2.79756288634616,15.2,-10.6258172007782));
#158790=CARTESIAN_POINT('Ctrl Pts',(2.79720133915979,15.2,-10.629862623057));
#158791=CARTESIAN_POINT('Ctrl Pts',(2.7968318871947,15.2,-10.6339215695569));
#158792=CARTESIAN_POINT('Ctrl Pts',(2.79646243527994,15.2,-10.6379805155037));
#158793=CARTESIAN_POINT('Ctrl Pts',(2.79608507960679,15.2,-10.6420529884215));
#158794=CARTESIAN_POINT('Ctrl Pts',(2.79569974956418,15.2,-10.6461388779571));
#158795=CARTESIAN_POINT('Ctrl Pts',(2.79531441946906,15.2,-10.6502247680494));
#158796=CARTESIAN_POINT('Ctrl Pts',(2.79492111494227,15.2,-10.6543240776252));
#158797=CARTESIAN_POINT('Ctrl Pts',(2.79451976997542,15.2,-10.658436700128));
#158798=CARTESIAN_POINT('Ctrl Pts',(2.79411842506326,15.2,-10.6625493220704));
#158799=CARTESIAN_POINT('Ctrl Pts',(2.7937090362805,15.2,-10.6666752574268));
#158800=CARTESIAN_POINT('Ctrl Pts',(2.79329153959323,15.2,-10.6708144013649));
#158801=CARTESIAN_POINT('Ctrl Pts',(2.79287404284908,15.2,-10.6749535458669));
#158802=CARTESIAN_POINT('Ctrl Pts',(2.79244843563643,15.2,-10.6791058987179));
#158803=CARTESIAN_POINT('Ctrl Pts',(2.79201465349968,15.2,-10.6832713565195));
#158804=CARTESIAN_POINT('Ctrl Pts',(2.79158087142203,15.2,-10.6874368137535));
#158805=CARTESIAN_POINT('Ctrl Pts',(2.79113891289982,15.2,-10.6916153767586));
#158806=CARTESIAN_POINT('Ctrl Pts',(2.79068871354858,15.2,-10.6958069400813));
#158807=CARTESIAN_POINT('Ctrl Pts',(2.79023851413599,15.2,-10.6999985039751));
#158808=CARTESIAN_POINT('Ctrl Pts',(2.78978007311709,15.2,-10.7042030703534));
#158809=CARTESIAN_POINT('Ctrl Pts',(2.78931332525831,15.2,-10.70842053425));
#158810=CARTESIAN_POINT('Ctrl Pts',(2.78884657739954,15.2,-10.7126379981465));
#158811=CARTESIAN_POINT('Ctrl Pts',(2.78837152399258,15.2,-10.7168683615917));
#158812=CARTESIAN_POINT('Ctrl Pts',(2.7878881011876,15.2,-10.7211115214354));
#158813=CARTESIAN_POINT('Ctrl Pts',(2.78740467844849,15.2,-10.7253546807009));
#158814=CARTESIAN_POINT('Ctrl Pts',(2.786912884895,15.2,-10.7296106377989));
#158815=CARTESIAN_POINT('Ctrl Pts',(2.78641265893365,15.2,-10.7338792892471));
#158816=CARTESIAN_POINT('Ctrl Pts',(2.78578737643084,15.2,-10.7392151039935));
#158817=CARTESIAN_POINT('Ctrl Pts',(2.78514891843887,15.2,-10.7445707558777));
#158818=CARTESIAN_POINT('Ctrl Pts',(2.78449716100831,15.2,-10.749946048725));
#158819=CARTESIAN_POINT('Ctrl Pts',(2.78397575503545,15.2,-10.7542462832371));
#158820=CARTESIAN_POINT('Ctrl Pts',(2.78344583953104,15.2,-10.7585590878674));
#158821=CARTESIAN_POINT('Ctrl Pts',(2.78290735161193,15.2,-10.7628843617155));
#158822=CARTESIAN_POINT('Ctrl Pts',(2.78236886376619,15.2,-10.7672096349743));
#158823=CARTESIAN_POINT('Ctrl Pts',(2.78182180514631,15.2,-10.7715473781996));
#158824=CARTESIAN_POINT('Ctrl Pts',(2.78126611396702,15.2,-10.775897492197));
#158825=CARTESIAN_POINT('Ctrl Pts',(2.78071042271202,15.2,-10.7802476067871));
#158826=CARTESIAN_POINT('Ctrl Pts',(2.78014610013007,15.2,-10.7846100922089));
#158827=CARTESIAN_POINT('Ctrl Pts',(2.77957308493129,15.2,-10.7889848494486));
#158828=CARTESIAN_POINT('Ctrl Pts',(2.77900006981057,15.2,-10.7933596060922));
#158829=CARTESIAN_POINT('Ctrl Pts',(2.77841836502432,15.2,-10.7977466358703));
#158830=CARTESIAN_POINT('Ctrl Pts',(2.77782790857317,15.2,-10.8021458378988));
#158831=CARTESIAN_POINT('Ctrl Pts',(2.77723745204156,15.2,-10.8065450405266));
#158832=CARTESIAN_POINT('Ctrl Pts',(2.77663824584543,15.2,-10.810956418026));
#158833=CARTESIAN_POINT('Ctrl Pts',(2.77603023117004,15.2,-10.8153798721002));
#158834=CARTESIAN_POINT('Ctrl Pts',(2.77542221657749,15.2,-10.8198033255718));
#158835=CARTESIAN_POINT('Ctrl Pts',(2.77480539426876,15.2,-10.8242388543981));
#158836=CARTESIAN_POINT('Ctrl Pts',(2.77417970637605,15.2,-10.8286863636448));
#158837=CARTESIAN_POINT('Ctrl Pts',(2.7737104404352,15.2,-10.8320219957314));
#158838=CARTESIAN_POINT('Ctrl Pts',(2.77323618803636,15.2,-10.8353643661758));
#158839=CARTESIAN_POINT('Ctrl Pts',(2.77275692463779,15.2,-10.8387134343032));
#158840=CARTESIAN_POINT('Ctrl Pts',(2.77227766115215,15.2,-10.842062503039));
#158841=CARTESIAN_POINT('Ctrl Pts',(2.77179338669844,15.2,-10.8454182695767));
#158842=CARTESIAN_POINT('Ctrl Pts',(2.77130407866831,15.2,-10.848780694233));
#158843=CARTESIAN_POINT('Ctrl Pts',(2.77048856549216,15.2,-10.8543847339014));
#158844=CARTESIAN_POINT('Ctrl Pts',(2.76965906716166,15.2,-10.8600072646896));
#158845=CARTESIAN_POINT('Ctrl Pts',(2.76881547739365,15.2,-10.8656481027538));
#158846=CARTESIAN_POINT('Ctrl Pts',(2.76830932340411,15.2,-10.8690326064531));
#158847=CARTESIAN_POINT('Ctrl Pts',(2.76779809661315,15.2,-10.8724236997293));
#158848=CARTESIAN_POINT('Ctrl Pts',(2.76728177362075,15.2,-10.8758213439323));
#158849=CARTESIAN_POINT('Ctrl Pts',(2.76659334312055,15.2,-10.8803515351743));
#158850=CARTESIAN_POINT('Ctrl Pts',(2.76589585300763,15.2,-10.8848933709842));
#158851=CARTESIAN_POINT('Ctrl Pts',(2.76518924856599,15.2,-10.8894467576112));
#158852=CARTESIAN_POINT('Ctrl Pts',(2.76465929521069,15.2,-10.8928617977365));
#158853=CARTESIAN_POINT('Ctrl Pts',(2.76412421582788,15.2,-10.8962833349908));
#158854=CARTESIAN_POINT('Ctrl Pts',(2.76358398786278,15.2,-10.8997113293701));
#158855=CARTESIAN_POINT('Ctrl Pts',(2.76304375989769,15.2,-10.9031393237494));
#158856=CARTESIAN_POINT('Ctrl Pts',(2.76249838229929,15.2,-10.9065737765924));
#158857=CARTESIAN_POINT('Ctrl Pts',(2.76194783436166,15.2,-10.9100146467582));
#158858=CARTESIAN_POINT('Ctrl Pts',(2.76139728632402,15.2,-10.9134555175491));
#158859=CARTESIAN_POINT('Ctrl Pts',(2.76084156679326,15.2,-10.9169028060167));
#158860=CARTESIAN_POINT('Ctrl Pts',(2.7602806533777,15.2,-10.9203564737695));
#158861=CARTESIAN_POINT('Ctrl Pts',(2.75953276899345,15.2,-10.9249613630609));
#158862=CARTESIAN_POINT('Ctrl Pts',(2.75877565484929,15.2,-10.9295775922202));
#158863=CARTESIAN_POINT('Ctrl Pts',(2.75800925457921,15.2,-10.9342050688968));
#158864=CARTESIAN_POINT('Ctrl Pts',(2.75743445435055,15.2,-10.9376756765618));
#158865=CARTESIAN_POINT('Ctrl Pts',(2.75685443320387,15.2,-10.9411526111794));
#158866=CARTESIAN_POINT('Ctrl Pts',(2.7562691673215,15.2,-10.9446358331011));
#158867=CARTESIAN_POINT('Ctrl Pts',(2.75568390143913,15.2,-10.9481190550229));
#158868=CARTESIAN_POINT('Ctrl Pts',(2.75509339110749,15.2,-10.9516085654824));
#158869=CARTESIAN_POINT('Ctrl Pts',(2.75449761662986,15.2,-10.9551043237296));
#158870=CARTESIAN_POINT('Ctrl Pts',(2.75390184204398,15.2,-10.9586000826118));
#158871=CARTESIAN_POINT('Ctrl Pts',(2.75330080200663,15.2,-10.9621020915207));
#158872=CARTESIAN_POINT('Ctrl Pts',(2.7526944764178,15.2,-10.9656103103231));
#158873=CARTESIAN_POINT('Ctrl Pts',(2.75188604248293,15.2,-10.9702879343307));
#158874=CARTESIAN_POINT('Ctrl Pts',(2.75106820964095,15.2,-10.974976599273));
#158875=CARTESIAN_POINT('Ctrl Pts',(2.75024093054252,15.2,-10.9796762133326));
#158876=CARTESIAN_POINT('Ctrl Pts',(2.74962047119052,15.2,-10.9832009240373));
#158877=CARTESIAN_POINT('Ctrl Pts',(2.7489946975139,15.2,-10.9867317943249));
#158878=CARTESIAN_POINT('Ctrl Pts',(2.74836358912089,15.2,-10.9902687850289));
#158879=CARTESIAN_POINT('Ctrl Pts',(2.74773248061323,15.2,-10.9938057763754));
#158880=CARTESIAN_POINT('Ctrl Pts',(2.7470960371874,15.2,-10.9973488891737));
#158881=CARTESIAN_POINT('Ctrl Pts',(2.74645423913506,15.2,-11.0008980845237));
#158882=CARTESIAN_POINT('Ctrl Pts',(2.74559850859293,15.2,-11.0056303439157));
#158883=CARTESIAN_POINT('Ctrl Pts',(2.74473325802745,15.2,-11.0103734190054));
#158884=CARTESIAN_POINT('Ctrl Pts',(2.74385843898391,15.2,-11.0151272164717));
#158885=CARTESIAN_POINT('Ctrl Pts',(2.74320232467146,15.2,-11.0186925647334));
#158886=CARTESIAN_POINT('Ctrl Pts',(2.74254082774788,15.2,-11.022263945224));
#158887=CARTESIAN_POINT('Ctrl Pts',(2.74187392981425,15.2,-11.0258413208435));
#158888=CARTESIAN_POINT('Ctrl Pts',(2.74120703188062,15.2,-11.029418696463));
#158889=CARTESIAN_POINT('Ctrl Pts',(2.74053473130569,15.2,-11.0330020662821));
#158890=CARTESIAN_POINT('Ctrl Pts',(2.73985700941439,15.2,-11.0365913929842));
#158891=CARTESIAN_POINT('Ctrl Pts',(2.73917928739996,15.2,-11.0401807203384));
#158892=CARTESIAN_POINT('Ctrl Pts',(2.73849614306735,15.2,-11.0437760055109));
#158893=CARTESIAN_POINT('Ctrl Pts',(2.73780755809153,15.2,-11.047377210285));
#158894=CARTESIAN_POINT('Ctrl Pts',(2.73711897324081,15.2,-11.050978414405));
#158895=CARTESIAN_POINT('Ctrl Pts',(2.73642494695809,15.2,-11.0545855374825));
#158896=CARTESIAN_POINT('Ctrl Pts',(2.73572546007293,15.2,-11.0581985437407));
#158897=CARTESIAN_POINT('Ctrl Pts',(2.73502597318777,15.2,-11.061811549999));
#158898=CARTESIAN_POINT('Ctrl Pts',(2.73432102499712,15.2,-11.065430437293));
#158899=CARTESIAN_POINT('Ctrl Pts',(2.73361059710579,15.2,-11.0690551704118));
#158900=CARTESIAN_POINT('Ctrl Pts',(2.73290016921445,15.2,-11.0726799035306));
#158901=CARTESIAN_POINT('Ctrl Pts',(2.73218426090711,15.2,-11.0763104805487));
#158902=CARTESIAN_POINT('Ctrl Pts',(2.73146285451665,15.2,-11.07994686725));
#158903=CARTESIAN_POINT('Ctrl Pts',(2.7307414481262,15.2,-11.0835832539512));
#158904=CARTESIAN_POINT('Ctrl Pts',(2.73001454315263,15.2,-11.0872254500688));
#158905=CARTESIAN_POINT('Ctrl Pts',(2.72928212034639,15.2,-11.0908734168108));
#158906=CARTESIAN_POINT('Ctrl Pts',(2.72854969754015,15.2,-11.0945213835527));
#158907=CARTESIAN_POINT('Ctrl Pts',(2.72781175750326,15.2,-11.0981751224262));
#158908=CARTESIAN_POINT('Ctrl Pts',(2.72706828016044,15.2,-11.1018345948087));
#158909=CARTESIAN_POINT('Ctrl Pts',(2.72632480281762,15.2,-11.1054940671912));
#158910=CARTESIAN_POINT('Ctrl Pts',(2.7255757884863,15.2,-11.1091592726339));
#158911=CARTESIAN_POINT('Ctrl Pts',(2.72482121918114,15.2,-11.1128301753747));
#158912=CARTESIAN_POINT('Ctrl Pts',(2.7240666497389,15.2,-11.1165010787825));
#158913=CARTESIAN_POINT('Ctrl Pts',(2.72330652472843,15.2,-11.1201776796668));
#158914=CARTESIAN_POINT('Ctrl Pts',(2.72254082832472,15.2,-11.123859945036));
#158915=CARTESIAN_POINT('Ctrl Pts',(2.72177513206012,15.2,-11.1275422097363));
#158916=CARTESIAN_POINT('Ctrl Pts',(2.72100386497081,15.2,-11.1312301395697));
#158917=CARTESIAN_POINT('Ctrl Pts',(2.72022700716521,15.2,-11.1349236961443));
#158918=CARTESIAN_POINT('Ctrl Pts',(2.71945014935962,15.2,-11.1386172527189));
#158919=CARTESIAN_POINT('Ctrl Pts',(2.71866770180757,15.2,-11.1423164359544));
#158920=CARTESIAN_POINT('Ctrl Pts',(2.71787964049927,15.2,-11.146021201045));
#158921=CARTESIAN_POINT('Ctrl Pts',(2.71709157919096,15.2,-11.1497259661356));
#158922=CARTESIAN_POINT('Ctrl Pts',(2.7162979039086,15.2,-11.1534363114981));
#158923=CARTESIAN_POINT('Ctrl Pts',(2.71549860022571,15.2,-11.1571522050049));
#158924=CARTESIAN_POINT('Ctrl Pts',(2.71416642737248,15.2,-11.1633453610747));
#158925=CARTESIAN_POINT('Ctrl Pts',(2.71281861163052,15.2,-11.1695539323099));
#158926=CARTESIAN_POINT('Ctrl Pts',(2.71145515299994,15.2,-11.175777867));
#158927=CARTESIAN_POINT('Ctrl Pts',(1.76496130699994,15.2,-10.223773109));
#158928=CARTESIAN_POINT('Ctrl Pts',(1.76496130699994,11.6,-10.223773109));
#158929=CARTESIAN_POINT('Ctrl Pts',(1.76500562299994,15.2,-10.223941741));
#158930=CARTESIAN_POINT('Ctrl Pts',(1.76500562299994,11.6,-10.223941741));
#158931=CARTESIAN_POINT('Ctrl Pts',(1.76509588899994,15.2,-10.224284873));
#158932=CARTESIAN_POINT('Ctrl Pts',(1.76509588899994,11.6,-10.224284873));
#158933=CARTESIAN_POINT('Ctrl Pts',(1.76523291899994,15.2,-10.224804731));
#158934=CARTESIAN_POINT('Ctrl Pts',(1.76523291899994,11.6,-10.224804731));
#158935=CARTESIAN_POINT('Ctrl Pts',(1.76541803299994,15.2,-10.22550489));
#158936=CARTESIAN_POINT('Ctrl Pts',(1.76541803299994,11.6,-10.22550489));
#158937=CARTESIAN_POINT('Ctrl Pts',(1.76565305799994,15.2,-10.226390254));
#158938=CARTESIAN_POINT('Ctrl Pts',(1.76565305799994,11.6,-10.226390254));
#158939=CARTESIAN_POINT('Ctrl Pts',(1.76589279499994,15.2,-10.227289727));
#158940=CARTESIAN_POINT('Ctrl Pts',(1.76589279499994,11.6,-10.227289727));
#158941=CARTESIAN_POINT('Ctrl Pts',(1.76613589399994,15.2,-10.228198149));
#158942=CARTESIAN_POINT('Ctrl Pts',(1.76613589399994,11.6,-10.228198149));
#158943=CARTESIAN_POINT('Ctrl Pts',(1.76638236599994,15.2,-10.229115492));
#158944=CARTESIAN_POINT('Ctrl Pts',(1.76638236599994,11.6,-10.229115492));
#158945=CARTESIAN_POINT('Ctrl Pts',(1.76663221999994,15.2,-10.230041723));
#158946=CARTESIAN_POINT('Ctrl Pts',(1.76663221999994,11.6,-10.230041723));
#158947=CARTESIAN_POINT('Ctrl Pts',(1.76688546699994,15.2,-10.230976812));
#158948=CARTESIAN_POINT('Ctrl Pts',(1.76688546699994,11.6,-10.230976812));
#158949=CARTESIAN_POINT('Ctrl Pts',(1.76714211699994,15.2,-10.231920729));
#158950=CARTESIAN_POINT('Ctrl Pts',(1.76714211699994,11.6,-10.231920729));
#158951=CARTESIAN_POINT('Ctrl Pts',(1.76740218099994,15.2,-10.232873443));
#158952=CARTESIAN_POINT('Ctrl Pts',(1.76740218099994,11.6,-10.232873443));
#158953=CARTESIAN_POINT('Ctrl Pts',(1.76766566999994,15.2,-10.233834926));
#158954=CARTESIAN_POINT('Ctrl Pts',(1.76766566999994,11.6,-10.233834926));
#158955=CARTESIAN_POINT('Ctrl Pts',(1.76793259299994,15.2,-10.234805146));
#158956=CARTESIAN_POINT('Ctrl Pts',(1.76793259299994,11.6,-10.234805146));
#158957=CARTESIAN_POINT('Ctrl Pts',(1.76820295999994,15.2,-10.235784073));
#158958=CARTESIAN_POINT('Ctrl Pts',(1.76820295999994,11.6,-10.235784073));
#158959=CARTESIAN_POINT('Ctrl Pts',(1.76847678199994,15.2,-10.23677168));
#158960=CARTESIAN_POINT('Ctrl Pts',(1.76847678199994,11.6,-10.23677168));
#158961=CARTESIAN_POINT('Ctrl Pts',(1.76875406799994,15.2,-10.237767935));
#158962=CARTESIAN_POINT('Ctrl Pts',(1.76875406799994,11.6,-10.237767935));
#158963=CARTESIAN_POINT('Ctrl Pts',(1.76903482799994,15.2,-10.238772809));
#158964=CARTESIAN_POINT('Ctrl Pts',(1.76903482799994,11.6,-10.238772809));
#158965=CARTESIAN_POINT('Ctrl Pts',(1.76931907099994,15.2,-10.239786274));
#158966=CARTESIAN_POINT('Ctrl Pts',(1.76931907099994,11.6,-10.239786274));
#158967=CARTESIAN_POINT('Ctrl Pts',(1.76960680899994,15.2,-10.2408083));
#158968=CARTESIAN_POINT('Ctrl Pts',(1.76960680899994,11.6,-10.2408083));
#158969=CARTESIAN_POINT('Ctrl Pts',(1.76989805199994,15.2,-10.241838858));
#158970=CARTESIAN_POINT('Ctrl Pts',(1.76989805199994,11.6,-10.241838858));
#158971=CARTESIAN_POINT('Ctrl Pts',(1.77019280699994,15.2,-10.24287792));
#158972=CARTESIAN_POINT('Ctrl Pts',(1.77019280699994,11.6,-10.24287792));
#158973=CARTESIAN_POINT('Ctrl Pts',(1.77049108499994,15.2,-10.243925456));
#158974=CARTESIAN_POINT('Ctrl Pts',(1.77049108499994,11.6,-10.243925456));
#158975=CARTESIAN_POINT('Ctrl Pts',(1.77079289599994,15.2,-10.244981439));
#158976=CARTESIAN_POINT('Ctrl Pts',(1.77079289599994,11.6,-10.244981439));
#158977=CARTESIAN_POINT('Ctrl Pts',(1.77109824899994,15.2,-10.246045839));
#158978=CARTESIAN_POINT('Ctrl Pts',(1.77109824899994,11.6,-10.246045839));
#158979=CARTESIAN_POINT('Ctrl Pts',(1.77140715299994,15.2,-10.247118629));
#158980=CARTESIAN_POINT('Ctrl Pts',(1.77140715299994,11.6,-10.247118629));
#158981=CARTESIAN_POINT('Ctrl Pts',(1.77171961899994,15.2,-10.248199781));
#158982=CARTESIAN_POINT('Ctrl Pts',(1.77171961899994,11.6,-10.248199781));
#158983=CARTESIAN_POINT('Ctrl Pts',(1.77203565399994,15.2,-10.249289267));
#158984=CARTESIAN_POINT('Ctrl Pts',(1.77203565399994,11.6,-10.249289267));
#158985=CARTESIAN_POINT('Ctrl Pts',(1.77235526999994,15.2,-10.250387057));
#158986=CARTESIAN_POINT('Ctrl Pts',(1.77235526999994,11.6,-10.250387057));
#158987=CARTESIAN_POINT('Ctrl Pts',(1.77267847299994,15.2,-10.251493125));
#158988=CARTESIAN_POINT('Ctrl Pts',(1.77267847299994,11.6,-10.251493125));
#158989=CARTESIAN_POINT('Ctrl Pts',(1.77300527499994,15.2,-10.252607443));
#158990=CARTESIAN_POINT('Ctrl Pts',(1.77300527499994,11.6,-10.252607443));
#158991=CARTESIAN_POINT('Ctrl Pts',(1.77333568299994,15.2,-10.253729984));
#158992=CARTESIAN_POINT('Ctrl Pts',(1.77333568299994,11.6,-10.253729984));
#158993=CARTESIAN_POINT('Ctrl Pts',(1.77366970799994,15.2,-10.25486072));
#158994=CARTESIAN_POINT('Ctrl Pts',(1.77366970799994,11.6,-10.25486072));
#158995=CARTESIAN_POINT('Ctrl Pts',(1.77400735799994,15.2,-10.255999624));
#158996=CARTESIAN_POINT('Ctrl Pts',(1.77400735799994,11.6,-10.255999624));
#158997=CARTESIAN_POINT('Ctrl Pts',(1.77434864199994,15.2,-10.257146668));
#158998=CARTESIAN_POINT('Ctrl Pts',(1.77434864199994,11.6,-10.257146668));
#158999=CARTESIAN_POINT('Ctrl Pts',(1.77469356799994,15.2,-10.258301827));
#159000=CARTESIAN_POINT('Ctrl Pts',(1.77469356799994,11.6,-10.258301827));
#159001=CARTESIAN_POINT('Ctrl Pts',(1.77504214599994,15.2,-10.259465073));
#159002=CARTESIAN_POINT('Ctrl Pts',(1.77504214599994,11.6,-10.259465073));
#159003=CARTESIAN_POINT('Ctrl Pts',(1.77539438599994,15.2,-10.260636378));
#159004=CARTESIAN_POINT('Ctrl Pts',(1.77539438599994,11.6,-10.260636378));
#159005=CARTESIAN_POINT('Ctrl Pts',(1.77575029399994,15.2,-10.261815716));
#159006=CARTESIAN_POINT('Ctrl Pts',(1.77575029399994,11.6,-10.261815716));
#159007=CARTESIAN_POINT('Ctrl Pts',(1.77610987999994,15.2,-10.263003061));
#159008=CARTESIAN_POINT('Ctrl Pts',(1.77610987999994,11.6,-10.263003061));
#159009=CARTESIAN_POINT('Ctrl Pts',(1.77647315199994,15.2,-10.264198387));
#159010=CARTESIAN_POINT('Ctrl Pts',(1.77647315199994,11.6,-10.264198387));
#159011=CARTESIAN_POINT('Ctrl Pts',(1.77684011999994,15.2,-10.265401666));
#159012=CARTESIAN_POINT('Ctrl Pts',(1.77684011999994,11.6,-10.265401666));
#159013=CARTESIAN_POINT('Ctrl Pts',(1.77721079199994,15.2,-10.266612874));
#159014=CARTESIAN_POINT('Ctrl Pts',(1.77721079199994,11.6,-10.266612874));
#159015=CARTESIAN_POINT('Ctrl Pts',(1.77758517499994,15.2,-10.267831982));
#159016=CARTESIAN_POINT('Ctrl Pts',(1.77758517499994,11.6,-10.267831982));
#159017=CARTESIAN_POINT('Ctrl Pts',(1.77796327899994,15.2,-10.269058966));
#159018=CARTESIAN_POINT('Ctrl Pts',(1.77796327899994,11.6,-10.269058966));
#159019=CARTESIAN_POINT('Ctrl Pts',(1.77834511299995,15.2,-10.2702938));
#159020=CARTESIAN_POINT('Ctrl Pts',(1.77834511299995,11.6,-10.2702938));
#159021=CARTESIAN_POINT('Ctrl Pts',(1.77873068199994,15.2,-10.271536458));
#159022=CARTESIAN_POINT('Ctrl Pts',(1.77873068199994,11.6,-10.271536458));
#159023=CARTESIAN_POINT('Ctrl Pts',(1.77911999799994,15.2,-10.272786914));
#159024=CARTESIAN_POINT('Ctrl Pts',(1.77911999799994,11.6,-10.272786914));
#159025=CARTESIAN_POINT('Ctrl Pts',(1.77951306799994,15.2,-10.274045143));
#159026=CARTESIAN_POINT('Ctrl Pts',(1.77951306799994,11.6,-10.274045143));
#159027=CARTESIAN_POINT('Ctrl Pts',(1.77990989999994,15.2,-10.275311119));
#159028=CARTESIAN_POINT('Ctrl Pts',(1.77990989999994,11.6,-10.275311119));
#159029=CARTESIAN_POINT('Ctrl Pts',(1.78031050099994,15.2,-10.276584816));
#159030=CARTESIAN_POINT('Ctrl Pts',(1.78031050099994,11.6,-10.276584816));
#159031=CARTESIAN_POINT('Ctrl Pts',(1.78071487999994,15.2,-10.27786621));
#159032=CARTESIAN_POINT('Ctrl Pts',(1.78071487999994,11.6,-10.27786621));
#159033=CARTESIAN_POINT('Ctrl Pts',(1.78112304599994,15.2,-10.279155276));
#159034=CARTESIAN_POINT('Ctrl Pts',(1.78112304599994,11.6,-10.279155276));
#159035=CARTESIAN_POINT('Ctrl Pts',(1.78153500599994,15.2,-10.280451988));
#159036=CARTESIAN_POINT('Ctrl Pts',(1.78153500599994,11.6,-10.280451988));
#159037=CARTESIAN_POINT('Ctrl Pts',(1.78195076699994,15.2,-10.281756321));
#159038=CARTESIAN_POINT('Ctrl Pts',(1.78195076699994,11.6,-10.281756321));
#159039=CARTESIAN_POINT('Ctrl Pts',(1.78237033899994,15.2,-10.283068252));
#159040=CARTESIAN_POINT('Ctrl Pts',(1.78237033899994,11.6,-10.283068252));
#159041=CARTESIAN_POINT('Ctrl Pts',(1.78279372899994,15.2,-10.284387754));
#159042=CARTESIAN_POINT('Ctrl Pts',(1.78279372899994,11.6,-10.284387754));
#159043=CARTESIAN_POINT('Ctrl Pts',(1.78322094399994,15.2,-10.285714803));
#159044=CARTESIAN_POINT('Ctrl Pts',(1.78322094399994,11.6,-10.285714803));
#159045=CARTESIAN_POINT('Ctrl Pts',(1.78365199299995,15.2,-10.287049375));
#159046=CARTESIAN_POINT('Ctrl Pts',(1.78365199299995,11.6,-10.287049375));
#159047=CARTESIAN_POINT('Ctrl Pts',(1.78408688299994,15.2,-10.288391446));
#159048=CARTESIAN_POINT('Ctrl Pts',(1.78408688299994,11.6,-10.288391446));
#159049=CARTESIAN_POINT('Ctrl Pts',(1.78452562099994,15.2,-10.28974099));
#159050=CARTESIAN_POINT('Ctrl Pts',(1.78452562099994,11.6,-10.28974099));
#159051=CARTESIAN_POINT('Ctrl Pts',(1.78496821499994,15.2,-10.291097983));
#159052=CARTESIAN_POINT('Ctrl Pts',(1.78496821499994,11.6,-10.291097983));
#159053=CARTESIAN_POINT('Ctrl Pts',(1.78541467399994,15.2,-10.292462403));
#159054=CARTESIAN_POINT('Ctrl Pts',(1.78541467399994,11.6,-10.292462403));
#159055=CARTESIAN_POINT('Ctrl Pts',(1.78586500399994,15.2,-10.293834224));
#159056=CARTESIAN_POINT('Ctrl Pts',(1.78586500399994,11.6,-10.293834224));
#159057=CARTESIAN_POINT('Ctrl Pts',(1.78631921299994,15.2,-10.295213422));
#159058=CARTESIAN_POINT('Ctrl Pts',(1.78631921299994,11.6,-10.295213422));
#159059=CARTESIAN_POINT('Ctrl Pts',(1.78677730899994,15.2,-10.296599975));
#159060=CARTESIAN_POINT('Ctrl Pts',(1.78677730899994,11.6,-10.296599975));
#159061=CARTESIAN_POINT('Ctrl Pts',(1.78723929699994,15.2,-10.297993858));
#159062=CARTESIAN_POINT('Ctrl Pts',(1.78723929699994,11.6,-10.297993858));
#159063=CARTESIAN_POINT('Ctrl Pts',(1.78770518699994,15.2,-10.299395046));
#159064=CARTESIAN_POINT('Ctrl Pts',(1.78770518699994,11.6,-10.299395046));
#159065=CARTESIAN_POINT('Ctrl Pts',(1.78817498599994,15.2,-10.300803517));
#159066=CARTESIAN_POINT('Ctrl Pts',(1.78817498599994,11.6,-10.300803517));
#159067=CARTESIAN_POINT('Ctrl Pts',(1.78864869999994,15.2,-10.302219248));
#159068=CARTESIAN_POINT('Ctrl Pts',(1.78864869999994,11.6,-10.302219248));
#159069=CARTESIAN_POINT('Ctrl Pts',(1.78912633699994,15.2,-10.303642215));
#159070=CARTESIAN_POINT('Ctrl Pts',(1.78912633699994,11.6,-10.303642215));
#159071=CARTESIAN_POINT('Ctrl Pts',(1.78960790399994,15.2,-10.305072393));
#159072=CARTESIAN_POINT('Ctrl Pts',(1.78960790399994,11.6,-10.305072393));
#159073=CARTESIAN_POINT('Ctrl Pts',(1.79009340899994,15.2,-10.306509762));
#159074=CARTESIAN_POINT('Ctrl Pts',(1.79009340899994,11.6,-10.306509762));
#159075=CARTESIAN_POINT('Ctrl Pts',(1.79058285799994,15.2,-10.307954296));
#159076=CARTESIAN_POINT('Ctrl Pts',(1.79058285799994,11.6,-10.307954296));
#159077=CARTESIAN_POINT('Ctrl Pts',(1.79107625799994,15.2,-10.309405975));
#159078=CARTESIAN_POINT('Ctrl Pts',(1.79107625799994,11.6,-10.309405975));
#159079=CARTESIAN_POINT('Ctrl Pts',(1.79157361699994,15.2,-10.310864772));
#159080=CARTESIAN_POINT('Ctrl Pts',(1.79157361699994,11.6,-10.310864772));
#159081=CARTESIAN_POINT('Ctrl Pts',(1.79207494099994,15.2,-10.312330668));
#159082=CARTESIAN_POINT('Ctrl Pts',(1.79207494099994,11.6,-10.312330668));
#159083=CARTESIAN_POINT('Ctrl Pts',(1.79258023699994,15.2,-10.313803638));
#159084=CARTESIAN_POINT('Ctrl Pts',(1.79258023699994,11.6,-10.313803638));
#159085=CARTESIAN_POINT('Ctrl Pts',(1.79308951199994,15.2,-10.315283661));
#159086=CARTESIAN_POINT('Ctrl Pts',(1.79308951199994,11.6,-10.315283661));
#159087=CARTESIAN_POINT('Ctrl Pts',(1.79360277399994,15.2,-10.316770712));
#159088=CARTESIAN_POINT('Ctrl Pts',(1.79360277399994,11.6,-10.316770712));
#159089=CARTESIAN_POINT('Ctrl Pts',(1.79412002899994,15.2,-10.318264771));
#159090=CARTESIAN_POINT('Ctrl Pts',(1.79412002899994,11.6,-10.318264771));
#159091=CARTESIAN_POINT('Ctrl Pts',(1.79464128299994,15.2,-10.319765813));
#159092=CARTESIAN_POINT('Ctrl Pts',(1.79464128299994,11.6,-10.319765813));
#159093=CARTESIAN_POINT('Ctrl Pts',(1.79516654299994,15.2,-10.321273818));
#159094=CARTESIAN_POINT('Ctrl Pts',(1.79516654299994,11.6,-10.321273818));
#159095=CARTESIAN_POINT('Ctrl Pts',(1.79569581699994,15.2,-10.322788763));
#159096=CARTESIAN_POINT('Ctrl Pts',(1.79569581699994,11.6,-10.322788763));
#159097=CARTESIAN_POINT('Ctrl Pts',(1.79622910999994,15.2,-10.324310627));
#159098=CARTESIAN_POINT('Ctrl Pts',(1.79622910999994,11.6,-10.324310627));
#159099=CARTESIAN_POINT('Ctrl Pts',(1.79676642999994,15.2,-10.325839385));
#159100=CARTESIAN_POINT('Ctrl Pts',(1.79676642999994,11.6,-10.325839385));
#159101=CARTESIAN_POINT('Ctrl Pts',(1.79730778399994,15.2,-10.327375017));
#159102=CARTESIAN_POINT('Ctrl Pts',(1.79730778399994,11.6,-10.327375017));
#159103=CARTESIAN_POINT('Ctrl Pts',(1.79785317499994,15.2,-10.328917501));
#159104=CARTESIAN_POINT('Ctrl Pts',(1.79785317499994,11.6,-10.328917501));
#159105=CARTESIAN_POINT('Ctrl Pts',(1.79840261399994,15.2,-10.330466814));
#159106=CARTESIAN_POINT('Ctrl Pts',(1.79840261399994,11.6,-10.330466814));
#159107=CARTESIAN_POINT('Ctrl Pts',(1.79895610399994,15.2,-10.332022936));
#159108=CARTESIAN_POINT('Ctrl Pts',(1.79895610399994,11.6,-10.332022936));
#159109=CARTESIAN_POINT('Ctrl Pts',(1.79951365499994,15.2,-10.333585844));
#159110=CARTESIAN_POINT('Ctrl Pts',(1.79951365499994,11.6,-10.333585844));
#159111=CARTESIAN_POINT('Ctrl Pts',(1.80007526999994,15.2,-10.335155517));
#159112=CARTESIAN_POINT('Ctrl Pts',(1.80007526999994,11.6,-10.335155517));
#159113=CARTESIAN_POINT('Ctrl Pts',(1.80064095699994,15.2,-10.336731933));
#159114=CARTESIAN_POINT('Ctrl Pts',(1.80064095699994,11.6,-10.336731933));
#159115=CARTESIAN_POINT('Ctrl Pts',(1.80121072099994,15.2,-10.338315071));
#159116=CARTESIAN_POINT('Ctrl Pts',(1.80121072099994,11.6,-10.338315071));
#159117=CARTESIAN_POINT('Ctrl Pts',(1.80178457199994,15.2,-10.33990491));
#159118=CARTESIAN_POINT('Ctrl Pts',(1.80178457199994,11.6,-10.33990491));
#159119=CARTESIAN_POINT('Ctrl Pts',(1.80236250999994,15.2,-10.341501427));
#159120=CARTESIAN_POINT('Ctrl Pts',(1.80236250999994,11.6,-10.341501427));
#159121=CARTESIAN_POINT('Ctrl Pts',(1.80294454699994,15.2,-10.343104603));
#159122=CARTESIAN_POINT('Ctrl Pts',(1.80294454699994,11.6,-10.343104603));
#159123=CARTESIAN_POINT('Ctrl Pts',(1.80353068699994,15.2,-10.344714415));
#159124=CARTESIAN_POINT('Ctrl Pts',(1.80353068699994,11.6,-10.344714415));
#159125=CARTESIAN_POINT('Ctrl Pts',(1.80412093499994,15.2,-10.346330843));
#159126=CARTESIAN_POINT('Ctrl Pts',(1.80412093499994,11.6,-10.346330843));
#159127=CARTESIAN_POINT('Ctrl Pts',(1.80471529899994,15.2,-10.347953866));
#159128=CARTESIAN_POINT('Ctrl Pts',(1.80471529899994,11.6,-10.347953866));
#159129=CARTESIAN_POINT('Ctrl Pts',(1.80531378399994,15.2,-10.349583463));
#159130=CARTESIAN_POINT('Ctrl Pts',(1.80531378399994,11.6,-10.349583463));
#159131=CARTESIAN_POINT('Ctrl Pts',(1.80591639699994,15.2,-10.351219612));
#159132=CARTESIAN_POINT('Ctrl Pts',(1.80591639699994,11.6,-10.351219612));
#159133=CARTESIAN_POINT('Ctrl Pts',(1.80652314299994,15.2,-10.352862295));
#159134=CARTESIAN_POINT('Ctrl Pts',(1.80652314299994,11.6,-10.352862295));
#159135=CARTESIAN_POINT('Ctrl Pts',(1.80713402799994,15.2,-10.354511488));
#159136=CARTESIAN_POINT('Ctrl Pts',(1.80713402799994,11.6,-10.354511488));
#159137=CARTESIAN_POINT('Ctrl Pts',(1.80774905899994,15.2,-10.356167172));
#159138=CARTESIAN_POINT('Ctrl Pts',(1.80774905899994,11.6,-10.356167172));
#159139=CARTESIAN_POINT('Ctrl Pts',(1.80836823999994,15.2,-10.357829328));
#159140=CARTESIAN_POINT('Ctrl Pts',(1.80836823999994,11.6,-10.357829328));
#159141=CARTESIAN_POINT('Ctrl Pts',(1.80899157899994,15.2,-10.359497933));
#159142=CARTESIAN_POINT('Ctrl Pts',(1.80899157899994,11.6,-10.359497933));
#159143=CARTESIAN_POINT('Ctrl Pts',(1.80961908099994,15.2,-10.361172966));
#159144=CARTESIAN_POINT('Ctrl Pts',(1.80961908099994,11.6,-10.361172966));
#159145=CARTESIAN_POINT('Ctrl Pts',(1.81025075099994,15.2,-10.36285441));
#159146=CARTESIAN_POINT('Ctrl Pts',(1.81025075099994,11.6,-10.36285441));
#159147=CARTESIAN_POINT('Ctrl Pts',(1.81088659599994,15.2,-10.364542242));
#159148=CARTESIAN_POINT('Ctrl Pts',(1.81088659599994,11.6,-10.364542242));
#159149=CARTESIAN_POINT('Ctrl Pts',(1.81152661999994,15.2,-10.366236444));
#159150=CARTESIAN_POINT('Ctrl Pts',(1.81152661999994,11.6,-10.366236444));
#159151=CARTESIAN_POINT('Ctrl Pts',(1.81217083099994,15.2,-10.367936993));
#159152=CARTESIAN_POINT('Ctrl Pts',(1.81217083099994,11.6,-10.367936993));
#159153=CARTESIAN_POINT('Ctrl Pts',(1.81281923299994,15.2,-10.369643871));
#159154=CARTESIAN_POINT('Ctrl Pts',(1.81281923299994,11.6,-10.369643871));
#159155=CARTESIAN_POINT('Ctrl Pts',(1.81347183299994,15.2,-10.371357057));
#159156=CARTESIAN_POINT('Ctrl Pts',(1.81347183299994,11.6,-10.371357057));
#159157=CARTESIAN_POINT('Ctrl Pts',(1.81412863499994,15.2,-10.373076533));
#159158=CARTESIAN_POINT('Ctrl Pts',(1.81412863499994,11.6,-10.373076533));
#159159=CARTESIAN_POINT('Ctrl Pts',(1.81478964499994,15.2,-10.374802277));
#159160=CARTESIAN_POINT('Ctrl Pts',(1.81478964499994,11.6,-10.374802277));
#159161=CARTESIAN_POINT('Ctrl Pts',(1.81545486999994,15.2,-10.37653427));
#159162=CARTESIAN_POINT('Ctrl Pts',(1.81545486999994,11.6,-10.37653427));
#159163=CARTESIAN_POINT('Ctrl Pts',(1.81612431399994,15.2,-10.378272492));
#159164=CARTESIAN_POINT('Ctrl Pts',(1.81612431399994,11.6,-10.378272492));
#159165=CARTESIAN_POINT('Ctrl Pts',(1.81679798299994,15.2,-10.380016924));
#159166=CARTESIAN_POINT('Ctrl Pts',(1.81679798299994,11.6,-10.380016924));
#159167=CARTESIAN_POINT('Ctrl Pts',(1.81747588199994,15.2,-10.381767545));
#159168=CARTESIAN_POINT('Ctrl Pts',(1.81747588199994,11.6,-10.381767545));
#159169=CARTESIAN_POINT('Ctrl Pts',(1.81815801699994,15.2,-10.383524338));
#159170=CARTESIAN_POINT('Ctrl Pts',(1.81815801699994,11.6,-10.383524338));
#159171=CARTESIAN_POINT('Ctrl Pts',(1.81884439299994,15.2,-10.385287281));
#159172=CARTESIAN_POINT('Ctrl Pts',(1.81884439299994,11.6,-10.385287281));
#159173=CARTESIAN_POINT('Ctrl Pts',(1.81953501599994,15.2,-10.387056356));
#159174=CARTESIAN_POINT('Ctrl Pts',(1.81953501599994,11.6,-10.387056356));
#159175=CARTESIAN_POINT('Ctrl Pts',(1.82022989099994,15.2,-10.388831543));
#159176=CARTESIAN_POINT('Ctrl Pts',(1.82022989099994,11.6,-10.388831543));
#159177=CARTESIAN_POINT('Ctrl Pts',(1.82092902199994,15.2,-10.390612824));
#159178=CARTESIAN_POINT('Ctrl Pts',(1.82092902199994,11.6,-10.390612824));
#159179=CARTESIAN_POINT('Ctrl Pts',(1.82163241599994,15.2,-10.392400178));
#159180=CARTESIAN_POINT('Ctrl Pts',(1.82163241599994,11.6,-10.392400178));
#159181=CARTESIAN_POINT('Ctrl Pts',(1.82234007799994,15.2,-10.394193587));
#159182=CARTESIAN_POINT('Ctrl Pts',(1.82234007799994,11.6,-10.394193587));
#159183=CARTESIAN_POINT('Ctrl Pts',(1.82305201199994,15.2,-10.395993031));
#159184=CARTESIAN_POINT('Ctrl Pts',(1.82305201199994,11.6,-10.395993031));
#159185=CARTESIAN_POINT('Ctrl Pts',(1.82376822599994,15.2,-10.397798492));
#159186=CARTESIAN_POINT('Ctrl Pts',(1.82376822599994,11.6,-10.397798492));
#159187=CARTESIAN_POINT('Ctrl Pts',(1.82448872099994,15.2,-10.399609952));
#159188=CARTESIAN_POINT('Ctrl Pts',(1.82448872099994,11.6,-10.399609952));
#159189=CARTESIAN_POINT('Ctrl Pts',(1.82521350499994,15.2,-10.401427389));
#159190=CARTESIAN_POINT('Ctrl Pts',(1.82521350499994,11.6,-10.401427389));
#159191=CARTESIAN_POINT('Ctrl Pts',(1.82594258299994,15.2,-10.403250787));
#159192=CARTESIAN_POINT('Ctrl Pts',(1.82594258299994,11.6,-10.403250787));
#159193=CARTESIAN_POINT('Ctrl Pts',(1.82667595799994,15.2,-10.405080125));
#159194=CARTESIAN_POINT('Ctrl Pts',(1.82667595799994,11.6,-10.405080125));
#159195=CARTESIAN_POINT('Ctrl Pts',(1.82741363699994,15.2,-10.406915387));
#159196=CARTESIAN_POINT('Ctrl Pts',(1.82741363699994,11.6,-10.406915387));
#159197=CARTESIAN_POINT('Ctrl Pts',(1.82815562499994,15.2,-10.408756552));
#159198=CARTESIAN_POINT('Ctrl Pts',(1.82815562499994,11.6,-10.408756552));
#159199=CARTESIAN_POINT('Ctrl Pts',(1.82890192699994,15.2,-10.410603603));
#159200=CARTESIAN_POINT('Ctrl Pts',(1.82890192699994,11.6,-10.410603603));
#159201=CARTESIAN_POINT('Ctrl Pts',(1.82965254599994,15.2,-10.41245652));
#159202=CARTESIAN_POINT('Ctrl Pts',(1.82965254599994,11.6,-10.41245652));
#159203=CARTESIAN_POINT('Ctrl Pts',(1.83040748999994,15.2,-10.414315286));
#159204=CARTESIAN_POINT('Ctrl Pts',(1.83040748999994,11.6,-10.414315286));
#159205=CARTESIAN_POINT('Ctrl Pts',(1.83116676099994,15.2,-10.416179881));
#159206=CARTESIAN_POINT('Ctrl Pts',(1.83116676099994,11.6,-10.416179881));
#159207=CARTESIAN_POINT('Ctrl Pts',(1.83193036499994,15.2,-10.418050288));
#159208=CARTESIAN_POINT('Ctrl Pts',(1.83193036499994,11.6,-10.418050288));
#159209=CARTESIAN_POINT('Ctrl Pts',(1.83269830799994,15.2,-10.419926488));
#159210=CARTESIAN_POINT('Ctrl Pts',(1.83269830799994,11.6,-10.419926488));
#159211=CARTESIAN_POINT('Ctrl Pts',(1.83347059199994,15.2,-10.421808463));
#159212=CARTESIAN_POINT('Ctrl Pts',(1.83347059199994,11.6,-10.421808463));
#159213=CARTESIAN_POINT('Ctrl Pts',(1.83424722399994,15.2,-10.423696194));
#159214=CARTESIAN_POINT('Ctrl Pts',(1.83424722399994,11.6,-10.423696194));
#159215=CARTESIAN_POINT('Ctrl Pts',(1.83502820899994,15.2,-10.425589665));
#159216=CARTESIAN_POINT('Ctrl Pts',(1.83502820899994,11.6,-10.425589665));
#159217=CARTESIAN_POINT('Ctrl Pts',(1.83581354999994,15.2,-10.427488857));
#159218=CARTESIAN_POINT('Ctrl Pts',(1.83581354999994,11.6,-10.427488857));
#159219=CARTESIAN_POINT('Ctrl Pts',(1.83660325299994,15.2,-10.429393751));
#159220=CARTESIAN_POINT('Ctrl Pts',(1.83660325299994,11.6,-10.429393751));
#159221=CARTESIAN_POINT('Ctrl Pts',(1.83739732299994,15.2,-10.431304329));
#159222=CARTESIAN_POINT('Ctrl Pts',(1.83739732299994,11.6,-10.431304329));
#159223=CARTESIAN_POINT('Ctrl Pts',(1.83819576299994,15.2,-10.433220574));
#159224=CARTESIAN_POINT('Ctrl Pts',(1.83819576299994,11.6,-10.433220574));
#159225=CARTESIAN_POINT('Ctrl Pts',(1.83899857899994,15.2,-10.435142468));
#159226=CARTESIAN_POINT('Ctrl Pts',(1.83899857899994,11.6,-10.435142468));
#159227=CARTESIAN_POINT('Ctrl Pts',(1.83980577599994,15.2,-10.437069993));
#159228=CARTESIAN_POINT('Ctrl Pts',(1.83980577599994,11.6,-10.437069993));
#159229=CARTESIAN_POINT('Ctrl Pts',(1.84061735599994,15.2,-10.439003132));
#159230=CARTESIAN_POINT('Ctrl Pts',(1.84061735599994,11.6,-10.439003132));
#159231=CARTESIAN_POINT('Ctrl Pts',(1.84143332699994,15.2,-10.440941867));
#159232=CARTESIAN_POINT('Ctrl Pts',(1.84143332699994,11.6,-10.440941867));
#159233=CARTESIAN_POINT('Ctrl Pts',(1.84225369099994,15.2,-10.442886179));
#159234=CARTESIAN_POINT('Ctrl Pts',(1.84225369099994,11.6,-10.442886179));
#159235=CARTESIAN_POINT('Ctrl Pts',(1.84307845299994,15.2,-10.444836053));
#159236=CARTESIAN_POINT('Ctrl Pts',(1.84307845299994,11.6,-10.444836053));
#159237=CARTESIAN_POINT('Ctrl Pts',(1.84390761699994,15.2,-10.446791469));
#159238=CARTESIAN_POINT('Ctrl Pts',(1.84390761699994,11.6,-10.446791469));
#159239=CARTESIAN_POINT('Ctrl Pts',(1.84474118899994,15.2,-10.44875241));
#159240=CARTESIAN_POINT('Ctrl Pts',(1.84474118899994,11.6,-10.44875241));
#159241=CARTESIAN_POINT('Ctrl Pts',(1.84557917199994,15.2,-10.45071886));
#159242=CARTESIAN_POINT('Ctrl Pts',(1.84557917199994,11.6,-10.45071886));
#159243=CARTESIAN_POINT('Ctrl Pts',(1.84642157199994,15.2,-10.452690801));
#159244=CARTESIAN_POINT('Ctrl Pts',(1.84642157199994,11.6,-10.452690801));
#159245=CARTESIAN_POINT('Ctrl Pts',(1.84726839199994,15.2,-10.454668215));
#159246=CARTESIAN_POINT('Ctrl Pts',(1.84726839199994,11.6,-10.454668215));
#159247=CARTESIAN_POINT('Ctrl Pts',(1.84811963599994,15.2,-10.456651085));
#159248=CARTESIAN_POINT('Ctrl Pts',(1.84811963599994,11.6,-10.456651085));
#159249=CARTESIAN_POINT('Ctrl Pts',(1.84897530999994,15.2,-10.458639395));
#159250=CARTESIAN_POINT('Ctrl Pts',(1.84897530999994,11.6,-10.458639395));
#159251=CARTESIAN_POINT('Ctrl Pts',(1.84983541599994,15.2,-10.460633126));
#159252=CARTESIAN_POINT('Ctrl Pts',(1.84983541599994,11.6,-10.460633126));
#159253=CARTESIAN_POINT('Ctrl Pts',(1.85069995999994,15.2,-10.462632262));
#159254=CARTESIAN_POINT('Ctrl Pts',(1.85069995999994,11.6,-10.462632262));
#159255=CARTESIAN_POINT('Ctrl Pts',(1.85156894599994,15.2,-10.464636786));
#159256=CARTESIAN_POINT('Ctrl Pts',(1.85156894599994,11.6,-10.464636786));
#159257=CARTESIAN_POINT('Ctrl Pts',(1.85244237799994,15.2,-10.46664668));
#159258=CARTESIAN_POINT('Ctrl Pts',(1.85244237799994,11.6,-10.46664668));
#159259=CARTESIAN_POINT('Ctrl Pts',(1.85332025899994,15.2,-10.468661929));
#159260=CARTESIAN_POINT('Ctrl Pts',(1.85332025899994,11.6,-10.468661929));
#159261=CARTESIAN_POINT('Ctrl Pts',(1.85420259499994,15.2,-10.470682514));
#159262=CARTESIAN_POINT('Ctrl Pts',(1.85420259499994,11.6,-10.470682514));
#159263=CARTESIAN_POINT('Ctrl Pts',(1.85508938999994,15.2,-10.47270842));
#159264=CARTESIAN_POINT('Ctrl Pts',(1.85508938999994,11.6,-10.47270842));
#159265=CARTESIAN_POINT('Ctrl Pts',(1.85598064599994,15.2,-10.474739628));
#159266=CARTESIAN_POINT('Ctrl Pts',(1.85598064599994,11.6,-10.474739628));
#159267=CARTESIAN_POINT('Ctrl Pts',(1.85687636999994,15.2,-10.476776123));
#159268=CARTESIAN_POINT('Ctrl Pts',(1.85687636999994,11.6,-10.476776123));
#159269=CARTESIAN_POINT('Ctrl Pts',(1.85777656499994,15.2,-10.478817888));
#159270=CARTESIAN_POINT('Ctrl Pts',(1.85777656499994,11.6,-10.478817888));
#159271=CARTESIAN_POINT('Ctrl Pts',(1.85868123399994,15.2,-10.480864906));
#159272=CARTESIAN_POINT('Ctrl Pts',(1.85868123399994,11.6,-10.480864906));
#159273=CARTESIAN_POINT('Ctrl Pts',(1.85959038199994,15.2,-10.48291716));
#159274=CARTESIAN_POINT('Ctrl Pts',(1.85959038199994,11.6,-10.48291716));
#159275=CARTESIAN_POINT('Ctrl Pts',(1.86050401199994,15.2,-10.484974634));
#159276=CARTESIAN_POINT('Ctrl Pts',(1.86050401199994,11.6,-10.484974634));
#159277=CARTESIAN_POINT('Ctrl Pts',(1.86142212899994,15.2,-10.487037312));
#159278=CARTESIAN_POINT('Ctrl Pts',(1.86142212899994,11.6,-10.487037312));
#159279=CARTESIAN_POINT('Ctrl Pts',(1.86234473699994,15.2,-10.489105177));
#159280=CARTESIAN_POINT('Ctrl Pts',(1.86234473699994,11.6,-10.489105177));
#159281=CARTESIAN_POINT('Ctrl Pts',(1.86327183899994,15.2,-10.491178213));
#159282=CARTESIAN_POINT('Ctrl Pts',(1.86327183899994,11.6,-10.491178213));
#159283=CARTESIAN_POINT('Ctrl Pts',(1.86420344099994,15.2,-10.493256403));
#159284=CARTESIAN_POINT('Ctrl Pts',(1.86420344099994,11.6,-10.493256403));
#159285=CARTESIAN_POINT('Ctrl Pts',(1.86513954299994,15.2,-10.49533973));
#159286=CARTESIAN_POINT('Ctrl Pts',(1.86513954299994,11.6,-10.49533973));
#159287=CARTESIAN_POINT('Ctrl Pts',(1.86608015299994,15.2,-10.497428179));
#159288=CARTESIAN_POINT('Ctrl Pts',(1.86608015299994,11.6,-10.497428179));
#159289=CARTESIAN_POINT('Ctrl Pts',(1.86702527199994,15.2,-10.499521733));
#159290=CARTESIAN_POINT('Ctrl Pts',(1.86702527199994,11.6,-10.499521733));
#159291=CARTESIAN_POINT('Ctrl Pts',(1.86797490499994,15.2,-10.501620377));
#159292=CARTESIAN_POINT('Ctrl Pts',(1.86797490499994,11.6,-10.501620377));
#159293=CARTESIAN_POINT('Ctrl Pts',(1.86892905699994,15.2,-10.503724094));
#159294=CARTESIAN_POINT('Ctrl Pts',(1.86892905699994,11.6,-10.503724094));
#159295=CARTESIAN_POINT('Ctrl Pts',(1.86988772999995,15.2,-10.505832868));
#159296=CARTESIAN_POINT('Ctrl Pts',(1.86988772999995,11.6,-10.505832868));
#159297=CARTESIAN_POINT('Ctrl Pts',(1.87085092699994,15.2,-10.507946683));
#159298=CARTESIAN_POINT('Ctrl Pts',(1.87085092699994,11.6,-10.507946683));
#159299=CARTESIAN_POINT('Ctrl Pts',(1.87181865399994,15.2,-10.510065522));
#159300=CARTESIAN_POINT('Ctrl Pts',(1.87181865399994,11.6,-10.510065522));
#159301=CARTESIAN_POINT('Ctrl Pts',(1.87279091299994,15.2,-10.512189371));
#159302=CARTESIAN_POINT('Ctrl Pts',(1.87279091299994,11.6,-10.512189371));
#159303=CARTESIAN_POINT('Ctrl Pts',(1.87376770899994,15.2,-10.514318212));
#159304=CARTESIAN_POINT('Ctrl Pts',(1.87376770899994,11.6,-10.514318212));
#159305=CARTESIAN_POINT('Ctrl Pts',(1.87474904299994,15.2,-10.516452031));
#159306=CARTESIAN_POINT('Ctrl Pts',(1.87474904299994,11.6,-10.516452031));
#159307=CARTESIAN_POINT('Ctrl Pts',(1.87573492299994,15.2,-10.518590811));
#159308=CARTESIAN_POINT('Ctrl Pts',(1.87573492299994,11.6,-10.518590811));
#159309=CARTESIAN_POINT('Ctrl Pts',(1.87672534799994,15.2,-10.520734536));
#159310=CARTESIAN_POINT('Ctrl Pts',(1.87672534799994,11.6,-10.520734536));
#159311=CARTESIAN_POINT('Ctrl Pts',(1.87772032499994,15.2,-10.522883192));
#159312=CARTESIAN_POINT('Ctrl Pts',(1.87772032499994,11.6,-10.522883192));
#159313=CARTESIAN_POINT('Ctrl Pts',(1.87871985699994,15.2,-10.525036762));
#159314=CARTESIAN_POINT('Ctrl Pts',(1.87871985699994,11.6,-10.525036762));
#159315=CARTESIAN_POINT('Ctrl Pts',(1.87972394599994,15.2,-10.52719523));
#159316=CARTESIAN_POINT('Ctrl Pts',(1.87972394599994,11.6,-10.52719523));
#159317=CARTESIAN_POINT('Ctrl Pts',(1.88073259699994,15.2,-10.529358581));
#159318=CARTESIAN_POINT('Ctrl Pts',(1.88073259699994,11.6,-10.529358581));
#159319=CARTESIAN_POINT('Ctrl Pts',(1.88174581199994,15.2,-10.531526798));
#159320=CARTESIAN_POINT('Ctrl Pts',(1.88174581199994,11.6,-10.531526798));
#159321=CARTESIAN_POINT('Ctrl Pts',(1.88276359599994,15.2,-10.533699869));
#159322=CARTESIAN_POINT('Ctrl Pts',(1.88276359599994,11.6,-10.533699869));
#159323=CARTESIAN_POINT('Ctrl Pts',(1.88378595299994,15.2,-10.535877775));
#159324=CARTESIAN_POINT('Ctrl Pts',(1.88378595299994,11.6,-10.535877775));
#159325=CARTESIAN_POINT('Ctrl Pts',(1.88481288399994,15.2,-10.538060503));
#159326=CARTESIAN_POINT('Ctrl Pts',(1.88481288399994,11.6,-10.538060503));
#159327=CARTESIAN_POINT('Ctrl Pts',(1.88584439399994,15.2,-10.540248035));
#159328=CARTESIAN_POINT('Ctrl Pts',(1.88584439399994,11.6,-10.540248035));
#159329=CARTESIAN_POINT('Ctrl Pts',(1.88688048599994,15.2,-10.542440358));
#159330=CARTESIAN_POINT('Ctrl Pts',(1.88688048599994,11.6,-10.542440358));
#159331=CARTESIAN_POINT('Ctrl Pts',(1.88792116399994,15.2,-10.544637455));
#159332=CARTESIAN_POINT('Ctrl Pts',(1.88792116399994,11.6,-10.544637455));
#159333=CARTESIAN_POINT('Ctrl Pts',(1.88896643099994,15.2,-10.546839313));
#159334=CARTESIAN_POINT('Ctrl Pts',(1.88896643099994,11.6,-10.546839313));
#159335=CARTESIAN_POINT('Ctrl Pts',(1.89001628999994,15.2,-10.549045913));
#159336=CARTESIAN_POINT('Ctrl Pts',(1.89001628999994,11.6,-10.549045913));
#159337=CARTESIAN_POINT('Ctrl Pts',(1.89107074499994,15.2,-10.551257244));
#159338=CARTESIAN_POINT('Ctrl Pts',(1.89107074499994,11.6,-10.551257244));
#159339=CARTESIAN_POINT('Ctrl Pts',(1.89212979899994,15.2,-10.553473288));
#159340=CARTESIAN_POINT('Ctrl Pts',(1.89212979899994,11.6,-10.553473288));
#159341=CARTESIAN_POINT('Ctrl Pts',(1.89319345499994,15.2,-10.555694032));
#159342=CARTESIAN_POINT('Ctrl Pts',(1.89319345499994,11.6,-10.555694032));
#159343=CARTESIAN_POINT('Ctrl Pts',(1.89426171599994,15.2,-10.557919458));
#159344=CARTESIAN_POINT('Ctrl Pts',(1.89426171599994,11.6,-10.557919458));
#159345=CARTESIAN_POINT('Ctrl Pts',(1.89533458699994,15.2,-10.560149554));
#159346=CARTESIAN_POINT('Ctrl Pts',(1.89533458699994,11.6,-10.560149554));
#159347=CARTESIAN_POINT('Ctrl Pts',(1.89641206899994,15.2,-10.562384303));
#159348=CARTESIAN_POINT('Ctrl Pts',(1.89641206899994,11.6,-10.562384303));
#159349=CARTESIAN_POINT('Ctrl Pts',(1.89749416599994,15.2,-10.564623691));
#159350=CARTESIAN_POINT('Ctrl Pts',(1.89749416599994,11.6,-10.564623691));
#159351=CARTESIAN_POINT('Ctrl Pts',(1.89858088099994,15.2,-10.566867703));
#159352=CARTESIAN_POINT('Ctrl Pts',(1.89858088099994,11.6,-10.566867703));
#159353=CARTESIAN_POINT('Ctrl Pts',(1.89967221899994,15.2,-10.569116324));
#159354=CARTESIAN_POINT('Ctrl Pts',(1.89967221899994,11.6,-10.569116324));
#159355=CARTESIAN_POINT('Ctrl Pts',(1.90076818099994,15.2,-10.571369539));
#159356=CARTESIAN_POINT('Ctrl Pts',(1.90076818099994,11.6,-10.571369539));
#159357=CARTESIAN_POINT('Ctrl Pts',(1.90186877099994,15.2,-10.573627333));
#159358=CARTESIAN_POINT('Ctrl Pts',(1.90186877099994,11.6,-10.573627333));
#159359=CARTESIAN_POINT('Ctrl Pts',(1.90297399099994,15.2,-10.575889692));
#159360=CARTESIAN_POINT('Ctrl Pts',(1.90297399099994,11.6,-10.575889692));
#159361=CARTESIAN_POINT('Ctrl Pts',(1.90408384599994,15.2,-10.578156601));
#159362=CARTESIAN_POINT('Ctrl Pts',(1.90408384599994,11.6,-10.578156601));
#159363=CARTESIAN_POINT('Ctrl Pts',(1.90519833799994,15.2,-10.580428044));
#159364=CARTESIAN_POINT('Ctrl Pts',(1.90519833799994,11.6,-10.580428044));
#159365=CARTESIAN_POINT('Ctrl Pts',(1.90631746999994,15.2,-10.582704009));
#159366=CARTESIAN_POINT('Ctrl Pts',(1.90631746999994,11.6,-10.582704009));
#159367=CARTESIAN_POINT('Ctrl Pts',(1.90744124499994,15.2,-10.584984479));
#159368=CARTESIAN_POINT('Ctrl Pts',(1.90744124499994,11.6,-10.584984479));
#159369=CARTESIAN_POINT('Ctrl Pts',(1.90856966599994,15.2,-10.587269441));
#159370=CARTESIAN_POINT('Ctrl Pts',(1.90856966599994,11.6,-10.587269441));
#159371=CARTESIAN_POINT('Ctrl Pts',(1.90970273699994,15.2,-10.58955888));
#159372=CARTESIAN_POINT('Ctrl Pts',(1.90970273699994,11.6,-10.58955888));
#159373=CARTESIAN_POINT('Ctrl Pts',(1.91084045999994,15.2,-10.59185278));
#159374=CARTESIAN_POINT('Ctrl Pts',(1.91084045999994,11.6,-10.59185278));
#159375=CARTESIAN_POINT('Ctrl Pts',(1.91198283799994,15.2,-10.594151129));
#159376=CARTESIAN_POINT('Ctrl Pts',(1.91198283799994,11.6,-10.594151129));
#159377=CARTESIAN_POINT('Ctrl Pts',(1.91312987399994,15.2,-10.59645391));
#159378=CARTESIAN_POINT('Ctrl Pts',(1.91312987399994,11.6,-10.59645391));
#159379=CARTESIAN_POINT('Ctrl Pts',(1.91428157099994,15.2,-10.598761112));
#159380=CARTESIAN_POINT('Ctrl Pts',(1.91428157099994,11.6,-10.598761112));
#159381=CARTESIAN_POINT('Ctrl Pts',(1.91543793199994,15.2,-10.601072717));
#159382=CARTESIAN_POINT('Ctrl Pts',(1.91543793199994,11.6,-10.601072717));
#159383=CARTESIAN_POINT('Ctrl Pts',(1.91659895999994,15.2,-10.603388714));
#159384=CARTESIAN_POINT('Ctrl Pts',(1.91659895999994,11.6,-10.603388714));
#159385=CARTESIAN_POINT('Ctrl Pts',(1.91776465699994,15.2,-10.605709085));
#159386=CARTESIAN_POINT('Ctrl Pts',(1.91776465699994,11.6,-10.605709085));
#159387=CARTESIAN_POINT('Ctrl Pts',(1.91893502699994,15.2,-10.60803382));
#159388=CARTESIAN_POINT('Ctrl Pts',(1.91893502699994,11.6,-10.60803382));
#159389=CARTESIAN_POINT('Ctrl Pts',(1.92011007299994,15.2,-10.610362901));
#159390=CARTESIAN_POINT('Ctrl Pts',(1.92011007299994,11.6,-10.610362901));
#159391=CARTESIAN_POINT('Ctrl Pts',(1.92128979599994,15.2,-10.612696316));
#159392=CARTESIAN_POINT('Ctrl Pts',(1.92128979599994,11.6,-10.612696316));
#159393=CARTESIAN_POINT('Ctrl Pts',(1.92247420099994,15.2,-10.615034051));
#159394=CARTESIAN_POINT('Ctrl Pts',(1.92247420099994,11.6,-10.615034051));
#159395=CARTESIAN_POINT('Ctrl Pts',(1.92366328999994,15.2,-10.617376091));
#159396=CARTESIAN_POINT('Ctrl Pts',(1.92366328999994,11.6,-10.617376091));
#159397=CARTESIAN_POINT('Ctrl Pts',(1.92485706499994,15.2,-10.619722422));
#159398=CARTESIAN_POINT('Ctrl Pts',(1.92485706499994,11.6,-10.619722422));
#159399=CARTESIAN_POINT('Ctrl Pts',(1.92605552899994,15.2,-10.622073029));
#159400=CARTESIAN_POINT('Ctrl Pts',(1.92605552899994,11.6,-10.622073029));
#159401=CARTESIAN_POINT('Ctrl Pts',(1.92725868499994,15.2,-10.6244279));
#159402=CARTESIAN_POINT('Ctrl Pts',(1.92725868499994,11.6,-10.6244279));
#159403=CARTESIAN_POINT('Ctrl Pts',(1.92846653599994,15.2,-10.62678702));
#159404=CARTESIAN_POINT('Ctrl Pts',(1.92846653599994,11.6,-10.62678702));
#159405=CARTESIAN_POINT('Ctrl Pts',(1.92967908399994,15.2,-10.629150376));
#159406=CARTESIAN_POINT('Ctrl Pts',(1.92967908399994,11.6,-10.629150376));
#159407=CARTESIAN_POINT('Ctrl Pts',(1.93089633299994,15.2,-10.631517953));
#159408=CARTESIAN_POINT('Ctrl Pts',(1.93089633299994,11.6,-10.631517953));
#159409=CARTESIAN_POINT('Ctrl Pts',(1.93211828499994,15.2,-10.633889738));
#159410=CARTESIAN_POINT('Ctrl Pts',(1.93211828499994,11.6,-10.633889738));
#159411=CARTESIAN_POINT('Ctrl Pts',(1.93334494199994,15.2,-10.636265715));
#159412=CARTESIAN_POINT('Ctrl Pts',(1.93334494199994,11.6,-10.636265715));
#159413=CARTESIAN_POINT('Ctrl Pts',(1.93457630699994,15.2,-10.638645874));
#159414=CARTESIAN_POINT('Ctrl Pts',(1.93457630699994,11.6,-10.638645874));
#159415=CARTESIAN_POINT('Ctrl Pts',(1.93581238299994,15.2,-10.641030197));
#159416=CARTESIAN_POINT('Ctrl Pts',(1.93581238299994,11.6,-10.641030197));
#159417=CARTESIAN_POINT('Ctrl Pts',(1.93705317299994,15.2,-10.643418674));
#159418=CARTESIAN_POINT('Ctrl Pts',(1.93705317299994,11.6,-10.643418674));
#159419=CARTESIAN_POINT('Ctrl Pts',(1.93829867699994,15.2,-10.645811289));
#159420=CARTESIAN_POINT('Ctrl Pts',(1.93829867699994,11.6,-10.645811289));
#159421=CARTESIAN_POINT('Ctrl Pts',(1.93954889999994,15.2,-10.648208029));
#159422=CARTESIAN_POINT('Ctrl Pts',(1.93954889999994,11.6,-10.648208029));
#159423=CARTESIAN_POINT('Ctrl Pts',(1.94080384499994,15.2,-10.650608881));
#159424=CARTESIAN_POINT('Ctrl Pts',(1.94080384499994,11.6,-10.650608881));
#159425=CARTESIAN_POINT('Ctrl Pts',(1.94206351299994,15.2,-10.65301383));
#159426=CARTESIAN_POINT('Ctrl Pts',(1.94206351299994,11.6,-10.65301383));
#159427=CARTESIAN_POINT('Ctrl Pts',(1.94332790699994,15.2,-10.655422864));
#159428=CARTESIAN_POINT('Ctrl Pts',(1.94332790699994,11.6,-10.655422864));
#159429=CARTESIAN_POINT('Ctrl Pts',(1.94459702899994,15.2,-10.657835968));
#159430=CARTESIAN_POINT('Ctrl Pts',(1.94459702899994,11.6,-10.657835968));
#159431=CARTESIAN_POINT('Ctrl Pts',(1.94587088199994,15.2,-10.660253129));
#159432=CARTESIAN_POINT('Ctrl Pts',(1.94587088199994,11.6,-10.660253129));
#159433=CARTESIAN_POINT('Ctrl Pts',(1.94714946899994,15.2,-10.662674334));
#159434=CARTESIAN_POINT('Ctrl Pts',(1.94714946899994,11.6,-10.662674334));
#159435=CARTESIAN_POINT('Ctrl Pts',(1.94843279199994,15.2,-10.665099571));
#159436=CARTESIAN_POINT('Ctrl Pts',(1.94843279199994,11.6,-10.665099571));
#159437=CARTESIAN_POINT('Ctrl Pts',(1.94972085299994,15.2,-10.667528823));
#159438=CARTESIAN_POINT('Ctrl Pts',(1.94972085299994,11.6,-10.667528823));
#159439=CARTESIAN_POINT('Ctrl Pts',(1.95101365499994,15.2,-10.66996208));
#159440=CARTESIAN_POINT('Ctrl Pts',(1.95101365499994,11.6,-10.66996208));
#159441=CARTESIAN_POINT('Ctrl Pts',(1.95231119999994,15.2,-10.672399326));
#159442=CARTESIAN_POINT('Ctrl Pts',(1.95231119999994,11.6,-10.672399326));
#159443=CARTESIAN_POINT('Ctrl Pts',(1.95361349099994,15.2,-10.674840549));
#159444=CARTESIAN_POINT('Ctrl Pts',(1.95361349099994,11.6,-10.674840549));
#159445=CARTESIAN_POINT('Ctrl Pts',(1.95492052999994,15.2,-10.677285737));
#159446=CARTESIAN_POINT('Ctrl Pts',(1.95492052999994,11.6,-10.677285737));
#159447=CARTESIAN_POINT('Ctrl Pts',(1.95623231799994,15.2,-10.679734874));
#159448=CARTESIAN_POINT('Ctrl Pts',(1.95623231799994,11.6,-10.679734874));
#159449=CARTESIAN_POINT('Ctrl Pts',(1.95754885999994,15.2,-10.682187948));
#159450=CARTESIAN_POINT('Ctrl Pts',(1.95754885999994,11.6,-10.682187948));
#159451=CARTESIAN_POINT('Ctrl Pts',(1.95887015699994,15.2,-10.684644947));
#159452=CARTESIAN_POINT('Ctrl Pts',(1.95887015699994,11.6,-10.684644947));
#159453=CARTESIAN_POINT('Ctrl Pts',(1.96019620999994,15.2,-10.687105856));
#159454=CARTESIAN_POINT('Ctrl Pts',(1.96019620999994,11.6,-10.687105856));
#159455=CARTESIAN_POINT('Ctrl Pts',(1.96152702299994,15.2,-10.689570664));
#159456=CARTESIAN_POINT('Ctrl Pts',(1.96152702299994,11.6,-10.689570664));
#159457=CARTESIAN_POINT('Ctrl Pts',(1.96286259899994,15.2,-10.692039356));
#159458=CARTESIAN_POINT('Ctrl Pts',(1.96286259899994,11.6,-10.692039356));
#159459=CARTESIAN_POINT('Ctrl Pts',(1.96420293799994,15.2,-10.694511919));
#159460=CARTESIAN_POINT('Ctrl Pts',(1.96420293799994,11.6,-10.694511919));
#159461=CARTESIAN_POINT('Ctrl Pts',(1.96554804399994,15.2,-10.696988341));
#159462=CARTESIAN_POINT('Ctrl Pts',(1.96554804399994,11.6,-10.696988341));
#159463=CARTESIAN_POINT('Ctrl Pts',(1.96689791799994,15.2,-10.699468609));
#159464=CARTESIAN_POINT('Ctrl Pts',(1.96689791799994,11.6,-10.699468609));
#159465=CARTESIAN_POINT('Ctrl Pts',(1.96825256199994,15.2,-10.70195271));
#159466=CARTESIAN_POINT('Ctrl Pts',(1.96825256199994,11.6,-10.70195271));
#159467=CARTESIAN_POINT('Ctrl Pts',(1.96961197999994,15.2,-10.704440629));
#159468=CARTESIAN_POINT('Ctrl Pts',(1.96961197999994,11.6,-10.704440629));
#159469=CARTESIAN_POINT('Ctrl Pts',(1.97097617299994,15.2,-10.706932355));
#159470=CARTESIAN_POINT('Ctrl Pts',(1.97097617299994,11.6,-10.706932355));
#159471=CARTESIAN_POINT('Ctrl Pts',(1.97234514399994,15.2,-10.709427876));
#159472=CARTESIAN_POINT('Ctrl Pts',(1.97234514399994,11.6,-10.709427876));
#159473=CARTESIAN_POINT('Ctrl Pts',(1.97371889299994,15.2,-10.711927177));
#159474=CARTESIAN_POINT('Ctrl Pts',(1.97371889299994,11.6,-10.711927177));
#159475=CARTESIAN_POINT('Ctrl Pts',(1.97509742499994,15.2,-10.714430247));
#159476=CARTESIAN_POINT('Ctrl Pts',(1.97509742499994,11.6,-10.714430247));
#159477=CARTESIAN_POINT('Ctrl Pts',(1.97648073999994,15.2,-10.716937073));
#159478=CARTESIAN_POINT('Ctrl Pts',(1.97648073999994,11.6,-10.716937073));
#159479=CARTESIAN_POINT('Ctrl Pts',(1.97786884099994,15.2,-10.71944764));
#159480=CARTESIAN_POINT('Ctrl Pts',(1.97786884099994,11.6,-10.71944764));
#159481=CARTESIAN_POINT('Ctrl Pts',(1.97926172999994,15.2,-10.721961937));
#159482=CARTESIAN_POINT('Ctrl Pts',(1.97926172999994,11.6,-10.721961937));
#159483=CARTESIAN_POINT('Ctrl Pts',(1.98065940899994,15.2,-10.724479952));
#159484=CARTESIAN_POINT('Ctrl Pts',(1.98065940899994,11.6,-10.724479952));
#159485=CARTESIAN_POINT('Ctrl Pts',(1.98206188099994,15.2,-10.727001672));
#159486=CARTESIAN_POINT('Ctrl Pts',(1.98206188099994,11.6,-10.727001672));
#159487=CARTESIAN_POINT('Ctrl Pts',(1.98346914499994,15.2,-10.729527083));
#159488=CARTESIAN_POINT('Ctrl Pts',(1.98346914499994,11.6,-10.729527083));
#159489=CARTESIAN_POINT('Ctrl Pts',(1.98488120699994,15.2,-10.732056173));
#159490=CARTESIAN_POINT('Ctrl Pts',(1.98488120699994,11.6,-10.732056173));
#159491=CARTESIAN_POINT('Ctrl Pts',(1.98629806699994,15.2,-10.73458893));
#159492=CARTESIAN_POINT('Ctrl Pts',(1.98629806699994,11.6,-10.73458893));
#159493=CARTESIAN_POINT('Ctrl Pts',(1.98771972699994,15.2,-10.737125341));
#159494=CARTESIAN_POINT('Ctrl Pts',(1.98771972699994,11.6,-10.737125341));
#159495=CARTESIAN_POINT('Ctrl Pts',(1.98914618999994,15.2,-10.739665394));
#159496=CARTESIAN_POINT('Ctrl Pts',(1.98914618999994,11.6,-10.739665394));
#159497=CARTESIAN_POINT('Ctrl Pts',(1.99057745699994,15.2,-10.742209076));
#159498=CARTESIAN_POINT('Ctrl Pts',(1.99057745699994,11.6,-10.742209076));
#159499=CARTESIAN_POINT('Ctrl Pts',(1.99201352899994,15.2,-10.744756374));
#159500=CARTESIAN_POINT('Ctrl Pts',(1.99201352899994,11.6,-10.744756374));
#159501=CARTESIAN_POINT('Ctrl Pts',(1.99345441099994,15.2,-10.747307276));
#159502=CARTESIAN_POINT('Ctrl Pts',(1.99345441099994,11.6,-10.747307276));
#159503=CARTESIAN_POINT('Ctrl Pts',(1.99490010199994,15.2,-10.74986177));
#159504=CARTESIAN_POINT('Ctrl Pts',(1.99490010199994,11.6,-10.74986177));
#159505=CARTESIAN_POINT('Ctrl Pts',(1.99635060499994,15.2,-10.752419844));
#159506=CARTESIAN_POINT('Ctrl Pts',(1.99635060499994,11.6,-10.752419844));
#159507=CARTESIAN_POINT('Ctrl Pts',(1.99780592199994,15.2,-10.754981484));
#159508=CARTESIAN_POINT('Ctrl Pts',(1.99780592199994,11.6,-10.754981484));
#159509=CARTESIAN_POINT('Ctrl Pts',(1.99926605499994,15.2,-10.757546678));
#159510=CARTESIAN_POINT('Ctrl Pts',(1.99926605499994,11.6,-10.757546678));
#159511=CARTESIAN_POINT('Ctrl Pts',(2.00073100599994,15.2,-10.760115415));
#159512=CARTESIAN_POINT('Ctrl Pts',(2.00073100599994,11.6,-10.760115415));
#159513=CARTESIAN_POINT('Ctrl Pts',(2.00220077599994,15.2,-10.762687682));
#159514=CARTESIAN_POINT('Ctrl Pts',(2.00220077599994,11.6,-10.762687682));
#159515=CARTESIAN_POINT('Ctrl Pts',(2.00367536799994,15.2,-10.765263466));
#159516=CARTESIAN_POINT('Ctrl Pts',(2.00367536799994,11.6,-10.765263466));
#159517=CARTESIAN_POINT('Ctrl Pts',(2.00515478199994,15.2,-10.767842756));
#159518=CARTESIAN_POINT('Ctrl Pts',(2.00515478199994,11.6,-10.767842756));
#159519=CARTESIAN_POINT('Ctrl Pts',(2.00663902299994,15.2,-10.77042554));
#159520=CARTESIAN_POINT('Ctrl Pts',(2.00663902299994,11.6,-10.77042554));
#159521=CARTESIAN_POINT('Ctrl Pts',(2.00812808999994,15.2,-10.773011803));
#159522=CARTESIAN_POINT('Ctrl Pts',(2.00812808999994,11.6,-10.773011803));
#159523=CARTESIAN_POINT('Ctrl Pts',(2.00962198599994,15.2,-10.775601537));
#159524=CARTESIAN_POINT('Ctrl Pts',(2.00962198599994,11.6,-10.775601537));
#159525=CARTESIAN_POINT('Ctrl Pts',(2.01112071299994,15.2,-10.778194727));
#159526=CARTESIAN_POINT('Ctrl Pts',(2.01112071299994,11.6,-10.778194727));
#159527=CARTESIAN_POINT('Ctrl Pts',(2.01262427099994,15.2,-10.780791361));
#159528=CARTESIAN_POINT('Ctrl Pts',(2.01262427099994,11.6,-10.780791361));
#159529=CARTESIAN_POINT('Ctrl Pts',(2.01413266399994,15.2,-10.783391428));
#159530=CARTESIAN_POINT('Ctrl Pts',(2.01413266399994,11.6,-10.783391428));
#159531=CARTESIAN_POINT('Ctrl Pts',(2.01564589299994,15.2,-10.785994916));
#159532=CARTESIAN_POINT('Ctrl Pts',(2.01564589299994,11.6,-10.785994916));
#159533=CARTESIAN_POINT('Ctrl Pts',(2.01716395899994,15.2,-10.788601812));
#159534=CARTESIAN_POINT('Ctrl Pts',(2.01716395899994,11.6,-10.788601812));
#159535=CARTESIAN_POINT('Ctrl Pts',(2.01868686499994,15.2,-10.791212104));
#159536=CARTESIAN_POINT('Ctrl Pts',(2.01868686499994,11.6,-10.791212104));
#159537=CARTESIAN_POINT('Ctrl Pts',(2.02021461099994,15.2,-10.793825781));
#159538=CARTESIAN_POINT('Ctrl Pts',(2.02021461099994,11.6,-10.793825781));
#159539=CARTESIAN_POINT('Ctrl Pts',(2.02174720099995,15.2,-10.796442831));
#159540=CARTESIAN_POINT('Ctrl Pts',(2.02174720099995,11.6,-10.796442831));
#159541=CARTESIAN_POINT('Ctrl Pts',(2.02328463399994,15.2,-10.799063241));
#159542=CARTESIAN_POINT('Ctrl Pts',(2.02328463399994,11.6,-10.799063241));
#159543=CARTESIAN_POINT('Ctrl Pts',(2.02482691399994,15.2,-10.801687));
#159544=CARTESIAN_POINT('Ctrl Pts',(2.02482691399994,11.6,-10.801687));
#159545=CARTESIAN_POINT('Ctrl Pts',(2.02637404199994,15.2,-10.804314097));
#159546=CARTESIAN_POINT('Ctrl Pts',(2.02637404199994,11.6,-10.804314097));
#159547=CARTESIAN_POINT('Ctrl Pts',(2.02792601899994,15.2,-10.806944517));
#159548=CARTESIAN_POINT('Ctrl Pts',(2.02792601899994,11.6,-10.806944517));
#159549=CARTESIAN_POINT('Ctrl Pts',(2.02948284599994,15.2,-10.809578251));
#159550=CARTESIAN_POINT('Ctrl Pts',(2.02948284599994,11.6,-10.809578251));
#159551=CARTESIAN_POINT('Ctrl Pts',(2.03104452699994,15.2,-10.812215287));
#159552=CARTESIAN_POINT('Ctrl Pts',(2.03104452699994,11.6,-10.812215287));
#159553=CARTESIAN_POINT('Ctrl Pts',(2.03261106199994,15.2,-10.814855611));
#159554=CARTESIAN_POINT('Ctrl Pts',(2.03261106199994,11.6,-10.814855611));
#159555=CARTESIAN_POINT('Ctrl Pts',(2.03418245199994,15.2,-10.817499214));
#159556=CARTESIAN_POINT('Ctrl Pts',(2.03418245199994,11.6,-10.817499214));
#159557=CARTESIAN_POINT('Ctrl Pts',(2.03575870099994,15.2,-10.820146083));
#159558=CARTESIAN_POINT('Ctrl Pts',(2.03575870099994,11.6,-10.820146083));
#159559=CARTESIAN_POINT('Ctrl Pts',(2.03733980799994,15.2,-10.822796206));
#159560=CARTESIAN_POINT('Ctrl Pts',(2.03733980799994,11.6,-10.822796206));
#159561=CARTESIAN_POINT('Ctrl Pts',(2.03892577499994,15.2,-10.825449572));
#159562=CARTESIAN_POINT('Ctrl Pts',(2.03892577499994,11.6,-10.825449572));
#159563=CARTESIAN_POINT('Ctrl Pts',(2.04051660599994,15.2,-10.82810617));
#159564=CARTESIAN_POINT('Ctrl Pts',(2.04051660599994,11.6,-10.82810617));
#159565=CARTESIAN_POINT('Ctrl Pts',(2.04211229899994,15.2,-10.830765986));
#159566=CARTESIAN_POINT('Ctrl Pts',(2.04211229899994,11.6,-10.830765986));
#159567=CARTESIAN_POINT('Ctrl Pts',(2.04371285699994,15.2,-10.833429011));
#159568=CARTESIAN_POINT('Ctrl Pts',(2.04371285699994,11.6,-10.833429011));
#159569=CARTESIAN_POINT('Ctrl Pts',(2.04531828199995,15.2,-10.836095232));
#159570=CARTESIAN_POINT('Ctrl Pts',(2.04531828199995,11.6,-10.836095232));
#159571=CARTESIAN_POINT('Ctrl Pts',(2.04692857599994,15.2,-10.838764637));
#159572=CARTESIAN_POINT('Ctrl Pts',(2.04692857599994,11.6,-10.838764637));
#159573=CARTESIAN_POINT('Ctrl Pts',(2.04854373899995,15.2,-10.841437216));
#159574=CARTESIAN_POINT('Ctrl Pts',(2.04854373899995,11.6,-10.841437216));
#159575=CARTESIAN_POINT('Ctrl Pts',(2.05016377299994,15.2,-10.844112955));
#159576=CARTESIAN_POINT('Ctrl Pts',(2.05016377299994,11.6,-10.844112955));
#159577=CARTESIAN_POINT('Ctrl Pts',(2.05178868099994,15.2,-10.846791846));
#159578=CARTESIAN_POINT('Ctrl Pts',(2.05178868099994,11.6,-10.846791846));
#159579=CARTESIAN_POINT('Ctrl Pts',(2.05341846199994,15.2,-10.849473875));
#159580=CARTESIAN_POINT('Ctrl Pts',(2.05341846199994,11.6,-10.849473875));
#159581=CARTESIAN_POINT('Ctrl Pts',(2.05505311799994,15.2,-10.852159032));
#159582=CARTESIAN_POINT('Ctrl Pts',(2.05505311799994,11.6,-10.852159032));
#159583=CARTESIAN_POINT('Ctrl Pts',(2.05669265099994,15.2,-10.854847303));
#159584=CARTESIAN_POINT('Ctrl Pts',(2.05669265099994,11.6,-10.854847303));
#159585=CARTESIAN_POINT('Ctrl Pts',(2.05833706199994,15.2,-10.85753868));
#159586=CARTESIAN_POINT('Ctrl Pts',(2.05833706199994,11.6,-10.85753868));
#159587=CARTESIAN_POINT('Ctrl Pts',(2.05998635399994,15.2,-10.86023315));
#159588=CARTESIAN_POINT('Ctrl Pts',(2.05998635399994,11.6,-10.86023315));
#159589=CARTESIAN_POINT('Ctrl Pts',(2.06164052499994,15.2,-10.862930702));
#159590=CARTESIAN_POINT('Ctrl Pts',(2.06164052499994,11.6,-10.862930702));
#159591=CARTESIAN_POINT('Ctrl Pts',(2.06329958099994,15.2,-10.865631323));
#159592=CARTESIAN_POINT('Ctrl Pts',(2.06329958099994,11.6,-10.865631323));
#159593=CARTESIAN_POINT('Ctrl Pts',(2.06496351899994,15.2,-10.868335004));
#159594=CARTESIAN_POINT('Ctrl Pts',(2.06496351899994,11.6,-10.868335004));
#159595=CARTESIAN_POINT('Ctrl Pts',(2.06663234299994,15.2,-10.871041734));
#159596=CARTESIAN_POINT('Ctrl Pts',(2.06663234299994,11.6,-10.871041734));
#159597=CARTESIAN_POINT('Ctrl Pts',(2.06830605399994,15.2,-10.873751499));
#159598=CARTESIAN_POINT('Ctrl Pts',(2.06830605399994,11.6,-10.873751499));
#159599=CARTESIAN_POINT('Ctrl Pts',(2.06998465199994,15.2,-10.876464289));
#159600=CARTESIAN_POINT('Ctrl Pts',(2.06998465199994,11.6,-10.876464289));
#159601=CARTESIAN_POINT('Ctrl Pts',(2.07166813899994,15.2,-10.879180094));
#159602=CARTESIAN_POINT('Ctrl Pts',(2.07166813899994,11.6,-10.879180094));
#159603=CARTESIAN_POINT('Ctrl Pts',(2.07335651799994,15.2,-10.881898902));
#159604=CARTESIAN_POINT('Ctrl Pts',(2.07335651799994,11.6,-10.881898902));
#159605=CARTESIAN_POINT('Ctrl Pts',(2.07504978799994,15.2,-10.884620701));
#159606=CARTESIAN_POINT('Ctrl Pts',(2.07504978799994,11.6,-10.884620701));
#159607=CARTESIAN_POINT('Ctrl Pts',(2.07674794999994,15.2,-10.887345482));
#159608=CARTESIAN_POINT('Ctrl Pts',(2.07674794999994,11.6,-10.887345482));
#159609=CARTESIAN_POINT('Ctrl Pts',(2.07845100699994,15.2,-10.890073231));
#159610=CARTESIAN_POINT('Ctrl Pts',(2.07845100699994,11.6,-10.890073231));
#159611=CARTESIAN_POINT('Ctrl Pts',(2.08015896099994,15.2,-10.89280394));
#159612=CARTESIAN_POINT('Ctrl Pts',(2.08015896099994,11.6,-10.89280394));
#159613=CARTESIAN_POINT('Ctrl Pts',(2.08187181099994,15.2,-10.895537595));
#159614=CARTESIAN_POINT('Ctrl Pts',(2.08187181099994,11.6,-10.895537595));
#159615=CARTESIAN_POINT('Ctrl Pts',(2.08358955799994,15.2,-10.898274186));
#159616=CARTESIAN_POINT('Ctrl Pts',(2.08358955799994,11.6,-10.898274186));
#159617=CARTESIAN_POINT('Ctrl Pts',(2.08531220499994,15.2,-10.901013703));
#159618=CARTESIAN_POINT('Ctrl Pts',(2.08531220499994,11.6,-10.901013703));
#159619=CARTESIAN_POINT('Ctrl Pts',(2.08703975299994,15.2,-10.903756135));
#159620=CARTESIAN_POINT('Ctrl Pts',(2.08703975299994,11.6,-10.903756135));
#159621=CARTESIAN_POINT('Ctrl Pts',(2.08877220299994,15.2,-10.906501469));
#159622=CARTESIAN_POINT('Ctrl Pts',(2.08877220299994,11.6,-10.906501469));
#159623=CARTESIAN_POINT('Ctrl Pts',(2.09050955499994,15.2,-10.909249695));
#159624=CARTESIAN_POINT('Ctrl Pts',(2.09050955499994,11.6,-10.909249695));
#159625=CARTESIAN_POINT('Ctrl Pts',(2.09225181099994,15.2,-10.912000804));
#159626=CARTESIAN_POINT('Ctrl Pts',(2.09225181099994,11.6,-10.912000804));
#159627=CARTESIAN_POINT('Ctrl Pts',(2.09399897299994,15.2,-10.914754782));
#159628=CARTESIAN_POINT('Ctrl Pts',(2.09399897299994,11.6,-10.914754782));
#159629=CARTESIAN_POINT('Ctrl Pts',(2.09575104199994,15.2,-10.91751162));
#159630=CARTESIAN_POINT('Ctrl Pts',(2.09575104199994,11.6,-10.91751162));
#159631=CARTESIAN_POINT('Ctrl Pts',(2.09750801799994,15.2,-10.920271306));
#159632=CARTESIAN_POINT('Ctrl Pts',(2.09750801799994,11.6,-10.920271306));
#159633=CARTESIAN_POINT('Ctrl Pts',(2.09926990199994,15.2,-10.92303383));
#159634=CARTESIAN_POINT('Ctrl Pts',(2.09926990199994,11.6,-10.92303383));
#159635=CARTESIAN_POINT('Ctrl Pts',(2.10103669699994,15.2,-10.925799182));
#159636=CARTESIAN_POINT('Ctrl Pts',(2.10103669699994,11.6,-10.925799182));
#159637=CARTESIAN_POINT('Ctrl Pts',(2.10280840299994,15.2,-10.928567349));
#159638=CARTESIAN_POINT('Ctrl Pts',(2.10280840299994,11.6,-10.928567349));
#159639=CARTESIAN_POINT('Ctrl Pts',(2.10458501999994,15.2,-10.931338321));
#159640=CARTESIAN_POINT('Ctrl Pts',(2.10458501999994,11.6,-10.931338321));
#159641=CARTESIAN_POINT('Ctrl Pts',(2.10636655199994,15.2,-10.934112088));
#159642=CARTESIAN_POINT('Ctrl Pts',(2.10636655199994,11.6,-10.934112088));
#159643=CARTESIAN_POINT('Ctrl Pts',(2.10815299699994,15.2,-10.936888638));
#159644=CARTESIAN_POINT('Ctrl Pts',(2.10815299699994,11.6,-10.936888638));
#159645=CARTESIAN_POINT('Ctrl Pts',(2.10994435799994,15.2,-10.939667962));
#159646=CARTESIAN_POINT('Ctrl Pts',(2.10994435799994,11.6,-10.939667962));
#159647=CARTESIAN_POINT('Ctrl Pts',(2.11174063499994,15.2,-10.942450048));
#159648=CARTESIAN_POINT('Ctrl Pts',(2.11174063499994,11.6,-10.942450048));
#159649=CARTESIAN_POINT('Ctrl Pts',(2.11354182899994,15.2,-10.945234885));
#159650=CARTESIAN_POINT('Ctrl Pts',(2.11354182899994,11.6,-10.945234885));
#159651=CARTESIAN_POINT('Ctrl Pts',(2.11534794299994,15.2,-10.948022463));
#159652=CARTESIAN_POINT('Ctrl Pts',(2.11534794299994,11.6,-10.948022463));
#159653=CARTESIAN_POINT('Ctrl Pts',(2.11715897499994,15.2,-10.950812772));
#159654=CARTESIAN_POINT('Ctrl Pts',(2.11715897499994,11.6,-10.950812772));
#159655=CARTESIAN_POINT('Ctrl Pts',(2.11897492799995,15.2,-10.953605801));
#159656=CARTESIAN_POINT('Ctrl Pts',(2.11897492799995,11.6,-10.953605801));
#159657=CARTESIAN_POINT('Ctrl Pts',(2.12079580299994,15.2,-10.956401537));
#159658=CARTESIAN_POINT('Ctrl Pts',(2.12079580299994,11.6,-10.956401537));
#159659=CARTESIAN_POINT('Ctrl Pts',(2.12262159999994,15.2,-10.959199973));
#159660=CARTESIAN_POINT('Ctrl Pts',(2.12262159999994,11.6,-10.959199973));
#159661=CARTESIAN_POINT('Ctrl Pts',(2.12445232199994,15.2,-10.962001096));
#159662=CARTESIAN_POINT('Ctrl Pts',(2.12445232199994,11.6,-10.962001096));
#159663=CARTESIAN_POINT('Ctrl Pts',(2.12628796699994,15.2,-10.964804897));
#159664=CARTESIAN_POINT('Ctrl Pts',(2.12628796699994,11.6,-10.964804897));
#159665=CARTESIAN_POINT('Ctrl Pts',(2.12812853899994,15.2,-10.967611364));
#159666=CARTESIAN_POINT('Ctrl Pts',(2.12812853899994,11.6,-10.967611364));
#159667=CARTESIAN_POINT('Ctrl Pts',(2.12997403599994,15.2,-10.970420488));
#159668=CARTESIAN_POINT('Ctrl Pts',(2.12997403599994,11.6,-10.970420488));
#159669=CARTESIAN_POINT('Ctrl Pts',(2.13182446099994,15.2,-10.973232257));
#159670=CARTESIAN_POINT('Ctrl Pts',(2.13182446099994,11.6,-10.973232257));
#159671=CARTESIAN_POINT('Ctrl Pts',(2.13367981499994,15.2,-10.976046662));
#159672=CARTESIAN_POINT('Ctrl Pts',(2.13367981499994,11.6,-10.976046662));
#159673=CARTESIAN_POINT('Ctrl Pts',(2.13554009799994,15.2,-10.978863691));
#159674=CARTESIAN_POINT('Ctrl Pts',(2.13554009799994,11.6,-10.978863691));
#159675=CARTESIAN_POINT('Ctrl Pts',(2.13740531099994,15.2,-10.981683335));
#159676=CARTESIAN_POINT('Ctrl Pts',(2.13740531099994,11.6,-10.981683335));
#159677=CARTESIAN_POINT('Ctrl Pts',(2.13927545499994,15.2,-10.984505583));
#159678=CARTESIAN_POINT('Ctrl Pts',(2.13927545499994,11.6,-10.984505583));
#159679=CARTESIAN_POINT('Ctrl Pts',(2.14115053099994,15.2,-10.987330423));
#159680=CARTESIAN_POINT('Ctrl Pts',(2.14115053099994,11.6,-10.987330423));
#159681=CARTESIAN_POINT('Ctrl Pts',(2.14303053999994,15.2,-10.990157848));
#159682=CARTESIAN_POINT('Ctrl Pts',(2.14303053999994,11.6,-10.990157848));
#159683=CARTESIAN_POINT('Ctrl Pts',(2.14491548299994,15.2,-10.992987845));
#159684=CARTESIAN_POINT('Ctrl Pts',(2.14491548299994,11.6,-10.992987845));
#159685=CARTESIAN_POINT('Ctrl Pts',(2.14680536099995,15.2,-10.995820404));
#159686=CARTESIAN_POINT('Ctrl Pts',(2.14680536099995,11.6,-10.995820404));
#159687=CARTESIAN_POINT('Ctrl Pts',(2.14870017399994,15.2,-10.998655516));
#159688=CARTESIAN_POINT('Ctrl Pts',(2.14870017399994,11.6,-10.998655516));
#159689=CARTESIAN_POINT('Ctrl Pts',(2.15059992399994,15.2,-11.00149317));
#159690=CARTESIAN_POINT('Ctrl Pts',(2.15059992399994,11.6,-11.00149317));
#159691=CARTESIAN_POINT('Ctrl Pts',(2.15250460999994,15.2,-11.004333355));
#159692=CARTESIAN_POINT('Ctrl Pts',(2.15250460999994,11.6,-11.004333355));
#159693=CARTESIAN_POINT('Ctrl Pts',(2.15441423499994,15.2,-11.007176061));
#159694=CARTESIAN_POINT('Ctrl Pts',(2.15441423499994,11.6,-11.007176061));
#159695=CARTESIAN_POINT('Ctrl Pts',(2.15632879899994,15.2,-11.010021278));
#159696=CARTESIAN_POINT('Ctrl Pts',(2.15632879899994,11.6,-11.010021278));
#159697=CARTESIAN_POINT('Ctrl Pts',(2.15824830199994,15.2,-11.012868997));
#159698=CARTESIAN_POINT('Ctrl Pts',(2.15824830199994,11.6,-11.012868997));
#159699=CARTESIAN_POINT('Ctrl Pts',(2.16017274599994,15.2,-11.015719205));
#159700=CARTESIAN_POINT('Ctrl Pts',(2.16017274599994,11.6,-11.015719205));
#159701=CARTESIAN_POINT('Ctrl Pts',(2.16210213199994,15.2,-11.018571894));
#159702=CARTESIAN_POINT('Ctrl Pts',(2.16210213199994,11.6,-11.018571894));
#159703=CARTESIAN_POINT('Ctrl Pts',(2.16403645899994,15.2,-11.021427054));
#159704=CARTESIAN_POINT('Ctrl Pts',(2.16403645899994,11.6,-11.021427054));
#159705=CARTESIAN_POINT('Ctrl Pts',(2.16597572899994,15.2,-11.024284674));
#159706=CARTESIAN_POINT('Ctrl Pts',(2.16597572899994,11.6,-11.024284674));
#159707=CARTESIAN_POINT('Ctrl Pts',(2.16791994199994,15.2,-11.027144743));
#159708=CARTESIAN_POINT('Ctrl Pts',(2.16791994199994,11.6,-11.027144743));
#159709=CARTESIAN_POINT('Ctrl Pts',(2.16986909999994,15.2,-11.030007252));
#159710=CARTESIAN_POINT('Ctrl Pts',(2.16986909999994,11.6,-11.030007252));
#159711=CARTESIAN_POINT('Ctrl Pts',(2.17182320399994,15.2,-11.032872191));
#159712=CARTESIAN_POINT('Ctrl Pts',(2.17182320399994,11.6,-11.032872191));
#159713=CARTESIAN_POINT('Ctrl Pts',(2.17378225199994,15.2,-11.03573955));
#159714=CARTESIAN_POINT('Ctrl Pts',(2.17378225199994,11.6,-11.03573955));
#159715=CARTESIAN_POINT('Ctrl Pts',(2.17574624699994,15.2,-11.038609318));
#159716=CARTESIAN_POINT('Ctrl Pts',(2.17574624699994,11.6,-11.038609318));
#159717=CARTESIAN_POINT('Ctrl Pts',(2.17771518999994,15.2,-11.041481486));
#159718=CARTESIAN_POINT('Ctrl Pts',(2.17771518999994,11.6,-11.041481486));
#159719=CARTESIAN_POINT('Ctrl Pts',(2.17968908099994,15.2,-11.044356044));
#159720=CARTESIAN_POINT('Ctrl Pts',(2.17968908099994,11.6,-11.044356044));
#159721=CARTESIAN_POINT('Ctrl Pts',(2.18166791999994,15.2,-11.047232981));
#159722=CARTESIAN_POINT('Ctrl Pts',(2.18166791999994,11.6,-11.047232981));
#159723=CARTESIAN_POINT('Ctrl Pts',(2.18365170899994,15.2,-11.050112287));
#159724=CARTESIAN_POINT('Ctrl Pts',(2.18365170899994,11.6,-11.050112287));
#159725=CARTESIAN_POINT('Ctrl Pts',(2.18564044699994,15.2,-11.052993953));
#159726=CARTESIAN_POINT('Ctrl Pts',(2.18564044699994,11.6,-11.052993953));
#159727=CARTESIAN_POINT('Ctrl Pts',(2.18763413599994,15.2,-11.055877969));
#159728=CARTESIAN_POINT('Ctrl Pts',(2.18763413599994,11.6,-11.055877969));
#159729=CARTESIAN_POINT('Ctrl Pts',(2.18963277699994,15.2,-11.058764325));
#159730=CARTESIAN_POINT('Ctrl Pts',(2.18963277699994,11.6,-11.058764325));
#159731=CARTESIAN_POINT('Ctrl Pts',(2.19163636999994,15.2,-11.06165301));
#159732=CARTESIAN_POINT('Ctrl Pts',(2.19163636999994,11.6,-11.06165301));
#159733=CARTESIAN_POINT('Ctrl Pts',(2.19364491499995,15.2,-11.064544015));
#159734=CARTESIAN_POINT('Ctrl Pts',(2.19364491499995,11.6,-11.064544015));
#159735=CARTESIAN_POINT('Ctrl Pts',(2.19565841299994,15.2,-11.067437331));
#159736=CARTESIAN_POINT('Ctrl Pts',(2.19565841299994,11.6,-11.067437331));
#159737=CARTESIAN_POINT('Ctrl Pts',(2.19767686499994,15.2,-11.070332945));
#159738=CARTESIAN_POINT('Ctrl Pts',(2.19767686499994,11.6,-11.070332945));
#159739=CARTESIAN_POINT('Ctrl Pts',(2.19970027199994,15.2,-11.073230851));
#159740=CARTESIAN_POINT('Ctrl Pts',(2.19970027199994,11.6,-11.073230851));
#159741=CARTESIAN_POINT('Ctrl Pts',(2.20172863299994,15.2,-11.076131037));
#159742=CARTESIAN_POINT('Ctrl Pts',(2.20172863299994,11.6,-11.076131037));
#159743=CARTESIAN_POINT('Ctrl Pts',(2.20376195099994,15.2,-11.079033493));
#159744=CARTESIAN_POINT('Ctrl Pts',(2.20376195099994,11.6,-11.079033493));
#159745=CARTESIAN_POINT('Ctrl Pts',(2.20580022499994,15.2,-11.081938212));
#159746=CARTESIAN_POINT('Ctrl Pts',(2.20580022499994,11.6,-11.081938212));
#159747=CARTESIAN_POINT('Ctrl Pts',(2.20784345599994,15.2,-11.08484518));
#159748=CARTESIAN_POINT('Ctrl Pts',(2.20784345599994,11.6,-11.08484518));
#159749=CARTESIAN_POINT('Ctrl Pts',(2.20989164299994,15.2,-11.08775439));
#159750=CARTESIAN_POINT('Ctrl Pts',(2.20989164299994,11.6,-11.08775439));
#159751=CARTESIAN_POINT('Ctrl Pts',(2.21194478899994,15.2,-11.090665832));
#159752=CARTESIAN_POINT('Ctrl Pts',(2.21194478899994,11.6,-11.090665832));
#159753=CARTESIAN_POINT('Ctrl Pts',(2.21400289399994,15.2,-11.093579495));
#159754=CARTESIAN_POINT('Ctrl Pts',(2.21400289399994,11.6,-11.093579495));
#159755=CARTESIAN_POINT('Ctrl Pts',(2.21606595699994,15.2,-11.096495371));
#159756=CARTESIAN_POINT('Ctrl Pts',(2.21606595699994,11.6,-11.096495371));
#159757=CARTESIAN_POINT('Ctrl Pts',(2.21813398099994,15.2,-11.099413448));
#159758=CARTESIAN_POINT('Ctrl Pts',(2.21813398099994,11.6,-11.099413448));
#159759=CARTESIAN_POINT('Ctrl Pts',(2.22020696299994,15.2,-11.10233372));
#159760=CARTESIAN_POINT('Ctrl Pts',(2.22020696299994,11.6,-11.10233372));
#159761=CARTESIAN_POINT('Ctrl Pts',(2.22228490799994,15.2,-11.105256173));
#159762=CARTESIAN_POINT('Ctrl Pts',(2.22228490799994,11.6,-11.105256173));
#159763=CARTESIAN_POINT('Ctrl Pts',(2.22436781299994,15.2,-11.1081808));
#159764=CARTESIAN_POINT('Ctrl Pts',(2.22436781299994,11.6,-11.1081808));
#159765=CARTESIAN_POINT('Ctrl Pts',(2.22645567899994,15.2,-11.111107592));
#159766=CARTESIAN_POINT('Ctrl Pts',(2.22645567899994,11.6,-11.111107592));
#159767=CARTESIAN_POINT('Ctrl Pts',(2.22854850699994,15.2,-11.114036538));
#159768=CARTESIAN_POINT('Ctrl Pts',(2.22854850699994,11.6,-11.114036538));
#159769=CARTESIAN_POINT('Ctrl Pts',(2.23064629799994,15.2,-11.116967627));
#159770=CARTESIAN_POINT('Ctrl Pts',(2.23064629799994,11.6,-11.116967627));
#159771=CARTESIAN_POINT('Ctrl Pts',(2.23274905199994,15.2,-11.119900853));
#159772=CARTESIAN_POINT('Ctrl Pts',(2.23274905199994,11.6,-11.119900853));
#159773=CARTESIAN_POINT('Ctrl Pts',(2.23485676999994,15.2,-11.122836204));
#159774=CARTESIAN_POINT('Ctrl Pts',(2.23485676999994,11.6,-11.122836204));
#159775=CARTESIAN_POINT('Ctrl Pts',(2.23696945199995,15.2,-11.125773671));
#159776=CARTESIAN_POINT('Ctrl Pts',(2.23696945199995,11.6,-11.125773671));
#159777=CARTESIAN_POINT('Ctrl Pts',(2.23908709799994,15.2,-11.128713243));
#159778=CARTESIAN_POINT('Ctrl Pts',(2.23908709799994,11.6,-11.128713243));
#159779=CARTESIAN_POINT('Ctrl Pts',(2.24120970899994,15.2,-11.131654914));
#159780=CARTESIAN_POINT('Ctrl Pts',(2.24120970899994,11.6,-11.131654914));
#159781=CARTESIAN_POINT('Ctrl Pts',(2.24333728499994,15.2,-11.134598671));
#159782=CARTESIAN_POINT('Ctrl Pts',(2.24333728499994,11.6,-11.134598671));
#159783=CARTESIAN_POINT('Ctrl Pts',(2.24546982699994,15.2,-11.137544507));
#159784=CARTESIAN_POINT('Ctrl Pts',(2.24546982699994,11.6,-11.137544507));
#159785=CARTESIAN_POINT('Ctrl Pts',(2.24760733499994,15.2,-11.140492411));
#159786=CARTESIAN_POINT('Ctrl Pts',(2.24760733499994,11.6,-11.140492411));
#159787=CARTESIAN_POINT('Ctrl Pts',(2.24974980999994,15.2,-11.143442374));
#159788=CARTESIAN_POINT('Ctrl Pts',(2.24974980999994,11.6,-11.143442374));
#159789=CARTESIAN_POINT('Ctrl Pts',(2.25189725099994,15.2,-11.146394387));
#159790=CARTESIAN_POINT('Ctrl Pts',(2.25189725099994,11.6,-11.146394387));
#159791=CARTESIAN_POINT('Ctrl Pts',(2.25404965899994,15.2,-11.14934844));
#159792=CARTESIAN_POINT('Ctrl Pts',(2.25404965899994,11.6,-11.14934844));
#159793=CARTESIAN_POINT('Ctrl Pts',(2.25620703599994,15.2,-11.152304524));
#159794=CARTESIAN_POINT('Ctrl Pts',(2.25620703599994,11.6,-11.152304524));
#159795=CARTESIAN_POINT('Ctrl Pts',(2.25836937999994,15.2,-11.15526263));
#159796=CARTESIAN_POINT('Ctrl Pts',(2.25836937999994,11.6,-11.15526263));
#159797=CARTESIAN_POINT('Ctrl Pts',(2.26053669299994,15.2,-11.158222747));
#159798=CARTESIAN_POINT('Ctrl Pts',(2.26053669299994,11.6,-11.158222747));
#159799=CARTESIAN_POINT('Ctrl Pts',(2.26270897299994,15.2,-11.161184868));
#159800=CARTESIAN_POINT('Ctrl Pts',(2.26270897299994,11.6,-11.161184868));
#159801=CARTESIAN_POINT('Ctrl Pts',(2.26488622499994,15.2,-11.164148983));
#159802=CARTESIAN_POINT('Ctrl Pts',(2.26488622499994,11.6,-11.164148983));
#159803=CARTESIAN_POINT('Ctrl Pts',(2.26706844499994,15.2,-11.16711508));
#159804=CARTESIAN_POINT('Ctrl Pts',(2.26706844499994,11.6,-11.16711508));
#159805=CARTESIAN_POINT('Ctrl Pts',(2.26925563399994,15.2,-11.170083153));
#159806=CARTESIAN_POINT('Ctrl Pts',(2.26925563399994,11.6,-11.170083153));
#159807=CARTESIAN_POINT('Ctrl Pts',(2.27144779299994,15.2,-11.173053191));
#159808=CARTESIAN_POINT('Ctrl Pts',(2.27144779299994,11.6,-11.173053191));
#159809=CARTESIAN_POINT('Ctrl Pts',(2.27364492299994,15.2,-11.176025185));
#159810=CARTESIAN_POINT('Ctrl Pts',(2.27364492299994,11.6,-11.176025185));
#159811=CARTESIAN_POINT('Ctrl Pts',(2.27584702399994,15.2,-11.178999126));
#159812=CARTESIAN_POINT('Ctrl Pts',(2.27584702399994,11.6,-11.178999126));
#159813=CARTESIAN_POINT('Ctrl Pts',(2.27805409499994,15.2,-11.181975005));
#159814=CARTESIAN_POINT('Ctrl Pts',(2.27805409499994,11.6,-11.181975005));
#159815=CARTESIAN_POINT('Ctrl Pts',(2.28026613799994,15.2,-11.184952813));
#159816=CARTESIAN_POINT('Ctrl Pts',(2.28026613799994,11.6,-11.184952813));
#159817=CARTESIAN_POINT('Ctrl Pts',(2.28248315299994,15.2,-11.187932541));
#159818=CARTESIAN_POINT('Ctrl Pts',(2.28248315299994,11.6,-11.187932541));
#159819=CARTESIAN_POINT('Ctrl Pts',(2.28470513799994,15.2,-11.190914179));
#159820=CARTESIAN_POINT('Ctrl Pts',(2.28470513799994,11.6,-11.190914179));
#159821=CARTESIAN_POINT('Ctrl Pts',(2.28693209699994,15.2,-11.193897718));
#159822=CARTESIAN_POINT('Ctrl Pts',(2.28693209699994,11.6,-11.193897718));
#159823=CARTESIAN_POINT('Ctrl Pts',(2.28916402699994,15.2,-11.19688315));
#159824=CARTESIAN_POINT('Ctrl Pts',(2.28916402699994,11.6,-11.19688315));
#159825=CARTESIAN_POINT('Ctrl Pts',(2.29140092999994,15.2,-11.199870463));
#159826=CARTESIAN_POINT('Ctrl Pts',(2.29140092999994,11.6,-11.199870463));
#159827=CARTESIAN_POINT('Ctrl Pts',(2.29364280599994,15.2,-11.202859649));
#159828=CARTESIAN_POINT('Ctrl Pts',(2.29364280599994,11.6,-11.202859649));
#159829=CARTESIAN_POINT('Ctrl Pts',(2.29588965499994,15.2,-11.205850698));
#159830=CARTESIAN_POINT('Ctrl Pts',(2.29588965499994,11.6,-11.205850698));
#159831=CARTESIAN_POINT('Ctrl Pts',(2.29814147699994,15.2,-11.208843602));
#159832=CARTESIAN_POINT('Ctrl Pts',(2.29814147699994,11.6,-11.208843602));
#159833=CARTESIAN_POINT('Ctrl Pts',(2.30039827299994,15.2,-11.211838352));
#159834=CARTESIAN_POINT('Ctrl Pts',(2.30039827299994,11.6,-11.211838352));
#159835=CARTESIAN_POINT('Ctrl Pts',(2.30266004099994,15.2,-11.214834939));
#159836=CARTESIAN_POINT('Ctrl Pts',(2.30266004099994,11.6,-11.214834939));
#159837=CARTESIAN_POINT('Ctrl Pts',(2.30492678499994,15.2,-11.217833355));
#159838=CARTESIAN_POINT('Ctrl Pts',(2.30492678499994,11.6,-11.217833355));
#159839=CARTESIAN_POINT('Ctrl Pts',(2.30719850199994,15.2,-11.220833593));
#159840=CARTESIAN_POINT('Ctrl Pts',(2.30719850199994,11.6,-11.220833593));
#159841=CARTESIAN_POINT('Ctrl Pts',(2.30947519299994,15.2,-11.223835644));
#159842=CARTESIAN_POINT('Ctrl Pts',(2.30947519299994,11.6,-11.223835644));
#159843=CARTESIAN_POINT('Ctrl Pts',(2.31175685799994,15.2,-11.226839497));
#159844=CARTESIAN_POINT('Ctrl Pts',(2.31175685799994,11.6,-11.226839497));
#159845=CARTESIAN_POINT('Ctrl Pts',(2.31404349799994,15.2,-11.229845144));
#159846=CARTESIAN_POINT('Ctrl Pts',(2.31404349799994,11.6,-11.229845144));
#159847=CARTESIAN_POINT('Ctrl Pts',(2.31633511299994,15.2,-11.232852572));
#159848=CARTESIAN_POINT('Ctrl Pts',(2.31633511299994,11.6,-11.232852572));
#159849=CARTESIAN_POINT('Ctrl Pts',(2.31863170299994,15.2,-11.235861771));
#159850=CARTESIAN_POINT('Ctrl Pts',(2.31863170299994,11.6,-11.235861771));
#159851=CARTESIAN_POINT('Ctrl Pts',(2.32093326799994,15.2,-11.238872729));
#159852=CARTESIAN_POINT('Ctrl Pts',(2.32093326799994,11.6,-11.238872729));
#159853=CARTESIAN_POINT('Ctrl Pts',(2.32323980899994,15.2,-11.241885437));
#159854=CARTESIAN_POINT('Ctrl Pts',(2.32323980899994,11.6,-11.241885437));
#159855=CARTESIAN_POINT('Ctrl Pts',(2.32555132399995,15.2,-11.244899887));
#159856=CARTESIAN_POINT('Ctrl Pts',(2.32555132399995,11.6,-11.244899887));
#159857=CARTESIAN_POINT('Ctrl Pts',(2.32786781499994,15.2,-11.247916073));
#159858=CARTESIAN_POINT('Ctrl Pts',(2.32786781499994,11.6,-11.247916073));
#159859=CARTESIAN_POINT('Ctrl Pts',(2.33018928299995,15.2,-11.250933991));
#159860=CARTESIAN_POINT('Ctrl Pts',(2.33018928299995,11.6,-11.250933991));
#159861=CARTESIAN_POINT('Ctrl Pts',(2.33251572399995,15.2,-11.253953638));
#159862=CARTESIAN_POINT('Ctrl Pts',(2.33251572399995,11.6,-11.253953638));
#159863=CARTESIAN_POINT('Ctrl Pts',(2.33438085799994,15.2,-11.256370739));
#159864=CARTESIAN_POINT('Ctrl Pts',(2.33438085799994,11.6,-11.256370739));
#159865=CARTESIAN_POINT('Ctrl Pts',(2.33578194799994,15.2,-11.258184341));
#159866=CARTESIAN_POINT('Ctrl Pts',(2.33578194799994,11.6,-11.258184341));
#159867=CARTESIAN_POINT('Ctrl Pts',(2.33671700199995,15.2,-11.259393754));
#159868=CARTESIAN_POINT('Ctrl Pts',(2.33671700199995,11.6,-11.259393754));
#159869=CARTESIAN_POINT('Ctrl Pts',(2.33718477799994,15.2,-11.259998548));
#159870=CARTESIAN_POINT('Ctrl Pts',(2.33718477799994,11.6,-11.259998548));
#159871=CARTESIAN_POINT('Ctrl Pts',(1.76496130699994,15.2,-10.223773109));
#159872=CARTESIAN_POINT('Ctrl Pts',(1.76500562299994,15.2,-10.223941741));
#159873=CARTESIAN_POINT('Ctrl Pts',(1.76509588899994,15.2,-10.224284873));
#159874=CARTESIAN_POINT('Ctrl Pts',(1.76523291899994,15.2,-10.224804731));
#159875=CARTESIAN_POINT('Ctrl Pts',(1.76541803299994,15.2,-10.22550489));
#159876=CARTESIAN_POINT('Ctrl Pts',(1.76565305799994,15.2,-10.226390254));
#159877=CARTESIAN_POINT('Ctrl Pts',(1.76589279499994,15.2,-10.227289727));
#159878=CARTESIAN_POINT('Ctrl Pts',(1.76613589399994,15.2,-10.228198149));
#159879=CARTESIAN_POINT('Ctrl Pts',(1.76638236599994,15.2,-10.229115492));
#159880=CARTESIAN_POINT('Ctrl Pts',(1.76663221999994,15.2,-10.230041723));
#159881=CARTESIAN_POINT('Ctrl Pts',(1.76688546699994,15.2,-10.230976812));
#159882=CARTESIAN_POINT('Ctrl Pts',(1.76714211699994,15.2,-10.231920729));
#159883=CARTESIAN_POINT('Ctrl Pts',(1.76740218099994,15.2,-10.232873443));
#159884=CARTESIAN_POINT('Ctrl Pts',(1.76766566999994,15.2,-10.233834926));
#159885=CARTESIAN_POINT('Ctrl Pts',(1.76793259299994,15.2,-10.234805146));
#159886=CARTESIAN_POINT('Ctrl Pts',(1.76820295999994,15.2,-10.235784073));
#159887=CARTESIAN_POINT('Ctrl Pts',(1.76847678199994,15.2,-10.23677168));
#159888=CARTESIAN_POINT('Ctrl Pts',(1.76875406799994,15.2,-10.237767935));
#159889=CARTESIAN_POINT('Ctrl Pts',(1.76903482799994,15.2,-10.238772809));
#159890=CARTESIAN_POINT('Ctrl Pts',(1.76931907099994,15.2,-10.239786274));
#159891=CARTESIAN_POINT('Ctrl Pts',(1.76960680899994,15.2,-10.2408083));
#159892=CARTESIAN_POINT('Ctrl Pts',(1.76989805199994,15.2,-10.241838858));
#159893=CARTESIAN_POINT('Ctrl Pts',(1.77019280699994,15.2,-10.24287792));
#159894=CARTESIAN_POINT('Ctrl Pts',(1.77049108499994,15.2,-10.243925456));
#159895=CARTESIAN_POINT('Ctrl Pts',(1.77079289599994,15.2,-10.244981439));
#159896=CARTESIAN_POINT('Ctrl Pts',(1.77109824899994,15.2,-10.246045839));
#159897=CARTESIAN_POINT('Ctrl Pts',(1.77140715299994,15.2,-10.247118629));
#159898=CARTESIAN_POINT('Ctrl Pts',(1.77171961899994,15.2,-10.248199781));
#159899=CARTESIAN_POINT('Ctrl Pts',(1.77203565399994,15.2,-10.249289267));
#159900=CARTESIAN_POINT('Ctrl Pts',(1.77235526999994,15.2,-10.250387057));
#159901=CARTESIAN_POINT('Ctrl Pts',(1.77267847299994,15.2,-10.251493125));
#159902=CARTESIAN_POINT('Ctrl Pts',(1.77300527499994,15.2,-10.252607443));
#159903=CARTESIAN_POINT('Ctrl Pts',(1.77333568299994,15.2,-10.253729984));
#159904=CARTESIAN_POINT('Ctrl Pts',(1.77366970799994,15.2,-10.25486072));
#159905=CARTESIAN_POINT('Ctrl Pts',(1.77400735799994,15.2,-10.255999624));
#159906=CARTESIAN_POINT('Ctrl Pts',(1.77434864199994,15.2,-10.257146668));
#159907=CARTESIAN_POINT('Ctrl Pts',(1.77469356799994,15.2,-10.258301827));
#159908=CARTESIAN_POINT('Ctrl Pts',(1.77504214599994,15.2,-10.259465073));
#159909=CARTESIAN_POINT('Ctrl Pts',(1.77539438599994,15.2,-10.260636378));
#159910=CARTESIAN_POINT('Ctrl Pts',(1.77575029399994,15.2,-10.261815716));
#159911=CARTESIAN_POINT('Ctrl Pts',(1.77610987999994,15.2,-10.263003061));
#159912=CARTESIAN_POINT('Ctrl Pts',(1.77647315199994,15.2,-10.264198387));
#159913=CARTESIAN_POINT('Ctrl Pts',(1.77684011999994,15.2,-10.265401666));
#159914=CARTESIAN_POINT('Ctrl Pts',(1.77721079199994,15.2,-10.266612874));
#159915=CARTESIAN_POINT('Ctrl Pts',(1.77758517499994,15.2,-10.267831982));
#159916=CARTESIAN_POINT('Ctrl Pts',(1.77796327899994,15.2,-10.269058966));
#159917=CARTESIAN_POINT('Ctrl Pts',(1.77834511299995,15.2,-10.2702938));
#159918=CARTESIAN_POINT('Ctrl Pts',(1.77873068199994,15.2,-10.271536458));
#159919=CARTESIAN_POINT('Ctrl Pts',(1.77911999799994,15.2,-10.272786914));
#159920=CARTESIAN_POINT('Ctrl Pts',(1.77951306799994,15.2,-10.274045143));
#159921=CARTESIAN_POINT('Ctrl Pts',(1.77990989999994,15.2,-10.275311119));
#159922=CARTESIAN_POINT('Ctrl Pts',(1.78031050099994,15.2,-10.276584816));
#159923=CARTESIAN_POINT('Ctrl Pts',(1.78071487999994,15.2,-10.27786621));
#159924=CARTESIAN_POINT('Ctrl Pts',(1.78112304599994,15.2,-10.279155276));
#159925=CARTESIAN_POINT('Ctrl Pts',(1.78153500599994,15.2,-10.280451988));
#159926=CARTESIAN_POINT('Ctrl Pts',(1.78195076699994,15.2,-10.281756321));
#159927=CARTESIAN_POINT('Ctrl Pts',(1.78237033899994,15.2,-10.283068252));
#159928=CARTESIAN_POINT('Ctrl Pts',(1.78279372899994,15.2,-10.284387754));
#159929=CARTESIAN_POINT('Ctrl Pts',(1.78322094399994,15.2,-10.285714803));
#159930=CARTESIAN_POINT('Ctrl Pts',(1.78365199299995,15.2,-10.287049375));
#159931=CARTESIAN_POINT('Ctrl Pts',(1.78408688299994,15.2,-10.288391446));
#159932=CARTESIAN_POINT('Ctrl Pts',(1.78452562099994,15.2,-10.28974099));
#159933=CARTESIAN_POINT('Ctrl Pts',(1.78496821499994,15.2,-10.291097983));
#159934=CARTESIAN_POINT('Ctrl Pts',(1.78541467399994,15.2,-10.292462403));
#159935=CARTESIAN_POINT('Ctrl Pts',(1.78586500399994,15.2,-10.293834224));
#159936=CARTESIAN_POINT('Ctrl Pts',(1.78631921299994,15.2,-10.295213422));
#159937=CARTESIAN_POINT('Ctrl Pts',(1.78677730899994,15.2,-10.296599975));
#159938=CARTESIAN_POINT('Ctrl Pts',(1.78723929699994,15.2,-10.297993858));
#159939=CARTESIAN_POINT('Ctrl Pts',(1.78770518699994,15.2,-10.299395046));
#159940=CARTESIAN_POINT('Ctrl Pts',(1.78817498599994,15.2,-10.300803517));
#159941=CARTESIAN_POINT('Ctrl Pts',(1.78864869999994,15.2,-10.302219248));
#159942=CARTESIAN_POINT('Ctrl Pts',(1.78912633699994,15.2,-10.303642215));
#159943=CARTESIAN_POINT('Ctrl Pts',(1.78960790399994,15.2,-10.305072393));
#159944=CARTESIAN_POINT('Ctrl Pts',(1.79009340899994,15.2,-10.306509762));
#159945=CARTESIAN_POINT('Ctrl Pts',(1.79058285799994,15.2,-10.307954296));
#159946=CARTESIAN_POINT('Ctrl Pts',(1.79107625799994,15.2,-10.309405975));
#159947=CARTESIAN_POINT('Ctrl Pts',(1.79157361699994,15.2,-10.310864772));
#159948=CARTESIAN_POINT('Ctrl Pts',(1.79207494099994,15.2,-10.312330668));
#159949=CARTESIAN_POINT('Ctrl Pts',(1.79258023699994,15.2,-10.313803638));
#159950=CARTESIAN_POINT('Ctrl Pts',(1.79308951199994,15.2,-10.315283661));
#159951=CARTESIAN_POINT('Ctrl Pts',(1.79360277399994,15.2,-10.316770712));
#159952=CARTESIAN_POINT('Ctrl Pts',(1.79412002899994,15.2,-10.318264771));
#159953=CARTESIAN_POINT('Ctrl Pts',(1.79464128299994,15.2,-10.319765813));
#159954=CARTESIAN_POINT('Ctrl Pts',(1.79516654299994,15.2,-10.321273818));
#159955=CARTESIAN_POINT('Ctrl Pts',(1.79569581699994,15.2,-10.322788763));
#159956=CARTESIAN_POINT('Ctrl Pts',(1.79622910999994,15.2,-10.324310627));
#159957=CARTESIAN_POINT('Ctrl Pts',(1.79676642999994,15.2,-10.325839385));
#159958=CARTESIAN_POINT('Ctrl Pts',(1.79730778399994,15.2,-10.327375017));
#159959=CARTESIAN_POINT('Ctrl Pts',(1.79785317499994,15.2,-10.328917501));
#159960=CARTESIAN_POINT('Ctrl Pts',(1.79840261399994,15.2,-10.330466814));
#159961=CARTESIAN_POINT('Ctrl Pts',(1.79895610399994,15.2,-10.332022936));
#159962=CARTESIAN_POINT('Ctrl Pts',(1.79951365499994,15.2,-10.333585844));
#159963=CARTESIAN_POINT('Ctrl Pts',(1.80007526999994,15.2,-10.335155517));
#159964=CARTESIAN_POINT('Ctrl Pts',(1.80064095699994,15.2,-10.336731933));
#159965=CARTESIAN_POINT('Ctrl Pts',(1.80121072099994,15.2,-10.338315071));
#159966=CARTESIAN_POINT('Ctrl Pts',(1.80178457199994,15.2,-10.33990491));
#159967=CARTESIAN_POINT('Ctrl Pts',(1.80236250999994,15.2,-10.341501427));
#159968=CARTESIAN_POINT('Ctrl Pts',(1.80294454699994,15.2,-10.343104603));
#159969=CARTESIAN_POINT('Ctrl Pts',(1.80353068699994,15.2,-10.344714415));
#159970=CARTESIAN_POINT('Ctrl Pts',(1.80412093499994,15.2,-10.346330843));
#159971=CARTESIAN_POINT('Ctrl Pts',(1.80471529899994,15.2,-10.347953866));
#159972=CARTESIAN_POINT('Ctrl Pts',(1.80531378399994,15.2,-10.349583463));
#159973=CARTESIAN_POINT('Ctrl Pts',(1.80591639699994,15.2,-10.351219612));
#159974=CARTESIAN_POINT('Ctrl Pts',(1.80652314299994,15.2,-10.352862295));
#159975=CARTESIAN_POINT('Ctrl Pts',(1.80713402799994,15.2,-10.354511488));
#159976=CARTESIAN_POINT('Ctrl Pts',(1.80774905899994,15.2,-10.356167172));
#159977=CARTESIAN_POINT('Ctrl Pts',(1.80836823999994,15.2,-10.357829328));
#159978=CARTESIAN_POINT('Ctrl Pts',(1.80899157899994,15.2,-10.359497933));
#159979=CARTESIAN_POINT('Ctrl Pts',(1.80961908099994,15.2,-10.361172966));
#159980=CARTESIAN_POINT('Ctrl Pts',(1.81025075099994,15.2,-10.36285441));
#159981=CARTESIAN_POINT('Ctrl Pts',(1.81088659599994,15.2,-10.364542242));
#159982=CARTESIAN_POINT('Ctrl Pts',(1.81152661999994,15.2,-10.366236444));
#159983=CARTESIAN_POINT('Ctrl Pts',(1.81217083099994,15.2,-10.367936993));
#159984=CARTESIAN_POINT('Ctrl Pts',(1.81281923299994,15.2,-10.369643871));
#159985=CARTESIAN_POINT('Ctrl Pts',(1.81347183299994,15.2,-10.371357057));
#159986=CARTESIAN_POINT('Ctrl Pts',(1.81412863499994,15.2,-10.373076533));
#159987=CARTESIAN_POINT('Ctrl Pts',(1.81478964499994,15.2,-10.374802277));
#159988=CARTESIAN_POINT('Ctrl Pts',(1.81545486999994,15.2,-10.37653427));
#159989=CARTESIAN_POINT('Ctrl Pts',(1.81612431399994,15.2,-10.378272492));
#159990=CARTESIAN_POINT('Ctrl Pts',(1.81679798299994,15.2,-10.380016924));
#159991=CARTESIAN_POINT('Ctrl Pts',(1.81747588199994,15.2,-10.381767545));
#159992=CARTESIAN_POINT('Ctrl Pts',(1.81815801699994,15.2,-10.383524338));
#159993=CARTESIAN_POINT('Ctrl Pts',(1.81884439299994,15.2,-10.385287281));
#159994=CARTESIAN_POINT('Ctrl Pts',(1.81953501599994,15.2,-10.387056356));
#159995=CARTESIAN_POINT('Ctrl Pts',(1.82022989099994,15.2,-10.388831543));
#159996=CARTESIAN_POINT('Ctrl Pts',(1.82092902199994,15.2,-10.390612824));
#159997=CARTESIAN_POINT('Ctrl Pts',(1.82163241599994,15.2,-10.392400178));
#159998=CARTESIAN_POINT('Ctrl Pts',(1.82234007799994,15.2,-10.394193587));
#159999=CARTESIAN_POINT('Ctrl Pts',(1.82305201199994,15.2,-10.395993031));
#160000=CARTESIAN_POINT('Ctrl Pts',(1.82376822599994,15.2,-10.397798492));
#160001=CARTESIAN_POINT('Ctrl Pts',(1.82448872099994,15.2,-10.399609952));
#160002=CARTESIAN_POINT('Ctrl Pts',(1.82521350499994,15.2,-10.401427389));
#160003=CARTESIAN_POINT('Ctrl Pts',(1.82594258299994,15.2,-10.403250787));
#160004=CARTESIAN_POINT('Ctrl Pts',(1.82667595799994,15.2,-10.405080125));
#160005=CARTESIAN_POINT('Ctrl Pts',(1.82741363699994,15.2,-10.406915387));
#160006=CARTESIAN_POINT('Ctrl Pts',(1.82815562499994,15.2,-10.408756552));
#160007=CARTESIAN_POINT('Ctrl Pts',(1.82890192699994,15.2,-10.410603603));
#160008=CARTESIAN_POINT('Ctrl Pts',(1.82965254599994,15.2,-10.41245652));
#160009=CARTESIAN_POINT('Ctrl Pts',(1.83040748999994,15.2,-10.414315286));
#160010=CARTESIAN_POINT('Ctrl Pts',(1.83116676099994,15.2,-10.416179881));
#160011=CARTESIAN_POINT('Ctrl Pts',(1.83193036499994,15.2,-10.418050288));
#160012=CARTESIAN_POINT('Ctrl Pts',(1.83269830799994,15.2,-10.419926488));
#160013=CARTESIAN_POINT('Ctrl Pts',(1.83347059199994,15.2,-10.421808463));
#160014=CARTESIAN_POINT('Ctrl Pts',(1.83424722399994,15.2,-10.423696194));
#160015=CARTESIAN_POINT('Ctrl Pts',(1.83502820899994,15.2,-10.425589665));
#160016=CARTESIAN_POINT('Ctrl Pts',(1.83581354999994,15.2,-10.427488857));
#160017=CARTESIAN_POINT('Ctrl Pts',(1.83660325299994,15.2,-10.429393751));
#160018=CARTESIAN_POINT('Ctrl Pts',(1.83739732299994,15.2,-10.431304329));
#160019=CARTESIAN_POINT('Ctrl Pts',(1.83819576299994,15.2,-10.433220574));
#160020=CARTESIAN_POINT('Ctrl Pts',(1.83899857899994,15.2,-10.435142468));
#160021=CARTESIAN_POINT('Ctrl Pts',(1.83980577599994,15.2,-10.437069993));
#160022=CARTESIAN_POINT('Ctrl Pts',(1.84061735599994,15.2,-10.439003132));
#160023=CARTESIAN_POINT('Ctrl Pts',(1.84143332699994,15.2,-10.440941867));
#160024=CARTESIAN_POINT('Ctrl Pts',(1.84225369099994,15.2,-10.442886179));
#160025=CARTESIAN_POINT('Ctrl Pts',(1.84307845299994,15.2,-10.444836053));
#160026=CARTESIAN_POINT('Ctrl Pts',(1.84390761699994,15.2,-10.446791469));
#160027=CARTESIAN_POINT('Ctrl Pts',(1.84474118899994,15.2,-10.44875241));
#160028=CARTESIAN_POINT('Ctrl Pts',(1.84557917199994,15.2,-10.45071886));
#160029=CARTESIAN_POINT('Ctrl Pts',(1.84642157199994,15.2,-10.452690801));
#160030=CARTESIAN_POINT('Ctrl Pts',(1.84726839199994,15.2,-10.454668215));
#160031=CARTESIAN_POINT('Ctrl Pts',(1.84811963599994,15.2,-10.456651085));
#160032=CARTESIAN_POINT('Ctrl Pts',(1.84897530999994,15.2,-10.458639395));
#160033=CARTESIAN_POINT('Ctrl Pts',(1.84983541599994,15.2,-10.460633126));
#160034=CARTESIAN_POINT('Ctrl Pts',(1.85069995999994,15.2,-10.462632262));
#160035=CARTESIAN_POINT('Ctrl Pts',(1.85156894599994,15.2,-10.464636786));
#160036=CARTESIAN_POINT('Ctrl Pts',(1.85244237799994,15.2,-10.46664668));
#160037=CARTESIAN_POINT('Ctrl Pts',(1.85332025899994,15.2,-10.468661929));
#160038=CARTESIAN_POINT('Ctrl Pts',(1.85420259499994,15.2,-10.470682514));
#160039=CARTESIAN_POINT('Ctrl Pts',(1.85508938999994,15.2,-10.47270842));
#160040=CARTESIAN_POINT('Ctrl Pts',(1.85598064599994,15.2,-10.474739628));
#160041=CARTESIAN_POINT('Ctrl Pts',(1.85687636999994,15.2,-10.476776123));
#160042=CARTESIAN_POINT('Ctrl Pts',(1.85777656499994,15.2,-10.478817888));
#160043=CARTESIAN_POINT('Ctrl Pts',(1.85868123399994,15.2,-10.480864906));
#160044=CARTESIAN_POINT('Ctrl Pts',(1.85959038199994,15.2,-10.48291716));
#160045=CARTESIAN_POINT('Ctrl Pts',(1.86050401199994,15.2,-10.484974634));
#160046=CARTESIAN_POINT('Ctrl Pts',(1.86142212899994,15.2,-10.487037312));
#160047=CARTESIAN_POINT('Ctrl Pts',(1.86234473699994,15.2,-10.489105177));
#160048=CARTESIAN_POINT('Ctrl Pts',(1.86327183899994,15.2,-10.491178213));
#160049=CARTESIAN_POINT('Ctrl Pts',(1.86420344099994,15.2,-10.493256403));
#160050=CARTESIAN_POINT('Ctrl Pts',(1.86513954299994,15.2,-10.49533973));
#160051=CARTESIAN_POINT('Ctrl Pts',(1.86608015299994,15.2,-10.497428179));
#160052=CARTESIAN_POINT('Ctrl Pts',(1.86702527199994,15.2,-10.499521733));
#160053=CARTESIAN_POINT('Ctrl Pts',(1.86797490499994,15.2,-10.501620377));
#160054=CARTESIAN_POINT('Ctrl Pts',(1.86892905699994,15.2,-10.503724094));
#160055=CARTESIAN_POINT('Ctrl Pts',(1.86988772999995,15.2,-10.505832868));
#160056=CARTESIAN_POINT('Ctrl Pts',(1.87085092699994,15.2,-10.507946683));
#160057=CARTESIAN_POINT('Ctrl Pts',(1.87181865399994,15.2,-10.510065522));
#160058=CARTESIAN_POINT('Ctrl Pts',(1.87279091299994,15.2,-10.512189371));
#160059=CARTESIAN_POINT('Ctrl Pts',(1.87376770899994,15.2,-10.514318212));
#160060=CARTESIAN_POINT('Ctrl Pts',(1.87474904299994,15.2,-10.516452031));
#160061=CARTESIAN_POINT('Ctrl Pts',(1.87573492299994,15.2,-10.518590811));
#160062=CARTESIAN_POINT('Ctrl Pts',(1.87672534799994,15.2,-10.520734536));
#160063=CARTESIAN_POINT('Ctrl Pts',(1.87772032499994,15.2,-10.522883192));
#160064=CARTESIAN_POINT('Ctrl Pts',(1.87871985699994,15.2,-10.525036762));
#160065=CARTESIAN_POINT('Ctrl Pts',(1.87972394599994,15.2,-10.52719523));
#160066=CARTESIAN_POINT('Ctrl Pts',(1.88073259699994,15.2,-10.529358581));
#160067=CARTESIAN_POINT('Ctrl Pts',(1.88174581199994,15.2,-10.531526798));
#160068=CARTESIAN_POINT('Ctrl Pts',(1.88276359599994,15.2,-10.533699869));
#160069=CARTESIAN_POINT('Ctrl Pts',(1.88378595299994,15.2,-10.535877775));
#160070=CARTESIAN_POINT('Ctrl Pts',(1.88481288399994,15.2,-10.538060503));
#160071=CARTESIAN_POINT('Ctrl Pts',(1.88584439399994,15.2,-10.540248035));
#160072=CARTESIAN_POINT('Ctrl Pts',(1.88688048599994,15.2,-10.542440358));
#160073=CARTESIAN_POINT('Ctrl Pts',(1.88792116399994,15.2,-10.544637455));
#160074=CARTESIAN_POINT('Ctrl Pts',(1.88896643099994,15.2,-10.546839313));
#160075=CARTESIAN_POINT('Ctrl Pts',(1.89001628999994,15.2,-10.549045913));
#160076=CARTESIAN_POINT('Ctrl Pts',(1.89107074499994,15.2,-10.551257244));
#160077=CARTESIAN_POINT('Ctrl Pts',(1.89212979899994,15.2,-10.553473288));
#160078=CARTESIAN_POINT('Ctrl Pts',(1.89319345499994,15.2,-10.555694032));
#160079=CARTESIAN_POINT('Ctrl Pts',(1.89426171599994,15.2,-10.557919458));
#160080=CARTESIAN_POINT('Ctrl Pts',(1.89533458699994,15.2,-10.560149554));
#160081=CARTESIAN_POINT('Ctrl Pts',(1.89641206899994,15.2,-10.562384303));
#160082=CARTESIAN_POINT('Ctrl Pts',(1.89749416599994,15.2,-10.564623691));
#160083=CARTESIAN_POINT('Ctrl Pts',(1.89858088099994,15.2,-10.566867703));
#160084=CARTESIAN_POINT('Ctrl Pts',(1.89967221899994,15.2,-10.569116324));
#160085=CARTESIAN_POINT('Ctrl Pts',(1.90076818099994,15.2,-10.571369539));
#160086=CARTESIAN_POINT('Ctrl Pts',(1.90186877099994,15.2,-10.573627333));
#160087=CARTESIAN_POINT('Ctrl Pts',(1.90297399099994,15.2,-10.575889692));
#160088=CARTESIAN_POINT('Ctrl Pts',(1.90408384599994,15.2,-10.578156601));
#160089=CARTESIAN_POINT('Ctrl Pts',(1.90519833799994,15.2,-10.580428044));
#160090=CARTESIAN_POINT('Ctrl Pts',(1.90631746999994,15.2,-10.582704009));
#160091=CARTESIAN_POINT('Ctrl Pts',(1.90744124499994,15.2,-10.584984479));
#160092=CARTESIAN_POINT('Ctrl Pts',(1.90856966599994,15.2,-10.587269441));
#160093=CARTESIAN_POINT('Ctrl Pts',(1.90970273699994,15.2,-10.58955888));
#160094=CARTESIAN_POINT('Ctrl Pts',(1.91084045999994,15.2,-10.59185278));
#160095=CARTESIAN_POINT('Ctrl Pts',(1.91198283799994,15.2,-10.594151129));
#160096=CARTESIAN_POINT('Ctrl Pts',(1.91312987399994,15.2,-10.59645391));
#160097=CARTESIAN_POINT('Ctrl Pts',(1.91428157099994,15.2,-10.598761112));
#160098=CARTESIAN_POINT('Ctrl Pts',(1.91543793199994,15.2,-10.601072717));
#160099=CARTESIAN_POINT('Ctrl Pts',(1.91659895999994,15.2,-10.603388714));
#160100=CARTESIAN_POINT('Ctrl Pts',(1.91776465699994,15.2,-10.605709085));
#160101=CARTESIAN_POINT('Ctrl Pts',(1.91893502699994,15.2,-10.60803382));
#160102=CARTESIAN_POINT('Ctrl Pts',(1.92011007299994,15.2,-10.610362901));
#160103=CARTESIAN_POINT('Ctrl Pts',(1.92128979599994,15.2,-10.612696316));
#160104=CARTESIAN_POINT('Ctrl Pts',(1.92247420099994,15.2,-10.615034051));
#160105=CARTESIAN_POINT('Ctrl Pts',(1.92366328999994,15.2,-10.617376091));
#160106=CARTESIAN_POINT('Ctrl Pts',(1.92485706499994,15.2,-10.619722422));
#160107=CARTESIAN_POINT('Ctrl Pts',(1.92605552899994,15.2,-10.622073029));
#160108=CARTESIAN_POINT('Ctrl Pts',(1.92725868499994,15.2,-10.6244279));
#160109=CARTESIAN_POINT('Ctrl Pts',(1.92846653599994,15.2,-10.62678702));
#160110=CARTESIAN_POINT('Ctrl Pts',(1.92967908399994,15.2,-10.629150376));
#160111=CARTESIAN_POINT('Ctrl Pts',(1.93089633299994,15.2,-10.631517953));
#160112=CARTESIAN_POINT('Ctrl Pts',(1.93211828499994,15.2,-10.633889738));
#160113=CARTESIAN_POINT('Ctrl Pts',(1.93334494199994,15.2,-10.636265715));
#160114=CARTESIAN_POINT('Ctrl Pts',(1.93457630699994,15.2,-10.638645874));
#160115=CARTESIAN_POINT('Ctrl Pts',(1.93581238299994,15.2,-10.641030197));
#160116=CARTESIAN_POINT('Ctrl Pts',(1.93705317299994,15.2,-10.643418674));
#160117=CARTESIAN_POINT('Ctrl Pts',(1.93829867699994,15.2,-10.645811289));
#160118=CARTESIAN_POINT('Ctrl Pts',(1.93954889999994,15.2,-10.648208029));
#160119=CARTESIAN_POINT('Ctrl Pts',(1.94080384499994,15.2,-10.650608881));
#160120=CARTESIAN_POINT('Ctrl Pts',(1.94206351299994,15.2,-10.65301383));
#160121=CARTESIAN_POINT('Ctrl Pts',(1.94332790699994,15.2,-10.655422864));
#160122=CARTESIAN_POINT('Ctrl Pts',(1.94459702899994,15.2,-10.657835968));
#160123=CARTESIAN_POINT('Ctrl Pts',(1.94587088199994,15.2,-10.660253129));
#160124=CARTESIAN_POINT('Ctrl Pts',(1.94714946899994,15.2,-10.662674334));
#160125=CARTESIAN_POINT('Ctrl Pts',(1.94843279199994,15.2,-10.665099571));
#160126=CARTESIAN_POINT('Ctrl Pts',(1.94972085299994,15.2,-10.667528823));
#160127=CARTESIAN_POINT('Ctrl Pts',(1.95101365499994,15.2,-10.66996208));
#160128=CARTESIAN_POINT('Ctrl Pts',(1.95231119999994,15.2,-10.672399326));
#160129=CARTESIAN_POINT('Ctrl Pts',(1.95361349099994,15.2,-10.674840549));
#160130=CARTESIAN_POINT('Ctrl Pts',(1.95492052999994,15.2,-10.677285737));
#160131=CARTESIAN_POINT('Ctrl Pts',(1.95623231799994,15.2,-10.679734874));
#160132=CARTESIAN_POINT('Ctrl Pts',(1.95754885999994,15.2,-10.682187948));
#160133=CARTESIAN_POINT('Ctrl Pts',(1.95887015699994,15.2,-10.684644947));
#160134=CARTESIAN_POINT('Ctrl Pts',(1.96019620999994,15.2,-10.687105856));
#160135=CARTESIAN_POINT('Ctrl Pts',(1.96152702299994,15.2,-10.689570664));
#160136=CARTESIAN_POINT('Ctrl Pts',(1.96286259899994,15.2,-10.692039356));
#160137=CARTESIAN_POINT('Ctrl Pts',(1.96420293799994,15.2,-10.694511919));
#160138=CARTESIAN_POINT('Ctrl Pts',(1.96554804399994,15.2,-10.696988341));
#160139=CARTESIAN_POINT('Ctrl Pts',(1.96689791799994,15.2,-10.699468609));
#160140=CARTESIAN_POINT('Ctrl Pts',(1.96825256199994,15.2,-10.70195271));
#160141=CARTESIAN_POINT('Ctrl Pts',(1.96961197999994,15.2,-10.704440629));
#160142=CARTESIAN_POINT('Ctrl Pts',(1.97097617299994,15.2,-10.706932355));
#160143=CARTESIAN_POINT('Ctrl Pts',(1.97234514399994,15.2,-10.709427876));
#160144=CARTESIAN_POINT('Ctrl Pts',(1.97371889299994,15.2,-10.711927177));
#160145=CARTESIAN_POINT('Ctrl Pts',(1.97509742499994,15.2,-10.714430247));
#160146=CARTESIAN_POINT('Ctrl Pts',(1.97648073999994,15.2,-10.716937073));
#160147=CARTESIAN_POINT('Ctrl Pts',(1.97786884099994,15.2,-10.71944764));
#160148=CARTESIAN_POINT('Ctrl Pts',(1.97926172999994,15.2,-10.721961937));
#160149=CARTESIAN_POINT('Ctrl Pts',(1.98065940899994,15.2,-10.724479952));
#160150=CARTESIAN_POINT('Ctrl Pts',(1.98206188099994,15.2,-10.727001672));
#160151=CARTESIAN_POINT('Ctrl Pts',(1.98346914499994,15.2,-10.729527083));
#160152=CARTESIAN_POINT('Ctrl Pts',(1.98488120699994,15.2,-10.732056173));
#160153=CARTESIAN_POINT('Ctrl Pts',(1.98629806699994,15.2,-10.73458893));
#160154=CARTESIAN_POINT('Ctrl Pts',(1.98771972699994,15.2,-10.737125341));
#160155=CARTESIAN_POINT('Ctrl Pts',(1.98914618999994,15.2,-10.739665394));
#160156=CARTESIAN_POINT('Ctrl Pts',(1.99057745699994,15.2,-10.742209076));
#160157=CARTESIAN_POINT('Ctrl Pts',(1.99201352899994,15.2,-10.744756374));
#160158=CARTESIAN_POINT('Ctrl Pts',(1.99345441099994,15.2,-10.747307276));
#160159=CARTESIAN_POINT('Ctrl Pts',(1.99490010199994,15.2,-10.74986177));
#160160=CARTESIAN_POINT('Ctrl Pts',(1.99635060499994,15.2,-10.752419844));
#160161=CARTESIAN_POINT('Ctrl Pts',(1.99780592199994,15.2,-10.754981484));
#160162=CARTESIAN_POINT('Ctrl Pts',(1.99926605499994,15.2,-10.757546678));
#160163=CARTESIAN_POINT('Ctrl Pts',(2.00073100599994,15.2,-10.760115415));
#160164=CARTESIAN_POINT('Ctrl Pts',(2.00220077599994,15.2,-10.762687682));
#160165=CARTESIAN_POINT('Ctrl Pts',(2.00367536799994,15.2,-10.765263466));
#160166=CARTESIAN_POINT('Ctrl Pts',(2.00515478199994,15.2,-10.767842756));
#160167=CARTESIAN_POINT('Ctrl Pts',(2.00663902299994,15.2,-10.77042554));
#160168=CARTESIAN_POINT('Ctrl Pts',(2.00812808999994,15.2,-10.773011803));
#160169=CARTESIAN_POINT('Ctrl Pts',(2.00962198599994,15.2,-10.775601537));
#160170=CARTESIAN_POINT('Ctrl Pts',(2.01112071299994,15.2,-10.778194727));
#160171=CARTESIAN_POINT('Ctrl Pts',(2.01262427099994,15.2,-10.780791361));
#160172=CARTESIAN_POINT('Ctrl Pts',(2.01413266399994,15.2,-10.783391428));
#160173=CARTESIAN_POINT('Ctrl Pts',(2.01564589299994,15.2,-10.785994916));
#160174=CARTESIAN_POINT('Ctrl Pts',(2.01716395899994,15.2,-10.788601812));
#160175=CARTESIAN_POINT('Ctrl Pts',(2.01868686499994,15.2,-10.791212104));
#160176=CARTESIAN_POINT('Ctrl Pts',(2.02021461099994,15.2,-10.793825781));
#160177=CARTESIAN_POINT('Ctrl Pts',(2.02174720099995,15.2,-10.796442831));
#160178=CARTESIAN_POINT('Ctrl Pts',(2.02328463399994,15.2,-10.799063241));
#160179=CARTESIAN_POINT('Ctrl Pts',(2.02482691399994,15.2,-10.801687));
#160180=CARTESIAN_POINT('Ctrl Pts',(2.02637404199994,15.2,-10.804314097));
#160181=CARTESIAN_POINT('Ctrl Pts',(2.02792601899994,15.2,-10.806944517));
#160182=CARTESIAN_POINT('Ctrl Pts',(2.02948284599994,15.2,-10.809578251));
#160183=CARTESIAN_POINT('Ctrl Pts',(2.03104452699994,15.2,-10.812215287));
#160184=CARTESIAN_POINT('Ctrl Pts',(2.03261106199994,15.2,-10.814855611));
#160185=CARTESIAN_POINT('Ctrl Pts',(2.03418245199994,15.2,-10.817499214));
#160186=CARTESIAN_POINT('Ctrl Pts',(2.03575870099994,15.2,-10.820146083));
#160187=CARTESIAN_POINT('Ctrl Pts',(2.03733980799994,15.2,-10.822796206));
#160188=CARTESIAN_POINT('Ctrl Pts',(2.03892577499994,15.2,-10.825449572));
#160189=CARTESIAN_POINT('Ctrl Pts',(2.04051660599994,15.2,-10.82810617));
#160190=CARTESIAN_POINT('Ctrl Pts',(2.04211229899994,15.2,-10.830765986));
#160191=CARTESIAN_POINT('Ctrl Pts',(2.04371285699994,15.2,-10.833429011));
#160192=CARTESIAN_POINT('Ctrl Pts',(2.04531828199995,15.2,-10.836095232));
#160193=CARTESIAN_POINT('Ctrl Pts',(2.04692857599994,15.2,-10.838764637));
#160194=CARTESIAN_POINT('Ctrl Pts',(2.04854373899995,15.2,-10.841437216));
#160195=CARTESIAN_POINT('Ctrl Pts',(2.05016377299994,15.2,-10.844112955));
#160196=CARTESIAN_POINT('Ctrl Pts',(2.05178868099994,15.2,-10.846791846));
#160197=CARTESIAN_POINT('Ctrl Pts',(2.05341846199994,15.2,-10.849473875));
#160198=CARTESIAN_POINT('Ctrl Pts',(2.05505311799994,15.2,-10.852159032));
#160199=CARTESIAN_POINT('Ctrl Pts',(2.05669265099994,15.2,-10.854847303));
#160200=CARTESIAN_POINT('Ctrl Pts',(2.05833706199994,15.2,-10.85753868));
#160201=CARTESIAN_POINT('Ctrl Pts',(2.05998635399994,15.2,-10.86023315));
#160202=CARTESIAN_POINT('Ctrl Pts',(2.06164052499994,15.2,-10.862930702));
#160203=CARTESIAN_POINT('Ctrl Pts',(2.06329958099994,15.2,-10.865631323));
#160204=CARTESIAN_POINT('Ctrl Pts',(2.06496351899994,15.2,-10.868335004));
#160205=CARTESIAN_POINT('Ctrl Pts',(2.06663234299994,15.2,-10.871041734));
#160206=CARTESIAN_POINT('Ctrl Pts',(2.06830605399994,15.2,-10.873751499));
#160207=CARTESIAN_POINT('Ctrl Pts',(2.06998465199994,15.2,-10.876464289));
#160208=CARTESIAN_POINT('Ctrl Pts',(2.07166813899994,15.2,-10.879180094));
#160209=CARTESIAN_POINT('Ctrl Pts',(2.07335651799994,15.2,-10.881898902));
#160210=CARTESIAN_POINT('Ctrl Pts',(2.07504978799994,15.2,-10.884620701));
#160211=CARTESIAN_POINT('Ctrl Pts',(2.07674794999994,15.2,-10.887345482));
#160212=CARTESIAN_POINT('Ctrl Pts',(2.07845100699994,15.2,-10.890073231));
#160213=CARTESIAN_POINT('Ctrl Pts',(2.08015896099994,15.2,-10.89280394));
#160214=CARTESIAN_POINT('Ctrl Pts',(2.08187181099994,15.2,-10.895537595));
#160215=CARTESIAN_POINT('Ctrl Pts',(2.08358955799994,15.2,-10.898274186));
#160216=CARTESIAN_POINT('Ctrl Pts',(2.08531220499994,15.2,-10.901013703));
#160217=CARTESIAN_POINT('Ctrl Pts',(2.08703975299994,15.2,-10.903756135));
#160218=CARTESIAN_POINT('Ctrl Pts',(2.08877220299994,15.2,-10.906501469));
#160219=CARTESIAN_POINT('Ctrl Pts',(2.09050955499994,15.2,-10.909249695));
#160220=CARTESIAN_POINT('Ctrl Pts',(2.09225181099994,15.2,-10.912000804));
#160221=CARTESIAN_POINT('Ctrl Pts',(2.09399897299994,15.2,-10.914754782));
#160222=CARTESIAN_POINT('Ctrl Pts',(2.09575104199994,15.2,-10.91751162));
#160223=CARTESIAN_POINT('Ctrl Pts',(2.09750801799994,15.2,-10.920271306));
#160224=CARTESIAN_POINT('Ctrl Pts',(2.09926990199994,15.2,-10.92303383));
#160225=CARTESIAN_POINT('Ctrl Pts',(2.10103669699994,15.2,-10.925799182));
#160226=CARTESIAN_POINT('Ctrl Pts',(2.10280840299994,15.2,-10.928567349));
#160227=CARTESIAN_POINT('Ctrl Pts',(2.10458501999994,15.2,-10.931338321));
#160228=CARTESIAN_POINT('Ctrl Pts',(2.10636655199994,15.2,-10.934112088));
#160229=CARTESIAN_POINT('Ctrl Pts',(2.10815299699994,15.2,-10.936888638));
#160230=CARTESIAN_POINT('Ctrl Pts',(2.10994435799994,15.2,-10.939667962));
#160231=CARTESIAN_POINT('Ctrl Pts',(2.11174063499994,15.2,-10.942450048));
#160232=CARTESIAN_POINT('Ctrl Pts',(2.11354182899994,15.2,-10.945234885));
#160233=CARTESIAN_POINT('Ctrl Pts',(2.11534794299994,15.2,-10.948022463));
#160234=CARTESIAN_POINT('Ctrl Pts',(2.11715897499994,15.2,-10.950812772));
#160235=CARTESIAN_POINT('Ctrl Pts',(2.11897492799995,15.2,-10.953605801));
#160236=CARTESIAN_POINT('Ctrl Pts',(2.12079580299994,15.2,-10.956401537));
#160237=CARTESIAN_POINT('Ctrl Pts',(2.12262159999994,15.2,-10.959199973));
#160238=CARTESIAN_POINT('Ctrl Pts',(2.12445232199994,15.2,-10.962001096));
#160239=CARTESIAN_POINT('Ctrl Pts',(2.12628796699994,15.2,-10.964804897));
#160240=CARTESIAN_POINT('Ctrl Pts',(2.12812853899994,15.2,-10.967611364));
#160241=CARTESIAN_POINT('Ctrl Pts',(2.12997403599994,15.2,-10.970420488));
#160242=CARTESIAN_POINT('Ctrl Pts',(2.13182446099994,15.2,-10.973232257));
#160243=CARTESIAN_POINT('Ctrl Pts',(2.13367981499994,15.2,-10.976046662));
#160244=CARTESIAN_POINT('Ctrl Pts',(2.13554009799994,15.2,-10.978863691));
#160245=CARTESIAN_POINT('Ctrl Pts',(2.13740531099994,15.2,-10.981683335));
#160246=CARTESIAN_POINT('Ctrl Pts',(2.13927545499994,15.2,-10.984505583));
#160247=CARTESIAN_POINT('Ctrl Pts',(2.14115053099994,15.2,-10.987330423));
#160248=CARTESIAN_POINT('Ctrl Pts',(2.14303053999994,15.2,-10.990157848));
#160249=CARTESIAN_POINT('Ctrl Pts',(2.14491548299994,15.2,-10.992987845));
#160250=CARTESIAN_POINT('Ctrl Pts',(2.14680536099995,15.2,-10.995820404));
#160251=CARTESIAN_POINT('Ctrl Pts',(2.14870017399994,15.2,-10.998655516));
#160252=CARTESIAN_POINT('Ctrl Pts',(2.15059992399994,15.2,-11.00149317));
#160253=CARTESIAN_POINT('Ctrl Pts',(2.15250460999994,15.2,-11.004333355));
#160254=CARTESIAN_POINT('Ctrl Pts',(2.15441423499994,15.2,-11.007176061));
#160255=CARTESIAN_POINT('Ctrl Pts',(2.15632879899994,15.2,-11.010021278));
#160256=CARTESIAN_POINT('Ctrl Pts',(2.15824830199994,15.2,-11.012868997));
#160257=CARTESIAN_POINT('Ctrl Pts',(2.16017274599994,15.2,-11.015719205));
#160258=CARTESIAN_POINT('Ctrl Pts',(2.16210213199994,15.2,-11.018571894));
#160259=CARTESIAN_POINT('Ctrl Pts',(2.16403645899994,15.2,-11.021427054));
#160260=CARTESIAN_POINT('Ctrl Pts',(2.16597572899994,15.2,-11.024284674));
#160261=CARTESIAN_POINT('Ctrl Pts',(2.16791994199994,15.2,-11.027144743));
#160262=CARTESIAN_POINT('Ctrl Pts',(2.16986909999994,15.2,-11.030007252));
#160263=CARTESIAN_POINT('Ctrl Pts',(2.17182320399994,15.2,-11.032872191));
#160264=CARTESIAN_POINT('Ctrl Pts',(2.17378225199994,15.2,-11.03573955));
#160265=CARTESIAN_POINT('Ctrl Pts',(2.17574624699994,15.2,-11.038609318));
#160266=CARTESIAN_POINT('Ctrl Pts',(2.17771518999994,15.2,-11.041481486));
#160267=CARTESIAN_POINT('Ctrl Pts',(2.17968908099994,15.2,-11.044356044));
#160268=CARTESIAN_POINT('Ctrl Pts',(2.18166791999994,15.2,-11.047232981));
#160269=CARTESIAN_POINT('Ctrl Pts',(2.18365170899994,15.2,-11.050112287));
#160270=CARTESIAN_POINT('Ctrl Pts',(2.18564044699994,15.2,-11.052993953));
#160271=CARTESIAN_POINT('Ctrl Pts',(2.18763413599994,15.2,-11.055877969));
#160272=CARTESIAN_POINT('Ctrl Pts',(2.18963277699994,15.2,-11.058764325));
#160273=CARTESIAN_POINT('Ctrl Pts',(2.19163636999994,15.2,-11.06165301));
#160274=CARTESIAN_POINT('Ctrl Pts',(2.19364491499995,15.2,-11.064544015));
#160275=CARTESIAN_POINT('Ctrl Pts',(2.19565841299994,15.2,-11.067437331));
#160276=CARTESIAN_POINT('Ctrl Pts',(2.19767686499994,15.2,-11.070332945));
#160277=CARTESIAN_POINT('Ctrl Pts',(2.19970027199994,15.2,-11.073230851));
#160278=CARTESIAN_POINT('Ctrl Pts',(2.20172863299994,15.2,-11.076131037));
#160279=CARTESIAN_POINT('Ctrl Pts',(2.20376195099994,15.2,-11.079033493));
#160280=CARTESIAN_POINT('Ctrl Pts',(2.20580022499994,15.2,-11.081938212));
#160281=CARTESIAN_POINT('Ctrl Pts',(2.20784345599994,15.2,-11.08484518));
#160282=CARTESIAN_POINT('Ctrl Pts',(2.20989164299994,15.2,-11.08775439));
#160283=CARTESIAN_POINT('Ctrl Pts',(2.21194478899994,15.2,-11.090665832));
#160284=CARTESIAN_POINT('Ctrl Pts',(2.21400289399994,15.2,-11.093579495));
#160285=CARTESIAN_POINT('Ctrl Pts',(2.21606595699994,15.2,-11.096495371));
#160286=CARTESIAN_POINT('Ctrl Pts',(2.21813398099994,15.2,-11.099413448));
#160287=CARTESIAN_POINT('Ctrl Pts',(2.22020696299994,15.2,-11.10233372));
#160288=CARTESIAN_POINT('Ctrl Pts',(2.22228490799994,15.2,-11.105256173));
#160289=CARTESIAN_POINT('Ctrl Pts',(2.22436781299994,15.2,-11.1081808));
#160290=CARTESIAN_POINT('Ctrl Pts',(2.22645567899994,15.2,-11.111107592));
#160291=CARTESIAN_POINT('Ctrl Pts',(2.22854850699994,15.2,-11.114036538));
#160292=CARTESIAN_POINT('Ctrl Pts',(2.23064629799994,15.2,-11.116967627));
#160293=CARTESIAN_POINT('Ctrl Pts',(2.23274905199994,15.2,-11.119900853));
#160294=CARTESIAN_POINT('Ctrl Pts',(2.23485676999994,15.2,-11.122836204));
#160295=CARTESIAN_POINT('Ctrl Pts',(2.23696945199995,15.2,-11.125773671));
#160296=CARTESIAN_POINT('Ctrl Pts',(2.23908709799994,15.2,-11.128713243));
#160297=CARTESIAN_POINT('Ctrl Pts',(2.24120970899994,15.2,-11.131654914));
#160298=CARTESIAN_POINT('Ctrl Pts',(2.24333728499994,15.2,-11.134598671));
#160299=CARTESIAN_POINT('Ctrl Pts',(2.24546982699994,15.2,-11.137544507));
#160300=CARTESIAN_POINT('Ctrl Pts',(2.24760733499994,15.2,-11.140492411));
#160301=CARTESIAN_POINT('Ctrl Pts',(2.24974980999994,15.2,-11.143442374));
#160302=CARTESIAN_POINT('Ctrl Pts',(2.25189725099994,15.2,-11.146394387));
#160303=CARTESIAN_POINT('Ctrl Pts',(2.25404965899994,15.2,-11.14934844));
#160304=CARTESIAN_POINT('Ctrl Pts',(2.25620703599994,15.2,-11.152304524));
#160305=CARTESIAN_POINT('Ctrl Pts',(2.25836937999994,15.2,-11.15526263));
#160306=CARTESIAN_POINT('Ctrl Pts',(2.26053669299994,15.2,-11.158222747));
#160307=CARTESIAN_POINT('Ctrl Pts',(2.26270897299994,15.2,-11.161184868));
#160308=CARTESIAN_POINT('Ctrl Pts',(2.26488622499994,15.2,-11.164148983));
#160309=CARTESIAN_POINT('Ctrl Pts',(2.26706844499994,15.2,-11.16711508));
#160310=CARTESIAN_POINT('Ctrl Pts',(2.26925563399994,15.2,-11.170083153));
#160311=CARTESIAN_POINT('Ctrl Pts',(2.27144779299994,15.2,-11.173053191));
#160312=CARTESIAN_POINT('Ctrl Pts',(2.27364492299994,15.2,-11.176025185));
#160313=CARTESIAN_POINT('Ctrl Pts',(2.27584702399994,15.2,-11.178999126));
#160314=CARTESIAN_POINT('Ctrl Pts',(2.27805409499994,15.2,-11.181975005));
#160315=CARTESIAN_POINT('Ctrl Pts',(2.28026613799994,15.2,-11.184952813));
#160316=CARTESIAN_POINT('Ctrl Pts',(2.28248315299994,15.2,-11.187932541));
#160317=CARTESIAN_POINT('Ctrl Pts',(2.28470513799994,15.2,-11.190914179));
#160318=CARTESIAN_POINT('Ctrl Pts',(2.28693209699994,15.2,-11.193897718));
#160319=CARTESIAN_POINT('Ctrl Pts',(2.28916402699994,15.2,-11.19688315));
#160320=CARTESIAN_POINT('Ctrl Pts',(2.29140092999994,15.2,-11.199870463));
#160321=CARTESIAN_POINT('Ctrl Pts',(2.29364280599994,15.2,-11.202859649));
#160322=CARTESIAN_POINT('Ctrl Pts',(2.29588965499994,15.2,-11.205850698));
#160323=CARTESIAN_POINT('Ctrl Pts',(2.29814147699994,15.2,-11.208843602));
#160324=CARTESIAN_POINT('Ctrl Pts',(2.30039827299994,15.2,-11.211838352));
#160325=CARTESIAN_POINT('Ctrl Pts',(2.30266004099994,15.2,-11.214834939));
#160326=CARTESIAN_POINT('Ctrl Pts',(2.30492678499994,15.2,-11.217833355));
#160327=CARTESIAN_POINT('Ctrl Pts',(2.30719850199994,15.2,-11.220833593));
#160328=CARTESIAN_POINT('Ctrl Pts',(2.30947519299994,15.2,-11.223835644));
#160329=CARTESIAN_POINT('Ctrl Pts',(2.31175685799994,15.2,-11.226839497));
#160330=CARTESIAN_POINT('Ctrl Pts',(2.31404349799994,15.2,-11.229845144));
#160331=CARTESIAN_POINT('Ctrl Pts',(2.31633511299994,15.2,-11.232852572));
#160332=CARTESIAN_POINT('Ctrl Pts',(2.31863170299994,15.2,-11.235861771));
#160333=CARTESIAN_POINT('Ctrl Pts',(2.32093326799994,15.2,-11.238872729));
#160334=CARTESIAN_POINT('Ctrl Pts',(2.32323980899994,15.2,-11.241885437));
#160335=CARTESIAN_POINT('Ctrl Pts',(2.32555132399995,15.2,-11.244899887));
#160336=CARTESIAN_POINT('Ctrl Pts',(2.32786781499994,15.2,-11.247916073));
#160337=CARTESIAN_POINT('Ctrl Pts',(2.33018928299995,15.2,-11.250933991));
#160338=CARTESIAN_POINT('Ctrl Pts',(2.33251572399995,15.2,-11.253953638));
#160339=CARTESIAN_POINT('Ctrl Pts',(2.33438085799994,15.2,-11.256370739));
#160340=CARTESIAN_POINT('Ctrl Pts',(2.33578194799994,15.2,-11.258184341));
#160341=CARTESIAN_POINT('Ctrl Pts',(2.33671700199995,15.2,-11.259393754));
#160342=CARTESIAN_POINT('Ctrl Pts',(2.33718477799994,15.2,-11.259998548));
#160343=CARTESIAN_POINT('Ctrl Pts',(1.76496130699994,12.2,-10.223773109));
#160344=CARTESIAN_POINT('Ctrl Pts',(1.76500562299994,12.2,-10.223941741));
#160345=CARTESIAN_POINT('Ctrl Pts',(1.76509588899994,12.2,-10.224284873));
#160346=CARTESIAN_POINT('Ctrl Pts',(1.76523291899994,12.2,-10.224804731));
#160347=CARTESIAN_POINT('Ctrl Pts',(1.76541803299994,12.2,-10.22550489));
#160348=CARTESIAN_POINT('Ctrl Pts',(1.76565305799994,12.2,-10.226390254));
#160349=CARTESIAN_POINT('Ctrl Pts',(1.76589279499994,12.2,-10.227289727));
#160350=CARTESIAN_POINT('Ctrl Pts',(1.76613589399994,12.2,-10.228198149));
#160351=CARTESIAN_POINT('Ctrl Pts',(1.76638236599994,12.2,-10.229115492));
#160352=CARTESIAN_POINT('Ctrl Pts',(1.76663221999994,12.2,-10.230041723));
#160353=CARTESIAN_POINT('Ctrl Pts',(1.76688546699994,12.2,-10.230976812));
#160354=CARTESIAN_POINT('Ctrl Pts',(1.76714211699994,12.2,-10.231920729));
#160355=CARTESIAN_POINT('Ctrl Pts',(1.76740218099994,12.2,-10.232873443));
#160356=CARTESIAN_POINT('Ctrl Pts',(1.76766566999994,12.2,-10.233834926));
#160357=CARTESIAN_POINT('Ctrl Pts',(1.76793259299994,12.2,-10.234805146));
#160358=CARTESIAN_POINT('Ctrl Pts',(1.76820295999994,12.2,-10.235784073));
#160359=CARTESIAN_POINT('Ctrl Pts',(1.76847678199994,12.2,-10.23677168));
#160360=CARTESIAN_POINT('Ctrl Pts',(1.76875406799994,12.2,-10.237767935));
#160361=CARTESIAN_POINT('Ctrl Pts',(1.76903482799994,12.2,-10.238772809));
#160362=CARTESIAN_POINT('Ctrl Pts',(1.76931907099994,12.2,-10.239786274));
#160363=CARTESIAN_POINT('Ctrl Pts',(1.76960680899994,12.2,-10.2408083));
#160364=CARTESIAN_POINT('Ctrl Pts',(1.76989805199994,12.2,-10.241838858));
#160365=CARTESIAN_POINT('Ctrl Pts',(1.77019280699994,12.2,-10.24287792));
#160366=CARTESIAN_POINT('Ctrl Pts',(1.77049108499994,12.2,-10.243925456));
#160367=CARTESIAN_POINT('Ctrl Pts',(1.77079289599994,12.2,-10.244981439));
#160368=CARTESIAN_POINT('Ctrl Pts',(1.77109824899994,12.2,-10.246045839));
#160369=CARTESIAN_POINT('Ctrl Pts',(1.77140715299994,12.2,-10.247118629));
#160370=CARTESIAN_POINT('Ctrl Pts',(1.77171961899994,12.2,-10.248199781));
#160371=CARTESIAN_POINT('Ctrl Pts',(1.77203565399994,12.2,-10.249289267));
#160372=CARTESIAN_POINT('Ctrl Pts',(1.77235526999994,12.2,-10.250387057));
#160373=CARTESIAN_POINT('Ctrl Pts',(1.77267847299994,12.2,-10.251493125));
#160374=CARTESIAN_POINT('Ctrl Pts',(1.77300527499994,12.2,-10.252607443));
#160375=CARTESIAN_POINT('Ctrl Pts',(1.77333568299994,12.2,-10.253729984));
#160376=CARTESIAN_POINT('Ctrl Pts',(1.77366970799994,12.2,-10.25486072));
#160377=CARTESIAN_POINT('Ctrl Pts',(1.77400735799994,12.2,-10.255999624));
#160378=CARTESIAN_POINT('Ctrl Pts',(1.77434864199994,12.2,-10.257146668));
#160379=CARTESIAN_POINT('Ctrl Pts',(1.77469356799994,12.2,-10.258301827));
#160380=CARTESIAN_POINT('Ctrl Pts',(1.77504214599994,12.2,-10.259465073));
#160381=CARTESIAN_POINT('Ctrl Pts',(1.77539438599994,12.2,-10.260636378));
#160382=CARTESIAN_POINT('Ctrl Pts',(1.77575029399994,12.2,-10.261815716));
#160383=CARTESIAN_POINT('Ctrl Pts',(1.77610987999994,12.2,-10.263003061));
#160384=CARTESIAN_POINT('Ctrl Pts',(1.77647315199994,12.2,-10.264198387));
#160385=CARTESIAN_POINT('Ctrl Pts',(1.77684011999994,12.2,-10.265401666));
#160386=CARTESIAN_POINT('Ctrl Pts',(1.77721079199994,12.2,-10.266612874));
#160387=CARTESIAN_POINT('Ctrl Pts',(1.77758517499994,12.2,-10.267831982));
#160388=CARTESIAN_POINT('Ctrl Pts',(1.77796327899994,12.2,-10.269058966));
#160389=CARTESIAN_POINT('Ctrl Pts',(1.77834511299995,12.2,-10.2702938));
#160390=CARTESIAN_POINT('Ctrl Pts',(1.77873068199994,12.2,-10.271536458));
#160391=CARTESIAN_POINT('Ctrl Pts',(1.77911999799994,12.2,-10.272786914));
#160392=CARTESIAN_POINT('Ctrl Pts',(1.77951306799994,12.2,-10.274045143));
#160393=CARTESIAN_POINT('Ctrl Pts',(1.77990989999994,12.2,-10.275311119));
#160394=CARTESIAN_POINT('Ctrl Pts',(1.78031050099994,12.2,-10.276584816));
#160395=CARTESIAN_POINT('Ctrl Pts',(1.78071487999994,12.2,-10.27786621));
#160396=CARTESIAN_POINT('Ctrl Pts',(1.78112304599994,12.2,-10.279155276));
#160397=CARTESIAN_POINT('Ctrl Pts',(1.78153500599994,12.2,-10.280451988));
#160398=CARTESIAN_POINT('Ctrl Pts',(1.78195076699994,12.2,-10.281756321));
#160399=CARTESIAN_POINT('Ctrl Pts',(1.78237033899994,12.2,-10.283068252));
#160400=CARTESIAN_POINT('Ctrl Pts',(1.78279372899994,12.2,-10.284387754));
#160401=CARTESIAN_POINT('Ctrl Pts',(1.78322094399994,12.2,-10.285714803));
#160402=CARTESIAN_POINT('Ctrl Pts',(1.78365199299995,12.2,-10.287049375));
#160403=CARTESIAN_POINT('Ctrl Pts',(1.78408688299994,12.2,-10.288391446));
#160404=CARTESIAN_POINT('Ctrl Pts',(1.78452562099994,12.2,-10.28974099));
#160405=CARTESIAN_POINT('Ctrl Pts',(1.78496821499994,12.2,-10.291097983));
#160406=CARTESIAN_POINT('Ctrl Pts',(1.78541467399994,12.2,-10.292462403));
#160407=CARTESIAN_POINT('Ctrl Pts',(1.78586500399994,12.2,-10.293834224));
#160408=CARTESIAN_POINT('Ctrl Pts',(1.78631921299994,12.2,-10.295213422));
#160409=CARTESIAN_POINT('Ctrl Pts',(1.78677730899994,12.2,-10.296599975));
#160410=CARTESIAN_POINT('Ctrl Pts',(1.78723929699994,12.2,-10.297993858));
#160411=CARTESIAN_POINT('Ctrl Pts',(1.78770518699994,12.2,-10.299395046));
#160412=CARTESIAN_POINT('Ctrl Pts',(1.78817498599994,12.2,-10.300803517));
#160413=CARTESIAN_POINT('Ctrl Pts',(1.78864869999994,12.2,-10.302219248));
#160414=CARTESIAN_POINT('Ctrl Pts',(1.78912633699994,12.2,-10.303642215));
#160415=CARTESIAN_POINT('Ctrl Pts',(1.78960790399994,12.2,-10.305072393));
#160416=CARTESIAN_POINT('Ctrl Pts',(1.79009340899994,12.2,-10.306509762));
#160417=CARTESIAN_POINT('Ctrl Pts',(1.79058285799994,12.2,-10.307954296));
#160418=CARTESIAN_POINT('Ctrl Pts',(1.79107625799994,12.2,-10.309405975));
#160419=CARTESIAN_POINT('Ctrl Pts',(1.79157361699994,12.2,-10.310864772));
#160420=CARTESIAN_POINT('Ctrl Pts',(1.79207494099994,12.2,-10.312330668));
#160421=CARTESIAN_POINT('Ctrl Pts',(1.79258023699994,12.2,-10.313803638));
#160422=CARTESIAN_POINT('Ctrl Pts',(1.79308951199994,12.2,-10.315283661));
#160423=CARTESIAN_POINT('Ctrl Pts',(1.79360277399994,12.2,-10.316770712));
#160424=CARTESIAN_POINT('Ctrl Pts',(1.79412002899994,12.2,-10.318264771));
#160425=CARTESIAN_POINT('Ctrl Pts',(1.79464128299994,12.2,-10.319765813));
#160426=CARTESIAN_POINT('Ctrl Pts',(1.79516654299994,12.2,-10.321273818));
#160427=CARTESIAN_POINT('Ctrl Pts',(1.79569581699994,12.2,-10.322788763));
#160428=CARTESIAN_POINT('Ctrl Pts',(1.79622910999994,12.2,-10.324310627));
#160429=CARTESIAN_POINT('Ctrl Pts',(1.79676642999994,12.2,-10.325839385));
#160430=CARTESIAN_POINT('Ctrl Pts',(1.79730778399994,12.2,-10.327375017));
#160431=CARTESIAN_POINT('Ctrl Pts',(1.79785317499994,12.2,-10.328917501));
#160432=CARTESIAN_POINT('Ctrl Pts',(1.79840261399994,12.2,-10.330466814));
#160433=CARTESIAN_POINT('Ctrl Pts',(1.79895610399994,12.2,-10.332022936));
#160434=CARTESIAN_POINT('Ctrl Pts',(1.79951365499994,12.2,-10.333585844));
#160435=CARTESIAN_POINT('Ctrl Pts',(1.80007526999994,12.2,-10.335155517));
#160436=CARTESIAN_POINT('Ctrl Pts',(1.80064095699994,12.2,-10.336731933));
#160437=CARTESIAN_POINT('Ctrl Pts',(1.80121072099994,12.2,-10.338315071));
#160438=CARTESIAN_POINT('Ctrl Pts',(1.80178457199994,12.2,-10.33990491));
#160439=CARTESIAN_POINT('Ctrl Pts',(1.80236250999994,12.2,-10.341501427));
#160440=CARTESIAN_POINT('Ctrl Pts',(1.80294454699994,12.2,-10.343104603));
#160441=CARTESIAN_POINT('Ctrl Pts',(1.80353068699994,12.2,-10.344714415));
#160442=CARTESIAN_POINT('Ctrl Pts',(1.80412093499994,12.2,-10.346330843));
#160443=CARTESIAN_POINT('Ctrl Pts',(1.80471529899994,12.2,-10.347953866));
#160444=CARTESIAN_POINT('Ctrl Pts',(1.80531378399994,12.2,-10.349583463));
#160445=CARTESIAN_POINT('Ctrl Pts',(1.80591639699994,12.2,-10.351219612));
#160446=CARTESIAN_POINT('Ctrl Pts',(1.80652314299994,12.2,-10.352862295));
#160447=CARTESIAN_POINT('Ctrl Pts',(1.80713402799994,12.2,-10.354511488));
#160448=CARTESIAN_POINT('Ctrl Pts',(1.80774905899994,12.2,-10.356167172));
#160449=CARTESIAN_POINT('Ctrl Pts',(1.80836823999994,12.2,-10.357829328));
#160450=CARTESIAN_POINT('Ctrl Pts',(1.80899157899994,12.2,-10.359497933));
#160451=CARTESIAN_POINT('Ctrl Pts',(1.80961908099994,12.2,-10.361172966));
#160452=CARTESIAN_POINT('Ctrl Pts',(1.81025075099994,12.2,-10.36285441));
#160453=CARTESIAN_POINT('Ctrl Pts',(1.81088659599994,12.2,-10.364542242));
#160454=CARTESIAN_POINT('Ctrl Pts',(1.81152661999994,12.2,-10.366236444));
#160455=CARTESIAN_POINT('Ctrl Pts',(1.81217083099994,12.2,-10.367936993));
#160456=CARTESIAN_POINT('Ctrl Pts',(1.81281923299994,12.2,-10.369643871));
#160457=CARTESIAN_POINT('Ctrl Pts',(1.81347183299994,12.2,-10.371357057));
#160458=CARTESIAN_POINT('Ctrl Pts',(1.81412863499994,12.2,-10.373076533));
#160459=CARTESIAN_POINT('Ctrl Pts',(1.81478964499994,12.2,-10.374802277));
#160460=CARTESIAN_POINT('Ctrl Pts',(1.81545486999994,12.2,-10.37653427));
#160461=CARTESIAN_POINT('Ctrl Pts',(1.81612431399994,12.2,-10.378272492));
#160462=CARTESIAN_POINT('Ctrl Pts',(1.81679798299994,12.2,-10.380016924));
#160463=CARTESIAN_POINT('Ctrl Pts',(1.81747588199994,12.2,-10.381767545));
#160464=CARTESIAN_POINT('Ctrl Pts',(1.81815801699994,12.2,-10.383524338));
#160465=CARTESIAN_POINT('Ctrl Pts',(1.81884439299994,12.2,-10.385287281));
#160466=CARTESIAN_POINT('Ctrl Pts',(1.81953501599994,12.2,-10.387056356));
#160467=CARTESIAN_POINT('Ctrl Pts',(1.82022989099994,12.2,-10.388831543));
#160468=CARTESIAN_POINT('Ctrl Pts',(1.82092902199994,12.2,-10.390612824));
#160469=CARTESIAN_POINT('Ctrl Pts',(1.82163241599994,12.2,-10.392400178));
#160470=CARTESIAN_POINT('Ctrl Pts',(1.82234007799994,12.2,-10.394193587));
#160471=CARTESIAN_POINT('Ctrl Pts',(1.82305201199994,12.2,-10.395993031));
#160472=CARTESIAN_POINT('Ctrl Pts',(1.82376822599994,12.2,-10.397798492));
#160473=CARTESIAN_POINT('Ctrl Pts',(1.82448872099994,12.2,-10.399609952));
#160474=CARTESIAN_POINT('Ctrl Pts',(1.82521350499994,12.2,-10.401427389));
#160475=CARTESIAN_POINT('Ctrl Pts',(1.82594258299994,12.2,-10.403250787));
#160476=CARTESIAN_POINT('Ctrl Pts',(1.82667595799994,12.2,-10.405080125));
#160477=CARTESIAN_POINT('Ctrl Pts',(1.82741363699994,12.2,-10.406915387));
#160478=CARTESIAN_POINT('Ctrl Pts',(1.82815562499994,12.2,-10.408756552));
#160479=CARTESIAN_POINT('Ctrl Pts',(1.82890192699994,12.2,-10.410603603));
#160480=CARTESIAN_POINT('Ctrl Pts',(1.82965254599994,12.2,-10.41245652));
#160481=CARTESIAN_POINT('Ctrl Pts',(1.83040748999994,12.2,-10.414315286));
#160482=CARTESIAN_POINT('Ctrl Pts',(1.83116676099994,12.2,-10.416179881));
#160483=CARTESIAN_POINT('Ctrl Pts',(1.83193036499994,12.2,-10.418050288));
#160484=CARTESIAN_POINT('Ctrl Pts',(1.83269830799994,12.2,-10.419926488));
#160485=CARTESIAN_POINT('Ctrl Pts',(1.83347059199994,12.2,-10.421808463));
#160486=CARTESIAN_POINT('Ctrl Pts',(1.83424722399994,12.2,-10.423696194));
#160487=CARTESIAN_POINT('Ctrl Pts',(1.83502820899994,12.2,-10.425589665));
#160488=CARTESIAN_POINT('Ctrl Pts',(1.83581354999994,12.2,-10.427488857));
#160489=CARTESIAN_POINT('Ctrl Pts',(1.83660325299994,12.2,-10.429393751));
#160490=CARTESIAN_POINT('Ctrl Pts',(1.83739732299994,12.2,-10.431304329));
#160491=CARTESIAN_POINT('Ctrl Pts',(1.83819576299994,12.2,-10.433220574));
#160492=CARTESIAN_POINT('Ctrl Pts',(1.83899857899994,12.2,-10.435142468));
#160493=CARTESIAN_POINT('Ctrl Pts',(1.83980577599994,12.2,-10.437069993));
#160494=CARTESIAN_POINT('Ctrl Pts',(1.84061735599994,12.2,-10.439003132));
#160495=CARTESIAN_POINT('Ctrl Pts',(1.84143332699994,12.2,-10.440941867));
#160496=CARTESIAN_POINT('Ctrl Pts',(1.84225369099994,12.2,-10.442886179));
#160497=CARTESIAN_POINT('Ctrl Pts',(1.84307845299994,12.2,-10.444836053));
#160498=CARTESIAN_POINT('Ctrl Pts',(1.84390761699994,12.2,-10.446791469));
#160499=CARTESIAN_POINT('Ctrl Pts',(1.84474118899994,12.2,-10.44875241));
#160500=CARTESIAN_POINT('Ctrl Pts',(1.84557917199994,12.2,-10.45071886));
#160501=CARTESIAN_POINT('Ctrl Pts',(1.84642157199994,12.2,-10.452690801));
#160502=CARTESIAN_POINT('Ctrl Pts',(1.84726839199994,12.2,-10.454668215));
#160503=CARTESIAN_POINT('Ctrl Pts',(1.84811963599994,12.2,-10.456651085));
#160504=CARTESIAN_POINT('Ctrl Pts',(1.84897530999994,12.2,-10.458639395));
#160505=CARTESIAN_POINT('Ctrl Pts',(1.84983541599994,12.2,-10.460633126));
#160506=CARTESIAN_POINT('Ctrl Pts',(1.85069995999994,12.2,-10.462632262));
#160507=CARTESIAN_POINT('Ctrl Pts',(1.85156894599994,12.2,-10.464636786));
#160508=CARTESIAN_POINT('Ctrl Pts',(1.85244237799994,12.2,-10.46664668));
#160509=CARTESIAN_POINT('Ctrl Pts',(1.85332025899994,12.2,-10.468661929));
#160510=CARTESIAN_POINT('Ctrl Pts',(1.85420259499994,12.2,-10.470682514));
#160511=CARTESIAN_POINT('Ctrl Pts',(1.85508938999994,12.2,-10.47270842));
#160512=CARTESIAN_POINT('Ctrl Pts',(1.85598064599994,12.2,-10.474739628));
#160513=CARTESIAN_POINT('Ctrl Pts',(1.85687636999994,12.2,-10.476776123));
#160514=CARTESIAN_POINT('Ctrl Pts',(1.85777656499994,12.2,-10.478817888));
#160515=CARTESIAN_POINT('Ctrl Pts',(1.85868123399994,12.2,-10.480864906));
#160516=CARTESIAN_POINT('Ctrl Pts',(1.85959038199994,12.2,-10.48291716));
#160517=CARTESIAN_POINT('Ctrl Pts',(1.86050401199994,12.2,-10.484974634));
#160518=CARTESIAN_POINT('Ctrl Pts',(1.86142212899994,12.2,-10.487037312));
#160519=CARTESIAN_POINT('Ctrl Pts',(1.86234473699994,12.2,-10.489105177));
#160520=CARTESIAN_POINT('Ctrl Pts',(1.86327183899994,12.2,-10.491178213));
#160521=CARTESIAN_POINT('Ctrl Pts',(1.86420344099994,12.2,-10.493256403));
#160522=CARTESIAN_POINT('Ctrl Pts',(1.86513954299994,12.2,-10.49533973));
#160523=CARTESIAN_POINT('Ctrl Pts',(1.86608015299994,12.2,-10.497428179));
#160524=CARTESIAN_POINT('Ctrl Pts',(1.86702527199994,12.2,-10.499521733));
#160525=CARTESIAN_POINT('Ctrl Pts',(1.86797490499994,12.2,-10.501620377));
#160526=CARTESIAN_POINT('Ctrl Pts',(1.86892905699994,12.2,-10.503724094));
#160527=CARTESIAN_POINT('Ctrl Pts',(1.86988772999995,12.2,-10.505832868));
#160528=CARTESIAN_POINT('Ctrl Pts',(1.87085092699994,12.2,-10.507946683));
#160529=CARTESIAN_POINT('Ctrl Pts',(1.87181865399994,12.2,-10.510065522));
#160530=CARTESIAN_POINT('Ctrl Pts',(1.87279091299994,12.2,-10.512189371));
#160531=CARTESIAN_POINT('Ctrl Pts',(1.87376770899994,12.2,-10.514318212));
#160532=CARTESIAN_POINT('Ctrl Pts',(1.87474904299994,12.2,-10.516452031));
#160533=CARTESIAN_POINT('Ctrl Pts',(1.87573492299994,12.2,-10.518590811));
#160534=CARTESIAN_POINT('Ctrl Pts',(1.87672534799994,12.2,-10.520734536));
#160535=CARTESIAN_POINT('Ctrl Pts',(1.87772032499994,12.2,-10.522883192));
#160536=CARTESIAN_POINT('Ctrl Pts',(1.87871985699994,12.2,-10.525036762));
#160537=CARTESIAN_POINT('Ctrl Pts',(1.87972394599994,12.2,-10.52719523));
#160538=CARTESIAN_POINT('Ctrl Pts',(1.88073259699994,12.2,-10.529358581));
#160539=CARTESIAN_POINT('Ctrl Pts',(1.88174581199994,12.2,-10.531526798));
#160540=CARTESIAN_POINT('Ctrl Pts',(1.88276359599994,12.2,-10.533699869));
#160541=CARTESIAN_POINT('Ctrl Pts',(1.88378595299994,12.2,-10.535877775));
#160542=CARTESIAN_POINT('Ctrl Pts',(1.88481288399994,12.2,-10.538060503));
#160543=CARTESIAN_POINT('Ctrl Pts',(1.88584439399994,12.2,-10.540248035));
#160544=CARTESIAN_POINT('Ctrl Pts',(1.88688048599994,12.2,-10.542440358));
#160545=CARTESIAN_POINT('Ctrl Pts',(1.88792116399994,12.2,-10.544637455));
#160546=CARTESIAN_POINT('Ctrl Pts',(1.88896643099994,12.2,-10.546839313));
#160547=CARTESIAN_POINT('Ctrl Pts',(1.89001628999994,12.2,-10.549045913));
#160548=CARTESIAN_POINT('Ctrl Pts',(1.89107074499994,12.2,-10.551257244));
#160549=CARTESIAN_POINT('Ctrl Pts',(1.89212979899994,12.2,-10.553473288));
#160550=CARTESIAN_POINT('Ctrl Pts',(1.89319345499994,12.2,-10.555694032));
#160551=CARTESIAN_POINT('Ctrl Pts',(1.89426171599994,12.2,-10.557919458));
#160552=CARTESIAN_POINT('Ctrl Pts',(1.89533458699994,12.2,-10.560149554));
#160553=CARTESIAN_POINT('Ctrl Pts',(1.89641206899994,12.2,-10.562384303));
#160554=CARTESIAN_POINT('Ctrl Pts',(1.89749416599994,12.2,-10.564623691));
#160555=CARTESIAN_POINT('Ctrl Pts',(1.89858088099994,12.2,-10.566867703));
#160556=CARTESIAN_POINT('Ctrl Pts',(1.89967221899994,12.2,-10.569116324));
#160557=CARTESIAN_POINT('Ctrl Pts',(1.90076818099994,12.2,-10.571369539));
#160558=CARTESIAN_POINT('Ctrl Pts',(1.90186877099994,12.2,-10.573627333));
#160559=CARTESIAN_POINT('Ctrl Pts',(1.90297399099994,12.2,-10.575889692));
#160560=CARTESIAN_POINT('Ctrl Pts',(1.90408384599994,12.2,-10.578156601));
#160561=CARTESIAN_POINT('Ctrl Pts',(1.90519833799994,12.2,-10.580428044));
#160562=CARTESIAN_POINT('Ctrl Pts',(1.90631746999994,12.2,-10.582704009));
#160563=CARTESIAN_POINT('Ctrl Pts',(1.90744124499994,12.2,-10.584984479));
#160564=CARTESIAN_POINT('Ctrl Pts',(1.90856966599994,12.2,-10.587269441));
#160565=CARTESIAN_POINT('Ctrl Pts',(1.90970273699994,12.2,-10.58955888));
#160566=CARTESIAN_POINT('Ctrl Pts',(1.91084045999994,12.2,-10.59185278));
#160567=CARTESIAN_POINT('Ctrl Pts',(1.91198283799994,12.2,-10.594151129));
#160568=CARTESIAN_POINT('Ctrl Pts',(1.91312987399994,12.2,-10.59645391));
#160569=CARTESIAN_POINT('Ctrl Pts',(1.91428157099994,12.2,-10.598761112));
#160570=CARTESIAN_POINT('Ctrl Pts',(1.91543793199994,12.2,-10.601072717));
#160571=CARTESIAN_POINT('Ctrl Pts',(1.91659895999994,12.2,-10.603388714));
#160572=CARTESIAN_POINT('Ctrl Pts',(1.91776465699994,12.2,-10.605709085));
#160573=CARTESIAN_POINT('Ctrl Pts',(1.91893502699994,12.2,-10.60803382));
#160574=CARTESIAN_POINT('Ctrl Pts',(1.92011007299994,12.2,-10.610362901));
#160575=CARTESIAN_POINT('Ctrl Pts',(1.92128979599994,12.2,-10.612696316));
#160576=CARTESIAN_POINT('Ctrl Pts',(1.92247420099994,12.2,-10.615034051));
#160577=CARTESIAN_POINT('Ctrl Pts',(1.92366328999994,12.2,-10.617376091));
#160578=CARTESIAN_POINT('Ctrl Pts',(1.92485706499994,12.2,-10.619722422));
#160579=CARTESIAN_POINT('Ctrl Pts',(1.92605552899994,12.2,-10.622073029));
#160580=CARTESIAN_POINT('Ctrl Pts',(1.92725868499994,12.2,-10.6244279));
#160581=CARTESIAN_POINT('Ctrl Pts',(1.92846653599994,12.2,-10.62678702));
#160582=CARTESIAN_POINT('Ctrl Pts',(1.92967908399994,12.2,-10.629150376));
#160583=CARTESIAN_POINT('Ctrl Pts',(1.93089633299994,12.2,-10.631517953));
#160584=CARTESIAN_POINT('Ctrl Pts',(1.93211828499994,12.2,-10.633889738));
#160585=CARTESIAN_POINT('Ctrl Pts',(1.93334494199994,12.2,-10.636265715));
#160586=CARTESIAN_POINT('Ctrl Pts',(1.93457630699994,12.2,-10.638645874));
#160587=CARTESIAN_POINT('Ctrl Pts',(1.93581238299994,12.2,-10.641030197));
#160588=CARTESIAN_POINT('Ctrl Pts',(1.93705317299994,12.2,-10.643418674));
#160589=CARTESIAN_POINT('Ctrl Pts',(1.93829867699994,12.2,-10.645811289));
#160590=CARTESIAN_POINT('Ctrl Pts',(1.93954889999994,12.2,-10.648208029));
#160591=CARTESIAN_POINT('Ctrl Pts',(1.94080384499994,12.2,-10.650608881));
#160592=CARTESIAN_POINT('Ctrl Pts',(1.94206351299994,12.2,-10.65301383));
#160593=CARTESIAN_POINT('Ctrl Pts',(1.94332790699994,12.2,-10.655422864));
#160594=CARTESIAN_POINT('Ctrl Pts',(1.94459702899994,12.2,-10.657835968));
#160595=CARTESIAN_POINT('Ctrl Pts',(1.94587088199994,12.2,-10.660253129));
#160596=CARTESIAN_POINT('Ctrl Pts',(1.94714946899994,12.2,-10.662674334));
#160597=CARTESIAN_POINT('Ctrl Pts',(1.94843279199994,12.2,-10.665099571));
#160598=CARTESIAN_POINT('Ctrl Pts',(1.94972085299994,12.2,-10.667528823));
#160599=CARTESIAN_POINT('Ctrl Pts',(1.95101365499994,12.2,-10.66996208));
#160600=CARTESIAN_POINT('Ctrl Pts',(1.95231119999994,12.2,-10.672399326));
#160601=CARTESIAN_POINT('Ctrl Pts',(1.95361349099994,12.2,-10.674840549));
#160602=CARTESIAN_POINT('Ctrl Pts',(1.95492052999994,12.2,-10.677285737));
#160603=CARTESIAN_POINT('Ctrl Pts',(1.95623231799994,12.2,-10.679734874));
#160604=CARTESIAN_POINT('Ctrl Pts',(1.95754885999994,12.2,-10.682187948));
#160605=CARTESIAN_POINT('Ctrl Pts',(1.95887015699994,12.2,-10.684644947));
#160606=CARTESIAN_POINT('Ctrl Pts',(1.96019620999994,12.2,-10.687105856));
#160607=CARTESIAN_POINT('Ctrl Pts',(1.96152702299994,12.2,-10.689570664));
#160608=CARTESIAN_POINT('Ctrl Pts',(1.96286259899994,12.2,-10.692039356));
#160609=CARTESIAN_POINT('Ctrl Pts',(1.96420293799994,12.2,-10.694511919));
#160610=CARTESIAN_POINT('Ctrl Pts',(1.96554804399994,12.2,-10.696988341));
#160611=CARTESIAN_POINT('Ctrl Pts',(1.96689791799994,12.2,-10.699468609));
#160612=CARTESIAN_POINT('Ctrl Pts',(1.96825256199994,12.2,-10.70195271));
#160613=CARTESIAN_POINT('Ctrl Pts',(1.96961197999994,12.2,-10.704440629));
#160614=CARTESIAN_POINT('Ctrl Pts',(1.97097617299994,12.2,-10.706932355));
#160615=CARTESIAN_POINT('Ctrl Pts',(1.97234514399994,12.2,-10.709427876));
#160616=CARTESIAN_POINT('Ctrl Pts',(1.97371889299994,12.2,-10.711927177));
#160617=CARTESIAN_POINT('Ctrl Pts',(1.97509742499994,12.2,-10.714430247));
#160618=CARTESIAN_POINT('Ctrl Pts',(1.97648073999994,12.2,-10.716937073));
#160619=CARTESIAN_POINT('Ctrl Pts',(1.97786884099994,12.2,-10.71944764));
#160620=CARTESIAN_POINT('Ctrl Pts',(1.97926172999994,12.2,-10.721961937));
#160621=CARTESIAN_POINT('Ctrl Pts',(1.98065940899994,12.2,-10.724479952));
#160622=CARTESIAN_POINT('Ctrl Pts',(1.98206188099994,12.2,-10.727001672));
#160623=CARTESIAN_POINT('Ctrl Pts',(1.98346914499994,12.2,-10.729527083));
#160624=CARTESIAN_POINT('Ctrl Pts',(1.98488120699994,12.2,-10.732056173));
#160625=CARTESIAN_POINT('Ctrl Pts',(1.98629806699994,12.2,-10.73458893));
#160626=CARTESIAN_POINT('Ctrl Pts',(1.98771972699994,12.2,-10.737125341));
#160627=CARTESIAN_POINT('Ctrl Pts',(1.98914618999994,12.2,-10.739665394));
#160628=CARTESIAN_POINT('Ctrl Pts',(1.99057745699994,12.2,-10.742209076));
#160629=CARTESIAN_POINT('Ctrl Pts',(1.99201352899994,12.2,-10.744756374));
#160630=CARTESIAN_POINT('Ctrl Pts',(1.99345441099994,12.2,-10.747307276));
#160631=CARTESIAN_POINT('Ctrl Pts',(1.99490010199994,12.2,-10.74986177));
#160632=CARTESIAN_POINT('Ctrl Pts',(1.99635060499994,12.2,-10.752419844));
#160633=CARTESIAN_POINT('Ctrl Pts',(1.99780592199994,12.2,-10.754981484));
#160634=CARTESIAN_POINT('Ctrl Pts',(1.99926605499994,12.2,-10.757546678));
#160635=CARTESIAN_POINT('Ctrl Pts',(2.00073100599994,12.2,-10.760115415));
#160636=CARTESIAN_POINT('Ctrl Pts',(2.00220077599994,12.2,-10.762687682));
#160637=CARTESIAN_POINT('Ctrl Pts',(2.00367536799994,12.2,-10.765263466));
#160638=CARTESIAN_POINT('Ctrl Pts',(2.00515478199994,12.2,-10.767842756));
#160639=CARTESIAN_POINT('Ctrl Pts',(2.00663902299994,12.2,-10.77042554));
#160640=CARTESIAN_POINT('Ctrl Pts',(2.00812808999994,12.2,-10.773011803));
#160641=CARTESIAN_POINT('Ctrl Pts',(2.00962198599994,12.2,-10.775601537));
#160642=CARTESIAN_POINT('Ctrl Pts',(2.01112071299994,12.2,-10.778194727));
#160643=CARTESIAN_POINT('Ctrl Pts',(2.01262427099994,12.2,-10.780791361));
#160644=CARTESIAN_POINT('Ctrl Pts',(2.01413266399994,12.2,-10.783391428));
#160645=CARTESIAN_POINT('Ctrl Pts',(2.01564589299994,12.2,-10.785994916));
#160646=CARTESIAN_POINT('Ctrl Pts',(2.01716395899994,12.2,-10.788601812));
#160647=CARTESIAN_POINT('Ctrl Pts',(2.01868686499994,12.2,-10.791212104));
#160648=CARTESIAN_POINT('Ctrl Pts',(2.02021461099994,12.2,-10.793825781));
#160649=CARTESIAN_POINT('Ctrl Pts',(2.02174720099995,12.2,-10.796442831));
#160650=CARTESIAN_POINT('Ctrl Pts',(2.02328463399994,12.2,-10.799063241));
#160651=CARTESIAN_POINT('Ctrl Pts',(2.02482691399994,12.2,-10.801687));
#160652=CARTESIAN_POINT('Ctrl Pts',(2.02637404199994,12.2,-10.804314097));
#160653=CARTESIAN_POINT('Ctrl Pts',(2.02792601899994,12.2,-10.806944517));
#160654=CARTESIAN_POINT('Ctrl Pts',(2.02948284599994,12.2,-10.809578251));
#160655=CARTESIAN_POINT('Ctrl Pts',(2.03104452699994,12.2,-10.812215287));
#160656=CARTESIAN_POINT('Ctrl Pts',(2.03261106199994,12.2,-10.814855611));
#160657=CARTESIAN_POINT('Ctrl Pts',(2.03418245199994,12.2,-10.817499214));
#160658=CARTESIAN_POINT('Ctrl Pts',(2.03575870099994,12.2,-10.820146083));
#160659=CARTESIAN_POINT('Ctrl Pts',(2.03733980799994,12.2,-10.822796206));
#160660=CARTESIAN_POINT('Ctrl Pts',(2.03892577499994,12.2,-10.825449572));
#160661=CARTESIAN_POINT('Ctrl Pts',(2.04051660599994,12.2,-10.82810617));
#160662=CARTESIAN_POINT('Ctrl Pts',(2.04211229899994,12.2,-10.830765986));
#160663=CARTESIAN_POINT('Ctrl Pts',(2.04371285699994,12.2,-10.833429011));
#160664=CARTESIAN_POINT('Ctrl Pts',(2.04531828199995,12.2,-10.836095232));
#160665=CARTESIAN_POINT('Ctrl Pts',(2.04692857599994,12.2,-10.838764637));
#160666=CARTESIAN_POINT('Ctrl Pts',(2.04854373899995,12.2,-10.841437216));
#160667=CARTESIAN_POINT('Ctrl Pts',(2.05016377299994,12.2,-10.844112955));
#160668=CARTESIAN_POINT('Ctrl Pts',(2.05178868099994,12.2,-10.846791846));
#160669=CARTESIAN_POINT('Ctrl Pts',(2.05341846199994,12.2,-10.849473875));
#160670=CARTESIAN_POINT('Ctrl Pts',(2.05505311799994,12.2,-10.852159032));
#160671=CARTESIAN_POINT('Ctrl Pts',(2.05669265099994,12.2,-10.854847303));
#160672=CARTESIAN_POINT('Ctrl Pts',(2.05833706199994,12.2,-10.85753868));
#160673=CARTESIAN_POINT('Ctrl Pts',(2.05998635399994,12.2,-10.86023315));
#160674=CARTESIAN_POINT('Ctrl Pts',(2.06164052499994,12.2,-10.862930702));
#160675=CARTESIAN_POINT('Ctrl Pts',(2.06329958099994,12.2,-10.865631323));
#160676=CARTESIAN_POINT('Ctrl Pts',(2.06496351899994,12.2,-10.868335004));
#160677=CARTESIAN_POINT('Ctrl Pts',(2.06663234299994,12.2,-10.871041734));
#160678=CARTESIAN_POINT('Ctrl Pts',(2.06830605399994,12.2,-10.873751499));
#160679=CARTESIAN_POINT('Ctrl Pts',(2.06998465199994,12.2,-10.876464289));
#160680=CARTESIAN_POINT('Ctrl Pts',(2.07166813899994,12.2,-10.879180094));
#160681=CARTESIAN_POINT('Ctrl Pts',(2.07335651799994,12.2,-10.881898902));
#160682=CARTESIAN_POINT('Ctrl Pts',(2.07504978799994,12.2,-10.884620701));
#160683=CARTESIAN_POINT('Ctrl Pts',(2.07674794999994,12.2,-10.887345482));
#160684=CARTESIAN_POINT('Ctrl Pts',(2.07845100699994,12.2,-10.890073231));
#160685=CARTESIAN_POINT('Ctrl Pts',(2.08015896099994,12.2,-10.89280394));
#160686=CARTESIAN_POINT('Ctrl Pts',(2.08187181099994,12.2,-10.895537595));
#160687=CARTESIAN_POINT('Ctrl Pts',(2.08358955799994,12.2,-10.898274186));
#160688=CARTESIAN_POINT('Ctrl Pts',(2.08531220499994,12.2,-10.901013703));
#160689=CARTESIAN_POINT('Ctrl Pts',(2.08703975299994,12.2,-10.903756135));
#160690=CARTESIAN_POINT('Ctrl Pts',(2.08877220299994,12.2,-10.906501469));
#160691=CARTESIAN_POINT('Ctrl Pts',(2.09050955499994,12.2,-10.909249695));
#160692=CARTESIAN_POINT('Ctrl Pts',(2.09225181099994,12.2,-10.912000804));
#160693=CARTESIAN_POINT('Ctrl Pts',(2.09399897299994,12.2,-10.914754782));
#160694=CARTESIAN_POINT('Ctrl Pts',(2.09575104199994,12.2,-10.91751162));
#160695=CARTESIAN_POINT('Ctrl Pts',(2.09750801799994,12.2,-10.920271306));
#160696=CARTESIAN_POINT('Ctrl Pts',(2.09926990199994,12.2,-10.92303383));
#160697=CARTESIAN_POINT('Ctrl Pts',(2.10103669699994,12.2,-10.925799182));
#160698=CARTESIAN_POINT('Ctrl Pts',(2.10280840299994,12.2,-10.928567349));
#160699=CARTESIAN_POINT('Ctrl Pts',(2.10458501999994,12.2,-10.931338321));
#160700=CARTESIAN_POINT('Ctrl Pts',(2.10636655199994,12.2,-10.934112088));
#160701=CARTESIAN_POINT('Ctrl Pts',(2.10815299699994,12.2,-10.936888638));
#160702=CARTESIAN_POINT('Ctrl Pts',(2.10994435799994,12.2,-10.939667962));
#160703=CARTESIAN_POINT('Ctrl Pts',(2.11174063499994,12.2,-10.942450048));
#160704=CARTESIAN_POINT('Ctrl Pts',(2.11354182899994,12.2,-10.945234885));
#160705=CARTESIAN_POINT('Ctrl Pts',(2.11534794299994,12.2,-10.948022463));
#160706=CARTESIAN_POINT('Ctrl Pts',(2.11715897499994,12.2,-10.950812772));
#160707=CARTESIAN_POINT('Ctrl Pts',(2.11897492799995,12.2,-10.953605801));
#160708=CARTESIAN_POINT('Ctrl Pts',(2.12079580299994,12.2,-10.956401537));
#160709=CARTESIAN_POINT('Ctrl Pts',(2.12262159999994,12.2,-10.959199973));
#160710=CARTESIAN_POINT('Ctrl Pts',(2.12445232199994,12.2,-10.962001096));
#160711=CARTESIAN_POINT('Ctrl Pts',(2.12628796699994,12.2,-10.964804897));
#160712=CARTESIAN_POINT('Ctrl Pts',(2.12812853899994,12.2,-10.967611364));
#160713=CARTESIAN_POINT('Ctrl Pts',(2.12997403599994,12.2,-10.970420488));
#160714=CARTESIAN_POINT('Ctrl Pts',(2.13182446099994,12.2,-10.973232257));
#160715=CARTESIAN_POINT('Ctrl Pts',(2.13367981499994,12.2,-10.976046662));
#160716=CARTESIAN_POINT('Ctrl Pts',(2.13554009799994,12.2,-10.978863691));
#160717=CARTESIAN_POINT('Ctrl Pts',(2.13740531099994,12.2,-10.981683335));
#160718=CARTESIAN_POINT('Ctrl Pts',(2.13927545499994,12.2,-10.984505583));
#160719=CARTESIAN_POINT('Ctrl Pts',(2.14115053099994,12.2,-10.987330423));
#160720=CARTESIAN_POINT('Ctrl Pts',(2.14303053999994,12.2,-10.990157848));
#160721=CARTESIAN_POINT('Ctrl Pts',(2.14491548299994,12.2,-10.992987845));
#160722=CARTESIAN_POINT('Ctrl Pts',(2.14680536099995,12.2,-10.995820404));
#160723=CARTESIAN_POINT('Ctrl Pts',(2.14870017399994,12.2,-10.998655516));
#160724=CARTESIAN_POINT('Ctrl Pts',(2.15059992399994,12.2,-11.00149317));
#160725=CARTESIAN_POINT('Ctrl Pts',(2.15250460999994,12.2,-11.004333355));
#160726=CARTESIAN_POINT('Ctrl Pts',(2.15441423499994,12.2,-11.007176061));
#160727=CARTESIAN_POINT('Ctrl Pts',(2.15632879899994,12.2,-11.010021278));
#160728=CARTESIAN_POINT('Ctrl Pts',(2.15824830199994,12.2,-11.012868997));
#160729=CARTESIAN_POINT('Ctrl Pts',(2.16017274599994,12.2,-11.015719205));
#160730=CARTESIAN_POINT('Ctrl Pts',(2.16210213199994,12.2,-11.018571894));
#160731=CARTESIAN_POINT('Ctrl Pts',(2.16403645899994,12.2,-11.021427054));
#160732=CARTESIAN_POINT('Ctrl Pts',(2.16597572899994,12.2,-11.024284674));
#160733=CARTESIAN_POINT('Ctrl Pts',(2.16791994199994,12.2,-11.027144743));
#160734=CARTESIAN_POINT('Ctrl Pts',(2.16986909999994,12.2,-11.030007252));
#160735=CARTESIAN_POINT('Ctrl Pts',(2.17182320399994,12.2,-11.032872191));
#160736=CARTESIAN_POINT('Ctrl Pts',(2.17378225199994,12.2,-11.03573955));
#160737=CARTESIAN_POINT('Ctrl Pts',(2.17574624699994,12.2,-11.038609318));
#160738=CARTESIAN_POINT('Ctrl Pts',(2.17771518999994,12.2,-11.041481486));
#160739=CARTESIAN_POINT('Ctrl Pts',(2.17968908099994,12.2,-11.044356044));
#160740=CARTESIAN_POINT('Ctrl Pts',(2.18166791999994,12.2,-11.047232981));
#160741=CARTESIAN_POINT('Ctrl Pts',(2.18365170899994,12.2,-11.050112287));
#160742=CARTESIAN_POINT('Ctrl Pts',(2.18564044699994,12.2,-11.052993953));
#160743=CARTESIAN_POINT('Ctrl Pts',(2.18763413599994,12.2,-11.055877969));
#160744=CARTESIAN_POINT('Ctrl Pts',(2.18963277699994,12.2,-11.058764325));
#160745=CARTESIAN_POINT('Ctrl Pts',(2.19163636999994,12.2,-11.06165301));
#160746=CARTESIAN_POINT('Ctrl Pts',(2.19364491499995,12.2,-11.064544015));
#160747=CARTESIAN_POINT('Ctrl Pts',(2.19565841299994,12.2,-11.067437331));
#160748=CARTESIAN_POINT('Ctrl Pts',(2.19767686499994,12.2,-11.070332945));
#160749=CARTESIAN_POINT('Ctrl Pts',(2.19970027199994,12.2,-11.073230851));
#160750=CARTESIAN_POINT('Ctrl Pts',(2.20172863299994,12.2,-11.076131037));
#160751=CARTESIAN_POINT('Ctrl Pts',(2.20376195099994,12.2,-11.079033493));
#160752=CARTESIAN_POINT('Ctrl Pts',(2.20580022499994,12.2,-11.081938212));
#160753=CARTESIAN_POINT('Ctrl Pts',(2.20784345599994,12.2,-11.08484518));
#160754=CARTESIAN_POINT('Ctrl Pts',(2.20989164299994,12.2,-11.08775439));
#160755=CARTESIAN_POINT('Ctrl Pts',(2.21194478899994,12.2,-11.090665832));
#160756=CARTESIAN_POINT('Ctrl Pts',(2.21400289399994,12.2,-11.093579495));
#160757=CARTESIAN_POINT('Ctrl Pts',(2.21606595699994,12.2,-11.096495371));
#160758=CARTESIAN_POINT('Ctrl Pts',(2.21813398099994,12.2,-11.099413448));
#160759=CARTESIAN_POINT('Ctrl Pts',(2.22020696299994,12.2,-11.10233372));
#160760=CARTESIAN_POINT('Ctrl Pts',(2.22228490799994,12.2,-11.105256173));
#160761=CARTESIAN_POINT('Ctrl Pts',(2.22436781299994,12.2,-11.1081808));
#160762=CARTESIAN_POINT('Ctrl Pts',(2.22645567899994,12.2,-11.111107592));
#160763=CARTESIAN_POINT('Ctrl Pts',(2.22854850699994,12.2,-11.114036538));
#160764=CARTESIAN_POINT('Ctrl Pts',(2.23064629799994,12.2,-11.116967627));
#160765=CARTESIAN_POINT('Ctrl Pts',(2.23274905199994,12.2,-11.119900853));
#160766=CARTESIAN_POINT('Ctrl Pts',(2.23485676999994,12.2,-11.122836204));
#160767=CARTESIAN_POINT('Ctrl Pts',(2.23696945199995,12.2,-11.125773671));
#160768=CARTESIAN_POINT('Ctrl Pts',(2.23908709799994,12.2,-11.128713243));
#160769=CARTESIAN_POINT('Ctrl Pts',(2.24120970899994,12.2,-11.131654914));
#160770=CARTESIAN_POINT('Ctrl Pts',(2.24333728499994,12.2,-11.134598671));
#160771=CARTESIAN_POINT('Ctrl Pts',(2.24546982699994,12.2,-11.137544507));
#160772=CARTESIAN_POINT('Ctrl Pts',(2.24760733499994,12.2,-11.140492411));
#160773=CARTESIAN_POINT('Ctrl Pts',(2.24974980999994,12.2,-11.143442374));
#160774=CARTESIAN_POINT('Ctrl Pts',(2.25189725099994,12.2,-11.146394387));
#160775=CARTESIAN_POINT('Ctrl Pts',(2.25404965899994,12.2,-11.14934844));
#160776=CARTESIAN_POINT('Ctrl Pts',(2.25620703599994,12.2,-11.152304524));
#160777=CARTESIAN_POINT('Ctrl Pts',(2.25836937999994,12.2,-11.15526263));
#160778=CARTESIAN_POINT('Ctrl Pts',(2.26053669299994,12.2,-11.158222747));
#160779=CARTESIAN_POINT('Ctrl Pts',(2.26270897299994,12.2,-11.161184868));
#160780=CARTESIAN_POINT('Ctrl Pts',(2.26488622499994,12.2,-11.164148983));
#160781=CARTESIAN_POINT('Ctrl Pts',(2.26706844499994,12.2,-11.16711508));
#160782=CARTESIAN_POINT('Ctrl Pts',(2.26925563399994,12.2,-11.170083153));
#160783=CARTESIAN_POINT('Ctrl Pts',(2.27144779299994,12.2,-11.173053191));
#160784=CARTESIAN_POINT('Ctrl Pts',(2.27364492299994,12.2,-11.176025185));
#160785=CARTESIAN_POINT('Ctrl Pts',(2.27584702399994,12.2,-11.178999126));
#160786=CARTESIAN_POINT('Ctrl Pts',(2.27805409499994,12.2,-11.181975005));
#160787=CARTESIAN_POINT('Ctrl Pts',(2.28026613799994,12.2,-11.184952813));
#160788=CARTESIAN_POINT('Ctrl Pts',(2.28248315299994,12.2,-11.187932541));
#160789=CARTESIAN_POINT('Ctrl Pts',(2.28470513799994,12.2,-11.190914179));
#160790=CARTESIAN_POINT('Ctrl Pts',(2.28693209699994,12.2,-11.193897718));
#160791=CARTESIAN_POINT('Ctrl Pts',(2.28916402699994,12.2,-11.19688315));
#160792=CARTESIAN_POINT('Ctrl Pts',(2.29140092999994,12.2,-11.199870463));
#160793=CARTESIAN_POINT('Ctrl Pts',(2.29364280599994,12.2,-11.202859649));
#160794=CARTESIAN_POINT('Ctrl Pts',(2.29588965499994,12.2,-11.205850698));
#160795=CARTESIAN_POINT('Ctrl Pts',(2.29814147699994,12.2,-11.208843602));
#160796=CARTESIAN_POINT('Ctrl Pts',(2.30039827299994,12.2,-11.211838352));
#160797=CARTESIAN_POINT('Ctrl Pts',(2.30266004099994,12.2,-11.214834939));
#160798=CARTESIAN_POINT('Ctrl Pts',(2.30492678499994,12.2,-11.217833355));
#160799=CARTESIAN_POINT('Ctrl Pts',(2.30719850199994,12.2,-11.220833593));
#160800=CARTESIAN_POINT('Ctrl Pts',(2.30947519299994,12.2,-11.223835644));
#160801=CARTESIAN_POINT('Ctrl Pts',(2.31175685799994,12.2,-11.226839497));
#160802=CARTESIAN_POINT('Ctrl Pts',(2.31404349799994,12.2,-11.229845144));
#160803=CARTESIAN_POINT('Ctrl Pts',(2.31633511299994,12.2,-11.232852572));
#160804=CARTESIAN_POINT('Ctrl Pts',(2.31863170299994,12.2,-11.235861771));
#160805=CARTESIAN_POINT('Ctrl Pts',(2.32093326799994,12.2,-11.238872729));
#160806=CARTESIAN_POINT('Ctrl Pts',(2.32323980899994,12.2,-11.241885437));
#160807=CARTESIAN_POINT('Ctrl Pts',(2.32555132399995,12.2,-11.244899887));
#160808=CARTESIAN_POINT('Ctrl Pts',(2.32786781499994,12.2,-11.247916073));
#160809=CARTESIAN_POINT('Ctrl Pts',(2.33018928299995,12.2,-11.250933991));
#160810=CARTESIAN_POINT('Ctrl Pts',(2.33251572399995,12.2,-11.253953638));
#160811=CARTESIAN_POINT('Ctrl Pts',(2.33438085799994,12.2,-11.256370739));
#160812=CARTESIAN_POINT('Ctrl Pts',(2.33578194799994,12.2,-11.258184341));
#160813=CARTESIAN_POINT('Ctrl Pts',(2.33671700199995,12.2,-11.259393754));
#160814=CARTESIAN_POINT('Ctrl Pts',(2.33718477799994,12.2,-11.259998548));
#160815=CARTESIAN_POINT('Origin',(-5.66257110645729E-14,15.2,-1.77635683940025E-14));
#160816=CARTESIAN_POINT('',(3.20199116203656,15.2,-9.8685296574462));
#160817=CARTESIAN_POINT('',(3.20199116203656,12.2,-9.8685296574462));
#160818=CARTESIAN_POINT('',(3.20199116199994,15.2,-9.86852965700001));
#160819=CARTESIAN_POINT('Origin',(-5.66257110645729E-14,12.2,-1.77635683940025E-14));
#160820=CARTESIAN_POINT('Origin',(-5.66257110645729E-14,15.2,-1.77635683940025E-14));
#160821=CARTESIAN_POINT('Origin',(-5.66257110645729E-14,15.2,-1.77635683940025E-14));
#160822=CARTESIAN_POINT('',(3.91586047899994,15.2,-10.812771925));
#160823=CARTESIAN_POINT('',(4.27433546799994,15.2,-10.676144262));
#160824=CARTESIAN_POINT('Origin',(-5.66257110645729E-14,15.2,-1.77635683940025E-14));
#160825=CARTESIAN_POINT('',(4.27433546799994,12.2,-10.676144262));
#160826=CARTESIAN_POINT('',(4.27433546799994,15.2,-10.676144262));
#160827=CARTESIAN_POINT('',(3.91586047899994,12.2,-10.812771925));
#160828=CARTESIAN_POINT('Origin',(-5.66257110645729E-14,12.2,-1.77635683940025E-14));
#160829=CARTESIAN_POINT('',(3.91586047899994,15.2,-10.812771925));
#160830=CARTESIAN_POINT('Ctrl Pts',(3.20199116199994,15.2,-9.86852965800001));
#160831=CARTESIAN_POINT('Ctrl Pts',(3.20199116199994,11.6,-9.86852965800001));
#160832=CARTESIAN_POINT('Ctrl Pts',(3.20205902599994,15.2,-9.86869026600001));
#160833=CARTESIAN_POINT('Ctrl Pts',(3.20205902599994,11.6,-9.86869026600001));
#160834=CARTESIAN_POINT('Ctrl Pts',(3.20219720499994,15.2,-9.86901706000001));
#160835=CARTESIAN_POINT('Ctrl Pts',(3.20219720499994,11.6,-9.86901706000001));
#160836=CARTESIAN_POINT('Ctrl Pts',(3.20240682399994,15.2,-9.86951212500001));
#160837=CARTESIAN_POINT('Ctrl Pts',(3.20240682399994,11.6,-9.86951212500001));
#160838=CARTESIAN_POINT('Ctrl Pts',(3.20268969699995,15.2,-9.87017881300001));
#160839=CARTESIAN_POINT('Ctrl Pts',(3.20268969699995,11.6,-9.87017881300001));
#160840=CARTESIAN_POINT('Ctrl Pts',(3.20304832999994,15.2,-9.87102171600001));
#160841=CARTESIAN_POINT('Ctrl Pts',(3.20304832999994,11.6,-9.87102171600001));
#160842=CARTESIAN_POINT('Ctrl Pts',(3.20341363499994,15.2,-9.87187791600001));
#160843=CARTESIAN_POINT('Ctrl Pts',(3.20341363499994,11.6,-9.87187791600001));
#160844=CARTESIAN_POINT('Ctrl Pts',(3.20378354199994,15.2,-9.87274249600001));
#160845=CARTESIAN_POINT('Ctrl Pts',(3.20378354199994,11.6,-9.87274249600001));
#160846=CARTESIAN_POINT('Ctrl Pts',(3.20415805699994,15.2,-9.87361542400001));
#160847=CARTESIAN_POINT('Ctrl Pts',(3.20415805699994,11.6,-9.87361542400001));
#160848=CARTESIAN_POINT('Ctrl Pts',(3.20453718399994,15.2,-9.87449667000002));
#160849=CARTESIAN_POINT('Ctrl Pts',(3.20453718399994,11.6,-9.87449667000002));
#160850=CARTESIAN_POINT('Ctrl Pts',(3.20492092999995,15.2,-9.87538620000001));
#160851=CARTESIAN_POINT('Ctrl Pts',(3.20492092999995,11.6,-9.87538620000001));
#160852=CARTESIAN_POINT('Ctrl Pts',(3.20530930299994,15.2,-9.87628398500001));
#160853=CARTESIAN_POINT('Ctrl Pts',(3.20530930299994,11.6,-9.87628398500001));
#160854=CARTESIAN_POINT('Ctrl Pts',(3.20570230499994,15.2,-9.87718999100001));
#160855=CARTESIAN_POINT('Ctrl Pts',(3.20570230499994,11.6,-9.87718999100001));
#160856=CARTESIAN_POINT('Ctrl Pts',(3.20609994399994,15.2,-9.87810418800001));
#160857=CARTESIAN_POINT('Ctrl Pts',(3.20609994399994,11.6,-9.87810418800001));
#160858=CARTESIAN_POINT('Ctrl Pts',(3.20650222799994,15.2,-9.87902654500001));
#160859=CARTESIAN_POINT('Ctrl Pts',(3.20650222799994,11.6,-9.87902654500001));
#160860=CARTESIAN_POINT('Ctrl Pts',(3.20690915899994,15.2,-9.87995703200001));
#160861=CARTESIAN_POINT('Ctrl Pts',(3.20690915899994,11.6,-9.87995703200001));
#160862=CARTESIAN_POINT('Ctrl Pts',(3.20732074299994,15.2,-9.88089561700001));
#160863=CARTESIAN_POINT('Ctrl Pts',(3.20732074299994,11.6,-9.88089561700001));
#160864=CARTESIAN_POINT('Ctrl Pts',(3.20773698899994,15.2,-9.88184227000001));
#160865=CARTESIAN_POINT('Ctrl Pts',(3.20773698899994,11.6,-9.88184227000001));
#160866=CARTESIAN_POINT('Ctrl Pts',(3.20815789999994,15.2,-9.88279696000001));
#160867=CARTESIAN_POINT('Ctrl Pts',(3.20815789999994,11.6,-9.88279696000001));
#160868=CARTESIAN_POINT('Ctrl Pts',(3.20858348199994,15.2,-9.88375965700001));
#160869=CARTESIAN_POINT('Ctrl Pts',(3.20858348199994,11.6,-9.88375965700001));
#160870=CARTESIAN_POINT('Ctrl Pts',(3.20901374099994,15.2,-9.88473033000002));
#160871=CARTESIAN_POINT('Ctrl Pts',(3.20901374099994,11.6,-9.88473033000002));
#160872=CARTESIAN_POINT('Ctrl Pts',(3.20944868199994,15.2,-9.88570895100001));
#160873=CARTESIAN_POINT('Ctrl Pts',(3.20944868199994,11.6,-9.88570895100001));
#160874=CARTESIAN_POINT('Ctrl Pts',(3.20988831099994,15.2,-9.88669548800001));
#160875=CARTESIAN_POINT('Ctrl Pts',(3.20988831099994,11.6,-9.88669548800001));
#160876=CARTESIAN_POINT('Ctrl Pts',(3.21033263399995,15.2,-9.88768991300001));
#160877=CARTESIAN_POINT('Ctrl Pts',(3.21033263399995,11.6,-9.88768991300001));
#160878=CARTESIAN_POINT('Ctrl Pts',(3.21078165499994,15.2,-9.88869219500001));
#160879=CARTESIAN_POINT('Ctrl Pts',(3.21078165499994,11.6,-9.88869219500001));
#160880=CARTESIAN_POINT('Ctrl Pts',(3.21123537899994,15.2,-9.88970230500001));
#160881=CARTESIAN_POINT('Ctrl Pts',(3.21123537899994,11.6,-9.88970230500001));
#160882=CARTESIAN_POINT('Ctrl Pts',(3.21169381299995,15.2,-9.89072021500001));
#160883=CARTESIAN_POINT('Ctrl Pts',(3.21169381299995,11.6,-9.89072021500001));
#160884=CARTESIAN_POINT('Ctrl Pts',(3.21215696199994,15.2,-9.89174589300001));
#160885=CARTESIAN_POINT('Ctrl Pts',(3.21215696199994,11.6,-9.89174589300001));
#160886=CARTESIAN_POINT('Ctrl Pts',(3.21262482999995,15.2,-9.89277931200001));
#160887=CARTESIAN_POINT('Ctrl Pts',(3.21262482999995,11.6,-9.89277931200001));
#160888=CARTESIAN_POINT('Ctrl Pts',(3.21309742399994,15.2,-9.89382044200001));
#160889=CARTESIAN_POINT('Ctrl Pts',(3.21309742399994,11.6,-9.89382044200001));
#160890=CARTESIAN_POINT('Ctrl Pts',(3.21357474799994,15.2,-9.89486925600001));
#160891=CARTESIAN_POINT('Ctrl Pts',(3.21357474799994,11.6,-9.89486925600001));
#160892=CARTESIAN_POINT('Ctrl Pts',(3.21405680799994,15.2,-9.89592572400001));
#160893=CARTESIAN_POINT('Ctrl Pts',(3.21405680799994,11.6,-9.89592572400001));
#160894=CARTESIAN_POINT('Ctrl Pts',(3.21454360799994,15.2,-9.89698981600001));
#160895=CARTESIAN_POINT('Ctrl Pts',(3.21454360799994,11.6,-9.89698981600001));
#160896=CARTESIAN_POINT('Ctrl Pts',(3.21503515299994,15.2,-9.89806150600001));
#160897=CARTESIAN_POINT('Ctrl Pts',(3.21503515299994,11.6,-9.89806150600001));
#160898=CARTESIAN_POINT('Ctrl Pts',(3.21553144899994,15.2,-9.89914076600001));
#160899=CARTESIAN_POINT('Ctrl Pts',(3.21553144899994,11.6,-9.89914076600001));
#160900=CARTESIAN_POINT('Ctrl Pts',(3.21603250099994,15.2,-9.90022756600001));
#160901=CARTESIAN_POINT('Ctrl Pts',(3.21603250099994,11.6,-9.90022756600001));
#160902=CARTESIAN_POINT('Ctrl Pts',(3.21653831299994,15.2,-9.90132187800001));
#160903=CARTESIAN_POINT('Ctrl Pts',(3.21653831299994,11.6,-9.90132187800001));
#160904=CARTESIAN_POINT('Ctrl Pts',(3.21704888999994,15.2,-9.90242367500001));
#160905=CARTESIAN_POINT('Ctrl Pts',(3.21704888999994,11.6,-9.90242367500001));
#160906=CARTESIAN_POINT('Ctrl Pts',(3.21756423699994,15.2,-9.90353292900001));
#160907=CARTESIAN_POINT('Ctrl Pts',(3.21756423699994,11.6,-9.90353292900001));
#160908=CARTESIAN_POINT('Ctrl Pts',(3.21808435999994,15.2,-9.90464961300001));
#160909=CARTESIAN_POINT('Ctrl Pts',(3.21808435999994,11.6,-9.90464961300001));
#160910=CARTESIAN_POINT('Ctrl Pts',(3.21860926299995,15.2,-9.90577369800001));
#160911=CARTESIAN_POINT('Ctrl Pts',(3.21860926299995,11.6,-9.90577369800001));
#160912=CARTESIAN_POINT('Ctrl Pts',(3.21913895099994,15.2,-9.90690515700001));
#160913=CARTESIAN_POINT('Ctrl Pts',(3.21913895099994,11.6,-9.90690515700001));
#160914=CARTESIAN_POINT('Ctrl Pts',(3.21967342799995,15.2,-9.90804396500001));
#160915=CARTESIAN_POINT('Ctrl Pts',(3.21967342799995,11.6,-9.90804396500001));
#160916=CARTESIAN_POINT('Ctrl Pts',(3.22021269999994,15.2,-9.90919009100001));
#160917=CARTESIAN_POINT('Ctrl Pts',(3.22021269999994,11.6,-9.90919009100001));
#160918=CARTESIAN_POINT('Ctrl Pts',(3.22075676999994,15.2,-9.91034351100001));
#160919=CARTESIAN_POINT('Ctrl Pts',(3.22075676999994,11.6,-9.91034351100001));
#160920=CARTESIAN_POINT('Ctrl Pts',(3.22130564299994,15.2,-9.91150419600001));
#160921=CARTESIAN_POINT('Ctrl Pts',(3.22130564299994,11.6,-9.91150419600001));
#160922=CARTESIAN_POINT('Ctrl Pts',(3.22185932499994,15.2,-9.91267212100001));
#160923=CARTESIAN_POINT('Ctrl Pts',(3.22185932499994,11.6,-9.91267212100001));
#160924=CARTESIAN_POINT('Ctrl Pts',(3.22241781899994,15.2,-9.91384725700001));
#160925=CARTESIAN_POINT('Ctrl Pts',(3.22241781899994,11.6,-9.91384725700001));
#160926=CARTESIAN_POINT('Ctrl Pts',(3.22298112999994,15.2,-9.91502958000001));
#160927=CARTESIAN_POINT('Ctrl Pts',(3.22298112999994,11.6,-9.91502958000001));
#160928=CARTESIAN_POINT('Ctrl Pts',(3.22354926399994,15.2,-9.91621906300001));
#160929=CARTESIAN_POINT('Ctrl Pts',(3.22354926399994,11.6,-9.91621906300001));
#160930=CARTESIAN_POINT('Ctrl Pts',(3.22412222299994,15.2,-9.91741567800001));
#160931=CARTESIAN_POINT('Ctrl Pts',(3.22412222299994,11.6,-9.91741567800001));
#160932=CARTESIAN_POINT('Ctrl Pts',(3.22470001299994,15.2,-9.91861939900001));
#160933=CARTESIAN_POINT('Ctrl Pts',(3.22470001299994,11.6,-9.91861939900001));
#160934=CARTESIAN_POINT('Ctrl Pts',(3.22528263699994,15.2,-9.91983020100001));
#160935=CARTESIAN_POINT('Ctrl Pts',(3.22528263699994,11.6,-9.91983020100001));
#160936=CARTESIAN_POINT('Ctrl Pts',(3.22587010199994,15.2,-9.92104805800001));
#160937=CARTESIAN_POINT('Ctrl Pts',(3.22587010199994,11.6,-9.92104805800001));
#160938=CARTESIAN_POINT('Ctrl Pts',(3.22646240999994,15.2,-9.92227294400001));
#160939=CARTESIAN_POINT('Ctrl Pts',(3.22646240999994,11.6,-9.92227294400001));
#160940=CARTESIAN_POINT('Ctrl Pts',(3.22705956599994,15.2,-9.92350483200001));
#160941=CARTESIAN_POINT('Ctrl Pts',(3.22705956599994,11.6,-9.92350483200001));
#160942=CARTESIAN_POINT('Ctrl Pts',(3.22766157399994,15.2,-9.92474369700002));
#160943=CARTESIAN_POINT('Ctrl Pts',(3.22766157399994,11.6,-9.92474369700002));
#160944=CARTESIAN_POINT('Ctrl Pts',(3.22826843899994,15.2,-9.92598951400001));
#160945=CARTESIAN_POINT('Ctrl Pts',(3.22826843899994,11.6,-9.92598951400001));
#160946=CARTESIAN_POINT('Ctrl Pts',(3.22888016499994,15.2,-9.92724225700002));
#160947=CARTESIAN_POINT('Ctrl Pts',(3.22888016499994,11.6,-9.92724225700002));
#160948=CARTESIAN_POINT('Ctrl Pts',(3.22949675499994,15.2,-9.92850190100001));
#160949=CARTESIAN_POINT('Ctrl Pts',(3.22949675499994,11.6,-9.92850190100001));
#160950=CARTESIAN_POINT('Ctrl Pts',(3.23011821499994,15.2,-9.92976841900001));
#160951=CARTESIAN_POINT('Ctrl Pts',(3.23011821499994,11.6,-9.92976841900001));
#160952=CARTESIAN_POINT('Ctrl Pts',(3.23074454799994,15.2,-9.93104178700001));
#160953=CARTESIAN_POINT('Ctrl Pts',(3.23074454799994,11.6,-9.93104178700001));
#160954=CARTESIAN_POINT('Ctrl Pts',(3.23137575799994,15.2,-9.93232198200001));
#160955=CARTESIAN_POINT('Ctrl Pts',(3.23137575799994,11.6,-9.93232198200001));
#160956=CARTESIAN_POINT('Ctrl Pts',(3.23201184999995,15.2,-9.93360897500001));
#160957=CARTESIAN_POINT('Ctrl Pts',(3.23201184999995,11.6,-9.93360897500001));
#160958=CARTESIAN_POINT('Ctrl Pts',(3.23265282699994,15.2,-9.93490274500001));
#160959=CARTESIAN_POINT('Ctrl Pts',(3.23265282699994,11.6,-9.93490274500001));
#160960=CARTESIAN_POINT('Ctrl Pts',(3.23329869199994,15.2,-9.93620326500001));
#160961=CARTESIAN_POINT('Ctrl Pts',(3.23329869199994,11.6,-9.93620326500001));
#160962=CARTESIAN_POINT('Ctrl Pts',(3.23394945199994,15.2,-9.93751051000001));
#160963=CARTESIAN_POINT('Ctrl Pts',(3.23394945199994,11.6,-9.93751051000001));
#160964=CARTESIAN_POINT('Ctrl Pts',(3.23460510899995,15.2,-9.93882445600001));
#160965=CARTESIAN_POINT('Ctrl Pts',(3.23460510899995,11.6,-9.93882445600001));
#160966=CARTESIAN_POINT('Ctrl Pts',(3.23526566599994,15.2,-9.94014508000001));
#160967=CARTESIAN_POINT('Ctrl Pts',(3.23526566599994,11.6,-9.94014508000001));
#160968=CARTESIAN_POINT('Ctrl Pts',(3.23593112999994,15.2,-9.94147235600001));
#160969=CARTESIAN_POINT('Ctrl Pts',(3.23593112999994,11.6,-9.94147235600001));
#160970=CARTESIAN_POINT('Ctrl Pts',(3.23660150199995,15.2,-9.94280625900001));
#160971=CARTESIAN_POINT('Ctrl Pts',(3.23660150199995,11.6,-9.94280625900001));
#160972=CARTESIAN_POINT('Ctrl Pts',(3.23727678699994,15.2,-9.94414676800002));
#160973=CARTESIAN_POINT('Ctrl Pts',(3.23727678699994,11.6,-9.94414676800002));
#160974=CARTESIAN_POINT('Ctrl Pts',(3.23795698799994,15.2,-9.94549385500001));
#160975=CARTESIAN_POINT('Ctrl Pts',(3.23795698799994,11.6,-9.94549385500001));
#160976=CARTESIAN_POINT('Ctrl Pts',(3.23864210899994,15.2,-9.94684749900001));
#160977=CARTESIAN_POINT('Ctrl Pts',(3.23864210899994,11.6,-9.94684749900001));
#160978=CARTESIAN_POINT('Ctrl Pts',(3.23933215499994,15.2,-9.94820767400001));
#160979=CARTESIAN_POINT('Ctrl Pts',(3.23933215499994,11.6,-9.94820767400001));
#160980=CARTESIAN_POINT('Ctrl Pts',(3.24002712899994,15.2,-9.94957435800002));
#160981=CARTESIAN_POINT('Ctrl Pts',(3.24002712899994,11.6,-9.94957435800002));
#160982=CARTESIAN_POINT('Ctrl Pts',(3.24072703299994,15.2,-9.95094752600002));
#160983=CARTESIAN_POINT('Ctrl Pts',(3.24072703299994,11.6,-9.95094752600002));
#160984=CARTESIAN_POINT('Ctrl Pts',(3.24143187299994,15.2,-9.95232715500001));
#160985=CARTESIAN_POINT('Ctrl Pts',(3.24143187299994,11.6,-9.95232715500001));
#160986=CARTESIAN_POINT('Ctrl Pts',(3.24214165199994,15.2,-9.95371322200001));
#160987=CARTESIAN_POINT('Ctrl Pts',(3.24214165199994,11.6,-9.95371322200001));
#160988=CARTESIAN_POINT('Ctrl Pts',(3.24285637299994,15.2,-9.95510570200001));
#160989=CARTESIAN_POINT('Ctrl Pts',(3.24285637299994,11.6,-9.95510570200001));
#160990=CARTESIAN_POINT('Ctrl Pts',(3.24357603899994,15.2,-9.95650457300002));
#160991=CARTESIAN_POINT('Ctrl Pts',(3.24357603899994,11.6,-9.95650457300002));
#160992=CARTESIAN_POINT('Ctrl Pts',(3.24430065599994,15.2,-9.95790981100001));
#160993=CARTESIAN_POINT('Ctrl Pts',(3.24430065599994,11.6,-9.95790981100001));
#160994=CARTESIAN_POINT('Ctrl Pts',(3.24503022499994,15.2,-9.95932139400001));
#160995=CARTESIAN_POINT('Ctrl Pts',(3.24503022499994,11.6,-9.95932139400001));
#160996=CARTESIAN_POINT('Ctrl Pts',(3.24576475099994,15.2,-9.96073929700001));
#160997=CARTESIAN_POINT('Ctrl Pts',(3.24576475099994,11.6,-9.96073929700001));
#160998=CARTESIAN_POINT('Ctrl Pts',(3.24650423699994,15.2,-9.96216349800001));
#160999=CARTESIAN_POINT('Ctrl Pts',(3.24650423699994,11.6,-9.96216349800001));
#161000=CARTESIAN_POINT('Ctrl Pts',(3.24724868499994,15.2,-9.96359397500001));
#161001=CARTESIAN_POINT('Ctrl Pts',(3.24724868499994,11.6,-9.96359397500001));
#161002=CARTESIAN_POINT('Ctrl Pts',(3.24799810099994,15.2,-9.96503070400001));
#161003=CARTESIAN_POINT('Ctrl Pts',(3.24799810099994,11.6,-9.96503070400001));
#161004=CARTESIAN_POINT('Ctrl Pts',(3.24875248699994,15.2,-9.96647366400001));
#161005=CARTESIAN_POINT('Ctrl Pts',(3.24875248699994,11.6,-9.96647366400001));
#161006=CARTESIAN_POINT('Ctrl Pts',(3.24951184599994,15.2,-9.96792282900001));
#161007=CARTESIAN_POINT('Ctrl Pts',(3.24951184599994,11.6,-9.96792282900001));
#161008=CARTESIAN_POINT('Ctrl Pts',(3.25027618199994,15.2,-9.96937818000001));
#161009=CARTESIAN_POINT('Ctrl Pts',(3.25027618199994,11.6,-9.96937818000001));
#161010=CARTESIAN_POINT('Ctrl Pts',(3.25104549799994,15.2,-9.97083969300001));
#161011=CARTESIAN_POINT('Ctrl Pts',(3.25104549799994,11.6,-9.97083969300001));
#161012=CARTESIAN_POINT('Ctrl Pts',(3.25181979799994,15.2,-9.97230734500001));
#161013=CARTESIAN_POINT('Ctrl Pts',(3.25181979799994,11.6,-9.97230734500001));
#161014=CARTESIAN_POINT('Ctrl Pts',(3.25259908499994,15.2,-9.97378111500001));
#161015=CARTESIAN_POINT('Ctrl Pts',(3.25259908499994,11.6,-9.97378111500001));
#161016=CARTESIAN_POINT('Ctrl Pts',(3.25338336099994,15.2,-9.97526098000001));
#161017=CARTESIAN_POINT('Ctrl Pts',(3.25338336099994,11.6,-9.97526098000001));
#161018=CARTESIAN_POINT('Ctrl Pts',(3.25417263099995,15.2,-9.97674691700001));
#161019=CARTESIAN_POINT('Ctrl Pts',(3.25417263099995,11.6,-9.97674691700001));
#161020=CARTESIAN_POINT('Ctrl Pts',(3.25496689699994,15.2,-9.97823890700001));
#161021=CARTESIAN_POINT('Ctrl Pts',(3.25496689699994,11.6,-9.97823890700001));
#161022=CARTESIAN_POINT('Ctrl Pts',(3.25576616299994,15.2,-9.97973692400001));
#161023=CARTESIAN_POINT('Ctrl Pts',(3.25576616299994,11.6,-9.97973692400001));
#161024=CARTESIAN_POINT('Ctrl Pts',(3.25657042999994,15.2,-9.98124094900001));
#161025=CARTESIAN_POINT('Ctrl Pts',(3.25657042999994,11.6,-9.98124094900001));
#161026=CARTESIAN_POINT('Ctrl Pts',(3.25737970399994,15.2,-9.98275096000001));
#161027=CARTESIAN_POINT('Ctrl Pts',(3.25737970399994,11.6,-9.98275096000001));
#161028=CARTESIAN_POINT('Ctrl Pts',(3.25819398599994,15.2,-9.98426693500001));
#161029=CARTESIAN_POINT('Ctrl Pts',(3.25819398599994,11.6,-9.98426693500001));
#161030=CARTESIAN_POINT('Ctrl Pts',(3.25901327999994,15.2,-9.98578885000001));
#161031=CARTESIAN_POINT('Ctrl Pts',(3.25901327999994,11.6,-9.98578885000001));
#161032=CARTESIAN_POINT('Ctrl Pts',(3.25983758999994,15.2,-9.98731668600001));
#161033=CARTESIAN_POINT('Ctrl Pts',(3.25983758999994,11.6,-9.98731668600001));
#161034=CARTESIAN_POINT('Ctrl Pts',(3.26066691699994,15.2,-9.98885042200001));
#161035=CARTESIAN_POINT('Ctrl Pts',(3.26066691699994,11.6,-9.98885042200001));
#161036=CARTESIAN_POINT('Ctrl Pts',(3.26150126499994,15.2,-9.99039003500001));
#161037=CARTESIAN_POINT('Ctrl Pts',(3.26150126499994,11.6,-9.99039003500001));
#161038=CARTESIAN_POINT('Ctrl Pts',(3.26234063699995,15.2,-9.99193550400001));
#161039=CARTESIAN_POINT('Ctrl Pts',(3.26234063699995,11.6,-9.99193550400001));
#161040=CARTESIAN_POINT('Ctrl Pts',(3.26318503599994,15.2,-9.99348680800001));
#161041=CARTESIAN_POINT('Ctrl Pts',(3.26318503599994,11.6,-9.99348680800001));
#161042=CARTESIAN_POINT('Ctrl Pts',(3.26403446499994,15.2,-9.99504392600001));
#161043=CARTESIAN_POINT('Ctrl Pts',(3.26403446499994,11.6,-9.99504392600001));
#161044=CARTESIAN_POINT('Ctrl Pts',(3.26488892599994,15.2,-9.99660683600001));
#161045=CARTESIAN_POINT('Ctrl Pts',(3.26488892599994,11.6,-9.99660683600001));
#161046=CARTESIAN_POINT('Ctrl Pts',(3.26574842199994,15.2,-9.99817551900001));
#161047=CARTESIAN_POINT('Ctrl Pts',(3.26574842199994,11.6,-9.99817551900001));
#161048=CARTESIAN_POINT('Ctrl Pts',(3.26661295799994,15.2,-9.99974995100001));
#161049=CARTESIAN_POINT('Ctrl Pts',(3.26661295799994,11.6,-9.99974995100001));
#161050=CARTESIAN_POINT('Ctrl Pts',(3.26748253399994,15.2,-10.001330114));
#161051=CARTESIAN_POINT('Ctrl Pts',(3.26748253399994,11.6,-10.001330114));
#161052=CARTESIAN_POINT('Ctrl Pts',(3.26835715399994,15.2,-10.002915985));
#161053=CARTESIAN_POINT('Ctrl Pts',(3.26835715399994,11.6,-10.002915985));
#161054=CARTESIAN_POINT('Ctrl Pts',(3.26923682099994,15.2,-10.004507545));
#161055=CARTESIAN_POINT('Ctrl Pts',(3.26923682099994,11.6,-10.004507545));
#161056=CARTESIAN_POINT('Ctrl Pts',(3.27012153799994,15.2,-10.006104772));
#161057=CARTESIAN_POINT('Ctrl Pts',(3.27012153799994,11.6,-10.006104772));
#161058=CARTESIAN_POINT('Ctrl Pts',(3.27101130699994,15.2,-10.007707647));
#161059=CARTESIAN_POINT('Ctrl Pts',(3.27101130699994,11.6,-10.007707647));
#161060=CARTESIAN_POINT('Ctrl Pts',(3.27190612999994,15.2,-10.009316148));
#161061=CARTESIAN_POINT('Ctrl Pts',(3.27190612999994,11.6,-10.009316148));
#161062=CARTESIAN_POINT('Ctrl Pts',(3.27280601099994,15.2,-10.010930254));
#161063=CARTESIAN_POINT('Ctrl Pts',(3.27280601099994,11.6,-10.010930254));
#161064=CARTESIAN_POINT('Ctrl Pts',(3.27371095399994,15.2,-10.012549947));
#161065=CARTESIAN_POINT('Ctrl Pts',(3.27371095399994,11.6,-10.012549947));
#161066=CARTESIAN_POINT('Ctrl Pts',(3.27462095799994,15.2,-10.014175204));
#161067=CARTESIAN_POINT('Ctrl Pts',(3.27462095799994,11.6,-10.014175204));
#161068=CARTESIAN_POINT('Ctrl Pts',(3.27553602799994,15.2,-10.015806007));
#161069=CARTESIAN_POINT('Ctrl Pts',(3.27553602799994,11.6,-10.015806007));
#161070=CARTESIAN_POINT('Ctrl Pts',(3.27645616799995,15.2,-10.017442335));
#161071=CARTESIAN_POINT('Ctrl Pts',(3.27645616799995,11.6,-10.017442335));
#161072=CARTESIAN_POINT('Ctrl Pts',(3.27738137599995,15.2,-10.019084168));
#161073=CARTESIAN_POINT('Ctrl Pts',(3.27738137599995,11.6,-10.019084168));
#161074=CARTESIAN_POINT('Ctrl Pts',(3.27831165899994,15.2,-10.020731486));
#161075=CARTESIAN_POINT('Ctrl Pts',(3.27831165899994,11.6,-10.020731486));
#161076=CARTESIAN_POINT('Ctrl Pts',(3.27924701799994,15.2,-10.022384268));
#161077=CARTESIAN_POINT('Ctrl Pts',(3.27924701799994,11.6,-10.022384268));
#161078=CARTESIAN_POINT('Ctrl Pts',(3.28018745599994,15.2,-10.024042495));
#161079=CARTESIAN_POINT('Ctrl Pts',(3.28018745599994,11.6,-10.024042495));
#161080=CARTESIAN_POINT('Ctrl Pts',(3.28113297399995,15.2,-10.025706148));
#161081=CARTESIAN_POINT('Ctrl Pts',(3.28113297399995,11.6,-10.025706148));
#161082=CARTESIAN_POINT('Ctrl Pts',(3.28208357499994,15.2,-10.027375206));
#161083=CARTESIAN_POINT('Ctrl Pts',(3.28208357499994,11.6,-10.027375206));
#161084=CARTESIAN_POINT('Ctrl Pts',(3.28303926199994,15.2,-10.02904965));
#161085=CARTESIAN_POINT('Ctrl Pts',(3.28303926199994,11.6,-10.02904965));
#161086=CARTESIAN_POINT('Ctrl Pts',(3.28400003899994,15.2,-10.03072946));
#161087=CARTESIAN_POINT('Ctrl Pts',(3.28400003899994,11.6,-10.03072946));
#161088=CARTESIAN_POINT('Ctrl Pts',(3.28496590599994,15.2,-10.032414616));
#161089=CARTESIAN_POINT('Ctrl Pts',(3.28496590599994,11.6,-10.032414616));
#161090=CARTESIAN_POINT('Ctrl Pts',(3.28593686499994,15.2,-10.0341051));
#161091=CARTESIAN_POINT('Ctrl Pts',(3.28593686499994,11.6,-10.0341051));
#161092=CARTESIAN_POINT('Ctrl Pts',(3.28691291999994,15.2,-10.035800892));
#161093=CARTESIAN_POINT('Ctrl Pts',(3.28691291999994,11.6,-10.035800892));
#161094=CARTESIAN_POINT('Ctrl Pts',(3.28789407299994,15.2,-10.037501971));
#161095=CARTESIAN_POINT('Ctrl Pts',(3.28789407299994,11.6,-10.037501971));
#161096=CARTESIAN_POINT('Ctrl Pts',(3.28888032599994,15.2,-10.039208319));
#161097=CARTESIAN_POINT('Ctrl Pts',(3.28888032599994,11.6,-10.039208319));
#161098=CARTESIAN_POINT('Ctrl Pts',(3.28987168199995,15.2,-10.040919917));
#161099=CARTESIAN_POINT('Ctrl Pts',(3.28987168199995,11.6,-10.040919917));
#161100=CARTESIAN_POINT('Ctrl Pts',(3.29086814199994,15.2,-10.042636746));
#161101=CARTESIAN_POINT('Ctrl Pts',(3.29086814199994,11.6,-10.042636746));
#161102=CARTESIAN_POINT('Ctrl Pts',(3.29186971099994,15.2,-10.044358787));
#161103=CARTESIAN_POINT('Ctrl Pts',(3.29186971099994,11.6,-10.044358787));
#161104=CARTESIAN_POINT('Ctrl Pts',(3.29287638699994,15.2,-10.04608602));
#161105=CARTESIAN_POINT('Ctrl Pts',(3.29287638699994,11.6,-10.04608602));
#161106=CARTESIAN_POINT('Ctrl Pts',(3.29388817699994,15.2,-10.047818426));
#161107=CARTESIAN_POINT('Ctrl Pts',(3.29388817699994,11.6,-10.047818426));
#161108=CARTESIAN_POINT('Ctrl Pts',(3.29490507899994,15.2,-10.049555987));
#161109=CARTESIAN_POINT('Ctrl Pts',(3.29490507899994,11.6,-10.049555987));
#161110=CARTESIAN_POINT('Ctrl Pts',(3.29592709799994,15.2,-10.051298684));
#161111=CARTESIAN_POINT('Ctrl Pts',(3.29592709799994,11.6,-10.051298684));
#161112=CARTESIAN_POINT('Ctrl Pts',(3.29695423399994,15.2,-10.053046497));
#161113=CARTESIAN_POINT('Ctrl Pts',(3.29695423399994,11.6,-10.053046497));
#161114=CARTESIAN_POINT('Ctrl Pts',(3.29798649099994,15.2,-10.054799409));
#161115=CARTESIAN_POINT('Ctrl Pts',(3.29798649099994,11.6,-10.054799409));
#161116=CARTESIAN_POINT('Ctrl Pts',(3.29902387099994,15.2,-10.0565574));
#161117=CARTESIAN_POINT('Ctrl Pts',(3.29902387099994,11.6,-10.0565574));
#161118=CARTESIAN_POINT('Ctrl Pts',(3.30006637499995,15.2,-10.058320452));
#161119=CARTESIAN_POINT('Ctrl Pts',(3.30006637499995,11.6,-10.058320452));
#161120=CARTESIAN_POINT('Ctrl Pts',(3.30111400599994,15.2,-10.060088546));
#161121=CARTESIAN_POINT('Ctrl Pts',(3.30111400599994,11.6,-10.060088546));
#161122=CARTESIAN_POINT('Ctrl Pts',(3.30216676499994,15.2,-10.061861665));
#161123=CARTESIAN_POINT('Ctrl Pts',(3.30216676499994,11.6,-10.061861665));
#161124=CARTESIAN_POINT('Ctrl Pts',(3.30322465599994,15.2,-10.063639788));
#161125=CARTESIAN_POINT('Ctrl Pts',(3.30322465599994,11.6,-10.063639788));
#161126=CARTESIAN_POINT('Ctrl Pts',(3.30428767999994,15.2,-10.065422899));
#161127=CARTESIAN_POINT('Ctrl Pts',(3.30428767999994,11.6,-10.065422899));
#161128=CARTESIAN_POINT('Ctrl Pts',(3.30535583799994,15.2,-10.067210978));
#161129=CARTESIAN_POINT('Ctrl Pts',(3.30535583799994,11.6,-10.067210978));
#161130=CARTESIAN_POINT('Ctrl Pts',(3.30642913399994,15.2,-10.069004008));
#161131=CARTESIAN_POINT('Ctrl Pts',(3.30642913399994,11.6,-10.069004008));
#161132=CARTESIAN_POINT('Ctrl Pts',(3.30750756699994,15.2,-10.070801971));
#161133=CARTESIAN_POINT('Ctrl Pts',(3.30750756699994,11.6,-10.070801971));
#161134=CARTESIAN_POINT('Ctrl Pts',(3.30859114299995,15.2,-10.072604847));
#161135=CARTESIAN_POINT('Ctrl Pts',(3.30859114299995,11.6,-10.072604847));
#161136=CARTESIAN_POINT('Ctrl Pts',(3.30967986099994,15.2,-10.074412619));
#161137=CARTESIAN_POINT('Ctrl Pts',(3.30967986099994,11.6,-10.074412619));
#161138=CARTESIAN_POINT('Ctrl Pts',(3.31077372499994,15.2,-10.07622527));
#161139=CARTESIAN_POINT('Ctrl Pts',(3.31077372499994,11.6,-10.07622527));
#161140=CARTESIAN_POINT('Ctrl Pts',(3.31187273499994,15.2,-10.07804278));
#161141=CARTESIAN_POINT('Ctrl Pts',(3.31187273499994,11.6,-10.07804278));
#161142=CARTESIAN_POINT('Ctrl Pts',(3.31297689299995,15.2,-10.079865133));
#161143=CARTESIAN_POINT('Ctrl Pts',(3.31297689299995,11.6,-10.079865133));
#161144=CARTESIAN_POINT('Ctrl Pts',(3.31408620199994,15.2,-10.081692309));
#161145=CARTESIAN_POINT('Ctrl Pts',(3.31408620199994,11.6,-10.081692309));
#161146=CARTESIAN_POINT('Ctrl Pts',(3.31520066299994,15.2,-10.083524293));
#161147=CARTESIAN_POINT('Ctrl Pts',(3.31520066299994,11.6,-10.083524293));
#161148=CARTESIAN_POINT('Ctrl Pts',(3.31632027899994,15.2,-10.085361064));
#161149=CARTESIAN_POINT('Ctrl Pts',(3.31632027899994,11.6,-10.085361064));
#161150=CARTESIAN_POINT('Ctrl Pts',(3.31744505099994,15.2,-10.087202608));
#161151=CARTESIAN_POINT('Ctrl Pts',(3.31744505099994,11.6,-10.087202608));
#161152=CARTESIAN_POINT('Ctrl Pts',(3.31857498099994,15.2,-10.089048904));
#161153=CARTESIAN_POINT('Ctrl Pts',(3.31857498099994,11.6,-10.089048904));
#161154=CARTESIAN_POINT('Ctrl Pts',(3.31971006999995,15.2,-10.090899936));
#161155=CARTESIAN_POINT('Ctrl Pts',(3.31971006999995,11.6,-10.090899936));
#161156=CARTESIAN_POINT('Ctrl Pts',(3.32085032099994,15.2,-10.092755686));
#161157=CARTESIAN_POINT('Ctrl Pts',(3.32085032099994,11.6,-10.092755686));
#161158=CARTESIAN_POINT('Ctrl Pts',(3.32199573599994,15.2,-10.094616137));
#161159=CARTESIAN_POINT('Ctrl Pts',(3.32199573599994,11.6,-10.094616137));
#161160=CARTESIAN_POINT('Ctrl Pts',(3.32314631399994,15.2,-10.096481272));
#161161=CARTESIAN_POINT('Ctrl Pts',(3.32314631399994,11.6,-10.096481272));
#161162=CARTESIAN_POINT('Ctrl Pts',(3.32430206099994,15.2,-10.098351072));
#161163=CARTESIAN_POINT('Ctrl Pts',(3.32430206099994,11.6,-10.098351072));
#161164=CARTESIAN_POINT('Ctrl Pts',(3.32546297499994,15.2,-10.100225521));
#161165=CARTESIAN_POINT('Ctrl Pts',(3.32546297499994,11.6,-10.100225521));
#161166=CARTESIAN_POINT('Ctrl Pts',(3.32662905999995,15.2,-10.102104602));
#161167=CARTESIAN_POINT('Ctrl Pts',(3.32662905999995,11.6,-10.102104602));
#161168=CARTESIAN_POINT('Ctrl Pts',(3.32780031599994,15.2,-10.103988296));
#161169=CARTESIAN_POINT('Ctrl Pts',(3.32780031599994,11.6,-10.103988296));
#161170=CARTESIAN_POINT('Ctrl Pts',(3.32897674599994,15.2,-10.105876587));
#161171=CARTESIAN_POINT('Ctrl Pts',(3.32897674599994,11.6,-10.105876587));
#161172=CARTESIAN_POINT('Ctrl Pts',(3.33015835099994,15.2,-10.10776946));
#161173=CARTESIAN_POINT('Ctrl Pts',(3.33015835099994,11.6,-10.10776946));
#161174=CARTESIAN_POINT('Ctrl Pts',(3.33134513299994,15.2,-10.109666894));
#161175=CARTESIAN_POINT('Ctrl Pts',(3.33134513299994,11.6,-10.109666894));
#161176=CARTESIAN_POINT('Ctrl Pts',(3.33253709299994,15.2,-10.111568874));
#161177=CARTESIAN_POINT('Ctrl Pts',(3.33253709299994,11.6,-10.111568874));
#161178=CARTESIAN_POINT('Ctrl Pts',(3.33373423399994,15.2,-10.113475383));
#161179=CARTESIAN_POINT('Ctrl Pts',(3.33373423399994,11.6,-10.113475383));
#161180=CARTESIAN_POINT('Ctrl Pts',(3.33493655499994,15.2,-10.115386404));
#161181=CARTESIAN_POINT('Ctrl Pts',(3.33493655499994,11.6,-10.115386404));
#161182=CARTESIAN_POINT('Ctrl Pts',(3.33614405999994,15.2,-10.117301921));
#161183=CARTESIAN_POINT('Ctrl Pts',(3.33614405999994,11.6,-10.117301921));
#161184=CARTESIAN_POINT('Ctrl Pts',(3.33735674999994,15.2,-10.119221915));
#161185=CARTESIAN_POINT('Ctrl Pts',(3.33735674999994,11.6,-10.119221915));
#161186=CARTESIAN_POINT('Ctrl Pts',(3.33857462499994,15.2,-10.121146371));
#161187=CARTESIAN_POINT('Ctrl Pts',(3.33857462499994,11.6,-10.121146371));
#161188=CARTESIAN_POINT('Ctrl Pts',(3.33979768899995,15.2,-10.123075272));
#161189=CARTESIAN_POINT('Ctrl Pts',(3.33979768899995,11.6,-10.123075272));
#161190=CARTESIAN_POINT('Ctrl Pts',(3.34102594099994,15.2,-10.125008601));
#161191=CARTESIAN_POINT('Ctrl Pts',(3.34102594099994,11.6,-10.125008601));
#161192=CARTESIAN_POINT('Ctrl Pts',(3.34225938399995,15.2,-10.126946341));
#161193=CARTESIAN_POINT('Ctrl Pts',(3.34225938399995,11.6,-10.126946341));
#161194=CARTESIAN_POINT('Ctrl Pts',(3.34349802099994,15.2,-10.128888477));
#161195=CARTESIAN_POINT('Ctrl Pts',(3.34349802099994,11.6,-10.128888477));
#161196=CARTESIAN_POINT('Ctrl Pts',(3.34474184999995,15.2,-10.130834991));
#161197=CARTESIAN_POINT('Ctrl Pts',(3.34474184999995,11.6,-10.130834991));
#161198=CARTESIAN_POINT('Ctrl Pts',(3.34599087399994,15.2,-10.132785867));
#161199=CARTESIAN_POINT('Ctrl Pts',(3.34599087399994,11.6,-10.132785867));
#161200=CARTESIAN_POINT('Ctrl Pts',(3.34724509499994,15.2,-10.134741089));
#161201=CARTESIAN_POINT('Ctrl Pts',(3.34724509499994,11.6,-10.134741089));
#161202=CARTESIAN_POINT('Ctrl Pts',(3.34850451299994,15.2,-10.13670064));
#161203=CARTESIAN_POINT('Ctrl Pts',(3.34850451299994,11.6,-10.13670064));
#161204=CARTESIAN_POINT('Ctrl Pts',(3.34976913199994,15.2,-10.138664504));
#161205=CARTESIAN_POINT('Ctrl Pts',(3.34976913199994,11.6,-10.138664504));
#161206=CARTESIAN_POINT('Ctrl Pts',(3.35103895099994,15.2,-10.140632665));
#161207=CARTESIAN_POINT('Ctrl Pts',(3.35103895099994,11.6,-10.140632665));
#161208=CARTESIAN_POINT('Ctrl Pts',(3.35231397199995,15.2,-10.142605106));
#161209=CARTESIAN_POINT('Ctrl Pts',(3.35231397199995,11.6,-10.142605106));
#161210=CARTESIAN_POINT('Ctrl Pts',(3.35359419599994,15.2,-10.14458181));
#161211=CARTESIAN_POINT('Ctrl Pts',(3.35359419599994,11.6,-10.14458181));
#161212=CARTESIAN_POINT('Ctrl Pts',(3.35487962399994,15.2,-10.146562764));
#161213=CARTESIAN_POINT('Ctrl Pts',(3.35487962399994,11.6,-10.146562764));
#161214=CARTESIAN_POINT('Ctrl Pts',(3.35617025999994,15.2,-10.148547949));
#161215=CARTESIAN_POINT('Ctrl Pts',(3.35617025999994,11.6,-10.148547949));
#161216=CARTESIAN_POINT('Ctrl Pts',(3.35746610199994,15.2,-10.15053735));
#161217=CARTESIAN_POINT('Ctrl Pts',(3.35746610199994,11.6,-10.15053735));
#161218=CARTESIAN_POINT('Ctrl Pts',(3.35876715299994,15.2,-10.152530951));
#161219=CARTESIAN_POINT('Ctrl Pts',(3.35876715299994,11.6,-10.152530951));
#161220=CARTESIAN_POINT('Ctrl Pts',(3.36007341499994,15.2,-10.154528737));
#161221=CARTESIAN_POINT('Ctrl Pts',(3.36007341499994,11.6,-10.154528737));
#161222=CARTESIAN_POINT('Ctrl Pts',(3.36138488699994,15.2,-10.156530691));
#161223=CARTESIAN_POINT('Ctrl Pts',(3.36138488699994,11.6,-10.156530691));
#161224=CARTESIAN_POINT('Ctrl Pts',(3.36270157099994,15.2,-10.158536796));
#161225=CARTESIAN_POINT('Ctrl Pts',(3.36270157099994,11.6,-10.158536796));
#161226=CARTESIAN_POINT('Ctrl Pts',(3.36402346899995,15.2,-10.160547038));
#161227=CARTESIAN_POINT('Ctrl Pts',(3.36402346899995,11.6,-10.160547038));
#161228=CARTESIAN_POINT('Ctrl Pts',(3.36535058199994,15.2,-10.1625614));
#161229=CARTESIAN_POINT('Ctrl Pts',(3.36535058199994,11.6,-10.1625614));
#161230=CARTESIAN_POINT('Ctrl Pts',(3.36668291199994,15.2,-10.164579868));
#161231=CARTESIAN_POINT('Ctrl Pts',(3.36668291199994,11.6,-10.164579868));
#161232=CARTESIAN_POINT('Ctrl Pts',(3.36802045799995,15.2,-10.166602424));
#161233=CARTESIAN_POINT('Ctrl Pts',(3.36802045799995,11.6,-10.166602424));
#161234=CARTESIAN_POINT('Ctrl Pts',(3.36936322299994,15.2,-10.168629055));
#161235=CARTESIAN_POINT('Ctrl Pts',(3.36936322299994,11.6,-10.168629055));
#161236=CARTESIAN_POINT('Ctrl Pts',(3.37071120799994,15.2,-10.170659743));
#161237=CARTESIAN_POINT('Ctrl Pts',(3.37071120799994,11.6,-10.170659743));
#161238=CARTESIAN_POINT('Ctrl Pts',(3.37206441299994,15.2,-10.172694474));
#161239=CARTESIAN_POINT('Ctrl Pts',(3.37206441299994,11.6,-10.172694474));
#161240=CARTESIAN_POINT('Ctrl Pts',(3.37342283999994,15.2,-10.174733232));
#161241=CARTESIAN_POINT('Ctrl Pts',(3.37342283999994,11.6,-10.174733232));
#161242=CARTESIAN_POINT('Ctrl Pts',(3.37478648999994,15.2,-10.176776001));
#161243=CARTESIAN_POINT('Ctrl Pts',(3.37478648999994,11.6,-10.176776001));
#161244=CARTESIAN_POINT('Ctrl Pts',(3.37615536399994,15.2,-10.178822767));
#161245=CARTESIAN_POINT('Ctrl Pts',(3.37615536399994,11.6,-10.178822767));
#161246=CARTESIAN_POINT('Ctrl Pts',(3.37752946399994,15.2,-10.180873512));
#161247=CARTESIAN_POINT('Ctrl Pts',(3.37752946399994,11.6,-10.180873512));
#161248=CARTESIAN_POINT('Ctrl Pts',(3.37890878999994,15.2,-10.182928223));
#161249=CARTESIAN_POINT('Ctrl Pts',(3.37890878999994,11.6,-10.182928223));
#161250=CARTESIAN_POINT('Ctrl Pts',(3.38029334199994,15.2,-10.184986883));
#161251=CARTESIAN_POINT('Ctrl Pts',(3.38029334199994,11.6,-10.184986883));
#161252=CARTESIAN_POINT('Ctrl Pts',(3.38168312399994,15.2,-10.18704948));
#161253=CARTESIAN_POINT('Ctrl Pts',(3.38168312399994,11.6,-10.18704948));
#161254=CARTESIAN_POINT('Ctrl Pts',(3.38307813499994,15.2,-10.189115995));
#161255=CARTESIAN_POINT('Ctrl Pts',(3.38307813499994,11.6,-10.189115995));
#161256=CARTESIAN_POINT('Ctrl Pts',(3.38447837599994,15.2,-10.191186414));
#161257=CARTESIAN_POINT('Ctrl Pts',(3.38447837599994,11.6,-10.191186414));
#161258=CARTESIAN_POINT('Ctrl Pts',(3.38588384799994,15.2,-10.193260724));
#161259=CARTESIAN_POINT('Ctrl Pts',(3.38588384799994,11.6,-10.193260724));
#161260=CARTESIAN_POINT('Ctrl Pts',(3.38729455299994,15.2,-10.195338907));
#161261=CARTESIAN_POINT('Ctrl Pts',(3.38729455299994,11.6,-10.195338907));
#161262=CARTESIAN_POINT('Ctrl Pts',(3.38871049099994,15.2,-10.197420949));
#161263=CARTESIAN_POINT('Ctrl Pts',(3.38871049099994,11.6,-10.197420949));
#161264=CARTESIAN_POINT('Ctrl Pts',(3.39013166399994,15.2,-10.199506834));
#161265=CARTESIAN_POINT('Ctrl Pts',(3.39013166399994,11.6,-10.199506834));
#161266=CARTESIAN_POINT('Ctrl Pts',(3.39155807199994,15.2,-10.201596549));
#161267=CARTESIAN_POINT('Ctrl Pts',(3.39155807199994,11.6,-10.201596549));
#161268=CARTESIAN_POINT('Ctrl Pts',(3.39298971599994,15.2,-10.203690078));
#161269=CARTESIAN_POINT('Ctrl Pts',(3.39298971599994,11.6,-10.203690078));
#161270=CARTESIAN_POINT('Ctrl Pts',(3.39442659799994,15.2,-10.205787407));
#161271=CARTESIAN_POINT('Ctrl Pts',(3.39442659799994,11.6,-10.205787407));
#161272=CARTESIAN_POINT('Ctrl Pts',(3.39586871699994,15.2,-10.20788852));
#161273=CARTESIAN_POINT('Ctrl Pts',(3.39586871699994,11.6,-10.20788852));
#161274=CARTESIAN_POINT('Ctrl Pts',(3.39731607599994,15.2,-10.209993402));
#161275=CARTESIAN_POINT('Ctrl Pts',(3.39731607599994,11.6,-10.209993402));
#161276=CARTESIAN_POINT('Ctrl Pts',(3.39876867499994,15.2,-10.21210204));
#161277=CARTESIAN_POINT('Ctrl Pts',(3.39876867499994,11.6,-10.21210204));
#161278=CARTESIAN_POINT('Ctrl Pts',(3.40022651399994,15.2,-10.214214417));
#161279=CARTESIAN_POINT('Ctrl Pts',(3.40022651399994,11.6,-10.214214417));
#161280=CARTESIAN_POINT('Ctrl Pts',(3.40168959499994,15.2,-10.21633052));
#161281=CARTESIAN_POINT('Ctrl Pts',(3.40168959499994,11.6,-10.21633052));
#161282=CARTESIAN_POINT('Ctrl Pts',(3.40315791799994,15.2,-10.218450334));
#161283=CARTESIAN_POINT('Ctrl Pts',(3.40315791799994,11.6,-10.218450334));
#161284=CARTESIAN_POINT('Ctrl Pts',(3.40463148499994,15.2,-10.220573843));
#161285=CARTESIAN_POINT('Ctrl Pts',(3.40463148499994,11.6,-10.220573843));
#161286=CARTESIAN_POINT('Ctrl Pts',(3.40611029499994,15.2,-10.222701034));
#161287=CARTESIAN_POINT('Ctrl Pts',(3.40611029499994,11.6,-10.222701034));
#161288=CARTESIAN_POINT('Ctrl Pts',(3.40759435099995,15.2,-10.224831893));
#161289=CARTESIAN_POINT('Ctrl Pts',(3.40759435099995,11.6,-10.224831893));
#161290=CARTESIAN_POINT('Ctrl Pts',(3.40908365299994,15.2,-10.226966403));
#161291=CARTESIAN_POINT('Ctrl Pts',(3.40908365299994,11.6,-10.226966403));
#161292=CARTESIAN_POINT('Ctrl Pts',(3.41057820099994,15.2,-10.229104552));
#161293=CARTESIAN_POINT('Ctrl Pts',(3.41057820099994,11.6,-10.229104552));
#161294=CARTESIAN_POINT('Ctrl Pts',(3.41207799599994,15.2,-10.231246323));
#161295=CARTESIAN_POINT('Ctrl Pts',(3.41207799599994,11.6,-10.231246323));
#161296=CARTESIAN_POINT('Ctrl Pts',(3.41358303899994,15.2,-10.233391704));
#161297=CARTESIAN_POINT('Ctrl Pts',(3.41358303899994,11.6,-10.233391704));
#161298=CARTESIAN_POINT('Ctrl Pts',(3.41509333199994,15.2,-10.235540681));
#161299=CARTESIAN_POINT('Ctrl Pts',(3.41509333199994,11.6,-10.235540681));
#161300=CARTESIAN_POINT('Ctrl Pts',(3.41660887299994,15.2,-10.237693237));
#161301=CARTESIAN_POINT('Ctrl Pts',(3.41660887299994,11.6,-10.237693237));
#161302=CARTESIAN_POINT('Ctrl Pts',(3.41812966599994,15.2,-10.239849361));
#161303=CARTESIAN_POINT('Ctrl Pts',(3.41812966599994,11.6,-10.239849361));
#161304=CARTESIAN_POINT('Ctrl Pts',(3.41965570899994,15.2,-10.242009036));
#161305=CARTESIAN_POINT('Ctrl Pts',(3.41965570899994,11.6,-10.242009036));
#161306=CARTESIAN_POINT('Ctrl Pts',(3.42118700299994,15.2,-10.244172248));
#161307=CARTESIAN_POINT('Ctrl Pts',(3.42118700299994,11.6,-10.244172248));
#161308=CARTESIAN_POINT('Ctrl Pts',(3.42272355099994,15.2,-10.246338985));
#161309=CARTESIAN_POINT('Ctrl Pts',(3.42272355099994,11.6,-10.246338985));
#161310=CARTESIAN_POINT('Ctrl Pts',(3.42426535099994,15.2,-10.24850923));
#161311=CARTESIAN_POINT('Ctrl Pts',(3.42426535099994,11.6,-10.24850923));
#161312=CARTESIAN_POINT('Ctrl Pts',(3.42581240499995,15.2,-10.250682971));
#161313=CARTESIAN_POINT('Ctrl Pts',(3.42581240499995,11.6,-10.250682971));
#161314=CARTESIAN_POINT('Ctrl Pts',(3.42736471299995,15.2,-10.252860194));
#161315=CARTESIAN_POINT('Ctrl Pts',(3.42736471299995,11.6,-10.252860194));
#161316=CARTESIAN_POINT('Ctrl Pts',(3.42892227699994,15.2,-10.255040883));
#161317=CARTESIAN_POINT('Ctrl Pts',(3.42892227699994,11.6,-10.255040883));
#161318=CARTESIAN_POINT('Ctrl Pts',(3.43048509499994,15.2,-10.257225027));
#161319=CARTESIAN_POINT('Ctrl Pts',(3.43048509499994,11.6,-10.257225027));
#161320=CARTESIAN_POINT('Ctrl Pts',(3.43205317099994,15.2,-10.259412609));
#161321=CARTESIAN_POINT('Ctrl Pts',(3.43205317099994,11.6,-10.259412609));
#161322=CARTESIAN_POINT('Ctrl Pts',(3.43362650399994,15.2,-10.261603617));
#161323=CARTESIAN_POINT('Ctrl Pts',(3.43362650399994,11.6,-10.261603617));
#161324=CARTESIAN_POINT('Ctrl Pts',(3.43520509299994,15.2,-10.263798037));
#161325=CARTESIAN_POINT('Ctrl Pts',(3.43520509299994,11.6,-10.263798037));
#161326=CARTESIAN_POINT('Ctrl Pts',(3.43678893999994,15.2,-10.265995854));
#161327=CARTESIAN_POINT('Ctrl Pts',(3.43678893999994,11.6,-10.265995854));
#161328=CARTESIAN_POINT('Ctrl Pts',(3.43837804699994,15.2,-10.268197055));
#161329=CARTESIAN_POINT('Ctrl Pts',(3.43837804699994,11.6,-10.268197055));
#161330=CARTESIAN_POINT('Ctrl Pts',(3.43997241199994,15.2,-10.270401626));
#161331=CARTESIAN_POINT('Ctrl Pts',(3.43997241199994,11.6,-10.270401626));
#161332=CARTESIAN_POINT('Ctrl Pts',(3.44157203699994,15.2,-10.272609553));
#161333=CARTESIAN_POINT('Ctrl Pts',(3.44157203699994,11.6,-10.272609553));
#161334=CARTESIAN_POINT('Ctrl Pts',(3.44317692299994,15.2,-10.274820824));
#161335=CARTESIAN_POINT('Ctrl Pts',(3.44317692299994,11.6,-10.274820824));
#161336=CARTESIAN_POINT('Ctrl Pts',(3.44478706899995,15.2,-10.277035423));
#161337=CARTESIAN_POINT('Ctrl Pts',(3.44478706899995,11.6,-10.277035423));
#161338=CARTESIAN_POINT('Ctrl Pts',(3.44640247599994,15.2,-10.279253337));
#161339=CARTESIAN_POINT('Ctrl Pts',(3.44640247599994,11.6,-10.279253337));
#161340=CARTESIAN_POINT('Ctrl Pts',(3.44802314499994,15.2,-10.281474553));
#161341=CARTESIAN_POINT('Ctrl Pts',(3.44802314499994,11.6,-10.281474553));
#161342=CARTESIAN_POINT('Ctrl Pts',(3.44964907799994,15.2,-10.283699057));
#161343=CARTESIAN_POINT('Ctrl Pts',(3.44964907799994,11.6,-10.283699057));
#161344=CARTESIAN_POINT('Ctrl Pts',(3.45128027199994,15.2,-10.285926837));
#161345=CARTESIAN_POINT('Ctrl Pts',(3.45128027199994,11.6,-10.285926837));
#161346=CARTESIAN_POINT('Ctrl Pts',(3.45291672899994,15.2,-10.288157876));
#161347=CARTESIAN_POINT('Ctrl Pts',(3.45291672899994,11.6,-10.288157876));
#161348=CARTESIAN_POINT('Ctrl Pts',(3.45455844999994,15.2,-10.290392164));
#161349=CARTESIAN_POINT('Ctrl Pts',(3.45455844999994,11.6,-10.290392164));
#161350=CARTESIAN_POINT('Ctrl Pts',(3.45620543599995,15.2,-10.292629685));
#161351=CARTESIAN_POINT('Ctrl Pts',(3.45620543599995,11.6,-10.292629685));
#161352=CARTESIAN_POINT('Ctrl Pts',(3.45785768599994,15.2,-10.294870428));
#161353=CARTESIAN_POINT('Ctrl Pts',(3.45785768599994,11.6,-10.294870428));
#161354=CARTESIAN_POINT('Ctrl Pts',(3.45951520099995,15.2,-10.297114378));
#161355=CARTESIAN_POINT('Ctrl Pts',(3.45951520099995,11.6,-10.297114378));
#161356=CARTESIAN_POINT('Ctrl Pts',(3.46117798099994,15.2,-10.299361521));
#161357=CARTESIAN_POINT('Ctrl Pts',(3.46117798099994,11.6,-10.299361521));
#161358=CARTESIAN_POINT('Ctrl Pts',(3.46284602699995,15.2,-10.301611846));
#161359=CARTESIAN_POINT('Ctrl Pts',(3.46284602699995,11.6,-10.301611846));
#161360=CARTESIAN_POINT('Ctrl Pts',(3.46451933999994,15.2,-10.303865339));
#161361=CARTESIAN_POINT('Ctrl Pts',(3.46451933999994,11.6,-10.303865339));
#161362=CARTESIAN_POINT('Ctrl Pts',(3.46619791799994,15.2,-10.306121984));
#161363=CARTESIAN_POINT('Ctrl Pts',(3.46619791799994,11.6,-10.306121984));
#161364=CARTESIAN_POINT('Ctrl Pts',(3.46788176499994,15.2,-10.308381772));
#161365=CARTESIAN_POINT('Ctrl Pts',(3.46788176499994,11.6,-10.308381772));
#161366=CARTESIAN_POINT('Ctrl Pts',(3.46957087699994,15.2,-10.310644687));
#161367=CARTESIAN_POINT('Ctrl Pts',(3.46957087699994,11.6,-10.310644687));
#161368=CARTESIAN_POINT('Ctrl Pts',(3.47126525899994,15.2,-10.312910717));
#161369=CARTESIAN_POINT('Ctrl Pts',(3.47126525899994,11.6,-10.312910717));
#161370=CARTESIAN_POINT('Ctrl Pts',(3.47296490699994,15.2,-10.315179847));
#161371=CARTESIAN_POINT('Ctrl Pts',(3.47296490699994,11.6,-10.315179847));
#161372=CARTESIAN_POINT('Ctrl Pts',(3.47466982399995,15.2,-10.317452067));
#161373=CARTESIAN_POINT('Ctrl Pts',(3.47466982399995,11.6,-10.317452067));
#161374=CARTESIAN_POINT('Ctrl Pts',(3.47638000999994,15.2,-10.319727362));
#161375=CARTESIAN_POINT('Ctrl Pts',(3.47638000999994,11.6,-10.319727362));
#161376=CARTESIAN_POINT('Ctrl Pts',(3.47809546499994,15.2,-10.322005719));
#161377=CARTESIAN_POINT('Ctrl Pts',(3.47809546499994,11.6,-10.322005719));
#161378=CARTESIAN_POINT('Ctrl Pts',(3.47981618899994,15.2,-10.324287126));
#161379=CARTESIAN_POINT('Ctrl Pts',(3.47981618899994,11.6,-10.324287126));
#161380=CARTESIAN_POINT('Ctrl Pts',(3.48154218299995,15.2,-10.326571569));
#161381=CARTESIAN_POINT('Ctrl Pts',(3.48154218299995,11.6,-10.326571569));
#161382=CARTESIAN_POINT('Ctrl Pts',(3.48327344499994,15.2,-10.328859035));
#161383=CARTESIAN_POINT('Ctrl Pts',(3.48327344499994,11.6,-10.328859035));
#161384=CARTESIAN_POINT('Ctrl Pts',(3.48500997899994,15.2,-10.331149511));
#161385=CARTESIAN_POINT('Ctrl Pts',(3.48500997899994,11.6,-10.331149511));
#161386=CARTESIAN_POINT('Ctrl Pts',(3.48675178199994,15.2,-10.333442986));
#161387=CARTESIAN_POINT('Ctrl Pts',(3.48675178199994,11.6,-10.333442986));
#161388=CARTESIAN_POINT('Ctrl Pts',(3.48849885699994,15.2,-10.335739446));
#161389=CARTESIAN_POINT('Ctrl Pts',(3.48849885699994,11.6,-10.335739446));
#161390=CARTESIAN_POINT('Ctrl Pts',(3.49025120099994,15.2,-10.338038877));
#161391=CARTESIAN_POINT('Ctrl Pts',(3.49025120099994,11.6,-10.338038877));
#161392=CARTESIAN_POINT('Ctrl Pts',(3.49200881699995,15.2,-10.340341267));
#161393=CARTESIAN_POINT('Ctrl Pts',(3.49200881699995,11.6,-10.340341267));
#161394=CARTESIAN_POINT('Ctrl Pts',(3.49377170499995,15.2,-10.342646604));
#161395=CARTESIAN_POINT('Ctrl Pts',(3.49377170499995,11.6,-10.342646604));
#161396=CARTESIAN_POINT('Ctrl Pts',(3.49553986299994,15.2,-10.344954875));
#161397=CARTESIAN_POINT('Ctrl Pts',(3.49553986299994,11.6,-10.344954875));
#161398=CARTESIAN_POINT('Ctrl Pts',(3.49731329299994,15.2,-10.347266067));
#161399=CARTESIAN_POINT('Ctrl Pts',(3.49731329299994,11.6,-10.347266067));
#161400=CARTESIAN_POINT('Ctrl Pts',(3.49909199599994,15.2,-10.349580167));
#161401=CARTESIAN_POINT('Ctrl Pts',(3.49909199599994,11.6,-10.349580167));
#161402=CARTESIAN_POINT('Ctrl Pts',(3.50087596999994,15.2,-10.351897163));
#161403=CARTESIAN_POINT('Ctrl Pts',(3.50087596999994,11.6,-10.351897163));
#161404=CARTESIAN_POINT('Ctrl Pts',(3.50266521599994,15.2,-10.354217042));
#161405=CARTESIAN_POINT('Ctrl Pts',(3.50266521599994,11.6,-10.354217042));
#161406=CARTESIAN_POINT('Ctrl Pts',(3.50445973399994,15.2,-10.356539792));
#161407=CARTESIAN_POINT('Ctrl Pts',(3.50445973399994,11.6,-10.356539792));
#161408=CARTESIAN_POINT('Ctrl Pts',(3.50625952499994,15.2,-10.358865399));
#161409=CARTESIAN_POINT('Ctrl Pts',(3.50625952499994,11.6,-10.358865399));
#161410=CARTESIAN_POINT('Ctrl Pts',(3.50806458899994,15.2,-10.361193853));
#161411=CARTESIAN_POINT('Ctrl Pts',(3.50806458899994,11.6,-10.361193853));
#161412=CARTESIAN_POINT('Ctrl Pts',(3.50987492499994,15.2,-10.363525138));
#161413=CARTESIAN_POINT('Ctrl Pts',(3.50987492499994,11.6,-10.363525138));
#161414=CARTESIAN_POINT('Ctrl Pts',(3.51169053399994,15.2,-10.365859245));
#161415=CARTESIAN_POINT('Ctrl Pts',(3.51169053399994,11.6,-10.365859245));
#161416=CARTESIAN_POINT('Ctrl Pts',(3.51351141599994,15.2,-10.36819616));
#161417=CARTESIAN_POINT('Ctrl Pts',(3.51351141599994,11.6,-10.36819616));
#161418=CARTESIAN_POINT('Ctrl Pts',(3.51533757099994,15.2,-10.37053587));
#161419=CARTESIAN_POINT('Ctrl Pts',(3.51533757099994,11.6,-10.37053587));
#161420=CARTESIAN_POINT('Ctrl Pts',(3.51716899799994,15.2,-10.372878365));
#161421=CARTESIAN_POINT('Ctrl Pts',(3.51716899799994,11.6,-10.372878365));
#161422=CARTESIAN_POINT('Ctrl Pts',(3.51900569999994,15.2,-10.375223629));
#161423=CARTESIAN_POINT('Ctrl Pts',(3.51900569999994,11.6,-10.375223629));
#161424=CARTESIAN_POINT('Ctrl Pts',(3.52084767399994,15.2,-10.377571653));
#161425=CARTESIAN_POINT('Ctrl Pts',(3.52084767399994,11.6,-10.377571653));
#161426=CARTESIAN_POINT('Ctrl Pts',(3.52269492199994,15.2,-10.379922422));
#161427=CARTESIAN_POINT('Ctrl Pts',(3.52269492199994,11.6,-10.379922422));
#161428=CARTESIAN_POINT('Ctrl Pts',(3.52454744299994,15.2,-10.382275926));
#161429=CARTESIAN_POINT('Ctrl Pts',(3.52454744299994,11.6,-10.382275926));
#161430=CARTESIAN_POINT('Ctrl Pts',(3.52640523699994,15.2,-10.384632152));
#161431=CARTESIAN_POINT('Ctrl Pts',(3.52640523699994,11.6,-10.384632152));
#161432=CARTESIAN_POINT('Ctrl Pts',(3.52826830499994,15.2,-10.386991088));
#161433=CARTESIAN_POINT('Ctrl Pts',(3.52826830499994,11.6,-10.386991088));
#161434=CARTESIAN_POINT('Ctrl Pts',(3.53013664599994,15.2,-10.38935272));
#161435=CARTESIAN_POINT('Ctrl Pts',(3.53013664599994,11.6,-10.38935272));
#161436=CARTESIAN_POINT('Ctrl Pts',(3.53201025999994,15.2,-10.391717039));
#161437=CARTESIAN_POINT('Ctrl Pts',(3.53201025999994,11.6,-10.391717039));
#161438=CARTESIAN_POINT('Ctrl Pts',(3.53388914899994,15.2,-10.394084031));
#161439=CARTESIAN_POINT('Ctrl Pts',(3.53388914899994,11.6,-10.394084031));
#161440=CARTESIAN_POINT('Ctrl Pts',(3.53577330999994,15.2,-10.396453683));
#161441=CARTESIAN_POINT('Ctrl Pts',(3.53577330999994,11.6,-10.396453683));
#161442=CARTESIAN_POINT('Ctrl Pts',(3.53766274399994,15.2,-10.398825985));
#161443=CARTESIAN_POINT('Ctrl Pts',(3.53766274399994,11.6,-10.398825985));
#161444=CARTESIAN_POINT('Ctrl Pts',(3.53955745299994,15.2,-10.401200923));
#161445=CARTESIAN_POINT('Ctrl Pts',(3.53955745299994,11.6,-10.401200923));
#161446=CARTESIAN_POINT('Ctrl Pts',(3.54145743399994,15.2,-10.403578486));
#161447=CARTESIAN_POINT('Ctrl Pts',(3.54145743399994,11.6,-10.403578486));
#161448=CARTESIAN_POINT('Ctrl Pts',(3.54336268899994,15.2,-10.405958663));
#161449=CARTESIAN_POINT('Ctrl Pts',(3.54336268899994,11.6,-10.405958663));
#161450=CARTESIAN_POINT('Ctrl Pts',(3.54527321699994,15.2,-10.408341441));
#161451=CARTESIAN_POINT('Ctrl Pts',(3.54527321699994,11.6,-10.408341441));
#161452=CARTESIAN_POINT('Ctrl Pts',(3.54718901799994,15.2,-10.410726808));
#161453=CARTESIAN_POINT('Ctrl Pts',(3.54718901799994,11.6,-10.410726808));
#161454=CARTESIAN_POINT('Ctrl Pts',(3.54911009199994,15.2,-10.413114751));
#161455=CARTESIAN_POINT('Ctrl Pts',(3.54911009199994,11.6,-10.413114751));
#161456=CARTESIAN_POINT('Ctrl Pts',(3.55103643899994,15.2,-10.41550526));
#161457=CARTESIAN_POINT('Ctrl Pts',(3.55103643899994,11.6,-10.41550526));
#161458=CARTESIAN_POINT('Ctrl Pts',(3.55296805999994,15.2,-10.417898323));
#161459=CARTESIAN_POINT('Ctrl Pts',(3.55296805999994,11.6,-10.417898323));
#161460=CARTESIAN_POINT('Ctrl Pts',(3.55490495199994,15.2,-10.420293927));
#161461=CARTESIAN_POINT('Ctrl Pts',(3.55490495199994,11.6,-10.420293927));
#161462=CARTESIAN_POINT('Ctrl Pts',(3.55684711799995,15.2,-10.422692061));
#161463=CARTESIAN_POINT('Ctrl Pts',(3.55684711799995,11.6,-10.422692061));
#161464=CARTESIAN_POINT('Ctrl Pts',(3.55879455699994,15.2,-10.425092713));
#161465=CARTESIAN_POINT('Ctrl Pts',(3.55879455699994,11.6,-10.425092713));
#161466=CARTESIAN_POINT('Ctrl Pts',(3.56074726699994,15.2,-10.427495871));
#161467=CARTESIAN_POINT('Ctrl Pts',(3.56074726699994,11.6,-10.427495871));
#161468=CARTESIAN_POINT('Ctrl Pts',(3.56270524999994,15.2,-10.429901524));
#161469=CARTESIAN_POINT('Ctrl Pts',(3.56270524999994,11.6,-10.429901524));
#161470=CARTESIAN_POINT('Ctrl Pts',(3.56466850499995,15.2,-10.432309659));
#161471=CARTESIAN_POINT('Ctrl Pts',(3.56466850499995,11.6,-10.432309659));
#161472=CARTESIAN_POINT('Ctrl Pts',(3.56663703199994,15.2,-10.434720266));
#161473=CARTESIAN_POINT('Ctrl Pts',(3.56663703199994,11.6,-10.434720266));
#161474=CARTESIAN_POINT('Ctrl Pts',(3.56861083099994,15.2,-10.437133332));
#161475=CARTESIAN_POINT('Ctrl Pts',(3.56861083099994,11.6,-10.437133332));
#161476=CARTESIAN_POINT('Ctrl Pts',(3.57058990199994,15.2,-10.439548846));
#161477=CARTESIAN_POINT('Ctrl Pts',(3.57058990199994,11.6,-10.439548846));
#161478=CARTESIAN_POINT('Ctrl Pts',(3.57257424399994,15.2,-10.441966796));
#161479=CARTESIAN_POINT('Ctrl Pts',(3.57257424399994,11.6,-10.441966796));
#161480=CARTESIAN_POINT('Ctrl Pts',(3.57456385699995,15.2,-10.444387171));
#161481=CARTESIAN_POINT('Ctrl Pts',(3.57456385699995,11.6,-10.444387171));
#161482=CARTESIAN_POINT('Ctrl Pts',(3.57655874199994,15.2,-10.446809959));
#161483=CARTESIAN_POINT('Ctrl Pts',(3.57655874199994,11.6,-10.446809959));
#161484=CARTESIAN_POINT('Ctrl Pts',(3.57855889699994,15.2,-10.449235148));
#161485=CARTESIAN_POINT('Ctrl Pts',(3.57855889699994,11.6,-10.449235148));
#161486=CARTESIAN_POINT('Ctrl Pts',(3.58056432299994,15.2,-10.451662727));
#161487=CARTESIAN_POINT('Ctrl Pts',(3.58056432299994,11.6,-10.451662727));
#161488=CARTESIAN_POINT('Ctrl Pts',(3.58257501999994,15.2,-10.454092686));
#161489=CARTESIAN_POINT('Ctrl Pts',(3.58257501999994,11.6,-10.454092686));
#161490=CARTESIAN_POINT('Ctrl Pts',(3.58459098699994,15.2,-10.456525011));
#161491=CARTESIAN_POINT('Ctrl Pts',(3.58459098699994,11.6,-10.456525011));
#161492=CARTESIAN_POINT('Ctrl Pts',(3.58661222399994,15.2,-10.458959692));
#161493=CARTESIAN_POINT('Ctrl Pts',(3.58661222399994,11.6,-10.458959692));
#161494=CARTESIAN_POINT('Ctrl Pts',(3.58863872999994,15.2,-10.461396718));
#161495=CARTESIAN_POINT('Ctrl Pts',(3.58863872999994,11.6,-10.461396718));
#161496=CARTESIAN_POINT('Ctrl Pts',(3.59067050699994,15.2,-10.463836075));
#161497=CARTESIAN_POINT('Ctrl Pts',(3.59067050699994,11.6,-10.463836075));
#161498=CARTESIAN_POINT('Ctrl Pts',(3.59270755199994,15.2,-10.466277755));
#161499=CARTESIAN_POINT('Ctrl Pts',(3.59270755199994,11.6,-10.466277755));
#161500=CARTESIAN_POINT('Ctrl Pts',(3.59474986599994,15.2,-10.468721745));
#161501=CARTESIAN_POINT('Ctrl Pts',(3.59474986599994,11.6,-10.468721745));
#161502=CARTESIAN_POINT('Ctrl Pts',(3.59679744899994,15.2,-10.471168034));
#161503=CARTESIAN_POINT('Ctrl Pts',(3.59679744899994,11.6,-10.471168034));
#161504=CARTESIAN_POINT('Ctrl Pts',(3.59885029999994,15.2,-10.473616611));
#161505=CARTESIAN_POINT('Ctrl Pts',(3.59885029999994,11.6,-10.473616611));
#161506=CARTESIAN_POINT('Ctrl Pts',(3.60090841999994,15.2,-10.476067464));
#161507=CARTESIAN_POINT('Ctrl Pts',(3.60090841999994,11.6,-10.476067464));
#161508=CARTESIAN_POINT('Ctrl Pts',(3.60297180699995,15.2,-10.478520582));
#161509=CARTESIAN_POINT('Ctrl Pts',(3.60297180699995,11.6,-10.478520582));
#161510=CARTESIAN_POINT('Ctrl Pts',(3.60504046199994,15.2,-10.480975954));
#161511=CARTESIAN_POINT('Ctrl Pts',(3.60504046199994,11.6,-10.480975954));
#161512=CARTESIAN_POINT('Ctrl Pts',(3.60711438399994,15.2,-10.483433569));
#161513=CARTESIAN_POINT('Ctrl Pts',(3.60711438399994,11.6,-10.483433569));
#161514=CARTESIAN_POINT('Ctrl Pts',(3.60919357199994,15.2,-10.485893415));
#161515=CARTESIAN_POINT('Ctrl Pts',(3.60919357199994,11.6,-10.485893415));
#161516=CARTESIAN_POINT('Ctrl Pts',(3.61127802799994,15.2,-10.488355482));
#161517=CARTESIAN_POINT('Ctrl Pts',(3.61127802799994,11.6,-10.488355482));
#161518=CARTESIAN_POINT('Ctrl Pts',(3.61336774899994,15.2,-10.490819758));
#161519=CARTESIAN_POINT('Ctrl Pts',(3.61336774899994,11.6,-10.490819758));
#161520=CARTESIAN_POINT('Ctrl Pts',(3.61546273499994,15.2,-10.493286233));
#161521=CARTESIAN_POINT('Ctrl Pts',(3.61546273499994,11.6,-10.493286233));
#161522=CARTESIAN_POINT('Ctrl Pts',(3.61756298799994,15.2,-10.495754894));
#161523=CARTESIAN_POINT('Ctrl Pts',(3.61756298799994,11.6,-10.495754894));
#161524=CARTESIAN_POINT('Ctrl Pts',(3.61966850599994,15.2,-10.498225732));
#161525=CARTESIAN_POINT('Ctrl Pts',(3.61966850599994,11.6,-10.498225732));
#161526=CARTESIAN_POINT('Ctrl Pts',(3.62177928799994,15.2,-10.500698735));
#161527=CARTESIAN_POINT('Ctrl Pts',(3.62177928799994,11.6,-10.500698735));
#161528=CARTESIAN_POINT('Ctrl Pts',(3.62389533499994,15.2,-10.503173891));
#161529=CARTESIAN_POINT('Ctrl Pts',(3.62389533499994,11.6,-10.503173891));
#161530=CARTESIAN_POINT('Ctrl Pts',(3.62601664499994,15.2,-10.505651191));
#161531=CARTESIAN_POINT('Ctrl Pts',(3.62601664499994,11.6,-10.505651191));
#161532=CARTESIAN_POINT('Ctrl Pts',(3.62814321899994,15.2,-10.508130623));
#161533=CARTESIAN_POINT('Ctrl Pts',(3.62814321899994,11.6,-10.508130623));
#161534=CARTESIAN_POINT('Ctrl Pts',(3.63027505499994,15.2,-10.510612176));
#161535=CARTESIAN_POINT('Ctrl Pts',(3.63027505499994,11.6,-10.510612176));
#161536=CARTESIAN_POINT('Ctrl Pts',(3.63241215499994,15.2,-10.513095839));
#161537=CARTESIAN_POINT('Ctrl Pts',(3.63241215499994,11.6,-10.513095839));
#161538=CARTESIAN_POINT('Ctrl Pts',(3.63455451699994,15.2,-10.515581602));
#161539=CARTESIAN_POINT('Ctrl Pts',(3.63455451699994,11.6,-10.515581602));
#161540=CARTESIAN_POINT('Ctrl Pts',(3.63670213999994,15.2,-10.518069453));
#161541=CARTESIAN_POINT('Ctrl Pts',(3.63670213999994,11.6,-10.518069453));
#161542=CARTESIAN_POINT('Ctrl Pts',(3.63885502399994,15.2,-10.520559382));
#161543=CARTESIAN_POINT('Ctrl Pts',(3.63885502399994,11.6,-10.520559382));
#161544=CARTESIAN_POINT('Ctrl Pts',(3.64101316999994,15.2,-10.523051377));
#161545=CARTESIAN_POINT('Ctrl Pts',(3.64101316999994,11.6,-10.523051377));
#161546=CARTESIAN_POINT('Ctrl Pts',(3.64317657699994,15.2,-10.525545429));
#161547=CARTESIAN_POINT('Ctrl Pts',(3.64317657699994,11.6,-10.525545429));
#161548=CARTESIAN_POINT('Ctrl Pts',(3.64534524299994,15.2,-10.528041526));
#161549=CARTESIAN_POINT('Ctrl Pts',(3.64534524299994,11.6,-10.528041526));
#161550=CARTESIAN_POINT('Ctrl Pts',(3.64751916799994,15.2,-10.530539657));
#161551=CARTESIAN_POINT('Ctrl Pts',(3.64751916799994,11.6,-10.530539657));
#161552=CARTESIAN_POINT('Ctrl Pts',(3.64969835399994,15.2,-10.533039812));
#161553=CARTESIAN_POINT('Ctrl Pts',(3.64969835399994,11.6,-10.533039812));
#161554=CARTESIAN_POINT('Ctrl Pts',(3.65188279699994,15.2,-10.53554198));
#161555=CARTESIAN_POINT('Ctrl Pts',(3.65188279699994,11.6,-10.53554198));
#161556=CARTESIAN_POINT('Ctrl Pts',(3.65407249799994,15.2,-10.538046151));
#161557=CARTESIAN_POINT('Ctrl Pts',(3.65407249799994,11.6,-10.538046151));
#161558=CARTESIAN_POINT('Ctrl Pts',(3.65626745699994,15.2,-10.540552312));
#161559=CARTESIAN_POINT('Ctrl Pts',(3.65626745699994,11.6,-10.540552312));
#161560=CARTESIAN_POINT('Ctrl Pts',(3.65846767199994,15.2,-10.543060456));
#161561=CARTESIAN_POINT('Ctrl Pts',(3.65846767199994,11.6,-10.543060456));
#161562=CARTESIAN_POINT('Ctrl Pts',(3.66067314499994,15.2,-10.545570569));
#161563=CARTESIAN_POINT('Ctrl Pts',(3.66067314499994,11.6,-10.545570569));
#161564=CARTESIAN_POINT('Ctrl Pts',(3.66288387299994,15.2,-10.548082642));
#161565=CARTESIAN_POINT('Ctrl Pts',(3.66288387299994,11.6,-10.548082642));
#161566=CARTESIAN_POINT('Ctrl Pts',(3.66509985699994,15.2,-10.550596665));
#161567=CARTESIAN_POINT('Ctrl Pts',(3.66509985699994,11.6,-10.550596665));
#161568=CARTESIAN_POINT('Ctrl Pts',(3.66732109599994,15.2,-10.553112626));
#161569=CARTESIAN_POINT('Ctrl Pts',(3.66732109599994,11.6,-10.553112626));
#161570=CARTESIAN_POINT('Ctrl Pts',(3.66954758799994,15.2,-10.555630515));
#161571=CARTESIAN_POINT('Ctrl Pts',(3.66954758799994,11.6,-10.555630515));
#161572=CARTESIAN_POINT('Ctrl Pts',(3.67177933599994,15.2,-10.558150321));
#161573=CARTESIAN_POINT('Ctrl Pts',(3.67177933599994,11.6,-10.558150321));
#161574=CARTESIAN_POINT('Ctrl Pts',(3.67401633599994,15.2,-10.560672035));
#161575=CARTESIAN_POINT('Ctrl Pts',(3.67401633599994,11.6,-10.560672035));
#161576=CARTESIAN_POINT('Ctrl Pts',(3.67625858899994,15.2,-10.563195645));
#161577=CARTESIAN_POINT('Ctrl Pts',(3.67625858899994,11.6,-10.563195645));
#161578=CARTESIAN_POINT('Ctrl Pts',(3.67850609399994,15.2,-10.565721142));
#161579=CARTESIAN_POINT('Ctrl Pts',(3.67850609399994,11.6,-10.565721142));
#161580=CARTESIAN_POINT('Ctrl Pts',(3.68075885099994,15.2,-10.568248513));
#161581=CARTESIAN_POINT('Ctrl Pts',(3.68075885099994,11.6,-10.568248513));
#161582=CARTESIAN_POINT('Ctrl Pts',(3.68301685699994,15.2,-10.57077775));
#161583=CARTESIAN_POINT('Ctrl Pts',(3.68301685699994,11.6,-10.57077775));
#161584=CARTESIAN_POINT('Ctrl Pts',(3.68528011599994,15.2,-10.573308843));
#161585=CARTESIAN_POINT('Ctrl Pts',(3.68528011599994,11.6,-10.573308843));
#161586=CARTESIAN_POINT('Ctrl Pts',(3.68754862299994,15.2,-10.57584178));
#161587=CARTESIAN_POINT('Ctrl Pts',(3.68754862299994,11.6,-10.57584178));
#161588=CARTESIAN_POINT('Ctrl Pts',(3.68982237999994,15.2,-10.578376549));
#161589=CARTESIAN_POINT('Ctrl Pts',(3.68982237999994,11.6,-10.578376549));
#161590=CARTESIAN_POINT('Ctrl Pts',(3.69210138499994,15.2,-10.580913144));
#161591=CARTESIAN_POINT('Ctrl Pts',(3.69210138499994,11.6,-10.580913144));
#161592=CARTESIAN_POINT('Ctrl Pts',(3.69438563799994,15.2,-10.583451551));
#161593=CARTESIAN_POINT('Ctrl Pts',(3.69438563799994,11.6,-10.583451551));
#161594=CARTESIAN_POINT('Ctrl Pts',(3.69667513799994,15.2,-10.585991763));
#161595=CARTESIAN_POINT('Ctrl Pts',(3.69667513799994,11.6,-10.585991763));
#161596=CARTESIAN_POINT('Ctrl Pts',(3.69896988599994,15.2,-10.588533766));
#161597=CARTESIAN_POINT('Ctrl Pts',(3.69896988599994,11.6,-10.588533766));
#161598=CARTESIAN_POINT('Ctrl Pts',(3.70126987899994,15.2,-10.591077552));
#161599=CARTESIAN_POINT('Ctrl Pts',(3.70126987899994,11.6,-10.591077552));
#161600=CARTESIAN_POINT('Ctrl Pts',(3.70357511699994,15.2,-10.593623111));
#161601=CARTESIAN_POINT('Ctrl Pts',(3.70357511699994,11.6,-10.593623111));
#161602=CARTESIAN_POINT('Ctrl Pts',(3.70588559899994,15.2,-10.596170432));
#161603=CARTESIAN_POINT('Ctrl Pts',(3.70588559899994,11.6,-10.596170432));
#161604=CARTESIAN_POINT('Ctrl Pts',(3.70820132699994,15.2,-10.598719505));
#161605=CARTESIAN_POINT('Ctrl Pts',(3.70820132699994,11.6,-10.598719505));
#161606=CARTESIAN_POINT('Ctrl Pts',(3.71052229599994,15.2,-10.601270319));
#161607=CARTESIAN_POINT('Ctrl Pts',(3.71052229599994,11.6,-10.601270319));
#161608=CARTESIAN_POINT('Ctrl Pts',(3.71284850899994,15.2,-10.603822866));
#161609=CARTESIAN_POINT('Ctrl Pts',(3.71284850899994,11.6,-10.603822866));
#161610=CARTESIAN_POINT('Ctrl Pts',(3.71517996399994,15.2,-10.606377133));
#161611=CARTESIAN_POINT('Ctrl Pts',(3.71517996399994,11.6,-10.606377133));
#161612=CARTESIAN_POINT('Ctrl Pts',(3.71751665899994,15.2,-10.608933112));
#161613=CARTESIAN_POINT('Ctrl Pts',(3.71751665899994,11.6,-10.608933112));
#161614=CARTESIAN_POINT('Ctrl Pts',(3.71985859599994,15.2,-10.611490793));
#161615=CARTESIAN_POINT('Ctrl Pts',(3.71985859599994,11.6,-10.611490793));
#161616=CARTESIAN_POINT('Ctrl Pts',(3.72220577199994,15.2,-10.614050164));
#161617=CARTESIAN_POINT('Ctrl Pts',(3.72220577199994,11.6,-10.614050164));
#161618=CARTESIAN_POINT('Ctrl Pts',(3.72455818799994,15.2,-10.616611217));
#161619=CARTESIAN_POINT('Ctrl Pts',(3.72455818799994,11.6,-10.616611217));
#161620=CARTESIAN_POINT('Ctrl Pts',(3.72691584199994,15.2,-10.61917394));
#161621=CARTESIAN_POINT('Ctrl Pts',(3.72691584199994,11.6,-10.61917394));
#161622=CARTESIAN_POINT('Ctrl Pts',(3.72927873299994,15.2,-10.621738325));
#161623=CARTESIAN_POINT('Ctrl Pts',(3.72927873299994,11.6,-10.621738325));
#161624=CARTESIAN_POINT('Ctrl Pts',(3.73164686099994,15.2,-10.62430436));
#161625=CARTESIAN_POINT('Ctrl Pts',(3.73164686099994,11.6,-10.62430436));
#161626=CARTESIAN_POINT('Ctrl Pts',(3.73402022599994,15.2,-10.626872037));
#161627=CARTESIAN_POINT('Ctrl Pts',(3.73402022599994,11.6,-10.626872037));
#161628=CARTESIAN_POINT('Ctrl Pts',(3.73639882499994,15.2,-10.629441346));
#161629=CARTESIAN_POINT('Ctrl Pts',(3.73639882499994,11.6,-10.629441346));
#161630=CARTESIAN_POINT('Ctrl Pts',(3.73878265999994,15.2,-10.632012274));
#161631=CARTESIAN_POINT('Ctrl Pts',(3.73878265999994,11.6,-10.632012274));
#161632=CARTESIAN_POINT('Ctrl Pts',(3.74117172899994,15.2,-10.634584815));
#161633=CARTESIAN_POINT('Ctrl Pts',(3.74117172899994,11.6,-10.634584815));
#161634=CARTESIAN_POINT('Ctrl Pts',(3.74356602999994,15.2,-10.637158956));
#161635=CARTESIAN_POINT('Ctrl Pts',(3.74356602999994,11.6,-10.637158956));
#161636=CARTESIAN_POINT('Ctrl Pts',(3.74596556399994,15.2,-10.63973469));
#161637=CARTESIAN_POINT('Ctrl Pts',(3.74596556399994,11.6,-10.63973469));
#161638=CARTESIAN_POINT('Ctrl Pts',(3.74837032999995,15.2,-10.642312004));
#161639=CARTESIAN_POINT('Ctrl Pts',(3.74837032999995,11.6,-10.642312004));
#161640=CARTESIAN_POINT('Ctrl Pts',(3.75078032599994,15.2,-10.64489089));
#161641=CARTESIAN_POINT('Ctrl Pts',(3.75078032599994,11.6,-10.64489089));
#161642=CARTESIAN_POINT('Ctrl Pts',(3.75319555299995,15.2,-10.647471338));
#161643=CARTESIAN_POINT('Ctrl Pts',(3.75319555299995,11.6,-10.647471338));
#161644=CARTESIAN_POINT('Ctrl Pts',(3.75561600799994,15.2,-10.650053339));
#161645=CARTESIAN_POINT('Ctrl Pts',(3.75561600799994,11.6,-10.650053339));
#161646=CARTESIAN_POINT('Ctrl Pts',(3.75804169099994,15.2,-10.652636882));
#161647=CARTESIAN_POINT('Ctrl Pts',(3.75804169099994,11.6,-10.652636882));
#161648=CARTESIAN_POINT('Ctrl Pts',(3.76047260299994,15.2,-10.655221957));
#161649=CARTESIAN_POINT('Ctrl Pts',(3.76047260299994,11.6,-10.655221957));
#161650=CARTESIAN_POINT('Ctrl Pts',(3.76290874199994,15.2,-10.657808554));
#161651=CARTESIAN_POINT('Ctrl Pts',(3.76290874199994,11.6,-10.657808554));
#161652=CARTESIAN_POINT('Ctrl Pts',(3.76535010599994,15.2,-10.660396666));
#161653=CARTESIAN_POINT('Ctrl Pts',(3.76535010599994,11.6,-10.660396666));
#161654=CARTESIAN_POINT('Ctrl Pts',(3.76779669499994,15.2,-10.66298628));
#161655=CARTESIAN_POINT('Ctrl Pts',(3.76779669499994,11.6,-10.66298628));
#161656=CARTESIAN_POINT('Ctrl Pts',(3.77024850799994,15.2,-10.665577387));
#161657=CARTESIAN_POINT('Ctrl Pts',(3.77024850799994,11.6,-10.665577387));
#161658=CARTESIAN_POINT('Ctrl Pts',(3.77270554499994,15.2,-10.668169979));
#161659=CARTESIAN_POINT('Ctrl Pts',(3.77270554499994,11.6,-10.668169979));
#161660=CARTESIAN_POINT('Ctrl Pts',(3.77516780399994,15.2,-10.670764045));
#161661=CARTESIAN_POINT('Ctrl Pts',(3.77516780399994,11.6,-10.670764045));
#161662=CARTESIAN_POINT('Ctrl Pts',(3.77763528499994,15.2,-10.673359575));
#161663=CARTESIAN_POINT('Ctrl Pts',(3.77763528499994,11.6,-10.673359575));
#161664=CARTESIAN_POINT('Ctrl Pts',(3.78010798799994,15.2,-10.675956561));
#161665=CARTESIAN_POINT('Ctrl Pts',(3.78010798799994,11.6,-10.675956561));
#161666=CARTESIAN_POINT('Ctrl Pts',(3.78258590899994,15.2,-10.678554991));
#161667=CARTESIAN_POINT('Ctrl Pts',(3.78258590899994,11.6,-10.678554991));
#161668=CARTESIAN_POINT('Ctrl Pts',(3.78506904999994,15.2,-10.681154858));
#161669=CARTESIAN_POINT('Ctrl Pts',(3.78506904999994,11.6,-10.681154858));
#161670=CARTESIAN_POINT('Ctrl Pts',(3.78755740999994,15.2,-10.68375615));
#161671=CARTESIAN_POINT('Ctrl Pts',(3.78755740999994,11.6,-10.68375615));
#161672=CARTESIAN_POINT('Ctrl Pts',(3.79005098599994,15.2,-10.686358859));
#161673=CARTESIAN_POINT('Ctrl Pts',(3.79005098599994,11.6,-10.686358859));
#161674=CARTESIAN_POINT('Ctrl Pts',(3.79254977799994,15.2,-10.688962975));
#161675=CARTESIAN_POINT('Ctrl Pts',(3.79254977799994,11.6,-10.688962975));
#161676=CARTESIAN_POINT('Ctrl Pts',(3.79505378699994,15.2,-10.691568489));
#161677=CARTESIAN_POINT('Ctrl Pts',(3.79505378699994,11.6,-10.691568489));
#161678=CARTESIAN_POINT('Ctrl Pts',(3.79756300899994,15.2,-10.69417539));
#161679=CARTESIAN_POINT('Ctrl Pts',(3.79756300899994,11.6,-10.69417539));
#161680=CARTESIAN_POINT('Ctrl Pts',(3.80007744599994,15.2,-10.696783671));
#161681=CARTESIAN_POINT('Ctrl Pts',(3.80007744599994,11.6,-10.696783671));
#161682=CARTESIAN_POINT('Ctrl Pts',(3.80259709499994,15.2,-10.69939332));
#161683=CARTESIAN_POINT('Ctrl Pts',(3.80259709499994,11.6,-10.69939332));
#161684=CARTESIAN_POINT('Ctrl Pts',(3.80512195499994,15.2,-10.702004329));
#161685=CARTESIAN_POINT('Ctrl Pts',(3.80512195499994,11.6,-10.702004329));
#161686=CARTESIAN_POINT('Ctrl Pts',(3.80765202699994,15.2,-10.704616687));
#161687=CARTESIAN_POINT('Ctrl Pts',(3.80765202699994,11.6,-10.704616687));
#161688=CARTESIAN_POINT('Ctrl Pts',(3.81018730899994,15.2,-10.707230387));
#161689=CARTESIAN_POINT('Ctrl Pts',(3.81018730899994,11.6,-10.707230387));
#161690=CARTESIAN_POINT('Ctrl Pts',(3.81272779999994,15.2,-10.709845418));
#161691=CARTESIAN_POINT('Ctrl Pts',(3.81272779999994,11.6,-10.709845418));
#161692=CARTESIAN_POINT('Ctrl Pts',(3.81527349799994,15.2,-10.712461771));
#161693=CARTESIAN_POINT('Ctrl Pts',(3.81527349799994,11.6,-10.712461771));
#161694=CARTESIAN_POINT('Ctrl Pts',(3.81782440399994,15.2,-10.715079437));
#161695=CARTESIAN_POINT('Ctrl Pts',(3.81782440399994,11.6,-10.715079437));
#161696=CARTESIAN_POINT('Ctrl Pts',(3.82038051599995,15.2,-10.717698405));
#161697=CARTESIAN_POINT('Ctrl Pts',(3.82038051599995,11.6,-10.717698405));
#161698=CARTESIAN_POINT('Ctrl Pts',(3.82294183299994,15.2,-10.720318668));
#161699=CARTESIAN_POINT('Ctrl Pts',(3.82294183299994,11.6,-10.720318668));
#161700=CARTESIAN_POINT('Ctrl Pts',(3.82550835399994,15.2,-10.722940215));
#161701=CARTESIAN_POINT('Ctrl Pts',(3.82550835399994,11.6,-10.722940215));
#161702=CARTESIAN_POINT('Ctrl Pts',(3.82808007799994,15.2,-10.725563038));
#161703=CARTESIAN_POINT('Ctrl Pts',(3.82808007799994,11.6,-10.725563038));
#161704=CARTESIAN_POINT('Ctrl Pts',(3.83065700499994,15.2,-10.728187126));
#161705=CARTESIAN_POINT('Ctrl Pts',(3.83065700499994,11.6,-10.728187126));
#161706=CARTESIAN_POINT('Ctrl Pts',(3.83323913199995,15.2,-10.730812471));
#161707=CARTESIAN_POINT('Ctrl Pts',(3.83323913199995,11.6,-10.730812471));
#161708=CARTESIAN_POINT('Ctrl Pts',(3.83582646099994,15.2,-10.733439064));
#161709=CARTESIAN_POINT('Ctrl Pts',(3.83582646099994,11.6,-10.733439064));
#161710=CARTESIAN_POINT('Ctrl Pts',(3.83841898699994,15.2,-10.736066894));
#161711=CARTESIAN_POINT('Ctrl Pts',(3.83841898699994,11.6,-10.736066894));
#161712=CARTESIAN_POINT('Ctrl Pts',(3.84101671199994,15.2,-10.738695953));
#161713=CARTESIAN_POINT('Ctrl Pts',(3.84101671199994,11.6,-10.738695953));
#161714=CARTESIAN_POINT('Ctrl Pts',(3.84361963499994,15.2,-10.741326232));
#161715=CARTESIAN_POINT('Ctrl Pts',(3.84361963499994,11.6,-10.741326232));
#161716=CARTESIAN_POINT('Ctrl Pts',(3.84622775399994,15.2,-10.743957723));
#161717=CARTESIAN_POINT('Ctrl Pts',(3.84622775399994,11.6,-10.743957723));
#161718=CARTESIAN_POINT('Ctrl Pts',(3.84884106699994,15.2,-10.746590413));
#161719=CARTESIAN_POINT('Ctrl Pts',(3.84884106699994,11.6,-10.746590413));
#161720=CARTESIAN_POINT('Ctrl Pts',(3.85145957499994,15.2,-10.749224299));
#161721=CARTESIAN_POINT('Ctrl Pts',(3.85145957499994,11.6,-10.749224299));
#161722=CARTESIAN_POINT('Ctrl Pts',(3.85408327599994,15.2,-10.751859366));
#161723=CARTESIAN_POINT('Ctrl Pts',(3.85408327599994,11.6,-10.751859366));
#161724=CARTESIAN_POINT('Ctrl Pts',(3.85671216899994,15.2,-10.754495609));
#161725=CARTESIAN_POINT('Ctrl Pts',(3.85671216899994,11.6,-10.754495609));
#161726=CARTESIAN_POINT('Ctrl Pts',(3.85934625299994,15.2,-10.757133015));
#161727=CARTESIAN_POINT('Ctrl Pts',(3.85934625299994,11.6,-10.757133015));
#161728=CARTESIAN_POINT('Ctrl Pts',(3.86198552599994,15.2,-10.759771578));
#161729=CARTESIAN_POINT('Ctrl Pts',(3.86198552599994,11.6,-10.759771578));
#161730=CARTESIAN_POINT('Ctrl Pts',(3.86462998899994,15.2,-10.762411286));
#161731=CARTESIAN_POINT('Ctrl Pts',(3.86462998899994,11.6,-10.762411286));
#161732=CARTESIAN_POINT('Ctrl Pts',(3.86727963799994,15.2,-10.765052131));
#161733=CARTESIAN_POINT('Ctrl Pts',(3.86727963799994,11.6,-10.765052131));
#161734=CARTESIAN_POINT('Ctrl Pts',(3.86993447399994,15.2,-10.767694104));
#161735=CARTESIAN_POINT('Ctrl Pts',(3.86993447399994,11.6,-10.767694104));
#161736=CARTESIAN_POINT('Ctrl Pts',(3.87259449699994,15.2,-10.770337195));
#161737=CARTESIAN_POINT('Ctrl Pts',(3.87259449699994,11.6,-10.770337195));
#161738=CARTESIAN_POINT('Ctrl Pts',(3.87525970299994,15.2,-10.772981398));
#161739=CARTESIAN_POINT('Ctrl Pts',(3.87525970299994,11.6,-10.772981398));
#161740=CARTESIAN_POINT('Ctrl Pts',(3.87793009299994,15.2,-10.775626704));
#161741=CARTESIAN_POINT('Ctrl Pts',(3.87793009299994,11.6,-10.775626704));
#161742=CARTESIAN_POINT('Ctrl Pts',(3.88060566599994,15.2,-10.778273105));
#161743=CARTESIAN_POINT('Ctrl Pts',(3.88060566599994,11.6,-10.778273105));
#161744=CARTESIAN_POINT('Ctrl Pts',(3.88328641999994,15.2,-10.780920592));
#161745=CARTESIAN_POINT('Ctrl Pts',(3.88328641999994,11.6,-10.780920592));
#161746=CARTESIAN_POINT('Ctrl Pts',(3.88597235399994,15.2,-10.783569155));
#161747=CARTESIAN_POINT('Ctrl Pts',(3.88597235399994,11.6,-10.783569155));
#161748=CARTESIAN_POINT('Ctrl Pts',(3.88866346799994,15.2,-10.786218787));
#161749=CARTESIAN_POINT('Ctrl Pts',(3.88866346799994,11.6,-10.786218787));
#161750=CARTESIAN_POINT('Ctrl Pts',(3.89135975899995,15.2,-10.788869473));
#161751=CARTESIAN_POINT('Ctrl Pts',(3.89135975899995,11.6,-10.788869473));
#161752=CARTESIAN_POINT('Ctrl Pts',(3.89406122599994,15.2,-10.791521204));
#161753=CARTESIAN_POINT('Ctrl Pts',(3.89406122599994,11.6,-10.791521204));
#161754=CARTESIAN_POINT('Ctrl Pts',(3.89676786899994,15.2,-10.794173967));
#161755=CARTESIAN_POINT('Ctrl Pts',(3.89676786899994,11.6,-10.794173967));
#161756=CARTESIAN_POINT('Ctrl Pts',(3.89947968399994,15.2,-10.796827756));
#161757=CARTESIAN_POINT('Ctrl Pts',(3.89947968399994,11.6,-10.796827756));
#161758=CARTESIAN_POINT('Ctrl Pts',(3.90219667399994,15.2,-10.79948256));
#161759=CARTESIAN_POINT('Ctrl Pts',(3.90219667399994,11.6,-10.79948256));
#161760=CARTESIAN_POINT('Ctrl Pts',(3.90491883499994,15.2,-10.802138374));
#161761=CARTESIAN_POINT('Ctrl Pts',(3.90491883499994,11.6,-10.802138374));
#161762=CARTESIAN_POINT('Ctrl Pts',(3.90764616599994,15.2,-10.804795195));
#161763=CARTESIAN_POINT('Ctrl Pts',(3.90764616599994,11.6,-10.804795195));
#161764=CARTESIAN_POINT('Ctrl Pts',(3.91037866899994,15.2,-10.807453018));
#161765=CARTESIAN_POINT('Ctrl Pts',(3.91037866899994,11.6,-10.807453018));
#161766=CARTESIAN_POINT('Ctrl Pts',(3.91256880799994,15.2,-10.80958008));
#161767=CARTESIAN_POINT('Ctrl Pts',(3.91256880799994,11.6,-10.80958008));
#161768=CARTESIAN_POINT('Ctrl Pts',(3.91421373899994,15.2,-10.811175827));
#161769=CARTESIAN_POINT('Ctrl Pts',(3.91421373899994,11.6,-10.811175827));
#161770=CARTESIAN_POINT('Ctrl Pts',(3.91531139299994,15.2,-10.812239859));
#161771=CARTESIAN_POINT('Ctrl Pts',(3.91531139299994,11.6,-10.812239859));
#161772=CARTESIAN_POINT('Ctrl Pts',(3.91586047899994,15.2,-10.812771925));
#161773=CARTESIAN_POINT('Ctrl Pts',(3.91586047899994,11.6,-10.812771925));
#161774=CARTESIAN_POINT('Ctrl Pts',(3.20199116199994,15.2,-9.86852965800001));
#161775=CARTESIAN_POINT('Ctrl Pts',(3.20268657132788,15.2,-9.87017542455285));
#161776=CARTESIAN_POINT('Ctrl Pts',(3.20340918399116,15.2,-9.87187175340483));
#161777=CARTESIAN_POINT('Ctrl Pts',(3.20415920994276,15.2,-9.8736175032754));
#161778=CARTESIAN_POINT('Ctrl Pts',(3.20491285289861,15.2,-9.87537167203426));
#161779=CARTESIAN_POINT('Ctrl Pts',(3.20569417410877,15.2,-9.87717573863291));
#161780=CARTESIAN_POINT('Ctrl Pts',(3.20650338986158,15.2,-9.87902857766262));
#161781=CARTESIAN_POINT('Ctrl Pts',(3.2073126055409,15.2,-9.88088141652404));
#161782=CARTESIAN_POINT('Ctrl Pts',(3.20814971062299,15.2,-9.8827830280374));
#161783=CARTESIAN_POINT('Ctrl Pts',(3.20901491150822,15.2,-9.88473231696659));
#161784=CARTESIAN_POINT('Ctrl Pts',(3.20988011239345,15.2,-9.88668160589576));
#161785=CARTESIAN_POINT('Ctrl Pts',(3.21077340789157,15.1999999999999,-9.88867857373555));
#161786=CARTESIAN_POINT('Ctrl Pts',(3.21169499165248,15.2,-9.89072215684402));
#161787=CARTESIAN_POINT('Ctrl Pts',(3.2126165754971,15.2,-9.89276574013813));
#161788=CARTESIAN_POINT('Ctrl Pts',(3.21356644839295,15.2,-9.89485593809657));
#161789=CARTESIAN_POINT('Ctrl Pts',(3.21454479436487,15.2,-9.89699171571608));
#161790=CARTESIAN_POINT('Ctrl Pts',(3.21552314024793,15.2,-9.89912749314159));
#161791=CARTESIAN_POINT('Ctrl Pts',(3.21652996018322,15.2,-9.9013088532216));
#161792=CARTESIAN_POINT('Ctrl Pts',(3.2175654309837,15.2,-9.90353478648428));
#161793=CARTESIAN_POINT('Ctrl Pts',(3.21860090178418,15.2,-9.90576071974695));
#161794=CARTESIAN_POINT('Ctrl Pts',(3.21966502682308,15.2,-9.90803122674332));
#161795=CARTESIAN_POINT('Ctrl Pts',(3.22075797069878,15.2,-9.91034532715734));
#161796=CARTESIAN_POINT('Ctrl Pts',(3.22185091467376,15.2,-9.91265942778154));
#161797=CARTESIAN_POINT('Ctrl Pts',(3.22297268103564,15.2,-9.91501712288619));
#161798=CARTESIAN_POINT('Ctrl Pts',(3.22412343085033,15.2,-9.91741745476992));
#161799=CARTESIAN_POINT('Ctrl Pts',(3.2252741805605,15.2,-9.91981778643561));
#161800=CARTESIAN_POINT('Ctrl Pts',(3.22645391460024,15.2,-9.92226075746568));
#161801=CARTESIAN_POINT('Ctrl Pts',(3.22766278830756,15.2,-9.9247454351272));
#161802=CARTESIAN_POINT('Ctrl Pts',(3.2288716620149,15.2,-9.92723011278871));
#161803=CARTESIAN_POINT('Ctrl Pts',(3.23010967579493,15.2,-9.92975649768857));
#161804=CARTESIAN_POINT('Ctrl Pts',(3.23137697841428,15.2,-9.93232368142687));
#161805=CARTESIAN_POINT('Ctrl Pts',(3.23264428103363,15.2,-9.93489086516516));
#161806=CARTESIAN_POINT('Ctrl Pts',(3.23394087093888,15.2,-9.93749884706859));
#161807=CARTESIAN_POINT('Ctrl Pts',(3.23526689255536,15.2,-9.94014674271966));
#161808=CARTESIAN_POINT('Ctrl Pts',(3.23659291429229,15.2,-9.94279463861126));
#161809=CARTESIAN_POINT('Ctrl Pts',(3.23794836657372,15.2,-9.94548244614007));
#161810=CARTESIAN_POINT('Ctrl Pts',(3.23933338706717,15.2,-9.94820930137372));
#161811=CARTESIAN_POINT('Ctrl Pts',(3.2407184074348,15.2,-9.95093615635967));
#161812=CARTESIAN_POINT('Ctrl Pts',(3.24213299317023,15.2,-9.95370205968793));
#161813=CARTESIAN_POINT('Ctrl Pts',(3.24357727670757,15.2,-9.95650616476535));
#161814=CARTESIAN_POINT('Ctrl Pts',(3.24502156024492,15.2,-9.95931026984277));
#161815=CARTESIAN_POINT('Ctrl Pts',(3.24649554098433,15.2,-9.96215257641826));
#161816=CARTESIAN_POINT('Ctrl Pts',(3.24799934334432,15.2,-9.9650322613944));
#161817=CARTESIAN_POINT('Ctrl Pts',(3.2495031458409,15.2,-9.96791194663211));
#161818=CARTESIAN_POINT('Ctrl Pts',(3.25103676869038,15.2,-9.97082900758185));
#161819=CARTESIAN_POINT('Ctrl Pts',(3.25260033236023,15.2,-9.97378263891107));
#161820=CARTESIAN_POINT('Ctrl Pts',(3.25416389588806,15.2,-9.976736269972));
#161821=CARTESIAN_POINT('Ctrl Pts',(3.25575739965917,15.2,-9.97972646891152));
#161822=CARTESIAN_POINT('Ctrl Pts',(3.25738095602416,15.2,-9.98275245098191));
#161823=CARTESIAN_POINT('Ctrl Pts',(3.25900451238914,15.2,-9.9857784330523));
#161824=CARTESIAN_POINT('Ctrl Pts',(3.2606581221296,15.2,-9.98884019302732));
#161825=CARTESIAN_POINT('Ctrl Pts',(3.26234189356637,15.2,-9.99193696241241));
#161826=CARTESIAN_POINT('Ctrl Pts',(3.26402566515607,15.2,-9.99503373207878));
#161827=CARTESIAN_POINT('Ctrl Pts',(3.26573959839307,15.2,-9.99816551050694));
#161828=CARTESIAN_POINT('Ctrl Pts',(3.26748379516036,15.2,-10.0013315413396));
#161829=CARTESIAN_POINT('Ctrl Pts',(3.26922799176922,15.2,-10.0044975718848));
#161830=CARTESIAN_POINT('Ctrl Pts',(3.27100245227379,15.2,-10.0076978552424));
#161831=CARTESIAN_POINT('Ctrl Pts',(3.27280727645822,15.2,-10.0109316507083));
#161832=CARTESIAN_POINT('Ctrl Pts',(3.27491290478269,15.2,-10.014704412281));
#161833=CARTESIAN_POINT('Ctrl Pts',(3.27705985754708,15.2,-10.0185227891761));
#161834=CARTESIAN_POINT('Ctrl Pts',(3.27924828791476,15.2,-10.0223856295703));
#161835=CARTESIAN_POINT('Ctrl Pts',(3.28112408527542,15.2,-10.0256966354507));
#161836=CARTESIAN_POINT('Ctrl Pts',(3.28303035258691,15.2,-10.0290403112726));
#161837=CARTESIAN_POINT('Ctrl Pts',(3.28496717901655,15.2,-10.0324159479833));
#161838=CARTESIAN_POINT('Ctrl Pts',(3.28722680996841,15.2,-10.0363541910169));
#161839=CARTESIAN_POINT('Ctrl Pts',(3.28952803487752,15.2,-10.0403359358679));
#161840=CARTESIAN_POINT('Ctrl Pts',(3.29187098801924,15.2,-10.044360085342));
#161841=CARTESIAN_POINT('Ctrl Pts',(3.29354452595155,15.2,-10.0472344777788));
#161842=CARTESIAN_POINT('Ctrl Pts',(3.29523935320595,15.2,-10.0501305038409));
#161843=CARTESIAN_POINT('Ctrl Pts',(3.2969555144577,15.2,-10.0530477721065));
#161844=CARTESIAN_POINT('Ctrl Pts',(3.29867167570945,15.2,-10.0559650403722));
#161845=CARTESIAN_POINT('Ctrl Pts',(3.30040917285599,15.2,-10.0589035506631));
#161846=CARTESIAN_POINT('Ctrl Pts',(3.30216804820496,15.2,-10.0618629164287));
#161847=CARTESIAN_POINT('Ctrl Pts',(3.30392692336221,15.2,-10.0648222818718));
#161848=CARTESIAN_POINT('Ctrl Pts',(3.30570717814016,15.2,-10.067802502614));
#161849=CARTESIAN_POINT('Ctrl Pts',(3.3075088524559,15.2,-10.0708031988825));
#161850=CARTESIAN_POINT('Ctrl Pts',(3.30931052696803,15.2,-10.073803895478));
#161851=CARTESIAN_POINT('Ctrl Pts',(3.31113362438261,15.2,-10.0768250666594));
#161852=CARTESIAN_POINT('Ctrl Pts',(3.31297818049196,15.2,-10.0798663383938));
#161853=CARTESIAN_POINT('Ctrl Pts',(3.31482273660131,15.2,-10.0829076101283));
#161854=CARTESIAN_POINT('Ctrl Pts',(3.3166887543436,15.2,-10.0859689831676));
#161855=CARTESIAN_POINT('Ctrl Pts',(3.31857627054752,15.2,-10.0890500876257));
#161856=CARTESIAN_POINT('Ctrl Pts',(3.32046378675144,15.2,-10.0921311920838));
#161857=CARTESIAN_POINT('Ctrl Pts',(3.32237280170266,15.2,-10.0952320288304));
#161858=CARTESIAN_POINT('Ctrl Pts',(3.32430335267376,15.2,-10.0983522340377));
#161859=CARTESIAN_POINT('Ctrl Pts',(3.32623390364487,15.2,-10.101472439245));
#161860=CARTESIAN_POINT('Ctrl Pts',(3.32818598907207,15.2,-10.1046120134278));
#161861=CARTESIAN_POINT('Ctrl Pts',(3.33015964511261,15.2,-10.1077706000935));
#161862=CARTESIAN_POINT('Ctrl Pts',(3.33213330115316,15.2,-10.1109291867592));
#161863=CARTESIAN_POINT('Ctrl Pts',(3.33412852699525,15.2,-10.1141067834615));
#161864=CARTESIAN_POINT('Ctrl Pts',(3.33614535624046,15.2,-10.1173030402816));
#161865=CARTESIAN_POINT('Ctrl Pts',(3.33816218548567,15.2,-10.1204992971016));
#161866=CARTESIAN_POINT('Ctrl Pts',(3.34020061572211,15.2,-10.1237142122666));
#161867=CARTESIAN_POINT('Ctrl Pts',(3.34226068245822,15.2,-10.126947439975));
#161868=CARTESIAN_POINT('Ctrl Pts',(3.34432074919432,15.2,-10.1301806676833));
#161869=CARTESIAN_POINT('Ctrl Pts',(3.34640244882476,15.2,-10.1334322079591));
#161870=CARTESIAN_POINT('Ctrl Pts',(3.34850581320937,15.2,-10.1367017182518));
#161871=CARTESIAN_POINT('Ctrl Pts',(3.35060917759399,15.2,-10.1399712285444));
#161872=CARTESIAN_POINT('Ctrl Pts',(3.3527342059504,15.2,-10.1432587085264));
#161873=CARTESIAN_POINT('Ctrl Pts',(3.35488092609042,15.2,-10.1465638219996));
#161874=CARTESIAN_POINT('Ctrl Pts',(3.35702764623043,15.2,-10.1498689354727));
#161875=CARTESIAN_POINT('Ctrl Pts',(3.35919605986436,15.2,-10.1531916819787));
#161876=CARTESIAN_POINT('Ctrl Pts',(3.36138619014326,15.2,-10.1565317289935));
#161877=CARTESIAN_POINT('Ctrl Pts',(3.36357632042216,15.2,-10.1598717760083));
#161878=CARTESIAN_POINT('Ctrl Pts',(3.36578817010052,15.2,-10.163229122581));
#161879=CARTESIAN_POINT('Ctrl Pts',(3.36802176287943,15.2,-10.1666034429291));
#161880=CARTESIAN_POINT('Ctrl Pts',(3.37025535565835,15.2,-10.1699777632772));
#161881=CARTESIAN_POINT('Ctrl Pts',(3.3725106926157,15.2,-10.1733690568298));
#161882=CARTESIAN_POINT('Ctrl Pts',(3.37478779627264,15.2,-10.1767770006123));
#161883=CARTESIAN_POINT('Ctrl Pts',(3.37706489992957,15.2,-10.1801849443948));
#161884=CARTESIAN_POINT('Ctrl Pts',(3.37936377073499,15.2,-10.1836095356154));
#161885=CARTESIAN_POINT('Ctrl Pts',(3.3816844315701,15.2,-10.1870504599917));
#161886=CARTESIAN_POINT('Ctrl Pts',(3.38354096008642,15.2,-10.1898031992677));
#161887=CARTESIAN_POINT('Ctrl Pts',(3.38541143248982,15.2,-10.1925663900674));
#161888=CARTESIAN_POINT('Ctrl Pts',(3.38729586111264,15.2,-10.1953398715067));
#161889=CARTESIAN_POINT('Ctrl Pts',(3.38918028999221,15.2,-10.1981133533238));
#161890=CARTESIAN_POINT('Ctrl Pts',(3.39107867482927,15.2,-10.2008971244294));
#161891=CARTESIAN_POINT('Ctrl Pts',(3.39299102575246,15.2,-10.2036910283888));
#161892=CARTESIAN_POINT('Ctrl Pts',(3.3949033764151,15.2,-10.2064849319675));
#161893=CARTESIAN_POINT('Ctrl Pts',(3.39682969290649,15.2,-10.2092889664507));
#161894=CARTESIAN_POINT('Ctrl Pts',(3.39876998485807,15.2,-10.2121029745534));
#161895=CARTESIAN_POINT('Ctrl Pts',(3.40071027707402,15.2,-10.2149169830394));
#161896=CARTESIAN_POINT('Ctrl Pts',(3.40266454439163,15.2,-10.2177409650683));
#161897=CARTESIAN_POINT('Ctrl Pts',(3.40463279594426,15.2,-10.2205747637234));
#161898=CARTESIAN_POINT('Ctrl Pts',(3.40660104722872,15.2,-10.2234085619924));
#161899=CARTESIAN_POINT('Ctrl Pts',(3.4085832837472,15.2,-10.2262521788303));
#161900=CARTESIAN_POINT('Ctrl Pts',(3.4105795124603,15.2,-10.2291054571277));
#161901=CARTESIAN_POINT('Ctrl Pts',(3.41257574144538,15.2,-10.2319587358138));
#161902=CARTESIAN_POINT('Ctrl Pts',(3.4145859632265,15.2,-10.23482167725));
#161903=CARTESIAN_POINT('Ctrl Pts',(3.4166101861155,15.2,-10.2376941291849));
#161904=CARTESIAN_POINT('Ctrl Pts',(3.41863440872871,15.2,-10.2405665807285));
#161905=CARTESIAN_POINT('Ctrl Pts',(3.42067263186689,15.2,-10.243448542084));
#161906=CARTESIAN_POINT('Ctrl Pts',(3.42272486369769,15.2,-10.2463398615689));
#161907=CARTESIAN_POINT('Ctrl Pts',(3.42477709580811,15.2,-10.2492311814478));
#161908=CARTESIAN_POINT('Ctrl Pts',(3.42684333565066,15.2,-10.252131859419));
#161909=CARTESIAN_POINT('Ctrl Pts',(3.42892359055131,15.2,-10.255041746702));
#161910=CARTESIAN_POINT('Ctrl Pts',(3.43100384516853,15.2,-10.2579516335884));
#161911=CARTESIAN_POINT('Ctrl Pts',(3.43309811644008,15.2,-10.2608707295837));
#161912=CARTESIAN_POINT('Ctrl Pts',(3.43520640715519,15.2,-10.2637988857879));
#161913=CARTESIAN_POINT('Ctrl Pts',(3.43731469815756,15.2,-10.266727042391));
#161914=CARTESIAN_POINT('Ctrl Pts',(3.43943701145012,15.2,-10.2696642583616));
#161915=CARTESIAN_POINT('Ctrl Pts',(3.44157335223322,15.2,-10.2726103889666));
#161916=CARTESIAN_POINT('Ctrl Pts',(3.44370969301631,15.2,-10.2755565195716));
#161917=CARTESIAN_POINT('Ctrl Pts',(3.44586005991494,15.2,-10.2785115634499));
#161918=CARTESIAN_POINT('Ctrl Pts',(3.44802446131211,15.2,-10.2814753755012));
#161919=CARTESIAN_POINT('Ctrl Pts',(3.45018886241438,15.2,-10.2844391871487));
#161920=CARTESIAN_POINT('Ctrl Pts',(3.45236729506773,15.2,-10.2874117680198));
#161921=CARTESIAN_POINT('Ctrl Pts',(3.45455976623173,15.2,-10.2903929722896));
#161922=CARTESIAN_POINT('Ctrl Pts',(3.45675223769445,15.2,-10.2933741769656));
#161923=CARTESIAN_POINT('Ctrl Pts',(3.45895874696272,15.2,-10.2963640061898));
#161924=CARTESIAN_POINT('Ctrl Pts',(3.46117929786295,15.2,-10.2993623169652));
#161925=CARTESIAN_POINT('Ctrl Pts',(3.46339984846063,15.2,-10.3023606273321));
#161926=CARTESIAN_POINT('Ctrl Pts',(3.46563444193705,15.2,-10.3053674200062));
#161927=CARTESIAN_POINT('Ctrl Pts',(3.46788308114119,15.2,-10.3083825535369));
#161928=CARTESIAN_POINT('Ctrl Pts',(3.47013172065172,15.2,-10.3113976874785));
#161929=CARTESIAN_POINT('Ctrl Pts',(3.47239440600795,15.2,-10.3144211607781));
#161930=CARTESIAN_POINT('Ctrl Pts',(3.47467114158033,15.2,-10.3174528362066));
#161931=CARTESIAN_POINT('Ctrl Pts',(3.47694787684251,15.2,-10.3204845112221));
#161932=CARTESIAN_POINT('Ctrl Pts',(3.47923866260649,15.2,-10.3235243868617));
#161933=CARTESIAN_POINT('Ctrl Pts',(3.4815434998616,15.2,-10.3265723245009));
#161934=CARTESIAN_POINT('Ctrl Pts',(3.48384833743075,15.2,-10.3296202625554));
#161935=CARTESIAN_POINT('Ctrl Pts',(3.48616722836268,15.2,-10.3326762629608));
#161936=CARTESIAN_POINT('Ctrl Pts',(3.48850017449074,15.2,-10.3357401890172));
#161937=CARTESIAN_POINT('Ctrl Pts',(3.49083312030094,15.2,-10.3388041146561));
#161938=CARTESIAN_POINT('Ctrl Pts',(3.49318012189196,15.2,-10.3418759643461));
#161939=CARTESIAN_POINT('Ctrl Pts',(3.49554118064903,15.2,-10.3449556048032));
#161940=CARTESIAN_POINT('Ctrl Pts',(3.4979022397278,15.2,-10.3480352456798));
#161941=CARTESIAN_POINT('Ctrl Pts',(3.50027735801699,15.2,-10.3511226752617));
#161942=CARTESIAN_POINT('Ctrl Pts',(3.50266653420367,15.2,-10.3542177599864));
#161943=CARTESIAN_POINT('Ctrl Pts',(3.50505571006482,15.2,-10.3573128442894));
#161944=CARTESIAN_POINT('Ctrl Pts',(3.50745894632316,15.2,-10.3604155831493));
#161945=CARTESIAN_POINT('Ctrl Pts',(3.50987624284634,15.2,-10.3635258429498));
#161946=CARTESIAN_POINT('Ctrl Pts',(3.51229353969887,15.2,-10.3666361031741));
#161947=CARTESIAN_POINT('Ctrl Pts',(3.51472489722379,15.2,-10.3697538858481));
#161948=CARTESIAN_POINT('Ctrl Pts',(3.51717031670156,15.2,-10.3728790573104));
#161949=CARTESIAN_POINT('Ctrl Pts',(3.51961573584613,15.2,-10.376004228347));
#161950=CARTESIAN_POINT('Ctrl Pts',(3.52207521766857,15.2,-10.3791367876413));
#161951=CARTESIAN_POINT('Ctrl Pts',(3.52454876085381,15.2,-10.382276605995));
#161952=CARTESIAN_POINT('Ctrl Pts',(3.52702230437607,15.2,-10.3854164247765));
#161953=CARTESIAN_POINT('Ctrl Pts',(3.52950990996076,15.2,-10.3885635012531));
#161954=CARTESIAN_POINT('Ctrl Pts',(3.53201157870822,15.2,-10.3917177072583));
#161955=CARTESIAN_POINT('Ctrl Pts',(3.53451324745567,15.2,-10.3948719132636));
#161956=CARTESIAN_POINT('Ctrl Pts',(3.53702897803809,15.2,-10.3980332468168));
#161957=CARTESIAN_POINT('Ctrl Pts',(3.53955877145519,15.2,-10.401201579768));
#161958=CARTESIAN_POINT('Ctrl Pts',(3.54272101305421,15.2,-10.4051619957411));
#161959=CARTESIAN_POINT('Ctrl Pts',(3.54590522643969,15.2,-10.4091333511977));
#161960=CARTESIAN_POINT('Ctrl Pts',(3.5491114106776,15.2,-10.4131153930042));
#161961=CARTESIAN_POINT('Ctrl Pts',(3.55167635785825,15.2,-10.4163010261889));
#161962=CARTESIAN_POINT('Ctrl Pts',(3.55425536660671,15.2,-10.4194935014115));
#161963=CARTESIAN_POINT('Ctrl Pts',(3.55684843623979,15.2,-10.4226926904978));
#161964=CARTESIAN_POINT('Ctrl Pts',(3.55944150622618,15.2,-10.42589188002));
#161965=CARTESIAN_POINT('Ctrl Pts',(3.56204863528416,15.2,-10.4290977839356));
#161966=CARTESIAN_POINT('Ctrl Pts',(3.56466982342846,15.2,-10.4323102775002));
#161967=CARTESIAN_POINT('Ctrl Pts',(3.56729101121562,15.2,-10.4355227706272));
#161968=CARTESIAN_POINT('Ctrl Pts',(3.56992625837039,15.2,-10.4387418535199));
#161969=CARTESIAN_POINT('Ctrl Pts',(3.57257556154178,15.2,-10.441967401978));
#161970=CARTESIAN_POINT('Ctrl Pts',(3.57522486507413,15.2,-10.4451929508756));
#161971=CARTESIAN_POINT('Ctrl Pts',(3.57788822557147,15.2,-10.4484249647644));
#161972=CARTESIAN_POINT('Ctrl Pts',(3.58056564113014,15.2,-10.4516633224366));
#161973=CARTESIAN_POINT('Ctrl Pts',(3.58324305632402,15.2,-10.4549016796675));
#161974=CARTESIAN_POINT('Ctrl Pts',(3.58593452576483,15.2,-10.4581463800227));
#161975=CARTESIAN_POINT('Ctrl Pts',(3.58864004748718,15.2,-10.4613973005343));
#161976=CARTESIAN_POINT('Ctrl Pts',(3.59134556957816,15.2,-10.4646482214888));
#161977=CARTESIAN_POINT('Ctrl Pts',(3.59406514342359,15.2,-10.467905363358));
#161978=CARTESIAN_POINT('Ctrl Pts',(3.59679876624016,15.2,-10.4711686062585));
#161979=CARTESIAN_POINT('Ctrl Pts',(3.59953238868429,15.2,-10.4744318487143));
#161980=CARTESIAN_POINT('Ctrl Pts',(3.60228006054934,15.2,-10.4777011909822));
#161981=CARTESIAN_POINT('Ctrl Pts',(3.60504177834923,15.2,-10.4809765142664));
#161982=CARTESIAN_POINT('Ctrl Pts',(3.6078034965254,15.2,-10.484251837997));
#161983=CARTESIAN_POINT('Ctrl Pts',(3.61057926056401,15.2,-10.4875331417587));
#161984=CARTESIAN_POINT('Ctrl Pts',(3.61336906549476,15.2,-10.4908203079938));
#161985=CARTESIAN_POINT('Ctrl Pts',(3.61615887004539,15.2,-10.494107473781));
#161986=CARTESIAN_POINT('Ctrl Pts',(3.61896271805152,15.2,-10.4974005015059));
#161987=CARTESIAN_POINT('Ctrl Pts',(3.62178060376417,15.2,-10.5006992727356));
#161988=CARTESIAN_POINT('Ctrl Pts',(3.62459848986076,15.2,-10.5039980444149));
#161989=CARTESIAN_POINT('Ctrl Pts',(3.62743041346709,15.2,-10.5073025604818));
#161990=CARTESIAN_POINT('Ctrl Pts',(3.6302763709685,15.2,-10.5106127035106));
#161991=CARTESIAN_POINT('Ctrl Pts',(3.63312232808215,15.2,-10.5139228460884));
#161992=CARTESIAN_POINT('Ctrl Pts',(3.6359823192497,15.2,-10.517238616754));
#161993=CARTESIAN_POINT('Ctrl Pts',(3.63885633901333,15.2,-10.520559897982));
#161994=CARTESIAN_POINT('Ctrl Pts',(3.64173035916854,15.2,-10.5238811796624));
#161995=CARTESIAN_POINT('Ctrl Pts',(3.64461840915283,15.2,-10.5272079733101));
#161996=CARTESIAN_POINT('Ctrl Pts',(3.64752048319988,15.2,-10.5305401629917));
#161997=CARTESIAN_POINT('Ctrl Pts',(3.65042255724694,15.2,-10.5338723526733));
#161998=CARTESIAN_POINT('Ctrl Pts',(3.65333865535118,15.2,-10.5372099392222));
#161999=CARTESIAN_POINT('Ctrl Pts',(3.6562687715123,15.2,-10.5405528082382));
#162000=CARTESIAN_POINT('Ctrl Pts',(3.65846635843353,15.2,-10.5430599597725));
#162001=CARTESIAN_POINT('Ctrl Pts',(3.66067183138046,15.2,-10.5455700828517));
#162002=CARTESIAN_POINT('Ctrl Pts',(3.66288518741153,15.2,-10.5480831299696));
#162003=CARTESIAN_POINT('Ctrl Pts',(3.6650985434426,15.2,-10.5505961770875));
#162004=CARTESIAN_POINT('Ctrl Pts',(3.66731978230663,15.2,-10.5531121479659));
#162005=CARTESIAN_POINT('Ctrl Pts',(3.66954890218466,15.2,-10.5556309945413));
#162006=CARTESIAN_POINT('Ctrl Pts',(3.6717780220627,15.2,-10.5581498411167));
#162007=CARTESIAN_POINT('Ctrl Pts',(3.67401502313145,15.2,-10.560671564225));
#162008=CARTESIAN_POINT('Ctrl Pts',(3.67625990200822,15.2,-10.5631961167167));
#162009=CARTESIAN_POINT('Ctrl Pts',(3.67850478088499,15.2,-10.5657206692083));
#162010=CARTESIAN_POINT('Ctrl Pts',(3.6807575375531,15.2,-10.5682480497164));
#162011=CARTESIAN_POINT('Ctrl Pts',(3.68301816992861,15.2,-10.5707782137076));
#162012=CARTESIAN_POINT('Ctrl Pts',(3.68527880230413,15.2,-10.5733083776987));
#162013=CARTESIAN_POINT('Ctrl Pts',(3.68754731062943,15.2,-10.5758413237418));
#162014=CARTESIAN_POINT('Ctrl Pts',(3.68982369157621,15.2,-10.5783770049428));
#162015=CARTESIAN_POINT('Ctrl Pts',(3.692100072523,15.2,-10.5809126861437));
#162016=CARTESIAN_POINT('Ctrl Pts',(3.69438432563456,15.2,-10.5834511037554));
#162017=CARTESIAN_POINT('Ctrl Pts',(3.69667644946688,15.2,-10.585992210246));
#162018=CARTESIAN_POINT('Ctrl Pts',(3.6989685737156,15.2,-10.5885333171983));
#162019=CARTESIAN_POINT('Ctrl Pts',(3.70126856814986,15.2,-10.591077112568));
#162020=CARTESIAN_POINT('Ctrl Pts',(3.70357642852801,15.2,-10.5936235520635));
#162021=CARTESIAN_POINT('Ctrl Pts',(3.7058842884869,15.2,-10.5961699910963));
#162022=CARTESIAN_POINT('Ctrl Pts',(3.7082000162537,15.2,-10.598719072954));
#162023=CARTESIAN_POINT('Ctrl Pts',(3.71052360721163,15.2,-10.6012707524865));
#162024=CARTESIAN_POINT('Ctrl Pts',(3.71284719816956,15.2,-10.603822432019));
#162025=CARTESIAN_POINT('Ctrl Pts',(3.71517865357636,15.2,-10.6063767084836));
#162026=CARTESIAN_POINT('Ctrl Pts',(3.71751796946035,15.2,-10.6089335374856));
#162027=CARTESIAN_POINT('Ctrl Pts',(3.71985728534434,15.2,-10.6114903664877));
#162028=CARTESIAN_POINT('Ctrl Pts',(3.722204462706,15.2,-10.6140497474458));
#162029=CARTESIAN_POINT('Ctrl Pts',(3.72455949750608,15.2,-10.616611634531));
#162030=CARTESIAN_POINT('Ctrl Pts',(3.72691453230618,15.2,-10.6191735216162));
#162031=CARTESIAN_POINT('Ctrl Pts',(3.72927742367842,15.2,-10.621737915047));
#162032=CARTESIAN_POINT('Ctrl Pts',(3.73164816996661,15.2,-10.6243047702036));
#162033=CARTESIAN_POINT('Ctrl Pts',(3.7340189162548,15.2,-10.6268716253601));
#162034=CARTESIAN_POINT('Ctrl Pts',(3.73639751623409,15.2,-10.6294409430165));
#162035=CARTESIAN_POINT('Ctrl Pts',(3.73878396797965,15.2,-10.632012676631));
#162036=CARTESIAN_POINT('Ctrl Pts',(3.74117042015876,15.2,-10.6345844107128));
#162037=CARTESIAN_POINT('Ctrl Pts',(3.74356472229005,15.2,-10.6371585621036));
#162038=CARTESIAN_POINT('Ctrl Pts',(3.74596687251523,15.2,-10.6397350856033));
#162039=CARTESIAN_POINT('Ctrl Pts',(3.74836902230402,15.2,-10.6423116086351));
#162040=CARTESIAN_POINT('Ctrl Pts',(3.7507790195839,15.2,-10.6448905030306));
#162041=CARTESIAN_POINT('Ctrl Pts',(3.75319686049276,15.2,-10.6474717267328));
#162042=CARTESIAN_POINT('Ctrl Pts',(3.75561470140162,15.2,-10.6500529504349));
#162043=CARTESIAN_POINT('Ctrl Pts',(3.75804038476968,15.2,-10.652636502609));
#162044=CARTESIAN_POINT('Ctrl Pts',(3.76047391001527,15.2,-10.6552223378069));
#162045=CARTESIAN_POINT('Ctrl Pts',(3.76290743526087,15.2,-10.6578081730048));
#162046=CARTESIAN_POINT('Ctrl Pts',(3.76534880013888,15.2,-10.6603962935608));
#162047=CARTESIAN_POINT('Ctrl Pts',(3.76779800100822,15.2,-10.6629866532583));
#162048=CARTESIAN_POINT('Ctrl Pts',(3.77024720187756,15.2,-10.6655770129559));
#162049=CARTESIAN_POINT('Ctrl Pts',(3.77270423932158,15.2,-10.6681696135783));
#162050=CARTESIAN_POINT('Ctrl Pts',(3.77516910923135,15.2,-10.6707644107339));
#162051=CARTESIAN_POINT('Ctrl Pts',(3.77763397914112,15.2,-10.6733592078894));
#162052=CARTESIAN_POINT('Ctrl Pts',(3.78010668248367,15.2,-10.6759562020281));
#162053=CARTESIAN_POINT('Ctrl Pts',(3.78258721343414,15.2,-10.6785553496417));
#162054=CARTESIAN_POINT('Ctrl Pts',(3.78506774483524,15.2,-10.6811544977275));
#162055=CARTESIAN_POINT('Ctrl Pts',(3.78755610614688,15.2,-10.6837557992389));
#162056=CARTESIAN_POINT('Ctrl Pts',(3.7900522905524,15.2,-10.6863592113259));
#162057=CARTESIAN_POINT('Ctrl Pts',(3.79254847450444,15.2,-10.6889626229399));
#162058=CARTESIAN_POINT('Ctrl Pts',(3.79505248370082,15.2,-10.6915681452188));
#162059=CARTESIAN_POINT('Ctrl Pts',(3.79756431319427,15.2,-10.6941757354629));
#162060=CARTESIAN_POINT('Ctrl Pts',(3.80007614268773,15.2,-10.6967833257069));
#162061=CARTESIAN_POINT('Ctrl Pts',(3.80259579238333,15.2,-10.6993929839127));
#162062=CARTESIAN_POINT('Ctrl Pts',(3.80512325825051,15.2,-10.702004666568));
#162063=CARTESIAN_POINT('Ctrl Pts',(3.80765072411769,15.2,-10.7046163492233));
#162064=CARTESIAN_POINT('Ctrl Pts',(3.81018600740895,15.2,-10.707230057345));
#162065=CARTESIAN_POINT('Ctrl Pts',(3.81272910177488,15.2,-10.7098457485));
#162066=CARTESIAN_POINT('Ctrl Pts',(3.81527219614082,15.2,-10.712461439655));
#162067=CARTESIAN_POINT('Ctrl Pts',(3.8178231026481,15.2,-10.7150791137765));
#162068=CARTESIAN_POINT('Ctrl Pts',(3.82038181697112,15.2,-10.7176987284312));
#162069=CARTESIAN_POINT('Ctrl Pts',(3.82294053129414,15.2,-10.7203183430858));
#162070=CARTESIAN_POINT('Ctrl Pts',(3.82550705281773,15.2,-10.7229398990236));
#162071=CARTESIAN_POINT('Ctrl Pts',(3.8280813782269,15.2,-10.7255633537674));
#162072=CARTESIAN_POINT('Ctrl Pts',(3.83065570363607,15.2,-10.7281868085113));
#162073=CARTESIAN_POINT('Ctrl Pts',(3.83323783246379,15.2,-10.7308121620896));
#162074=CARTESIAN_POINT('Ctrl Pts',(3.83582775974363,15.2,-10.7334393727023));
#162075=CARTESIAN_POINT('Ctrl Pts',(3.83841768749397,15.2,-10.7360665837922));
#162076=CARTESIAN_POINT('Ctrl Pts',(3.84101541335483,15.2,-10.7386956510243));
#162077=CARTESIAN_POINT('Ctrl Pts',(3.8436209345679,15.2,-10.7413265355319));
#162078=CARTESIAN_POINT('Ctrl Pts',(3.84622645530763,15.2,-10.7439574195615));
#162079=CARTESIAN_POINT('Ctrl Pts',(3.84883976926361,15.2,-10.7465901190494));
#162080=CARTESIAN_POINT('Ctrl Pts',(3.85146087354406,15.2,-10.7492245946205));
#162081=CARTESIAN_POINT('Ctrl Pts',(3.8540819778245,15.2,-10.7518590701916));
#162082=CARTESIAN_POINT('Ctrl Pts',(3.85671087190274,15.2,-10.7544953205363));
#162083=CARTESIAN_POINT('Ctrl Pts',(3.85934755027729,15.2,-10.7571333042024));
#162084=CARTESIAN_POINT('Ctrl Pts',(3.86198422865183,15.2,-10.7597712878685));
#162085=CARTESIAN_POINT('Ctrl Pts',(3.86462869228184,15.2,-10.7624110048649));
#162086=CARTESIAN_POINT('Ctrl Pts',(3.86728093473915,15.2,-10.7650524129893));
#162087=CARTESIAN_POINT('Ctrl Pts',(3.86993317719647,15.2,-10.7676938211136));
#162088=CARTESIAN_POINT('Ctrl Pts',(3.87259320079017,15.2,-10.7703369197747));
#162089=CARTESIAN_POINT('Ctrl Pts',(3.87526099869257,15.2,-10.7729816734701));
#162090=CARTESIAN_POINT('Ctrl Pts',(3.87792879659497,15.2,-10.7756264271655));
#162091=CARTESIAN_POINT('Ctrl Pts',(3.88060437056348,15.2,-10.7782728362525));
#162092=CARTESIAN_POINT('Ctrl Pts',(3.88328771442326,15.2,-10.7809208604477));
#162093=CARTESIAN_POINT('Ctrl Pts',(3.88597105877052,15.2,-10.783568885124));
#162094=CARTESIAN_POINT('Ctrl Pts',(3.88866217424496,15.2,-10.7862185268258));
#162095=CARTESIAN_POINT('Ctrl Pts',(3.89136105359659,15.2,-10.7888697347946));
#162096=CARTESIAN_POINT('Ctrl Pts',(3.89405993245792,15.2,-10.7915209422819));
#162097=CARTESIAN_POINT('Ctrl Pts',(3.89676657572058,15.2,-10.7941737144439));
#162098=CARTESIAN_POINT('Ctrl Pts',(3.8994809782168,15.2,-10.7968280103136));
#162099=CARTESIAN_POINT('Ctrl Pts',(3.90219538071302,15.2,-10.7994823061832));
#162100=CARTESIAN_POINT('Ctrl Pts',(3.90491754234274,15.2,-10.8021381240576));
#162101=CARTESIAN_POINT('Ctrl Pts',(3.90764745926926,15.2,-10.804795445851));
#162102=CARTESIAN_POINT('Ctrl Pts',(3.91037737619578,15.2,-10.8074527676443));
#162103=CARTESIAN_POINT('Ctrl Pts',(3.91311504850119,15.2,-10.8101115945167));
#162104=CARTESIAN_POINT('Ctrl Pts',(3.91586047899994,15.2,-10.812771925));
#162105=CARTESIAN_POINT('Ctrl Pts',(3.20199116199994,12.2,-9.86852965800001));
#162106=CARTESIAN_POINT('Ctrl Pts',(3.20268657132788,12.2,-9.87017542455285));
#162107=CARTESIAN_POINT('Ctrl Pts',(3.20340918399116,12.2,-9.87187175340483));
#162108=CARTESIAN_POINT('Ctrl Pts',(3.20415920994276,12.2,-9.8736175032754));
#162109=CARTESIAN_POINT('Ctrl Pts',(3.20491285289861,12.2,-9.87537167203426));
#162110=CARTESIAN_POINT('Ctrl Pts',(3.20569417410877,12.2,-9.87717573863291));
#162111=CARTESIAN_POINT('Ctrl Pts',(3.20650338986158,12.2,-9.87902857766262));
#162112=CARTESIAN_POINT('Ctrl Pts',(3.2073126055409,12.2,-9.88088141652404));
#162113=CARTESIAN_POINT('Ctrl Pts',(3.20814971062299,12.2,-9.8827830280374));
#162114=CARTESIAN_POINT('Ctrl Pts',(3.20901491150822,12.2,-9.88473231696659));
#162115=CARTESIAN_POINT('Ctrl Pts',(3.20988011239345,12.2,-9.88668160589576));
#162116=CARTESIAN_POINT('Ctrl Pts',(3.21077340789157,12.2,-9.88867857373555));
#162117=CARTESIAN_POINT('Ctrl Pts',(3.21169499165248,12.2,-9.89072215684402));
#162118=CARTESIAN_POINT('Ctrl Pts',(3.2126165754971,12.2,-9.89276574013813));
#162119=CARTESIAN_POINT('Ctrl Pts',(3.21356644839295,12.2,-9.89485593809657));
#162120=CARTESIAN_POINT('Ctrl Pts',(3.21454479436487,12.2,-9.89699171571608));
#162121=CARTESIAN_POINT('Ctrl Pts',(3.21552314024793,12.2,-9.89912749314159));
#162122=CARTESIAN_POINT('Ctrl Pts',(3.21652996018322,12.2,-9.9013088532216));
#162123=CARTESIAN_POINT('Ctrl Pts',(3.2175654309837,12.2,-9.90353478648428));
#162124=CARTESIAN_POINT('Ctrl Pts',(3.21860090178418,12.2,-9.90576071974695));
#162125=CARTESIAN_POINT('Ctrl Pts',(3.21966502682308,12.2,-9.90803122674332));
#162126=CARTESIAN_POINT('Ctrl Pts',(3.22075797069878,12.2,-9.91034532715734));
#162127=CARTESIAN_POINT('Ctrl Pts',(3.22185091467376,12.2,-9.91265942778154));
#162128=CARTESIAN_POINT('Ctrl Pts',(3.22297268103564,12.2,-9.91501712288619));
#162129=CARTESIAN_POINT('Ctrl Pts',(3.22412343085033,12.2,-9.91741745476992));
#162130=CARTESIAN_POINT('Ctrl Pts',(3.2252741805605,12.2,-9.91981778643561));
#162131=CARTESIAN_POINT('Ctrl Pts',(3.22645391460024,12.2,-9.92226075746568));
#162132=CARTESIAN_POINT('Ctrl Pts',(3.22766278830756,12.2,-9.9247454351272));
#162133=CARTESIAN_POINT('Ctrl Pts',(3.2288716620149,12.2,-9.92723011278871));
#162134=CARTESIAN_POINT('Ctrl Pts',(3.23010967579493,12.2,-9.92975649768857));
#162135=CARTESIAN_POINT('Ctrl Pts',(3.23137697841428,12.2,-9.93232368142687));
#162136=CARTESIAN_POINT('Ctrl Pts',(3.23264428103363,12.2,-9.93489086516516));
#162137=CARTESIAN_POINT('Ctrl Pts',(3.23394087093888,12.2,-9.93749884706859));
#162138=CARTESIAN_POINT('Ctrl Pts',(3.23526689255536,12.2,-9.94014674271966));
#162139=CARTESIAN_POINT('Ctrl Pts',(3.23659291429229,12.2,-9.94279463861126));
#162140=CARTESIAN_POINT('Ctrl Pts',(3.23794836657372,12.2,-9.94548244614007));
#162141=CARTESIAN_POINT('Ctrl Pts',(3.23933338706717,12.2,-9.94820930137372));
#162142=CARTESIAN_POINT('Ctrl Pts',(3.2407184074348,12.2,-9.95093615635967));
#162143=CARTESIAN_POINT('Ctrl Pts',(3.24213299317023,12.2,-9.95370205968793));
#162144=CARTESIAN_POINT('Ctrl Pts',(3.24357727670757,12.2,-9.95650616476534));
#162145=CARTESIAN_POINT('Ctrl Pts',(3.24502156024491,12.2,-9.95931026984276));
#162146=CARTESIAN_POINT('Ctrl Pts',(3.24649554098433,12.2,-9.96215257641826));
#162147=CARTESIAN_POINT('Ctrl Pts',(3.24799934334432,12.2,-9.9650322613944));
#162148=CARTESIAN_POINT('Ctrl Pts',(3.2495031458409,12.2,-9.96791194663211));
#162149=CARTESIAN_POINT('Ctrl Pts',(3.25103676869038,12.2,-9.97082900758185));
#162150=CARTESIAN_POINT('Ctrl Pts',(3.25260033236023,12.2,-9.97378263891107));
#162151=CARTESIAN_POINT('Ctrl Pts',(3.25416389588806,12.2,-9.976736269972));
#162152=CARTESIAN_POINT('Ctrl Pts',(3.25575739965918,12.2,-9.97972646891153));
#162153=CARTESIAN_POINT('Ctrl Pts',(3.25738095602416,12.2,-9.98275245098191));
#162154=CARTESIAN_POINT('Ctrl Pts',(3.25900451238914,12.2,-9.9857784330523));
#162155=CARTESIAN_POINT('Ctrl Pts',(3.26065812212961,12.2,-9.98884019302732));
#162156=CARTESIAN_POINT('Ctrl Pts',(3.26234189356637,12.2,-9.99193696241241));
#162157=CARTESIAN_POINT('Ctrl Pts',(3.26402566515607,12.2,-9.99503373207879));
#162158=CARTESIAN_POINT('Ctrl Pts',(3.26573959839308,12.2,-9.99816551050695));
#162159=CARTESIAN_POINT('Ctrl Pts',(3.26748379516037,12.2,-10.0013315413397));
#162160=CARTESIAN_POINT('Ctrl Pts',(3.26922799176922,12.2,-10.0044975718848));
#162161=CARTESIAN_POINT('Ctrl Pts',(3.27100245227379,12.2,-10.0076978552424));
#162162=CARTESIAN_POINT('Ctrl Pts',(3.27280727645822,12.2,-10.0109316507083));
#162163=CARTESIAN_POINT('Ctrl Pts',(3.27461210064265,12.2,-10.0141654461741));
#162164=CARTESIAN_POINT('Ctrl Pts',(3.27644728547917,12.2,-10.0174327549877));
#162165=CARTESIAN_POINT('Ctrl Pts',(3.27831292783616,12.2,-10.0207328516975));
#162166=CARTESIAN_POINT('Ctrl Pts',(3.28017857036261,12.2,-10.0240329487069));
#162167=CARTESIAN_POINT('Ctrl Pts',(3.28207466745283,12.2,-10.0273658338645));
#162168=CARTESIAN_POINT('Ctrl Pts',(3.28400131172657,12.2,-10.0307307968834));
#162169=CARTESIAN_POINT('Ctrl Pts',(3.28592795582531,12.2,-10.0340957595966));
#162170=CARTESIAN_POINT('Ctrl Pts',(3.28788514159727,12.2,-10.0374928010271));
#162171=CARTESIAN_POINT('Ctrl Pts',(3.28987295803413,12.2,-10.0409212247515));
#162172=CARTESIAN_POINT('Ctrl Pts',(3.29186077447099,12.2,-10.0443496484759));
#162173=CARTESIAN_POINT('Ctrl Pts',(3.29387922191414,12.2,-10.0478094560464));
#162174=CARTESIAN_POINT('Ctrl Pts',(3.29592837717168,12.2,-10.0512999628349));
#162175=CARTESIAN_POINT('Ctrl Pts',(3.29763600661501,12.2,-10.0542087185976));
#162176=CARTESIAN_POINT('Ctrl Pts',(3.29936496256444,12.2,-10.0571387938304));
#162177=CARTESIAN_POINT('Ctrl Pts',(3.30111528791055,12.2,-10.0600898020238));
#162178=CARTESIAN_POINT('Ctrl Pts',(3.30286561325665,12.2,-10.0630408102171));
#162179=CARTESIAN_POINT('Ctrl Pts',(3.30463731045194,12.2,-10.0660127496903));
#162180=CARTESIAN_POINT('Ctrl Pts',(3.30643041830724,12.2,-10.0690052412317));
#162181=CARTESIAN_POINT('Ctrl Pts',(3.30822352616255,12.2,-10.071997732773));
#162182=CARTESIAN_POINT('Ctrl Pts',(3.31003804832766,12.2,-10.0750107740499));
#162183=CARTESIAN_POINT('Ctrl Pts',(3.31187402200822,12.2,-10.0780439907166));
#162184=CARTESIAN_POINT('Ctrl Pts',(3.31370999568878,12.2,-10.0810772073833));
#162185=CARTESIAN_POINT('Ctrl Pts',(3.31556742194232,12.2,-10.0841305985987));
#162186=CARTESIAN_POINT('Ctrl Pts',(3.31744634049258,12.2,-10.0872037960433));
#162187=CARTESIAN_POINT('Ctrl Pts',(3.31932525904285,12.2,-10.0902769934879));
#162188=CARTESIAN_POINT('Ctrl Pts',(3.32122566853014,12.2,-10.0933699950749));
#162189=CARTESIAN_POINT('Ctrl Pts',(3.32314760630905,12.2,-10.0964824384786));
#162190=CARTESIAN_POINT('Ctrl Pts',(3.32506954408795,12.2,-10.0995948818824));
#162191=CARTESIAN_POINT('Ctrl Pts',(3.32701301051074,12.2,-10.1027267651552));
#162192=CARTESIAN_POINT('Ctrl Pts',(3.32897803988687,12.2,-10.1058777326562));
#162193=CARTESIAN_POINT('Ctrl Pts',(3.33094306926299,12.2,-10.1090287001571));
#162194=CARTESIAN_POINT('Ctrl Pts',(3.33292966242571,12.2,-10.1121987489485));
#162195=CARTESIAN_POINT('Ctrl Pts',(3.33493785120809,12.2,-10.1153875283452));
#162196=CARTESIAN_POINT('Ctrl Pts',(3.33694603999046,12.2,-10.1185763077419));
#162197=CARTESIAN_POINT('Ctrl Pts',(3.33897582609978,12.2,-10.121783815576));
#162198=CARTESIAN_POINT('Ctrl Pts',(3.34102723901821,12.2,-10.1250097041886));
#162199=CARTESIAN_POINT('Ctrl Pts',(3.34307865193664,12.2,-10.1282355928012));
#162200=CARTESIAN_POINT('Ctrl Pts',(3.34515169511101,12.2,-10.1314798631419));
#162201=CARTESIAN_POINT('Ctrl Pts',(3.34724639455722,12.2,-10.134742171685));
#162202=CARTESIAN_POINT('Ctrl Pts',(3.34934109377511,12.2,-10.1380044798726));
#162203=CARTESIAN_POINT('Ctrl Pts',(3.3514574532995,12.2,-10.1412848262684));
#162204=CARTESIAN_POINT('Ctrl Pts',(3.35359549674524,12.2,-10.1445828720186));
#162205=CARTESIAN_POINT('Ctrl Pts',(3.35573354042403,12.2,-10.1478809181283));
#162206=CARTESIAN_POINT('Ctrl Pts',(3.3578932721719,12.2,-10.1511966642599));
#162207=CARTESIAN_POINT('Ctrl Pts',(3.36007471723956,12.2,-10.154529778564));
#162208=CARTESIAN_POINT('Ctrl Pts',(3.36225616230723,12.2,-10.1578628928681));
#162209=CARTESIAN_POINT('Ctrl Pts',(3.36445931893843,12.2,-10.1612133717553));
#162210=CARTESIAN_POINT('Ctrl Pts',(3.36668421574221,12.2,-10.1645808896012));
#162211=CARTESIAN_POINT('Ctrl Pts',(3.36890911254599,12.2,-10.167948407447));
#162212=CARTESIAN_POINT('Ctrl Pts',(3.37115574773594,12.2,-10.1713329637864));
#162213=CARTESIAN_POINT('Ctrl Pts',(3.37342414548664,12.2,-10.1747342343719));
#162214=CARTESIAN_POINT('Ctrl Pts',(3.37569254323735,12.2,-10.1781355049573));
#162215=CARTESIAN_POINT('Ctrl Pts',(3.37798270409996,12.2,-10.1815534882874));
#162216=CARTESIAN_POINT('Ctrl Pts',(3.38029464930715,12.2,-10.1849878669671));
#162217=CARTESIAN_POINT('Ctrl Pts',(3.38260659451435,12.2,-10.1884222456468));
#162218=CARTESIAN_POINT('Ctrl Pts',(3.38494032514155,12.2,-10.1918730194242));
#162219=CARTESIAN_POINT('Ctrl Pts',(3.38729586111264,12.2,-10.1953398715067));
#162220=CARTESIAN_POINT('Ctrl Pts',(3.38965139708372,12.2,-10.1988067235892));
#162221=CARTESIAN_POINT('Ctrl Pts',(3.39202873963218,12.2,-10.2022896534767));
#162222=CARTESIAN_POINT('Ctrl Pts',(3.39442790728192,12.2,-10.2057883530064));
#162223=CARTESIAN_POINT('Ctrl Pts',(3.39634724150631,12.2,-10.2085873127827));
#162224=CARTESIAN_POINT('Ctrl Pts',(3.39828054458294,12.2,-10.2113963636784));
#162225=CARTESIAN_POINT('Ctrl Pts',(3.40022782480161,12.2,-10.2142153489442));
#162226=CARTESIAN_POINT('Ctrl Pts',(3.40217510475497,12.2,-10.2170343338259));
#162227=CARTESIAN_POINT('Ctrl Pts',(3.40413636230927,12.2,-10.2198632526979));
#162228=CARTESIAN_POINT('Ctrl Pts',(3.40611160631355,12.2,-10.222701950743));
#162229=CARTESIAN_POINT('Ctrl Pts',(3.40808685058695,12.2,-10.2255406491748));
#162230=CARTESIAN_POINT('Ctrl Pts',(3.41007608258852,12.2,-10.2283891257098));
#162231=CARTESIAN_POINT('Ctrl Pts',(3.41207930829898,12.2,-10.2312472258981));
#162232=CARTESIAN_POINT('Ctrl Pts',(3.4140825337365,12.2,-10.2341053256969));
#162233=CARTESIAN_POINT('Ctrl Pts',(3.41609975458148,12.2,-10.2369730511646));
#162234=CARTESIAN_POINT('Ctrl Pts',(3.41813097835897,12.2,-10.2398502485399));
#162235=CARTESIAN_POINT('Ctrl Pts',(3.42016220241321,12.2,-10.2427274463072));
#162236=CARTESIAN_POINT('Ctrl Pts',(3.42220742842744,12.2,-10.2456141148395));
#162237=CARTESIAN_POINT('Ctrl Pts',(3.4242666646517,12.2,-10.2485101042202));
#162238=CARTESIAN_POINT('Ctrl Pts',(3.42632590059539,12.2,-10.2514060932062));
#162239=CARTESIAN_POINT('Ctrl Pts',(3.42839914638966,12.2,-10.2543114038233));
#162240=CARTESIAN_POINT('Ctrl Pts',(3.43048640915543,12.2,-10.2572258861188));
#162241=CARTESIAN_POINT('Ctrl Pts',(3.43257367220559,12.2,-10.2601403688113));
#162242=CARTESIAN_POINT('Ctrl Pts',(3.43467495235674,12.2,-10.2630640229044));
#162243=CARTESIAN_POINT('Ctrl Pts',(3.43679025513961,12.2,-10.2659967002315));
#162244=CARTESIAN_POINT('Ctrl Pts',(3.43890555763427,12.2,-10.268929377159));
#162245=CARTESIAN_POINT('Ctrl Pts',(3.44103488317611,12.2,-10.2718710773958));
#162246=CARTESIAN_POINT('Ctrl Pts',(3.44317823766613,12.2,-10.2748216555426));
#162247=CARTESIAN_POINT('Ctrl Pts',(3.44532159244817,12.2,-10.2777722340913));
#162248=CARTESIAN_POINT('Ctrl Pts',(3.44747897522034,12.2,-10.2807316880628));
#162249=CARTESIAN_POINT('Ctrl Pts',(3.44965039329304,12.2,-10.2836998759603));
#162250=CARTESIAN_POINT('Ctrl Pts',(3.45182181106988,12.2,-10.2866680634534));
#162251=CARTESIAN_POINT('Ctrl Pts',(3.45400726117153,12.2,-10.2896449823346));
#162252=CARTESIAN_POINT('Ctrl Pts',(3.45620675165695,12.2,-10.2926304899785));
#162253=CARTESIAN_POINT('Ctrl Pts',(3.45840624244204,12.2,-10.2956159980292));
#162254=CARTESIAN_POINT('Ctrl Pts',(3.46061977099237,12.2,-10.298610094153));
#162255=CARTESIAN_POINT('Ctrl Pts',(3.46284734372488,12.2,-10.3016126379833));
#162256=CARTESIAN_POINT('Ctrl Pts',(3.4650749164574,12.2,-10.3046151818136));
#162257=CARTESIAN_POINT('Ctrl Pts',(3.46731653194711,12.2,-10.3076261708866));
#162258=CARTESIAN_POINT('Ctrl Pts',(3.46957219479369,12.2,-10.3106454662186));
#162259=CARTESIAN_POINT('Ctrl Pts',(3.47182785733294,12.2,-10.3136647611393));
#162260=CARTESIAN_POINT('Ctrl Pts',(3.47409756675805,12.2,-10.3166923611296));
#162261=CARTESIAN_POINT('Ctrl Pts',(3.47638132724833,12.2,-10.3197281275062));
#162262=CARTESIAN_POINT('Ctrl Pts',(3.47866508804978,12.2,-10.3227638942965));
#162263=CARTESIAN_POINT('Ctrl Pts',(3.48096289913657,12.2,-10.3258078278485));
#162264=CARTESIAN_POINT('Ctrl Pts',(3.48327476331955,12.2,-10.3288597880156));
#162265=CARTESIAN_POINT('Ctrl Pts',(3.48558662718754,12.2,-10.331911747767));
#162266=CARTESIAN_POINT('Ctrl Pts',(3.48791254547593,12.2,-10.3349717374172));
#162267=CARTESIAN_POINT('Ctrl Pts',(3.49025251878373,12.2,-10.3380396164993));
#162268=CARTESIAN_POINT('Ctrl Pts',(3.49259249241036,12.2,-10.3411074959993));
#162269=CARTESIAN_POINT('Ctrl Pts',(3.49494652270889,12.2,-10.3441832675219));
#162270=CARTESIAN_POINT('Ctrl Pts',(3.49731461156859,12.2,-10.3472667944558));
#162271=CARTESIAN_POINT('Ctrl Pts',(3.49968270010564,12.2,-10.3503503209696));
#162272=CARTESIAN_POINT('Ctrl Pts',(3.50206484618705,12.2,-10.3534416029506));
#162273=CARTESIAN_POINT('Ctrl Pts',(3.5044610520458,12.2,-10.3565405060301));
#162274=CARTESIAN_POINT('Ctrl Pts',(3.50745630961409,12.2,-10.3604141351961));
#162275=CARTESIAN_POINT('Ctrl Pts',(3.51047353661352,12.2,-10.364299672618));
#162276=CARTESIAN_POINT('Ctrl Pts',(3.51351273404293,12.2,-10.3681968585202));
#162277=CARTESIAN_POINT('Ctrl Pts',(3.51594409211897,12.2,-10.3713146074118));
#162278=CARTESIAN_POINT('Ctrl Pts',(3.51838951118483,12.2,-10.3744398121406));
#162279=CARTESIAN_POINT('Ctrl Pts',(3.52084899283185,12.2,-10.3775723397462));
#162280=CARTESIAN_POINT('Ctrl Pts',(3.52330847414376,12.2,-10.3807048669251));
#162281=CARTESIAN_POINT('Ctrl Pts',(3.52578201731481,12.2,-10.3838447179866));
#162282=CARTESIAN_POINT('Ctrl Pts',(3.52826962305499,12.2,-10.3869917617845));
#162283=CARTESIAN_POINT('Ctrl Pts',(3.53075722913411,12.2,-10.3901388060111));
#162284=CARTESIAN_POINT('Ctrl Pts',(3.53325889815932,12.2,-10.3932930442191));
#162285=CARTESIAN_POINT('Ctrl Pts',(3.53577462846402,12.2,-10.3964543457252));
#162286=CARTESIAN_POINT('Ctrl Pts',(3.53829035842594,12.2,-10.3996156468005));
#162287=CARTESIAN_POINT('Ctrl Pts',(3.54082015177394,12.2,-10.402784011055));
#162288=CARTESIAN_POINT('Ctrl Pts',(3.54336400684231,12.2,-10.4059593127392));
#162289=CARTESIAN_POINT('Ctrl Pts',(3.54590786225728,12.2,-10.4091346148559));
#162290=CARTESIAN_POINT('Ctrl Pts',(3.54846577876086,12.2,-10.4123168516944));
#162291=CARTESIAN_POINT('Ctrl Pts',(3.55103775746831,12.2,-10.4155058984938));
#162292=CARTESIAN_POINT('Ctrl Pts',(3.55360973582534,12.2,-10.4186949448587));
#162293=CARTESIAN_POINT('Ctrl Pts',(3.55619577523877,12.2,-10.421890800525));
#162294=CARTESIAN_POINT('Ctrl Pts',(3.55879587435811,12.2,-10.4250933389847));
#162295=CARTESIAN_POINT('Ctrl Pts',(3.56139597383172,12.2,-10.4282958778808));
#162296=CARTESIAN_POINT('Ctrl Pts',(3.56401013252331,12.2,-10.4315050999247));
#162297=CARTESIAN_POINT('Ctrl Pts',(3.56663834999989,12.2,-10.4347208807667));
#162298=CARTESIAN_POINT('Ctrl Pts',(3.56926656747646,12.2,-10.4379366616086));
#162299=CARTESIAN_POINT('Ctrl Pts',(3.57190884331856,12.2,-10.4411590006013));
#162300=CARTESIAN_POINT('Ctrl Pts',(3.57456517540921,12.2,-10.4443877747779));
#162301=CARTESIAN_POINT('Ctrl Pts',(3.57722150713793,12.2,-10.4476165485146));
#162302=CARTESIAN_POINT('Ctrl Pts',(3.57989189510259,12.2,-10.4508517564481));
#162303=CARTESIAN_POINT('Ctrl Pts',(3.5825763375064,12.2,-10.4540932775311));
#162304=CARTESIAN_POINT('Ctrl Pts',(3.58526078027596,12.2,-10.4573347990558));
#162305=CARTESIAN_POINT('Ctrl Pts',(3.58795927643857,12.2,-10.4605826325624));
#162306=CARTESIAN_POINT('Ctrl Pts',(3.59067182447673,12.2,-10.4638366562404));
#162307=CARTESIAN_POINT('Ctrl Pts',(3.5933843721453,12.2,-10.467090679475));
#162308=CARTESIAN_POINT('Ctrl Pts',(3.59611096994815,12.2,-10.4703508946199));
#162309=CARTESIAN_POINT('Ctrl Pts',(3.59885161700098,12.2,-10.4736171797414));
#162310=CARTESIAN_POINT('Ctrl Pts',(3.60159226442721,12.2,-10.4768834653079));
#162311=CARTESIAN_POINT('Ctrl Pts',(3.60434696058074,12.2,-10.4801558207883));
#162312=CARTESIAN_POINT('Ctrl Pts',(3.60711570092673,12.2,-10.4834341272424));
#162313=CARTESIAN_POINT('Ctrl Pts',(3.60988444089548,12.2,-10.4867124332498));
#162314=CARTESIAN_POINT('Ctrl Pts',(3.61266722571761,12.2,-10.4899966900893));
#162315=CARTESIAN_POINT('Ctrl Pts',(3.61546405148805,12.2,-10.4932867792644));
#162316=CARTESIAN_POINT('Ctrl Pts',(3.61826087763956,12.2,-10.4965768688878));
#162317=CARTESIAN_POINT('Ctrl Pts',(3.62107174623998,12.2,-10.499872790898));
#162318=CARTESIAN_POINT('Ctrl Pts',(3.62389665100596,12.2,-10.503174427245));
#162319=CARTESIAN_POINT('Ctrl Pts',(3.62672155538705,12.2,-10.5064760631421));
#162320=CARTESIAN_POINT('Ctrl Pts',(3.62956049568624,12.2,-10.509783414164));
#162321=CARTESIAN_POINT('Ctrl Pts',(3.63241347009432,12.2,-10.5130963635026));
#162322=CARTESIAN_POINT('Ctrl Pts',(3.63526644489112,12.2,-10.5164093132926));
#162323=CARTESIAN_POINT('Ctrl Pts',(3.63813345015262,12.2,-10.5197278611486));
#162324=CARTESIAN_POINT('Ctrl Pts',(3.64101448547721,12.2,-10.5230518914968));
#162325=CARTESIAN_POINT('Ctrl Pts',(3.64461577943667,12.2,-10.5272069292056));
#162326=CARTESIAN_POINT('Ctrl Pts',(3.64823899165949,12.2,-10.531370533428));
#162327=CARTESIAN_POINT('Ctrl Pts',(3.65188411173008,12.2,-10.5355424809979));
#162328=CARTESIAN_POINT('Ctrl Pts',(3.65480020754816,12.2,-10.5388800387809));
#162329=CARTESIAN_POINT('Ctrl Pts',(3.65773032456201,12.2,-10.5422229356683));
#162330=CARTESIAN_POINT('Ctrl Pts',(3.66067445835609,12.2,-10.5455710585059));
#162331=CARTESIAN_POINT('Ctrl Pts',(3.66288255880193,12.2,-10.5480821507481));
#162332=CARTESIAN_POINT('Ctrl Pts',(3.66509854334697,12.2,-10.5505961834098));
#162333=CARTESIAN_POINT('Ctrl Pts',(3.66732240880676,12.2,-10.553113107443));
#162334=CARTESIAN_POINT('Ctrl Pts',(3.66954627467056,12.2,-10.5556300319334));
#162335=CARTESIAN_POINT('Ctrl Pts',(3.67177802289491,12.2,-10.5581498480829));
#162336=CARTESIAN_POINT('Ctrl Pts',(3.67401764972147,12.2,-10.5606725095749));
#162337=CARTESIAN_POINT('Ctrl Pts',(3.67625727614117,12.2,-10.5631951706087));
#162338=CARTESIAN_POINT('Ctrl Pts',(3.67850478209378,12.2,-10.5657206766006));
#162339=CARTESIAN_POINT('Ctrl Pts',(3.68076016355419,12.2,-10.568248979759));
#162340=CARTESIAN_POINT('Ctrl Pts',(3.6830155450146,12.2,-10.5707772829173));
#162341=CARTESIAN_POINT('Ctrl Pts',(3.68527880354079,12.2,-10.5733083858828));
#162342=CARTESIAN_POINT('Ctrl Pts',(3.68754993546862,12.2,-10.5758422380523));
#162343=CARTESIAN_POINT('Ctrl Pts',(3.68982106739646,12.2,-10.5783760902218));
#162344=CARTESIAN_POINT('Ctrl Pts',(3.69210007333722,12.2,-10.5809126936451));
#162345=CARTESIAN_POINT('Ctrl Pts',(3.69438694976448,12.2,-10.5834520021894));
#162346=CARTESIAN_POINT('Ctrl Pts',(3.69667382619174,12.2,-10.5859913107336));
#162347=CARTESIAN_POINT('Ctrl Pts',(3.69896857461671,12.2,-10.588533323432));
#162348=CARTESIAN_POINT('Ctrl Pts',(3.70127118999071,12.2,-10.5910779949643));
#162349=CARTESIAN_POINT('Ctrl Pts',(3.7035738053647,12.2,-10.5936226664967));
#162350=CARTESIAN_POINT('Ctrl Pts',(3.70588428847979,12.2,-10.5961699971038));
#162351=CARTESIAN_POINT('Ctrl Pts',(3.70820263681116,12.2,-10.5987199397191));
#162352=CARTESIAN_POINT('Ctrl Pts',(3.71052098556369,12.2,-10.6012698827977));
#162353=CARTESIAN_POINT('Ctrl Pts',(3.71284719920176,12.2,-10.6038224389186));
#162354=CARTESIAN_POINT('Ctrl Pts',(3.71518127454206,12.2,-10.6063775615403));
#162355=CARTESIAN_POINT('Ctrl Pts',(3.71751534945832,12.2,-10.6089326836979));
#162356=CARTESIAN_POINT('Ctrl Pts',(3.71985728643833,12.2,-10.6114903737602));
#162357=CARTESIAN_POINT('Ctrl Pts',(3.72220708242959,12.2,-10.614050584962));
#162358=CARTESIAN_POINT('Ctrl Pts',(3.72455687842085,12.2,-10.6166107961639));
#162359=CARTESIAN_POINT('Ctrl Pts',(3.72691453309312,12.2,-10.6191735287393));
#162360=CARTESIAN_POINT('Ctrl Pts',(3.72928004250786,12.2,-10.621738737813));
#162361=CARTESIAN_POINT('Ctrl Pts',(3.7316455519226,12.2,-10.6243039468867));
#162362=CARTESIAN_POINT('Ctrl Pts',(3.73401891705308,12.2,-10.6268716331934));
#162363=CARTESIAN_POINT('Ctrl Pts',(3.73640013396655,12.2,-10.6294417508083));
#162364=CARTESIAN_POINT('Ctrl Pts',(3.73878135088002,12.2,-10.6320118684233));
#162365=CARTESIAN_POINT('Ctrl Pts',(3.74117042055986,12.2,-10.6345844173465));
#162366=CARTESIAN_POINT('Ctrl Pts',(3.74356733797209,12.2,-10.6371593539194));
#162367=CARTESIAN_POINT('Ctrl Pts',(3.74596425538433,12.2,-10.6397342904923));
#162368=CARTESIAN_POINT('Ctrl Pts',(3.74836902180121,12.2,-10.642311613766));
#162369=CARTESIAN_POINT('Ctrl Pts',(3.75078163324985,12.2,-10.6448912800092));
#162370=CARTESIAN_POINT('Ctrl Pts',(3.75319424469849,12.2,-10.6474709462525));
#162371=CARTESIAN_POINT('Ctrl Pts',(3.75561470032649,12.2,-10.6500529563642));
#162372=CARTESIAN_POINT('Ctrl Pts',(3.75804299769553,12.2,-10.6526372644366));
#162373=CARTESIAN_POINT('Ctrl Pts',(3.76047129550572,12.2,-10.6552215729786));
#162374=CARTESIAN_POINT('Ctrl Pts',(3.76290743595977,12.2,-10.6578081796378));
#162375=CARTESIAN_POINT('Ctrl Pts',(3.76535141277436,12.2,-10.6603970420977));
#162376=CARTESIAN_POINT('Ctrl Pts',(3.76779538914495,12.2,-10.6629859040873));
#162377=CARTESIAN_POINT('Ctrl Pts',(3.77024720295681,12.2,-10.6655770197601));
#162378=CARTESIAN_POINT('Ctrl Pts',(3.77270685078479,12.2,-10.668170347791));
#162379=CARTESIAN_POINT('Ctrl Pts',(3.77516649861278,12.2,-10.670763675822));
#162380=CARTESIAN_POINT('Ctrl Pts',(3.77763398072316,12.2,-10.6733592149277));
#162381=CARTESIAN_POINT('Ctrl Pts',(3.78010929254988,12.2,-10.6759569220417));
#162382=CARTESIAN_POINT('Ctrl Pts',(3.78258460437661,12.2,-10.6785546291556));
#162383=CARTESIAN_POINT('Ctrl Pts',(3.78506774596969,12.2,-10.6811545042945));
#162384=CARTESIAN_POINT('Ctrl Pts',(3.7875587137535,12.2,-10.6837565039497));
#162385=CARTESIAN_POINT('Ctrl Pts',(3.79004968153732,12.2,-10.686358503605));
#162386=CARTESIAN_POINT('Ctrl Pts',(3.79254847436508,12.2,-10.6889626284939));
#162387=CARTESIAN_POINT('Ctrl Pts',(3.795055089815,12.2,-10.6915688352791));
#162388=CARTESIAN_POINT('Ctrl Pts',(3.79756170526491,12.2,-10.6941750420644));
#162389=CARTESIAN_POINT('Ctrl Pts',(3.80007614280942,12.2,-10.6967833312927));
#162390=CARTESIAN_POINT('Ctrl Pts',(3.80259839721671,12.2,-10.6993936594059));
#162391=CARTESIAN_POINT('Ctrl Pts',(3.80512065208222,12.2,-10.7020039879934));
#162392=CARTESIAN_POINT('Ctrl Pts',(3.80765072504991,12.2,-10.7046163552897));
#162393=CARTESIAN_POINT('Ctrl Pts',(3.81018861179482,12.2,-10.7072307203366));
#162394=CARTESIAN_POINT('Ctrl Pts',(3.81357246001961,12.2,-10.7107165396076));
#162395=CARTESIAN_POINT('Ctrl Pts',(3.81697019802871,12.2,-10.7142059090503));
#162396=CARTESIAN_POINT('Ctrl Pts',(3.82038181697112,12.2,-10.7176987284312));
#162397=CARTESIAN_POINT('Ctrl Pts',(3.82294053129414,12.2,-10.7203183430858));
#162398=CARTESIAN_POINT('Ctrl Pts',(3.82550705281773,12.2,-10.7229398990236));
#162399=CARTESIAN_POINT('Ctrl Pts',(3.8280813782269,12.2,-10.7255633537674));
#162400=CARTESIAN_POINT('Ctrl Pts',(3.83065570363607,12.2,-10.7281868085113));
#162401=CARTESIAN_POINT('Ctrl Pts',(3.83323783246379,12.2,-10.7308121620896));
#162402=CARTESIAN_POINT('Ctrl Pts',(3.83582775974363,12.2,-10.7334393727023));
#162403=CARTESIAN_POINT('Ctrl Pts',(3.83841768749397,12.2,-10.7360665837922));
#162404=CARTESIAN_POINT('Ctrl Pts',(3.84101541335483,12.2,-10.7386956510243));
#162405=CARTESIAN_POINT('Ctrl Pts',(3.8436209345679,12.2,-10.7413265355319));
#162406=CARTESIAN_POINT('Ctrl Pts',(3.84622645530763,12.2,-10.7439574195615));
#162407=CARTESIAN_POINT('Ctrl Pts',(3.84883976926361,12.2,-10.7465901190494));
#162408=CARTESIAN_POINT('Ctrl Pts',(3.85146087354406,12.2,-10.7492245946205));
#162409=CARTESIAN_POINT('Ctrl Pts',(3.8540819778245,12.2,-10.7518590701916));
#162410=CARTESIAN_POINT('Ctrl Pts',(3.85671087190274,12.2,-10.7544953205363));
#162411=CARTESIAN_POINT('Ctrl Pts',(3.85934755027728,12.2,-10.7571333042024));
#162412=CARTESIAN_POINT('Ctrl Pts',(3.86286312128368,12.2,-10.7606506155975));
#162413=CARTESIAN_POINT('Ctrl Pts',(3.8663925313172,12.2,-10.7641710081345));
#162414=CARTESIAN_POINT('Ctrl Pts',(3.86993577013724,12.2,-10.7676943829573));
#162415=CARTESIAN_POINT('Ctrl Pts',(3.87259319985574,12.2,-10.7703369146744));
#162416=CARTESIAN_POINT('Ctrl Pts',(3.87525840755974,12.2,-10.772981125142));
#162417=CARTESIAN_POINT('Ctrl Pts',(3.87793138932427,12.2,-10.7756269783185));
#162418=CARTESIAN_POINT('Ctrl Pts',(3.88060437060321,12.2,-10.7782728310142));
#162419=CARTESIAN_POINT('Ctrl Pts',(3.88328512549008,12.2,-10.7809203259849));
#162420=CARTESIAN_POINT('Ctrl Pts',(3.88597364926807,12.2,-10.7835694224721));
#162421=CARTESIAN_POINT('Ctrl Pts',(3.88866217304606,12.2,-10.7862185189593));
#162422=CARTESIAN_POINT('Ctrl Pts',(3.89135846522161,12.2,-10.7888692159367));
#162423=CARTESIAN_POINT('Ctrl Pts',(3.89406251996902,12.2,-10.7915214620607));
#162424=CARTESIAN_POINT('Ctrl Pts',(3.89676657471642,12.2,-10.7941737081848));
#162425=CARTESIAN_POINT('Ctrl Pts',(3.89947839156725,12.2,-10.796827503932));
#162426=CARTESIAN_POINT('Ctrl Pts',(3.90219796677242,12.2,-10.7994828125143));
#162427=CARTESIAN_POINT('Ctrl Pts',(3.90673059227906,12.2,-10.8039083269788));
#162428=CARTESIAN_POINT('Ctrl Pts',(3.91128476133577,12.2,-10.8083380407001));
#162429=CARTESIAN_POINT('Ctrl Pts',(3.91586047899994,12.2,-10.812771925));
#162430=CARTESIAN_POINT('Ctrl Pts',(4.27433546799994,15.2,-10.676144262));
#162431=CARTESIAN_POINT('Ctrl Pts',(4.27433546799994,11.6,-10.676144262));
#162432=CARTESIAN_POINT('Ctrl Pts',(4.27439112799994,15.2,-10.675381706));
#162433=CARTESIAN_POINT('Ctrl Pts',(4.27439112799994,11.6,-10.675381706));
#162434=CARTESIAN_POINT('Ctrl Pts',(4.27450212599994,15.2,-10.673857013));
#162435=CARTESIAN_POINT('Ctrl Pts',(4.27450212599994,11.6,-10.673857013));
#162436=CARTESIAN_POINT('Ctrl Pts',(4.27466766699994,15.2,-10.671571231));
#162437=CARTESIAN_POINT('Ctrl Pts',(4.27466766699994,11.6,-10.671571231));
#162438=CARTESIAN_POINT('Ctrl Pts',(4.27488647299994,15.2,-10.668526034));
#162439=CARTESIAN_POINT('Ctrl Pts',(4.27488647299994,11.6,-10.668526034));
#162440=CARTESIAN_POINT('Ctrl Pts',(4.27515678899994,15.2,-10.664723728));
#162441=CARTESIAN_POINT('Ctrl Pts',(4.27515678899994,11.6,-10.664723728));
#162442=CARTESIAN_POINT('Ctrl Pts',(4.27542391299994,15.2,-10.660925613));
#162443=CARTESIAN_POINT('Ctrl Pts',(4.27542391299994,11.6,-10.660925613));
#162444=CARTESIAN_POINT('Ctrl Pts',(4.27568784799994,15.2,-10.65713169));
#162445=CARTESIAN_POINT('Ctrl Pts',(4.27568784799994,11.6,-10.65713169));
#162446=CARTESIAN_POINT('Ctrl Pts',(4.27594859599994,15.2,-10.653341964));
#162447=CARTESIAN_POINT('Ctrl Pts',(4.27594859599994,11.6,-10.653341964));
#162448=CARTESIAN_POINT('Ctrl Pts',(4.27620615899994,15.2,-10.649556439));
#162449=CARTESIAN_POINT('Ctrl Pts',(4.27620615899994,11.6,-10.649556439));
#162450=CARTESIAN_POINT('Ctrl Pts',(4.27646054199994,15.2,-10.645775121));
#162451=CARTESIAN_POINT('Ctrl Pts',(4.27646054199994,11.6,-10.645775121));
#162452=CARTESIAN_POINT('Ctrl Pts',(4.27671175199994,15.2,-10.641998021));
#162453=CARTESIAN_POINT('Ctrl Pts',(4.27671175199994,11.6,-10.641998021));
#162454=CARTESIAN_POINT('Ctrl Pts',(4.27695979299994,15.2,-10.638225143));
#162455=CARTESIAN_POINT('Ctrl Pts',(4.27695979299994,11.6,-10.638225143));
#162456=CARTESIAN_POINT('Ctrl Pts',(4.27720467299994,15.2,-10.6344565));
#162457=CARTESIAN_POINT('Ctrl Pts',(4.27720467299994,11.6,-10.6344565));
#162458=CARTESIAN_POINT('Ctrl Pts',(4.27744639699995,15.2,-10.630692101));
#162459=CARTESIAN_POINT('Ctrl Pts',(4.27744639699995,11.6,-10.630692101));
#162460=CARTESIAN_POINT('Ctrl Pts',(4.27768497199995,15.2,-10.626931954));
#162461=CARTESIAN_POINT('Ctrl Pts',(4.27768497199995,11.6,-10.626931954));
#162462=CARTESIAN_POINT('Ctrl Pts',(4.27792040199994,15.2,-10.623176065));
#162463=CARTESIAN_POINT('Ctrl Pts',(4.27792040199994,11.6,-10.623176065));
#162464=CARTESIAN_POINT('Ctrl Pts',(4.27815269399995,15.2,-10.619424443));
#162465=CARTESIAN_POINT('Ctrl Pts',(4.27815269399995,11.6,-10.619424443));
#162466=CARTESIAN_POINT('Ctrl Pts',(4.27838185099994,15.2,-10.615677095));
#162467=CARTESIAN_POINT('Ctrl Pts',(4.27838185099994,11.6,-10.615677095));
#162468=CARTESIAN_POINT('Ctrl Pts',(4.27860787799994,15.2,-10.611934026));
#162469=CARTESIAN_POINT('Ctrl Pts',(4.27860787799994,11.6,-10.611934026));
#162470=CARTESIAN_POINT('Ctrl Pts',(4.27883078099994,15.2,-10.608195244));
#162471=CARTESIAN_POINT('Ctrl Pts',(4.27883078099994,11.6,-10.608195244));
#162472=CARTESIAN_POINT('Ctrl Pts',(4.27905056299995,15.2,-10.604460756));
#162473=CARTESIAN_POINT('Ctrl Pts',(4.27905056299995,11.6,-10.604460756));
#162474=CARTESIAN_POINT('Ctrl Pts',(4.27926722999994,15.2,-10.600730569));
#162475=CARTESIAN_POINT('Ctrl Pts',(4.27926722999994,11.6,-10.600730569));
#162476=CARTESIAN_POINT('Ctrl Pts',(4.27948078599994,15.2,-10.59700469));
#162477=CARTESIAN_POINT('Ctrl Pts',(4.27948078599994,11.6,-10.59700469));
#162478=CARTESIAN_POINT('Ctrl Pts',(4.27969123899994,15.2,-10.593283128));
#162479=CARTESIAN_POINT('Ctrl Pts',(4.27969123899994,11.6,-10.593283128));
#162480=CARTESIAN_POINT('Ctrl Pts',(4.27989859299994,15.2,-10.589565891));
#162481=CARTESIAN_POINT('Ctrl Pts',(4.27989859299994,11.6,-10.589565891));
#162482=CARTESIAN_POINT('Ctrl Pts',(4.28010285399994,15.2,-10.585852985));
#162483=CARTESIAN_POINT('Ctrl Pts',(4.28010285399994,11.6,-10.585852985));
#162484=CARTESIAN_POINT('Ctrl Pts',(4.28030402699994,15.2,-10.58214442));
#162485=CARTESIAN_POINT('Ctrl Pts',(4.28030402699994,11.6,-10.58214442));
#162486=CARTESIAN_POINT('Ctrl Pts',(4.28050211699994,15.2,-10.578440202));
#162487=CARTESIAN_POINT('Ctrl Pts',(4.28050211699994,11.6,-10.578440202));
#162488=CARTESIAN_POINT('Ctrl Pts',(4.28069712999995,15.2,-10.574740338));
#162489=CARTESIAN_POINT('Ctrl Pts',(4.28069712999995,11.6,-10.574740338));
#162490=CARTESIAN_POINT('Ctrl Pts',(4.28088907099994,15.2,-10.571044837));
#162491=CARTESIAN_POINT('Ctrl Pts',(4.28088907099994,11.6,-10.571044837));
#162492=CARTESIAN_POINT('Ctrl Pts',(4.28107794499994,15.2,-10.567353704));
#162493=CARTESIAN_POINT('Ctrl Pts',(4.28107794499994,11.6,-10.567353704));
#162494=CARTESIAN_POINT('Ctrl Pts',(4.28126375699994,15.2,-10.563666949));
#162495=CARTESIAN_POINT('Ctrl Pts',(4.28126375699994,11.6,-10.563666949));
#162496=CARTESIAN_POINT('Ctrl Pts',(4.28144651399994,15.2,-10.559984579));
#162497=CARTESIAN_POINT('Ctrl Pts',(4.28144651399994,11.6,-10.559984579));
#162498=CARTESIAN_POINT('Ctrl Pts',(4.28162621799994,15.2,-10.5563066));
#162499=CARTESIAN_POINT('Ctrl Pts',(4.28162621799994,11.6,-10.5563066));
#162500=CARTESIAN_POINT('Ctrl Pts',(4.28180287799994,15.2,-10.552633021));
#162501=CARTESIAN_POINT('Ctrl Pts',(4.28180287799994,11.6,-10.552633021));
#162502=CARTESIAN_POINT('Ctrl Pts',(4.28197649799994,15.2,-10.548963849));
#162503=CARTESIAN_POINT('Ctrl Pts',(4.28197649799994,11.6,-10.548963849));
#162504=CARTESIAN_POINT('Ctrl Pts',(4.28214708299994,15.2,-10.545299093));
#162505=CARTESIAN_POINT('Ctrl Pts',(4.28214708299994,11.6,-10.545299093));
#162506=CARTESIAN_POINT('Ctrl Pts',(4.28231463999994,15.2,-10.541638759));
#162507=CARTESIAN_POINT('Ctrl Pts',(4.28231463999994,11.6,-10.541638759));
#162508=CARTESIAN_POINT('Ctrl Pts',(4.28247917299994,15.2,-10.537982854));
#162509=CARTESIAN_POINT('Ctrl Pts',(4.28247917299994,11.6,-10.537982854));
#162510=CARTESIAN_POINT('Ctrl Pts',(4.28264068799994,15.2,-10.534331388));
#162511=CARTESIAN_POINT('Ctrl Pts',(4.28264068799994,11.6,-10.534331388));
#162512=CARTESIAN_POINT('Ctrl Pts',(4.28279918999994,15.2,-10.530684367));
#162513=CARTESIAN_POINT('Ctrl Pts',(4.28279918999994,11.6,-10.530684367));
#162514=CARTESIAN_POINT('Ctrl Pts',(4.28295468599994,15.2,-10.5270418));
#162515=CARTESIAN_POINT('Ctrl Pts',(4.28295468599994,11.6,-10.5270418));
#162516=CARTESIAN_POINT('Ctrl Pts',(4.28310717999994,15.2,-10.523403692));
#162517=CARTESIAN_POINT('Ctrl Pts',(4.28310717999994,11.6,-10.523403692));
#162518=CARTESIAN_POINT('Ctrl Pts',(4.28325667799994,15.2,-10.519770053));
#162519=CARTESIAN_POINT('Ctrl Pts',(4.28325667799994,11.6,-10.519770053));
#162520=CARTESIAN_POINT('Ctrl Pts',(4.28340318699994,15.2,-10.51614089));
#162521=CARTESIAN_POINT('Ctrl Pts',(4.28340318699994,11.6,-10.51614089));
#162522=CARTESIAN_POINT('Ctrl Pts',(4.28354670899994,15.2,-10.512516211));
#162523=CARTESIAN_POINT('Ctrl Pts',(4.28354670899994,11.6,-10.512516211));
#162524=CARTESIAN_POINT('Ctrl Pts',(4.28368725299995,15.2,-10.508896023));
#162525=CARTESIAN_POINT('Ctrl Pts',(4.28368725299995,11.6,-10.508896023));
#162526=CARTESIAN_POINT('Ctrl Pts',(4.28382482299994,15.2,-10.505280333));
#162527=CARTESIAN_POINT('Ctrl Pts',(4.28382482299994,11.6,-10.505280333));
#162528=CARTESIAN_POINT('Ctrl Pts',(4.28395942599994,15.2,-10.501669151));
#162529=CARTESIAN_POINT('Ctrl Pts',(4.28395942599994,11.6,-10.501669151));
#162530=CARTESIAN_POINT('Ctrl Pts',(4.28409106599995,15.2,-10.498062482));
#162531=CARTESIAN_POINT('Ctrl Pts',(4.28409106599995,11.6,-10.498062482));
#162532=CARTESIAN_POINT('Ctrl Pts',(4.28421974899994,15.2,-10.494460336));
#162533=CARTESIAN_POINT('Ctrl Pts',(4.28421974899994,11.6,-10.494460336));
#162534=CARTESIAN_POINT('Ctrl Pts',(4.28434548199994,15.2,-10.490862719));
#162535=CARTESIAN_POINT('Ctrl Pts',(4.28434548199994,11.6,-10.490862719));
#162536=CARTESIAN_POINT('Ctrl Pts',(4.28446826999994,15.2,-10.48726964));
#162537=CARTESIAN_POINT('Ctrl Pts',(4.28446826999994,11.6,-10.48726964));
#162538=CARTESIAN_POINT('Ctrl Pts',(4.28458811799994,15.2,-10.483681106));
#162539=CARTESIAN_POINT('Ctrl Pts',(4.28458811799994,11.6,-10.483681106));
#162540=CARTESIAN_POINT('Ctrl Pts',(4.28470503199994,15.2,-10.480097126));
#162541=CARTESIAN_POINT('Ctrl Pts',(4.28470503199994,11.6,-10.480097126));
#162542=CARTESIAN_POINT('Ctrl Pts',(4.28481901899994,15.2,-10.476517706));
#162543=CARTESIAN_POINT('Ctrl Pts',(4.28481901899994,11.6,-10.476517706));
#162544=CARTESIAN_POINT('Ctrl Pts',(4.28493008199994,15.2,-10.472942854));
#162545=CARTESIAN_POINT('Ctrl Pts',(4.28493008199994,11.6,-10.472942854));
#162546=CARTESIAN_POINT('Ctrl Pts',(4.28503822999994,15.2,-10.469372579));
#162547=CARTESIAN_POINT('Ctrl Pts',(4.28503822999994,11.6,-10.469372579));
#162548=CARTESIAN_POINT('Ctrl Pts',(4.28514346699994,15.2,-10.465806888));
#162549=CARTESIAN_POINT('Ctrl Pts',(4.28514346699994,11.6,-10.465806888));
#162550=CARTESIAN_POINT('Ctrl Pts',(4.28524579799994,15.2,-10.462245789));
#162551=CARTESIAN_POINT('Ctrl Pts',(4.28524579799994,11.6,-10.462245789));
#162552=CARTESIAN_POINT('Ctrl Pts',(4.28534523099994,15.2,-10.458689288));
#162553=CARTESIAN_POINT('Ctrl Pts',(4.28534523099994,11.6,-10.458689288));
#162554=CARTESIAN_POINT('Ctrl Pts',(4.28544177099994,15.2,-10.455137397));
#162555=CARTESIAN_POINT('Ctrl Pts',(4.28544177099994,11.6,-10.455137397));
#162556=CARTESIAN_POINT('Ctrl Pts',(4.28553542399994,15.2,-10.451590119));
#162557=CARTESIAN_POINT('Ctrl Pts',(4.28553542399994,11.6,-10.451590119));
#162558=CARTESIAN_POINT('Ctrl Pts',(4.28562619399994,15.2,-10.448047466));
#162559=CARTESIAN_POINT('Ctrl Pts',(4.28562619399994,11.6,-10.448047466));
#162560=CARTESIAN_POINT('Ctrl Pts',(4.28571408899994,15.2,-10.444509443));
#162561=CARTESIAN_POINT('Ctrl Pts',(4.28571408899994,11.6,-10.444509443));
#162562=CARTESIAN_POINT('Ctrl Pts',(4.28579911599994,15.2,-10.440976059));
#162563=CARTESIAN_POINT('Ctrl Pts',(4.28579911599994,11.6,-10.440976059));
#162564=CARTESIAN_POINT('Ctrl Pts',(4.28588127799994,15.2,-10.437447322));
#162565=CARTESIAN_POINT('Ctrl Pts',(4.28588127799994,11.6,-10.437447322));
#162566=CARTESIAN_POINT('Ctrl Pts',(4.28596058199994,15.2,-10.43392324));
#162567=CARTESIAN_POINT('Ctrl Pts',(4.28596058199994,11.6,-10.43392324));
#162568=CARTESIAN_POINT('Ctrl Pts',(4.28603703499994,15.2,-10.430403819));
#162569=CARTESIAN_POINT('Ctrl Pts',(4.28603703499994,11.6,-10.430403819));
#162570=CARTESIAN_POINT('Ctrl Pts',(4.28611064099994,15.2,-10.426889069));
#162571=CARTESIAN_POINT('Ctrl Pts',(4.28611064099994,11.6,-10.426889069));
#162572=CARTESIAN_POINT('Ctrl Pts',(4.28618140799994,15.2,-10.423378997));
#162573=CARTESIAN_POINT('Ctrl Pts',(4.28618140799994,11.6,-10.423378997));
#162574=CARTESIAN_POINT('Ctrl Pts',(4.28624934099994,15.2,-10.419873612));
#162575=CARTESIAN_POINT('Ctrl Pts',(4.28624934099994,11.6,-10.419873612));
#162576=CARTESIAN_POINT('Ctrl Pts',(4.28631444799994,15.2,-10.41637292));
#162577=CARTESIAN_POINT('Ctrl Pts',(4.28631444799994,11.6,-10.41637292));
#162578=CARTESIAN_POINT('Ctrl Pts',(4.28637673099994,15.2,-10.41287693));
#162579=CARTESIAN_POINT('Ctrl Pts',(4.28637673099994,11.6,-10.41287693));
#162580=CARTESIAN_POINT('Ctrl Pts',(4.28643619899994,15.2,-10.40938565));
#162581=CARTESIAN_POINT('Ctrl Pts',(4.28643619899994,11.6,-10.40938565));
#162582=CARTESIAN_POINT('Ctrl Pts',(4.28649285899994,15.2,-10.405899088));
#162583=CARTESIAN_POINT('Ctrl Pts',(4.28649285899994,11.6,-10.405899088));
#162584=CARTESIAN_POINT('Ctrl Pts',(4.28654671399994,15.2,-10.402417252));
#162585=CARTESIAN_POINT('Ctrl Pts',(4.28654671399994,11.6,-10.402417252));
#162586=CARTESIAN_POINT('Ctrl Pts',(4.28659777199994,15.2,-10.398940149));
#162587=CARTESIAN_POINT('Ctrl Pts',(4.28659777199994,11.6,-10.398940149));
#162588=CARTESIAN_POINT('Ctrl Pts',(4.28664603899994,15.2,-10.395467789));
#162589=CARTESIAN_POINT('Ctrl Pts',(4.28664603899994,11.6,-10.395467789));
#162590=CARTESIAN_POINT('Ctrl Pts',(4.28669152099994,15.2,-10.392000178));
#162591=CARTESIAN_POINT('Ctrl Pts',(4.28669152099994,11.6,-10.392000178));
#162592=CARTESIAN_POINT('Ctrl Pts',(4.28673422399994,15.2,-10.388537325));
#162593=CARTESIAN_POINT('Ctrl Pts',(4.28673422399994,11.6,-10.388537325));
#162594=CARTESIAN_POINT('Ctrl Pts',(4.28677415499994,15.2,-10.385079237));
#162595=CARTESIAN_POINT('Ctrl Pts',(4.28677415499994,11.6,-10.385079237));
#162596=CARTESIAN_POINT('Ctrl Pts',(4.28681131899994,15.2,-10.381625923));
#162597=CARTESIAN_POINT('Ctrl Pts',(4.28681131899994,11.6,-10.381625923));
#162598=CARTESIAN_POINT('Ctrl Pts',(4.28684572299994,15.2,-10.378177391));
#162599=CARTESIAN_POINT('Ctrl Pts',(4.28684572299994,11.6,-10.378177391));
#162600=CARTESIAN_POINT('Ctrl Pts',(4.28687737399994,15.2,-10.374733649));
#162601=CARTESIAN_POINT('Ctrl Pts',(4.28687737399994,11.6,-10.374733649));
#162602=CARTESIAN_POINT('Ctrl Pts',(4.28690627599994,15.2,-10.371294704));
#162603=CARTESIAN_POINT('Ctrl Pts',(4.28690627599994,11.6,-10.371294704));
#162604=CARTESIAN_POINT('Ctrl Pts',(4.28693243799994,15.2,-10.367860566));
#162605=CARTESIAN_POINT('Ctrl Pts',(4.28693243799994,11.6,-10.367860566));
#162606=CARTESIAN_POINT('Ctrl Pts',(4.28695586299995,15.2,-10.364431241));
#162607=CARTESIAN_POINT('Ctrl Pts',(4.28695586299995,11.6,-10.364431241));
#162608=CARTESIAN_POINT('Ctrl Pts',(4.28697656099994,15.2,-10.361006739));
#162609=CARTESIAN_POINT('Ctrl Pts',(4.28697656099994,11.6,-10.361006739));
#162610=CARTESIAN_POINT('Ctrl Pts',(4.28699453599994,15.2,-10.357587066));
#162611=CARTESIAN_POINT('Ctrl Pts',(4.28699453599994,11.6,-10.357587066));
#162612=CARTESIAN_POINT('Ctrl Pts',(4.28700979599994,15.2,-10.354172232));
#162613=CARTESIAN_POINT('Ctrl Pts',(4.28700979599994,11.6,-10.354172232));
#162614=CARTESIAN_POINT('Ctrl Pts',(4.28702234599994,15.2,-10.350762244));
#162615=CARTESIAN_POINT('Ctrl Pts',(4.28702234599994,11.6,-10.350762244));
#162616=CARTESIAN_POINT('Ctrl Pts',(4.28703219199994,15.2,-10.34735711));
#162617=CARTESIAN_POINT('Ctrl Pts',(4.28703219199994,11.6,-10.34735711));
#162618=CARTESIAN_POINT('Ctrl Pts',(4.28703934099994,15.2,-10.343956839));
#162619=CARTESIAN_POINT('Ctrl Pts',(4.28703934099994,11.6,-10.343956839));
#162620=CARTESIAN_POINT('Ctrl Pts',(4.28704380099994,15.2,-10.340561439));
#162621=CARTESIAN_POINT('Ctrl Pts',(4.28704380099994,11.6,-10.340561439));
#162622=CARTESIAN_POINT('Ctrl Pts',(4.28704557599994,15.2,-10.337170918));
#162623=CARTESIAN_POINT('Ctrl Pts',(4.28704557599994,11.6,-10.337170918));
#162624=CARTESIAN_POINT('Ctrl Pts',(4.28704467399994,15.2,-10.333785284));
#162625=CARTESIAN_POINT('Ctrl Pts',(4.28704467399994,11.6,-10.333785284));
#162626=CARTESIAN_POINT('Ctrl Pts',(4.28704110099994,15.2,-10.330404544));
#162627=CARTESIAN_POINT('Ctrl Pts',(4.28704110099994,11.6,-10.330404544));
#162628=CARTESIAN_POINT('Ctrl Pts',(4.28703486299994,15.2,-10.327028709));
#162629=CARTESIAN_POINT('Ctrl Pts',(4.28703486299994,11.6,-10.327028709));
#162630=CARTESIAN_POINT('Ctrl Pts',(4.28702596899995,15.2,-10.323657784));
#162631=CARTESIAN_POINT('Ctrl Pts',(4.28702596899995,11.6,-10.323657784));
#162632=CARTESIAN_POINT('Ctrl Pts',(4.28701442199994,15.2,-10.320291779));
#162633=CARTESIAN_POINT('Ctrl Pts',(4.28701442199994,11.6,-10.320291779));
#162634=CARTESIAN_POINT('Ctrl Pts',(4.28700022999995,15.2,-10.316930704));
#162635=CARTESIAN_POINT('Ctrl Pts',(4.28700022999995,11.6,-10.316930704));
#162636=CARTESIAN_POINT('Ctrl Pts',(4.28698340099994,15.2,-10.313574564));
#162637=CARTESIAN_POINT('Ctrl Pts',(4.28698340099994,11.6,-10.313574564));
#162638=CARTESIAN_POINT('Ctrl Pts',(4.28696393999994,15.2,-10.310223367));
#162639=CARTESIAN_POINT('Ctrl Pts',(4.28696393999994,11.6,-10.310223367));
#162640=CARTESIAN_POINT('Ctrl Pts',(4.28694185399995,15.2,-10.306877123));
#162641=CARTESIAN_POINT('Ctrl Pts',(4.28694185399995,11.6,-10.306877123));
#162642=CARTESIAN_POINT('Ctrl Pts',(4.28691714999994,15.2,-10.303535842));
#162643=CARTESIAN_POINT('Ctrl Pts',(4.28691714999994,11.6,-10.303535842));
#162644=CARTESIAN_POINT('Ctrl Pts',(4.28688983399994,15.2,-10.300199528));
#162645=CARTESIAN_POINT('Ctrl Pts',(4.28688983399994,11.6,-10.300199528));
#162646=CARTESIAN_POINT('Ctrl Pts',(4.28685991299994,15.2,-10.296868192));
#162647=CARTESIAN_POINT('Ctrl Pts',(4.28685991299994,11.6,-10.296868192));
#162648=CARTESIAN_POINT('Ctrl Pts',(4.28682739499994,15.2,-10.293541843));
#162649=CARTESIAN_POINT('Ctrl Pts',(4.28682739499994,11.6,-10.293541843));
#162650=CARTESIAN_POINT('Ctrl Pts',(4.28679228399994,15.2,-10.290220487));
#162651=CARTESIAN_POINT('Ctrl Pts',(4.28679228399994,11.6,-10.290220487));
#162652=CARTESIAN_POINT('Ctrl Pts',(4.28675458899994,15.2,-10.286904133));
#162653=CARTESIAN_POINT('Ctrl Pts',(4.28675458899994,11.6,-10.286904133));
#162654=CARTESIAN_POINT('Ctrl Pts',(4.28671431599995,15.2,-10.283592791));
#162655=CARTESIAN_POINT('Ctrl Pts',(4.28671431599995,11.6,-10.283592791));
#162656=CARTESIAN_POINT('Ctrl Pts',(4.28667147199994,15.2,-10.280286467));
#162657=CARTESIAN_POINT('Ctrl Pts',(4.28667147199994,11.6,-10.280286467));
#162658=CARTESIAN_POINT('Ctrl Pts',(4.28662606299994,15.2,-10.276985171));
#162659=CARTESIAN_POINT('Ctrl Pts',(4.28662606299994,11.6,-10.276985171));
#162660=CARTESIAN_POINT('Ctrl Pts',(4.28657809699994,15.2,-10.273688909));
#162661=CARTESIAN_POINT('Ctrl Pts',(4.28657809699994,11.6,-10.273688909));
#162662=CARTESIAN_POINT('Ctrl Pts',(4.28652757999994,15.2,-10.270397694));
#162663=CARTESIAN_POINT('Ctrl Pts',(4.28652757999994,11.6,-10.270397694));
#162664=CARTESIAN_POINT('Ctrl Pts',(4.28647451899994,15.2,-10.26711153));
#162665=CARTESIAN_POINT('Ctrl Pts',(4.28647451899994,11.6,-10.26711153));
#162666=CARTESIAN_POINT('Ctrl Pts',(4.28641892199995,15.2,-10.263830426));
#162667=CARTESIAN_POINT('Ctrl Pts',(4.28641892199995,11.6,-10.263830426));
#162668=CARTESIAN_POINT('Ctrl Pts',(4.28636079499995,15.2,-10.260554392));
#162669=CARTESIAN_POINT('Ctrl Pts',(4.28636079499995,11.6,-10.260554392));
#162670=CARTESIAN_POINT('Ctrl Pts',(4.28630014399995,15.2,-10.257283436));
#162671=CARTESIAN_POINT('Ctrl Pts',(4.28630014399995,11.6,-10.257283436));
#162672=CARTESIAN_POINT('Ctrl Pts',(4.28623697699994,15.2,-10.254017565));
#162673=CARTESIAN_POINT('Ctrl Pts',(4.28623697699994,11.6,-10.254017565));
#162674=CARTESIAN_POINT('Ctrl Pts',(4.28617130099994,15.2,-10.25075679));
#162675=CARTESIAN_POINT('Ctrl Pts',(4.28617130099994,11.6,-10.25075679));
#162676=CARTESIAN_POINT('Ctrl Pts',(4.28610312299995,15.2,-10.247501117));
#162677=CARTESIAN_POINT('Ctrl Pts',(4.28610312299995,11.6,-10.247501117));
#162678=CARTESIAN_POINT('Ctrl Pts',(4.28603244999994,15.2,-10.244250556));
#162679=CARTESIAN_POINT('Ctrl Pts',(4.28603244999994,11.6,-10.244250556));
#162680=CARTESIAN_POINT('Ctrl Pts',(4.28595928899994,15.2,-10.241005114));
#162681=CARTESIAN_POINT('Ctrl Pts',(4.28595928899994,11.6,-10.241005114));
#162682=CARTESIAN_POINT('Ctrl Pts',(4.28588364699994,15.2,-10.237764801));
#162683=CARTESIAN_POINT('Ctrl Pts',(4.28588364699994,11.6,-10.237764801));
#162684=CARTESIAN_POINT('Ctrl Pts',(4.28580552999995,15.2,-10.234529625));
#162685=CARTESIAN_POINT('Ctrl Pts',(4.28580552999995,11.6,-10.234529625));
#162686=CARTESIAN_POINT('Ctrl Pts',(4.28572494699995,15.2,-10.231299594));
#162687=CARTESIAN_POINT('Ctrl Pts',(4.28572494699995,11.6,-10.231299594));
#162688=CARTESIAN_POINT('Ctrl Pts',(4.28564190399995,15.2,-10.228074718));
#162689=CARTESIAN_POINT('Ctrl Pts',(4.28564190399995,11.6,-10.228074718));
#162690=CARTESIAN_POINT('Ctrl Pts',(4.28555640899994,15.2,-10.224855003));
#162691=CARTESIAN_POINT('Ctrl Pts',(4.28555640899994,11.6,-10.224855003));
#162692=CARTESIAN_POINT('Ctrl Pts',(4.28546846799994,15.2,-10.22164046));
#162693=CARTESIAN_POINT('Ctrl Pts',(4.28546846799994,11.6,-10.22164046));
#162694=CARTESIAN_POINT('Ctrl Pts',(4.28537808899994,15.2,-10.218431097));
#162695=CARTESIAN_POINT('Ctrl Pts',(4.28537808899994,11.6,-10.218431097));
#162696=CARTESIAN_POINT('Ctrl Pts',(4.28528527899994,15.2,-10.215226921));
#162697=CARTESIAN_POINT('Ctrl Pts',(4.28528527899994,11.6,-10.215226921));
#162698=CARTESIAN_POINT('Ctrl Pts',(4.28519004399995,15.2,-10.212027942));
#162699=CARTESIAN_POINT('Ctrl Pts',(4.28519004399995,11.6,-10.212027942));
#162700=CARTESIAN_POINT('Ctrl Pts',(4.28509239399994,15.2,-10.208834168));
#162701=CARTESIAN_POINT('Ctrl Pts',(4.28509239399994,11.6,-10.208834168));
#162702=CARTESIAN_POINT('Ctrl Pts',(4.28499233399994,15.2,-10.205645608));
#162703=CARTESIAN_POINT('Ctrl Pts',(4.28499233399994,11.6,-10.205645608));
#162704=CARTESIAN_POINT('Ctrl Pts',(4.28488987199994,15.2,-10.20246227));
#162705=CARTESIAN_POINT('Ctrl Pts',(4.28488987199994,11.6,-10.20246227));
#162706=CARTESIAN_POINT('Ctrl Pts',(4.28478501599994,15.2,-10.199284164));
#162707=CARTESIAN_POINT('Ctrl Pts',(4.28478501599994,11.6,-10.199284164));
#162708=CARTESIAN_POINT('Ctrl Pts',(4.28467777299994,15.2,-10.196111298));
#162709=CARTESIAN_POINT('Ctrl Pts',(4.28467777299994,11.6,-10.196111298));
#162710=CARTESIAN_POINT('Ctrl Pts',(4.28456814799994,15.2,-10.19294368));
#162711=CARTESIAN_POINT('Ctrl Pts',(4.28456814799994,11.6,-10.19294368));
#162712=CARTESIAN_POINT('Ctrl Pts',(4.28445615199994,15.2,-10.189781319));
#162713=CARTESIAN_POINT('Ctrl Pts',(4.28445615199994,11.6,-10.189781319));
#162714=CARTESIAN_POINT('Ctrl Pts',(4.28434179099995,15.2,-10.186624223));
#162715=CARTESIAN_POINT('Ctrl Pts',(4.28434179099995,11.6,-10.186624223));
#162716=CARTESIAN_POINT('Ctrl Pts',(4.28422507099994,15.2,-10.183472403));
#162717=CARTESIAN_POINT('Ctrl Pts',(4.28422507099994,11.6,-10.183472403));
#162718=CARTESIAN_POINT('Ctrl Pts',(4.28410600199994,15.2,-10.180325865));
#162719=CARTESIAN_POINT('Ctrl Pts',(4.28410600199994,11.6,-10.180325865));
#162720=CARTESIAN_POINT('Ctrl Pts',(4.28398458899994,15.2,-10.177184619));
#162721=CARTESIAN_POINT('Ctrl Pts',(4.28398458899994,11.6,-10.177184619));
#162722=CARTESIAN_POINT('Ctrl Pts',(4.28386084099994,15.2,-10.174048674));
#162723=CARTESIAN_POINT('Ctrl Pts',(4.28386084099994,11.6,-10.174048674));
#162724=CARTESIAN_POINT('Ctrl Pts',(4.28373476599995,15.2,-10.170918038));
#162725=CARTESIAN_POINT('Ctrl Pts',(4.28373476599995,11.6,-10.170918038));
#162726=CARTESIAN_POINT('Ctrl Pts',(4.28360636999995,15.2,-10.16779272));
#162727=CARTESIAN_POINT('Ctrl Pts',(4.28360636999995,11.6,-10.16779272));
#162728=CARTESIAN_POINT('Ctrl Pts',(4.28347566099994,15.2,-10.16467273));
#162729=CARTESIAN_POINT('Ctrl Pts',(4.28347566099994,11.6,-10.16467273));
#162730=CARTESIAN_POINT('Ctrl Pts',(4.28334264699994,15.2,-10.161558075));
#162731=CARTESIAN_POINT('Ctrl Pts',(4.28334264699994,11.6,-10.161558075));
#162732=CARTESIAN_POINT('Ctrl Pts',(4.28320733599994,15.2,-10.158448763));
#162733=CARTESIAN_POINT('Ctrl Pts',(4.28320733599994,11.6,-10.158448763));
#162734=CARTESIAN_POINT('Ctrl Pts',(4.28306973599994,15.2,-10.155344806));
#162735=CARTESIAN_POINT('Ctrl Pts',(4.28306973599994,11.6,-10.155344806));
#162736=CARTESIAN_POINT('Ctrl Pts',(4.28292985199994,15.2,-10.152246211));
#162737=CARTESIAN_POINT('Ctrl Pts',(4.28292985199994,11.6,-10.152246211));
#162738=CARTESIAN_POINT('Ctrl Pts',(4.28278769399994,15.2,-10.149152985));
#162739=CARTESIAN_POINT('Ctrl Pts',(4.28278769399994,11.6,-10.149152985));
#162740=CARTESIAN_POINT('Ctrl Pts',(4.28264326899995,15.2,-10.146065141));
#162741=CARTESIAN_POINT('Ctrl Pts',(4.28264326899995,11.6,-10.146065141));
#162742=CARTESIAN_POINT('Ctrl Pts',(4.28249658599994,15.2,-10.142982685));
#162743=CARTESIAN_POINT('Ctrl Pts',(4.28249658599994,11.6,-10.142982685));
#162744=CARTESIAN_POINT('Ctrl Pts',(4.28234765099995,15.2,-10.139905626));
#162745=CARTESIAN_POINT('Ctrl Pts',(4.28234765099995,11.6,-10.139905626));
#162746=CARTESIAN_POINT('Ctrl Pts',(4.28219647199994,15.2,-10.136833973));
#162747=CARTESIAN_POINT('Ctrl Pts',(4.28219647199994,11.6,-10.136833973));
#162748=CARTESIAN_POINT('Ctrl Pts',(4.28204305799994,15.2,-10.133767736));
#162749=CARTESIAN_POINT('Ctrl Pts',(4.28204305799994,11.6,-10.133767736));
#162750=CARTESIAN_POINT('Ctrl Pts',(4.28188741599994,15.2,-10.130706922));
#162751=CARTESIAN_POINT('Ctrl Pts',(4.28188741599994,11.6,-10.130706922));
#162752=CARTESIAN_POINT('Ctrl Pts',(4.28172955299994,15.2,-10.127651542));
#162753=CARTESIAN_POINT('Ctrl Pts',(4.28172955299994,11.6,-10.127651542));
#162754=CARTESIAN_POINT('Ctrl Pts',(4.28156947799994,15.2,-10.124601604));
#162755=CARTESIAN_POINT('Ctrl Pts',(4.28156947799994,11.6,-10.124601604));
#162756=CARTESIAN_POINT('Ctrl Pts',(4.28140719899995,15.2,-10.121557117));
#162757=CARTESIAN_POINT('Ctrl Pts',(4.28140719899995,11.6,-10.121557117));
#162758=CARTESIAN_POINT('Ctrl Pts',(4.28124272399994,15.2,-10.11851809));
#162759=CARTESIAN_POINT('Ctrl Pts',(4.28124272399994,11.6,-10.11851809));
#162760=CARTESIAN_POINT('Ctrl Pts',(4.28107605999995,15.2,-10.115484533));
#162761=CARTESIAN_POINT('Ctrl Pts',(4.28107605999995,11.6,-10.115484533));
#162762=CARTESIAN_POINT('Ctrl Pts',(4.28090721599994,15.2,-10.112456452));
#162763=CARTESIAN_POINT('Ctrl Pts',(4.28090721599994,11.6,-10.112456452));
#162764=CARTESIAN_POINT('Ctrl Pts',(4.28073619899994,15.2,-10.109433858));
#162765=CARTESIAN_POINT('Ctrl Pts',(4.28073619899994,11.6,-10.109433858));
#162766=CARTESIAN_POINT('Ctrl Pts',(4.28056301799994,15.2,-10.106416761));
#162767=CARTESIAN_POINT('Ctrl Pts',(4.28056301799994,11.6,-10.106416761));
#162768=CARTESIAN_POINT('Ctrl Pts',(4.28038768099994,15.2,-10.103405168));
#162769=CARTESIAN_POINT('Ctrl Pts',(4.28038768099994,11.6,-10.103405168));
#162770=CARTESIAN_POINT('Ctrl Pts',(4.28021019399994,15.2,-10.100399089));
#162771=CARTESIAN_POINT('Ctrl Pts',(4.28021019399994,11.6,-10.100399089));
#162772=CARTESIAN_POINT('Ctrl Pts',(4.28003056799994,15.2,-10.097398535));
#162773=CARTESIAN_POINT('Ctrl Pts',(4.28003056799994,11.6,-10.097398535));
#162774=CARTESIAN_POINT('Ctrl Pts',(4.27984880999994,15.2,-10.094403512));
#162775=CARTESIAN_POINT('Ctrl Pts',(4.27984880999994,11.6,-10.094403512));
#162776=CARTESIAN_POINT('Ctrl Pts',(4.27966492699994,15.2,-10.091414029));
#162777=CARTESIAN_POINT('Ctrl Pts',(4.27966492699994,11.6,-10.091414029));
#162778=CARTESIAN_POINT('Ctrl Pts',(4.27947892899994,15.2,-10.088430099));
#162779=CARTESIAN_POINT('Ctrl Pts',(4.27947892899994,11.6,-10.088430099));
#162780=CARTESIAN_POINT('Ctrl Pts',(4.27929082299995,15.2,-10.085451726));
#162781=CARTESIAN_POINT('Ctrl Pts',(4.27929082299995,11.6,-10.085451726));
#162782=CARTESIAN_POINT('Ctrl Pts',(4.27910061799994,15.2,-10.082478923));
#162783=CARTESIAN_POINT('Ctrl Pts',(4.27910061799994,11.6,-10.082478923));
#162784=CARTESIAN_POINT('Ctrl Pts',(4.27890832199994,15.2,-10.079511697));
#162785=CARTESIAN_POINT('Ctrl Pts',(4.27890832199994,11.6,-10.079511697));
#162786=CARTESIAN_POINT('Ctrl Pts',(4.27871394199994,15.2,-10.076550058));
#162787=CARTESIAN_POINT('Ctrl Pts',(4.27871394199994,11.6,-10.076550058));
#162788=CARTESIAN_POINT('Ctrl Pts',(4.27851748899994,15.2,-10.073594016));
#162789=CARTESIAN_POINT('Ctrl Pts',(4.27851748899994,11.6,-10.073594016));
#162790=CARTESIAN_POINT('Ctrl Pts',(4.27831896899994,15.2,-10.070643579));
#162791=CARTESIAN_POINT('Ctrl Pts',(4.27831896899994,11.6,-10.070643579));
#162792=CARTESIAN_POINT('Ctrl Pts',(4.27811839099994,15.2,-10.067698756));
#162793=CARTESIAN_POINT('Ctrl Pts',(4.27811839099994,11.6,-10.067698756));
#162794=CARTESIAN_POINT('Ctrl Pts',(4.27791576299995,15.2,-10.064759557));
#162795=CARTESIAN_POINT('Ctrl Pts',(4.27791576299995,11.6,-10.064759557));
#162796=CARTESIAN_POINT('Ctrl Pts',(4.27771109499994,15.2,-10.061825991));
#162797=CARTESIAN_POINT('Ctrl Pts',(4.27771109499994,11.6,-10.061825991));
#162798=CARTESIAN_POINT('Ctrl Pts',(4.27750439299994,15.2,-10.058898068));
#162799=CARTESIAN_POINT('Ctrl Pts',(4.27750439299994,11.6,-10.058898068));
#162800=CARTESIAN_POINT('Ctrl Pts',(4.27729566799994,15.2,-10.055975796));
#162801=CARTESIAN_POINT('Ctrl Pts',(4.27729566799994,11.6,-10.055975796));
#162802=CARTESIAN_POINT('Ctrl Pts',(4.27708492699994,15.2,-10.053059184));
#162803=CARTESIAN_POINT('Ctrl Pts',(4.27708492699994,11.6,-10.053059184));
#162804=CARTESIAN_POINT('Ctrl Pts',(4.27687217899994,15.2,-10.050148243));
#162805=CARTESIAN_POINT('Ctrl Pts',(4.27687217899994,11.6,-10.050148243));
#162806=CARTESIAN_POINT('Ctrl Pts',(4.27665743099995,15.2,-10.047242982));
#162807=CARTESIAN_POINT('Ctrl Pts',(4.27665743099995,11.6,-10.047242982));
#162808=CARTESIAN_POINT('Ctrl Pts',(4.27644069399994,15.2,-10.044343408));
#162809=CARTESIAN_POINT('Ctrl Pts',(4.27644069399994,11.6,-10.044343408));
#162810=CARTESIAN_POINT('Ctrl Pts',(4.27622197599994,15.2,-10.041449533));
#162811=CARTESIAN_POINT('Ctrl Pts',(4.27622197599994,11.6,-10.041449533));
#162812=CARTESIAN_POINT('Ctrl Pts',(4.27600128399994,15.2,-10.038561366));
#162813=CARTESIAN_POINT('Ctrl Pts',(4.27600128399994,11.6,-10.038561366));
#162814=CARTESIAN_POINT('Ctrl Pts',(4.27577862799995,15.2,-10.035678915));
#162815=CARTESIAN_POINT('Ctrl Pts',(4.27577862799995,11.6,-10.035678915));
#162816=CARTESIAN_POINT('Ctrl Pts',(4.27555401599994,15.2,-10.03280219));
#162817=CARTESIAN_POINT('Ctrl Pts',(4.27555401599994,11.6,-10.03280219));
#162818=CARTESIAN_POINT('Ctrl Pts',(4.27532745799994,15.2,-10.029931202));
#162819=CARTESIAN_POINT('Ctrl Pts',(4.27532745799994,11.6,-10.029931202));
#162820=CARTESIAN_POINT('Ctrl Pts',(4.27509896099994,15.2,-10.027065958));
#162821=CARTESIAN_POINT('Ctrl Pts',(4.27509896099994,11.6,-10.027065958));
#162822=CARTESIAN_POINT('Ctrl Pts',(4.27486853499994,15.2,-10.024206469));
#162823=CARTESIAN_POINT('Ctrl Pts',(4.27486853499994,11.6,-10.024206469));
#162824=CARTESIAN_POINT('Ctrl Pts',(4.27463618899994,15.2,-10.021352744));
#162825=CARTESIAN_POINT('Ctrl Pts',(4.27463618899994,11.6,-10.021352744));
#162826=CARTESIAN_POINT('Ctrl Pts',(4.27440193099994,15.2,-10.018504791));
#162827=CARTESIAN_POINT('Ctrl Pts',(4.27440193099994,11.6,-10.018504791));
#162828=CARTESIAN_POINT('Ctrl Pts',(4.27416576899994,15.2,-10.015662622));
#162829=CARTESIAN_POINT('Ctrl Pts',(4.27416576899994,11.6,-10.015662622));
#162830=CARTESIAN_POINT('Ctrl Pts',(4.27392771399994,15.2,-10.012826247));
#162831=CARTESIAN_POINT('Ctrl Pts',(4.27392771399994,11.6,-10.012826247));
#162832=CARTESIAN_POINT('Ctrl Pts',(4.27368777299994,15.2,-10.009995672));
#162833=CARTESIAN_POINT('Ctrl Pts',(4.27368777299994,11.6,-10.009995672));
#162834=CARTESIAN_POINT('Ctrl Pts',(4.27344595599994,15.2,-10.007170909));
#162835=CARTESIAN_POINT('Ctrl Pts',(4.27344595599994,11.6,-10.007170909));
#162836=CARTESIAN_POINT('Ctrl Pts',(4.27320227199994,15.2,-10.004351967));
#162837=CARTESIAN_POINT('Ctrl Pts',(4.27320227199994,11.6,-10.004351967));
#162838=CARTESIAN_POINT('Ctrl Pts',(4.27295672999994,15.2,-10.001538855));
#162839=CARTESIAN_POINT('Ctrl Pts',(4.27295672999994,11.6,-10.001538855));
#162840=CARTESIAN_POINT('Ctrl Pts',(4.27270933899994,15.2,-9.99873158300001));
#162841=CARTESIAN_POINT('Ctrl Pts',(4.27270933899994,11.6,-9.99873158300001));
#162842=CARTESIAN_POINT('Ctrl Pts',(4.27246010699994,15.2,-9.99593016200001));
#162843=CARTESIAN_POINT('Ctrl Pts',(4.27246010699994,11.6,-9.99593016200001));
#162844=CARTESIAN_POINT('Ctrl Pts',(4.27220904299995,15.2,-9.99313460000001));
#162845=CARTESIAN_POINT('Ctrl Pts',(4.27220904299995,11.6,-9.99313460000001));
#162846=CARTESIAN_POINT('Ctrl Pts',(4.27195615799994,15.2,-9.99034490700001));
#162847=CARTESIAN_POINT('Ctrl Pts',(4.27195615799994,11.6,-9.99034490700001));
#162848=CARTESIAN_POINT('Ctrl Pts',(4.27170145999994,15.2,-9.98756109200001));
#162849=CARTESIAN_POINT('Ctrl Pts',(4.27170145999994,11.6,-9.98756109200001));
#162850=CARTESIAN_POINT('Ctrl Pts',(4.27144495799994,15.2,-9.98478316600002));
#162851=CARTESIAN_POINT('Ctrl Pts',(4.27144495799994,11.6,-9.98478316600002));
#162852=CARTESIAN_POINT('Ctrl Pts',(4.27118666199994,15.2,-9.98201113800001));
#162853=CARTESIAN_POINT('Ctrl Pts',(4.27118666199994,11.6,-9.98201113800001));
#162854=CARTESIAN_POINT('Ctrl Pts',(4.27092657999994,15.2,-9.97924501800002));
#162855=CARTESIAN_POINT('Ctrl Pts',(4.27092657999994,11.6,-9.97924501800002));
#162856=CARTESIAN_POINT('Ctrl Pts',(4.27066472199995,15.2,-9.97648481500001));
#162857=CARTESIAN_POINT('Ctrl Pts',(4.27066472199995,11.6,-9.97648481500001));
#162858=CARTESIAN_POINT('Ctrl Pts',(4.27040109699994,15.2,-9.97373053900001));
#162859=CARTESIAN_POINT('Ctrl Pts',(4.27040109699994,11.6,-9.97373053900001));
#162860=CARTESIAN_POINT('Ctrl Pts',(4.27013571399994,15.2,-9.97098220000001));
#162861=CARTESIAN_POINT('Ctrl Pts',(4.27013571399994,11.6,-9.97098220000001));
#162862=CARTESIAN_POINT('Ctrl Pts',(4.26986858399994,15.2,-9.96823980900001));
#162863=CARTESIAN_POINT('Ctrl Pts',(4.26986858399994,11.6,-9.96823980900001));
#162864=CARTESIAN_POINT('Ctrl Pts',(4.26959971399994,15.2,-9.96550337300001));
#162865=CARTESIAN_POINT('Ctrl Pts',(4.26959971399994,11.6,-9.96550337300001));
#162866=CARTESIAN_POINT('Ctrl Pts',(4.26932911499994,15.2,-9.96277290400001));
#162867=CARTESIAN_POINT('Ctrl Pts',(4.26932911499994,11.6,-9.96277290400001));
#162868=CARTESIAN_POINT('Ctrl Pts',(4.26905679699995,15.2,-9.96004841000001));
#162869=CARTESIAN_POINT('Ctrl Pts',(4.26905679699995,11.6,-9.96004841000001));
#162870=CARTESIAN_POINT('Ctrl Pts',(4.26878276699994,15.2,-9.95732990400001));
#162871=CARTESIAN_POINT('Ctrl Pts',(4.26878276699994,11.6,-9.95732990400001));
#162872=CARTESIAN_POINT('Ctrl Pts',(4.26850703699994,15.2,-9.95461739200001));
#162873=CARTESIAN_POINT('Ctrl Pts',(4.26850703699994,11.6,-9.95461739200001));
#162874=CARTESIAN_POINT('Ctrl Pts',(4.26822961499994,15.2,-9.95191088700001));
#162875=CARTESIAN_POINT('Ctrl Pts',(4.26822961499994,11.6,-9.95191088700001));
#162876=CARTESIAN_POINT('Ctrl Pts',(4.26795051099994,15.2,-9.94921039700001));
#162877=CARTESIAN_POINT('Ctrl Pts',(4.26795051099994,11.6,-9.94921039700001));
#162878=CARTESIAN_POINT('Ctrl Pts',(4.26766973499995,15.2,-9.94651593200001));
#162879=CARTESIAN_POINT('Ctrl Pts',(4.26766973499995,11.6,-9.94651593200001));
#162880=CARTESIAN_POINT('Ctrl Pts',(4.26738729599994,15.2,-9.94382750400001));
#162881=CARTESIAN_POINT('Ctrl Pts',(4.26738729599994,11.6,-9.94382750400001));
#162882=CARTESIAN_POINT('Ctrl Pts',(4.26710320399994,15.2,-9.94114512000001));
#162883=CARTESIAN_POINT('Ctrl Pts',(4.26710320399994,11.6,-9.94114512000001));
#162884=CARTESIAN_POINT('Ctrl Pts',(4.26681746899995,15.2,-9.93846879200001));
#162885=CARTESIAN_POINT('Ctrl Pts',(4.26681746899995,11.6,-9.93846879200001));
#162886=CARTESIAN_POINT('Ctrl Pts',(4.26653009999994,15.2,-9.93579852900002));
#162887=CARTESIAN_POINT('Ctrl Pts',(4.26653009999994,11.6,-9.93579852900002));
#162888=CARTESIAN_POINT('Ctrl Pts',(4.26624110699994,15.2,-9.93313434100001));
#162889=CARTESIAN_POINT('Ctrl Pts',(4.26624110699994,11.6,-9.93313434100001));
#162890=CARTESIAN_POINT('Ctrl Pts',(4.26595049999994,15.2,-9.93047623900001));
#162891=CARTESIAN_POINT('Ctrl Pts',(4.26595049999994,11.6,-9.93047623900001));
#162892=CARTESIAN_POINT('Ctrl Pts',(4.26565828799994,15.2,-9.92782423300001));
#162893=CARTESIAN_POINT('Ctrl Pts',(4.26565828799994,11.6,-9.92782423300001));
#162894=CARTESIAN_POINT('Ctrl Pts',(4.26536448299994,15.2,-9.92517833100001));
#162895=CARTESIAN_POINT('Ctrl Pts',(4.26536448299994,11.6,-9.92517833100001));
#162896=CARTESIAN_POINT('Ctrl Pts',(4.26506909199994,15.2,-9.92253854600001));
#162897=CARTESIAN_POINT('Ctrl Pts',(4.26506909199994,11.6,-9.92253854600001));
#162898=CARTESIAN_POINT('Ctrl Pts',(4.26477212699994,15.2,-9.91990488600001));
#162899=CARTESIAN_POINT('Ctrl Pts',(4.26477212699994,11.6,-9.91990488600001));
#162900=CARTESIAN_POINT('Ctrl Pts',(4.26447359699995,15.2,-9.91727736200001));
#162901=CARTESIAN_POINT('Ctrl Pts',(4.26447359699995,11.6,-9.91727736200001));
#162902=CARTESIAN_POINT('Ctrl Pts',(4.26417351199994,15.2,-9.91465598400001));
#162903=CARTESIAN_POINT('Ctrl Pts',(4.26417351199994,11.6,-9.91465598400001));
#162904=CARTESIAN_POINT('Ctrl Pts',(4.26387188299994,15.2,-9.91204076200001));
#162905=CARTESIAN_POINT('Ctrl Pts',(4.26387188299994,11.6,-9.91204076200001));
#162906=CARTESIAN_POINT('Ctrl Pts',(4.26356871799995,15.2,-9.90943170600001));
#162907=CARTESIAN_POINT('Ctrl Pts',(4.26356871799995,11.6,-9.90943170600001));
#162908=CARTESIAN_POINT('Ctrl Pts',(4.26326402899995,15.2,-9.90682882600001));
#162909=CARTESIAN_POINT('Ctrl Pts',(4.26326402899995,11.6,-9.90682882600001));
#162910=CARTESIAN_POINT('Ctrl Pts',(4.26295782599994,15.2,-9.90423213400001));
#162911=CARTESIAN_POINT('Ctrl Pts',(4.26295782599994,11.6,-9.90423213400001));
#162912=CARTESIAN_POINT('Ctrl Pts',(4.26265011799994,15.2,-9.90164163800001));
#162913=CARTESIAN_POINT('Ctrl Pts',(4.26265011799994,11.6,-9.90164163800001));
#162914=CARTESIAN_POINT('Ctrl Pts',(4.26234091599994,15.2,-9.89905734900001));
#162915=CARTESIAN_POINT('Ctrl Pts',(4.26234091599994,11.6,-9.89905734900001));
#162916=CARTESIAN_POINT('Ctrl Pts',(4.26203022999994,15.2,-9.89647927800001));
#162917=CARTESIAN_POINT('Ctrl Pts',(4.26203022999994,11.6,-9.89647927800001));
#162918=CARTESIAN_POINT('Ctrl Pts',(4.26171806999994,15.2,-9.89390743400001));
#162919=CARTESIAN_POINT('Ctrl Pts',(4.26171806999994,11.6,-9.89390743400001));
#162920=CARTESIAN_POINT('Ctrl Pts',(4.26140444699994,15.2,-9.89134182800001));
#162921=CARTESIAN_POINT('Ctrl Pts',(4.26140444699994,11.6,-9.89134182800001));
#162922=CARTESIAN_POINT('Ctrl Pts',(4.26108937099994,15.2,-9.88878247200001));
#162923=CARTESIAN_POINT('Ctrl Pts',(4.26108937099994,11.6,-9.88878247200001));
#162924=CARTESIAN_POINT('Ctrl Pts',(4.26077285199994,15.2,-9.88622937300001));
#162925=CARTESIAN_POINT('Ctrl Pts',(4.26077285199994,11.6,-9.88622937300001));
#162926=CARTESIAN_POINT('Ctrl Pts',(4.26045489999994,15.2,-9.88368254300001));
#162927=CARTESIAN_POINT('Ctrl Pts',(4.26045489999994,11.6,-9.88368254300001));
#162928=CARTESIAN_POINT('Ctrl Pts',(4.26013552699995,15.2,-9.88114199300002));
#162929=CARTESIAN_POINT('Ctrl Pts',(4.26013552699995,11.6,-9.88114199300002));
#162930=CARTESIAN_POINT('Ctrl Pts',(4.25981474299994,15.2,-9.87860773300001));
#162931=CARTESIAN_POINT('Ctrl Pts',(4.25981474299994,11.6,-9.87860773300001));
#162932=CARTESIAN_POINT('Ctrl Pts',(4.25949255699994,15.2,-9.87607977400001));
#162933=CARTESIAN_POINT('Ctrl Pts',(4.25949255699994,11.6,-9.87607977400001));
#162934=CARTESIAN_POINT('Ctrl Pts',(4.25916897999994,15.2,-9.87355812500001));
#162935=CARTESIAN_POINT('Ctrl Pts',(4.25916897999994,11.6,-9.87355812500001));
#162936=CARTESIAN_POINT('Ctrl Pts',(4.25884402299994,15.2,-9.87104279600001));
#162937=CARTESIAN_POINT('Ctrl Pts',(4.25884402299994,11.6,-9.87104279600001));
#162938=CARTESIAN_POINT('Ctrl Pts',(4.25851769899994,15.2,-9.86853380100001));
#162939=CARTESIAN_POINT('Ctrl Pts',(4.25851769899994,11.6,-9.86853380100001));
#162940=CARTESIAN_POINT('Ctrl Pts',(4.25819001399994,15.2,-9.86603114700001));
#162941=CARTESIAN_POINT('Ctrl Pts',(4.25819001399994,11.6,-9.86603114700001));
#162942=CARTESIAN_POINT('Ctrl Pts',(4.25786098199994,15.2,-9.86353484700001));
#162943=CARTESIAN_POINT('Ctrl Pts',(4.25786098199994,11.6,-9.86353484700001));
#162944=CARTESIAN_POINT('Ctrl Pts',(4.25753061199994,15.2,-9.86104490900001));
#162945=CARTESIAN_POINT('Ctrl Pts',(4.25753061199994,11.6,-9.86104490900001));
#162946=CARTESIAN_POINT('Ctrl Pts',(4.25719891699995,15.2,-9.85856134500001));
#162947=CARTESIAN_POINT('Ctrl Pts',(4.25719891699995,11.6,-9.85856134500001));
#162948=CARTESIAN_POINT('Ctrl Pts',(4.25686590399994,15.2,-9.85608416600001));
#162949=CARTESIAN_POINT('Ctrl Pts',(4.25686590399994,11.6,-9.85608416600001));
#162950=CARTESIAN_POINT('Ctrl Pts',(4.25653158899994,15.2,-9.85361338200001));
#162951=CARTESIAN_POINT('Ctrl Pts',(4.25653158899994,11.6,-9.85361338200001));
#162952=CARTESIAN_POINT('Ctrl Pts',(4.25619597799994,15.2,-9.85114900400001));
#162953=CARTESIAN_POINT('Ctrl Pts',(4.25619597799994,11.6,-9.85114900400001));
#162954=CARTESIAN_POINT('Ctrl Pts',(4.25585908399994,15.2,-9.84869104300001));
#162955=CARTESIAN_POINT('Ctrl Pts',(4.25585908399994,11.6,-9.84869104300001));
#162956=CARTESIAN_POINT('Ctrl Pts',(4.25552091799995,15.2,-9.84623950800001));
#162957=CARTESIAN_POINT('Ctrl Pts',(4.25552091799995,11.6,-9.84623950800001));
#162958=CARTESIAN_POINT('Ctrl Pts',(4.25518148999994,15.2,-9.84379441200001));
#162959=CARTESIAN_POINT('Ctrl Pts',(4.25518148999994,11.6,-9.84379441200001));
#162960=CARTESIAN_POINT('Ctrl Pts',(4.25484081299994,15.2,-9.84135576400002));
#162961=CARTESIAN_POINT('Ctrl Pts',(4.25484081299994,11.6,-9.84135576400002));
#162962=CARTESIAN_POINT('Ctrl Pts',(4.25449889699994,15.2,-9.83892357600001));
#162963=CARTESIAN_POINT('Ctrl Pts',(4.25449889699994,11.6,-9.83892357600001));
#162964=CARTESIAN_POINT('Ctrl Pts',(4.25415575199994,15.2,-9.83649785800001));
#162965=CARTESIAN_POINT('Ctrl Pts',(4.25415575199994,11.6,-9.83649785800001));
#162966=CARTESIAN_POINT('Ctrl Pts',(4.25381139099995,15.2,-9.83407862100002));
#162967=CARTESIAN_POINT('Ctrl Pts',(4.25381139099995,11.6,-9.83407862100002));
#162968=CARTESIAN_POINT('Ctrl Pts',(4.25346582399994,15.2,-9.83166587500001));
#162969=CARTESIAN_POINT('Ctrl Pts',(4.25346582399994,11.6,-9.83166587500001));
#162970=CARTESIAN_POINT('Ctrl Pts',(4.25311906099994,15.2,-9.82925963300001));
#162971=CARTESIAN_POINT('Ctrl Pts',(4.25311906099994,11.6,-9.82925963300001));
#162972=CARTESIAN_POINT('Ctrl Pts',(4.25277111699994,15.2,-9.82685990200001));
#162973=CARTESIAN_POINT('Ctrl Pts',(4.25277111699994,11.6,-9.82685990200001));
#162974=CARTESIAN_POINT('Ctrl Pts',(4.25242199899994,15.2,-9.82446669800001));
#162975=CARTESIAN_POINT('Ctrl Pts',(4.25242199899994,11.6,-9.82446669800001));
#162976=CARTESIAN_POINT('Ctrl Pts',(4.25207172199995,15.2,-9.82208002900001));
#162977=CARTESIAN_POINT('Ctrl Pts',(4.25207172199995,11.6,-9.82208002900001));
#162978=CARTESIAN_POINT('Ctrl Pts',(4.25172029399994,15.2,-9.81969990500001));
#162979=CARTESIAN_POINT('Ctrl Pts',(4.25172029399994,11.6,-9.81969990500001));
#162980=CARTESIAN_POINT('Ctrl Pts',(4.25136772899994,15.2,-9.81732633900001));
#162981=CARTESIAN_POINT('Ctrl Pts',(4.25136772899994,11.6,-9.81732633900001));
#162982=CARTESIAN_POINT('Ctrl Pts',(4.25101403699994,15.2,-9.81495934100001));
#162983=CARTESIAN_POINT('Ctrl Pts',(4.25101403699994,11.6,-9.81495934100001));
#162984=CARTESIAN_POINT('Ctrl Pts',(4.25065923099995,15.2,-9.81259892200001));
#162985=CARTESIAN_POINT('Ctrl Pts',(4.25065923099995,11.6,-9.81259892200001));
#162986=CARTESIAN_POINT('Ctrl Pts',(4.25030331999994,15.2,-9.81024509500001));
#162987=CARTESIAN_POINT('Ctrl Pts',(4.25030331999994,11.6,-9.81024509500001));
#162988=CARTESIAN_POINT('Ctrl Pts',(4.24994631899995,15.2,-9.80789786800001));
#162989=CARTESIAN_POINT('Ctrl Pts',(4.24994631899995,11.6,-9.80789786800001));
#162990=CARTESIAN_POINT('Ctrl Pts',(4.24958823599995,15.2,-9.80555725300001));
#162991=CARTESIAN_POINT('Ctrl Pts',(4.24958823599995,11.6,-9.80555725300001));
#162992=CARTESIAN_POINT('Ctrl Pts',(4.24922908599994,15.2,-9.80322326100001));
#162993=CARTESIAN_POINT('Ctrl Pts',(4.24922908599994,11.6,-9.80322326100001));
#162994=CARTESIAN_POINT('Ctrl Pts',(4.24886887799994,15.2,-9.80089590500001));
#162995=CARTESIAN_POINT('Ctrl Pts',(4.24886887799994,11.6,-9.80089590500001));
#162996=CARTESIAN_POINT('Ctrl Pts',(4.24850762499995,15.2,-9.79857519500001));
#162997=CARTESIAN_POINT('Ctrl Pts',(4.24850762499995,11.6,-9.79857519500001));
#162998=CARTESIAN_POINT('Ctrl Pts',(4.24814533899994,15.2,-9.79626114200001));
#162999=CARTESIAN_POINT('Ctrl Pts',(4.24814533899994,11.6,-9.79626114200001));
#163000=CARTESIAN_POINT('Ctrl Pts',(4.24778202999994,15.2,-9.79395375600001));
#163001=CARTESIAN_POINT('Ctrl Pts',(4.24778202999994,11.6,-9.79395375600001));
#163002=CARTESIAN_POINT('Ctrl Pts',(4.24741771199994,15.2,-9.79165305000001));
#163003=CARTESIAN_POINT('Ctrl Pts',(4.24741771199994,11.6,-9.79165305000001));
#163004=CARTESIAN_POINT('Ctrl Pts',(4.24705239599994,15.2,-9.78935903500001));
#163005=CARTESIAN_POINT('Ctrl Pts',(4.24705239599994,11.6,-9.78935903500001));
#163006=CARTESIAN_POINT('Ctrl Pts',(4.24668609599994,15.2,-9.78707172100002));
#163007=CARTESIAN_POINT('Ctrl Pts',(4.24668609599994,11.6,-9.78707172100002));
#163008=CARTESIAN_POINT('Ctrl Pts',(4.24631881999994,15.2,-9.78479112100001));
#163009=CARTESIAN_POINT('Ctrl Pts',(4.24631881999994,11.6,-9.78479112100001));
#163010=CARTESIAN_POINT('Ctrl Pts',(4.24595058199994,15.2,-9.78251724500001));
#163011=CARTESIAN_POINT('Ctrl Pts',(4.24595058199994,11.6,-9.78251724500001));
#163012=CARTESIAN_POINT('Ctrl Pts',(4.24558139499995,15.2,-9.78025010500001));
#163013=CARTESIAN_POINT('Ctrl Pts',(4.24558139499995,11.6,-9.78025010500001));
#163014=CARTESIAN_POINT('Ctrl Pts',(4.24521126999994,15.2,-9.77798971300001));
#163015=CARTESIAN_POINT('Ctrl Pts',(4.24521126999994,11.6,-9.77798971300001));
#163016=CARTESIAN_POINT('Ctrl Pts',(4.24484021999994,15.2,-9.77573608000001));
#163017=CARTESIAN_POINT('Ctrl Pts',(4.24484021999994,11.6,-9.77573608000001));
#163018=CARTESIAN_POINT('Ctrl Pts',(4.24446825699994,15.2,-9.77348921500001));
#163019=CARTESIAN_POINT('Ctrl Pts',(4.24446825699994,11.6,-9.77348921500001));
#163020=CARTESIAN_POINT('Ctrl Pts',(4.24409539199995,15.2,-9.77124913400001));
#163021=CARTESIAN_POINT('Ctrl Pts',(4.24409539199995,11.6,-9.77124913400001));
#163022=CARTESIAN_POINT('Ctrl Pts',(4.24372163899995,15.2,-9.76901584600001));
#163023=CARTESIAN_POINT('Ctrl Pts',(4.24372163899995,11.6,-9.76901584600001));
#163024=CARTESIAN_POINT('Ctrl Pts',(4.24334700899994,15.2,-9.76678936100001));
#163025=CARTESIAN_POINT('Ctrl Pts',(4.24334700899994,11.6,-9.76678936100001));
#163026=CARTESIAN_POINT('Ctrl Pts',(4.24297151499994,15.2,-9.76456969300001));
#163027=CARTESIAN_POINT('Ctrl Pts',(4.24297151499994,11.6,-9.76456969300001));
#163028=CARTESIAN_POINT('Ctrl Pts',(4.24259516999994,15.2,-9.76235685300001));
#163029=CARTESIAN_POINT('Ctrl Pts',(4.24259516999994,11.6,-9.76235685300001));
#163030=CARTESIAN_POINT('Ctrl Pts',(4.24221798499994,15.2,-9.76015085200001));
#163031=CARTESIAN_POINT('Ctrl Pts',(4.24221798499994,11.6,-9.76015085200001));
#163032=CARTESIAN_POINT('Ctrl Pts',(4.24183997499994,15.2,-9.75795170200001));
#163033=CARTESIAN_POINT('Ctrl Pts',(4.24183997499994,11.6,-9.75795170200001));
#163034=CARTESIAN_POINT('Ctrl Pts',(4.24146114899994,15.2,-9.75575941500001));
#163035=CARTESIAN_POINT('Ctrl Pts',(4.24146114899994,11.6,-9.75575941500001));
#163036=CARTESIAN_POINT('Ctrl Pts',(4.24108152199994,15.2,-9.75357400100001));
#163037=CARTESIAN_POINT('Ctrl Pts',(4.24108152199994,11.6,-9.75357400100001));
#163038=CARTESIAN_POINT('Ctrl Pts',(4.24070110699994,15.2,-9.75139547400001));
#163039=CARTESIAN_POINT('Ctrl Pts',(4.24070110699994,11.6,-9.75139547400001));
#163040=CARTESIAN_POINT('Ctrl Pts',(4.24031991699994,15.2,-9.74922384400001));
#163041=CARTESIAN_POINT('Ctrl Pts',(4.24031991699994,11.6,-9.74922384400001));
#163042=CARTESIAN_POINT('Ctrl Pts',(4.23993796199994,15.2,-9.74705912500001));
#163043=CARTESIAN_POINT('Ctrl Pts',(4.23993796199994,11.6,-9.74705912500001));
#163044=CARTESIAN_POINT('Ctrl Pts',(4.23955525799994,15.2,-9.74490132500001));
#163045=CARTESIAN_POINT('Ctrl Pts',(4.23955525799994,11.6,-9.74490132500001));
#163046=CARTESIAN_POINT('Ctrl Pts',(4.23917181499994,15.2,-9.74275045900001));
#163047=CARTESIAN_POINT('Ctrl Pts',(4.23917181499994,11.6,-9.74275045900001));
#163048=CARTESIAN_POINT('Ctrl Pts',(4.23878764799994,15.2,-9.74060653900001));
#163049=CARTESIAN_POINT('Ctrl Pts',(4.23878764799994,11.6,-9.74060653900001));
#163050=CARTESIAN_POINT('Ctrl Pts',(4.23840276899994,15.2,-9.73846957500001));
#163051=CARTESIAN_POINT('Ctrl Pts',(4.23840276899994,11.6,-9.73846957500001));
#163052=CARTESIAN_POINT('Ctrl Pts',(4.23801719099994,15.2,-9.73633957900001));
#163053=CARTESIAN_POINT('Ctrl Pts',(4.23801719099994,11.6,-9.73633957900001));
#163054=CARTESIAN_POINT('Ctrl Pts',(4.23763092899994,15.2,-9.73421656400001));
#163055=CARTESIAN_POINT('Ctrl Pts',(4.23763092899994,11.6,-9.73421656400001));
#163056=CARTESIAN_POINT('Ctrl Pts',(4.23724399199994,15.2,-9.73210054100001));
#163057=CARTESIAN_POINT('Ctrl Pts',(4.23724399199994,11.6,-9.73210054100001));
#163058=CARTESIAN_POINT('Ctrl Pts',(4.23685639699994,15.2,-9.72999152300001));
#163059=CARTESIAN_POINT('Ctrl Pts',(4.23685639699994,11.6,-9.72999152300001));
#163060=CARTESIAN_POINT('Ctrl Pts',(4.23646815499994,15.2,-9.72788952200001));
#163061=CARTESIAN_POINT('Ctrl Pts',(4.23646815499994,11.6,-9.72788952200001));
#163062=CARTESIAN_POINT('Ctrl Pts',(4.23607928099995,15.2,-9.72579454900002));
#163063=CARTESIAN_POINT('Ctrl Pts',(4.23607928099995,11.6,-9.72579454900002));
#163064=CARTESIAN_POINT('Ctrl Pts',(4.23568978699994,15.2,-9.72370661700001));
#163065=CARTESIAN_POINT('Ctrl Pts',(4.23568978699994,11.6,-9.72370661700001));
#163066=CARTESIAN_POINT('Ctrl Pts',(4.23529968599994,15.2,-9.72162573800001));
#163067=CARTESIAN_POINT('Ctrl Pts',(4.23529968599994,11.6,-9.72162573800001));
#163068=CARTESIAN_POINT('Ctrl Pts',(4.23490899199995,15.2,-9.71955192300001));
#163069=CARTESIAN_POINT('Ctrl Pts',(4.23490899199995,11.6,-9.71955192300001));
#163070=CARTESIAN_POINT('Ctrl Pts',(4.23451771999994,15.2,-9.71748518500001));
#163071=CARTESIAN_POINT('Ctrl Pts',(4.23451771999994,11.6,-9.71748518500001));
#163072=CARTESIAN_POINT('Ctrl Pts',(4.23412588099994,15.2,-9.71542553700001));
#163073=CARTESIAN_POINT('Ctrl Pts',(4.23412588099994,11.6,-9.71542553700001));
#163074=CARTESIAN_POINT('Ctrl Pts',(4.23373348799994,15.2,-9.71337299000002));
#163075=CARTESIAN_POINT('Ctrl Pts',(4.23373348799994,11.6,-9.71337299000002));
#163076=CARTESIAN_POINT('Ctrl Pts',(4.23334055899994,15.2,-9.71132755800001));
#163077=CARTESIAN_POINT('Ctrl Pts',(4.23334055899994,11.6,-9.71132755800001));
#163078=CARTESIAN_POINT('Ctrl Pts',(4.23294710199994,15.2,-9.70928925100001));
#163079=CARTESIAN_POINT('Ctrl Pts',(4.23294710199994,11.6,-9.70928925100001));
#163080=CARTESIAN_POINT('Ctrl Pts',(4.23255313499994,15.2,-9.70725808200001));
#163081=CARTESIAN_POINT('Ctrl Pts',(4.23255313499994,11.6,-9.70725808200001));
#163082=CARTESIAN_POINT('Ctrl Pts',(4.23215866999994,15.2,-9.70523406400001));
#163083=CARTESIAN_POINT('Ctrl Pts',(4.23215866999994,11.6,-9.70523406400001));
#163084=CARTESIAN_POINT('Ctrl Pts',(4.23176372199995,15.2,-9.70321720900001));
#163085=CARTESIAN_POINT('Ctrl Pts',(4.23176372199995,11.6,-9.70321720900001));
#163086=CARTESIAN_POINT('Ctrl Pts',(4.23136830199994,15.2,-9.70120753000001));
#163087=CARTESIAN_POINT('Ctrl Pts',(4.23136830199994,11.6,-9.70120753000001));
#163088=CARTESIAN_POINT('Ctrl Pts',(4.23097242799995,15.2,-9.69920503800001));
#163089=CARTESIAN_POINT('Ctrl Pts',(4.23097242799995,11.6,-9.69920503800001));
#163090=CARTESIAN_POINT('Ctrl Pts',(4.23057610999995,15.2,-9.69720974700001));
#163091=CARTESIAN_POINT('Ctrl Pts',(4.23057610999995,11.6,-9.69720974700001));
#163092=CARTESIAN_POINT('Ctrl Pts',(4.23017936499994,15.2,-9.69522166900001));
#163093=CARTESIAN_POINT('Ctrl Pts',(4.23017936499994,11.6,-9.69522166900001));
#163094=CARTESIAN_POINT('Ctrl Pts',(4.22978220499994,15.2,-9.69324081500002));
#163095=CARTESIAN_POINT('Ctrl Pts',(4.22978220499994,11.6,-9.69324081500002));
#163096=CARTESIAN_POINT('Ctrl Pts',(4.22938464599994,15.2,-9.69126720100001));
#163097=CARTESIAN_POINT('Ctrl Pts',(4.22938464599994,11.6,-9.69126720100001));
#163098=CARTESIAN_POINT('Ctrl Pts',(4.22898670099995,15.2,-9.68930083700001));
#163099=CARTESIAN_POINT('Ctrl Pts',(4.22898670099995,11.6,-9.68930083700001));
#163100=CARTESIAN_POINT('Ctrl Pts',(4.22858838299994,15.2,-9.68734173600001));
#163101=CARTESIAN_POINT('Ctrl Pts',(4.22858838299994,11.6,-9.68734173600001));
#163102=CARTESIAN_POINT('Ctrl Pts',(4.22818970999994,15.2,-9.68538991100001));
#163103=CARTESIAN_POINT('Ctrl Pts',(4.22818970999994,11.6,-9.68538991100001));
#163104=CARTESIAN_POINT('Ctrl Pts',(4.22779069299995,15.2,-9.68344537500001));
#163105=CARTESIAN_POINT('Ctrl Pts',(4.22779069299995,11.6,-9.68344537500001));
#163106=CARTESIAN_POINT('Ctrl Pts',(4.22739134799994,15.2,-9.68150814100001));
#163107=CARTESIAN_POINT('Ctrl Pts',(4.22739134799994,11.6,-9.68150814100001));
#163108=CARTESIAN_POINT('Ctrl Pts',(4.22699168899995,15.2,-9.67957822000001));
#163109=CARTESIAN_POINT('Ctrl Pts',(4.22699168899995,11.6,-9.67957822000001));
#163110=CARTESIAN_POINT('Ctrl Pts',(4.22659172899994,15.2,-9.67765562600001));
#163111=CARTESIAN_POINT('Ctrl Pts',(4.22659172899994,11.6,-9.67765562600001));
#163112=CARTESIAN_POINT('Ctrl Pts',(4.22619148699994,15.2,-9.67574037200001));
#163113=CARTESIAN_POINT('Ctrl Pts',(4.22619148699994,11.6,-9.67574037200001));
#163114=CARTESIAN_POINT('Ctrl Pts',(4.22579097299994,15.2,-9.67383247200001));
#163115=CARTESIAN_POINT('Ctrl Pts',(4.22579097299994,11.6,-9.67383247200001));
#163116=CARTESIAN_POINT('Ctrl Pts',(4.22539020299994,15.2,-9.67193193700002));
#163117=CARTESIAN_POINT('Ctrl Pts',(4.22539020299994,11.6,-9.67193193700002));
#163118=CARTESIAN_POINT('Ctrl Pts',(4.22498919399994,15.2,-9.67003878000001));
#163119=CARTESIAN_POINT('Ctrl Pts',(4.22498919399994,11.6,-9.67003878000001));
#163120=CARTESIAN_POINT('Ctrl Pts',(4.22458795699994,15.2,-9.66815301400001));
#163121=CARTESIAN_POINT('Ctrl Pts',(4.22458795699994,11.6,-9.66815301400001));
#163122=CARTESIAN_POINT('Ctrl Pts',(4.22418651099994,15.2,-9.66627465400001));
#163123=CARTESIAN_POINT('Ctrl Pts',(4.22418651099994,11.6,-9.66627465400001));
#163124=CARTESIAN_POINT('Ctrl Pts',(4.22378486799994,15.2,-9.66440371000001));
#163125=CARTESIAN_POINT('Ctrl Pts',(4.22378486799994,11.6,-9.66440371000001));
#163126=CARTESIAN_POINT('Ctrl Pts',(4.22338304399995,15.2,-9.66254019800001));
#163127=CARTESIAN_POINT('Ctrl Pts',(4.22338304399995,11.6,-9.66254019800001));
#163128=CARTESIAN_POINT('Ctrl Pts',(4.22298105399994,15.2,-9.66068412900001));
#163129=CARTESIAN_POINT('Ctrl Pts',(4.22298105399994,11.6,-9.66068412900001));
#163130=CARTESIAN_POINT('Ctrl Pts',(4.22257891299994,15.2,-9.65883551800001));
#163131=CARTESIAN_POINT('Ctrl Pts',(4.22257891299994,11.6,-9.65883551800001));
#163132=CARTESIAN_POINT('Ctrl Pts',(4.22217663599994,15.2,-9.65699437700001));
#163133=CARTESIAN_POINT('Ctrl Pts',(4.22217663599994,11.6,-9.65699437700001));
#163134=CARTESIAN_POINT('Ctrl Pts',(4.22177423899995,15.2,-9.65516071900001));
#163135=CARTESIAN_POINT('Ctrl Pts',(4.22177423899995,11.6,-9.65516071900001));
#163136=CARTESIAN_POINT('Ctrl Pts',(4.22137173599994,15.2,-9.65333455800001));
#163137=CARTESIAN_POINT('Ctrl Pts',(4.22137173599994,11.6,-9.65333455800001));
#163138=CARTESIAN_POINT('Ctrl Pts',(4.22096914499994,15.2,-9.65151590700002));
#163139=CARTESIAN_POINT('Ctrl Pts',(4.22096914499994,11.6,-9.65151590700002));
#163140=CARTESIAN_POINT('Ctrl Pts',(4.22056647799994,15.2,-9.64970478000001));
#163141=CARTESIAN_POINT('Ctrl Pts',(4.22056647799994,11.6,-9.64970478000001));
#163142=CARTESIAN_POINT('Ctrl Pts',(4.22016375199994,15.2,-9.64790119000002));
#163143=CARTESIAN_POINT('Ctrl Pts',(4.22016375199994,11.6,-9.64790119000002));
#163144=CARTESIAN_POINT('Ctrl Pts',(4.21976098299994,15.2,-9.64610514900002));
#163145=CARTESIAN_POINT('Ctrl Pts',(4.21976098299994,11.6,-9.64610514900002));
#163146=CARTESIAN_POINT('Ctrl Pts',(4.21935818699995,15.2,-9.64431667300002));
#163147=CARTESIAN_POINT('Ctrl Pts',(4.21935818699995,11.6,-9.64431667300002));
#163148=CARTESIAN_POINT('Ctrl Pts',(4.21895537899994,15.2,-9.64253577300001));
#163149=CARTESIAN_POINT('Ctrl Pts',(4.21895537899994,11.6,-9.64253577300001));
#163150=CARTESIAN_POINT('Ctrl Pts',(4.21855257299994,15.2,-9.64076246400002));
#163151=CARTESIAN_POINT('Ctrl Pts',(4.21855257299994,11.6,-9.64076246400002));
#163152=CARTESIAN_POINT('Ctrl Pts',(4.21814978799994,15.2,-9.63899675900001));
#163153=CARTESIAN_POINT('Ctrl Pts',(4.21814978799994,11.6,-9.63899675900001));
#163154=CARTESIAN_POINT('Ctrl Pts',(4.21774703799994,15.2,-9.63723867200001));
#163155=CARTESIAN_POINT('Ctrl Pts',(4.21774703799994,11.6,-9.63723867200001));
#163156=CARTESIAN_POINT('Ctrl Pts',(4.21734433799995,15.2,-9.63548821700002));
#163157=CARTESIAN_POINT('Ctrl Pts',(4.21734433799995,11.6,-9.63548821700002));
#163158=CARTESIAN_POINT('Ctrl Pts',(4.21694170799995,15.2,-9.63374540800002));
#163159=CARTESIAN_POINT('Ctrl Pts',(4.21694170799995,11.6,-9.63374540800002));
#163160=CARTESIAN_POINT('Ctrl Pts',(4.21653915999994,15.2,-9.63201025700002));
#163161=CARTESIAN_POINT('Ctrl Pts',(4.21653915999994,11.6,-9.63201025700002));
#163162=CARTESIAN_POINT('Ctrl Pts',(4.21613671099994,15.2,-9.63028277900002));
#163163=CARTESIAN_POINT('Ctrl Pts',(4.21613671099994,11.6,-9.63028277900002));
#163164=CARTESIAN_POINT('Ctrl Pts',(4.21573437799994,15.2,-9.62856298800002));
#163165=CARTESIAN_POINT('Ctrl Pts',(4.21573437799994,11.6,-9.62856298800002));
#163166=CARTESIAN_POINT('Ctrl Pts',(4.21533217699994,15.2,-9.62685089700001));
#163167=CARTESIAN_POINT('Ctrl Pts',(4.21533217699994,11.6,-9.62685089700001));
#163168=CARTESIAN_POINT('Ctrl Pts',(4.21493012499994,15.2,-9.62514652000002));
#163169=CARTESIAN_POINT('Ctrl Pts',(4.21493012499994,11.6,-9.62514652000002));
#163170=CARTESIAN_POINT('Ctrl Pts',(4.21452823699994,15.2,-9.62344987300002));
#163171=CARTESIAN_POINT('Ctrl Pts',(4.21452823699994,11.6,-9.62344987300002));
#163172=CARTESIAN_POINT('Ctrl Pts',(4.21412653099994,15.2,-9.62176096700002));
#163173=CARTESIAN_POINT('Ctrl Pts',(4.21412653099994,11.6,-9.62176096700002));
#163174=CARTESIAN_POINT('Ctrl Pts',(4.21372502199994,15.2,-9.62007981800001));
#163175=CARTESIAN_POINT('Ctrl Pts',(4.21372502199994,11.6,-9.62007981800001));
#163176=CARTESIAN_POINT('Ctrl Pts',(4.21332372799994,15.2,-9.61840643900001));
#163177=CARTESIAN_POINT('Ctrl Pts',(4.21332372799994,11.6,-9.61840643900001));
#163178=CARTESIAN_POINT('Ctrl Pts',(4.21292266499994,15.2,-9.61674084500002));
#163179=CARTESIAN_POINT('Ctrl Pts',(4.21292266499994,11.6,-9.61674084500002));
#163180=CARTESIAN_POINT('Ctrl Pts',(4.21252184899994,15.2,-9.61508305000002));
#163181=CARTESIAN_POINT('Ctrl Pts',(4.21252184899994,11.6,-9.61508305000002));
#163182=CARTESIAN_POINT('Ctrl Pts',(4.21212129899994,15.2,-9.61343306700002));
#163183=CARTESIAN_POINT('Ctrl Pts',(4.21212129899994,11.6,-9.61343306700002));
#163184=CARTESIAN_POINT('Ctrl Pts',(4.21172102999994,15.2,-9.61179091100002));
#163185=CARTESIAN_POINT('Ctrl Pts',(4.21172102999994,11.6,-9.61179091100002));
#163186=CARTESIAN_POINT('Ctrl Pts',(4.21132105999994,15.2,-9.61015659800001));
#163187=CARTESIAN_POINT('Ctrl Pts',(4.21132105999994,11.6,-9.61015659800001));
#163188=CARTESIAN_POINT('Ctrl Pts',(4.21092140599994,15.2,-9.60853014000002));
#163189=CARTESIAN_POINT('Ctrl Pts',(4.21092140599994,11.6,-9.60853014000002));
#163190=CARTESIAN_POINT('Ctrl Pts',(4.21052208399994,15.2,-9.60691155200001));
#163191=CARTESIAN_POINT('Ctrl Pts',(4.21052208399994,11.6,-9.60691155200001));
#163192=CARTESIAN_POINT('Ctrl Pts',(4.21012311199994,15.2,-9.60530084900002));
#163193=CARTESIAN_POINT('Ctrl Pts',(4.21012311199994,11.6,-9.60530084900002));
#163194=CARTESIAN_POINT('Ctrl Pts',(4.20972450799994,15.2,-9.60369804500001));
#163195=CARTESIAN_POINT('Ctrl Pts',(4.20972450799994,11.6,-9.60369804500001));
#163196=CARTESIAN_POINT('Ctrl Pts',(4.20932628699994,15.2,-9.60210315400002));
#163197=CARTESIAN_POINT('Ctrl Pts',(4.20932628699994,11.6,-9.60210315400002));
#163198=CARTESIAN_POINT('Ctrl Pts',(4.20892846999994,15.2,-9.60051619200001));
#163199=CARTESIAN_POINT('Ctrl Pts',(4.20892846999994,11.6,-9.60051619200001));
#163200=CARTESIAN_POINT('Ctrl Pts',(4.20853107099994,15.2,-9.59893717100002));
#163201=CARTESIAN_POINT('Ctrl Pts',(4.20853107099994,11.6,-9.59893717100002));
#163202=CARTESIAN_POINT('Ctrl Pts',(4.20813410999994,15.2,-9.59736611000002));
#163203=CARTESIAN_POINT('Ctrl Pts',(4.20813410999994,11.6,-9.59736611000002));
#163204=CARTESIAN_POINT('Ctrl Pts',(4.20773760299994,15.2,-9.59580302000001));
#163205=CARTESIAN_POINT('Ctrl Pts',(4.20773760299994,11.6,-9.59580302000001));
#163206=CARTESIAN_POINT('Ctrl Pts',(4.20734156899994,15.2,-9.59424791600001));
#163207=CARTESIAN_POINT('Ctrl Pts',(4.20734156899994,11.6,-9.59424791600001));
#163208=CARTESIAN_POINT('Ctrl Pts',(4.20694602499994,15.2,-9.59270081500001));
#163209=CARTESIAN_POINT('Ctrl Pts',(4.20694602499994,11.6,-9.59270081500001));
#163210=CARTESIAN_POINT('Ctrl Pts',(4.20655098899995,15.2,-9.59116173000002));
#163211=CARTESIAN_POINT('Ctrl Pts',(4.20655098899995,11.6,-9.59116173000002));
#163212=CARTESIAN_POINT('Ctrl Pts',(4.20615647899994,15.2,-9.58963067600001));
#163213=CARTESIAN_POINT('Ctrl Pts',(4.20615647899994,11.6,-9.58963067600001));
#163214=CARTESIAN_POINT('Ctrl Pts',(4.20576251399994,15.2,-9.58810766900001));
#163215=CARTESIAN_POINT('Ctrl Pts',(4.20576251399994,11.6,-9.58810766900001));
#163216=CARTESIAN_POINT('Ctrl Pts',(4.20536911099994,15.2,-9.58659272300002));
#163217=CARTESIAN_POINT('Ctrl Pts',(4.20536911099994,11.6,-9.58659272300002));
#163218=CARTESIAN_POINT('Ctrl Pts',(4.20497628799995,15.2,-9.58508585300001));
#163219=CARTESIAN_POINT('Ctrl Pts',(4.20497628799995,11.6,-9.58508585300001));
#163220=CARTESIAN_POINT('Ctrl Pts',(4.20458406399994,15.2,-9.58358707500001));
#163221=CARTESIAN_POINT('Ctrl Pts',(4.20458406399994,11.6,-9.58358707500001));
#163222=CARTESIAN_POINT('Ctrl Pts',(4.20419245599994,15.2,-9.58209640400002));
#163223=CARTESIAN_POINT('Ctrl Pts',(4.20419245599994,11.6,-9.58209640400002));
#163224=CARTESIAN_POINT('Ctrl Pts',(4.20380148499994,15.2,-9.58061385400002));
#163225=CARTESIAN_POINT('Ctrl Pts',(4.20380148499994,11.6,-9.58061385400002));
#163226=CARTESIAN_POINT('Ctrl Pts',(4.20341116699994,15.2,-9.57913944200002));
#163227=CARTESIAN_POINT('Ctrl Pts',(4.20341116699994,11.6,-9.57913944200002));
#163228=CARTESIAN_POINT('Ctrl Pts',(4.20302152299994,15.2,-9.57767318000002));
#163229=CARTESIAN_POINT('Ctrl Pts',(4.20302152299994,11.6,-9.57767318000002));
#163230=CARTESIAN_POINT('Ctrl Pts',(4.20263256899994,15.2,-9.57621508900001));
#163231=CARTESIAN_POINT('Ctrl Pts',(4.20263256899994,11.6,-9.57621508900001));
#163232=CARTESIAN_POINT('Ctrl Pts',(4.20224432599994,15.2,-9.57476517800002));
#163233=CARTESIAN_POINT('Ctrl Pts',(4.20224432599994,11.6,-9.57476517800002));
#163234=CARTESIAN_POINT('Ctrl Pts',(4.20185681099994,15.2,-9.57332346700002));
#163235=CARTESIAN_POINT('Ctrl Pts',(4.20185681099994,11.6,-9.57332346700002));
#163236=CARTESIAN_POINT('Ctrl Pts',(4.20147004499994,15.2,-9.57188997100002));
#163237=CARTESIAN_POINT('Ctrl Pts',(4.20147004499994,11.6,-9.57188997100002));
#163238=CARTESIAN_POINT('Ctrl Pts',(4.20108404499994,15.2,-9.57046470300002));
#163239=CARTESIAN_POINT('Ctrl Pts',(4.20108404499994,11.6,-9.57046470300002));
#163240=CARTESIAN_POINT('Ctrl Pts',(4.20069883099994,15.2,-9.56904768000001));
#163241=CARTESIAN_POINT('Ctrl Pts',(4.20069883099994,11.6,-9.56904768000001));
#163242=CARTESIAN_POINT('Ctrl Pts',(4.20031442399995,15.2,-9.56763891900002));
#163243=CARTESIAN_POINT('Ctrl Pts',(4.20031442399995,11.6,-9.56763891900002));
#163244=CARTESIAN_POINT('Ctrl Pts',(4.19993083999994,15.2,-9.56623843500001));
#163245=CARTESIAN_POINT('Ctrl Pts',(4.19993083999994,11.6,-9.56623843500001));
#163246=CARTESIAN_POINT('Ctrl Pts',(4.19954810099994,15.2,-9.56484624100002));
#163247=CARTESIAN_POINT('Ctrl Pts',(4.19954810099994,11.6,-9.56484624100002));
#163248=CARTESIAN_POINT('Ctrl Pts',(4.19916622499994,15.2,-9.56346235600002));
#163249=CARTESIAN_POINT('Ctrl Pts',(4.19916622499994,11.6,-9.56346235600002));
#163250=CARTESIAN_POINT('Ctrl Pts',(4.19878523199994,15.2,-9.56208679600002));
#163251=CARTESIAN_POINT('Ctrl Pts',(4.19878523199994,11.6,-9.56208679600002));
#163252=CARTESIAN_POINT('Ctrl Pts',(4.19840514099994,15.2,-9.56071957500002));
#163253=CARTESIAN_POINT('Ctrl Pts',(4.19840514099994,11.6,-9.56071957500002));
#163254=CARTESIAN_POINT('Ctrl Pts',(4.19802597299994,15.2,-9.55936071100002));
#163255=CARTESIAN_POINT('Ctrl Pts',(4.19802597299994,11.6,-9.55936071100002));
#163256=CARTESIAN_POINT('Ctrl Pts',(4.19764774699994,15.2,-9.55801021800001));
#163257=CARTESIAN_POINT('Ctrl Pts',(4.19764774699994,11.6,-9.55801021800001));
#163258=CARTESIAN_POINT('Ctrl Pts',(4.19727048399994,15.2,-9.55666811400001));
#163259=CARTESIAN_POINT('Ctrl Pts',(4.19727048399994,11.6,-9.55666811400001));
#163260=CARTESIAN_POINT('Ctrl Pts',(4.19689420199994,15.2,-9.55533441300001));
#163261=CARTESIAN_POINT('Ctrl Pts',(4.19689420199994,11.6,-9.55533441300001));
#163262=CARTESIAN_POINT('Ctrl Pts',(4.19651892299994,15.2,-9.55400913400002));
#163263=CARTESIAN_POINT('Ctrl Pts',(4.19651892299994,11.6,-9.55400913400002));
#163264=CARTESIAN_POINT('Ctrl Pts',(4.19614466599994,15.2,-9.55269229000002));
#163265=CARTESIAN_POINT('Ctrl Pts',(4.19614466599994,11.6,-9.55269229000002));
#163266=CARTESIAN_POINT('Ctrl Pts',(4.19577145099994,15.2,-9.55138390000002));
#163267=CARTESIAN_POINT('Ctrl Pts',(4.19577145099994,11.6,-9.55138390000002));
#163268=CARTESIAN_POINT('Ctrl Pts',(4.19539930099995,15.2,-9.55008398000002));
#163269=CARTESIAN_POINT('Ctrl Pts',(4.19539930099995,11.6,-9.55008398000002));
#163270=CARTESIAN_POINT('Ctrl Pts',(4.19502823399994,15.2,-9.54879254600002));
#163271=CARTESIAN_POINT('Ctrl Pts',(4.19502823399994,11.6,-9.54879254600002));
#163272=CARTESIAN_POINT('Ctrl Pts',(4.19465827099994,15.2,-9.54750961300002));
#163273=CARTESIAN_POINT('Ctrl Pts',(4.19465827099994,11.6,-9.54750961300002));
#163274=CARTESIAN_POINT('Ctrl Pts',(4.19428943299994,15.2,-9.54623520100002));
#163275=CARTESIAN_POINT('Ctrl Pts',(4.19428943299994,11.6,-9.54623520100002));
#163276=CARTESIAN_POINT('Ctrl Pts',(4.19392174099994,15.2,-9.54496932300002));
#163277=CARTESIAN_POINT('Ctrl Pts',(4.19392174099994,11.6,-9.54496932300002));
#163278=CARTESIAN_POINT('Ctrl Pts',(4.19355521499994,15.2,-9.54371199800002));
#163279=CARTESIAN_POINT('Ctrl Pts',(4.19355521499994,11.6,-9.54371199800002));
#163280=CARTESIAN_POINT('Ctrl Pts',(4.19318987699994,15.2,-9.54246324200002));
#163281=CARTESIAN_POINT('Ctrl Pts',(4.19318987699994,11.6,-9.54246324200002));
#163282=CARTESIAN_POINT('Ctrl Pts',(4.19282574799994,15.2,-9.54122307200001));
#163283=CARTESIAN_POINT('Ctrl Pts',(4.19282574799994,11.6,-9.54122307200001));
#163284=CARTESIAN_POINT('Ctrl Pts',(4.19246284799994,15.2,-9.53999150600002));
#163285=CARTESIAN_POINT('Ctrl Pts',(4.19246284799994,11.6,-9.53999150600002));
#163286=CARTESIAN_POINT('Ctrl Pts',(4.19210119999994,15.2,-9.53876855900001));
#163287=CARTESIAN_POINT('Ctrl Pts',(4.19210119999994,11.6,-9.53876855900001));
#163288=CARTESIAN_POINT('Ctrl Pts',(4.19174082499994,15.2,-9.53755424900002));
#163289=CARTESIAN_POINT('Ctrl Pts',(4.19174082499994,11.6,-9.53755424900002));
#163290=CARTESIAN_POINT('Ctrl Pts',(4.19138174199994,15.2,-9.53634859200001));
#163291=CARTESIAN_POINT('Ctrl Pts',(4.19138174199994,11.6,-9.53634859200001));
#163292=CARTESIAN_POINT('Ctrl Pts',(4.19102397699994,15.2,-9.53515160700002));
#163293=CARTESIAN_POINT('Ctrl Pts',(4.19102397699994,11.6,-9.53515160700002));
#163294=CARTESIAN_POINT('Ctrl Pts',(4.19066754799994,15.2,-9.53396331100001));
#163295=CARTESIAN_POINT('Ctrl Pts',(4.19066754799994,11.6,-9.53396331100001));
#163296=CARTESIAN_POINT('Ctrl Pts',(4.19031247699994,15.2,-9.53278371900002));
#163297=CARTESIAN_POINT('Ctrl Pts',(4.19031247699994,11.6,-9.53278371900002));
#163298=CARTESIAN_POINT('Ctrl Pts',(4.18995878899994,15.2,-9.53161285200002));
#163299=CARTESIAN_POINT('Ctrl Pts',(4.18995878899994,11.6,-9.53161285200002));
#163300=CARTESIAN_POINT('Ctrl Pts',(4.18960650399994,15.2,-9.53045072400002));
#163301=CARTESIAN_POINT('Ctrl Pts',(4.18960650399994,11.6,-9.53045072400002));
#163302=CARTESIAN_POINT('Ctrl Pts',(4.18925564299994,15.2,-9.52929735300001));
#163303=CARTESIAN_POINT('Ctrl Pts',(4.18925564299994,11.6,-9.52929735300001));
#163304=CARTESIAN_POINT('Ctrl Pts',(4.18890623099994,15.2,-9.52815275900001));
#163305=CARTESIAN_POINT('Ctrl Pts',(4.18890623099994,11.6,-9.52815275900001));
#163306=CARTESIAN_POINT('Ctrl Pts',(4.18855828699995,15.2,-9.52701695700001));
#163307=CARTESIAN_POINT('Ctrl Pts',(4.18855828699995,11.6,-9.52701695700001));
#163308=CARTESIAN_POINT('Ctrl Pts',(4.18821183699994,15.2,-9.52588996600002));
#163309=CARTESIAN_POINT('Ctrl Pts',(4.18821183699994,11.6,-9.52588996600002));
#163310=CARTESIAN_POINT('Ctrl Pts',(4.18786690099994,15.2,-9.52477180400002));
#163311=CARTESIAN_POINT('Ctrl Pts',(4.18786690099994,11.6,-9.52477180400002));
#163312=CARTESIAN_POINT('Ctrl Pts',(4.18752350299994,15.2,-9.52366248700002));
#163313=CARTESIAN_POINT('Ctrl Pts',(4.18752350299994,11.6,-9.52366248700002));
#163314=CARTESIAN_POINT('Ctrl Pts',(4.18718166499994,15.2,-9.52256203500001));
#163315=CARTESIAN_POINT('Ctrl Pts',(4.18718166499994,11.6,-9.52256203500001));
#163316=CARTESIAN_POINT('Ctrl Pts',(4.18684140999994,15.2,-9.52147046600002));
#163317=CARTESIAN_POINT('Ctrl Pts',(4.18684140999994,11.6,-9.52147046600002));
#163318=CARTESIAN_POINT('Ctrl Pts',(4.18650276099994,15.2,-9.52038779600001));
#163319=CARTESIAN_POINT('Ctrl Pts',(4.18650276099994,11.6,-9.52038779600001));
#163320=CARTESIAN_POINT('Ctrl Pts',(4.18616574199994,15.2,-9.51931404500002));
#163321=CARTESIAN_POINT('Ctrl Pts',(4.18616574199994,11.6,-9.51931404500002));
#163322=CARTESIAN_POINT('Ctrl Pts',(4.18583037599995,15.2,-9.51824923000002));
#163323=CARTESIAN_POINT('Ctrl Pts',(4.18583037599995,11.6,-9.51824923000002));
#163324=CARTESIAN_POINT('Ctrl Pts',(4.18549668599994,15.2,-9.51719337100002));
#163325=CARTESIAN_POINT('Ctrl Pts',(4.18549668599994,11.6,-9.51719337100002));
#163326=CARTESIAN_POINT('Ctrl Pts',(4.18516469499994,15.2,-9.51614648400002));
#163327=CARTESIAN_POINT('Ctrl Pts',(4.18516469499994,11.6,-9.51614648400002));
#163328=CARTESIAN_POINT('Ctrl Pts',(4.18483442699995,15.2,-9.51510858900001));
#163329=CARTESIAN_POINT('Ctrl Pts',(4.18483442699995,11.6,-9.51510858900001));
#163330=CARTESIAN_POINT('Ctrl Pts',(4.18450590599994,15.2,-9.51407970500001));
#163331=CARTESIAN_POINT('Ctrl Pts',(4.18450590599994,11.6,-9.51407970500001));
#163332=CARTESIAN_POINT('Ctrl Pts',(4.18417915599994,15.2,-9.51305984900002));
#163333=CARTESIAN_POINT('Ctrl Pts',(4.18417915599994,11.6,-9.51305984900002));
#163334=CARTESIAN_POINT('Ctrl Pts',(4.18385420099994,15.2,-9.51204904000001));
#163335=CARTESIAN_POINT('Ctrl Pts',(4.18385420099994,11.6,-9.51204904000001));
#163336=CARTESIAN_POINT('Ctrl Pts',(4.18353106499994,15.2,-9.51104729700001));
#163337=CARTESIAN_POINT('Ctrl Pts',(4.18353106499994,11.6,-9.51104729700001));
#163338=CARTESIAN_POINT('Ctrl Pts',(4.18320977199994,15.2,-9.51005463900002));
#163339=CARTESIAN_POINT('Ctrl Pts',(4.18320977199994,11.6,-9.51005463900002));
#163340=CARTESIAN_POINT('Ctrl Pts',(4.18289034599994,15.2,-9.50907108500001));
#163341=CARTESIAN_POINT('Ctrl Pts',(4.18289034599994,11.6,-9.50907108500001));
#163342=CARTESIAN_POINT('Ctrl Pts',(4.18257281199994,15.2,-9.50809665400002));
#163343=CARTESIAN_POINT('Ctrl Pts',(4.18257281199994,11.6,-9.50809665400002));
#163344=CARTESIAN_POINT('Ctrl Pts',(4.18225719599994,15.2,-9.50713136500001));
#163345=CARTESIAN_POINT('Ctrl Pts',(4.18225719599994,11.6,-9.50713136500001));
#163346=CARTESIAN_POINT('Ctrl Pts',(4.18194351899994,15.2,-9.50617523600001));
#163347=CARTESIAN_POINT('Ctrl Pts',(4.18194351899994,11.6,-9.50617523600001));
#163348=CARTESIAN_POINT('Ctrl Pts',(4.18163180999994,15.2,-9.50522828700001));
#163349=CARTESIAN_POINT('Ctrl Pts',(4.18163180999994,11.6,-9.50522828700001));
#163350=CARTESIAN_POINT('Ctrl Pts',(4.18132209099995,15.2,-9.50429053800002));
#163351=CARTESIAN_POINT('Ctrl Pts',(4.18132209099995,11.6,-9.50429053800002));
#163352=CARTESIAN_POINT('Ctrl Pts',(4.18101438899994,15.2,-9.50336200800002));
#163353=CARTESIAN_POINT('Ctrl Pts',(4.18101438899994,11.6,-9.50336200800002));
#163354=CARTESIAN_POINT('Ctrl Pts',(4.18070872899994,15.2,-9.50244271600001));
#163355=CARTESIAN_POINT('Ctrl Pts',(4.18070872899994,11.6,-9.50244271600001));
#163356=CARTESIAN_POINT('Ctrl Pts',(4.18040513599994,15.2,-9.50153268300001));
#163357=CARTESIAN_POINT('Ctrl Pts',(4.18040513599994,11.6,-9.50153268300001));
#163358=CARTESIAN_POINT('Ctrl Pts',(4.18010363499994,15.2,-9.50063192600001));
#163359=CARTESIAN_POINT('Ctrl Pts',(4.18010363499994,11.6,-9.50063192600001));
#163360=CARTESIAN_POINT('Ctrl Pts',(4.17980425199994,15.2,-9.49974046600002));
#163361=CARTESIAN_POINT('Ctrl Pts',(4.17980425199994,11.6,-9.49974046600002));
#163362=CARTESIAN_POINT('Ctrl Pts',(4.17950701299994,15.2,-9.49885832400001));
#163363=CARTESIAN_POINT('Ctrl Pts',(4.17950701299994,11.6,-9.49885832400001));
#163364=CARTESIAN_POINT('Ctrl Pts',(4.17921364399994,15.2,-9.49799054600001));
#163365=CARTESIAN_POINT('Ctrl Pts',(4.17921364399994,11.6,-9.49799054600001));
#163366=CARTESIAN_POINT('Ctrl Pts',(4.17898101999994,15.2,-9.49730470700001));
#163367=CARTESIAN_POINT('Ctrl Pts',(4.17898101999994,11.6,-9.49730470700001));
#163368=CARTESIAN_POINT('Ctrl Pts',(4.17880795399994,15.2,-9.49679570900001));
#163369=CARTESIAN_POINT('Ctrl Pts',(4.17880795399994,11.6,-9.49679570900001));
#163370=CARTESIAN_POINT('Ctrl Pts',(4.17869357199994,15.2,-9.49645984600001));
#163371=CARTESIAN_POINT('Ctrl Pts',(4.17869357199994,11.6,-9.49645984600001));
#163372=CARTESIAN_POINT('Ctrl Pts',(4.17863732199994,15.2,-9.49629481100001));
#163373=CARTESIAN_POINT('Ctrl Pts',(4.17863732199994,11.6,-9.49629481100001));
#163374=CARTESIAN_POINT('',(4.17863732208248,12.2,-9.4962948105209));
#163375=CARTESIAN_POINT('',(4.17863732208248,15.2,-9.4962948105209));
#163376=CARTESIAN_POINT('',(4.17863732199994,12.2,-9.49629481000001));
#163377=CARTESIAN_POINT('Ctrl Pts',(4.27433546799994,12.2,-10.676144262));
#163378=CARTESIAN_POINT('Ctrl Pts',(4.2746137680505,12.2,-10.6723314813074));
#163379=CARTESIAN_POINT('Ctrl Pts',(4.2748872709057,12.2,-10.6685249864456));
#163380=CARTESIAN_POINT('Ctrl Pts',(4.2751559909999,12.2,-10.6647247761647));
#163381=CARTESIAN_POINT('Ctrl Pts',(4.2754247110941,12.2,-10.6609245658837));
#163382=CARTESIAN_POINT('Ctrl Pts',(4.27568864392904,12.2,-10.6571306401352));
#163383=CARTESIAN_POINT('Ctrl Pts',(4.27594779972479,12.2,-10.6533430149995));
#163384=CARTESIAN_POINT('Ctrl Pts',(4.27620695552054,12.2,-10.6495553898638));
#163385=CARTESIAN_POINT('Ctrl Pts',(4.27646133373731,12.2,-10.6457740655533));
#163386=CARTESIAN_POINT('Ctrl Pts',(4.27671095972889,12.2,-10.6419990773979));
#163387=CARTESIAN_POINT('Ctrl Pts',(4.27696058576582,12.2,-10.6382240885568));
#163388=CARTESIAN_POINT('Ctrl Pts',(4.27720545978473,12.2,-10.6344554361257));
#163389=CARTESIAN_POINT('Ctrl Pts',(4.27744560977733,12.2,-10.6306931631631));
#163390=CARTESIAN_POINT('Ctrl Pts',(4.27768575972629,12.2,-10.626930890884));
#163391=CARTESIAN_POINT('Ctrl Pts',(4.27792118546717,12.2,-10.6231749954379));
#163392=CARTESIAN_POINT('Ctrl Pts',(4.27815191029171,12.2,-10.6194255110747));
#163393=CARTESIAN_POINT('Ctrl Pts',(4.27845954337713,12.2,-10.6144261988175));
#163394=CARTESIAN_POINT('Ctrl Pts',(4.27875881764401,12.2,-10.6094382810372));
#163395=CARTESIAN_POINT('Ctrl Pts',(4.27904978419104,12.2,-10.6044618319721));
#163396=CARTESIAN_POINT('Ctrl Pts',(4.27934075077772,12.2,-10.5994853822291));
#163397=CARTESIAN_POINT('Ctrl Pts',(4.27962340913847,12.2,-10.5945204014255));
#163398=CARTESIAN_POINT('Ctrl Pts',(4.279897819764,12.2,-10.5895669733785));
#163399=CARTESIAN_POINT('Ctrl Pts',(4.28010362771445,12.2,-10.5858519026807));
#163400=CARTESIAN_POINT('Ctrl Pts',(4.28030479579045,12.2,-10.5821433307155));
#163401=CARTESIAN_POINT('Ctrl Pts',(4.28050134774165,12.2,-10.5784412905166));
#163402=CARTESIAN_POINT('Ctrl Pts',(4.28069789969284,12.2,-10.5747392503178));
#163403=CARTESIAN_POINT('Ctrl Pts',(4.28088983600255,12.2,-10.5710437420354));
#163404=CARTESIAN_POINT('Ctrl Pts',(4.28107717949615,12.2,-10.5673547988772));
#163405=CARTESIAN_POINT('Ctrl Pts',(4.28132697084363,12.2,-10.5624362075528));
#163406=CARTESIAN_POINT('Ctrl Pts',(4.28156859751846,12.2,-10.5575292890111));
#163407=CARTESIAN_POINT('Ctrl Pts',(4.28180211804215,12.2,-10.5526341220564));
#163408=CARTESIAN_POINT('Ctrl Pts',(4.28197725841901,12.2,-10.5489627471738));
#163409=CARTESIAN_POINT('Ctrl Pts',(4.28214783862442,12.2,-10.5452979845345));
#163410=CARTESIAN_POINT('Ctrl Pts',(4.28231388403466,12.2,-10.5416398658764));
#163411=CARTESIAN_POINT('Ctrl Pts',(4.28247992944491,12.2,-10.5379817472182));
#163412=CARTESIAN_POINT('Ctrl Pts',(4.28264143902235,12.2,-10.5343302737509));
#163413=CARTESIAN_POINT('Ctrl Pts',(4.28279843847498,12.2,-10.5306854804666));
#163414=CARTESIAN_POINT('Ctrl Pts',(4.28295543792761,12.2,-10.5270406871824));
#163415=CARTESIAN_POINT('Ctrl Pts',(4.28310792682209,12.2,-10.5234025726479));
#163416=CARTESIAN_POINT('Ctrl Pts',(4.2832559306921,12.2,-10.5197711724042));
#163417=CARTESIAN_POINT('Ctrl Pts',(4.28340393456211,12.2,-10.5161397721606));
#163418=CARTESIAN_POINT('Ctrl Pts',(4.28354745203728,12.2,-10.5125150865667));
#163419=CARTESIAN_POINT('Ctrl Pts',(4.28368650949803,12.2,-10.508897148225));
#163420=CARTESIAN_POINT('Ctrl Pts',(4.28382556695877,12.2,-10.5052792098833));
#163421=CARTESIAN_POINT('Ctrl Pts',(4.28396016469238,12.2,-10.5016680202057));
#163422=CARTESIAN_POINT('Ctrl Pts',(4.28409032672993,12.2,-10.4980636135024));
#163423=CARTESIAN_POINT('Ctrl Pts',(4.28422048879112,12.2,-10.4944592061443));
#163424=CARTESIAN_POINT('Ctrl Pts',(4.28434621655939,12.2,-10.4908615818381));
#163425=CARTESIAN_POINT('Ctrl Pts',(4.28446753503475,12.2,-10.4872707754838));
#163426=CARTESIAN_POINT('Ctrl Pts',(4.28458885348807,12.2,-10.4836799697819));
#163427=CARTESIAN_POINT('Ctrl Pts',(4.28470576256664,12.2,-10.4800959827796));
#163428=CARTESIAN_POINT('Ctrl Pts',(4.28481828806217,12.2,-10.4765188476185));
#163429=CARTESIAN_POINT('Ctrl Pts',(4.2849308135577,12.2,-10.4729417124574));
#163430=CARTESIAN_POINT('Ctrl Pts',(4.28503895598708,12.2,-10.4693714302705));
#163431=CARTESIAN_POINT('Ctrl Pts',(4.28514274052498,12.2,-10.4658080359833));
#163432=CARTESIAN_POINT('Ctrl Pts',(4.28524652506287,12.2,-10.4622446416961));
#163433=CARTESIAN_POINT('Ctrl Pts',(4.28534595230928,12.2,-10.4586881344586));
#163434=CARTESIAN_POINT('Ctrl Pts',(4.28544104922287,12.2,-10.455138550712));
#163435=CARTESIAN_POINT('Ctrl Pts',(4.28553614613646,12.2,-10.4515889669654));
#163436=CARTESIAN_POINT('Ctrl Pts',(4.28562691053153,12.2,-10.4480463062664));
#163437=CARTESIAN_POINT('Ctrl Pts',(4.28571337194987,12.2,-10.4445106034258));
#163438=CARTESIAN_POINT('Ctrl Pts',(4.28582865385147,12.2,-10.4397963325434));
#163439=CARTESIAN_POINT('Ctrl Pts',(4.28593628328645,12.2,-10.4350944329854));
#163440=CARTESIAN_POINT('Ctrl Pts',(4.28603632329141,12.2,-10.4304049863417));
#163441=CARTESIAN_POINT('Ctrl Pts',(4.28611135328832,12.2,-10.4268879016785));
#163442=CARTESIAN_POINT('Ctrl Pts',(4.28618211403573,12.2,-10.4233778230227));
#163443=CARTESIAN_POINT('Ctrl Pts',(4.28624863444998,12.2,-10.419874785275));
#163444=CARTESIAN_POINT('Ctrl Pts',(4.28631515486423,12.2,-10.4163717475272));
#163445=CARTESIAN_POINT('Ctrl Pts',(4.28637743254532,12.2,-10.4128757500875));
#163446=CARTESIAN_POINT('Ctrl Pts',(4.28643549696024,12.2,-10.4093868298804));
#163447=CARTESIAN_POINT('Ctrl Pts',(4.28649356137516,12.2,-10.4058979096732));
#163448=CARTESIAN_POINT('Ctrl Pts',(4.28654741123916,12.2,-10.4024160662705));
#163449=CARTESIAN_POINT('Ctrl Pts',(4.28659707424032,12.2,-10.398941335389));
#163450=CARTESIAN_POINT('Ctrl Pts',(4.28664673724149,12.2,-10.3954666045075));
#163451=CARTESIAN_POINT('Ctrl Pts',(4.28669221347523,12.2,-10.3919989867296));
#163452=CARTESIAN_POINT('Ctrl Pts',(4.2867335309743,12.2,-10.388538517021));
#163453=CARTESIAN_POINT('Ctrl Pts',(4.28677484848087,12.2,-10.3850780466838));
#163454=CARTESIAN_POINT('Ctrl Pts',(4.2868120067696,12.2,-10.3816247246152));
#163455=CARTESIAN_POINT('Ctrl Pts',(4.28684503473217,12.2,-10.3781785877404));
#163456=CARTESIAN_POINT('Ctrl Pts',(4.28690008132845,12.2,-10.372435027117));
#163457=CARTESIAN_POINT('Ctrl Pts',(4.28694365195511,12.2,-10.3667114235912));
#163458=CARTESIAN_POINT('Ctrl Pts',(4.28697588028752,12.2,-10.3610079455373));
#163459=CARTESIAN_POINT('Ctrl Pts',(4.28699521728626,12.2,-10.3575858588293));
#163460=CARTESIAN_POINT('Ctrl Pts',(4.28701047146908,12.2,-10.3541710171863));
#163461=CARTESIAN_POINT('Ctrl Pts',(4.28702167001043,12.2,-10.3507634568491));
#163462=CARTESIAN_POINT('Ctrl Pts',(4.28703286855178,12.2,-10.3473558965118));
#163463=CARTESIAN_POINT('Ctrl Pts',(4.28704001178405,12.2,-10.3439556180897));
#163464=CARTESIAN_POINT('Ctrl Pts',(4.28704312978358,12.2,-10.3405626583803));
#163465=CARTESIAN_POINT('Ctrl Pts',(4.28704624778312,12.2,-10.3371696986708));
#163466=CARTESIAN_POINT('Ctrl Pts',(4.28704533964979,12.2,-10.3337840569105));
#163467=CARTESIAN_POINT('Ctrl Pts',(4.28704043477497,12.2,-10.3304057702));
#163468=CARTESIAN_POINT('Ctrl Pts',(4.28703552990015,12.2,-10.3270274834894));
#163469=CARTESIAN_POINT('Ctrl Pts',(4.28702662958383,12.2,-10.3236565510785));
#163470=CARTESIAN_POINT('Ctrl Pts',(4.28701376075131,12.2,-10.320293011825));
#163471=CARTESIAN_POINT('Ctrl Pts',(4.28700089191879,12.2,-10.3169294725716));
#163472=CARTESIAN_POINT('Ctrl Pts',(4.28698405667044,12.2,-10.3135733256111));
#163473=CARTESIAN_POINT('Ctrl Pts',(4.28696328375395,12.2,-10.3102246058979));
#163474=CARTESIAN_POINT('Ctrl Pts',(4.28694251083746,12.2,-10.3068758861848));
#163475=CARTESIAN_POINT('Ctrl Pts',(4.28691780063797,12.2,-10.3035345972566));
#163476=CARTESIAN_POINT('Ctrl Pts',(4.28688918276454,12.2,-10.3002007732101));
#163477=CARTESIAN_POINT('Ctrl Pts',(4.2868510255965,12.2,-10.2957556740776));
#163478=CARTESIAN_POINT('Ctrl Pts',(4.28680592245558,12.2,-10.2913238493185));
#163479=CARTESIAN_POINT('Ctrl Pts',(4.28675394450831,12.2,-10.2869053859666));
#163480=CARTESIAN_POINT('Ctrl Pts',(4.28670196656103,12.2,-10.2824869226147));
#163481=CARTESIAN_POINT('Ctrl Pts',(4.28664311386295,12.2,-10.2780818205838));
#163482=CARTESIAN_POINT('Ctrl Pts',(4.28657745924757,12.2,-10.2736901699569));
#163483=CARTESIAN_POINT('Ctrl Pts',(4.28649539099176,12.2,-10.2682006075709));
#163484=CARTESIAN_POINT('Ctrl Pts',(4.28640269561802,12.2,-10.2627320619871));
#163485=CARTESIAN_POINT('Ctrl Pts',(4.28629951500513,12.2,-10.2572847079958));
#163486=CARTESIAN_POINT('Ctrl Pts',(4.28621697050132,12.2,-10.2529268240903));
#163487=CARTESIAN_POINT('Ctrl Pts',(4.28612771656075,12.2,-10.2485825037332));
#163488=CARTESIAN_POINT('Ctrl Pts',(4.28603182799997,12.2,-10.244251835775));
#163489=CARTESIAN_POINT('Ctrl Pts',(4.28593593943919,12.2,-10.2399211678167));
#163490=CARTESIAN_POINT('Ctrl Pts',(4.28583341522764,12.2,-10.2356041526906));
#163491=CARTESIAN_POINT('Ctrl Pts',(4.2857243319988,12.2,-10.231300882013));
#163492=CARTESIAN_POINT('Ctrl Pts',(4.28561524878483,12.2,-10.2269976119218));
#163493=CARTESIAN_POINT('Ctrl Pts',(4.28549960651005,12.2,-10.22270808517));
#163494=CARTESIAN_POINT('Ctrl Pts',(4.28537748124172,12.2,-10.2184323937779));
#163495=CARTESIAN_POINT('Ctrl Pts',(4.28525535595675,12.2,-10.2141567018032));
#163496=CARTESIAN_POINT('Ctrl Pts',(4.28512674726368,12.2,-10.2098948440522));
#163497=CARTESIAN_POINT('Ctrl Pts',(4.28499173347789,12.2,-10.2056469128221));
#163498=CARTESIAN_POINT('Ctrl Pts',(4.2848567197105,12.2,-10.2013989821708));
#163499=CARTESIAN_POINT('Ctrl Pts',(4.28471530159672,12.2,-10.1971649792982));
#163500=CARTESIAN_POINT('Ctrl Pts',(4.28456755522032,12.2,-10.1929449945867));
#163501=CARTESIAN_POINT('Ctrl Pts',(4.28441980882379,12.2,-10.1887250093003));
#163502=CARTESIAN_POINT('Ctrl Pts',(4.28426573658285,12.2,-10.1845190427645));
#163503=CARTESIAN_POINT('Ctrl Pts',(4.28410541601,12.2,-10.1803271873834));
#163504=CARTESIAN_POINT('Ctrl Pts',(4.283945095459,12.2,-10.1761353325735));
#163505=CARTESIAN_POINT('Ctrl Pts',(4.28377852752729,12.2,-10.1719575896982));
#163506=CARTESIAN_POINT('Ctrl Pts',(4.28360579176403,12.2,-10.1677940523155));
#163507=CARTESIAN_POINT('Ctrl Pts',(4.28343305597724,12.2,-10.1636305143654));
#163508=CARTESIAN_POINT('Ctrl Pts',(4.28325415353694,12.2,-10.1594811802754));
#163509=CARTESIAN_POINT('Ctrl Pts',(4.28306916502645,12.2,-10.155346146162));
#163510=CARTESIAN_POINT('Ctrl Pts',(4.28288417654118,12.2,-10.1512111126121));
#163511=CARTESIAN_POINT('Ctrl Pts',(4.2826931009273,12.2,-10.1470903770499));
#163512=CARTESIAN_POINT('Ctrl Pts',(4.2824960230452,12.2,-10.1429840348459));
#163513=CARTESIAN_POINT('Ctrl Pts',(4.28224967567244,12.2,-10.1378511066713));
#163514=CARTESIAN_POINT('Ctrl Pts',(4.2819939471612,12.2,-10.1327406666618));
#163515=CARTESIAN_POINT('Ctrl Pts',(4.28172900000891,12.2,-10.1276529028412));
#163516=CARTESIAN_POINT('Ctrl Pts',(4.28151704227552,12.2,-10.1235826915628));
#163517=CARTESIAN_POINT('Ctrl Pts',(4.28129918608864,12.2,-10.1195269929862));
#163518=CARTESIAN_POINT('Ctrl Pts',(4.28107551496496,12.2,-10.1154859017114));
#163519=CARTESIAN_POINT('Ctrl Pts',(4.2807959260756,12.2,-10.1104345378932));
#163520=CARTESIAN_POINT('Ctrl Pts',(4.28050725211425,12.2,-10.1054059961993));
#163521=CARTESIAN_POINT('Ctrl Pts',(4.28020965919712,12.2,-10.1004004698811));
#163522=CARTESIAN_POINT('Ctrl Pts',(4.27997158488287,12.2,-10.0963960491538));
#163523=CARTESIAN_POINT('Ctrl Pts',(4.27972780382215,12.2,-10.092406356499));
#163524=CARTESIAN_POINT('Ctrl Pts',(4.27947840205279,12.2,-10.0884314889018));
#163525=CARTESIAN_POINT('Ctrl Pts',(4.27922900024945,12.2,-10.0844566207631));
#163526=CARTESIAN_POINT('Ctrl Pts',(4.2789739780904,12.2,-10.0804965767916));
#163527=CARTESIAN_POINT('Ctrl Pts',(4.27871342368695,12.2,-10.0765514569109));
#163528=CARTESIAN_POINT('Ctrl Pts',(4.278452869319,12.2,-10.0726063375677));
#163529=CARTESIAN_POINT('Ctrl Pts',(4.27818678276605,12.2,-10.068676141191));
#163530=CARTESIAN_POINT('Ctrl Pts',(4.27791525301103,12.2,-10.0647609658984));
#163531=CARTESIAN_POINT('Ctrl Pts',(4.27764372321901,12.2,-10.0608457900724));
#163532=CARTESIAN_POINT('Ctrl Pts',(4.2773667503609,12.2,-10.0569456361822));
#163533=CARTESIAN_POINT('Ctrl Pts',(4.27708442523311,12.2,-10.0530606017306));
#163534=CARTESIAN_POINT('Ctrl Pts',(4.27680210014377,12.2,-10.0491755678084));
#163535=CARTESIAN_POINT('Ctrl Pts',(4.27651442160393,12.2,-10.0453056540305));
#163536=CARTESIAN_POINT('Ctrl Pts',(4.27622148257286,12.2,-10.0414509606219));
#163537=CARTESIAN_POINT('Ctrl Pts',(4.27592854350188,12.2,-10.037596266688));
#163538=CARTESIAN_POINT('Ctrl Pts',(4.27563034234705,12.2,-10.0337567919084));
#163539=CARTESIAN_POINT('Ctrl Pts',(4.27532697327497,12.2,-10.0299326380333));
#163540=CARTESIAN_POINT('Ctrl Pts',(4.27502360420288,12.2,-10.0261084841582));
#163541=CARTESIAN_POINT('Ctrl Pts',(4.27471506726908,12.2,-10.0222996500127));
#163542=CARTESIAN_POINT('Ctrl Pts',(4.27440145497368,12.2,-10.0185062363631));
#163543=CARTESIAN_POINT('Ctrl Pts',(4.27408784272103,12.2,-10.0147128232303));
#163544=CARTESIAN_POINT('Ctrl Pts',(4.27376915555851,12.2,-10.0109348329621));
#163545=CARTESIAN_POINT('Ctrl Pts',(4.27344548925018,12.2,-10.0071723642525));
#163546=CARTESIAN_POINT('Ctrl Pts',(4.27312182289776,12.2,-10.0034098950303));
#163547=CARTESIAN_POINT('Ctrl Pts',(4.27279317853633,12.2,-9.99966294735831));
#163548=CARTESIAN_POINT('Ctrl Pts',(4.2724596489621,12.2,-9.99593162615656));
#163549=CARTESIAN_POINT('Ctrl Pts',(4.27212611943331,12.2,-9.9922003054632));
#163550=CARTESIAN_POINT('Ctrl Pts',(4.2717877071496,12.2,-9.98848460878722));
#163551=CARTESIAN_POINT('Ctrl Pts',(4.27144450951131,12.2,-9.98478464081091));
#163552=CARTESIAN_POINT('Ctrl Pts',(4.27110131182625,12.2,-9.98108467233047));
#163553=CARTESIAN_POINT('Ctrl Pts',(4.27075332839156,12.2,-9.97740043194123));
#163554=CARTESIAN_POINT('Ctrl Pts',(4.27040065746543,12.2,-9.97373202272606));
#163555=CARTESIAN_POINT('Ctrl Pts',(4.27004798658734,12.2,-9.97006361401071));
#163556=CARTESIAN_POINT('Ctrl Pts',(4.26969062894684,12.2,-9.96641103862611));
#163557=CARTESIAN_POINT('Ctrl Pts',(4.26932868525451,12.2,-9.96277439808907));
#163558=CARTESIAN_POINT('Ctrl Pts',(4.26896674151286,12.2,-9.95913775705652));
#163559=CARTESIAN_POINT('Ctrl Pts',(4.26860021071232,12.2,-9.95551705300081));
#163560=CARTESIAN_POINT('Ctrl Pts',(4.26822919446959,12.2,-9.95191239047209));
#163561=CARTESIAN_POINT('Ctrl Pts',(4.2678581782774,12.2,-9.9483077284345));
#163562=CARTESIAN_POINT('Ctrl Pts',(4.26748267689538,12.2,-9.94471910788127));
#163563=CARTESIAN_POINT('Ctrl Pts',(4.26710279329673,12.2,-9.94114663449343));
#163564=CARTESIAN_POINT('Ctrl Pts',(4.26662793875959,12.2,-9.93668104239357));
#163565=CARTESIAN_POINT('Ctrl Pts',(4.2661462359204,12.2,-9.93224068120685));
#163566=CARTESIAN_POINT('Ctrl Pts',(4.26565788974019,12.2,-9.9278257593305));
#163567=CARTESIAN_POINT('Ctrl Pts',(4.26526721277473,12.2,-9.92429382163693));
#163568=CARTESIAN_POINT('Ctrl Pts',(4.26487228374765,12.2,-9.92077816529257));
#163569=CARTESIAN_POINT('Ctrl Pts',(4.26447320822563,12.2,-9.91727889821404));
#163570=CARTESIAN_POINT('Ctrl Pts',(4.26407413275798,12.2,-9.91377963161228));
#163571=CARTESIAN_POINT('Ctrl Pts',(4.26367091081518,12.2,-9.91029675358315));
#163572=CARTESIAN_POINT('Ctrl Pts',(4.2632636505507,12.2,-9.9068303734697));
#163573=CARTESIAN_POINT('Ctrl Pts',(4.26285639023073,12.2,-9.90336399288394));
#163574=CARTESIAN_POINT('Ctrl Pts',(4.2624450909972,12.2,-9.89991411022768));
#163575=CARTESIAN_POINT('Ctrl Pts',(4.26202986147431,12.2,-9.8964808344861));
#163576=CARTESIAN_POINT('Ctrl Pts',(4.261614632008,12.2,-9.89304755921231));
#163577=CARTESIAN_POINT('Ctrl Pts',(4.26119547324526,12.2,-9.88963089191018));
#163578=CARTESIAN_POINT('Ctrl Pts',(4.26077249383578,12.2,-9.88623094079752));
#163579=CARTESIAN_POINT('Ctrl Pts',(4.26034951436868,12.2,-9.88283098922162));
#163580=CARTESIAN_POINT('Ctrl Pts',(4.25992271671955,12.2,-9.8794477559825));
#163581=CARTESIAN_POINT('Ctrl Pts',(4.25949220924966,12.2,-9.87608135150599));
#163582=CARTESIAN_POINT('Ctrl Pts',(4.25906170183844,12.2,-9.87271494748816));
#163583=CARTESIAN_POINT('Ctrl Pts',(4.25862748729927,12.2,-9.86936537056578));
#163584=CARTESIAN_POINT('Ctrl Pts',(4.25818967727987,12.2,-9.86603273600318));
#163585=CARTESIAN_POINT('Ctrl Pts',(4.25775186720083,12.2,-9.86270010098649));
#163586=CARTESIAN_POINT('Ctrl Pts',(4.25731046255198,12.2,-9.85938440577137));
#163587=CARTESIAN_POINT('Ctrl Pts',(4.25686557841663,12.2,-9.85608576475827));
#163588=CARTESIAN_POINT('Ctrl Pts',(4.25630947327774,12.2,-9.85196246371662));
#163589=CARTESIAN_POINT('Ctrl Pts',(4.25574793029668,12.2,-9.84786580924946));
#163590=CARTESIAN_POINT('Ctrl Pts',(4.25518117772465,12.2,-9.84379602402273));
#163591=CARTESIAN_POINT('Ctrl Pts',(4.25461442515262,12.2,-9.83972623879599));
#163592=CARTESIAN_POINT('Ctrl Pts',(4.25404246493468,12.2,-9.83568332263054));
#163593=CARTESIAN_POINT('Ctrl Pts',(4.25346552500386,12.2,-9.83166750068747));
#163594=CARTESIAN_POINT('Ctrl Pts',(4.25277319711204,12.2,-9.82684851453089));
#163595=CARTESIAN_POINT('Ctrl Pts',(4.25207370237079,12.2,-9.82206854334627));
#163596=CARTESIAN_POINT('Ctrl Pts',(4.25136744731342,12.2,-9.8173279812668));
#163597=CARTESIAN_POINT('Ctrl Pts',(4.25077890141088,12.2,-9.8133775127237));
#163598=CARTESIAN_POINT('Ctrl Pts',(4.25018566173878,12.2,-9.80945441318965));
#163599=CARTESIAN_POINT('Ctrl Pts',(4.24958796923902,12.2,-9.80555890902155));
#163600=CARTESIAN_POINT('Ctrl Pts',(4.24899027673925,12.2,-9.80166340485343));
#163601=CARTESIAN_POINT('Ctrl Pts',(4.24838813182525,12.2,-9.79779550100289));
#163602=CARTESIAN_POINT('Ctrl Pts',(4.24778177772528,12.2,-9.79395542598537));
#163603=CARTESIAN_POINT('Ctrl Pts',(4.24717542362532,12.2,-9.79011535096786));
#163604=CARTESIAN_POINT('Ctrl Pts',(4.24656486389995,12.2,-9.78630310733326));
#163605=CARTESIAN_POINT('Ctrl Pts',(4.24595034473329,12.2,-9.78251892899994));
#163606=CARTESIAN_POINT('Ctrl Pts',(4.24533582556662,12.2,-9.77873475066662));
#163607=CARTESIAN_POINT('Ctrl Pts',(4.24471734990801,12.2,-9.77497863845365));
#163608=CARTESIAN_POINT('Ctrl Pts',(4.24409516997461,12.2,-9.77125083225624));
#163609=CARTESIAN_POINT('Ctrl Pts',(4.24347299004122,12.2,-9.76752302605884));
#163610=CARTESIAN_POINT('Ctrl Pts',(4.24284710615895,12.2,-9.76382352200855));
#163611=CARTESIAN_POINT('Ctrl Pts',(4.24221777865877,12.2,-9.76015256451003));
#163612=CARTESIAN_POINT('Ctrl Pts',(4.24158845115859,12.2,-9.75648160701152));
#163613=CARTESIAN_POINT('Ctrl Pts',(4.24095567811962,12.2,-9.75283919410117));
#163614=CARTESIAN_POINT('Ctrl Pts',(4.24031972575834,12.2,-9.74922557146379));
#163615=CARTESIAN_POINT('Ctrl Pts',(4.23968377339707,12.2,-9.74561194882641));
#163616=CARTESIAN_POINT('Ctrl Pts',(4.23904463977991,12.2,-9.7420271150351));
#163617=CARTESIAN_POINT('Ctrl Pts',(4.23840259419208,12.2,-9.7384713165956));
#163618=CARTESIAN_POINT('Ctrl Pts',(4.23776054860424,12.2,-9.73491551815611));
#163619=CARTESIAN_POINT('Ctrl Pts',(4.23711559168213,12.2,-9.73138875522341));
#163620=CARTESIAN_POINT('Ctrl Pts',(4.23646799689025,12.2,-9.72789127855915));
#163621=CARTESIAN_POINT('Ctrl Pts',(4.23582040209837,12.2,-9.72439380189489));
#163622=CARTESIAN_POINT('Ctrl Pts',(4.23517016901478,12.2,-9.72092561036443));
#163623=CARTESIAN_POINT('Ctrl Pts',(4.23451757818126,12.2,-9.71748695703351));
#163624=CARTESIAN_POINT('Ctrl Pts',(4.23386498741887,12.2,-9.71404830407741));
#163625=CARTESIAN_POINT('Ctrl Pts',(4.23321003533077,12.2,-9.7106391905816));
#163626=CARTESIAN_POINT('Ctrl Pts',(4.23255301061089,12.2,-9.70725987018364));
#163627=CARTESIAN_POINT('Ctrl Pts',(4.23189598581939,12.2,-9.70388054941731));
#163628=CARTESIAN_POINT('Ctrl Pts',(4.23123688711402,12.2,-9.70053102324771));
#163629=CARTESIAN_POINT('Ctrl Pts',(4.23057600329473,12.2,-9.6972115506758));
#163630=CARTESIAN_POINT('Ctrl Pts',(4.22991511947543,12.2,-9.6938920781039));
#163631=CARTESIAN_POINT('Ctrl Pts',(4.22925245145457,12.2,-9.69060265873774));
#163632=CARTESIAN_POINT('Ctrl Pts',(4.22858829426871,12.2,-9.68734355537837));
#163633=CARTESIAN_POINT('Ctrl Pts',(4.22779130560224,12.2,-9.68343263113398));
#163634=CARTESIAN_POINT('Ctrl Pts',(4.22699217283975,12.2,-9.67956536218024));
#163635=CARTESIAN_POINT('Ctrl Pts',(4.22619141896266,12.2,-9.67574221005821));
#163636=CARTESIAN_POINT('Ctrl Pts',(4.22539066515831,12.2,-9.67191905828345));
#163637=CARTESIAN_POINT('Ctrl Pts',(4.22458828713237,12.2,-9.66814002158775));
#163638=CARTESIAN_POINT('Ctrl Pts',(4.22378482274125,12.2,-9.66440556795657));
#163639=CARTESIAN_POINT('Ctrl Pts',(4.22298135835012,12.2,-9.6606711143254));
#163640=CARTESIAN_POINT('Ctrl Pts',(4.22217680546455,12.2,-9.65698124532664));
#163641=CARTESIAN_POINT('Ctrl Pts',(4.22137171399382,12.2,-9.6533364357071));
#163642=CARTESIAN_POINT('Ctrl Pts',(4.22056662244997,12.2,-9.64969162575649));
#163643=CARTESIAN_POINT('Ctrl Pts',(4.21976099074771,12.2,-9.64609187720316));
#163644=CARTESIAN_POINT('Ctrl Pts',(4.2189553794538,12.2,-9.64253767034587));
#163645=CARTESIAN_POINT('Ctrl Pts',(4.21814976823306,12.2,-9.6389834638114));
#163646=CARTESIAN_POINT('Ctrl Pts',(4.21734417884347,12.2,-9.63547480150858));
#163647=CARTESIAN_POINT('Ctrl Pts',(4.21653918470607,12.2,-9.63201217505308));
#163648=CARTESIAN_POINT('Ctrl Pts',(4.21573419056868,12.2,-9.62854954859757));
#163649=CARTESIAN_POINT('Ctrl Pts',(4.21492979253959,12.2,-9.62513295887173));
#163650=CARTESIAN_POINT('Ctrl Pts',(4.21412658031872,12.2,-9.6217629064088));
#163651=CARTESIAN_POINT('Ctrl Pts',(4.21332336809785,12.2,-9.61839285394588));
#163652=CARTESIAN_POINT('Ctrl Pts',(4.21252134088321,12.2,-9.61506933862457));
#163653=CARTESIAN_POINT('Ctrl Pts',(4.21172110482883,12.2,-9.61179287207375));
#163654=CARTESIAN_POINT('Ctrl Pts',(4.21092086870177,12.2,-9.60851640522533));
#163655=CARTESIAN_POINT('Ctrl Pts',(4.21012242302485,12.2,-9.60528698688144));
#163656=CARTESIAN_POINT('Ctrl Pts',(4.20932638789823,12.2,-9.60210513604339));
#163657=CARTESIAN_POINT('Ctrl Pts',(4.20853035284392,12.2,-9.59892328549437));
#163658=CARTESIAN_POINT('Ctrl Pts',(4.20773672901444,12.2,-9.59578900274161));
#163659=CARTESIAN_POINT('Ctrl Pts',(4.20694615204304,12.2,-9.592702819185));
#163660=CARTESIAN_POINT('Ctrl Pts',(4.20615557507164,12.2,-9.5896166356284));
#163661=CARTESIAN_POINT('Ctrl Pts',(4.20536804692382,12.2,-9.58657854854552));
#163662=CARTESIAN_POINT('Ctrl Pts',(4.20458421811871,12.2,-9.58358910206746));
#163663=CARTESIAN_POINT('Ctrl Pts',(4.20380038924239,12.2,-9.58059965531785));
#163664=CARTESIAN_POINT('Ctrl Pts',(4.20302026286642,12.2,-9.57765884703963));
#163665=CARTESIAN_POINT('Ctrl Pts',(4.202244507991,12.2,-9.57476722780085));
#163666=CARTESIAN_POINT('Ctrl Pts',(4.20146875318605,12.2,-9.57187560882474));
#163667=CARTESIAN_POINT('Ctrl Pts',(4.20069737085927,12.2,-9.56903318279588));
#163668=CARTESIAN_POINT('Ctrl Pts',(4.19993105121695,12.2,-9.5662405075512));
#163669=CARTESIAN_POINT('Ctrl Pts',(4.19916473157463,12.2,-9.56344783230653));
#163670=CARTESIAN_POINT('Ctrl Pts',(4.19840347353022,12.2,-9.56070490974903));
#163671=CARTESIAN_POINT('Ctrl Pts',(4.19764798780728,12.2,-9.55801231551009));
#163672=CARTESIAN_POINT('Ctrl Pts',(4.19689250201572,12.2,-9.5553197210266));
#163673=CARTESIAN_POINT('Ctrl Pts',(4.19614278553032,12.2,-9.55267745292545));
#163674=CARTESIAN_POINT('Ctrl Pts',(4.19539957170305,12.2,-9.55008610124103));
#163675=CARTESIAN_POINT('Ctrl Pts',(4.1946563579433,12.2,-9.54749474979199));
#163676=CARTESIAN_POINT('Ctrl Pts',(4.19391964279843,12.2,-9.54495431150118));
#163677=CARTESIAN_POINT('Ctrl Pts',(4.1931901792416,12.2,-9.54246538850825));
#163678=CARTESIAN_POINT('Ctrl Pts',(4.19246071568476,12.2,-9.53997646551533));
#163679=CARTESIAN_POINT('Ctrl Pts',(4.19173850177923,12.2,-9.537539057833));
#163680=CARTESIAN_POINT('Ctrl Pts',(4.19102431110237,12.2,-9.53515377946413));
#163681=CARTESIAN_POINT('Ctrl Pts',(4.19031012036064,12.2,-9.53276850087861));
#163682=CARTESIAN_POINT('Ctrl Pts',(4.18960395026966,12.2,-9.53043535007207));
#163683=CARTESIAN_POINT('Ctrl Pts',(4.18890659798225,12.2,-9.52815495678469));
#163684=CARTESIAN_POINT('Ctrl Pts',(4.18820924575818,12.2,-9.52587456370444));
#163685=CARTESIAN_POINT('Ctrl Pts',(4.18752071156967,12.2,-9.52364692671298));
#163686=CARTESIAN_POINT('Ctrl Pts',(4.18684181150795,12.2,-9.52147269078225));
#163687=CARTESIAN_POINT('Ctrl Pts',(4.18616291144622,12.2,-9.51929845485151));
#163688=CARTESIAN_POINT('Ctrl Pts',(4.18549364876241,12.2,-9.51717761777342));
#163689=CARTESIAN_POINT('Ctrl Pts',(4.18483486378587,12.2,-9.51511084184611));
#163690=CARTESIAN_POINT('Ctrl Pts',(4.18417607874951,12.2,-9.51304406573107));
#163691=CARTESIAN_POINT('Ctrl Pts',(4.18352777472325,12.2,-9.51103134747431));
#163692=CARTESIAN_POINT('Ctrl Pts',(4.18289081893893,12.2,-9.50907336553681));
#163693=CARTESIAN_POINT('Ctrl Pts',(4.18225386321247,12.2,-9.50711538377718));
#163694=CARTESIAN_POINT('Ctrl Pts',(4.18162825727706,12.2,-9.50521213601322));
#163695=CARTESIAN_POINT('Ctrl Pts',(4.18101489946655,12.2,-9.50336431741611));
#163696=CARTESIAN_POINT('Ctrl Pts',(4.18020003270377,12.2,-9.50090942741129));
#163697=CARTESIAN_POINT('Ctrl Pts',(4.17940677983145,12.2,-9.4985523660795));
#163698=CARTESIAN_POINT('Ctrl Pts',(4.17863732199994,12.2,-9.49629481100001));
#163699=CARTESIAN_POINT('Ctrl Pts',(4.17863732199994,15.2,-9.49629481100001));
#163700=CARTESIAN_POINT('Ctrl Pts',(4.1792137204524,15.2,-9.49798593844179));
#163701=CARTESIAN_POINT('Ctrl Pts',(4.17980347320419,15.2,-9.49973290552696));
#163702=CARTESIAN_POINT('Ctrl Pts',(4.18040565894231,15.2,-9.5015350018359));
#163703=CARTESIAN_POINT('Ctrl Pts',(4.18101074872444,15.2,-9.50334578876415));
#163704=CARTESIAN_POINT('Ctrl Pts',(4.18162839197776,15.2,-9.50521224016538));
#163705=CARTESIAN_POINT('Ctrl Pts',(4.18225768087749,15.2,-9.50713365520259));
#163706=CARTESIAN_POINT('Ctrl Pts',(4.18288696972008,15.2,-9.50905507006526));
#163707=CARTESIAN_POINT('Ctrl Pts',(4.18352790377333,15.2,-9.51103144898949));
#163708=CARTESIAN_POINT('Ctrl Pts',(4.18417960475002,15.2,-9.5130621107502));
#163709=CARTESIAN_POINT('Ctrl Pts',(4.18483130572671,15.2,-9.5150927725109));
#163710=CARTESIAN_POINT('Ctrl Pts',(4.18549377400967,15.2,-9.51717771587551));
#163711=CARTESIAN_POINT('Ctrl Pts',(4.18616615518491,15.2,-9.51931627881818));
#163712=CARTESIAN_POINT('Ctrl Pts',(4.18683853642122,15.2,-9.52145484195509));
#163713=CARTESIAN_POINT('Ctrl Pts',(4.18752083323699,15.2,-9.52364702318536));
#163714=CARTESIAN_POINT('Ctrl Pts',(4.18821221560862,15.2,-9.52589217347798));
#163715=CARTESIAN_POINT('Ctrl Pts',(4.18890359791745,15.2,-9.52813732356665));
#163716=CARTESIAN_POINT('Ctrl Pts',(4.1896040674811,15.2,-9.53043544418394));
#163717=CARTESIAN_POINT('Ctrl Pts',(4.19031282270859,15.2,-9.53278590019266));
#163718=CARTESIAN_POINT('Ctrl Pts',(4.19102157793607,15.2,-9.53513635620139));
#163719=CARTESIAN_POINT('Ctrl Pts',(4.19173861663712,15.2,-9.53753915048277));
#163720=CARTESIAN_POINT('Ctrl Pts',(4.19246316094381,15.2,-9.53999366064137));
#163721=CARTESIAN_POINT('Ctrl Pts',(4.19318770531631,15.2,-9.5424481710229));
#163722=CARTESIAN_POINT('Ctrl Pts',(4.19391975478974,15.2,-9.54495440107748));
#163723=CARTESIAN_POINT('Ctrl Pts',(4.19465855233046,15.2,-9.54751174347036));
#163724=CARTESIAN_POINT('Ctrl Pts',(4.19539734980408,15.2,-9.55006908563093));
#163725=CARTESIAN_POINT('Ctrl Pts',(4.19614289520964,15.2,-9.55267754135616));
#163726=CARTESIAN_POINT('Ctrl Pts',(4.19689445276592,15.2,-9.55533651859505));
#163727=CARTESIAN_POINT('Ctrl Pts',(4.19777126996042,15.2,-9.55843865886813));
#163728=CARTESIAN_POINT('Ctrl Pts',(4.19865626969675,15.2,-9.5616095630426));
#163729=CARTESIAN_POINT('Ctrl Pts',(4.19954831684995,15.2,-9.56484831852753));
#163730=CARTESIAN_POINT('Ctrl Pts',(4.20031292865584,15.2,-9.56762439451339));
#163731=CARTESIAN_POINT('Ctrl Pts',(4.20108272045344,15.2,-9.57045031632587));
#163732=CARTESIAN_POINT('Ctrl Pts',(4.20185699825882,15.2,-9.57332552089018));
#163733=CARTESIAN_POINT('Ctrl Pts',(4.20263127606421,15.2,-9.57620072545449));
#163734=CARTESIAN_POINT('Ctrl Pts',(4.20341003927757,15.2,-9.5791252158066));
#163735=CARTESIAN_POINT('Ctrl Pts',(4.20419261516564,15.2,-9.58209843411309));
#163736=CARTESIAN_POINT('Ctrl Pts',(4.2049751910537,15.2,-9.58507165241958));
#163737=CARTESIAN_POINT('Ctrl Pts',(4.20576157753445,15.2,-9.58809360112182));
#163738=CARTESIAN_POINT('Ctrl Pts',(4.20655112042221,15.2,-9.59116373742363));
#163739=CARTESIAN_POINT('Ctrl Pts',(4.20734066338169,15.2,-9.59423387400432));
#163740=CARTESIAN_POINT('Ctrl Pts',(4.20813336138319,15.2,-9.59735219688979));
#163741=CARTESIAN_POINT('Ctrl Pts',(4.20892857459329,15.2,-9.60051817748102));
#163742=CARTESIAN_POINT('Ctrl Pts',(4.20972378773116,15.2,-9.60368415778465));
#163743=CARTESIAN_POINT('Ctrl Pts',(4.21052151772717,15.2,-9.60689779296794));
#163744=CARTESIAN_POINT('Ctrl Pts',(4.21132113894804,15.2,-9.61015856159742));
#163745=CARTESIAN_POINT('Ctrl Pts',(4.21212076016891,15.2,-9.61341933022692));
#163746=CARTESIAN_POINT('Ctrl Pts',(4.21292227550836,15.2,-9.61672723460936));
#163747=CARTESIAN_POINT('Ctrl Pts',(4.21372507564577,15.2,-9.62008176015097));
#163748=CARTESIAN_POINT('Ctrl Pts',(4.2145278758561,15.2,-9.62343628599729));
#163749=CARTESIAN_POINT('Ctrl Pts',(4.21533196074159,15.2,-9.62683743398984));
#163750=CARTESIAN_POINT('Ctrl Pts',(4.21613674003548,15.2,-9.63028470092968));
#163751=CARTESIAN_POINT('Ctrl Pts',(4.21694151925626,15.2,-9.63373196755639));
#163752=CARTESIAN_POINT('Ctrl Pts',(4.21774698998353,15.2,-9.63722535336929));
#163753=CARTESIAN_POINT('Ctrl Pts',(4.21855257820791,15.2,-9.64076436500666));
#163754=CARTESIAN_POINT('Ctrl Pts',(4.21935816643229,15.2,-9.64430337664403));
#163755=CARTESIAN_POINT('Ctrl Pts',(4.22016387039973,15.2,-9.64788801198091));
#163756=CARTESIAN_POINT('Ctrl Pts',(4.22096912595384,15.2,-9.65151778759597));
#163757=CARTESIAN_POINT('Ctrl Pts',(4.2217743815811,15.2,-9.65514756354075));
#163758=CARTESIAN_POINT('Ctrl Pts',(4.22257919099379,15.2,-9.65882247991873));
#163759=CARTESIAN_POINT('Ctrl Pts',(4.2233830025777,15.2,-9.6625420591432));
#163760=CARTESIAN_POINT('Ctrl Pts',(4.2241868140886,15.2,-9.6662616380298));
#163761=CARTESIAN_POINT('Ctrl Pts',(4.2249896277874,15.2,-9.67002588040497));
#163762=CARTESIAN_POINT('Ctrl Pts',(4.22579090900828,15.2,-9.67383431326659));
#163763=CARTESIAN_POINT('Ctrl Pts',(4.22659219022916,15.2,-9.67764274612822));
#163764=CARTESIAN_POINT('Ctrl Pts',(4.22739193620345,15.2,-9.68149537398921));
#163765=CARTESIAN_POINT('Ctrl Pts',(4.22818962396444,15.2,-9.68539173287312));
#163766=CARTESIAN_POINT('Ctrl Pts',(4.22885436378942,15.2,-9.68863869872768));
#163767=CARTESIAN_POINT('Ctrl Pts',(4.22951767568436,15.2,-9.69191603336874));
#163768=CARTESIAN_POINT('Ctrl Pts',(4.23017926124,15.2,-9.69522347482548));
#163769=CARTESIAN_POINT('Ctrl Pts',(4.23084084679565,15.2,-9.69853091628222));
#163770=CARTESIAN_POINT('Ctrl Pts',(4.23150070681236,15.2,-9.70186846210921));
#163771=CARTESIAN_POINT('Ctrl Pts',(4.23215854917358,15.2,-9.70523585453823));
#163772=CARTESIAN_POINT('Ctrl Pts',(4.2328163915348,15.2,-9.70860324696723));
#163773=CARTESIAN_POINT('Ctrl Pts',(4.23347221802439,15.2,-9.71200048482705));
#163774=CARTESIAN_POINT('Ctrl Pts',(4.23412574254126,15.2,-9.71542731227307));
#163775=CARTESIAN_POINT('Ctrl Pts',(4.23477926705812,15.2,-9.7188541397191));
#163776=CARTESIAN_POINT('Ctrl Pts',(4.2354304877444,15.2,-9.72231055681104));
#163777=CARTESIAN_POINT('Ctrl Pts',(4.23607912600828,15.2,-9.7257963092416));
#163778=CARTESIAN_POINT('Ctrl Pts',(4.23672776427217,15.2,-9.72928206167215));
#163779=CARTESIAN_POINT('Ctrl Pts',(4.23737382161406,15.2,-9.73279715005236));
#163780=CARTESIAN_POINT('Ctrl Pts',(4.2380170199503,15.2,-9.73634132423521));
#163781=CARTESIAN_POINT('Ctrl Pts',(4.23866021828655,15.2,-9.73988549841805));
#163782=CARTESIAN_POINT('Ctrl Pts',(4.23930056071399,15.2,-9.74345875747307));
#163783=CARTESIAN_POINT('Ctrl Pts',(4.23993777474161,15.2,-9.74706085504403));
#163784=CARTESIAN_POINT('Ctrl Pts',(4.24057498876922,15.2,-9.75066295261499));
#163785=CARTESIAN_POINT('Ctrl Pts',(4.24120907609136,15.2,-9.75429388866574));
#163786=CARTESIAN_POINT('Ctrl Pts',(4.24183977109118,15.2,-9.75795341797278));
#163787=CARTESIAN_POINT('Ctrl Pts',(4.242470466091,15.2,-9.76161294727982));
#163788=CARTESIAN_POINT('Ctrl Pts',(4.24309776897477,15.2,-9.76530107119382));
#163789=CARTESIAN_POINT('Ctrl Pts',(4.243721419839,15.2,-9.7690175472148));
#163790=CARTESIAN_POINT('Ctrl Pts',(4.24434507070324,15.2,-9.77273402323579));
#163791=CARTESIAN_POINT('Ctrl Pts',(4.24496506893086,15.2,-9.77647885074671));
#163792=CARTESIAN_POINT('Ctrl Pts',(4.2455811605972,15.2,-9.78025179248512));
#163793=CARTESIAN_POINT('Ctrl Pts',(4.24619725226355,15.2,-9.78402473422354));
#163794=CARTESIAN_POINT('Ctrl Pts',(4.2468094360076,15.2,-9.78782579053184));
#163795=CARTESIAN_POINT('Ctrl Pts',(4.24741746260448,15.2,-9.79165472324244));
#163796=CARTESIAN_POINT('Ctrl Pts',(4.24802548913509,15.2,-9.7954836555357));
#163797=CARTESIAN_POINT('Ctrl Pts',(4.24862935804764,15.2,-9.79934046482307));
#163798=CARTESIAN_POINT('Ctrl Pts',(4.24922882145488,15.2,-9.80322491946687));
#163799=CARTESIAN_POINT('Ctrl Pts',(4.24982828492747,15.2,-9.80710937453407));
#163800=CARTESIAN_POINT('Ctrl Pts',(4.25042334491679,15.2,-9.81102147275356));
#163801=CARTESIAN_POINT('Ctrl Pts',(4.25101375838939,15.2,-9.81496098525133));
#163802=CARTESIAN_POINT('Ctrl Pts',(4.25160417186199,15.2,-9.8189004977491));
#163803=CARTESIAN_POINT('Ctrl Pts',(4.25218994001802,15.2,-9.82286742232974));
#163804=CARTESIAN_POINT('Ctrl Pts',(4.25277082349064,15.2,-9.82686153316086));
#163805=CARTESIAN_POINT('Ctrl Pts',(4.25335170696326,15.2,-9.83085564399197));
#163806=CARTESIAN_POINT('Ctrl Pts',(4.25392770711035,15.2,-9.83487693929639));
#163807=CARTESIAN_POINT('Ctrl Pts',(4.25449858970867,15.2,-9.83892519303844));
#163808=CARTESIAN_POINT('Ctrl Pts',(4.25506947230699,15.2,-9.84297344678047));
#163809=CARTESIAN_POINT('Ctrl Pts',(4.25563523802966,15.2,-9.84704866018881));
#163810=CARTESIAN_POINT('Ctrl Pts',(4.25619565719661,15.2,-9.85115060796518));
#163811=CARTESIAN_POINT('Ctrl Pts',(4.25675607636355,15.2,-9.85525255574156));
#163812=CARTESIAN_POINT('Ctrl Pts',(4.25731114735814,15.2,-9.85938124031862));
#163813=CARTESIAN_POINT('Ctrl Pts',(4.25786064749732,15.2,-9.86353643726169));
#163814=CARTESIAN_POINT('Ctrl Pts',(4.25830024763262,15.2,-9.86686059499732));
#163815=CARTESIAN_POINT('Ctrl Pts',(4.25873628036784,15.2,-9.87020172116841));
#163816=CARTESIAN_POINT('Ctrl Pts',(4.25916863507934,15.2,-9.87355970552063));
#163817=CARTESIAN_POINT('Ctrl Pts',(4.25960098973194,15.2,-9.87691768941533));
#163818=CARTESIAN_POINT('Ctrl Pts',(4.2600296626219,15.2,-9.88029252749288));
#163819=CARTESIAN_POINT('Ctrl Pts',(4.26045454469852,15.2,-9.88368411271452));
#163820=CARTESIAN_POINT('Ctrl Pts',(4.26098564733772,15.2,-9.88792359458814));
#163821=CARTESIAN_POINT('Ctrl Pts',(4.26151082459899,15.2,-9.89218924004301));
#163822=CARTESIAN_POINT('Ctrl Pts',(4.26202986147431,15.2,-9.89648083448611));
#163823=CARTESIAN_POINT('Ctrl Pts',(4.2624450909972,15.2,-9.89991411022769));
#163824=CARTESIAN_POINT('Ctrl Pts',(4.26285639023073,15.2,-9.90336399288395));
#163825=CARTESIAN_POINT('Ctrl Pts',(4.2632636505507,15.2,-9.9068303734697));
#163826=CARTESIAN_POINT('Ctrl Pts',(4.26367091081518,15.2,-9.91029675358314));
#163827=CARTESIAN_POINT('Ctrl Pts',(4.26407413275798,15.2,-9.91377963161227));
#163828=CARTESIAN_POINT('Ctrl Pts',(4.26447320822563,15.2,-9.91727889821404));
#163829=CARTESIAN_POINT('Ctrl Pts',(4.26487228374766,15.2,-9.92077816529258));
#163830=CARTESIAN_POINT('Ctrl Pts',(4.26526721277474,15.2,-9.92429382163696));
#163831=CARTESIAN_POINT('Ctrl Pts',(4.26565788974019,15.2,-9.9278257593305));
#163832=CARTESIAN_POINT('Ctrl Pts',(4.2661462359204,15.2,-9.93224068120682));
#163833=CARTESIAN_POINT('Ctrl Pts',(4.26662793875959,15.2,-9.93668104239357));
#163834=CARTESIAN_POINT('Ctrl Pts',(4.26710279329673,15.2,-9.94114663449343));
#163835=CARTESIAN_POINT('Ctrl Pts',(4.26748267689538,15.2,-9.94471910788126));
#163836=CARTESIAN_POINT('Ctrl Pts',(4.2678581782774,15.2,-9.94830772843448));
#163837=CARTESIAN_POINT('Ctrl Pts',(4.26822919446959,15.2,-9.95191239047209));
#163838=CARTESIAN_POINT('Ctrl Pts',(4.26860021071233,15.2,-9.95551705300083));
#163839=CARTESIAN_POINT('Ctrl Pts',(4.26896674151286,15.2,-9.95913775705649));
#163840=CARTESIAN_POINT('Ctrl Pts',(4.26932868525451,15.2,-9.96277439808907));
#163841=CARTESIAN_POINT('Ctrl Pts',(4.26969062894684,15.2,-9.96641103862614));
#163842=CARTESIAN_POINT('Ctrl Pts',(4.27004798658734,15.2,-9.97006361401073));
#163843=CARTESIAN_POINT('Ctrl Pts',(4.27040065746543,15.2,-9.97373202272606));
#163844=CARTESIAN_POINT('Ctrl Pts',(4.27075332839156,15.2,-9.97740043194123));
#163845=CARTESIAN_POINT('Ctrl Pts',(4.27110131182625,15.2,-9.98108467233046));
#163846=CARTESIAN_POINT('Ctrl Pts',(4.27144450951131,15.2,-9.9847846408109));
#163847=CARTESIAN_POINT('Ctrl Pts',(4.2717877071496,15.2,-9.98848460878723));
#163848=CARTESIAN_POINT('Ctrl Pts',(4.27212611943331,15.2,-9.99220030546318));
#163849=CARTESIAN_POINT('Ctrl Pts',(4.2724596489621,15.2,-9.99593162615656));
#163850=CARTESIAN_POINT('Ctrl Pts',(4.27279317853633,15.2,-9.99966294735833));
#163851=CARTESIAN_POINT('Ctrl Pts',(4.27312182289776,15.2,-10.0034098950303));
#163852=CARTESIAN_POINT('Ctrl Pts',(4.27344548925018,15.2,-10.0071723642525));
#163853=CARTESIAN_POINT('Ctrl Pts',(4.27376915555851,15.2,-10.0109348329621));
#163854=CARTESIAN_POINT('Ctrl Pts',(4.27408784272103,15.2,-10.0147128232303));
#163855=CARTESIAN_POINT('Ctrl Pts',(4.27440145497369,15.2,-10.0185062363631));
#163856=CARTESIAN_POINT('Ctrl Pts',(4.27471506726908,15.2,-10.0222996500127));
#163857=CARTESIAN_POINT('Ctrl Pts',(4.27502360420288,15.2,-10.0261084841582));
#163858=CARTESIAN_POINT('Ctrl Pts',(4.27532697327497,15.2,-10.0299326380333));
#163859=CARTESIAN_POINT('Ctrl Pts',(4.27563034234705,15.2,-10.0337567919083));
#163860=CARTESIAN_POINT('Ctrl Pts',(4.27592854350188,15.2,-10.037596266688));
#163861=CARTESIAN_POINT('Ctrl Pts',(4.27622148257286,15.2,-10.0414509606219));
#163862=CARTESIAN_POINT('Ctrl Pts',(4.27651442160393,15.2,-10.0453056540305));
#163863=CARTESIAN_POINT('Ctrl Pts',(4.27680210014377,15.2,-10.0491755678084));
#163864=CARTESIAN_POINT('Ctrl Pts',(4.27708442523311,15.2,-10.0530606017306));
#163865=CARTESIAN_POINT('Ctrl Pts',(4.27743733162362,15.2,-10.0579168945304));
#163866=CARTESIAN_POINT('Ctrl Pts',(4.27778187476663,15.2,-10.0627968116444));
#163867=CARTESIAN_POINT('Ctrl Pts',(4.27811787851663,15.2,-10.0677001619916));
#163868=CARTESIAN_POINT('Ctrl Pts',(4.27838668153128,15.2,-10.0716228424832));
#163869=CARTESIAN_POINT('Ctrl Pts',(4.27865001806196,15.2,-10.0755605186237));
#163870=CARTESIAN_POINT('Ctrl Pts',(4.27890780107544,15.2,-10.0795130943962));
#163871=CARTESIAN_POINT('Ctrl Pts',(4.2791655840538,15.2,-10.0834656696302));
#163872=CARTESIAN_POINT('Ctrl Pts',(4.27941781185492,15.2,-10.0874331430909));
#163873=CARTESIAN_POINT('Ctrl Pts',(4.2796643982248,15.2,-10.0914154171722));
#163874=CARTESIAN_POINT('Ctrl Pts',(4.27991098462826,15.2,-10.0953976917962));
#163875=CARTESIAN_POINT('Ctrl Pts',(4.2801519285123,15.2,-10.0993947667774));
#163876=CARTESIAN_POINT('Ctrl Pts',(4.28038714358009,15.2,-10.1034065471642));
#163877=CARTESIAN_POINT('Ctrl Pts',(4.28062235861583,15.2,-10.1074183270044));
#163878=CARTESIAN_POINT('Ctrl Pts',(4.28085184387175,15.2,-10.1114448109872));
#163879=CARTESIAN_POINT('Ctrl Pts',(4.28107551496496,15.2,-10.1154859017114));
#163880=CARTESIAN_POINT('Ctrl Pts',(4.28135510385433,15.2,-10.1205372655297));
#163881=CARTESIAN_POINT('Ctrl Pts',(4.28162560769345,15.2,-10.1256114531291));
#163882=CARTESIAN_POINT('Ctrl Pts',(4.28188686074949,15.2,-10.1307082801418));
#163883=CARTESIAN_POINT('Ctrl Pts',(4.28209586320572,15.2,-10.1347857419742));
#163884=CARTESIAN_POINT('Ctrl Pts',(4.28229894513625,15.2,-10.1388776920824));
#163885=CARTESIAN_POINT('Ctrl Pts',(4.2824960230452,15.2,-10.1429840348459));
#163886=CARTESIAN_POINT('Ctrl Pts',(4.2826931009273,15.2,-10.1470903770499));
#163887=CARTESIAN_POINT('Ctrl Pts',(4.28288417654118,15.2,-10.1512111126121));
#163888=CARTESIAN_POINT('Ctrl Pts',(4.28306916502645,15.2,-10.1553461461621));
#163889=CARTESIAN_POINT('Ctrl Pts',(4.28330040065195,15.2,-10.160514938522));
#163890=CARTESIAN_POINT('Ctrl Pts',(4.28352212755776,15.2,-10.1657060734881));
#163891=CARTESIAN_POINT('Ctrl Pts',(4.28373418575271,15.2,-10.1709193671675));
#163892=CARTESIAN_POINT('Ctrl Pts',(4.28394624394766,15.2,-10.1761326608469));
#163893=CARTESIAN_POINT('Ctrl Pts',(4.28414863489341,15.2,-10.1813681131122));
#163894=CARTESIAN_POINT('Ctrl Pts',(4.2843412012832,15.2,-10.1866255419554));
#163895=CARTESIAN_POINT('Ctrl Pts',(4.28449525440343,15.2,-10.1908314852593));
#163896=CARTESIAN_POINT('Ctrl Pts',(4.2846430205827,15.2,-10.1950514940156));
#163897=CARTESIAN_POINT('Ctrl Pts',(4.28478441925642,15.2,-10.1992854746922));
#163898=CARTESIAN_POINT('Ctrl Pts',(4.28492581791087,15.2,-10.203519454792));
#163899=CARTESIAN_POINT('Ctrl Pts',(4.28506085104115,15.2,-10.2077674088704));
#163900=CARTESIAN_POINT('Ctrl Pts',(4.28518944019773,15.2,-10.21202924291));
#163901=CARTESIAN_POINT('Ctrl Pts',(4.28535017665659,15.2,-10.217356535895));
#163902=CARTESIAN_POINT('Ctrl Pts',(4.28550084362145,15.2,-10.2227055169449));
#163903=CARTESIAN_POINT('Ctrl Pts',(4.28564129098323,15.2,-10.2280760082887));
#163904=CARTESIAN_POINT('Ctrl Pts',(4.28578173834501,15.2,-10.2334464996325));
#163905=CARTESIAN_POINT('Ctrl Pts',(4.28591196730553,15.2,-10.2388385011222));
#163906=CARTESIAN_POINT('Ctrl Pts',(4.28603182799997,15.2,-10.244251835775));
#163907=CARTESIAN_POINT('Ctrl Pts',(4.28612771656075,15.2,-10.2485825037332));
#163908=CARTESIAN_POINT('Ctrl Pts',(4.28621697050132,15.2,-10.2529268240903));
#163909=CARTESIAN_POINT('Ctrl Pts',(4.28629951500513,15.2,-10.2572847079958));
#163910=CARTESIAN_POINT('Ctrl Pts',(4.28638205949769,15.2,-10.2616425913076));
#163911=CARTESIAN_POINT('Ctrl Pts',(4.2864578928469,15.2,-10.2660140385161));
#163912=CARTESIAN_POINT('Ctrl Pts',(4.28652694400826,15.2,-10.2703989567886));
#163913=CARTESIAN_POINT('Ctrl Pts',(4.28659599517902,15.2,-10.2747838756586));
#163914=CARTESIAN_POINT('Ctrl Pts',(4.28665826263726,15.2,-10.2791822695684));
#163915=CARTESIAN_POINT('Ctrl Pts',(4.28671367325069,15.2,-10.2835940462546));
#163916=CARTESIAN_POINT('Ctrl Pts',(4.28676908385657,15.2,-10.2880058223398));
#163917=CARTESIAN_POINT('Ctrl Pts',(4.28681763838279,15.2,-10.2924309828926));
#163918=CARTESIAN_POINT('Ctrl Pts',(4.28685926371317,15.2,-10.2968694383622));
#163919=CARTESIAN_POINT('Ctrl Pts',(4.28689048271238,15.2,-10.3001982801156));
#163920=CARTESIAN_POINT('Ctrl Pts',(4.28691780502797,15.2,-10.3035346010917));
#163921=CARTESIAN_POINT('Ctrl Pts',(4.28694119948707,15.2,-10.3068783630531));
#163922=CARTESIAN_POINT('Ctrl Pts',(4.28698019025367,15.2,-10.3124512998579));
#163923=CARTESIAN_POINT('Ctrl Pts',(4.2870082723871,15.2,-10.3180449066895));
#163924=CARTESIAN_POINT('Ctrl Pts',(4.28702530579046,15.2,-10.3236590136329));
#163925=CARTESIAN_POINT('Ctrl Pts',(4.2870355258321,15.2,-10.3270274776766));
#163926=CARTESIAN_POINT('Ctrl Pts',(4.28704176924902,15.2,-10.3304033206697));
#163927=CARTESIAN_POINT('Ctrl Pts',(4.28704400624948,15.2,-10.3337865067958));
#163928=CARTESIAN_POINT('Ctrl Pts',(4.28704624325035,15.2,-10.3371696935365));
#163929=CARTESIAN_POINT('Ctrl Pts',(4.28704447371677,15.2,-10.3405602221626));
#163930=CARTESIAN_POINT('Ctrl Pts',(4.28703866871537,15.2,-10.3439580574907));
#163931=CARTESIAN_POINT('Ctrl Pts',(4.28702899371551,15.2,-10.3496211149306));
#163932=CARTESIAN_POINT('Ctrl Pts',(4.28700810861641,15.2,-10.3553044681051));
#163933=CARTESIAN_POINT('Ctrl Pts',(4.28697588028752,15.2,-10.3610079455373));
#163934=CARTESIAN_POINT('Ctrl Pts',(4.28695654328526,15.2,-10.364430032867));
#163935=CARTESIAN_POINT('Ctrl Pts',(4.28693312344853,15.2,-10.367859365132));
#163936=CARTESIAN_POINT('Ctrl Pts',(4.28690559094397,15.2,-10.3712959064658));
#163937=CARTESIAN_POINT('Ctrl Pts',(4.28686888094622,15.2,-10.375877960537));
#163938=CARTESIAN_POINT('Ctrl Pts',(4.28682486059943,15.2,-10.3804728301037));
#163939=CARTESIAN_POINT('Ctrl Pts',(4.28677346327077,15.2,-10.3850804301151));
#163940=CARTESIAN_POINT('Ctrl Pts',(4.28673491527254,15.2,-10.3885361302806));
#163941=CARTESIAN_POINT('Ctrl Pts',(4.28669221775916,15.2,-10.3919989906822));
#163942=CARTESIAN_POINT('Ctrl Pts',(4.286645342759,15.2,-10.3954689756037));
#163943=CARTESIAN_POINT('Ctrl Pts',(4.28659846775884,15.2,-10.3989389605252));
#163944=CARTESIAN_POINT('Ctrl Pts',(4.28654741575944,15.2,-10.4024160704847));
#163945=CARTESIAN_POINT('Ctrl Pts',(4.28649215780368,15.2,-10.4059002687321));
#163946=CARTESIAN_POINT('Ctrl Pts',(4.28643689983789,15.2,-10.4093844676125));
#163947=CARTESIAN_POINT('Ctrl Pts',(4.28637743751258,15.2,-10.4128757554532));
#163948=CARTESIAN_POINT('Ctrl Pts',(4.28631374204442,15.2,-10.4163740962543));
#163949=CARTESIAN_POINT('Ctrl Pts',(4.28622881477281,15.2,-10.4210385495965));
#163950=CARTESIAN_POINT('Ctrl Pts',(4.28613636328274,15.2,-10.425715540337));
#163951=CARTESIAN_POINT('Ctrl Pts',(4.28603632329141,15.2,-10.4304049863417));
#163952=CARTESIAN_POINT('Ctrl Pts',(4.28596129329451,15.2,-10.433922071005));
#163953=CARTESIAN_POINT('Ctrl Pts',(4.28588199471675,15.2,-10.4374461601862));
#163954=CARTESIAN_POINT('Ctrl Pts',(4.28579839979944,15.2,-10.4409772200669));
#163955=CARTESIAN_POINT('Ctrl Pts',(4.28571480488213,15.2,-10.4445082799475));
#163956=CARTESIAN_POINT('Ctrl Pts',(4.28562691529946,15.2,-10.4480463097569));
#163957=CARTESIAN_POINT('Ctrl Pts',(4.28553470330341,15.2,-10.4515912744188));
#163958=CARTESIAN_POINT('Ctrl Pts',(4.2854424912906,15.2,-10.4551362397248));
#163959=CARTESIAN_POINT('Ctrl Pts',(4.2853459560099,15.2,-10.4586881395576));
#163960=CARTESIAN_POINT('Ctrl Pts',(4.28524507345298,15.2,-10.4622469393258));
#163961=CARTESIAN_POINT('Ctrl Pts',(4.28511056340763,15.2,-10.4669920046058));
#163962=CARTESIAN_POINT('Ctrl Pts',(4.28496832204939,15.2,-10.471749334287));
#163963=CARTESIAN_POINT('Ctrl Pts',(4.28481828806217,15.2,-10.4765188476185));
#163964=CARTESIAN_POINT('Ctrl Pts',(4.28470576256664,15.2,-10.4800959827796));
#163965=CARTESIAN_POINT('Ctrl Pts',(4.28458885348807,15.2,-10.4836799697819));
#163966=CARTESIAN_POINT('Ctrl Pts',(4.28446753503475,15.2,-10.4872707754838));
#163967=CARTESIAN_POINT('Ctrl Pts',(4.28434621655939,15.2,-10.4908615818381));
#163968=CARTESIAN_POINT('Ctrl Pts',(4.28422048879112,15.2,-10.4944592061443));
#163969=CARTESIAN_POINT('Ctrl Pts',(4.28409032672993,15.2,-10.4980636135024));
#163970=CARTESIAN_POINT('Ctrl Pts',(4.28391677735442,15.2,-10.5028694888885));
#163971=CARTESIAN_POINT('Ctrl Pts',(4.28373534249934,15.2,-10.5076874235641));
#163972=CARTESIAN_POINT('Ctrl Pts',(4.28354596445844,15.2,-10.5125173337467));
#163973=CARTESIAN_POINT('Ctrl Pts',(4.28340393092131,15.2,-10.5161397665481));
#163974=CARTESIAN_POINT('Ctrl Pts',(4.28325742756048,15.2,-10.5197689361698));
#163975=CARTESIAN_POINT('Ctrl Pts',(4.28310643102469,15.2,-10.5234048088288));
#163976=CARTESIAN_POINT('Ctrl Pts',(4.2829554344889,15.2,-10.5270406814878));
#163977=CARTESIAN_POINT('Ctrl Pts',(4.28279994379509,15.2,-10.5306832557379));
#163978=CARTESIAN_POINT('Ctrl Pts',(4.28263993480152,15.2,-10.5343324984795));
#163979=CARTESIAN_POINT('Ctrl Pts',(4.28247992577888,15.2,-10.5379817418839));
#163980=CARTESIAN_POINT('Ctrl Pts',(4.28231539742164,15.2,-10.5416376543152));
#163981=CARTESIAN_POINT('Ctrl Pts',(4.28214632593811,15.2,-10.5453001993067));
#163982=CARTESIAN_POINT('Ctrl Pts',(4.2819772544853,15.2,-10.5489627436329));
#163983=CARTESIAN_POINT('Ctrl Pts',(4.28180363946841,15.2,-10.5526319223104));
#163984=CARTESIAN_POINT('Ctrl Pts',(4.28162545692379,15.2,-10.5563077006945));
#163985=CARTESIAN_POINT('Ctrl Pts',(4.28144727437917,15.2,-10.5599834790787));
#163986=CARTESIAN_POINT('Ctrl Pts',(4.28126452298974,15.2,-10.563665855719));
#163987=CARTESIAN_POINT('Ctrl Pts',(4.28107717949615,15.2,-10.5673547988772));
#163988=CARTESIAN_POINT('Ctrl Pts',(4.28088983600255,15.2,-10.5710437420354));
#163989=CARTESIAN_POINT('Ctrl Pts',(4.28069789969284,15.2,-10.5747392503178));
#163990=CARTESIAN_POINT('Ctrl Pts',(4.28050134774165,15.2,-10.5784412905166));
#163991=CARTESIAN_POINT('Ctrl Pts',(4.28030479579045,15.2,-10.5821433307155));
#163992=CARTESIAN_POINT('Ctrl Pts',(4.28010362771445,15.2,-10.5858519026807));
#163993=CARTESIAN_POINT('Ctrl Pts',(4.279897819764,15.2,-10.5895669733785));
#163994=CARTESIAN_POINT('Ctrl Pts',(4.27969201181354,15.2,-10.5932820440763));
#163995=CARTESIAN_POINT('Ctrl Pts',(4.27948156432727,15.2,-10.597003612912));
#163996=CARTESIAN_POINT('Ctrl Pts',(4.27926645232488,15.2,-10.6007316452954));
#163997=CARTESIAN_POINT('Ctrl Pts',(4.27905134032249,15.2,-10.6044596776788));
#163998=CARTESIAN_POINT('Ctrl Pts',(4.27883156239011,15.2,-10.6081941721879));
#163999=CARTESIAN_POINT('Ctrl Pts',(4.27860709702391,15.2,-10.6119350969261));
#164000=CARTESIAN_POINT('Ctrl Pts',(4.27838263161692,15.2,-10.6156760223439));
#164001=CARTESIAN_POINT('Ctrl Pts',(4.27815347886695,15.2,-10.6194233771719));
#164002=CARTESIAN_POINT('Ctrl Pts',(4.27791961741566,15.2,-10.6231771325516));
#164003=CARTESIAN_POINT('Ctrl Pts',(4.27768575600685,15.2,-10.6269308872494));
#164004=CARTESIAN_POINT('Ctrl Pts',(4.27744718648162,15.2,-10.6306910412469));
#164005=CARTESIAN_POINT('Ctrl Pts',(4.27720388399004,15.2,-10.6344575614023));
#164006=CARTESIAN_POINT('Ctrl Pts',(4.27696058149847,15.2,-10.6382240815577));
#164007=CARTESIAN_POINT('Ctrl Pts',(4.27671254567506,15.2,-10.6419969671902));
#164008=CARTESIAN_POINT('Ctrl Pts',(4.27645974872475,15.2,-10.6457761754451));
#164009=CARTESIAN_POINT('Ctrl Pts',(4.27620695177443,15.2,-10.6495553837));
#164010=CARTESIAN_POINT('Ctrl Pts',(4.27594939290852,15.2,-10.6533409152338));
#164011=CARTESIAN_POINT('Ctrl Pts',(4.27568705125021,15.2,-10.6571327392382));
#164012=CARTESIAN_POINT('Ctrl Pts',(4.27524981513715,15.2,-10.6634524461419));
#164013=CARTESIAN_POINT('Ctrl Pts',(4.27479930143439,15.2,-10.6697896272814));
#164014=CARTESIAN_POINT('Ctrl Pts',(4.27433546799994,15.2,-10.676144262));
#164015=CARTESIAN_POINT('Origin',(-5.66257110645729E-14,15.2,-1.77635683940025E-14));
#164016=CARTESIAN_POINT('',(4.57383771044509,15.2,-9.312391400561));
#164017=CARTESIAN_POINT('',(4.57383771044509,12.2,-9.31239140056099));
#164018=CARTESIAN_POINT('',(4.57383770999994,15.2,-9.31239140000002));
#164019=CARTESIAN_POINT('Origin',(-5.66257110645729E-14,12.2,-1.77635683940025E-14));
#164020=CARTESIAN_POINT('Origin',(-5.66257110645729E-14,15.2,-1.77635683940025E-14));
#164021=CARTESIAN_POINT('Origin',(-5.66257110645729E-14,15.2,-1.77635683940025E-14));
#164022=CARTESIAN_POINT('',(5.41482055299994,15.2,-10.145428447));
#164023=CARTESIAN_POINT('',(5.75020264099994,15.2,-9.95917514500001));
#164024=CARTESIAN_POINT('Origin',(-5.66257110645729E-14,15.2,-1.77635683940025E-14));
#164025=CARTESIAN_POINT('',(5.75020264099994,12.2,-9.95917514500001));
#164026=CARTESIAN_POINT('',(5.75020264099994,15.2,-9.95917514500001));
#164027=CARTESIAN_POINT('',(5.41482055299994,12.2,-10.145428447));
#164028=CARTESIAN_POINT('Origin',(-5.66257110645729E-14,12.2,-1.77635683940025E-14));
#164029=CARTESIAN_POINT('',(5.41482055299994,15.2,-10.145428447));
#164030=CARTESIAN_POINT('Ctrl Pts',(5.75020264099994,15.2,-9.95917514500001));
#164031=CARTESIAN_POINT('Ctrl Pts',(5.75020264099994,11.6,-9.95917514500001));
#164032=CARTESIAN_POINT('Ctrl Pts',(5.75014921099994,15.2,-9.95841243000001));
#164033=CARTESIAN_POINT('Ctrl Pts',(5.75014921099994,11.6,-9.95841243000001));
#164034=CARTESIAN_POINT('Ctrl Pts',(5.75004209299995,15.2,-9.95688746000001));
#164035=CARTESIAN_POINT('Ctrl Pts',(5.75004209299995,11.6,-9.95688746000001));
#164036=CARTESIAN_POINT('Ctrl Pts',(5.74988064799995,15.2,-9.95460138400001));
#164037=CARTESIAN_POINT('Ctrl Pts',(5.74988064799995,11.6,-9.95460138400001));
#164038=CARTESIAN_POINT('Ctrl Pts',(5.74966384999994,15.2,-9.95155604500001));
#164039=CARTESIAN_POINT('Ctrl Pts',(5.74966384999994,11.6,-9.95155604500001));
#164040=CARTESIAN_POINT('Ctrl Pts',(5.74939028899994,15.2,-9.94775397100001));
#164041=CARTESIAN_POINT('Ctrl Pts',(5.74939028899994,11.6,-9.94775397100001));
#164042=CARTESIAN_POINT('Ctrl Pts',(5.74911416699995,15.2,-9.94395649900001));
#164043=CARTESIAN_POINT('Ctrl Pts',(5.74911416699995,11.6,-9.94395649900001));
#164044=CARTESIAN_POINT('Ctrl Pts',(5.74883548399994,15.2,-9.94016363100001));
#164045=CARTESIAN_POINT('Ctrl Pts',(5.74883548399994,11.6,-9.94016363100001));
#164046=CARTESIAN_POINT('Ctrl Pts',(5.74855424299994,15.2,-9.93637537100001));
#164047=CARTESIAN_POINT('Ctrl Pts',(5.74855424299994,11.6,-9.93637537100001));
#164048=CARTESIAN_POINT('Ctrl Pts',(5.74827044899994,15.2,-9.93259172100001));
#164049=CARTESIAN_POINT('Ctrl Pts',(5.74827044899994,11.6,-9.93259172100001));
#164050=CARTESIAN_POINT('Ctrl Pts',(5.74798410499994,15.2,-9.92881269000001));
#164051=CARTESIAN_POINT('Ctrl Pts',(5.74798410499994,11.6,-9.92881269000001));
#164052=CARTESIAN_POINT('Ctrl Pts',(5.74769521999994,15.2,-9.92503828300001));
#164053=CARTESIAN_POINT('Ctrl Pts',(5.74769521999994,11.6,-9.92503828300001));
#164054=CARTESIAN_POINT('Ctrl Pts',(5.74740379999994,15.2,-9.92126850900001));
#164055=CARTESIAN_POINT('Ctrl Pts',(5.74740379999994,11.6,-9.92126850900001));
#164056=CARTESIAN_POINT('Ctrl Pts',(5.74710985299995,15.2,-9.91750337600001));
#164057=CARTESIAN_POINT('Ctrl Pts',(5.74710985299995,11.6,-9.91750337600001));
#164058=CARTESIAN_POINT('Ctrl Pts',(5.74681338699994,15.2,-9.91374289100001));
#164059=CARTESIAN_POINT('Ctrl Pts',(5.74681338699994,11.6,-9.91374289100001));
#164060=CARTESIAN_POINT('Ctrl Pts',(5.74651440799995,15.2,-9.90998706400001));
#164061=CARTESIAN_POINT('Ctrl Pts',(5.74651440799995,11.6,-9.90998706400001));
#164062=CARTESIAN_POINT('Ctrl Pts',(5.74621292399994,15.2,-9.90623590000001));
#164063=CARTESIAN_POINT('Ctrl Pts',(5.74621292399994,11.6,-9.90623590000001));
#164064=CARTESIAN_POINT('Ctrl Pts',(5.74590893999994,15.2,-9.90248940500001));
#164065=CARTESIAN_POINT('Ctrl Pts',(5.74590893999994,11.6,-9.90248940500001));
#164066=CARTESIAN_POINT('Ctrl Pts',(5.74560246199994,15.2,-9.89874758700001));
#164067=CARTESIAN_POINT('Ctrl Pts',(5.74560246199994,11.6,-9.89874758700001));
#164068=CARTESIAN_POINT('Ctrl Pts',(5.74529349399994,15.2,-9.89501045000001));
#164069=CARTESIAN_POINT('Ctrl Pts',(5.74529349399994,11.6,-9.89501045000001));
#164070=CARTESIAN_POINT('Ctrl Pts',(5.74498204299994,15.2,-9.89127800100001));
#164071=CARTESIAN_POINT('Ctrl Pts',(5.74498204299994,11.6,-9.89127800100001));
#164072=CARTESIAN_POINT('Ctrl Pts',(5.74466811499994,15.2,-9.88755024700001));
#164073=CARTESIAN_POINT('Ctrl Pts',(5.74466811499994,11.6,-9.88755024700001));
#164074=CARTESIAN_POINT('Ctrl Pts',(5.74435171599994,15.2,-9.88382719300001));
#164075=CARTESIAN_POINT('Ctrl Pts',(5.74435171599994,11.6,-9.88382719300001));
#164076=CARTESIAN_POINT('Ctrl Pts',(5.74403285199995,15.2,-9.88010884600001));
#164077=CARTESIAN_POINT('Ctrl Pts',(5.74403285199995,11.6,-9.88010884600001));
#164078=CARTESIAN_POINT('Ctrl Pts',(5.74371152899994,15.2,-9.87639521400001));
#164079=CARTESIAN_POINT('Ctrl Pts',(5.74371152899994,11.6,-9.87639521400001));
#164080=CARTESIAN_POINT('Ctrl Pts',(5.74338775399994,15.2,-9.87268630200001));
#164081=CARTESIAN_POINT('Ctrl Pts',(5.74338775399994,11.6,-9.87268630200001));
#164082=CARTESIAN_POINT('Ctrl Pts',(5.74306153399994,15.2,-9.86898212000001));
#164083=CARTESIAN_POINT('Ctrl Pts',(5.74306153399994,11.6,-9.86898212000001));
#164084=CARTESIAN_POINT('Ctrl Pts',(5.74273287599994,15.2,-9.86528267200001));
#164085=CARTESIAN_POINT('Ctrl Pts',(5.74273287599994,11.6,-9.86528267200001));
#164086=CARTESIAN_POINT('Ctrl Pts',(5.74240178399994,15.2,-9.86158796700001));
#164087=CARTESIAN_POINT('Ctrl Pts',(5.74240178399994,11.6,-9.86158796700001));
#164088=CARTESIAN_POINT('Ctrl Pts',(5.74206826599994,15.2,-9.85789800900001));
#164089=CARTESIAN_POINT('Ctrl Pts',(5.74206826599994,11.6,-9.85789800900001));
#164090=CARTESIAN_POINT('Ctrl Pts',(5.74173232899994,15.2,-9.85421280600001));
#164091=CARTESIAN_POINT('Ctrl Pts',(5.74173232899994,11.6,-9.85421280600001));
#164092=CARTESIAN_POINT('Ctrl Pts',(5.74139397699994,15.2,-9.85053236500001));
#164093=CARTESIAN_POINT('Ctrl Pts',(5.74139397699994,11.6,-9.85053236500001));
#164094=CARTESIAN_POINT('Ctrl Pts',(5.74105321799995,15.2,-9.84685669200001));
#164095=CARTESIAN_POINT('Ctrl Pts',(5.74105321799995,11.6,-9.84685669200001));
#164096=CARTESIAN_POINT('Ctrl Pts',(5.74071005799994,15.2,-9.84318579400002));
#164097=CARTESIAN_POINT('Ctrl Pts',(5.74071005799994,11.6,-9.84318579400002));
#164098=CARTESIAN_POINT('Ctrl Pts',(5.74036450299994,15.2,-9.83951967700001));
#164099=CARTESIAN_POINT('Ctrl Pts',(5.74036450299994,11.6,-9.83951967700001));
#164100=CARTESIAN_POINT('Ctrl Pts',(5.74001655999995,15.2,-9.83585834800001));
#164101=CARTESIAN_POINT('Ctrl Pts',(5.74001655999995,11.6,-9.83585834800001));
#164102=CARTESIAN_POINT('Ctrl Pts',(5.73966623499994,15.2,-9.83220181600001));
#164103=CARTESIAN_POINT('Ctrl Pts',(5.73966623499994,11.6,-9.83220181600001));
#164104=CARTESIAN_POINT('Ctrl Pts',(5.73931353499994,15.2,-9.82855008400001));
#164105=CARTESIAN_POINT('Ctrl Pts',(5.73931353499994,11.6,-9.82855008400001));
#164106=CARTESIAN_POINT('Ctrl Pts',(5.73895846599994,15.2,-9.82490316000001));
#164107=CARTESIAN_POINT('Ctrl Pts',(5.73895846599994,11.6,-9.82490316000001));
#164108=CARTESIAN_POINT('Ctrl Pts',(5.73860103599994,15.2,-9.82126105300001));
#164109=CARTESIAN_POINT('Ctrl Pts',(5.73860103599994,11.6,-9.82126105300001));
#164110=CARTESIAN_POINT('Ctrl Pts',(5.73824124899994,15.2,-9.81762376700001));
#164111=CARTESIAN_POINT('Ctrl Pts',(5.73824124899994,11.6,-9.81762376700001));
#164112=CARTESIAN_POINT('Ctrl Pts',(5.73787911299994,15.2,-9.81399131000001));
#164113=CARTESIAN_POINT('Ctrl Pts',(5.73787911299994,11.6,-9.81399131000001));
#164114=CARTESIAN_POINT('Ctrl Pts',(5.73751463399994,15.2,-9.81036368900001));
#164115=CARTESIAN_POINT('Ctrl Pts',(5.73751463399994,11.6,-9.81036368900001));
#164116=CARTESIAN_POINT('Ctrl Pts',(5.73714781999994,15.2,-9.80674091000001));
#164117=CARTESIAN_POINT('Ctrl Pts',(5.73714781999994,11.6,-9.80674091000001));
#164118=CARTESIAN_POINT('Ctrl Pts',(5.73677867499994,15.2,-9.80312298100001));
#164119=CARTESIAN_POINT('Ctrl Pts',(5.73677867499994,11.6,-9.80312298100001));
#164120=CARTESIAN_POINT('Ctrl Pts',(5.73640720799995,15.2,-9.79950990700001));
#164121=CARTESIAN_POINT('Ctrl Pts',(5.73640720799995,11.6,-9.79950990700001));
#164122=CARTESIAN_POINT('Ctrl Pts',(5.73603342399994,15.2,-9.79590169600001));
#164123=CARTESIAN_POINT('Ctrl Pts',(5.73603342399994,11.6,-9.79590169600001));
#164124=CARTESIAN_POINT('Ctrl Pts',(5.73565733099994,15.2,-9.79229835400002));
#164125=CARTESIAN_POINT('Ctrl Pts',(5.73565733099994,11.6,-9.79229835400002));
#164126=CARTESIAN_POINT('Ctrl Pts',(5.73527893499994,15.2,-9.78869989000001));
#164127=CARTESIAN_POINT('Ctrl Pts',(5.73527893499994,11.6,-9.78869989000001));
#164128=CARTESIAN_POINT('Ctrl Pts',(5.73489824299994,15.2,-9.78510630700001));
#164129=CARTESIAN_POINT('Ctrl Pts',(5.73489824299994,11.6,-9.78510630700001));
#164130=CARTESIAN_POINT('Ctrl Pts',(5.73451525999994,15.2,-9.78151761500001));
#164131=CARTESIAN_POINT('Ctrl Pts',(5.73451525999994,11.6,-9.78151761500001));
#164132=CARTESIAN_POINT('Ctrl Pts',(5.73412999599994,15.2,-9.77793382000001));
#164133=CARTESIAN_POINT('Ctrl Pts',(5.73412999599994,11.6,-9.77793382000001));
#164134=CARTESIAN_POINT('Ctrl Pts',(5.73374245399994,15.2,-9.77435492900001));
#164135=CARTESIAN_POINT('Ctrl Pts',(5.73374245399994,11.6,-9.77435492900001));
#164136=CARTESIAN_POINT('Ctrl Pts',(5.73335264299994,15.2,-9.77078094800001));
#164137=CARTESIAN_POINT('Ctrl Pts',(5.73335264299994,11.6,-9.77078094800001));
#164138=CARTESIAN_POINT('Ctrl Pts',(5.73296056899995,15.2,-9.76721188400001));
#164139=CARTESIAN_POINT('Ctrl Pts',(5.73296056899995,11.6,-9.76721188400001));
#164140=CARTESIAN_POINT('Ctrl Pts',(5.73256623999994,15.2,-9.76364774500001));
#164141=CARTESIAN_POINT('Ctrl Pts',(5.73256623999994,11.6,-9.76364774500001));
#164142=CARTESIAN_POINT('Ctrl Pts',(5.73216966099994,15.2,-9.76008853600001));
#164143=CARTESIAN_POINT('Ctrl Pts',(5.73216966099994,11.6,-9.76008853600001));
#164144=CARTESIAN_POINT('Ctrl Pts',(5.73177084099994,15.2,-9.75653426500001));
#164145=CARTESIAN_POINT('Ctrl Pts',(5.73177084099994,11.6,-9.75653426500001));
#164146=CARTESIAN_POINT('Ctrl Pts',(5.73136978399994,15.2,-9.75298493900001));
#164147=CARTESIAN_POINT('Ctrl Pts',(5.73136978399994,11.6,-9.75298493900001));
#164148=CARTESIAN_POINT('Ctrl Pts',(5.73096649899995,15.2,-9.74944056400001));
#164149=CARTESIAN_POINT('Ctrl Pts',(5.73096649899995,11.6,-9.74944056400001));
#164150=CARTESIAN_POINT('Ctrl Pts',(5.73056099299994,15.2,-9.74590114900001));
#164151=CARTESIAN_POINT('Ctrl Pts',(5.73056099299994,11.6,-9.74590114900001));
#164152=CARTESIAN_POINT('Ctrl Pts',(5.73015327099994,15.2,-9.74236669900001));
#164153=CARTESIAN_POINT('Ctrl Pts',(5.73015327099994,11.6,-9.74236669900001));
#164154=CARTESIAN_POINT('Ctrl Pts',(5.72974333999994,15.2,-9.73883722000001));
#164155=CARTESIAN_POINT('Ctrl Pts',(5.72974333999994,11.6,-9.73883722000001));
#164156=CARTESIAN_POINT('Ctrl Pts',(5.72933120899994,15.2,-9.73531272100001));
#164157=CARTESIAN_POINT('Ctrl Pts',(5.72933120899994,11.6,-9.73531272100001));
#164158=CARTESIAN_POINT('Ctrl Pts',(5.72891688399994,15.2,-9.73179320900002));
#164159=CARTESIAN_POINT('Ctrl Pts',(5.72891688399994,11.6,-9.73179320900002));
#164160=CARTESIAN_POINT('Ctrl Pts',(5.72850037199994,15.2,-9.72827868900001));
#164161=CARTESIAN_POINT('Ctrl Pts',(5.72850037199994,11.6,-9.72827868900001));
#164162=CARTESIAN_POINT('Ctrl Pts',(5.72808167899994,15.2,-9.72476917000001));
#164163=CARTESIAN_POINT('Ctrl Pts',(5.72808167899994,11.6,-9.72476917000001));
#164164=CARTESIAN_POINT('Ctrl Pts',(5.72766081399994,15.2,-9.72126465700001));
#164165=CARTESIAN_POINT('Ctrl Pts',(5.72766081399994,11.6,-9.72126465700001));
#164166=CARTESIAN_POINT('Ctrl Pts',(5.72723778199995,15.2,-9.71776515800001));
#164167=CARTESIAN_POINT('Ctrl Pts',(5.72723778199995,11.6,-9.71776515800001));
#164168=CARTESIAN_POINT('Ctrl Pts',(5.72681258999994,15.2,-9.71427068000001));
#164169=CARTESIAN_POINT('Ctrl Pts',(5.72681258999994,11.6,-9.71427068000001));
#164170=CARTESIAN_POINT('Ctrl Pts',(5.72638524699995,15.2,-9.71078123000001));
#164171=CARTESIAN_POINT('Ctrl Pts',(5.72638524699995,11.6,-9.71078123000001));
#164172=CARTESIAN_POINT('Ctrl Pts',(5.72595575799995,15.2,-9.70729681500002));
#164173=CARTESIAN_POINT('Ctrl Pts',(5.72595575799995,11.6,-9.70729681500002));
#164174=CARTESIAN_POINT('Ctrl Pts',(5.72552413199994,15.2,-9.70381744100001));
#164175=CARTESIAN_POINT('Ctrl Pts',(5.72552413199994,11.6,-9.70381744100001));
#164176=CARTESIAN_POINT('Ctrl Pts',(5.72509037399994,15.2,-9.70034311500001));
#164177=CARTESIAN_POINT('Ctrl Pts',(5.72509037399994,11.6,-9.70034311500001));
#164178=CARTESIAN_POINT('Ctrl Pts',(5.72465449299995,15.2,-9.69687384600001));
#164179=CARTESIAN_POINT('Ctrl Pts',(5.72465449299995,11.6,-9.69687384600001));
#164180=CARTESIAN_POINT('Ctrl Pts',(5.72421649499995,15.2,-9.69340963900001));
#164181=CARTESIAN_POINT('Ctrl Pts',(5.72421649499995,11.6,-9.69340963900001));
#164182=CARTESIAN_POINT('Ctrl Pts',(5.72377638699994,15.2,-9.68995050200001));
#164183=CARTESIAN_POINT('Ctrl Pts',(5.72377638699994,11.6,-9.68995050200001));
#164184=CARTESIAN_POINT('Ctrl Pts',(5.72333417799994,15.2,-9.68649644100001));
#164185=CARTESIAN_POINT('Ctrl Pts',(5.72333417799994,11.6,-9.68649644100001));
#164186=CARTESIAN_POINT('Ctrl Pts',(5.72288987299994,15.2,-9.68304746400001));
#164187=CARTESIAN_POINT('Ctrl Pts',(5.72288987299994,11.6,-9.68304746400001));
#164188=CARTESIAN_POINT('Ctrl Pts',(5.72244347999994,15.2,-9.67960357800001));
#164189=CARTESIAN_POINT('Ctrl Pts',(5.72244347999994,11.6,-9.67960357800001));
#164190=CARTESIAN_POINT('Ctrl Pts',(5.72199500699995,15.2,-9.67616478900001));
#164191=CARTESIAN_POINT('Ctrl Pts',(5.72199500699995,11.6,-9.67616478900001));
#164192=CARTESIAN_POINT('Ctrl Pts',(5.72154445999995,15.2,-9.67273110600001));
#164193=CARTESIAN_POINT('Ctrl Pts',(5.72154445999995,11.6,-9.67273110600001));
#164194=CARTESIAN_POINT('Ctrl Pts',(5.72109184699994,15.2,-9.66930253400001));
#164195=CARTESIAN_POINT('Ctrl Pts',(5.72109184699994,11.6,-9.66930253400001));
#164196=CARTESIAN_POINT('Ctrl Pts',(5.72063717499995,15.2,-9.66587908100001));
#164197=CARTESIAN_POINT('Ctrl Pts',(5.72063717499995,11.6,-9.66587908100001));
#164198=CARTESIAN_POINT('Ctrl Pts',(5.72018045099995,15.2,-9.66246075400001));
#164199=CARTESIAN_POINT('Ctrl Pts',(5.72018045099995,11.6,-9.66246075400001));
#164200=CARTESIAN_POINT('Ctrl Pts',(5.71972168399995,15.2,-9.65904755900001));
#164201=CARTESIAN_POINT('Ctrl Pts',(5.71972168399995,11.6,-9.65904755900001));
#164202=CARTESIAN_POINT('Ctrl Pts',(5.71926087999994,15.2,-9.65563950500002));
#164203=CARTESIAN_POINT('Ctrl Pts',(5.71926087999994,11.6,-9.65563950500002));
#164204=CARTESIAN_POINT('Ctrl Pts',(5.71879804599994,15.2,-9.65223659800002));
#164205=CARTESIAN_POINT('Ctrl Pts',(5.71879804599994,11.6,-9.65223659800002));
#164206=CARTESIAN_POINT('Ctrl Pts',(5.71833318999994,15.2,-9.64883884500002));
#164207=CARTESIAN_POINT('Ctrl Pts',(5.71833318999994,11.6,-9.64883884500002));
#164208=CARTESIAN_POINT('Ctrl Pts',(5.71786631899994,15.2,-9.64544625300002));
#164209=CARTESIAN_POINT('Ctrl Pts',(5.71786631899994,11.6,-9.64544625300002));
#164210=CARTESIAN_POINT('Ctrl Pts',(5.71739744199995,15.2,-9.64205883000002));
#164211=CARTESIAN_POINT('Ctrl Pts',(5.71739744199995,11.6,-9.64205883000002));
#164212=CARTESIAN_POINT('Ctrl Pts',(5.71692656399994,15.2,-9.63867658200002));
#164213=CARTESIAN_POINT('Ctrl Pts',(5.71692656399994,11.6,-9.63867658200002));
#164214=CARTESIAN_POINT('Ctrl Pts',(5.71645369399994,15.2,-9.63529951700002));
#164215=CARTESIAN_POINT('Ctrl Pts',(5.71645369399994,11.6,-9.63529951700002));
#164216=CARTESIAN_POINT('Ctrl Pts',(5.71597883899994,15.2,-9.63192764200001));
#164217=CARTESIAN_POINT('Ctrl Pts',(5.71597883899994,11.6,-9.63192764200001));
#164218=CARTESIAN_POINT('Ctrl Pts',(5.71550200799994,15.2,-9.62856096300002));
#164219=CARTESIAN_POINT('Ctrl Pts',(5.71550200799994,11.6,-9.62856096300002));
#164220=CARTESIAN_POINT('Ctrl Pts',(5.71502320499994,15.2,-9.62519948800002));
#164221=CARTESIAN_POINT('Ctrl Pts',(5.71502320499994,11.6,-9.62519948800002));
#164222=CARTESIAN_POINT('Ctrl Pts',(5.71454244099994,15.2,-9.62184322500002));
#164223=CARTESIAN_POINT('Ctrl Pts',(5.71454244099994,11.6,-9.62184322500002));
#164224=CARTESIAN_POINT('Ctrl Pts',(5.71405972199994,15.2,-9.61849218000001));
#164225=CARTESIAN_POINT('Ctrl Pts',(5.71405972199994,11.6,-9.61849218000001));
#164226=CARTESIAN_POINT('Ctrl Pts',(5.71357505599994,15.2,-9.61514636100001));
#164227=CARTESIAN_POINT('Ctrl Pts',(5.71357505599994,11.6,-9.61514636100001));
#164228=CARTESIAN_POINT('Ctrl Pts',(5.71308845099994,15.2,-9.61180577300001));
#164229=CARTESIAN_POINT('Ctrl Pts',(5.71308845099994,11.6,-9.61180577300001));
#164230=CARTESIAN_POINT('Ctrl Pts',(5.71259991299994,15.2,-9.60847042600001));
#164231=CARTESIAN_POINT('Ctrl Pts',(5.71259991299994,11.6,-9.60847042600001));
#164232=CARTESIAN_POINT('Ctrl Pts',(5.71210945199994,15.2,-9.60514032600001));
#164233=CARTESIAN_POINT('Ctrl Pts',(5.71210945199994,11.6,-9.60514032600001));
#164234=CARTESIAN_POINT('Ctrl Pts',(5.71161707499994,15.2,-9.60181548000002));
#164235=CARTESIAN_POINT('Ctrl Pts',(5.71161707499994,11.6,-9.60181548000002));
#164236=CARTESIAN_POINT('Ctrl Pts',(5.71112278699994,15.2,-9.59849589500001));
#164237=CARTESIAN_POINT('Ctrl Pts',(5.71112278699994,11.6,-9.59849589500001));
#164238=CARTESIAN_POINT('Ctrl Pts',(5.71062659999994,15.2,-9.59518158000002));
#164239=CARTESIAN_POINT('Ctrl Pts',(5.71062659999994,11.6,-9.59518158000002));
#164240=CARTESIAN_POINT('Ctrl Pts',(5.71012851799994,15.2,-9.59187253900001));
#164241=CARTESIAN_POINT('Ctrl Pts',(5.71012851799994,11.6,-9.59187253900001));
#164242=CARTESIAN_POINT('Ctrl Pts',(5.70962855099994,15.2,-9.58856878200002));
#164243=CARTESIAN_POINT('Ctrl Pts',(5.70962855099994,11.6,-9.58856878200002));
#164244=CARTESIAN_POINT('Ctrl Pts',(5.70912670599995,15.2,-9.58527031600001));
#164245=CARTESIAN_POINT('Ctrl Pts',(5.70912670599995,11.6,-9.58527031600001));
#164246=CARTESIAN_POINT('Ctrl Pts',(5.70862299199995,15.2,-9.58197714600002));
#164247=CARTESIAN_POINT('Ctrl Pts',(5.70862299199995,11.6,-9.58197714600002));
#164248=CARTESIAN_POINT('Ctrl Pts',(5.70811741599995,15.2,-9.57868928200002));
#164249=CARTESIAN_POINT('Ctrl Pts',(5.70811741599995,11.6,-9.57868928200002));
#164250=CARTESIAN_POINT('Ctrl Pts',(5.70760998399994,15.2,-9.57540673000001));
#164251=CARTESIAN_POINT('Ctrl Pts',(5.70760998399994,11.6,-9.57540673000001));
#164252=CARTESIAN_POINT('Ctrl Pts',(5.70710070599994,15.2,-9.57212949500001));
#164253=CARTESIAN_POINT('Ctrl Pts',(5.70710070599994,11.6,-9.57212949500001));
#164254=CARTESIAN_POINT('Ctrl Pts',(5.70658958999994,15.2,-9.56885759000001));
#164255=CARTESIAN_POINT('Ctrl Pts',(5.70658958999994,11.6,-9.56885759000001));
#164256=CARTESIAN_POINT('Ctrl Pts',(5.70607664199994,15.2,-9.56559101600002));
#164257=CARTESIAN_POINT('Ctrl Pts',(5.70607664199994,11.6,-9.56559101600002));
#164258=CARTESIAN_POINT('Ctrl Pts',(5.70556187299994,15.2,-9.56232978500001));
#164259=CARTESIAN_POINT('Ctrl Pts',(5.70556187299994,11.6,-9.56232978500001));
#164260=CARTESIAN_POINT('Ctrl Pts',(5.70504528799994,15.2,-9.55907390100002));
#164261=CARTESIAN_POINT('Ctrl Pts',(5.70504528799994,11.6,-9.55907390100002));
#164262=CARTESIAN_POINT('Ctrl Pts',(5.70452689699994,15.2,-9.55582337400001));
#164263=CARTESIAN_POINT('Ctrl Pts',(5.70452689699994,11.6,-9.55582337400001));
#164264=CARTESIAN_POINT('Ctrl Pts',(5.70400670599994,15.2,-9.55257821000002));
#164265=CARTESIAN_POINT('Ctrl Pts',(5.70400670599994,11.6,-9.55257821000002));
#164266=CARTESIAN_POINT('Ctrl Pts',(5.70348472499995,15.2,-9.54933841600001));
#164267=CARTESIAN_POINT('Ctrl Pts',(5.70348472499995,11.6,-9.54933841600001));
#164268=CARTESIAN_POINT('Ctrl Pts',(5.70296095999995,15.2,-9.54610399900002));
#164269=CARTESIAN_POINT('Ctrl Pts',(5.70296095999995,11.6,-9.54610399900002));
#164270=CARTESIAN_POINT('Ctrl Pts',(5.70243542199995,15.2,-9.54287496800001));
#164271=CARTESIAN_POINT('Ctrl Pts',(5.70243542199995,11.6,-9.54287496800001));
#164272=CARTESIAN_POINT('Ctrl Pts',(5.70190811599995,15.2,-9.53965133000001));
#164273=CARTESIAN_POINT('Ctrl Pts',(5.70190811599995,11.6,-9.53965133000001));
#164274=CARTESIAN_POINT('Ctrl Pts',(5.70137905199994,15.2,-9.53643309100002));
#164275=CARTESIAN_POINT('Ctrl Pts',(5.70137905199994,11.6,-9.53643309100002));
#164276=CARTESIAN_POINT('Ctrl Pts',(5.70084823799994,15.2,-9.53322025800002));
#164277=CARTESIAN_POINT('Ctrl Pts',(5.70084823799994,11.6,-9.53322025800002));
#164278=CARTESIAN_POINT('Ctrl Pts',(5.70031568099994,15.2,-9.53001284100001));
#164279=CARTESIAN_POINT('Ctrl Pts',(5.70031568099994,11.6,-9.53001284100001));
#164280=CARTESIAN_POINT('Ctrl Pts',(5.69978138899994,15.2,-9.52681084500002));
#164281=CARTESIAN_POINT('Ctrl Pts',(5.69978138899994,11.6,-9.52681084500002));
#164282=CARTESIAN_POINT('Ctrl Pts',(5.69924537299995,15.2,-9.52361427900002));
#164283=CARTESIAN_POINT('Ctrl Pts',(5.69924537299995,11.6,-9.52361427900002));
#164284=CARTESIAN_POINT('Ctrl Pts',(5.69870763799995,15.2,-9.52042315000002));
#164285=CARTESIAN_POINT('Ctrl Pts',(5.69870763799995,11.6,-9.52042315000002));
#164286=CARTESIAN_POINT('Ctrl Pts',(5.69816819399994,15.2,-9.51723746400001));
#164287=CARTESIAN_POINT('Ctrl Pts',(5.69816819399994,11.6,-9.51723746400001));
#164288=CARTESIAN_POINT('Ctrl Pts',(5.69762704799994,15.2,-9.51405723000001));
#164289=CARTESIAN_POINT('Ctrl Pts',(5.69762704799994,11.6,-9.51405723000001));
#164290=CARTESIAN_POINT('Ctrl Pts',(5.69708420999994,15.2,-9.51088245500002));
#164291=CARTESIAN_POINT('Ctrl Pts',(5.69708420999994,11.6,-9.51088245500002));
#164292=CARTESIAN_POINT('Ctrl Pts',(5.69653968699994,15.2,-9.50771314600001));
#164293=CARTESIAN_POINT('Ctrl Pts',(5.69653968699994,11.6,-9.50771314600001));
#164294=CARTESIAN_POINT('Ctrl Pts',(5.69599348799994,15.2,-9.50454931200002));
#164295=CARTESIAN_POINT('Ctrl Pts',(5.69599348799994,11.6,-9.50454931200002));
#164296=CARTESIAN_POINT('Ctrl Pts',(5.69544561999995,15.2,-9.50139095900001));
#164297=CARTESIAN_POINT('Ctrl Pts',(5.69544561999995,11.6,-9.50139095900001));
#164298=CARTESIAN_POINT('Ctrl Pts',(5.69489609299994,15.2,-9.49823809400002));
#164299=CARTESIAN_POINT('Ctrl Pts',(5.69489609299994,11.6,-9.49823809400002));
#164300=CARTESIAN_POINT('Ctrl Pts',(5.69434491599995,15.2,-9.49509072500001));
#164301=CARTESIAN_POINT('Ctrl Pts',(5.69434491599995,11.6,-9.49509072500001));
#164302=CARTESIAN_POINT('Ctrl Pts',(5.69379209399995,15.2,-9.49194886000001));
#164303=CARTESIAN_POINT('Ctrl Pts',(5.69379209399995,11.6,-9.49194886000001));
#164304=CARTESIAN_POINT('Ctrl Pts',(5.69323763999994,15.2,-9.48881250600002));
#164305=CARTESIAN_POINT('Ctrl Pts',(5.69323763999994,11.6,-9.48881250600002));
#164306=CARTESIAN_POINT('Ctrl Pts',(5.69268155899994,15.2,-9.48568167100002));
#164307=CARTESIAN_POINT('Ctrl Pts',(5.69268155899994,11.6,-9.48568167100002));
#164308=CARTESIAN_POINT('Ctrl Pts',(5.69212386099994,15.2,-9.48255636200001));
#164309=CARTESIAN_POINT('Ctrl Pts',(5.69212386099994,11.6,-9.48255636200001));
#164310=CARTESIAN_POINT('Ctrl Pts',(5.69156455399994,15.2,-9.47943658700002));
#164311=CARTESIAN_POINT('Ctrl Pts',(5.69156455399994,11.6,-9.47943658700002));
#164312=CARTESIAN_POINT('Ctrl Pts',(5.69100364599994,15.2,-9.47632235300001));
#164313=CARTESIAN_POINT('Ctrl Pts',(5.69100364599994,11.6,-9.47632235300001));
#164314=CARTESIAN_POINT('Ctrl Pts',(5.69044114799994,15.2,-9.47321366800002));
#164315=CARTESIAN_POINT('Ctrl Pts',(5.69044114799994,11.6,-9.47321366800002));
#164316=CARTESIAN_POINT('Ctrl Pts',(5.68987706599994,15.2,-9.47011053900002));
#164317=CARTESIAN_POINT('Ctrl Pts',(5.68987706599994,11.6,-9.47011053900002));
#164318=CARTESIAN_POINT('Ctrl Pts',(5.68931140899994,15.2,-9.46701297400002));
#164319=CARTESIAN_POINT('Ctrl Pts',(5.68931140899994,11.6,-9.46701297400002));
#164320=CARTESIAN_POINT('Ctrl Pts',(5.68874418599995,15.2,-9.46392098000001));
#164321=CARTESIAN_POINT('Ctrl Pts',(5.68874418599995,11.6,-9.46392098000001));
#164322=CARTESIAN_POINT('Ctrl Pts',(5.68817540599994,15.2,-9.46083456600002));
#164323=CARTESIAN_POINT('Ctrl Pts',(5.68817540599994,11.6,-9.46083456600002));
#164324=CARTESIAN_POINT('Ctrl Pts',(5.68760507799994,15.2,-9.45775373800002));
#164325=CARTESIAN_POINT('Ctrl Pts',(5.68760507799994,11.6,-9.45775373800002));
#164326=CARTESIAN_POINT('Ctrl Pts',(5.68703320999995,15.2,-9.45467850400001));
#164327=CARTESIAN_POINT('Ctrl Pts',(5.68703320999995,11.6,-9.45467850400001));
#164328=CARTESIAN_POINT('Ctrl Pts',(5.68645981099994,15.2,-9.45160887100002));
#164329=CARTESIAN_POINT('Ctrl Pts',(5.68645981099994,11.6,-9.45160887100002));
#164330=CARTESIAN_POINT('Ctrl Pts',(5.68588488999994,15.2,-9.44854484900001));
#164331=CARTESIAN_POINT('Ctrl Pts',(5.68588488999994,11.6,-9.44854484900001));
#164332=CARTESIAN_POINT('Ctrl Pts',(5.68530845499994,15.2,-9.44548644300001));
#164333=CARTESIAN_POINT('Ctrl Pts',(5.68530845499994,11.6,-9.44548644300001));
#164334=CARTESIAN_POINT('Ctrl Pts',(5.68473051499994,15.2,-9.44243366200002));
#164335=CARTESIAN_POINT('Ctrl Pts',(5.68473051499994,11.6,-9.44243366200002));
#164336=CARTESIAN_POINT('Ctrl Pts',(5.68415107899994,15.2,-9.43938651300002));
#164337=CARTESIAN_POINT('Ctrl Pts',(5.68415107899994,11.6,-9.43938651300002));
#164338=CARTESIAN_POINT('Ctrl Pts',(5.68357015699994,15.2,-9.43634500500002));
#164339=CARTESIAN_POINT('Ctrl Pts',(5.68357015699994,11.6,-9.43634500500002));
#164340=CARTESIAN_POINT('Ctrl Pts',(5.68298775599994,15.2,-9.43330914300001));
#164341=CARTESIAN_POINT('Ctrl Pts',(5.68298775599994,11.6,-9.43330914300001));
#164342=CARTESIAN_POINT('Ctrl Pts',(5.68240388599994,15.2,-9.43027893700001));
#164343=CARTESIAN_POINT('Ctrl Pts',(5.68240388599994,11.6,-9.43027893700001));
#164344=CARTESIAN_POINT('Ctrl Pts',(5.68181855599994,15.2,-9.42725439300002));
#164345=CARTESIAN_POINT('Ctrl Pts',(5.68181855599994,11.6,-9.42725439300002));
#164346=CARTESIAN_POINT('Ctrl Pts',(5.68123177399994,15.2,-9.42423552100001));
#164347=CARTESIAN_POINT('Ctrl Pts',(5.68123177399994,11.6,-9.42423552100001));
#164348=CARTESIAN_POINT('Ctrl Pts',(5.68064354999994,15.2,-9.42122232700001));
#164349=CARTESIAN_POINT('Ctrl Pts',(5.68064354999994,11.6,-9.42122232700001));
#164350=CARTESIAN_POINT('Ctrl Pts',(5.68005389299994,15.2,-9.41821481800002));
#164351=CARTESIAN_POINT('Ctrl Pts',(5.68005389299994,11.6,-9.41821481800002));
#164352=CARTESIAN_POINT('Ctrl Pts',(5.67946281099994,15.2,-9.41521300400002));
#164353=CARTESIAN_POINT('Ctrl Pts',(5.67946281099994,11.6,-9.41521300400002));
#164354=CARTESIAN_POINT('Ctrl Pts',(5.67887031499994,15.2,-9.41221689100002));
#164355=CARTESIAN_POINT('Ctrl Pts',(5.67887031499994,11.6,-9.41221689100002));
#164356=CARTESIAN_POINT('Ctrl Pts',(5.67827641199995,15.2,-9.40922648700001));
#164357=CARTESIAN_POINT('Ctrl Pts',(5.67827641199995,11.6,-9.40922648700001));
#164358=CARTESIAN_POINT('Ctrl Pts',(5.67768111099994,15.2,-9.40624180000002));
#164359=CARTESIAN_POINT('Ctrl Pts',(5.67768111099994,11.6,-9.40624180000002));
#164360=CARTESIAN_POINT('Ctrl Pts',(5.67708442399995,15.2,-9.40326283800001));
#164361=CARTESIAN_POINT('Ctrl Pts',(5.67708442399995,11.6,-9.40326283800001));
#164362=CARTESIAN_POINT('Ctrl Pts',(5.67648635699994,15.2,-9.40028960800002));
#164363=CARTESIAN_POINT('Ctrl Pts',(5.67648635699994,11.6,-9.40028960800002));
#164364=CARTESIAN_POINT('Ctrl Pts',(5.67588692199994,15.2,-9.39732211900001));
#164365=CARTESIAN_POINT('Ctrl Pts',(5.67588692199994,11.6,-9.39732211900001));
#164366=CARTESIAN_POINT('Ctrl Pts',(5.67528612499995,15.2,-9.39436037700002));
#164367=CARTESIAN_POINT('Ctrl Pts',(5.67528612499995,11.6,-9.39436037700002));
#164368=CARTESIAN_POINT('Ctrl Pts',(5.67468397799994,15.2,-9.39140439100001));
#164369=CARTESIAN_POINT('Ctrl Pts',(5.67468397799994,11.6,-9.39140439100001));
#164370=CARTESIAN_POINT('Ctrl Pts',(5.67408048899994,15.2,-9.38845416900002));
#164371=CARTESIAN_POINT('Ctrl Pts',(5.67408048899994,11.6,-9.38845416900002));
#164372=CARTESIAN_POINT('Ctrl Pts',(5.67347566799994,15.2,-9.38550971800002));
#164373=CARTESIAN_POINT('Ctrl Pts',(5.67347566799994,11.6,-9.38550971800002));
#164374=CARTESIAN_POINT('Ctrl Pts',(5.67286952299994,15.2,-9.38257104700002));
#164375=CARTESIAN_POINT('Ctrl Pts',(5.67286952299994,11.6,-9.38257104700002));
#164376=CARTESIAN_POINT('Ctrl Pts',(5.67226206399994,15.2,-9.37963816300002));
#164377=CARTESIAN_POINT('Ctrl Pts',(5.67226206399994,11.6,-9.37963816300002));
#164378=CARTESIAN_POINT('Ctrl Pts',(5.67165330199994,15.2,-9.37671107400002));
#164379=CARTESIAN_POINT('Ctrl Pts',(5.67165330199994,11.6,-9.37671107400002));
#164380=CARTESIAN_POINT('Ctrl Pts',(5.67104324399994,15.2,-9.37378978800002));
#164381=CARTESIAN_POINT('Ctrl Pts',(5.67104324399994,11.6,-9.37378978800002));
#164382=CARTESIAN_POINT('Ctrl Pts',(5.67043190099994,15.2,-9.37087431300002));
#164383=CARTESIAN_POINT('Ctrl Pts',(5.67043190099994,11.6,-9.37087431300002));
#164384=CARTESIAN_POINT('Ctrl Pts',(5.66981928099994,15.2,-9.36796465500001));
#164385=CARTESIAN_POINT('Ctrl Pts',(5.66981928099994,11.6,-9.36796465500001));
#164386=CARTESIAN_POINT('Ctrl Pts',(5.66920539599994,15.2,-9.36506082500001));
#164387=CARTESIAN_POINT('Ctrl Pts',(5.66920539599994,11.6,-9.36506082500001));
#164388=CARTESIAN_POINT('Ctrl Pts',(5.66859025199995,15.2,-9.36216282900002));
#164389=CARTESIAN_POINT('Ctrl Pts',(5.66859025199995,11.6,-9.36216282900002));
#164390=CARTESIAN_POINT('Ctrl Pts',(5.66797386299994,15.2,-9.35927067500002));
#164391=CARTESIAN_POINT('Ctrl Pts',(5.66797386299994,11.6,-9.35927067500002));
#164392=CARTESIAN_POINT('Ctrl Pts',(5.66735623499994,15.2,-9.35638437200002));
#164393=CARTESIAN_POINT('Ctrl Pts',(5.66735623499994,11.6,-9.35638437200002));
#164394=CARTESIAN_POINT('Ctrl Pts',(5.66673737799994,15.2,-9.35350392700002));
#164395=CARTESIAN_POINT('Ctrl Pts',(5.66673737799994,11.6,-9.35350392700002));
#164396=CARTESIAN_POINT('Ctrl Pts',(5.66611730199994,15.2,-9.35062934800002));
#164397=CARTESIAN_POINT('Ctrl Pts',(5.66611730199994,11.6,-9.35062934800002));
#164398=CARTESIAN_POINT('Ctrl Pts',(5.66549601799994,15.2,-9.34776064300002));
#164399=CARTESIAN_POINT('Ctrl Pts',(5.66549601799994,11.6,-9.34776064300002));
#164400=CARTESIAN_POINT('Ctrl Pts',(5.66487353399994,15.2,-9.34489782000002));
#164401=CARTESIAN_POINT('Ctrl Pts',(5.66487353399994,11.6,-9.34489782000002));
#164402=CARTESIAN_POINT('Ctrl Pts',(5.66424986199994,15.2,-9.34204088700002));
#164403=CARTESIAN_POINT('Ctrl Pts',(5.66424986199994,11.6,-9.34204088700002));
#164404=CARTESIAN_POINT('Ctrl Pts',(5.66362500799994,15.2,-9.33918985300001));
#164405=CARTESIAN_POINT('Ctrl Pts',(5.66362500799994,11.6,-9.33918985300001));
#164406=CARTESIAN_POINT('Ctrl Pts',(5.66299898499994,15.2,-9.33634472400002));
#164407=CARTESIAN_POINT('Ctrl Pts',(5.66299898499994,11.6,-9.33634472400002));
#164408=CARTESIAN_POINT('Ctrl Pts',(5.66237180199994,15.2,-9.33350551000002));
#164409=CARTESIAN_POINT('Ctrl Pts',(5.66237180199994,11.6,-9.33350551000002));
#164410=CARTESIAN_POINT('Ctrl Pts',(5.66174346799994,15.2,-9.33067221700002));
#164411=CARTESIAN_POINT('Ctrl Pts',(5.66174346799994,11.6,-9.33067221700002));
#164412=CARTESIAN_POINT('Ctrl Pts',(5.66111399299994,15.2,-9.32784485400001));
#164413=CARTESIAN_POINT('Ctrl Pts',(5.66111399299994,11.6,-9.32784485400001));
#164414=CARTESIAN_POINT('Ctrl Pts',(5.66048338799994,15.2,-9.32502343000002));
#164415=CARTESIAN_POINT('Ctrl Pts',(5.66048338799994,11.6,-9.32502343000002));
#164416=CARTESIAN_POINT('Ctrl Pts',(5.65985166199994,15.2,-9.32220795200001));
#164417=CARTESIAN_POINT('Ctrl Pts',(5.65985166199994,11.6,-9.32220795200001));
#164418=CARTESIAN_POINT('Ctrl Pts',(5.65921882599994,15.2,-9.31939842900002));
#164419=CARTESIAN_POINT('Ctrl Pts',(5.65921882599994,11.6,-9.31939842900002));
#164420=CARTESIAN_POINT('Ctrl Pts',(5.65858488799994,15.2,-9.31659486700001));
#164421=CARTESIAN_POINT('Ctrl Pts',(5.65858488799994,11.6,-9.31659486700001));
#164422=CARTESIAN_POINT('Ctrl Pts',(5.65794985999994,15.2,-9.31379727700002));
#164423=CARTESIAN_POINT('Ctrl Pts',(5.65794985999994,11.6,-9.31379727700002));
#164424=CARTESIAN_POINT('Ctrl Pts',(5.65731374999994,15.2,-9.31100566400002));
#164425=CARTESIAN_POINT('Ctrl Pts',(5.65731374999994,11.6,-9.31100566400002));
#164426=CARTESIAN_POINT('Ctrl Pts',(5.65667657099994,15.2,-9.30822003900002));
#164427=CARTESIAN_POINT('Ctrl Pts',(5.65667657099994,11.6,-9.30822003900002));
#164428=CARTESIAN_POINT('Ctrl Pts',(5.65603833099994,15.2,-9.30544040900001));
#164429=CARTESIAN_POINT('Ctrl Pts',(5.65603833099994,11.6,-9.30544040900001));
#164430=CARTESIAN_POINT('Ctrl Pts',(5.65539903999994,15.2,-9.30266678100002));
#164431=CARTESIAN_POINT('Ctrl Pts',(5.65539903999994,11.6,-9.30266678100002));
#164432=CARTESIAN_POINT('Ctrl Pts',(5.65475870899995,15.2,-9.29989916500002));
#164433=CARTESIAN_POINT('Ctrl Pts',(5.65475870899995,11.6,-9.29989916500002));
#164434=CARTESIAN_POINT('Ctrl Pts',(5.65411734799994,15.2,-9.29713756800002));
#164435=CARTESIAN_POINT('Ctrl Pts',(5.65411734799994,11.6,-9.29713756800002));
#164436=CARTESIAN_POINT('Ctrl Pts',(5.65347496699995,15.2,-9.29438199800002));
#164437=CARTESIAN_POINT('Ctrl Pts',(5.65347496699995,11.6,-9.29438199800002));
#164438=CARTESIAN_POINT('Ctrl Pts',(5.65283157699994,15.2,-9.29163246400002));
#164439=CARTESIAN_POINT('Ctrl Pts',(5.65283157699994,11.6,-9.29163246400002));
#164440=CARTESIAN_POINT('Ctrl Pts',(5.65218718599994,15.2,-9.28888897500002));
#164441=CARTESIAN_POINT('Ctrl Pts',(5.65218718599994,11.6,-9.28888897500002));
#164442=CARTESIAN_POINT('Ctrl Pts',(5.65154180699994,15.2,-9.28615153700001));
#164443=CARTESIAN_POINT('Ctrl Pts',(5.65154180699994,11.6,-9.28615153700001));
#164444=CARTESIAN_POINT('Ctrl Pts',(5.65089544999994,15.2,-9.28342016000002));
#164445=CARTESIAN_POINT('Ctrl Pts',(5.65089544999994,11.6,-9.28342016000002));
#164446=CARTESIAN_POINT('Ctrl Pts',(5.65024812399994,15.2,-9.28069485100002));
#164447=CARTESIAN_POINT('Ctrl Pts',(5.65024812399994,11.6,-9.28069485100002));
#164448=CARTESIAN_POINT('Ctrl Pts',(5.64959983999994,15.2,-9.27797561900002));
#164449=CARTESIAN_POINT('Ctrl Pts',(5.64959983999994,11.6,-9.27797561900002));
#164450=CARTESIAN_POINT('Ctrl Pts',(5.64895060899994,15.2,-9.27526247200002));
#164451=CARTESIAN_POINT('Ctrl Pts',(5.64895060899994,11.6,-9.27526247200002));
#164452=CARTESIAN_POINT('Ctrl Pts',(5.64830044099994,15.2,-9.27255541800001));
#164453=CARTESIAN_POINT('Ctrl Pts',(5.64830044099994,11.6,-9.27255541800001));
#164454=CARTESIAN_POINT('Ctrl Pts',(5.64764934599994,15.2,-9.26985446700002));
#164455=CARTESIAN_POINT('Ctrl Pts',(5.64764934599994,11.6,-9.26985446700002));
#164456=CARTESIAN_POINT('Ctrl Pts',(5.64699733599995,15.2,-9.26715962500002));
#164457=CARTESIAN_POINT('Ctrl Pts',(5.64699733599995,11.6,-9.26715962500002));
#164458=CARTESIAN_POINT('Ctrl Pts',(5.64634441999995,15.2,-9.26447090200002));
#164459=CARTESIAN_POINT('Ctrl Pts',(5.64634441999995,11.6,-9.26447090200002));
#164460=CARTESIAN_POINT('Ctrl Pts',(5.64569060899994,15.2,-9.26178830500002));
#164461=CARTESIAN_POINT('Ctrl Pts',(5.64569060899994,11.6,-9.26178830500002));
#164462=CARTESIAN_POINT('Ctrl Pts',(5.64503591399995,15.2,-9.25911184300002));
#164463=CARTESIAN_POINT('Ctrl Pts',(5.64503591399995,11.6,-9.25911184300002));
#164464=CARTESIAN_POINT('Ctrl Pts',(5.64438034599994,15.2,-9.25644152500002));
#164465=CARTESIAN_POINT('Ctrl Pts',(5.64438034599994,11.6,-9.25644152500002));
#164466=CARTESIAN_POINT('Ctrl Pts',(5.64372391599995,15.2,-9.25377735800001));
#164467=CARTESIAN_POINT('Ctrl Pts',(5.64372391599995,11.6,-9.25377735800001));
#164468=CARTESIAN_POINT('Ctrl Pts',(5.64306663299995,15.2,-9.25111935200002));
#164469=CARTESIAN_POINT('Ctrl Pts',(5.64306663299995,11.6,-9.25111935200002));
#164470=CARTESIAN_POINT('Ctrl Pts',(5.64240850899995,15.2,-9.24846751300001));
#164471=CARTESIAN_POINT('Ctrl Pts',(5.64240850899995,11.6,-9.24846751300001));
#164472=CARTESIAN_POINT('Ctrl Pts',(5.64174955499994,15.2,-9.24582185200002));
#164473=CARTESIAN_POINT('Ctrl Pts',(5.64174955499994,11.6,-9.24582185200002));
#164474=CARTESIAN_POINT('Ctrl Pts',(5.64108978099994,15.2,-9.24318237600002));
#164475=CARTESIAN_POINT('Ctrl Pts',(5.64108978099994,11.6,-9.24318237600002));
#164476=CARTESIAN_POINT('Ctrl Pts',(5.64042919799995,15.2,-9.24054909400001));
#164477=CARTESIAN_POINT('Ctrl Pts',(5.64042919799995,11.6,-9.24054909400001));
#164478=CARTESIAN_POINT('Ctrl Pts',(5.63976781599995,15.2,-9.23792201400002));
#164479=CARTESIAN_POINT('Ctrl Pts',(5.63976781599995,11.6,-9.23792201400002));
#164480=CARTESIAN_POINT('Ctrl Pts',(5.63910564999994,15.2,-9.23530114400002));
#164481=CARTESIAN_POINT('Ctrl Pts',(5.63910564999994,11.6,-9.23530114400002));
#164482=CARTESIAN_POINT('Ctrl Pts',(5.63844270699994,15.2,-9.23268649500002));
#164483=CARTESIAN_POINT('Ctrl Pts',(5.63844270699994,11.6,-9.23268649500002));
#164484=CARTESIAN_POINT('Ctrl Pts',(5.63777899799994,15.2,-9.23007807200002));
#164485=CARTESIAN_POINT('Ctrl Pts',(5.63777899799994,11.6,-9.23007807200002));
#164486=CARTESIAN_POINT('Ctrl Pts',(5.63711453599995,15.2,-9.22747588500001));
#164487=CARTESIAN_POINT('Ctrl Pts',(5.63711453599995,11.6,-9.22747588500001));
#164488=CARTESIAN_POINT('Ctrl Pts',(5.63644933199994,15.2,-9.22487994300001));
#164489=CARTESIAN_POINT('Ctrl Pts',(5.63644933199994,11.6,-9.22487994300001));
#164490=CARTESIAN_POINT('Ctrl Pts',(5.63578339499994,15.2,-9.22229025500001));
#164491=CARTESIAN_POINT('Ctrl Pts',(5.63578339499994,11.6,-9.22229025500001));
#164492=CARTESIAN_POINT('Ctrl Pts',(5.63511673699994,15.2,-9.21970682700002));
#164493=CARTESIAN_POINT('Ctrl Pts',(5.63511673699994,11.6,-9.21970682700002));
#164494=CARTESIAN_POINT('Ctrl Pts',(5.63444937099995,15.2,-9.21712967000002));
#164495=CARTESIAN_POINT('Ctrl Pts',(5.63444937099995,11.6,-9.21712967000002));
#164496=CARTESIAN_POINT('Ctrl Pts',(5.63378130699995,15.2,-9.21455879300002));
#164497=CARTESIAN_POINT('Ctrl Pts',(5.63378130699995,11.6,-9.21455879300002));
#164498=CARTESIAN_POINT('Ctrl Pts',(5.63311255499994,15.2,-9.21199420300002));
#164499=CARTESIAN_POINT('Ctrl Pts',(5.63311255499994,11.6,-9.21199420300002));
#164500=CARTESIAN_POINT('Ctrl Pts',(5.63244312799994,15.2,-9.20943590800002));
#164501=CARTESIAN_POINT('Ctrl Pts',(5.63244312799994,11.6,-9.20943590800002));
#164502=CARTESIAN_POINT('Ctrl Pts',(5.63177303699995,15.2,-9.20688391800002));
#164503=CARTESIAN_POINT('Ctrl Pts',(5.63177303699995,11.6,-9.20688391800002));
#164504=CARTESIAN_POINT('Ctrl Pts',(5.63110229299995,15.2,-9.20433824100002));
#164505=CARTESIAN_POINT('Ctrl Pts',(5.63110229299995,11.6,-9.20433824100002));
#164506=CARTESIAN_POINT('Ctrl Pts',(5.63043090699994,15.2,-9.20179888700002));
#164507=CARTESIAN_POINT('Ctrl Pts',(5.63043090699994,11.6,-9.20179888700002));
#164508=CARTESIAN_POINT('Ctrl Pts',(5.62975889099994,15.2,-9.19926586300001));
#164509=CARTESIAN_POINT('Ctrl Pts',(5.62975889099994,11.6,-9.19926586300001));
#164510=CARTESIAN_POINT('Ctrl Pts',(5.62908625599994,15.2,-9.19673917800001));
#164511=CARTESIAN_POINT('Ctrl Pts',(5.62908625599994,11.6,-9.19673917800001));
#164512=CARTESIAN_POINT('Ctrl Pts',(5.62841301499994,15.2,-9.19421884100002));
#164513=CARTESIAN_POINT('Ctrl Pts',(5.62841301499994,11.6,-9.19421884100002));
#164514=CARTESIAN_POINT('Ctrl Pts',(5.62773917699994,15.2,-9.19170486000001));
#164515=CARTESIAN_POINT('Ctrl Pts',(5.62773917699994,11.6,-9.19170486000001));
#164516=CARTESIAN_POINT('Ctrl Pts',(5.62706475599994,15.2,-9.18919724500002));
#164517=CARTESIAN_POINT('Ctrl Pts',(5.62706475599994,11.6,-9.18919724500002));
#164518=CARTESIAN_POINT('Ctrl Pts',(5.62638976199994,15.2,-9.18669600400002));
#164519=CARTESIAN_POINT('Ctrl Pts',(5.62638976199994,11.6,-9.18669600400002));
#164520=CARTESIAN_POINT('Ctrl Pts',(5.62571420699994,15.2,-9.18420114600002));
#164521=CARTESIAN_POINT('Ctrl Pts',(5.62571420699994,11.6,-9.18420114600002));
#164522=CARTESIAN_POINT('Ctrl Pts',(5.62503810399994,15.2,-9.18171268000001));
#164523=CARTESIAN_POINT('Ctrl Pts',(5.62503810399994,11.6,-9.18171268000001));
#164524=CARTESIAN_POINT('Ctrl Pts',(5.62436146299994,15.2,-9.17923061400002));
#164525=CARTESIAN_POINT('Ctrl Pts',(5.62436146299994,11.6,-9.17923061400002));
#164526=CARTESIAN_POINT('Ctrl Pts',(5.62368429599994,15.2,-9.17675495600001));
#164527=CARTESIAN_POINT('Ctrl Pts',(5.62368429599994,11.6,-9.17675495600001));
#164528=CARTESIAN_POINT('Ctrl Pts',(5.62300661499994,15.2,-9.17428571700002));
#164529=CARTESIAN_POINT('Ctrl Pts',(5.62300661499994,11.6,-9.17428571700002));
#164530=CARTESIAN_POINT('Ctrl Pts',(5.62232843199994,15.2,-9.17182290400002));
#164531=CARTESIAN_POINT('Ctrl Pts',(5.62232843199994,11.6,-9.17182290400002));
#164532=CARTESIAN_POINT('Ctrl Pts',(5.62164975999995,15.2,-9.16936652700001));
#164533=CARTESIAN_POINT('Ctrl Pts',(5.62164975999995,11.6,-9.16936652700001));
#164534=CARTESIAN_POINT('Ctrl Pts',(5.62097060899994,15.2,-9.16691659500002));
#164535=CARTESIAN_POINT('Ctrl Pts',(5.62097060899994,11.6,-9.16691659500002));
#164536=CARTESIAN_POINT('Ctrl Pts',(5.62029099199994,15.2,-9.16447311600002));
#164537=CARTESIAN_POINT('Ctrl Pts',(5.62029099199994,11.6,-9.16447311600002));
#164538=CARTESIAN_POINT('Ctrl Pts',(5.61961091999994,15.2,-9.16203609900002));
#164539=CARTESIAN_POINT('Ctrl Pts',(5.61961091999994,11.6,-9.16203609900002));
#164540=CARTESIAN_POINT('Ctrl Pts',(5.61893040599994,15.2,-9.15960555200002));
#164541=CARTESIAN_POINT('Ctrl Pts',(5.61893040599994,11.6,-9.15960555200002));
#164542=CARTESIAN_POINT('Ctrl Pts',(5.61824946299994,15.2,-9.15718148600002));
#164543=CARTESIAN_POINT('Ctrl Pts',(5.61824946299994,11.6,-9.15718148600002));
#164544=CARTESIAN_POINT('Ctrl Pts',(5.61756810099994,15.2,-9.15476390900002));
#164545=CARTESIAN_POINT('Ctrl Pts',(5.61756810099994,11.6,-9.15476390900002));
#164546=CARTESIAN_POINT('Ctrl Pts',(5.61688633399994,15.2,-9.15235283000002));
#164547=CARTESIAN_POINT('Ctrl Pts',(5.61688633399994,11.6,-9.15235283000002));
#164548=CARTESIAN_POINT('Ctrl Pts',(5.61620417199994,15.2,-9.14994825800001));
#164549=CARTESIAN_POINT('Ctrl Pts',(5.61620417199994,11.6,-9.14994825800001));
#164550=CARTESIAN_POINT('Ctrl Pts',(5.61552162899994,15.2,-9.14755020100002));
#164551=CARTESIAN_POINT('Ctrl Pts',(5.61552162899994,11.6,-9.14755020100002));
#164552=CARTESIAN_POINT('Ctrl Pts',(5.61483871699994,15.2,-9.14515867000001));
#164553=CARTESIAN_POINT('Ctrl Pts',(5.61483871699994,11.6,-9.14515867000001));
#164554=CARTESIAN_POINT('Ctrl Pts',(5.61415544799994,15.2,-9.14277367100001));
#164555=CARTESIAN_POINT('Ctrl Pts',(5.61415544799994,11.6,-9.14277367100001));
#164556=CARTESIAN_POINT('Ctrl Pts',(5.61347183399994,15.2,-9.14039521600002));
#164557=CARTESIAN_POINT('Ctrl Pts',(5.61347183399994,11.6,-9.14039521600002));
#164558=CARTESIAN_POINT('Ctrl Pts',(5.61278788899994,15.2,-9.13802331300002));
#164559=CARTESIAN_POINT('Ctrl Pts',(5.61278788899994,11.6,-9.13802331300002));
#164560=CARTESIAN_POINT('Ctrl Pts',(5.61210362299994,15.2,-9.13565797100001));
#164561=CARTESIAN_POINT('Ctrl Pts',(5.61210362299994,11.6,-9.13565797100001));
#164562=CARTESIAN_POINT('Ctrl Pts',(5.61141904999994,15.2,-9.13329919800002));
#164563=CARTESIAN_POINT('Ctrl Pts',(5.61141904999994,11.6,-9.13329919800002));
#164564=CARTESIAN_POINT('Ctrl Pts',(5.61073418199994,15.2,-9.13094700500002));
#164565=CARTESIAN_POINT('Ctrl Pts',(5.61073418199994,11.6,-9.13094700500002));
#164566=CARTESIAN_POINT('Ctrl Pts',(5.61004903199994,15.2,-9.12860140000002));
#164567=CARTESIAN_POINT('Ctrl Pts',(5.61004903199994,11.6,-9.12860140000002));
#164568=CARTESIAN_POINT('Ctrl Pts',(5.60936361399994,15.2,-9.12626239100002));
#164569=CARTESIAN_POINT('Ctrl Pts',(5.60936361399994,11.6,-9.12626239100002));
#164570=CARTESIAN_POINT('Ctrl Pts',(5.60867793699994,15.2,-9.12392999000001));
#164571=CARTESIAN_POINT('Ctrl Pts',(5.60867793699994,11.6,-9.12392999000001));
#164572=CARTESIAN_POINT('Ctrl Pts',(5.60799201599995,15.2,-9.12160420400001));
#164573=CARTESIAN_POINT('Ctrl Pts',(5.60799201599995,11.6,-9.12160420400001));
#164574=CARTESIAN_POINT('Ctrl Pts',(5.60730586399995,15.2,-9.11928504400001));
#164575=CARTESIAN_POINT('Ctrl Pts',(5.60730586399995,11.6,-9.11928504400001));
#164576=CARTESIAN_POINT('Ctrl Pts',(5.60661949299995,15.2,-9.11697251700001));
#164577=CARTESIAN_POINT('Ctrl Pts',(5.60661949299995,11.6,-9.11697251700001));
#164578=CARTESIAN_POINT('Ctrl Pts',(5.60593291599995,15.2,-9.11466663300001));
#164579=CARTESIAN_POINT('Ctrl Pts',(5.60593291599995,11.6,-9.11466663300001));
#164580=CARTESIAN_POINT('Ctrl Pts',(5.60524614599994,15.2,-9.11236740200002));
#164581=CARTESIAN_POINT('Ctrl Pts',(5.60524614599994,11.6,-9.11236740200002));
#164582=CARTESIAN_POINT('Ctrl Pts',(5.60455919499995,15.2,-9.11007483200001));
#164583=CARTESIAN_POINT('Ctrl Pts',(5.60455919499995,11.6,-9.11007483200001));
#164584=CARTESIAN_POINT('Ctrl Pts',(5.60387207799995,15.2,-9.10778893300002));
#164585=CARTESIAN_POINT('Ctrl Pts',(5.60387207799995,11.6,-9.10778893300002));
#164586=CARTESIAN_POINT('Ctrl Pts',(5.60318480499994,15.2,-9.10550971500001));
#164587=CARTESIAN_POINT('Ctrl Pts',(5.60318480499994,11.6,-9.10550971500001));
#164588=CARTESIAN_POINT('Ctrl Pts',(5.60249739199995,15.2,-9.10323718600001));
#164589=CARTESIAN_POINT('Ctrl Pts',(5.60249739199995,11.6,-9.10323718600001));
#164590=CARTESIAN_POINT('Ctrl Pts',(5.60180984999994,15.2,-9.10097135500001));
#164591=CARTESIAN_POINT('Ctrl Pts',(5.60180984999994,11.6,-9.10097135500001));
#164592=CARTESIAN_POINT('Ctrl Pts',(5.60112219399994,15.2,-9.09871223400001));
#164593=CARTESIAN_POINT('Ctrl Pts',(5.60112219399994,11.6,-9.09871223400001));
#164594=CARTESIAN_POINT('Ctrl Pts',(5.60043443499994,15.2,-9.09645983000001));
#164595=CARTESIAN_POINT('Ctrl Pts',(5.60043443499994,11.6,-9.09645983000001));
#164596=CARTESIAN_POINT('Ctrl Pts',(5.59974658699995,15.2,-9.09421415200002));
#164597=CARTESIAN_POINT('Ctrl Pts',(5.59974658699995,11.6,-9.09421415200002));
#164598=CARTESIAN_POINT('Ctrl Pts',(5.59905866399995,15.2,-9.09197521100002));
#164599=CARTESIAN_POINT('Ctrl Pts',(5.59905866399995,11.6,-9.09197521100002));
#164600=CARTESIAN_POINT('Ctrl Pts',(5.59837067799994,15.2,-9.08974301600002));
#164601=CARTESIAN_POINT('Ctrl Pts',(5.59837067799994,11.6,-9.08974301600002));
#164602=CARTESIAN_POINT('Ctrl Pts',(5.59768264499994,15.2,-9.08751757600001));
#164603=CARTESIAN_POINT('Ctrl Pts',(5.59768264499994,11.6,-9.08751757600001));
#164604=CARTESIAN_POINT('Ctrl Pts',(5.59699457499995,15.2,-9.08529890000001));
#164605=CARTESIAN_POINT('Ctrl Pts',(5.59699457499995,11.6,-9.08529890000001));
#164606=CARTESIAN_POINT('Ctrl Pts',(5.59630648299994,15.2,-9.08308699800001));
#164607=CARTESIAN_POINT('Ctrl Pts',(5.59630648299994,11.6,-9.08308699800001));
#164608=CARTESIAN_POINT('Ctrl Pts',(5.59561838299994,15.2,-9.08088187900002));
#164609=CARTESIAN_POINT('Ctrl Pts',(5.59561838299994,11.6,-9.08088187900002));
#164610=CARTESIAN_POINT('Ctrl Pts',(5.59493028699994,15.2,-9.07868355500002));
#164611=CARTESIAN_POINT('Ctrl Pts',(5.59493028699994,11.6,-9.07868355500002));
#164612=CARTESIAN_POINT('Ctrl Pts',(5.59424220999994,15.2,-9.07649203200002));
#164613=CARTESIAN_POINT('Ctrl Pts',(5.59424220999994,11.6,-9.07649203200002));
#164614=CARTESIAN_POINT('Ctrl Pts',(5.59355416599995,15.2,-9.07430732100002));
#164615=CARTESIAN_POINT('Ctrl Pts',(5.59355416599995,11.6,-9.07430732100002));
#164616=CARTESIAN_POINT('Ctrl Pts',(5.59286616599994,15.2,-9.07212943200001));
#164617=CARTESIAN_POINT('Ctrl Pts',(5.59286616599994,11.6,-9.07212943200001));
#164618=CARTESIAN_POINT('Ctrl Pts',(5.59217822699994,15.2,-9.06995837400002));
#164619=CARTESIAN_POINT('Ctrl Pts',(5.59217822699994,11.6,-9.06995837400002));
#164620=CARTESIAN_POINT('Ctrl Pts',(5.59149036099994,15.2,-9.06779415800001));
#164621=CARTESIAN_POINT('Ctrl Pts',(5.59149036099994,11.6,-9.06779415800001));
#164622=CARTESIAN_POINT('Ctrl Pts',(5.59080258099995,15.2,-9.06563679100002));
#164623=CARTESIAN_POINT('Ctrl Pts',(5.59080258099995,11.6,-9.06563679100002));
#164624=CARTESIAN_POINT('Ctrl Pts',(5.59011490299994,15.2,-9.06348628400002));
#164625=CARTESIAN_POINT('Ctrl Pts',(5.59011490299994,11.6,-9.06348628400002));
#164626=CARTESIAN_POINT('Ctrl Pts',(5.58942733899994,15.2,-9.06134264800002));
#164627=CARTESIAN_POINT('Ctrl Pts',(5.58942733899994,11.6,-9.06134264800002));
#164628=CARTESIAN_POINT('Ctrl Pts',(5.58873990499994,15.2,-9.05920589100001));
#164629=CARTESIAN_POINT('Ctrl Pts',(5.58873990499994,11.6,-9.05920589100001));
#164630=CARTESIAN_POINT('Ctrl Pts',(5.58805261299995,15.2,-9.05707602300001));
#164631=CARTESIAN_POINT('Ctrl Pts',(5.58805261299995,11.6,-9.05707602300001));
#164632=CARTESIAN_POINT('Ctrl Pts',(5.58736547799994,15.2,-9.05495305400001));
#164633=CARTESIAN_POINT('Ctrl Pts',(5.58736547799994,11.6,-9.05495305400001));
#164634=CARTESIAN_POINT('Ctrl Pts',(5.58667851399995,15.2,-9.05283699300002));
#164635=CARTESIAN_POINT('Ctrl Pts',(5.58667851399995,11.6,-9.05283699300002));
#164636=CARTESIAN_POINT('Ctrl Pts',(5.58599173399994,15.2,-9.05072785100002));
#164637=CARTESIAN_POINT('Ctrl Pts',(5.58599173399994,11.6,-9.05072785100002));
#164638=CARTESIAN_POINT('Ctrl Pts',(5.58530515499994,15.2,-9.04862563700001));
#164639=CARTESIAN_POINT('Ctrl Pts',(5.58530515499994,11.6,-9.04862563700001));
#164640=CARTESIAN_POINT('Ctrl Pts',(5.58461878799994,15.2,-9.04653036000001));
#164641=CARTESIAN_POINT('Ctrl Pts',(5.58461878799994,11.6,-9.04653036000001));
#164642=CARTESIAN_POINT('Ctrl Pts',(5.58393265099995,15.2,-9.04444203100002));
#164643=CARTESIAN_POINT('Ctrl Pts',(5.58393265099995,11.6,-9.04444203100002));
#164644=CARTESIAN_POINT('Ctrl Pts',(5.58324675399994,15.2,-9.04236066000001));
#164645=CARTESIAN_POINT('Ctrl Pts',(5.58324675399994,11.6,-9.04236066000001));
#164646=CARTESIAN_POINT('Ctrl Pts',(5.58256111399994,15.2,-9.04028625700001));
#164647=CARTESIAN_POINT('Ctrl Pts',(5.58256111399994,11.6,-9.04028625700001));
#164648=CARTESIAN_POINT('Ctrl Pts',(5.58187574599994,15.2,-9.03821883000001));
#164649=CARTESIAN_POINT('Ctrl Pts',(5.58187574599994,11.6,-9.03821883000001));
#164650=CARTESIAN_POINT('Ctrl Pts',(5.58119066299994,15.2,-9.03615839100001));
#164651=CARTESIAN_POINT('Ctrl Pts',(5.58119066299994,11.6,-9.03615839100001));
#164652=CARTESIAN_POINT('Ctrl Pts',(5.58050587999994,15.2,-9.03410495000001));
#164653=CARTESIAN_POINT('Ctrl Pts',(5.58050587999994,11.6,-9.03410495000001));
#164654=CARTESIAN_POINT('Ctrl Pts',(5.57982141099994,15.2,-9.03205851500001));
#164655=CARTESIAN_POINT('Ctrl Pts',(5.57982141099994,11.6,-9.03205851500001));
#164656=CARTESIAN_POINT('Ctrl Pts',(5.57913727299994,15.2,-9.03001909700002));
#164657=CARTESIAN_POINT('Ctrl Pts',(5.57913727299994,11.6,-9.03001909700002));
#164658=CARTESIAN_POINT('Ctrl Pts',(5.57845347799995,15.2,-9.02798670600001));
#164659=CARTESIAN_POINT('Ctrl Pts',(5.57845347799995,11.6,-9.02798670600001));
#164660=CARTESIAN_POINT('Ctrl Pts',(5.57777004199995,15.2,-9.02596135200002));
#164661=CARTESIAN_POINT('Ctrl Pts',(5.57777004199995,11.6,-9.02596135200002));
#164662=CARTESIAN_POINT('Ctrl Pts',(5.57708697999994,15.2,-9.02394304600002));
#164663=CARTESIAN_POINT('Ctrl Pts',(5.57708697999994,11.6,-9.02394304600002));
#164664=CARTESIAN_POINT('Ctrl Pts',(5.57640430699994,15.2,-9.02193179800001));
#164665=CARTESIAN_POINT('Ctrl Pts',(5.57640430699994,11.6,-9.02193179800001));
#164666=CARTESIAN_POINT('Ctrl Pts',(5.57572203699994,15.2,-9.01992761500002));
#164667=CARTESIAN_POINT('Ctrl Pts',(5.57572203699994,11.6,-9.01992761500002));
#164668=CARTESIAN_POINT('Ctrl Pts',(5.57504018499994,15.2,-9.01793051000002));
#164669=CARTESIAN_POINT('Ctrl Pts',(5.57504018499994,11.6,-9.01793051000002));
#164670=CARTESIAN_POINT('Ctrl Pts',(5.57435876799994,15.2,-9.01594049300002));
#164671=CARTESIAN_POINT('Ctrl Pts',(5.57435876799994,11.6,-9.01594049300002));
#164672=CARTESIAN_POINT('Ctrl Pts',(5.57367779799995,15.2,-9.01395757400002));
#164673=CARTESIAN_POINT('Ctrl Pts',(5.57367779799995,11.6,-9.01395757400002));
#164674=CARTESIAN_POINT('Ctrl Pts',(5.57299729299994,15.2,-9.01198176200002));
#164675=CARTESIAN_POINT('Ctrl Pts',(5.57299729299994,11.6,-9.01198176200002));
#164676=CARTESIAN_POINT('Ctrl Pts',(5.57231726599994,15.2,-9.01001306800002));
#164677=CARTESIAN_POINT('Ctrl Pts',(5.57231726599994,11.6,-9.01001306800002));
#164678=CARTESIAN_POINT('Ctrl Pts',(5.57163773399994,15.2,-9.00805150300002));
#164679=CARTESIAN_POINT('Ctrl Pts',(5.57163773399994,11.6,-9.00805150300002));
#164680=CARTESIAN_POINT('Ctrl Pts',(5.57095871099994,15.2,-9.00609707600001));
#164681=CARTESIAN_POINT('Ctrl Pts',(5.57095871099994,11.6,-9.00609707600001));
#164682=CARTESIAN_POINT('Ctrl Pts',(5.57028021399995,15.2,-9.00414979800002));
#164683=CARTESIAN_POINT('Ctrl Pts',(5.57028021399995,11.6,-9.00414979800002));
#164684=CARTESIAN_POINT('Ctrl Pts',(5.56960225599994,15.2,-9.00220967900001));
#164685=CARTESIAN_POINT('Ctrl Pts',(5.56960225599994,11.6,-9.00220967900001));
#164686=CARTESIAN_POINT('Ctrl Pts',(5.56892485499994,15.2,-9.00027672900002));
#164687=CARTESIAN_POINT('Ctrl Pts',(5.56892485499994,11.6,-9.00027672900002));
#164688=CARTESIAN_POINT('Ctrl Pts',(5.56824802499994,15.2,-8.99835095900002));
#164689=CARTESIAN_POINT('Ctrl Pts',(5.56824802499994,11.6,-8.99835095900002));
#164690=CARTESIAN_POINT('Ctrl Pts',(5.56757178199994,15.2,-8.99643237900002));
#164691=CARTESIAN_POINT('Ctrl Pts',(5.56757178199994,11.6,-8.99643237900002));
#164692=CARTESIAN_POINT('Ctrl Pts',(5.56689614199994,15.2,-8.99452099900002));
#164693=CARTESIAN_POINT('Ctrl Pts',(5.56689614199994,11.6,-8.99452099900002));
#164694=CARTESIAN_POINT('Ctrl Pts',(5.56622111999994,15.2,-8.99261683100002));
#164695=CARTESIAN_POINT('Ctrl Pts',(5.56622111999994,11.6,-8.99261683100002));
#164696=CARTESIAN_POINT('Ctrl Pts',(5.56554673199994,15.2,-8.99071988300001));
#164697=CARTESIAN_POINT('Ctrl Pts',(5.56554673199994,11.6,-8.99071988300001));
#164698=CARTESIAN_POINT('Ctrl Pts',(5.56487299499994,15.2,-8.98883016700001));
#164699=CARTESIAN_POINT('Ctrl Pts',(5.56487299499994,11.6,-8.98883016700001));
#164700=CARTESIAN_POINT('Ctrl Pts',(5.56419992299994,15.2,-8.98694769400001));
#164701=CARTESIAN_POINT('Ctrl Pts',(5.56419992299994,11.6,-8.98694769400001));
#164702=CARTESIAN_POINT('Ctrl Pts',(5.56352753399994,15.2,-8.98507247300002));
#164703=CARTESIAN_POINT('Ctrl Pts',(5.56352753399994,11.6,-8.98507247300002));
#164704=CARTESIAN_POINT('Ctrl Pts',(5.56285584299995,15.2,-8.98320451500001));
#164705=CARTESIAN_POINT('Ctrl Pts',(5.56285584299995,11.6,-8.98320451500001));
#164706=CARTESIAN_POINT('Ctrl Pts',(5.56218486399994,15.2,-8.98134383100002));
#164707=CARTESIAN_POINT('Ctrl Pts',(5.56218486399994,11.6,-8.98134383100002));
#164708=CARTESIAN_POINT('Ctrl Pts',(5.56151461599995,15.2,-8.97949043200001));
#164709=CARTESIAN_POINT('Ctrl Pts',(5.56151461599995,11.6,-8.97949043200001));
#164710=CARTESIAN_POINT('Ctrl Pts',(5.56084511599994,15.2,-8.97764432800002));
#164711=CARTESIAN_POINT('Ctrl Pts',(5.56084511599994,11.6,-8.97764432800002));
#164712=CARTESIAN_POINT('Ctrl Pts',(5.56017637699994,15.2,-8.97580552900001));
#164713=CARTESIAN_POINT('Ctrl Pts',(5.56017637699994,11.6,-8.97580552900001));
#164714=CARTESIAN_POINT('Ctrl Pts',(5.55950841699994,15.2,-8.97397404700002));
#164715=CARTESIAN_POINT('Ctrl Pts',(5.55950841699994,11.6,-8.97397404700002));
#164716=CARTESIAN_POINT('Ctrl Pts',(5.55884125299994,15.2,-8.97214989100002));
#164717=CARTESIAN_POINT('Ctrl Pts',(5.55884125299994,11.6,-8.97214989100002));
#164718=CARTESIAN_POINT('Ctrl Pts',(5.55817490099995,15.2,-8.97033307400001));
#164719=CARTESIAN_POINT('Ctrl Pts',(5.55817490099995,11.6,-8.97033307400001));
#164720=CARTESIAN_POINT('Ctrl Pts',(5.55750937599995,15.2,-8.96852360500001));
#164721=CARTESIAN_POINT('Ctrl Pts',(5.55750937599995,11.6,-8.96852360500001));
#164722=CARTESIAN_POINT('Ctrl Pts',(5.55684469699995,15.2,-8.96672149500001));
#164723=CARTESIAN_POINT('Ctrl Pts',(5.55684469699995,11.6,-8.96672149500001));
#164724=CARTESIAN_POINT('Ctrl Pts',(5.55618087999994,15.2,-8.96492675500001));
#164725=CARTESIAN_POINT('Ctrl Pts',(5.55618087999994,11.6,-8.96492675500001));
#164726=CARTESIAN_POINT('Ctrl Pts',(5.55551793999995,15.2,-8.96313939600001));
#164727=CARTESIAN_POINT('Ctrl Pts',(5.55551793999995,11.6,-8.96313939600001));
#164728=CARTESIAN_POINT('Ctrl Pts',(5.55485589499994,15.2,-8.96135942900001));
#164729=CARTESIAN_POINT('Ctrl Pts',(5.55485589499994,11.6,-8.96135942900001));
#164730=CARTESIAN_POINT('Ctrl Pts',(5.55419476299994,15.2,-8.95958686400002));
#164731=CARTESIAN_POINT('Ctrl Pts',(5.55419476299994,11.6,-8.95958686400002));
#164732=CARTESIAN_POINT('Ctrl Pts',(5.55353455899994,15.2,-8.95782171400001));
#164733=CARTESIAN_POINT('Ctrl Pts',(5.55353455899994,11.6,-8.95782171400001));
#164734=CARTESIAN_POINT('Ctrl Pts',(5.55287530099994,15.2,-8.95606398600002));
#164735=CARTESIAN_POINT('Ctrl Pts',(5.55287530099994,11.6,-8.95606398600002));
#164736=CARTESIAN_POINT('Ctrl Pts',(5.55221700599994,15.2,-8.95431369500002));
#164737=CARTESIAN_POINT('Ctrl Pts',(5.55221700599994,11.6,-8.95431369500002));
#164738=CARTESIAN_POINT('Ctrl Pts',(5.55155968999995,15.2,-8.95257085100001));
#164739=CARTESIAN_POINT('Ctrl Pts',(5.55155968999995,11.6,-8.95257085100001));
#164740=CARTESIAN_POINT('Ctrl Pts',(5.55090337199994,15.2,-8.95083546300001));
#164741=CARTESIAN_POINT('Ctrl Pts',(5.55090337199994,11.6,-8.95083546300001));
#164742=CARTESIAN_POINT('Ctrl Pts',(5.55024806799994,15.2,-8.94910754400002));
#164743=CARTESIAN_POINT('Ctrl Pts',(5.55024806799994,11.6,-8.94910754400002));
#164744=CARTESIAN_POINT('Ctrl Pts',(5.54959379599994,15.2,-8.94738710500001));
#164745=CARTESIAN_POINT('Ctrl Pts',(5.54959379599994,11.6,-8.94738710500001));
#164746=CARTESIAN_POINT('Ctrl Pts',(5.54894057199995,15.2,-8.94567415600001));
#164747=CARTESIAN_POINT('Ctrl Pts',(5.54894057199995,11.6,-8.94567415600001));
#164748=CARTESIAN_POINT('Ctrl Pts',(5.54828841499994,15.2,-8.94396870900002));
#164749=CARTESIAN_POINT('Ctrl Pts',(5.54828841499994,11.6,-8.94396870900002));
#164750=CARTESIAN_POINT('Ctrl Pts',(5.54763734099994,15.2,-8.94227077600002));
#164751=CARTESIAN_POINT('Ctrl Pts',(5.54763734099994,11.6,-8.94227077600002));
#164752=CARTESIAN_POINT('Ctrl Pts',(5.54698736999995,15.2,-8.94058036600001));
#164753=CARTESIAN_POINT('Ctrl Pts',(5.54698736999995,11.6,-8.94058036600001));
#164754=CARTESIAN_POINT('Ctrl Pts',(5.54633851699994,15.2,-8.93889749100002));
#164755=CARTESIAN_POINT('Ctrl Pts',(5.54633851699994,11.6,-8.93889749100002));
#164756=CARTESIAN_POINT('Ctrl Pts',(5.54569080099995,15.2,-8.93722216300001));
#164757=CARTESIAN_POINT('Ctrl Pts',(5.54569080099995,11.6,-8.93722216300001));
#164758=CARTESIAN_POINT('Ctrl Pts',(5.54504424099994,15.2,-8.93555439300001));
#164759=CARTESIAN_POINT('Ctrl Pts',(5.54504424099994,11.6,-8.93555439300001));
#164760=CARTESIAN_POINT('Ctrl Pts',(5.54439885199995,15.2,-8.93389419200001));
#164761=CARTESIAN_POINT('Ctrl Pts',(5.54439885199995,11.6,-8.93389419200001));
#164762=CARTESIAN_POINT('Ctrl Pts',(5.54375465499994,15.2,-8.93224157200001));
#164763=CARTESIAN_POINT('Ctrl Pts',(5.54375465499994,11.6,-8.93224157200001));
#164764=CARTESIAN_POINT('Ctrl Pts',(5.54311166499994,15.2,-8.93059654400002));
#164765=CARTESIAN_POINT('Ctrl Pts',(5.54311166499994,11.6,-8.93059654400002));
#164766=CARTESIAN_POINT('Ctrl Pts',(5.54246990199994,15.2,-8.92895911900002));
#164767=CARTESIAN_POINT('Ctrl Pts',(5.54246990199994,11.6,-8.92895911900002));
#164768=CARTESIAN_POINT('Ctrl Pts',(5.54182938399994,15.2,-8.92732930800002));
#164769=CARTESIAN_POINT('Ctrl Pts',(5.54182938399994,11.6,-8.92732930800002));
#164770=CARTESIAN_POINT('Ctrl Pts',(5.54119012799994,15.2,-8.92570712500002));
#164771=CARTESIAN_POINT('Ctrl Pts',(5.54119012799994,11.6,-8.92570712500002));
#164772=CARTESIAN_POINT('Ctrl Pts',(5.54055215399995,15.2,-8.92409257800002));
#164773=CARTESIAN_POINT('Ctrl Pts',(5.54055215399995,11.6,-8.92409257800002));
#164774=CARTESIAN_POINT('Ctrl Pts',(5.53991547999994,15.2,-8.92248568200002));
#164775=CARTESIAN_POINT('Ctrl Pts',(5.53991547999994,11.6,-8.92248568200002));
#164776=CARTESIAN_POINT('Ctrl Pts',(5.53928012499994,15.2,-8.92088644500001));
#164777=CARTESIAN_POINT('Ctrl Pts',(5.53928012499994,11.6,-8.92088644500001));
#164778=CARTESIAN_POINT('Ctrl Pts',(5.53864610499994,15.2,-8.91929488200002));
#164779=CARTESIAN_POINT('Ctrl Pts',(5.53864610499994,11.6,-8.91929488200002));
#164780=CARTESIAN_POINT('Ctrl Pts',(5.53801344099995,15.2,-8.91771100200001));
#164781=CARTESIAN_POINT('Ctrl Pts',(5.53801344099995,11.6,-8.91771100200001));
#164782=CARTESIAN_POINT('Ctrl Pts',(5.53738214999995,15.2,-8.91613481900002));
#164783=CARTESIAN_POINT('Ctrl Pts',(5.53738214999995,11.6,-8.91613481900002));
#164784=CARTESIAN_POINT('Ctrl Pts',(5.53675225199994,15.2,-8.91456634100001));
#164785=CARTESIAN_POINT('Ctrl Pts',(5.53675225199994,11.6,-8.91456634100001));
#164786=CARTESIAN_POINT('Ctrl Pts',(5.53612376599995,15.2,-8.91300558400001));
#164787=CARTESIAN_POINT('Ctrl Pts',(5.53612376599995,11.6,-8.91300558400001));
#164788=CARTESIAN_POINT('Ctrl Pts',(5.53549670999995,15.2,-8.91145255800001));
#164789=CARTESIAN_POINT('Ctrl Pts',(5.53549670999995,11.6,-8.91145255800001));
#164790=CARTESIAN_POINT('Ctrl Pts',(5.53487110399995,15.2,-8.90990727500002));
#164791=CARTESIAN_POINT('Ctrl Pts',(5.53487110399995,11.6,-8.90990727500002));
#164792=CARTESIAN_POINT('Ctrl Pts',(5.53424696599994,15.2,-8.90836974500001));
#164793=CARTESIAN_POINT('Ctrl Pts',(5.53424696599994,11.6,-8.90836974500001));
#164794=CARTESIAN_POINT('Ctrl Pts',(5.53362431699994,15.2,-8.90683998300002));
#164795=CARTESIAN_POINT('Ctrl Pts',(5.53362431699994,11.6,-8.90683998300002));
#164796=CARTESIAN_POINT('Ctrl Pts',(5.53300317299994,15.2,-8.90531799900002));
#164797=CARTESIAN_POINT('Ctrl Pts',(5.53300317299994,11.6,-8.90531799900002));
#164798=CARTESIAN_POINT('Ctrl Pts',(5.53238355599994,15.2,-8.90380380500002));
#164799=CARTESIAN_POINT('Ctrl Pts',(5.53238355599994,11.6,-8.90380380500002));
#164800=CARTESIAN_POINT('Ctrl Pts',(5.53176548499994,15.2,-8.90229741300002));
#164801=CARTESIAN_POINT('Ctrl Pts',(5.53176548499994,11.6,-8.90229741300002));
#164802=CARTESIAN_POINT('Ctrl Pts',(5.53114897799994,15.2,-8.90079883600002));
#164803=CARTESIAN_POINT('Ctrl Pts',(5.53114897799994,11.6,-8.90079883600002));
#164804=CARTESIAN_POINT('Ctrl Pts',(5.53053405599995,15.2,-8.89930808400001));
#164805=CARTESIAN_POINT('Ctrl Pts',(5.53053405599995,11.6,-8.89930808400001));
#164806=CARTESIAN_POINT('Ctrl Pts',(5.52992073899994,15.2,-8.89782517100001));
#164807=CARTESIAN_POINT('Ctrl Pts',(5.52992073899994,11.6,-8.89782517100001));
#164808=CARTESIAN_POINT('Ctrl Pts',(5.52930904599994,15.2,-8.89635010900001));
#164809=CARTESIAN_POINT('Ctrl Pts',(5.52930904599994,11.6,-8.89635010900001));
#164810=CARTESIAN_POINT('Ctrl Pts',(5.52869899599994,15.2,-8.89488290900001));
#164811=CARTESIAN_POINT('Ctrl Pts',(5.52869899599994,11.6,-8.89488290900001));
#164812=CARTESIAN_POINT('Ctrl Pts',(5.52809060999994,15.2,-8.89342358300001));
#164813=CARTESIAN_POINT('Ctrl Pts',(5.52809060999994,11.6,-8.89342358300001));
#164814=CARTESIAN_POINT('Ctrl Pts',(5.52748390799994,15.2,-8.89197214500001));
#164815=CARTESIAN_POINT('Ctrl Pts',(5.52748390799994,11.6,-8.89197214500001));
#164816=CARTESIAN_POINT('Ctrl Pts',(5.52687890999994,15.2,-8.89052860700002));
#164817=CARTESIAN_POINT('Ctrl Pts',(5.52687890999994,11.6,-8.89052860700002));
#164818=CARTESIAN_POINT('Ctrl Pts',(5.52627563499994,15.2,-8.88909298000002));
#164819=CARTESIAN_POINT('Ctrl Pts',(5.52627563499994,11.6,-8.88909298000002));
#164820=CARTESIAN_POINT('Ctrl Pts',(5.52567410499995,15.2,-8.88766527600002));
#164821=CARTESIAN_POINT('Ctrl Pts',(5.52567410499995,11.6,-8.88766527600002));
#164822=CARTESIAN_POINT('Ctrl Pts',(5.52507433899994,15.2,-8.88624550900002));
#164823=CARTESIAN_POINT('Ctrl Pts',(5.52507433899994,11.6,-8.88624550900002));
#164824=CARTESIAN_POINT('Ctrl Pts',(5.52447635799994,15.2,-8.88483369000001));
#164825=CARTESIAN_POINT('Ctrl Pts',(5.52447635799994,11.6,-8.88483369000001));
#164826=CARTESIAN_POINT('Ctrl Pts',(5.52388018299995,15.2,-8.88342983300002));
#164827=CARTESIAN_POINT('Ctrl Pts',(5.52388018299995,11.6,-8.88342983300002));
#164828=CARTESIAN_POINT('Ctrl Pts',(5.52328583399994,15.2,-8.88203395000002));
#164829=CARTESIAN_POINT('Ctrl Pts',(5.52328583399994,11.6,-8.88203395000002));
#164830=CARTESIAN_POINT('Ctrl Pts',(5.52269333099994,15.2,-8.88064605200002));
#164831=CARTESIAN_POINT('Ctrl Pts',(5.52269333099994,11.6,-8.88064605200002));
#164832=CARTESIAN_POINT('Ctrl Pts',(5.52210269599994,15.2,-8.87926615300002));
#164833=CARTESIAN_POINT('Ctrl Pts',(5.52210269599994,11.6,-8.87926615300002));
#164834=CARTESIAN_POINT('Ctrl Pts',(5.52151394899995,15.2,-8.87789426600002));
#164835=CARTESIAN_POINT('Ctrl Pts',(5.52151394899995,11.6,-8.87789426600002));
#164836=CARTESIAN_POINT('Ctrl Pts',(5.52092711099994,15.2,-8.87653040200002));
#164837=CARTESIAN_POINT('Ctrl Pts',(5.52092711099994,11.6,-8.87653040200002));
#164838=CARTESIAN_POINT('Ctrl Pts',(5.52034220399994,15.2,-8.87517457500002));
#164839=CARTESIAN_POINT('Ctrl Pts',(5.52034220399994,11.6,-8.87517457500002));
#164840=CARTESIAN_POINT('Ctrl Pts',(5.51975924799994,15.2,-8.87382679700002));
#164841=CARTESIAN_POINT('Ctrl Pts',(5.51975924799994,11.6,-8.87382679700002));
#164842=CARTESIAN_POINT('Ctrl Pts',(5.51917826499994,15.2,-8.87248708200002));
#164843=CARTESIAN_POINT('Ctrl Pts',(5.51917826499994,11.6,-8.87248708200002));
#164844=CARTESIAN_POINT('Ctrl Pts',(5.51859927599994,15.2,-8.87115544200002));
#164845=CARTESIAN_POINT('Ctrl Pts',(5.51859927599994,11.6,-8.87115544200002));
#164846=CARTESIAN_POINT('Ctrl Pts',(5.51802230199995,15.2,-8.86983188900002));
#164847=CARTESIAN_POINT('Ctrl Pts',(5.51802230199995,11.6,-8.86983188900002));
#164848=CARTESIAN_POINT('Ctrl Pts',(5.51744736599994,15.2,-8.86851643800001));
#164849=CARTESIAN_POINT('Ctrl Pts',(5.51744736599994,11.6,-8.86851643800001));
#164850=CARTESIAN_POINT('Ctrl Pts',(5.51687448799995,15.2,-8.86720909900001));
#164851=CARTESIAN_POINT('Ctrl Pts',(5.51687448799995,11.6,-8.86720909900001));
#164852=CARTESIAN_POINT('Ctrl Pts',(5.51630369099994,15.2,-8.86590988700002));
#164853=CARTESIAN_POINT('Ctrl Pts',(5.51630369099994,11.6,-8.86590988700002));
#164854=CARTESIAN_POINT('Ctrl Pts',(5.51573499599994,15.2,-8.86461881500002));
#164855=CARTESIAN_POINT('Ctrl Pts',(5.51573499599994,11.6,-8.86461881500002));
#164856=CARTESIAN_POINT('Ctrl Pts',(5.51516842399995,15.2,-8.86333589600002));
#164857=CARTESIAN_POINT('Ctrl Pts',(5.51516842399995,11.6,-8.86333589600002));
#164858=CARTESIAN_POINT('Ctrl Pts',(5.51460399899995,15.2,-8.86206114100002));
#164859=CARTESIAN_POINT('Ctrl Pts',(5.51460399899995,11.6,-8.86206114100002));
#164860=CARTESIAN_POINT('Ctrl Pts',(5.51404174199994,15.2,-8.86079456700001));
#164861=CARTESIAN_POINT('Ctrl Pts',(5.51404174199994,11.6,-8.86079456700001));
#164862=CARTESIAN_POINT('Ctrl Pts',(5.51348167599994,15.2,-8.85953618500002));
#164863=CARTESIAN_POINT('Ctrl Pts',(5.51348167599994,11.6,-8.85953618500002));
#164864=CARTESIAN_POINT('Ctrl Pts',(5.51292382199994,15.2,-8.85828600700002));
#164865=CARTESIAN_POINT('Ctrl Pts',(5.51292382199994,11.6,-8.85828600700002));
#164866=CARTESIAN_POINT('Ctrl Pts',(5.51236820399994,15.2,-8.85704404900002));
#164867=CARTESIAN_POINT('Ctrl Pts',(5.51236820399994,11.6,-8.85704404900002));
#164868=CARTESIAN_POINT('Ctrl Pts',(5.51181484299994,15.2,-8.85581032200001));
#164869=CARTESIAN_POINT('Ctrl Pts',(5.51181484299994,11.6,-8.85581032200001));
#164870=CARTESIAN_POINT('Ctrl Pts',(5.51126376199995,15.2,-8.85458484100001));
#164871=CARTESIAN_POINT('Ctrl Pts',(5.51126376199995,11.6,-8.85458484100001));
#164872=CARTESIAN_POINT('Ctrl Pts',(5.51071498499994,15.2,-8.85336761800002));
#164873=CARTESIAN_POINT('Ctrl Pts',(5.51071498499994,11.6,-8.85336761800002));
#164874=CARTESIAN_POINT('Ctrl Pts',(5.51016853299994,15.2,-8.85215866800002));
#164875=CARTESIAN_POINT('Ctrl Pts',(5.51016853299994,11.6,-8.85215866800002));
#164876=CARTESIAN_POINT('Ctrl Pts',(5.50962442999994,15.2,-8.85095800400002));
#164877=CARTESIAN_POINT('Ctrl Pts',(5.50962442999994,11.6,-8.85095800400002));
#164878=CARTESIAN_POINT('Ctrl Pts',(5.50908269899995,15.2,-8.84976563800001));
#164879=CARTESIAN_POINT('Ctrl Pts',(5.50908269899995,11.6,-8.84976563800001));
#164880=CARTESIAN_POINT('Ctrl Pts',(5.50854336299994,15.2,-8.84858158600002));
#164881=CARTESIAN_POINT('Ctrl Pts',(5.50854336299994,11.6,-8.84858158600002));
#164882=CARTESIAN_POINT('Ctrl Pts',(5.50800644599994,15.2,-8.84740586100002));
#164883=CARTESIAN_POINT('Ctrl Pts',(5.50800644599994,11.6,-8.84740586100002));
#164884=CARTESIAN_POINT('Ctrl Pts',(5.50747196999994,15.2,-8.84623847500002));
#164885=CARTESIAN_POINT('Ctrl Pts',(5.50747196999994,11.6,-8.84623847500002));
#164886=CARTESIAN_POINT('Ctrl Pts',(5.50693995899994,15.2,-8.84507944500001));
#164887=CARTESIAN_POINT('Ctrl Pts',(5.50693995899994,11.6,-8.84507944500001));
#164888=CARTESIAN_POINT('Ctrl Pts',(5.50641043699994,15.2,-8.84392878200002));
#164889=CARTESIAN_POINT('Ctrl Pts',(5.50641043699994,11.6,-8.84392878200002));
#164890=CARTESIAN_POINT('Ctrl Pts',(5.50588342799994,15.2,-8.84278649900001));
#164891=CARTESIAN_POINT('Ctrl Pts',(5.50588342799994,11.6,-8.84278649900001));
#164892=CARTESIAN_POINT('Ctrl Pts',(5.50535895399995,15.2,-8.84165261300002));
#164893=CARTESIAN_POINT('Ctrl Pts',(5.50535895399995,11.6,-8.84165261300002));
#164894=CARTESIAN_POINT('Ctrl Pts',(5.50483704099994,15.2,-8.84052713600001));
#164895=CARTESIAN_POINT('Ctrl Pts',(5.50483704099994,11.6,-8.84052713600001));
#164896=CARTESIAN_POINT('Ctrl Pts',(5.50431771199994,15.2,-8.83941008400001));
#164897=CARTESIAN_POINT('Ctrl Pts',(5.50431771199994,11.6,-8.83941008400001));
#164898=CARTESIAN_POINT('Ctrl Pts',(5.50380099099995,15.2,-8.83830146800002));
#164899=CARTESIAN_POINT('Ctrl Pts',(5.50380099099995,11.6,-8.83830146800002));
#164900=CARTESIAN_POINT('Ctrl Pts',(5.50328690399994,15.2,-8.83720130400001));
#164901=CARTESIAN_POINT('Ctrl Pts',(5.50328690399994,11.6,-8.83720130400001));
#164902=CARTESIAN_POINT('Ctrl Pts',(5.50277547299994,15.2,-8.83610960600001));
#164903=CARTESIAN_POINT('Ctrl Pts',(5.50277547299994,11.6,-8.83610960600001));
#164904=CARTESIAN_POINT('Ctrl Pts',(5.50226672399994,15.2,-8.83502638900002));
#164905=CARTESIAN_POINT('Ctrl Pts',(5.50226672399994,11.6,-8.83502638900002));
#164906=CARTESIAN_POINT('Ctrl Pts',(5.50176068099995,15.2,-8.83395166600002));
#164907=CARTESIAN_POINT('Ctrl Pts',(5.50176068099995,11.6,-8.83395166600002));
#164908=CARTESIAN_POINT('Ctrl Pts',(5.50125736899994,15.2,-8.83288545100001));
#164909=CARTESIAN_POINT('Ctrl Pts',(5.50125736899994,11.6,-8.83288545100001));
#164910=CARTESIAN_POINT('Ctrl Pts',(5.50075681299995,15.2,-8.83182776000002));
#164911=CARTESIAN_POINT('Ctrl Pts',(5.50075681299995,11.6,-8.83182776000002));
#164912=CARTESIAN_POINT('Ctrl Pts',(5.50025903799994,15.2,-8.83077860500002));
#164913=CARTESIAN_POINT('Ctrl Pts',(5.50025903799994,11.6,-8.83077860500002));
#164914=CARTESIAN_POINT('Ctrl Pts',(5.49976406799994,15.2,-8.82973800300002));
#164915=CARTESIAN_POINT('Ctrl Pts',(5.49976406799994,11.6,-8.82973800300002));
#164916=CARTESIAN_POINT('Ctrl Pts',(5.49927192999994,15.2,-8.82870596800002));
#164917=CARTESIAN_POINT('Ctrl Pts',(5.49927192999994,11.6,-8.82870596800002));
#164918=CARTESIAN_POINT('Ctrl Pts',(5.49878264899994,15.2,-8.82768251300002));
#164919=CARTESIAN_POINT('Ctrl Pts',(5.49878264899994,11.6,-8.82768251300002));
#164920=CARTESIAN_POINT('Ctrl Pts',(5.49829624999994,15.2,-8.82666765400002));
#164921=CARTESIAN_POINT('Ctrl Pts',(5.49829624999994,11.6,-8.82666765400002));
#164922=CARTESIAN_POINT('Ctrl Pts',(5.49781275699995,15.2,-8.82566140400002));
#164923=CARTESIAN_POINT('Ctrl Pts',(5.49781275699995,11.6,-8.82566140400002));
#164924=CARTESIAN_POINT('Ctrl Pts',(5.49733219899994,15.2,-8.82466378100002));
#164925=CARTESIAN_POINT('Ctrl Pts',(5.49733219899994,11.6,-8.82466378100002));
#164926=CARTESIAN_POINT('Ctrl Pts',(5.49685459999994,15.2,-8.82367479800001));
#164927=CARTESIAN_POINT('Ctrl Pts',(5.49685459999994,11.6,-8.82367479800001));
#164928=CARTESIAN_POINT('Ctrl Pts',(5.49637998599994,15.2,-8.82269446900001));
#164929=CARTESIAN_POINT('Ctrl Pts',(5.49637998599994,11.6,-8.82269446900001));
#164930=CARTESIAN_POINT('Ctrl Pts',(5.49590838399994,15.2,-8.82172281000001));
#164931=CARTESIAN_POINT('Ctrl Pts',(5.49590838399994,11.6,-8.82172281000001));
#164932=CARTESIAN_POINT('Ctrl Pts',(5.49543981999994,15.2,-8.82075983600001));
#164933=CARTESIAN_POINT('Ctrl Pts',(5.49543981999994,11.6,-8.82075983600001));
#164934=CARTESIAN_POINT('Ctrl Pts',(5.49497431799994,15.2,-8.81980556200002));
#164935=CARTESIAN_POINT('Ctrl Pts',(5.49497431799994,11.6,-8.81980556200002));
#164936=CARTESIAN_POINT('Ctrl Pts',(5.49451190799994,15.2,-8.81886000300002));
#164937=CARTESIAN_POINT('Ctrl Pts',(5.49451190799994,11.6,-8.81886000300002));
#164938=CARTESIAN_POINT('Ctrl Pts',(5.49405261599994,15.2,-8.81792317300001));
#164939=CARTESIAN_POINT('Ctrl Pts',(5.49405261599994,11.6,-8.81792317300001));
#164940=CARTESIAN_POINT('Ctrl Pts',(5.49359646699994,15.2,-8.81699508900001));
#164941=CARTESIAN_POINT('Ctrl Pts',(5.49359646699994,11.6,-8.81699508900001));
#164942=CARTESIAN_POINT('Ctrl Pts',(5.49314348999994,15.2,-8.81607576600001));
#164943=CARTESIAN_POINT('Ctrl Pts',(5.49314348999994,11.6,-8.81607576600001));
#164944=CARTESIAN_POINT('Ctrl Pts',(5.49269370999994,15.2,-8.81516521800001));
#164945=CARTESIAN_POINT('Ctrl Pts',(5.49269370999994,11.6,-8.81516521800001));
#164946=CARTESIAN_POINT('Ctrl Pts',(5.49224715599994,15.2,-8.81426346200002));
#164947=CARTESIAN_POINT('Ctrl Pts',(5.49224715599994,11.6,-8.81426346200002));
#164948=CARTESIAN_POINT('Ctrl Pts',(5.49180385399994,15.2,-8.81337051400001));
#164949=CARTESIAN_POINT('Ctrl Pts',(5.49180385399994,11.6,-8.81337051400001));
#164950=CARTESIAN_POINT('Ctrl Pts',(5.49136383199994,15.2,-8.81248638700002));
#164951=CARTESIAN_POINT('Ctrl Pts',(5.49136383199994,11.6,-8.81248638700002));
#164952=CARTESIAN_POINT('Ctrl Pts',(5.49092711899994,15.2,-8.81161109800002));
#164953=CARTESIAN_POINT('Ctrl Pts',(5.49092711899994,11.6,-8.81161109800002));
#164954=CARTESIAN_POINT('Ctrl Pts',(5.49049374099994,15.2,-8.81074466400002));
#164955=CARTESIAN_POINT('Ctrl Pts',(5.49049374099994,11.6,-8.81074466400002));
#164956=CARTESIAN_POINT('Ctrl Pts',(5.49006372599994,15.2,-8.80988709800001));
#164957=CARTESIAN_POINT('Ctrl Pts',(5.49006372599994,11.6,-8.80988709800001));
#164958=CARTESIAN_POINT('Ctrl Pts',(5.48963710299994,15.2,-8.80903841800002));
#164959=CARTESIAN_POINT('Ctrl Pts',(5.48963710299994,11.6,-8.80903841800002));
#164960=CARTESIAN_POINT('Ctrl Pts',(5.48921389899995,15.2,-8.80819864000001));
#164961=CARTESIAN_POINT('Ctrl Pts',(5.48921389899995,11.6,-8.80819864000001));
#164962=CARTESIAN_POINT('Ctrl Pts',(5.48879414499994,15.2,-8.80736777800001));
#164963=CARTESIAN_POINT('Ctrl Pts',(5.48879414499994,11.6,-8.80736777800001));
#164964=CARTESIAN_POINT('Ctrl Pts',(5.48838026299994,15.2,-8.80655058300002));
#164965=CARTESIAN_POINT('Ctrl Pts',(5.48838026299994,11.6,-8.80655058300002));
#164966=CARTESIAN_POINT('Ctrl Pts',(5.48805240199994,15.2,-8.80590483000002));
#164967=CARTESIAN_POINT('Ctrl Pts',(5.48805240199994,11.6,-8.80590483000002));
#164968=CARTESIAN_POINT('Ctrl Pts',(5.48780866099994,15.2,-8.80542564300002));
#164969=CARTESIAN_POINT('Ctrl Pts',(5.48780866099994,11.6,-8.80542564300002));
#164970=CARTESIAN_POINT('Ctrl Pts',(5.48764764299994,15.2,-8.80510947800002));
#164971=CARTESIAN_POINT('Ctrl Pts',(5.48764764299994,11.6,-8.80510947800002));
#164972=CARTESIAN_POINT('Ctrl Pts',(5.48756847899995,15.2,-8.80495412800002));
#164973=CARTESIAN_POINT('Ctrl Pts',(5.48756847899995,11.6,-8.80495412800002));
#164974=CARTESIAN_POINT('',(5.48756847908246,12.2,-8.80495412746575));
#164975=CARTESIAN_POINT('',(5.48756847908246,15.2,-8.80495412746575));
#164976=CARTESIAN_POINT('',(5.48756847899995,12.2,-8.80495412700002));
#164977=CARTESIAN_POINT('Ctrl Pts',(5.75020264099994,12.2,-9.95917514500001));
#164978=CARTESIAN_POINT('Ctrl Pts',(5.74993549095141,12.2,-9.95536156930721));
#164979=CARTESIAN_POINT('Ctrl Pts',(5.74966449014381,12.2,-9.95155489458726));
#164980=CARTESIAN_POINT('Ctrl Pts',(5.74938964875891,12.2,-9.94775512191045));
#164981=CARTESIAN_POINT('Ctrl Pts',(5.74911480737401,12.2,-9.94395534923364));
#164982=CARTESIAN_POINT('Ctrl Pts',(5.748836121958,12.2,-9.94016247888491));
#164983=CARTESIAN_POINT('Ctrl Pts',(5.74855360478793,12.2,-9.93637652429085));
#164984=CARTESIAN_POINT('Ctrl Pts',(5.74817691519361,12.2,-9.93132858437359));
#164985=CARTESIAN_POINT('Ctrl Pts',(5.74779341201749,12.2,-9.92629293960405));
#164986=CARTESIAN_POINT('Ctrl Pts',(5.747403168218,12.2,-9.9212696688311));
#164987=CARTESIAN_POINT('Ctrl Pts',(5.74711048539497,12.2,-9.91750221609359));
#164988=CARTESIAN_POINT('Ctrl Pts',(5.7468140126724,12.2,-9.91374172466357));
#164989=CARTESIAN_POINT('Ctrl Pts',(5.74651378172497,12.2,-9.90998822975829));
#164990=CARTESIAN_POINT('Ctrl Pts',(5.74611347375871,12.2,-9.90498356943));
#164991=CARTESIAN_POINT('Ctrl Pts',(5.74570648514168,12.2,-9.89999134467815));
#164992=CARTESIAN_POINT('Ctrl Pts',(5.74529287317401,12.2,-9.89501162118579));
#164993=CARTESIAN_POINT('Ctrl Pts',(5.74498266422643,12.2,-9.89127682890576));
#164994=CARTESIAN_POINT('Ctrl Pts',(5.74466873069324,12.2,-9.88754906896338));
#164995=CARTESIAN_POINT('Ctrl Pts',(5.74435109968848,12.2,-9.8838283690385));
#164996=CARTESIAN_POINT('Ctrl Pts',(5.74403346868372,12.2,-9.88010766911362));
#164997=CARTESIAN_POINT('Ctrl Pts',(5.74371213961966,12.2,-9.87639403032744));
#164998=CARTESIAN_POINT('Ctrl Pts',(5.74338714271448,12.2,-9.87268748404606));
#164999=CARTESIAN_POINT('Ctrl Pts',(5.7430621458093,12.2,-9.86898093776469));
#165000=CARTESIAN_POINT('Ctrl Pts',(5.74273348185456,12.2,-9.86528148464913));
#165001=CARTESIAN_POINT('Ctrl Pts',(5.74240117749164,12.2,-9.86158915378329));
#165002=CARTESIAN_POINT('Ctrl Pts',(5.74206887312871,12.2,-9.85789682291745));
#165003=CARTESIAN_POINT('Ctrl Pts',(5.74173293017427,12.2,-9.85421161373463));
#165004=CARTESIAN_POINT('Ctrl Pts',(5.74139337527026,12.2,-9.85053355740933));
#165005=CARTESIAN_POINT('Ctrl Pts',(5.74105382036624,12.2,-9.84685550108403));
#165006=CARTESIAN_POINT('Ctrl Pts',(5.74071065452133,12.2,-9.84318459710962));
#165007=CARTESIAN_POINT('Ctrl Pts',(5.74036390605869,12.2,-9.83952087472554));
#165008=CARTESIAN_POINT('Ctrl Pts',(5.74001715759605,12.2,-9.83585715234146));
#165009=CARTESIAN_POINT('Ctrl Pts',(5.73966682674711,12.2,-9.83220061396391));
#165010=CARTESIAN_POINT('Ctrl Pts',(5.73931294284378,12.2,-9.82855128680386));
#165011=CARTESIAN_POINT('Ctrl Pts',(5.73895905887616,12.2,-9.82490195898085));
#165012=CARTESIAN_POINT('Ctrl Pts',(5.73860162262422,12.2,-9.82125984485151));
#165013=CARTESIAN_POINT('Ctrl Pts',(5.73824066165461,12.2,-9.81762497344923));
#165014=CARTESIAN_POINT('Ctrl Pts',(5.73787970075058,12.2,-9.81399010270727));
#165015=CARTESIAN_POINT('Ctrl Pts',(5.73751521619673,12.2,-9.81036247540663));
#165016=CARTESIAN_POINT('Ctrl Pts',(5.73714723725147,12.2,-9.80674212208046));
#165017=CARTESIAN_POINT('Ctrl Pts',(5.73677925830621,12.2,-9.8031217687543));
#165018=CARTESIAN_POINT('Ctrl Pts',(5.73640778463773,12.2,-9.79950868903204));
#165019=CARTESIAN_POINT('Ctrl Pts',(5.73603284673296,12.2,-9.79590291327169));
#165020=CARTESIAN_POINT('Ctrl Pts',(5.73565790882819,12.2,-9.79229713751133));
#165021=CARTESIAN_POINT('Ctrl Pts',(5.73527950715483,12.2,-9.7886986664391));
#165022=CARTESIAN_POINT('Ctrl Pts',(5.73489767029198,12.2,-9.78510752971989));
#165023=CARTESIAN_POINT('Ctrl Pts',(5.73451583342913,12.2,-9.78151639300068));
#165024=CARTESIAN_POINT('Ctrl Pts',(5.73413056262785,12.2,-9.77793259222727));
#165025=CARTESIAN_POINT('Ctrl Pts',(5.73374188676728,12.2,-9.77435615689825));
#165026=CARTESIAN_POINT('Ctrl Pts',(5.73322365223943,12.2,-9.76958757602641));
#165027=CARTESIAN_POINT('Ctrl Pts',(5.73269936597196,12.2,-9.76483208952835));
#165028=CARTESIAN_POINT('Ctrl Pts',(5.7321691006649,12.2,-9.76008977010407));
#165029=CARTESIAN_POINT('Ctrl Pts',(5.73177140172072,12.2,-9.75653303085893));
#165030=CARTESIAN_POINT('Ctrl Pts',(5.73137033871861,12.2,-9.75298369825459));
#165031=CARTESIAN_POINT('Ctrl Pts',(5.7309659437333,12.2,-9.74944180396662));
#165032=CARTESIAN_POINT('Ctrl Pts',(5.73056154874799,12.2,-9.74589990967865));
#165033=CARTESIAN_POINT('Ctrl Pts',(5.7301538203795,12.2,-9.74236545357371));
#165034=CARTESIAN_POINT('Ctrl Pts',(5.72974279001971,12.2,-9.73883846536786));
#165035=CARTESIAN_POINT('Ctrl Pts',(5.72933175965994,12.2,-9.73531147716201));
#165036=CARTESIAN_POINT('Ctrl Pts',(5.72891742873604,12.2,-9.73179195886157));
#165037=CARTESIAN_POINT('Ctrl Pts',(5.72849982685573,12.2,-9.72827993989619));
#165038=CARTESIAN_POINT('Ctrl Pts',(5.72808222497542,12.2,-9.7247679209308));
#165039=CARTESIAN_POINT('Ctrl Pts',(5.72766135342657,12.2,-9.72126340180294));
#165040=CARTESIAN_POINT('Ctrl Pts',(5.72723724210909,12.2,-9.71776641401231));
#165041=CARTESIAN_POINT('Ctrl Pts',(5.72681313071456,12.2,-9.71426942558641));
#165042=CARTESIAN_POINT('Ctrl Pts',(5.72638578060245,12.2,-9.71077996896257));
#165043=CARTESIAN_POINT('Ctrl Pts',(5.72595522362277,12.2,-9.70729807449925));
#165044=CARTESIAN_POINT('Ctrl Pts',(5.72552466672131,12.2,-9.70381618066846));
#165045=CARTESIAN_POINT('Ctrl Pts',(5.72509090265336,12.2,-9.70034184847893));
#165046=CARTESIAN_POINT('Ctrl Pts',(5.72465396371062,12.2,-9.69687511114721));
#165047=CARTESIAN_POINT('Ctrl Pts',(5.72421702476789,12.2,-9.6934083738155));
#165048=CARTESIAN_POINT('Ctrl Pts',(5.72377691046882,12.2,-9.68994923025373));
#165049=CARTESIAN_POINT('Ctrl Pts',(5.72333365402456,12.2,-9.6864977119885));
#165050=CARTESIAN_POINT('Ctrl Pts',(5.72289039758031,12.2,-9.68304619372326));
#165051=CARTESIAN_POINT('Ctrl Pts',(5.7224439979194,12.2,-9.67960230077719));
#165052=CARTESIAN_POINT('Ctrl Pts',(5.72199448851704,12.2,-9.67616606546975));
#165053=CARTESIAN_POINT('Ctrl Pts',(5.72154497911468,12.2,-9.67272983016231));
#165054=CARTESIAN_POINT('Ctrl Pts',(5.72109235938276,12.2,-9.66930125219935));
#165055=CARTESIAN_POINT('Ctrl Pts',(5.72063666206625,12.2,-9.66588036286464));
#165056=CARTESIAN_POINT('Ctrl Pts',(5.72018096474975,12.2,-9.66245947352993));
#165057=CARTESIAN_POINT('Ctrl Pts',(5.71972219096677,12.2,-9.65904627233633));
#165058=CARTESIAN_POINT('Ctrl Pts',(5.71926037260897,12.2,-9.6556407925007));
#165059=CARTESIAN_POINT('Ctrl Pts',(5.71879855416727,12.2,-9.6522353120464));
#165060=CARTESIAN_POINT('Ctrl Pts',(5.7183336908497,12.2,-9.64883755190257));
#165061=CARTESIAN_POINT('Ctrl Pts',(5.71786581736463,12.2,-9.64544754449428));
#165062=CARTESIAN_POINT('Ctrl Pts',(5.71739794396455,12.2,-9.64205753770183));
#165063=CARTESIAN_POINT('Ctrl Pts',(5.71692705951506,12.2,-9.63867528334222));
#165064=CARTESIAN_POINT('Ctrl Pts',(5.71645319767492,12.2,-9.63530081383882));
#165065=CARTESIAN_POINT('Ctrl Pts',(5.71597933583479,12.2,-9.63192634433543));
#165066=CARTESIAN_POINT('Ctrl Pts',(5.71550249743045,12.2,-9.62855965891125));
#165067=CARTESIAN_POINT('Ctrl Pts',(5.71502271465595,12.2,-9.62520079061731));
#165068=CARTESIAN_POINT('Ctrl Pts',(5.71454293188147,12.2,-9.62184192232337));
#165069=CARTESIAN_POINT('Ctrl Pts',(5.71406020613232,12.2,-9.61849087154515));
#165070=CARTESIAN_POINT('Ctrl Pts',(5.7135745712333,12.2,-9.61514766879162));
#165071=CARTESIAN_POINT('Ctrl Pts',(5.71308893633428,12.2,-9.61180446603809));
#165072=CARTESIAN_POINT('Ctrl Pts',(5.71260039151871,12.2,-9.60846911215924));
#165073=CARTESIAN_POINT('Ctrl Pts',(5.71210897303681,12.2,-9.60514163986278));
#165074=CARTESIAN_POINT('Ctrl Pts',(5.71161755455492,12.2,-9.60181416756632));
#165075=CARTESIAN_POINT('Ctrl Pts',(5.71112326031923,12.2,-9.59849457665347));
#165076=CARTESIAN_POINT('Ctrl Pts',(5.71062612639612,12.2,-9.59518289919077));
#165077=CARTESIAN_POINT('Ctrl Pts',(5.71012899247301,12.2,-9.59187122172807));
#165078=CARTESIAN_POINT('Ctrl Pts',(5.70962901765759,12.2,-9.58856745801645));
#165079=CARTESIAN_POINT('Ctrl Pts',(5.7091262388429,12.2,-9.58527164076012));
#165080=CARTESIAN_POINT('Ctrl Pts',(5.7084558670291,12.2,-9.58087721735253));
#165081=CARTESIAN_POINT('Ctrl Pts',(5.70778050840926,12.2,-9.57649692019346));
#165082=CARTESIAN_POINT('Ctrl Pts',(5.7071002464833,12.2,-9.57213082739995));
#165083=CARTESIAN_POINT('Ctrl Pts',(5.70641998455734,12.2,-9.56776473460644));
#165084=CARTESIAN_POINT('Ctrl Pts',(5.70573481950302,12.2,-9.56341284618682));
#165085=CARTESIAN_POINT('Ctrl Pts',(5.70504483635381,12.2,-9.55907523950742));
#165086=CARTESIAN_POINT('Ctrl Pts',(5.70418235755832,12.2,-9.55365323204467));
#165087=CARTESIAN_POINT('Ctrl Pts',(5.70331234901849,12.2,-9.54825353962462));
#165088=CARTESIAN_POINT('Ctrl Pts',(5.70243498015639,12.2,-9.54287631694498));
#165089=CARTESIAN_POINT('Ctrl Pts',(5.70173308495194,12.2,-9.53857453809792));
#165090=CARTESIAN_POINT('Ctrl Pts',(5.70102647892484,12.2,-9.53428713773839));
#165091=CARTESIAN_POINT('Ctrl Pts',(5.70031524727496,12.2,-9.53001419628329));
#165092=CARTESIAN_POINT('Ctrl Pts',(5.69960401562509,12.2,-9.52574125482819));
#165093=CARTESIAN_POINT('Ctrl Pts',(5.69888816083579,12.2,-9.521482772297));
#165094=CARTESIAN_POINT('Ctrl Pts',(5.69816776840717,12.2,-9.51723882628941));
#165095=CARTESIAN_POINT('Ctrl Pts',(5.69744737607672,12.2,-9.51299488086007));
#165096=CARTESIAN_POINT('Ctrl Pts',(5.69672244777469,12.2,-9.50876547254694));
#165097=CARTESIAN_POINT('Ctrl Pts',(5.69599307077546,12.2,-9.50455068226116));
#165098=CARTESIAN_POINT('Ctrl Pts',(5.69526369367684,12.2,-9.50033589140112));
#165099=CARTESIAN_POINT('Ctrl Pts',(5.69452986885327,12.2,-9.49613571580055));
#165100=CARTESIAN_POINT('Ctrl Pts',(5.6937916858126,12.2,-9.49195023707397));
#165101=CARTESIAN_POINT('Ctrl Pts',(5.6930535028725,12.2,-9.48776475891764));
#165102=CARTESIAN_POINT('Ctrl Pts',(5.69231096271908,12.2,-9.48359397742607));
#165103=CARTESIAN_POINT('Ctrl Pts',(5.69156415383597,12.2,-9.47943797259818));
#165104=CARTESIAN_POINT('Ctrl Pts',(5.69081734485111,12.2,-9.47528196720405));
#165105=CARTESIAN_POINT('Ctrl Pts',(5.69006626980294,12.2,-9.47114073837547));
#165106=CARTESIAN_POINT('Ctrl Pts',(5.68931101739035,12.2,-9.46701436616794));
#165107=CARTESIAN_POINT('Ctrl Pts',(5.68855576508067,12.2,-9.46288799452263));
#165108=CARTESIAN_POINT('Ctrl Pts',(5.68779633758298,12.2,-9.45877648133163));
#165109=CARTESIAN_POINT('Ctrl Pts',(5.68703282731234,12.2,-9.45467990461));
#165110=CARTESIAN_POINT('Ctrl Pts',(5.68626931693766,12.2,-9.45058332733022));
#165111=CARTESIAN_POINT('Ctrl Pts',(5.68550172393193,12.2,-9.44650168901607));
#165112=CARTESIAN_POINT('Ctrl Pts',(5.68473014094518,12.2,-9.44243506968432));
#165113=CARTESIAN_POINT('Ctrl Pts',(5.68395855806355,12.2,-9.43836845090665));
#165114=CARTESIAN_POINT('Ctrl Pts',(5.68318298680181,12.2,-9.43431685210317));
#165115=CARTESIAN_POINT('Ctrl Pts',(5.68240352110471,12.2,-9.4302803531191));
#165116=CARTESIAN_POINT('Ctrl Pts',(5.68142918890369,12.2,-9.42523472897653));
#165117=CARTESIAN_POINT('Ctrl Pts',(5.68044877128079,12.2,-9.4202127011227));
#165118=CARTESIAN_POINT('Ctrl Pts',(5.6794624575311,12.2,-9.41521442959366));
#165119=CARTESIAN_POINT('Ctrl Pts',(5.67867340648834,12.2,-9.41121581215252));
#165120=CARTESIAN_POINT('Ctrl Pts',(5.67788058069513,12.2,-9.40723239801877));
#165121=CARTESIAN_POINT('Ctrl Pts',(5.67708407898481,12.2,-9.40326427069237));
#165122=CARTESIAN_POINT('Ctrl Pts',(5.67628757738301,12.2,-9.39929614390663));
#165123=CARTESIAN_POINT('Ctrl Pts',(5.6754873989153,12.2,-9.39534330348174));
#165124=CARTESIAN_POINT('Ctrl Pts',(5.67468364264804,12.2,-9.39140583263541));
#165125=CARTESIAN_POINT('Ctrl Pts',(5.67387988627127,12.2,-9.38746836125259));
#165126=CARTESIAN_POINT('Ctrl Pts',(5.67307255126396,12.2,-9.38354625975568));
#165127=CARTESIAN_POINT('Ctrl Pts',(5.67226173821607,12.2,-9.37963961174729));
#165128=CARTESIAN_POINT('Ctrl Pts',(5.67145092527866,12.2,-9.37573296427118));
#165129=CARTESIAN_POINT('Ctrl Pts',(5.67063663376646,12.2,-9.37184176999892));
#165130=CARTESIAN_POINT('Ctrl Pts',(5.66981896483365,12.2,-9.36796611259197));
#165131=CARTESIAN_POINT('Ctrl Pts',(5.66900129578943,12.2,-9.36409045465695));
#165132=CARTESIAN_POINT('Ctrl Pts',(5.66818025001711,12.2,-9.36023033455114));
#165133=CARTESIAN_POINT('Ctrl Pts',(5.66735592774996,12.2,-9.35638583650828));
#165134=CARTESIAN_POINT('Ctrl Pts',(5.66653160548281,12.2,-9.35254133846543));
#165135=CARTESIAN_POINT('Ctrl Pts',(5.66570400652639,12.2,-9.34871246181329));
#165136=CARTESIAN_POINT('Ctrl Pts',(5.66487323681413,12.2,-9.34489929188485));
#165137=CARTESIAN_POINT('Ctrl Pts',(5.66404246721504,12.2,-9.34108612247595));
#165138=CARTESIAN_POINT('Ctrl Pts',(5.66320852447201,12.2,-9.33728866048565));
#165139=CARTESIAN_POINT('Ctrl Pts',(5.66237151425886,12.2,-9.33350699027752));
#165140=CARTESIAN_POINT('Ctrl Pts',(5.66153450393166,12.2,-9.32972531955415));
#165141=CARTESIAN_POINT('Ctrl Pts',(5.66069442466114,12.2,-9.32595944014791));
#165142=CARTESIAN_POINT('Ctrl Pts',(5.65985138433712,12.2,-9.32220944011183));
#165143=CARTESIAN_POINT('Ctrl Pts',(5.65900834412796,12.2,-9.31845944058668));
#165144=CARTESIAN_POINT('Ctrl Pts',(5.65816234087474,12.2,-9.31472531863448));
#165145=CARTESIAN_POINT('Ctrl Pts',(5.65731348277766,12.2,-9.31100716127073));
#165146=CARTESIAN_POINT('Ctrl Pts',(5.65646462456492,12.2,-9.30728900340038));
#165147=CARTESIAN_POINT('Ctrl Pts',(5.65561291168768,12.2,-9.30358681077383));
#165148=CARTESIAN_POINT('Ctrl Pts',(5.65475845137595,12.2,-9.29990066922349));
#165149=CARTESIAN_POINT('Ctrl Pts',(5.65390399118066,12.2,-9.29621452817539));
#165150=CARTESIAN_POINT('Ctrl Pts',(5.65304678436365,12.2,-9.29254443822894));
#165151=CARTESIAN_POINT('Ctrl Pts',(5.65218693904522,12.2,-9.28889048808215));
#165152=CARTESIAN_POINT('Ctrl Pts',(5.65132709360964,12.2,-9.2852365374375));
#165153=CARTESIAN_POINT('Ctrl Pts',(5.65046461205152,12.2,-9.28159872526146));
#165154=CARTESIAN_POINT('Ctrl Pts',(5.64959960317088,12.2,-9.27797713995404));
#165155=CARTESIAN_POINT('Ctrl Pts',(5.64873459440811,12.2,-9.27435555514005));
#165156=CARTESIAN_POINT('Ctrl Pts',(5.64786705917053,12.2,-9.27075019752202));
#165157=CARTESIAN_POINT('Ctrl Pts',(5.64699710964284,12.2,-9.26716115524584));
#165158=CARTESIAN_POINT('Ctrl Pts',(5.64612715999663,12.2,-9.26357211248064));
#165159=CARTESIAN_POINT('Ctrl Pts',(5.6452547946818,12.2,-9.25999938506602));
#165160=CARTESIAN_POINT('Ctrl Pts',(5.64438013041176,12.2,-9.25644306248437));
#165161=CARTESIAN_POINT('Ctrl Pts',(5.64350546626089,12.2,-9.25288674038728));
#165162=CARTESIAN_POINT('Ctrl Pts',(5.64262850091326,12.2,-9.24934682233412));
#165163=CARTESIAN_POINT('Ctrl Pts',(5.64174935015203,12.2,-9.24582339884272));
#165164=CARTESIAN_POINT('Ctrl Pts',(5.64087019927102,12.2,-9.24229997487124));
#165165=CARTESIAN_POINT('Ctrl Pts',(5.63998886083485,12.2,-9.23879304451469));
#165166=CARTESIAN_POINT('Ctrl Pts',(5.63910545578269,12.2,-9.23530269919758));
#165167=CARTESIAN_POINT('Ctrl Pts',(5.63822205085089,12.2,-9.23181235435604));
#165168=CARTESIAN_POINT('Ctrl Pts',(5.63733657501396,12.2,-9.22833859259261));
#165169=CARTESIAN_POINT('Ctrl Pts',(5.63644914892005,12.2,-9.22488150704019));
#165170=CARTESIAN_POINT('Ctrl Pts',(5.63556172270521,12.2,-9.22142442101673));
#165171=CARTESIAN_POINT('Ctrl Pts',(5.63467234446241,12.2,-9.2179840087782));
#165172=CARTESIAN_POINT('Ctrl Pts',(5.63378113502495,12.2,-9.21456036475828));
#165173=CARTESIAN_POINT('Ctrl Pts',(5.63288992558749,12.2,-9.21113672073835));
#165174=CARTESIAN_POINT('Ctrl Pts',(5.63199688446648,12.2,-9.20772984107595));
#165175=CARTESIAN_POINT('Ctrl Pts',(5.63110213236199,12.2,-9.20433982117068));
#165176=CARTESIAN_POINT('Ctrl Pts',(5.63020738037941,12.2,-9.20094980172732));
#165177=CARTESIAN_POINT('Ctrl Pts',(5.62931091711177,12.2,-9.19757664075982));
#165178=CARTESIAN_POINT('Ctrl Pts',(5.62841286579223,12.2,-9.1942204300189));
#165179=CARTESIAN_POINT('Ctrl Pts',(5.62751481435033,12.2,-9.1908642188207));
#165180=CARTESIAN_POINT('Ctrl Pts',(5.62661517393243,12.2,-9.18752495868332));
#165181=CARTESIAN_POINT('Ctrl Pts',(5.62571406982762,12.2,-9.18420274344844));
#165182=CARTESIAN_POINT('Ctrl Pts',(5.62481296584558,12.2,-9.18088052866621));
#165183=CARTESIAN_POINT('Ctrl Pts',(5.62391039745263,12.2,-9.17757535724846));
#165184=CARTESIAN_POINT('Ctrl Pts',(5.62300648958216,12.2,-9.1742873237939));
#165185=CARTESIAN_POINT('Ctrl Pts',(5.62210258158854,12.2,-9.17099928989134));
#165186=CARTESIAN_POINT('Ctrl Pts',(5.62119733622986,12.2,-9.16772839441348));
#165187=CARTESIAN_POINT('Ctrl Pts',(5.62029087813507,12.2,-9.16447473101957));
#165188=CARTESIAN_POINT('Ctrl Pts',(5.6193844201638,12.2,-9.16122106806898));
#165189=CARTESIAN_POINT('Ctrl Pts',(5.61847675104986,12.2,-9.15798463650121));
#165190=CARTESIAN_POINT('Ctrl Pts',(5.6175679997909,12.2,-9.15476553376329));
#165191=CARTESIAN_POINT('Ctrl Pts',(5.61643206062433,12.2,-9.15074165501192));
#165192=CARTESIAN_POINT('Ctrl Pts',(5.61529442920214,12.2,-9.14674485083891));
#165193=CARTESIAN_POINT('Ctrl Pts',(5.6141553618411,12.2,-9.14277530722639));
#165194=CARTESIAN_POINT('Ctrl Pts',(5.61301629448007,12.2,-9.13880576361387));
#165195=CARTESIAN_POINT('Ctrl Pts',(5.61187579130575,12.2,-9.13486348257548));
#165196=CARTESIAN_POINT('Ctrl Pts',(5.6107341115089,12.2,-9.13094865200209));
#165197=CARTESIAN_POINT('Ctrl Pts',(5.60959243171206,12.2,-9.12703382142869));
#165198=CARTESIAN_POINT('Ctrl Pts',(5.60844957668883,12.2,-9.12314644026103));
#165199=CARTESIAN_POINT('Ctrl Pts',(5.60730580925828,12.2,-9.11928670227493));
#165200=CARTESIAN_POINT('Ctrl Pts',(5.60616204182773,12.2,-9.11542696428883));
#165201=CARTESIAN_POINT('Ctrl Pts',(5.60501736224439,12.2,-9.11159486614996));
#165202=CARTESIAN_POINT('Ctrl Pts',(5.60387203904995,12.2,-9.10779060323329));
#165203=CARTESIAN_POINT('Ctrl Pts',(5.60272671585551,12.2,-9.10398634031662));
#165204=CARTESIAN_POINT('Ctrl Pts',(5.60158074997676,12.2,-9.10020991180933));
#165205=CARTESIAN_POINT('Ctrl Pts',(5.60043441274932,12.2,-9.09646151151457));
#165206=CARTESIAN_POINT('Ctrl Pts',(5.59928807552188,12.2,-9.09271311121981));
#165207=CARTESIAN_POINT('Ctrl Pts',(5.59814136906938,12.2,-9.08899274026274));
#165208=CARTESIAN_POINT('Ctrl Pts',(5.59699456941661,12.2,-9.08530059325031));
#165209=CARTESIAN_POINT('Ctrl Pts',(5.59584776976382,12.2,-9.0816084462379));
#165210=CARTESIAN_POINT('Ctrl Pts',(5.59470087836385,12.2,-9.07794452493311));
#165211=CARTESIAN_POINT('Ctrl Pts',(5.59355417697495,12.2,-9.07430902625401));
#165212=CARTESIAN_POINT('Ctrl Pts',(5.59240747558606,12.2,-9.0706735275749));
#165213=CARTESIAN_POINT('Ctrl Pts',(5.59126096451302,12.2,-9.067066452667));
#165214=CARTESIAN_POINT('Ctrl Pts',(5.59011493140024,12.2,-9.06348800130964));
#165215=CARTESIAN_POINT('Ctrl Pts',(5.58896889828746,12.2,-9.05990954995228));
#165216=CARTESIAN_POINT('Ctrl Pts',(5.58782334446681,12.2,-9.05635972338149));
#165217=CARTESIAN_POINT('Ctrl Pts',(5.58667855988354,12.2,-9.05283872227274));
#165218=CARTESIAN_POINT('Ctrl Pts',(5.58553377530027,12.2,-9.04931772116399));
#165219=CARTESIAN_POINT('Ctrl Pts',(5.58438976336147,12.2,-9.04582554527794));
#165220=CARTESIAN_POINT('Ctrl Pts',(5.58324681808378,12.2,-9.04236240153031));
#165221=CARTESIAN_POINT('Ctrl Pts',(5.58210387293066,12.2,-9.03889925816016));
#165222=CARTESIAN_POINT('Ctrl Pts',(5.58096199755268,12.2,-9.03546514535989));
#165223=CARTESIAN_POINT('Ctrl Pts',(5.57982149385745,12.2,-9.03206026968698));
#165224=CARTESIAN_POINT('Ctrl Pts',(5.5786809900379,12.2,-9.02865539364294));
#165225=CARTESIAN_POINT('Ctrl Pts',(5.57754185839329,12.2,-9.02527975585112));
#165226=CARTESIAN_POINT('Ctrl Pts',(5.57640440790705,12.2,-9.02193356473764));
#165227=CARTESIAN_POINT('Ctrl Pts',(5.57526695742081,12.2,-9.01858737362414));
#165228=CARTESIAN_POINT('Ctrl Pts',(5.574131187305,12.2,-9.01527062885344));
#165229=CARTESIAN_POINT('Ctrl Pts',(5.5729974126649,12.2,-9.01198354188163));
#165230=CARTESIAN_POINT('Ctrl Pts',(5.57186363802479,12.2,-9.00869645490982));
#165231=CARTESIAN_POINT('Ctrl Pts',(5.57073185890172,12.2,-9.00543902751277));
#165232=CARTESIAN_POINT('Ctrl Pts',(5.56960239529048,12.2,-9.00221147146953));
#165233=CARTESIAN_POINT('Ctrl Pts',(5.56847293167925,12.2,-8.99898391542628));
#165234=CARTESIAN_POINT('Ctrl Pts',(5.56734578462364,12.2,-8.99578623151997));
#165235=CARTESIAN_POINT('Ctrl Pts',(5.56622127858183,12.2,-8.99261863624062));
#165236=CARTESIAN_POINT('Ctrl Pts',(5.5648718713807,12.2,-8.98881752204349));
#165237=CARTESIAN_POINT('Ctrl Pts',(5.56352627083102,12.2,-8.98505973376448));
#165238=CARTESIAN_POINT('Ctrl Pts',(5.56218504687946,12.2,-8.98134565264645));
#165239=CARTESIAN_POINT('Ctrl Pts',(5.56084382280607,12.2,-8.97763157119106));
#165240=CARTESIAN_POINT('Ctrl Pts',(5.55950698194974,12.2,-8.97396119534822));
#165241=CARTESIAN_POINT('Ctrl Pts',(5.5581751077107,12.2,-8.97033491081915));
#165242=CARTESIAN_POINT('Ctrl Pts',(5.55684323359264,12.2,-8.96670862661947));
#165243=CARTESIAN_POINT('Ctrl Pts',(5.55551632823354,12.2,-8.9631264309225));
#165244=CARTESIAN_POINT('Ctrl Pts',(5.55419499502554,12.2,-8.95958871770155));
#165245=CARTESIAN_POINT('Ctrl Pts',(5.55287366181754,12.2,-8.9560510044806));
#165246=CARTESIAN_POINT('Ctrl Pts',(5.55155789924552,12.2,-8.95255777049525));
#165247=CARTESIAN_POINT('Ctrl Pts',(5.55024832612601,12.2,-8.94910941436748));
#165248=CARTESIAN_POINT('Ctrl Pts',(5.54893875288755,12.2,-8.9456610579265));
#165249=CARTESIAN_POINT('Ctrl Pts',(5.54763536709289,12.2,-8.94225757884833));
#165250=CARTESIAN_POINT('Ctrl Pts',(5.54633880112452,12.2,-8.93889937741686));
#165251=CARTESIAN_POINT('Ctrl Pts',(5.54504223527394,12.2,-8.93554117629043));
#165252=CARTESIAN_POINT('Ctrl Pts',(5.54375249127834,12.2,-8.93222825632291));
#165253=CARTESIAN_POINT('Ctrl Pts',(5.5424702132416,12.2,-8.92896102252493));
#165254=CARTESIAN_POINT('Ctrl Pts',(5.54097422212106,12.2,-8.92514924956277));
#165255=CARTESIAN_POINT('Ctrl Pts',(5.5394883948182,12.2,-8.92139966416064));
#165256=CARTESIAN_POINT('Ctrl Pts',(5.53801378415268,12.2,-8.91771292589435));
#165257=CARTESIAN_POINT('Ctrl Pts',(5.53674983221926,12.2,-8.91455286468728));
#165258=CARTESIAN_POINT('Ctrl Pts',(5.53549412207964,12.2,-8.91143897676351));
#165259=CARTESIAN_POINT('Ctrl Pts',(5.53424733820826,12.2,-8.90837168695826));
#165260=CARTESIAN_POINT('Ctrl Pts',(5.53300055433687,12.2,-8.90530439715301));
#165261=CARTESIAN_POINT('Ctrl Pts',(5.53176269308149,12.2,-8.90228370678589));
#165262=CARTESIAN_POINT('Ctrl Pts',(5.53053445737548,12.2,-8.89931004405742));
#165263=CARTESIAN_POINT('Ctrl Pts',(5.52930622155789,12.2,-8.89633638105884));
#165264=CARTESIAN_POINT('Ctrl Pts',(5.52808761036701,12.2,-8.89340974786119));
#165265=CARTESIAN_POINT('Ctrl Pts',(5.52687934065807,12.2,-8.89053058447987));
#165266=CARTESIAN_POINT('Ctrl Pts',(5.52567107105887,12.2,-8.88765142136008));
#165267=CARTESIAN_POINT('Ctrl Pts',(5.52447314397346,12.2,-8.88481972509045));
#165268=CARTESIAN_POINT('Ctrl Pts',(5.52328629551659,12.2,-8.88203594627492));
#165269=CARTESIAN_POINT('Ctrl Pts',(5.52190163891169,12.2,-8.87878820415491));
#165270=CARTESIAN_POINT('Ctrl Pts',(5.52053206005894,12.2,-8.87560567919259));
#165271=CARTESIAN_POINT('Ctrl Pts',(5.51917876338774,12.2,-8.87248910049163));
#165272=CARTESIAN_POINT('Ctrl Pts',(5.51801879487263,12.2,-8.86981774745804));
#165273=CARTESIAN_POINT('Ctrl Pts',(5.51687078998367,12.2,-8.86719484213975));
#165274=CARTESIAN_POINT('Ctrl Pts',(5.51573552677492,12.2,-8.86462085323326));
#165275=CARTESIAN_POINT('Ctrl Pts',(5.51460026356616,12.2,-8.86204686432676));
#165276=CARTESIAN_POINT('Ctrl Pts',(5.51347774372312,12.2,-8.8595217898928));
#165277=CARTESIAN_POINT('Ctrl Pts',(5.5123687683739,12.2,-8.85704610702288));
#165278=CARTESIAN_POINT('Ctrl Pts',(5.51125979292394,12.2,-8.85457042392808));
#165279=CARTESIAN_POINT('Ctrl Pts',(5.51016436078168,12.2,-8.85214413192536));
#165280=CARTESIAN_POINT('Ctrl Pts',(5.50908329764042,12.2,-8.84976771621591));
#165281=CARTESIAN_POINT('Ctrl Pts',(5.50800223459734,12.2,-8.84739130072232));
#165282=CARTESIAN_POINT('Ctrl Pts',(5.50693554074929,12.2,-8.84506476471805));
#165283=CARTESIAN_POINT('Ctrl Pts',(5.50588406178277,12.2,-8.84278859820723));
#165284=CARTESIAN_POINT('Ctrl Pts',(5.50483258281625,12.2,-8.8405124316964));
#165285=CARTESIAN_POINT('Ctrl Pts',(5.5037963193359,12.2,-8.83828663894189));
#165286=CARTESIAN_POINT('Ctrl Pts',(5.50277614353892,12.2,-8.83611172635201));
#165287=CARTESIAN_POINT('Ctrl Pts',(5.50175596764927,12.2,-8.83393681356456));
#165288=CARTESIAN_POINT('Ctrl Pts',(5.50075187959496,12.2,-8.83181277937513));
#165289=CARTESIAN_POINT('Ctrl Pts',(5.49976477587566,12.2,-8.82974014451569));
#165290=CARTESIAN_POINT('Ctrl Pts',(5.49877767224603,12.2,-8.82766750984452));
#165291=CARTESIAN_POINT('Ctrl Pts',(5.49780755475439,12.2,-8.82564627083567));
#165292=CARTESIAN_POINT('Ctrl Pts',(5.49685534620643,12.2,-8.82367696140948));
#165293=CARTESIAN_POINT('Ctrl Pts',(5.49590313765847,12.2,-8.82170765198329));
#165294=CARTESIAN_POINT('Ctrl Pts',(5.49496883830079,12.2,-8.81979027085299));
#165295=CARTESIAN_POINT('Ctrl Pts',(5.49405340183321,12.2,-8.81792535958511));
#165296=CARTESIAN_POINT('Ctrl Pts',(5.49313796536564,12.2,-8.81606044831723));
#165297=CARTESIAN_POINT('Ctrl Pts',(5.49224138970664,12.2,-8.81424800979806));
#165298=CARTESIAN_POINT('Ctrl Pts',(5.49136465932048,12.2,-8.81248859669171));
#165299=CARTESIAN_POINT('Ctrl Pts',(5.49005377132756,12.2,-8.80985792077118));
#165300=CARTESIAN_POINT('Ctrl Pts',(5.48878723733333,12.2,-8.8073457972827));
#165301=CARTESIAN_POINT('Ctrl Pts',(5.48756847899995,12.2,-8.80495412800002));
#165302=CARTESIAN_POINT('Ctrl Pts',(5.48756847899995,15.2,-8.80495412800002));
#165303=CARTESIAN_POINT('Ctrl Pts',(5.48837968052293,15.2,-8.80654601517849));
#165304=CARTESIAN_POINT('Ctrl Pts',(5.48921205180367,15.2,-8.8081912649178));
#165305=CARTESIAN_POINT('Ctrl Pts',(5.49006457388987,15.2,-8.80988931929729));
#165306=CARTESIAN_POINT('Ctrl Pts',(5.49092120726851,15.2,-8.81159556255332));
#165307=CARTESIAN_POINT('Ctrl Pts',(5.49179818705027,15.2,-8.81335511472471));
#165308=CARTESIAN_POINT('Ctrl Pts',(5.49269451656167,15.2,-8.81516741616703));
#165309=CARTESIAN_POINT('Ctrl Pts',(5.49359084599165,15.2,-8.81697971744475));
#165310=CARTESIAN_POINT('Ctrl Pts',(5.49450652408385,15.2,-8.81884476556958));
#165311=CARTESIAN_POINT('Ctrl Pts',(5.49544058554991,15.2,-8.82076201099992));
#165312=CARTESIAN_POINT('Ctrl Pts',(5.49637464701597,15.2,-8.82267925643024));
#165313=CARTESIAN_POINT('Ctrl Pts',(5.49732708885225,15.2,-8.82464869965497));
#165314=CARTESIAN_POINT('Ctrl Pts',(5.4982969764478,15.2,-8.82666980609621));
#165315=CARTESIAN_POINT('Ctrl Pts',(5.49926686413145,15.2,-8.82869091272103));
#165316=CARTESIAN_POINT('Ctrl Pts',(5.50025419422016,15.2,-8.83076367841218));
#165317=CARTESIAN_POINT('Ctrl Pts',(5.50125805810934,15.2,-8.83288758219811));
#165318=CARTESIAN_POINT('Ctrl Pts',(5.50226192190734,15.2,-8.83501148579112));
#165319=CARTESIAN_POINT('Ctrl Pts',(5.50328231821661,15.2,-8.83718652736323));
#165320=CARTESIAN_POINT('Ctrl Pts',(5.50431836401705,15.2,-8.8394121930426));
#165321=CARTESIAN_POINT('Ctrl Pts',(5.5053544098175,15.2,-8.84163785872197));
#165322=CARTESIAN_POINT('Ctrl Pts',(5.50640610323126,15.2,-8.84391415024339));
#165323=CARTESIAN_POINT('Ctrl Pts',(5.50747258619186,15.2,-8.84624056382335));
#165324=CARTESIAN_POINT('Ctrl Pts',(5.50853906924934,15.2,-8.84856697761463));
#165325=CARTESIAN_POINT('Ctrl Pts',(5.50962034108367,15.2,-8.85094351569548));
#165326=CARTESIAN_POINT('Ctrl Pts',(5.5107155663943,15.2,-8.85336968649773));
#165327=CARTESIAN_POINT('Ctrl Pts',(5.51181079160544,15.2,-8.85579585707959));
#165328=CARTESIAN_POINT('Ctrl Pts',(5.51291997050134,15.2,-8.85827166115236));
#165329=CARTESIAN_POINT('Ctrl Pts',(5.51404228979448,15.2,-8.86079661514608));
#165330=CARTESIAN_POINT('Ctrl Pts',(5.51553871555263,15.2,-8.86416322054752));
#165331=CARTESIAN_POINT('Ctrl Pts',(5.51705850066996,15.2,-8.86761720947481));
#165332=CARTESIAN_POINT('Ctrl Pts',(5.51859977976712,15.2,-8.87115746377614));
#165333=CARTESIAN_POINT('Ctrl Pts',(5.51975573906372,15.2,-8.87381265444185));
#165334=CARTESIAN_POINT('Ctrl Pts',(5.52092378940405,15.2,-8.87651637193557));
#165335=CARTESIAN_POINT('Ctrl Pts',(5.52210316794403,15.2,-8.87926815583349));
#165336=CARTESIAN_POINT('Ctrl Pts',(5.52328254659114,15.2,-8.88201993998135));
#165337=CARTESIAN_POINT('Ctrl Pts',(5.52447325341468,15.2,-8.88481979146023));
#165338=CARTESIAN_POINT('Ctrl Pts',(5.52567454614754,15.2,-8.88766726053533));
#165339=CARTESIAN_POINT('Ctrl Pts',(5.52687583877127,15.2,-8.89051472935179));
#165340=CARTESIAN_POINT('Ctrl Pts',(5.52808771721051,15.2,-8.89340981469033));
#165341=CARTESIAN_POINT('Ctrl Pts',(5.52930945683322,15.2,-8.89635207466882));
#165342=CARTESIAN_POINT('Ctrl Pts',(5.53053119645593,15.2,-8.89929433464731));
#165343=CARTESIAN_POINT('Ctrl Pts',(5.53176279711951,15.2,-8.90228377044705));
#165344=CARTESIAN_POINT('Ctrl Pts',(5.53300355465734,15.2,-8.90531994633465));
#165345=CARTESIAN_POINT('Ctrl Pts',(5.53424431230788,15.2,-8.90835612249804));
#165346=CARTESIAN_POINT('Ctrl Pts',(5.53549422414293,15.2,-8.911439038534));
#165347=CARTESIAN_POINT('Ctrl Pts',(5.53675260512876,15.2,-8.91456827154103));
#165348=CARTESIAN_POINT('Ctrl Pts',(5.53801098600029,15.2,-8.91769750426382));
#165349=CARTESIAN_POINT('Ctrl Pts',(5.53927783420707,15.2,-8.92087304989906));
#165350=CARTESIAN_POINT('Ctrl Pts',(5.54055247907776,15.2,-8.92409449086736));
#165351=CARTESIAN_POINT('Ctrl Pts',(5.54182712394848,15.2,-8.92731593183566));
#165352=CARTESIAN_POINT('Ctrl Pts',(5.54310956692685,15.2,-8.93058326810029));
#165353=CARTESIAN_POINT('Ctrl Pts',(5.54439914987968,15.2,-8.93389608706124));
#165354=CARTESIAN_POINT('Ctrl Pts',(5.5456887328325,15.2,-8.93720890602218));
#165355=CARTESIAN_POINT('Ctrl Pts',(5.54698545768903,15.2,-8.94056720898073));
#165356=CARTESIAN_POINT('Ctrl Pts',(5.54828868564122,15.2,-8.94397058710398));
#165357=CARTESIAN_POINT('Ctrl Pts',(5.54959191371179,15.2,-8.94737396553636));
#165358=CARTESIAN_POINT('Ctrl Pts',(5.55090164269138,15.2,-8.9508224233232));
#165359=CARTESIAN_POINT('Ctrl Pts',(5.55221725084666,15.2,-8.95431555693216));
#165360=CARTESIAN_POINT('Ctrl Pts',(5.55353285888243,15.2,-8.95780869022383));
#165361=CARTESIAN_POINT('Ctrl Pts',(5.55485434506653,15.2,-8.96134650319564));
#165362=CARTESIAN_POINT('Ctrl Pts',(5.55618109927433,15.2,-8.96492860024832));
#165363=CARTESIAN_POINT('Ctrl Pts',(5.55750785348214,15.2,-8.968510697301));
#165364=CARTESIAN_POINT('Ctrl Pts',(5.55883987556145,15.2,-8.97213707871123));
#165365=CARTESIAN_POINT('Ctrl Pts',(5.56017657159591,15.2,-8.97580735782489));
#165366=CARTESIAN_POINT('Ctrl Pts',(5.56151326775177,15.2,-8.97947763727193));
#165367=CARTESIAN_POINT('Ctrl Pts',(5.56285463546433,15.2,-8.98319181465183));
#165368=CARTESIAN_POINT('Ctrl Pts',(5.5642000938551,15.2,-8.98694950738022));
#165369=CARTESIAN_POINT('Ctrl Pts',(5.56532130911965,15.2,-8.99008091781654));
#165370=CARTESIAN_POINT('Ctrl Pts',(5.56644536587487,15.2,-8.99324254762608));
#165371=CARTESIAN_POINT('Ctrl Pts',(5.56757193288896,15.2,-8.99643417943408));
#165372=CARTESIAN_POINT('Ctrl Pts',(5.56869849990304,15.2,-8.99962581124207));
#165373=CARTESIAN_POINT('Ctrl Pts',(5.56982757803107,15.2,-9.0028474442895));
#165374=CARTESIAN_POINT('Ctrl Pts',(5.57095884261458,15.2,-9.0060988636669));
#165375=CARTESIAN_POINT('Ctrl Pts',(5.57209010707476,15.2,-9.00935028268989));
#165376=CARTESIAN_POINT('Ctrl Pts',(5.57322355935868,15.2,-9.01263148874131));
#165377=CARTESIAN_POINT('Ctrl Pts',(5.57435887965144,15.2,-9.01594226705857));
#165378=CARTESIAN_POINT('Ctrl Pts',(5.57549420006795,15.2,-9.0192530457367));
#165379=CARTESIAN_POINT('Ctrl Pts',(5.57663138910113,15.2,-9.02259339834494));
#165380=CARTESIAN_POINT('Ctrl Pts',(5.57777013535099,15.2,-9.02596311355086));
#165381=CARTESIAN_POINT('Ctrl Pts',(5.57890888160086,15.2,-9.02933282875677));
#165382=CARTESIAN_POINT('Ctrl Pts',(5.58004918481604,15.2,-9.03273190783283));
#165383=CARTESIAN_POINT('Ctrl Pts',(5.5811907378591,15.2,-9.03616014008542));
#165384=CARTESIAN_POINT('Ctrl Pts',(5.58233229090214,15.2,-9.039588372338));
#165385=CARTESIAN_POINT('Ctrl Pts',(5.58347509396963,15.2,-9.04304575989028));
#165386=CARTESIAN_POINT('Ctrl Pts',(5.58461884535848,15.2,-9.04653209676378));
#165387=CARTESIAN_POINT('Ctrl Pts',(5.58576259674732,15.2,-9.0500184336373));
#165388=CARTESIAN_POINT('Ctrl Pts',(5.58690729834731,15.2,-9.05353371799764));
#165389=CARTESIAN_POINT('Ctrl Pts',(5.58805265216671,15.2,-9.05707774751));
#165390=CARTESIAN_POINT('Ctrl Pts',(5.58919800598611,15.2,-9.06062177702235));
#165391=CARTESIAN_POINT('Ctrl Pts',(5.59034401286633,15.2,-9.06419455234836));
#165392=CARTESIAN_POINT('Ctrl Pts',(5.59149038252432,15.2,-9.06779587028132));
#165393=CARTESIAN_POINT('Ctrl Pts',(5.59263675218231,15.2,-9.07139718821428));
#165394=CARTESIAN_POINT('Ctrl Pts',(5.59378348292216,15.2,-9.07502705063882));
#165395=CARTESIAN_POINT('Ctrl Pts',(5.59493029174161,15.2,-9.0786852552916));
#165396=CARTESIAN_POINT('Ctrl Pts',(5.59607710056105,15.2,-9.08234345994438));
#165397=CARTESIAN_POINT('Ctrl Pts',(5.59722398550091,15.2,-9.08603001015168));
#165398=CARTESIAN_POINT('Ctrl Pts',(5.59837066620057,15.2,-9.08974470475198));
#165399=CARTESIAN_POINT('Ctrl Pts',(5.59951734690023,15.2,-9.09345939935228));
#165400=CARTESIAN_POINT('Ctrl Pts',(5.60066382501381,15.2,-9.0972022406897));
#165401=CARTESIAN_POINT('Ctrl Pts',(5.60180982154156,15.2,-9.10097303270505));
#165402=CARTESIAN_POINT('Ctrl Pts',(5.60295581806932,15.2,-9.10474382472042));
#165403=CARTESIAN_POINT('Ctrl Pts',(5.60410133522485,15.2,-9.10854256793226));
#165404=CARTESIAN_POINT('Ctrl Pts',(5.60524610084981,15.2,-9.11236906751703));
#165405=CARTESIAN_POINT('Ctrl Pts',(5.60661981954985,15.2,-9.11696086685194));
#165406=CARTESIAN_POINT('Ctrl Pts',(5.60799245627496,15.2,-9.12159263445863));
#165407=CARTESIAN_POINT('Ctrl Pts',(5.60936354922522,15.2,-9.12626404270386));
#165408=CARTESIAN_POINT('Ctrl Pts',(5.61050612672528,15.2,-9.13015688304965));
#165409=CARTESIAN_POINT('Ctrl Pts',(5.61164763461081,15.2,-9.1340772502355));
#165410=CARTESIAN_POINT('Ctrl Pts',(5.61278780878266,15.2,-9.13802495323947));
#165411=CARTESIAN_POINT('Ctrl Pts',(5.6139279829545,15.2,-9.14197265624343));
#165412=CARTESIAN_POINT('Ctrl Pts',(5.61506682437216,15.2,-9.14594769726104));
#165413=CARTESIAN_POINT('Ctrl Pts',(5.61620407673328,15.2,-9.14994988677494));
#165414=CARTESIAN_POINT('Ctrl Pts',(5.61711387867176,15.2,-9.15315163856056));
#165415=CARTESIAN_POINT('Ctrl Pts',(5.61802266210177,15.2,-9.15637076496482));
#165416=CARTESIAN_POINT('Ctrl Pts',(5.61893029887335,15.2,-9.15960717275411));
#165417=CARTESIAN_POINT('Ctrl Pts',(5.61983793552126,15.2,-9.16284358010244));
#165418=CARTESIAN_POINT('Ctrl Pts',(5.62074442628866,15.2,-9.16609726676974));
#165419=CARTESIAN_POINT('Ctrl Pts',(5.62164964027433,15.2,-9.16936813823939));
#165420=CARTESIAN_POINT('Ctrl Pts',(5.62255485438335,15.2,-9.17263901015471));
#165421=CARTESIAN_POINT('Ctrl Pts',(5.62345879426513,15.2,-9.1759270681057));
#165422=CARTESIAN_POINT('Ctrl Pts',(5.62436133164751,15.2,-9.17923221656534));
#165423=CARTESIAN_POINT('Ctrl Pts',(5.62526386890692,15.2,-9.18253736457467));
#165424=CARTESIAN_POINT('Ctrl Pts',(5.62616500398872,15.2,-9.18585960212066));
#165425=CARTESIAN_POINT('Ctrl Pts',(5.62706461269306,15.2,-9.18919883823546));
#165426=CARTESIAN_POINT('Ctrl Pts',(5.62796422151997,15.2,-9.19253807480525));
#165427=CARTESIAN_POINT('Ctrl Pts',(5.62886230363652,15.2,-9.19589430955233));
#165428=CARTESIAN_POINT('Ctrl Pts',(5.62975873639669,15.2,-9.1992674482395));
#165429=CARTESIAN_POINT('Ctrl Pts',(5.63065516903472,15.2,-9.20264058646709));
#165430=CARTESIAN_POINT('Ctrl Pts',(5.63154995122204,15.2,-9.20603062856788));
#165431=CARTESIAN_POINT('Ctrl Pts',(5.63244296192693,15.2,-9.20943748395493));
#165432=CARTESIAN_POINT('Ctrl Pts',(5.63333597275349,15.2,-9.21284433980616));
#165433=CARTESIAN_POINT('Ctrl Pts',(5.63422721194373,15.2,-9.21626800593721));
#165434=CARTESIAN_POINT('Ctrl Pts',(5.63511656004764,15.2,-9.2197083950147));
#165435=CARTESIAN_POINT('Ctrl Pts',(5.63600590803037,15.2,-9.22314878362344));
#165436=CARTESIAN_POINT('Ctrl Pts',(5.63689336363277,15.2,-9.22660589165509));
#165437=CARTESIAN_POINT('Ctrl Pts',(5.63777880960479,15.2,-9.23007963048765));
#165438=CARTESIAN_POINT('Ctrl Pts',(5.63866425569746,15.2,-9.23355336979351));
#165439=CARTESIAN_POINT('Ctrl Pts',(5.63954768970464,15.2,-9.23704373748347));
#165440=CARTESIAN_POINT('Ctrl Pts',(5.64042899836365,15.2,-9.2405506447868));
#165441=CARTESIAN_POINT('Ctrl Pts',(5.64131030690258,15.2,-9.24405755161229));
#165442=CARTESIAN_POINT('Ctrl Pts',(5.64218948594748,15.2,-9.24758099778171));
#165443=CARTESIAN_POINT('Ctrl Pts',(5.64306642259824,15.2,-9.25112089321286));
#165444=CARTESIAN_POINT('Ctrl Pts',(5.64394335936849,15.2,-9.25466078912631));
#165445=CARTESIAN_POINT('Ctrl Pts',(5.64481805183794,15.2,-9.25821713354139));
#165446=CARTESIAN_POINT('Ctrl Pts',(5.64569038800055,15.2,-9.26178983875239));
#165447=CARTESIAN_POINT('Ctrl Pts',(5.6465627240443,15.2,-9.2653625434766));
#165448=CARTESIAN_POINT('Ctrl Pts',(5.647432701751,15.2,-9.26895160764578));
#165449=CARTESIAN_POINT('Ctrl Pts',(5.64830020912478,15.2,-9.27255694312716));
#165450=CARTESIAN_POINT('Ctrl Pts',(5.64916771661676,15.2,-9.27616227909976));
#165451=CARTESIAN_POINT('Ctrl Pts',(5.6500327534974,15.2,-9.27978388704058));
#165452=CARTESIAN_POINT('Ctrl Pts',(5.65089520776662,15.2,-9.28342167701661));
#165453=CARTESIAN_POINT('Ctrl Pts',(5.65175766203585,15.2,-9.28705946699264));
#165454=CARTESIAN_POINT('Ctrl Pts',(5.65261753520755,15.2,-9.29071343906502));
#165455=CARTESIAN_POINT('Ctrl Pts',(5.6534747148651,15.2,-9.29438350760002));
#165456=CARTESIAN_POINT('Ctrl Pts',(5.65433189440586,15.2,-9.29805357563497));
#165457=CARTESIAN_POINT('Ctrl Pts',(5.65518638215678,15.2,-9.30173973875276));
#165458=CARTESIAN_POINT('Ctrl Pts',(5.65603806825771,15.2,-9.30544190952244));
#165459=CARTESIAN_POINT('Ctrl Pts',(5.65688975447467,15.2,-9.30914408079652));
#165460=CARTESIAN_POINT('Ctrl Pts',(5.65773863933691,15.2,-9.31286225991089));
#165461=CARTESIAN_POINT('Ctrl Pts',(5.65858461560494,15.2,-9.31659636056049));
#165462=CARTESIAN_POINT('Ctrl Pts',(5.6594305917577,15.2,-9.32033046070131));
#165463=CARTESIAN_POINT('Ctrl Pts',(5.66027365826084,15.2,-9.32408048162337));
#165464=CARTESIAN_POINT('Ctrl Pts',(5.66111371041459,15.2,-9.32784633842558));
#165465=CARTESIAN_POINT('Ctrl Pts',(5.66195376268279,15.2,-9.33161219574089));
#165466=CARTESIAN_POINT('Ctrl Pts',(5.66279079897299,15.2,-9.33539388832526));
#165467=CARTESIAN_POINT('Ctrl Pts',(5.66362471583761,15.2,-9.33919132983441));
#165468=CARTESIAN_POINT('Ctrl Pts',(5.6644586325886,15.2,-9.34298877082616));
#165469=CARTESIAN_POINT('Ctrl Pts',(5.66528942769695,15.2,-9.34680196139004));
#165470=CARTESIAN_POINT('Ctrl Pts',(5.66611699990727,15.2,-9.3506308161871));
#165471=CARTESIAN_POINT('Ctrl Pts',(5.66694457223036,15.2,-9.35445967150584));
#165472=CARTESIAN_POINT('Ctrl Pts',(5.66776891981696,15.2,-9.35830419055702));
#165473=CARTESIAN_POINT('Ctrl Pts',(5.66858994075038,15.2,-9.362164289824));
#165474=CARTESIAN_POINT('Ctrl Pts',(5.66941096157194,15.2,-9.36602438856505));
#165475=CARTESIAN_POINT('Ctrl Pts',(5.67022865635459,15.2,-9.36990006707155));
#165476=CARTESIAN_POINT('Ctrl Pts',(5.67104292260678,15.2,-9.37379124016874));
#165477=CARTESIAN_POINT('Ctrl Pts',(5.67185718896992,15.2,-9.37768241379611));
#165478=CARTESIAN_POINT('Ctrl Pts',(5.67266802737214,15.2,-9.38158908264483));
#165479=CARTESIAN_POINT('Ctrl Pts',(5.67347533708259,15.2,-9.38551116330407));
#165480=CARTESIAN_POINT('Ctrl Pts',(5.67428264668304,15.2,-9.38943324342893));
#165481=CARTESIAN_POINT('Ctrl Pts',(5.6750864278175,15.2,-9.39337073562006));
#165482=CARTESIAN_POINT('Ctrl Pts',(5.67588658141914,15.2,-9.39732355512869));
#165483=CARTESIAN_POINT('Ctrl Pts',(5.67668673512979,15.2,-9.4012763751759));
#165484=CARTESIAN_POINT('Ctrl Pts',(5.67748326098175,15.2,-9.40524452292172));
#165485=CARTESIAN_POINT('Ctrl Pts',(5.67827606252496,15.2,-9.40922791624995));
#165486=CARTESIAN_POINT('Ctrl Pts',(5.67906886406817,15.2,-9.41321130957817));
#165487=CARTESIAN_POINT('Ctrl Pts',(5.67985793877206,15.2,-9.41720994765537));
#165488=CARTESIAN_POINT('Ctrl Pts',(5.68064319187001,15.2,-9.42122374893122));
#165489=CARTESIAN_POINT('Ctrl Pts',(5.68142844486097,15.2,-9.42523754966019));
#165490=CARTESIAN_POINT('Ctrl Pts',(5.68220987585667,15.2,-9.42926651283173));
#165491=CARTESIAN_POINT('Ctrl Pts',(5.6829873887411,15.2,-9.43331055696387));
#165492=CARTESIAN_POINT('Ctrl Pts',(5.68376490173146,15.2,-9.43735460164701));
#165493=CARTESIAN_POINT('Ctrl Pts',(5.68453849650092,15.2,-9.44141372589803));
#165494=CARTESIAN_POINT('Ctrl Pts',(5.68530807887578,15.2,-9.44548784989941));
#165495=CARTESIAN_POINT('Ctrl Pts',(5.6860776611458,15.2,-9.4495619733457));
#165496=CARTESIAN_POINT('Ctrl Pts',(5.68684322995243,15.2,-9.45365109599273));
#165497=CARTESIAN_POINT('Ctrl Pts',(5.68760469294601,15.2,-9.45775513615626));
#165498=CARTESIAN_POINT('Ctrl Pts',(5.68836615604333,15.2,-9.46185917687895));
#165499=CARTESIAN_POINT('Ctrl Pts',(5.68912351394759,15.2,-9.4659781349918));
#165500=CARTESIAN_POINT('Ctrl Pts',(5.68987667235922,15.2,-9.47011193059154));
#165501=CARTESIAN_POINT('Ctrl Pts',(5.69062983066824,15.2,-9.47424572562805));
#165502=CARTESIAN_POINT('Ctrl Pts',(5.69137878963853,15.2,-9.47839435699274));
#165503=CARTESIAN_POINT('Ctrl Pts',(5.69212345868904,15.2,-9.4825577451514));
#165504=CARTESIAN_POINT('Ctrl Pts',(5.69286812784101,15.2,-9.48672113387734));
#165505=CARTESIAN_POINT('Ctrl Pts',(5.6936085065036,15.2,-9.49089927927175));
#165506=CARTESIAN_POINT('Ctrl Pts',(5.69434450487675,15.2,-9.49509210133452));
#165507=CARTESIAN_POINT('Ctrl Pts',(5.69508050314962,15.2,-9.499284922826));
#165508=CARTESIAN_POINT('Ctrl Pts',(5.69581212078937,15.2,-9.5034924197479));
#165509=CARTESIAN_POINT('Ctrl Pts',(5.69653926787776,15.2,-9.50771451411239));
#165510=CARTESIAN_POINT('Ctrl Pts',(5.69744820181254,15.2,-9.51299213249944));
#165511=CARTESIAN_POINT('Ctrl Pts',(5.69835015177435,15.2,-9.51829255963091));
#165512=CARTESIAN_POINT('Ctrl Pts',(5.69924494323307,15.2,-9.52361563789364));
#165513=CARTESIAN_POINT('Ctrl Pts',(5.69996077643905,15.2,-9.52787410073591));
#165514=CARTESIAN_POINT('Ctrl Pts',(5.70067203001115,15.2,-9.53214706225213));
#165515=CARTESIAN_POINT('Ctrl Pts',(5.70137861454935,15.2,-9.53643444287558));
#165516=CARTESIAN_POINT('Ctrl Pts',(5.70208519899128,15.2,-9.54072182291489));
#165517=CARTESIAN_POINT('Ctrl Pts',(5.70278711590663,15.2,-9.54502362000108));
#165518=CARTESIAN_POINT('Ctrl Pts',(5.70348427894044,15.2,-9.54933975964041));
#165519=CARTESIAN_POINT('Ctrl Pts',(5.70418144206923,15.2,-9.55365589986781));
#165520=CARTESIAN_POINT('Ctrl Pts',(5.70487385056064,15.2,-9.557986379362));
#165521=CARTESIAN_POINT('Ctrl Pts',(5.70556141909779,15.2,-9.56233112215528));
#165522=CARTESIAN_POINT('Ctrl Pts',(5.70624898754126,15.2,-9.56667586435658));
#165523=CARTESIAN_POINT('Ctrl Pts',(5.70693171676072,15.2,-9.57103486862725));
#165524=CARTESIAN_POINT('Ctrl Pts',(5.70760952237247,15.2,-9.57540805860162));
#165525=CARTESIAN_POINT('Ctrl Pts',(5.70828732807658,15.2,-9.57978124917183));
#165526=CARTESIAN_POINT('Ctrl Pts',(5.70896020769989,15.2,-9.58416862314304));
#165527=CARTESIAN_POINT('Ctrl Pts',(5.70962808151709,15.2,-9.58857010473629));
#165528=CARTESIAN_POINT('Ctrl Pts',(5.71012898683448,15.2,-9.59187121563138));
#165529=CARTESIAN_POINT('Ctrl Pts',(5.71062707536524,15.2,-9.59518026310242));
#165530=CARTESIAN_POINT('Ctrl Pts',(5.71112231218285,15.2,-9.59849721245529));
#165531=CARTESIAN_POINT('Ctrl Pts',(5.71161754900046,15.2,-9.60181416180816));
#165532=CARTESIAN_POINT('Ctrl Pts',(5.71210993339743,15.2,-9.6051390145586));
#165533=CARTESIAN_POINT('Ctrl Pts',(5.71259943217156,15.2,-9.60847173739516));
#165534=CARTESIAN_POINT('Ctrl Pts',(5.71308893094569,15.2,-9.61180446023171));
#165535=CARTESIAN_POINT('Ctrl Pts',(5.71357554332836,15.2,-9.61514505440941));
#165536=CARTESIAN_POINT('Ctrl Pts',(5.71405923514452,15.2,-9.61849348574501));
#165537=CARTESIAN_POINT('Ctrl Pts',(5.71454292704854,15.2,-9.62184191768891));
#165538=CARTESIAN_POINT('Ctrl Pts',(5.71502369871842,15.2,-9.62519818791));
#165539=CARTESIAN_POINT('Ctrl Pts',(5.71550151516246,15.2,-9.62856226473333));
#165540=CARTESIAN_POINT('Ctrl Pts',(5.71629787569999,15.2,-9.63416905801289));
#165541=CARTESIAN_POINT('Ctrl Pts',(5.71708602842116,15.2,-9.63979753358412));
#165542=CARTESIAN_POINT('Ctrl Pts',(5.71786581736463,15.2,-9.64544754449428));
#165543=CARTESIAN_POINT('Ctrl Pts',(5.7183336908497,15.2,-9.64883755190256));
#165544=CARTESIAN_POINT('Ctrl Pts',(5.71879855416727,15.2,-9.65223531204639));
#165545=CARTESIAN_POINT('Ctrl Pts',(5.71926037260897,15.2,-9.6556407925007));
#165546=CARTESIAN_POINT('Ctrl Pts',(5.71972219096677,15.2,-9.65904627233634));
#165547=CARTESIAN_POINT('Ctrl Pts',(5.72018096474975,15.2,-9.66245947352992));
#165548=CARTESIAN_POINT('Ctrl Pts',(5.72063666206625,15.2,-9.66588036286463));
#165549=CARTESIAN_POINT('Ctrl Pts',(5.72109235938276,15.2,-9.66930125219934));
#165550=CARTESIAN_POINT('Ctrl Pts',(5.72154497911468,15.2,-9.6727298301623));
#165551=CARTESIAN_POINT('Ctrl Pts',(5.72199448851704,15.2,-9.67616606546974));
#165552=CARTESIAN_POINT('Ctrl Pts',(5.7224439979194,15.2,-9.67960230077718));
#165553=CARTESIAN_POINT('Ctrl Pts',(5.72289039758031,15.2,-9.68304619372326));
#165554=CARTESIAN_POINT('Ctrl Pts',(5.72333365402456,15.2,-9.68649771198849));
#165555=CARTESIAN_POINT('Ctrl Pts',(5.72377691046882,15.2,-9.68994923025373));
#165556=CARTESIAN_POINT('Ctrl Pts',(5.72421702476789,15.2,-9.69340837381549));
#165557=CARTESIAN_POINT('Ctrl Pts',(5.72465396371062,15.2,-9.69687511114722));
#165558=CARTESIAN_POINT('Ctrl Pts',(5.72509090265336,15.2,-9.70034184847895));
#165559=CARTESIAN_POINT('Ctrl Pts',(5.72552466672131,15.2,-9.70381618066846));
#165560=CARTESIAN_POINT('Ctrl Pts',(5.72595522362277,15.2,-9.70729807449925));
#165561=CARTESIAN_POINT('Ctrl Pts',(5.72638578060245,15.2,-9.71077996896258));
#165562=CARTESIAN_POINT('Ctrl Pts',(5.72681313071456,15.2,-9.71426942558639));
#165563=CARTESIAN_POINT('Ctrl Pts',(5.72723724210909,15.2,-9.71776641401231));
#165564=CARTESIAN_POINT('Ctrl Pts',(5.72766135342657,15.2,-9.72126340180294));
#165565=CARTESIAN_POINT('Ctrl Pts',(5.72808222497542,15.2,-9.7247679209308));
#165566=CARTESIAN_POINT('Ctrl Pts',(5.72849982685573,15.2,-9.72827993989619));
#165567=CARTESIAN_POINT('Ctrl Pts',(5.72905662933753,15.2,-9.73296263163737));
#165568=CARTESIAN_POINT('Ctrl Pts',(5.72960761765509,15.2,-9.73765865660929));
#165569=CARTESIAN_POINT('Ctrl Pts',(5.73015271872202,15.2,-9.7423679413901));
#165570=CARTESIAN_POINT('Ctrl Pts',(5.73056154454078,15.2,-9.74589990513612));
#165571=CARTESIAN_POINT('Ctrl Pts',(5.73096705657645,15.2,-9.74943932625664));
#165572=CARTESIAN_POINT('Ctrl Pts',(5.73136922689563,15.2,-9.75298617600176));
#165573=CARTESIAN_POINT('Ctrl Pts',(5.73177139728787,15.2,-9.75653302639121));
#165574=CARTESIAN_POINT('Ctrl Pts',(5.73217022414583,15.2,-9.76008730432445));
#165575=CARTESIAN_POINT('Ctrl Pts',(5.73256567761951,15.2,-9.76364897830141));
#165576=CARTESIAN_POINT('Ctrl Pts',(5.73296113102135,15.2,-9.76721065163135));
#165577=CARTESIAN_POINT('Ctrl Pts',(5.73335321090669,15.2,-9.77077972156922));
#165578=CARTESIAN_POINT('Ctrl Pts',(5.73374188676727,15.2,-9.77435615689825));
#165579=CARTESIAN_POINT('Ctrl Pts',(5.73413056262785,15.2,-9.77793259222727));
#165580=CARTESIAN_POINT('Ctrl Pts',(5.73451583342913,15.2,-9.78151639300068));
#165581=CARTESIAN_POINT('Ctrl Pts',(5.73489767029198,15.2,-9.78510752971989));
#165582=CARTESIAN_POINT('Ctrl Pts',(5.73527950715483,15.2,-9.7886986664391));
#165583=CARTESIAN_POINT('Ctrl Pts',(5.7356579088282,15.2,-9.79229713751135));
#165584=CARTESIAN_POINT('Ctrl Pts',(5.73603284673296,15.2,-9.79590291327169));
#165585=CARTESIAN_POINT('Ctrl Pts',(5.73640778463773,15.2,-9.79950868903203));
#165586=CARTESIAN_POINT('Ctrl Pts',(5.73677925830621,15.2,-9.80312176875431));
#165587=CARTESIAN_POINT('Ctrl Pts',(5.73714723725147,15.2,-9.80674212208047));
#165588=CARTESIAN_POINT('Ctrl Pts',(5.73751521619673,15.2,-9.81036247540663));
#165589=CARTESIAN_POINT('Ctrl Pts',(5.73787970075058,15.2,-9.81399010270728));
#165590=CARTESIAN_POINT('Ctrl Pts',(5.73824066165461,15.2,-9.81762497344923));
#165591=CARTESIAN_POINT('Ctrl Pts',(5.73860162262422,15.2,-9.82125984485152));
#165592=CARTESIAN_POINT('Ctrl Pts',(5.73895905887616,15.2,-9.82490195898083));
#165593=CARTESIAN_POINT('Ctrl Pts',(5.73931294284378,15.2,-9.82855128680385));
#165594=CARTESIAN_POINT('Ctrl Pts',(5.73966682674711,15.2,-9.83220061396391));
#165595=CARTESIAN_POINT('Ctrl Pts',(5.74001715759605,15.2,-9.83585715234145));
#165596=CARTESIAN_POINT('Ctrl Pts',(5.74036390605869,15.2,-9.83952087472554));
#165597=CARTESIAN_POINT('Ctrl Pts',(5.74071065452133,15.2,-9.84318459710964));
#165598=CARTESIAN_POINT('Ctrl Pts',(5.74105382036624,15.2,-9.84685550108401));
#165599=CARTESIAN_POINT('Ctrl Pts',(5.74139337527025,15.2,-9.85053355740932));
#165600=CARTESIAN_POINT('Ctrl Pts',(5.74173293017427,15.2,-9.85421161373463));
#165601=CARTESIAN_POINT('Ctrl Pts',(5.74206887312871,15.2,-9.85789682291744));
#165602=CARTESIAN_POINT('Ctrl Pts',(5.74240117749164,15.2,-9.86158915378329));
#165603=CARTESIAN_POINT('Ctrl Pts',(5.74273348185456,15.2,-9.86528148464913));
#165604=CARTESIAN_POINT('Ctrl Pts',(5.7430621458093,15.2,-9.86898093776469));
#165605=CARTESIAN_POINT('Ctrl Pts',(5.74338714271448,15.2,-9.87268748404607));
#165606=CARTESIAN_POINT('Ctrl Pts',(5.74371213961966,15.2,-9.87639403032745));
#165607=CARTESIAN_POINT('Ctrl Pts',(5.74403346868372,15.2,-9.88010766911364));
#165608=CARTESIAN_POINT('Ctrl Pts',(5.74435109968848,15.2,-9.88382836903851));
#165609=CARTESIAN_POINT('Ctrl Pts',(5.74466873069324,15.2,-9.88754906896337));
#165610=CARTESIAN_POINT('Ctrl Pts',(5.74498266422643,15.2,-9.89127682890577));
#165611=CARTESIAN_POINT('Ctrl Pts',(5.74529287317401,15.2,-9.89501162118579));
#165612=CARTESIAN_POINT('Ctrl Pts',(5.74560308217794,15.2,-9.89874641414431));
#165613=CARTESIAN_POINT('Ctrl Pts',(5.74590956548914,15.2,-9.90248823862143));
#165614=CARTESIAN_POINT('Ctrl Pts',(5.7462122990743,15.2,-9.90623706808388));
#165615=CARTESIAN_POINT('Ctrl Pts',(5.74661594376283,15.2,-9.91123550623208));
#165616=CARTESIAN_POINT('Ctrl Pts',(5.74701292447168,15.2,-9.91624639874254));
#165617=CARTESIAN_POINT('Ctrl Pts',(5.74740316821801,15.2,-9.9212696688311));
#165618=CARTESIAN_POINT('Ctrl Pts',(5.74769585104103,15.2,-9.92503712156862));
#165619=CARTESIAN_POINT('Ctrl Pts',(5.74798474299045,15.2,-9.92881153501771));
#165620=CARTESIAN_POINT('Ctrl Pts',(5.74826981149478,15.2,-9.93259287498512));
#165621=CARTESIAN_POINT('Ctrl Pts',(5.74855487999911,15.2,-9.93637421495252));
#165622=CARTESIAN_POINT('Ctrl Pts',(5.74883612434905,15.2,-9.94016247957813));
#165623=CARTESIAN_POINT('Ctrl Pts',(5.7491135267145,15.2,-9.9439576491893));
#165624=CARTESIAN_POINT('Ctrl Pts',(5.74948339656868,15.2,-9.94901787579716));
#165625=CARTESIAN_POINT('Ctrl Pts',(5.74984644090288,15.2,-9.95409037694775));
#165626=CARTESIAN_POINT('Ctrl Pts',(5.75020264099994,15.2,-9.95917514500001));
#165627=CARTESIAN_POINT('Ctrl Pts',(4.57383771099994,15.2,-9.31239140100002));
#165628=CARTESIAN_POINT('Ctrl Pts',(4.57383771099994,11.6,-9.31239140100002));
#165629=CARTESIAN_POINT('Ctrl Pts',(4.57392774199994,15.2,-9.31254071600002));
#165630=CARTESIAN_POINT('Ctrl Pts',(4.57392774199994,11.6,-9.31254071600002));
#165631=CARTESIAN_POINT('Ctrl Pts',(4.57411102199994,15.2,-9.31284451800002));
#165632=CARTESIAN_POINT('Ctrl Pts',(4.57411102199994,11.6,-9.31284451800002));
#165633=CARTESIAN_POINT('Ctrl Pts',(4.57438896199994,15.2,-9.31330471200001));
#165634=CARTESIAN_POINT('Ctrl Pts',(4.57438896199994,11.6,-9.31330471200001));
#165635=CARTESIAN_POINT('Ctrl Pts',(4.57476383499994,15.2,-9.31392435700002));
#165636=CARTESIAN_POINT('Ctrl Pts',(4.57476383499994,11.6,-9.31392435700002));
#165637=CARTESIAN_POINT('Ctrl Pts',(4.57523877599994,15.2,-9.31470764300002));
#165638=CARTESIAN_POINT('Ctrl Pts',(4.57523877599994,11.6,-9.31470764300002));
#165639=CARTESIAN_POINT('Ctrl Pts',(4.57572221399994,15.2,-9.31550314000001));
#165640=CARTESIAN_POINT('Ctrl Pts',(4.57572221399994,11.6,-9.31550314000001));
#165641=CARTESIAN_POINT('Ctrl Pts',(4.57621139799994,15.2,-9.31630627600001));
#165642=CARTESIAN_POINT('Ctrl Pts',(4.57621139799994,11.6,-9.31630627600001));
#165643=CARTESIAN_POINT('Ctrl Pts',(4.57670632999994,15.2,-9.31711702100002));
#165644=CARTESIAN_POINT('Ctrl Pts',(4.57670632999994,11.6,-9.31711702100002));
#165645=CARTESIAN_POINT('Ctrl Pts',(4.57720701299994,15.2,-9.31793534100001));
#165646=CARTESIAN_POINT('Ctrl Pts',(4.57720701299994,11.6,-9.31793534100001));
#165647=CARTESIAN_POINT('Ctrl Pts',(4.57771344599994,15.2,-9.31876120400002));
#165648=CARTESIAN_POINT('Ctrl Pts',(4.57771344599994,11.6,-9.31876120400002));
#165649=CARTESIAN_POINT('Ctrl Pts',(4.57822563299994,15.2,-9.31959457900001));
#165650=CARTESIAN_POINT('Ctrl Pts',(4.57822563299994,11.6,-9.31959457900001));
#165651=CARTESIAN_POINT('Ctrl Pts',(4.57874357399994,15.2,-9.32043543300002));
#165652=CARTESIAN_POINT('Ctrl Pts',(4.57874357399994,11.6,-9.32043543300002));
#165653=CARTESIAN_POINT('Ctrl Pts',(4.57926726999994,15.2,-9.32128373600002));
#165654=CARTESIAN_POINT('Ctrl Pts',(4.57926726999994,11.6,-9.32128373600002));
#165655=CARTESIAN_POINT('Ctrl Pts',(4.57979672299994,15.2,-9.32213945400001));
#165656=CARTESIAN_POINT('Ctrl Pts',(4.57979672299994,11.6,-9.32213945400001));
#165657=CARTESIAN_POINT('Ctrl Pts',(4.58033193499994,15.2,-9.32300255700002));
#165658=CARTESIAN_POINT('Ctrl Pts',(4.58033193499994,11.6,-9.32300255700002));
#165659=CARTESIAN_POINT('Ctrl Pts',(4.58087290499994,15.2,-9.32387301400002));
#165660=CARTESIAN_POINT('Ctrl Pts',(4.58087290499994,11.6,-9.32387301400002));
#165661=CARTESIAN_POINT('Ctrl Pts',(4.58141963599994,15.2,-9.32475079300002));
#165662=CARTESIAN_POINT('Ctrl Pts',(4.58141963599994,11.6,-9.32475079300002));
#165663=CARTESIAN_POINT('Ctrl Pts',(4.58197212899994,15.2,-9.32563586400001));
#165664=CARTESIAN_POINT('Ctrl Pts',(4.58197212899994,11.6,-9.32563586400001));
#165665=CARTESIAN_POINT('Ctrl Pts',(4.58253038599994,15.2,-9.32652819500002));
#165666=CARTESIAN_POINT('Ctrl Pts',(4.58253038599994,11.6,-9.32652819500002));
#165667=CARTESIAN_POINT('Ctrl Pts',(4.58309440599994,15.2,-9.32742775700002));
#165668=CARTESIAN_POINT('Ctrl Pts',(4.58309440599994,11.6,-9.32742775700002));
#165669=CARTESIAN_POINT('Ctrl Pts',(4.58366419299994,15.2,-9.32833451700001));
#165670=CARTESIAN_POINT('Ctrl Pts',(4.58366419299994,11.6,-9.32833451700001));
#165671=CARTESIAN_POINT('Ctrl Pts',(4.58423974599994,15.2,-9.32924844800001));
#165672=CARTESIAN_POINT('Ctrl Pts',(4.58423974599994,11.6,-9.32924844800001));
#165673=CARTESIAN_POINT('Ctrl Pts',(4.58482106699994,15.2,-9.33016951700001));
#165674=CARTESIAN_POINT('Ctrl Pts',(4.58482106699994,11.6,-9.33016951700001));
#165675=CARTESIAN_POINT('Ctrl Pts',(4.58540815599994,15.2,-9.33109769500001));
#165676=CARTESIAN_POINT('Ctrl Pts',(4.58540815599994,11.6,-9.33109769500001));
#165677=CARTESIAN_POINT('Ctrl Pts',(4.58600101699994,15.2,-9.33203295200002));
#165678=CARTESIAN_POINT('Ctrl Pts',(4.58600101699994,11.6,-9.33203295200002));
#165679=CARTESIAN_POINT('Ctrl Pts',(4.58659964899994,15.2,-9.33297525800001));
#165680=CARTESIAN_POINT('Ctrl Pts',(4.58659964899994,11.6,-9.33297525800001));
#165681=CARTESIAN_POINT('Ctrl Pts',(4.58720405199994,15.2,-9.33392458500002));
#165682=CARTESIAN_POINT('Ctrl Pts',(4.58720405199994,11.6,-9.33392458500002));
#165683=CARTESIAN_POINT('Ctrl Pts',(4.58781422999994,15.2,-9.33488090000001));
#165684=CARTESIAN_POINT('Ctrl Pts',(4.58781422999994,11.6,-9.33488090000001));
#165685=CARTESIAN_POINT('Ctrl Pts',(4.58843018199994,15.2,-9.33584417600001));
#165686=CARTESIAN_POINT('Ctrl Pts',(4.58843018199994,11.6,-9.33584417600001));
#165687=CARTESIAN_POINT('Ctrl Pts',(4.58905190799995,15.2,-9.33681438400002));
#165688=CARTESIAN_POINT('Ctrl Pts',(4.58905190799995,11.6,-9.33681438400002));
#165689=CARTESIAN_POINT('Ctrl Pts',(4.58967941299994,15.2,-9.33779149400002));
#165690=CARTESIAN_POINT('Ctrl Pts',(4.58967941299994,11.6,-9.33779149400002));
#165691=CARTESIAN_POINT('Ctrl Pts',(4.59031269299994,15.2,-9.33877547700002));
#165692=CARTESIAN_POINT('Ctrl Pts',(4.59031269299994,11.6,-9.33877547700002));
#165693=CARTESIAN_POINT('Ctrl Pts',(4.59095175299994,15.2,-9.33976630400002));
#165694=CARTESIAN_POINT('Ctrl Pts',(4.59095175299994,11.6,-9.33976630400002));
#165695=CARTESIAN_POINT('Ctrl Pts',(4.59159659199994,15.2,-9.34076394900002));
#165696=CARTESIAN_POINT('Ctrl Pts',(4.59159659199994,11.6,-9.34076394900002));
#165697=CARTESIAN_POINT('Ctrl Pts',(4.59224721199994,15.2,-9.34176837800001));
#165698=CARTESIAN_POINT('Ctrl Pts',(4.59224721199994,11.6,-9.34176837800001));
#165699=CARTESIAN_POINT('Ctrl Pts',(4.59290361199994,15.2,-9.34277956800001));
#165700=CARTESIAN_POINT('Ctrl Pts',(4.59290361199994,11.6,-9.34277956800001));
#165701=CARTESIAN_POINT('Ctrl Pts',(4.59356579399994,15.2,-9.34379748800002));
#165702=CARTESIAN_POINT('Ctrl Pts',(4.59356579399994,11.6,-9.34379748800002));
#165703=CARTESIAN_POINT('Ctrl Pts',(4.59423375999994,15.2,-9.34482211000002));
#165704=CARTESIAN_POINT('Ctrl Pts',(4.59423375999994,11.6,-9.34482211000002));
#165705=CARTESIAN_POINT('Ctrl Pts',(4.59490750999994,15.2,-9.34585340600002));
#165706=CARTESIAN_POINT('Ctrl Pts',(4.59490750999994,11.6,-9.34585340600002));
#165707=CARTESIAN_POINT('Ctrl Pts',(4.59558704399994,15.2,-9.34689134800001));
#165708=CARTESIAN_POINT('Ctrl Pts',(4.59558704399994,11.6,-9.34689134800001));
#165709=CARTESIAN_POINT('Ctrl Pts',(4.59627236399994,15.2,-9.34793590900002));
#165710=CARTESIAN_POINT('Ctrl Pts',(4.59627236399994,11.6,-9.34793590900002));
#165711=CARTESIAN_POINT('Ctrl Pts',(4.59696346899994,15.2,-9.34898706000002));
#165712=CARTESIAN_POINT('Ctrl Pts',(4.59696346899994,11.6,-9.34898706000002));
#165713=CARTESIAN_POINT('Ctrl Pts',(4.59766036299994,15.2,-9.35004477400001));
#165714=CARTESIAN_POINT('Ctrl Pts',(4.59766036299994,11.6,-9.35004477400001));
#165715=CARTESIAN_POINT('Ctrl Pts',(4.59836304399994,15.2,-9.35110902400002));
#165716=CARTESIAN_POINT('Ctrl Pts',(4.59836304399994,11.6,-9.35110902400002));
#165717=CARTESIAN_POINT('Ctrl Pts',(4.59907151299994,15.2,-9.35217978300001));
#165718=CARTESIAN_POINT('Ctrl Pts',(4.59907151299994,11.6,-9.35217978300001));
#165719=CARTESIAN_POINT('Ctrl Pts',(4.59978577199994,15.2,-9.35325702300002));
#165720=CARTESIAN_POINT('Ctrl Pts',(4.59978577199994,11.6,-9.35325702300002));
#165721=CARTESIAN_POINT('Ctrl Pts',(4.60050582099994,15.2,-9.35434071600002));
#165722=CARTESIAN_POINT('Ctrl Pts',(4.60050582099994,11.6,-9.35434071600002));
#165723=CARTESIAN_POINT('Ctrl Pts',(4.60123166099994,15.2,-9.35543083800002));
#165724=CARTESIAN_POINT('Ctrl Pts',(4.60123166099994,11.6,-9.35543083800002));
#165725=CARTESIAN_POINT('Ctrl Pts',(4.60196329199994,15.2,-9.35652735800002));
#165726=CARTESIAN_POINT('Ctrl Pts',(4.60196329199994,11.6,-9.35652735800002));
#165727=CARTESIAN_POINT('Ctrl Pts',(4.60270071599994,15.2,-9.35763025300002));
#165728=CARTESIAN_POINT('Ctrl Pts',(4.60270071599994,11.6,-9.35763025300002));
#165729=CARTESIAN_POINT('Ctrl Pts',(4.60344393199994,15.2,-9.35873949500002));
#165730=CARTESIAN_POINT('Ctrl Pts',(4.60344393199994,11.6,-9.35873949500002));
#165731=CARTESIAN_POINT('Ctrl Pts',(4.60419294099994,15.2,-9.35985505600001));
#165732=CARTESIAN_POINT('Ctrl Pts',(4.60419294099994,11.6,-9.35985505600001));
#165733=CARTESIAN_POINT('Ctrl Pts',(4.60494774599994,15.2,-9.36097691200001));
#165734=CARTESIAN_POINT('Ctrl Pts',(4.60494774599994,11.6,-9.36097691200001));
#165735=CARTESIAN_POINT('Ctrl Pts',(4.60570834399994,15.2,-9.36210503600002));
#165736=CARTESIAN_POINT('Ctrl Pts',(4.60570834399994,11.6,-9.36210503600002));
#165737=CARTESIAN_POINT('Ctrl Pts',(4.60647473799994,15.2,-9.36323940100002));
#165738=CARTESIAN_POINT('Ctrl Pts',(4.60647473799994,11.6,-9.36323940100002));
#165739=CARTESIAN_POINT('Ctrl Pts',(4.60724692799994,15.2,-9.36437998200002));
#165740=CARTESIAN_POINT('Ctrl Pts',(4.60724692799994,11.6,-9.36437998200002));
#165741=CARTESIAN_POINT('Ctrl Pts',(4.60802491399994,15.2,-9.36552675100002));
#165742=CARTESIAN_POINT('Ctrl Pts',(4.60802491399994,11.6,-9.36552675100002));
#165743=CARTESIAN_POINT('Ctrl Pts',(4.60880869699994,15.2,-9.36667968600002));
#165744=CARTESIAN_POINT('Ctrl Pts',(4.60880869699994,11.6,-9.36667968600002));
#165745=CARTESIAN_POINT('Ctrl Pts',(4.60959827699994,15.2,-9.36783875800002));
#165746=CARTESIAN_POINT('Ctrl Pts',(4.60959827699994,11.6,-9.36783875800002));
#165747=CARTESIAN_POINT('Ctrl Pts',(4.61039365599994,15.2,-9.36900394200002));
#165748=CARTESIAN_POINT('Ctrl Pts',(4.61039365599994,11.6,-9.36900394200002));
#165749=CARTESIAN_POINT('Ctrl Pts',(4.61119483299994,15.2,-9.37017521400002));
#165750=CARTESIAN_POINT('Ctrl Pts',(4.61119483299994,11.6,-9.37017521400002));
#165751=CARTESIAN_POINT('Ctrl Pts',(4.61200180799994,15.2,-9.37135254700001));
#165752=CARTESIAN_POINT('Ctrl Pts',(4.61200180799994,11.6,-9.37135254700001));
#165753=CARTESIAN_POINT('Ctrl Pts',(4.61281458299994,15.2,-9.37253591500001));
#165754=CARTESIAN_POINT('Ctrl Pts',(4.61281458299994,11.6,-9.37253591500001));
#165755=CARTESIAN_POINT('Ctrl Pts',(4.61363315799994,15.2,-9.37372529500001));
#165756=CARTESIAN_POINT('Ctrl Pts',(4.61363315799994,11.6,-9.37372529500001));
#165757=CARTESIAN_POINT('Ctrl Pts',(4.61445753499994,15.2,-9.37492066200001));
#165758=CARTESIAN_POINT('Ctrl Pts',(4.61445753499994,11.6,-9.37492066200001));
#165759=CARTESIAN_POINT('Ctrl Pts',(4.61528770999994,15.2,-9.37612198900002));
#165760=CARTESIAN_POINT('Ctrl Pts',(4.61528770999994,11.6,-9.37612198900002));
#165761=CARTESIAN_POINT('Ctrl Pts',(4.61612368799994,15.2,-9.37732925100002));
#165762=CARTESIAN_POINT('Ctrl Pts',(4.61612368799994,11.6,-9.37732925100002));
#165763=CARTESIAN_POINT('Ctrl Pts',(4.61696546699994,15.2,-9.37854242500002));
#165764=CARTESIAN_POINT('Ctrl Pts',(4.61696546699994,11.6,-9.37854242500002));
#165765=CARTESIAN_POINT('Ctrl Pts',(4.61781304699994,15.2,-9.37976148600002));
#165766=CARTESIAN_POINT('Ctrl Pts',(4.61781304699994,11.6,-9.37976148600002));
#165767=CARTESIAN_POINT('Ctrl Pts',(4.61866642999994,15.2,-9.38098640900002));
#165768=CARTESIAN_POINT('Ctrl Pts',(4.61866642999994,11.6,-9.38098640900002));
#165769=CARTESIAN_POINT('Ctrl Pts',(4.61952561499994,15.2,-9.38221716900001));
#165770=CARTESIAN_POINT('Ctrl Pts',(4.61952561499994,11.6,-9.38221716900001));
#165771=CARTESIAN_POINT('Ctrl Pts',(4.62039060399994,15.2,-9.38345374300001));
#165772=CARTESIAN_POINT('Ctrl Pts',(4.62039060399994,11.6,-9.38345374300001));
#165773=CARTESIAN_POINT('Ctrl Pts',(4.62126139499994,15.2,-9.38469610600002));
#165774=CARTESIAN_POINT('Ctrl Pts',(4.62126139499994,11.6,-9.38469610600002));
#165775=CARTESIAN_POINT('Ctrl Pts',(4.62213798999994,15.2,-9.38594423300002));
#165776=CARTESIAN_POINT('Ctrl Pts',(4.62213798999994,11.6,-9.38594423300002));
#165777=CARTESIAN_POINT('Ctrl Pts',(4.62302038999994,15.2,-9.38719810100002));
#165778=CARTESIAN_POINT('Ctrl Pts',(4.62302038999994,11.6,-9.38719810100002));
#165779=CARTESIAN_POINT('Ctrl Pts',(4.62390859299994,15.2,-9.38845768500002));
#165780=CARTESIAN_POINT('Ctrl Pts',(4.62390859299994,11.6,-9.38845768500002));
#165781=CARTESIAN_POINT('Ctrl Pts',(4.62480259899994,15.2,-9.38972296200001));
#165782=CARTESIAN_POINT('Ctrl Pts',(4.62480259899994,11.6,-9.38972296200001));
#165783=CARTESIAN_POINT('Ctrl Pts',(4.62570241199994,15.2,-9.39099390800001));
#165784=CARTESIAN_POINT('Ctrl Pts',(4.62570241199994,11.6,-9.39099390800001));
#165785=CARTESIAN_POINT('Ctrl Pts',(4.62660802799994,15.2,-9.39227050000002));
#165786=CARTESIAN_POINT('Ctrl Pts',(4.62660802799994,11.6,-9.39227050000002));
#165787=CARTESIAN_POINT('Ctrl Pts',(4.62751944999994,15.2,-9.39355271300002));
#165788=CARTESIAN_POINT('Ctrl Pts',(4.62751944999994,11.6,-9.39355271300002));
#165789=CARTESIAN_POINT('Ctrl Pts',(4.62843667699994,15.2,-9.39484052400001));
#165790=CARTESIAN_POINT('Ctrl Pts',(4.62843667699994,11.6,-9.39484052400001));
#165791=CARTESIAN_POINT('Ctrl Pts',(4.62935970899994,15.2,-9.39613391000002));
#165792=CARTESIAN_POINT('Ctrl Pts',(4.62935970899994,11.6,-9.39613391000002));
#165793=CARTESIAN_POINT('Ctrl Pts',(4.63028854799994,15.2,-9.39743284700001));
#165794=CARTESIAN_POINT('Ctrl Pts',(4.63028854799994,11.6,-9.39743284700001));
#165795=CARTESIAN_POINT('Ctrl Pts',(4.63122319099994,15.2,-9.39873731300001));
#165796=CARTESIAN_POINT('Ctrl Pts',(4.63122319099994,11.6,-9.39873731300001));
#165797=CARTESIAN_POINT('Ctrl Pts',(4.63216364099994,15.2,-9.40004728300002));
#165798=CARTESIAN_POINT('Ctrl Pts',(4.63216364099994,11.6,-9.40004728300002));
#165799=CARTESIAN_POINT('Ctrl Pts',(4.63310989699994,15.2,-9.40136273600002));
#165800=CARTESIAN_POINT('Ctrl Pts',(4.63310989699994,11.6,-9.40136273600002));
#165801=CARTESIAN_POINT('Ctrl Pts',(4.63406195899994,15.2,-9.40268364800002));
#165802=CARTESIAN_POINT('Ctrl Pts',(4.63406195899994,11.6,-9.40268364800002));
#165803=CARTESIAN_POINT('Ctrl Pts',(4.63501982699994,15.2,-9.40400999500002));
#165804=CARTESIAN_POINT('Ctrl Pts',(4.63501982699994,11.6,-9.40400999500002));
#165805=CARTESIAN_POINT('Ctrl Pts',(4.63598349999994,15.2,-9.40534175600002));
#165806=CARTESIAN_POINT('Ctrl Pts',(4.63598349999994,11.6,-9.40534175600002));
#165807=CARTESIAN_POINT('Ctrl Pts',(4.63695298199994,15.2,-9.40667890700002));
#165808=CARTESIAN_POINT('Ctrl Pts',(4.63695298199994,11.6,-9.40667890700002));
#165809=CARTESIAN_POINT('Ctrl Pts',(4.63792826799994,15.2,-9.40802142600001));
#165810=CARTESIAN_POINT('Ctrl Pts',(4.63792826799994,11.6,-9.40802142600001));
#165811=CARTESIAN_POINT('Ctrl Pts',(4.63890936299994,15.2,-9.40936929100002));
#165812=CARTESIAN_POINT('Ctrl Pts',(4.63890936299994,11.6,-9.40936929100002));
#165813=CARTESIAN_POINT('Ctrl Pts',(4.63989626199994,15.2,-9.41072247900001));
#165814=CARTESIAN_POINT('Ctrl Pts',(4.63989626199994,11.6,-9.41072247900001));
#165815=CARTESIAN_POINT('Ctrl Pts',(4.64088896899994,15.2,-9.41208096700001));
#165816=CARTESIAN_POINT('Ctrl Pts',(4.64088896899994,11.6,-9.41208096700001));
#165817=CARTESIAN_POINT('Ctrl Pts',(4.64188748399994,15.2,-9.41344473400001));
#165818=CARTESIAN_POINT('Ctrl Pts',(4.64188748399994,11.6,-9.41344473400001));
#165819=CARTESIAN_POINT('Ctrl Pts',(4.64289180299994,15.2,-9.41481375700001));
#165820=CARTESIAN_POINT('Ctrl Pts',(4.64289180299994,11.6,-9.41481375700001));
#165821=CARTESIAN_POINT('Ctrl Pts',(4.64390192999994,15.2,-9.41618801400002));
#165822=CARTESIAN_POINT('Ctrl Pts',(4.64390192999994,11.6,-9.41618801400002));
#165823=CARTESIAN_POINT('Ctrl Pts',(4.64491786299994,15.2,-9.41756748400002));
#165824=CARTESIAN_POINT('Ctrl Pts',(4.64491786299994,11.6,-9.41756748400002));
#165825=CARTESIAN_POINT('Ctrl Pts',(4.64593960299994,15.2,-9.41895214200001));
#165826=CARTESIAN_POINT('Ctrl Pts',(4.64593960299994,11.6,-9.41895214200001));
#165827=CARTESIAN_POINT('Ctrl Pts',(4.64696714999994,15.2,-9.42034197000002));
#165828=CARTESIAN_POINT('Ctrl Pts',(4.64696714999994,11.6,-9.42034197000002));
#165829=CARTESIAN_POINT('Ctrl Pts',(4.64800050299994,15.2,-9.42173694400001));
#165830=CARTESIAN_POINT('Ctrl Pts',(4.64800050299994,11.6,-9.42173694400001));
#165831=CARTESIAN_POINT('Ctrl Pts',(4.64903966199994,15.2,-9.42313704200001));
#165832=CARTESIAN_POINT('Ctrl Pts',(4.64903966199994,11.6,-9.42313704200001));
#165833=CARTESIAN_POINT('Ctrl Pts',(4.65008462699994,15.2,-9.42454224400001));
#165834=CARTESIAN_POINT('Ctrl Pts',(4.65008462699994,11.6,-9.42454224400001));
#165835=CARTESIAN_POINT('Ctrl Pts',(4.65113539899994,15.2,-9.42595252700002));
#165836=CARTESIAN_POINT('Ctrl Pts',(4.65113539899994,11.6,-9.42595252700002));
#165837=CARTESIAN_POINT('Ctrl Pts',(4.65219197599995,15.2,-9.42736787100002));
#165838=CARTESIAN_POINT('Ctrl Pts',(4.65219197599995,11.6,-9.42736787100002));
#165839=CARTESIAN_POINT('Ctrl Pts',(4.65325435999994,15.2,-9.42878825300001));
#165840=CARTESIAN_POINT('Ctrl Pts',(4.65325435999994,11.6,-9.42878825300001));
#165841=CARTESIAN_POINT('Ctrl Pts',(4.65432254899994,15.2,-9.43021365300002));
#165842=CARTESIAN_POINT('Ctrl Pts',(4.65432254899994,11.6,-9.43021365300002));
#165843=CARTESIAN_POINT('Ctrl Pts',(4.65539654399994,15.2,-9.43164405000001));
#165844=CARTESIAN_POINT('Ctrl Pts',(4.65539654399994,11.6,-9.43164405000001));
#165845=CARTESIAN_POINT('Ctrl Pts',(4.65647634499994,15.2,-9.43307942000001));
#165846=CARTESIAN_POINT('Ctrl Pts',(4.65647634499994,11.6,-9.43307942000001));
#165847=CARTESIAN_POINT('Ctrl Pts',(4.65756194999994,15.2,-9.43451974600002));
#165848=CARTESIAN_POINT('Ctrl Pts',(4.65756194999994,11.6,-9.43451974600002));
#165849=CARTESIAN_POINT('Ctrl Pts',(4.65865336199994,15.2,-9.43596500400002));
#165850=CARTESIAN_POINT('Ctrl Pts',(4.65865336199994,11.6,-9.43596500400002));
#165851=CARTESIAN_POINT('Ctrl Pts',(4.65975057699994,15.2,-9.43741517400002));
#165852=CARTESIAN_POINT('Ctrl Pts',(4.65975057699994,11.6,-9.43741517400002));
#165853=CARTESIAN_POINT('Ctrl Pts',(4.66085359799994,15.2,-9.43887023600002));
#165854=CARTESIAN_POINT('Ctrl Pts',(4.66085359799994,11.6,-9.43887023600002));
#165855=CARTESIAN_POINT('Ctrl Pts',(4.66196242299994,15.2,-9.44033016800002));
#165856=CARTESIAN_POINT('Ctrl Pts',(4.66196242299994,11.6,-9.44033016800002));
#165857=CARTESIAN_POINT('Ctrl Pts',(4.66307705199994,15.2,-9.44179494900002));
#165858=CARTESIAN_POINT('Ctrl Pts',(4.66307705199994,11.6,-9.44179494900002));
#165859=CARTESIAN_POINT('Ctrl Pts',(4.66419748599994,15.2,-9.44326456000002));
#165860=CARTESIAN_POINT('Ctrl Pts',(4.66419748599994,11.6,-9.44326456000002));
#165861=CARTESIAN_POINT('Ctrl Pts',(4.66532372199994,15.2,-9.44473898000001));
#165862=CARTESIAN_POINT('Ctrl Pts',(4.66532372199994,11.6,-9.44473898000001));
#165863=CARTESIAN_POINT('Ctrl Pts',(4.66645576299995,15.2,-9.44621818800002));
#165864=CARTESIAN_POINT('Ctrl Pts',(4.66645576299995,11.6,-9.44621818800002));
#165865=CARTESIAN_POINT('Ctrl Pts',(4.66759360699994,15.2,-9.44770216300002));
#165866=CARTESIAN_POINT('Ctrl Pts',(4.66759360699994,11.6,-9.44770216300002));
#165867=CARTESIAN_POINT('Ctrl Pts',(4.66873725299994,15.2,-9.44919088600002));
#165868=CARTESIAN_POINT('Ctrl Pts',(4.66873725299994,11.6,-9.44919088600002));
#165869=CARTESIAN_POINT('Ctrl Pts',(4.66988670199994,15.2,-9.45068433600002));
#165870=CARTESIAN_POINT('Ctrl Pts',(4.66988670199994,11.6,-9.45068433600002));
#165871=CARTESIAN_POINT('Ctrl Pts',(4.67104195499994,15.2,-9.45218249400002));
#165872=CARTESIAN_POINT('Ctrl Pts',(4.67104195499994,11.6,-9.45218249400002));
#165873=CARTESIAN_POINT('Ctrl Pts',(4.67220300799994,15.2,-9.45368533800002));
#165874=CARTESIAN_POINT('Ctrl Pts',(4.67220300799994,11.6,-9.45368533800002));
#165875=CARTESIAN_POINT('Ctrl Pts',(4.67336986399994,15.2,-9.45519284900002));
#165876=CARTESIAN_POINT('Ctrl Pts',(4.67336986399994,11.6,-9.45519284900002));
#165877=CARTESIAN_POINT('Ctrl Pts',(4.67454251999994,15.2,-9.45670500700002));
#165878=CARTESIAN_POINT('Ctrl Pts',(4.67454251999994,11.6,-9.45670500700002));
#165879=CARTESIAN_POINT('Ctrl Pts',(4.67572097799994,15.2,-9.45822179200002));
#165880=CARTESIAN_POINT('Ctrl Pts',(4.67572097799994,11.6,-9.45822179200002));
#165881=CARTESIAN_POINT('Ctrl Pts',(4.67690523599994,15.2,-9.45974318300001));
#165882=CARTESIAN_POINT('Ctrl Pts',(4.67690523599994,11.6,-9.45974318300001));
#165883=CARTESIAN_POINT('Ctrl Pts',(4.67809529399994,15.2,-9.46126916300001));
#165884=CARTESIAN_POINT('Ctrl Pts',(4.67809529399994,11.6,-9.46126916300001));
#165885=CARTESIAN_POINT('Ctrl Pts',(4.67929115299994,15.2,-9.46279970900001));
#165886=CARTESIAN_POINT('Ctrl Pts',(4.67929115299994,11.6,-9.46279970900001));
#165887=CARTESIAN_POINT('Ctrl Pts',(4.68049280999994,15.2,-9.46433480500002));
#165888=CARTESIAN_POINT('Ctrl Pts',(4.68049280999994,11.6,-9.46433480500002));
#165889=CARTESIAN_POINT('Ctrl Pts',(4.68170026699995,15.2,-9.46587442800002));
#165890=CARTESIAN_POINT('Ctrl Pts',(4.68170026699995,11.6,-9.46587442800002));
#165891=CARTESIAN_POINT('Ctrl Pts',(4.68291352099994,15.2,-9.46741856000001));
#165892=CARTESIAN_POINT('Ctrl Pts',(4.68291352099994,11.6,-9.46741856000001));
#165893=CARTESIAN_POINT('Ctrl Pts',(4.68413257499994,15.2,-9.46896718200002));
#165894=CARTESIAN_POINT('Ctrl Pts',(4.68413257499994,11.6,-9.46896718200002));
#165895=CARTESIAN_POINT('Ctrl Pts',(4.68535742699994,15.2,-9.47052027400002));
#165896=CARTESIAN_POINT('Ctrl Pts',(4.68535742699994,11.6,-9.47052027400002));
#165897=CARTESIAN_POINT('Ctrl Pts',(4.68658807499994,15.2,-9.47207781700002));
#165898=CARTESIAN_POINT('Ctrl Pts',(4.68658807499994,11.6,-9.47207781700002));
#165899=CARTESIAN_POINT('Ctrl Pts',(4.68782451899994,15.2,-9.47363979200002));
#165900=CARTESIAN_POINT('Ctrl Pts',(4.68782451899994,11.6,-9.47363979200002));
#165901=CARTESIAN_POINT('Ctrl Pts',(4.68906676199994,15.2,-9.47520617900001));
#165902=CARTESIAN_POINT('Ctrl Pts',(4.68906676199994,11.6,-9.47520617900001));
#165903=CARTESIAN_POINT('Ctrl Pts',(4.69031479799994,15.2,-9.47677695900002));
#165904=CARTESIAN_POINT('Ctrl Pts',(4.69031479799994,11.6,-9.47677695900002));
#165905=CARTESIAN_POINT('Ctrl Pts',(4.69156863099994,15.2,-9.47835211400001));
#165906=CARTESIAN_POINT('Ctrl Pts',(4.69156863099994,11.6,-9.47835211400001));
#165907=CARTESIAN_POINT('Ctrl Pts',(4.69282825799994,15.2,-9.47993162400002));
#165908=CARTESIAN_POINT('Ctrl Pts',(4.69282825799994,11.6,-9.47993162400002));
#165909=CARTESIAN_POINT('Ctrl Pts',(4.69409367999994,15.2,-9.48151547000002));
#165910=CARTESIAN_POINT('Ctrl Pts',(4.69409367999994,11.6,-9.48151547000002));
#165911=CARTESIAN_POINT('Ctrl Pts',(4.69536489499994,15.2,-9.48310363400001));
#165912=CARTESIAN_POINT('Ctrl Pts',(4.69536489499994,11.6,-9.48310363400001));
#165913=CARTESIAN_POINT('Ctrl Pts',(4.69664190399994,15.2,-9.48469609800001));
#165914=CARTESIAN_POINT('Ctrl Pts',(4.69664190399994,11.6,-9.48469609800001));
#165915=CARTESIAN_POINT('Ctrl Pts',(4.69792470499994,15.2,-9.48629284000001));
#165916=CARTESIAN_POINT('Ctrl Pts',(4.69792470499994,11.6,-9.48629284000001));
#165917=CARTESIAN_POINT('Ctrl Pts',(4.69921329899994,15.2,-9.48789384500002));
#165918=CARTESIAN_POINT('Ctrl Pts',(4.69921329899994,11.6,-9.48789384500002));
#165919=CARTESIAN_POINT('Ctrl Pts',(4.70050768499994,15.2,-9.48949909200002));
#165920=CARTESIAN_POINT('Ctrl Pts',(4.70050768499994,11.6,-9.48949909200002));
#165921=CARTESIAN_POINT('Ctrl Pts',(4.70180786099994,15.2,-9.49110856300001));
#165922=CARTESIAN_POINT('Ctrl Pts',(4.70180786099994,11.6,-9.49110856300001));
#165923=CARTESIAN_POINT('Ctrl Pts',(4.70311382699994,15.2,-9.49272224000002));
#165924=CARTESIAN_POINT('Ctrl Pts',(4.70311382699994,11.6,-9.49272224000002));
#165925=CARTESIAN_POINT('Ctrl Pts',(4.70442558399994,15.2,-9.49434010500001));
#165926=CARTESIAN_POINT('Ctrl Pts',(4.70442558399994,11.6,-9.49434010500001));
#165927=CARTESIAN_POINT('Ctrl Pts',(4.70574312999995,15.2,-9.49596213800002));
#165928=CARTESIAN_POINT('Ctrl Pts',(4.70574312999995,11.6,-9.49596213800002));
#165929=CARTESIAN_POINT('Ctrl Pts',(4.70706646299994,15.2,-9.49758832300001));
#165930=CARTESIAN_POINT('Ctrl Pts',(4.70706646299994,11.6,-9.49758832300001));
#165931=CARTESIAN_POINT('Ctrl Pts',(4.70839558499994,15.2,-9.49921863900002));
#165932=CARTESIAN_POINT('Ctrl Pts',(4.70839558499994,11.6,-9.49921863900002));
#165933=CARTESIAN_POINT('Ctrl Pts',(4.70973049599994,15.2,-9.50085307000002));
#165934=CARTESIAN_POINT('Ctrl Pts',(4.70973049599994,11.6,-9.50085307000002));
#165935=CARTESIAN_POINT('Ctrl Pts',(4.71107119199994,15.2,-9.50249159800002));
#165936=CARTESIAN_POINT('Ctrl Pts',(4.71107119199994,11.6,-9.50249159800002));
#165937=CARTESIAN_POINT('Ctrl Pts',(4.71241767399994,15.2,-9.50413420300002));
#165938=CARTESIAN_POINT('Ctrl Pts',(4.71241767399994,11.6,-9.50413420300002));
#165939=CARTESIAN_POINT('Ctrl Pts',(4.71376994199994,15.2,-9.50578086900002));
#165940=CARTESIAN_POINT('Ctrl Pts',(4.71376994199994,11.6,-9.50578086900002));
#165941=CARTESIAN_POINT('Ctrl Pts',(4.71512799299994,15.2,-9.50743157700002));
#165942=CARTESIAN_POINT('Ctrl Pts',(4.71512799299994,11.6,-9.50743157700002));
#165943=CARTESIAN_POINT('Ctrl Pts',(4.71649182999994,15.2,-9.50908630800001));
#165944=CARTESIAN_POINT('Ctrl Pts',(4.71649182999994,11.6,-9.50908630800001));
#165945=CARTESIAN_POINT('Ctrl Pts',(4.71786144899994,15.2,-9.51074504700001));
#165946=CARTESIAN_POINT('Ctrl Pts',(4.71786144899994,11.6,-9.51074504700001));
#165947=CARTESIAN_POINT('Ctrl Pts',(4.71923685099994,15.2,-9.51240777300002));
#165948=CARTESIAN_POINT('Ctrl Pts',(4.71923685099994,11.6,-9.51240777300002));
#165949=CARTESIAN_POINT('Ctrl Pts',(4.72061803499994,15.2,-9.51407447200001));
#165950=CARTESIAN_POINT('Ctrl Pts',(4.72061803499994,11.6,-9.51407447200001));
#165951=CARTESIAN_POINT('Ctrl Pts',(4.72200500099994,15.2,-9.51574512200001));
#165952=CARTESIAN_POINT('Ctrl Pts',(4.72200500099994,11.6,-9.51574512200001));
#165953=CARTESIAN_POINT('Ctrl Pts',(4.72339774699994,15.2,-9.51741970900001));
#165954=CARTESIAN_POINT('Ctrl Pts',(4.72339774699994,11.6,-9.51741970900001));
#165955=CARTESIAN_POINT('Ctrl Pts',(4.72479627199994,15.2,-9.51909821400001));
#165956=CARTESIAN_POINT('Ctrl Pts',(4.72479627199994,11.6,-9.51909821400001));
#165957=CARTESIAN_POINT('Ctrl Pts',(4.72620057599995,15.2,-9.52078061900002));
#165958=CARTESIAN_POINT('Ctrl Pts',(4.72620057599995,11.6,-9.52078061900002));
#165959=CARTESIAN_POINT('Ctrl Pts',(4.72761065899994,15.2,-9.52246690800001));
#165960=CARTESIAN_POINT('Ctrl Pts',(4.72761065899994,11.6,-9.52246690800001));
#165961=CARTESIAN_POINT('Ctrl Pts',(4.72902651799994,15.2,-9.52415706400001));
#165962=CARTESIAN_POINT('Ctrl Pts',(4.72902651799994,11.6,-9.52415706400001));
#165963=CARTESIAN_POINT('Ctrl Pts',(4.73044815599994,15.2,-9.52585106600001));
#165964=CARTESIAN_POINT('Ctrl Pts',(4.73044815599994,11.6,-9.52585106600001));
#165965=CARTESIAN_POINT('Ctrl Pts',(4.73187556799994,15.2,-9.52754890000002));
#165966=CARTESIAN_POINT('Ctrl Pts',(4.73187556799994,11.6,-9.52754890000002));
#165967=CARTESIAN_POINT('Ctrl Pts',(4.73330875499994,15.2,-9.52925054800002));
#165968=CARTESIAN_POINT('Ctrl Pts',(4.73330875499994,11.6,-9.52925054800002));
#165969=CARTESIAN_POINT('Ctrl Pts',(4.73474771699994,15.2,-9.53095599300001));
#165970=CARTESIAN_POINT('Ctrl Pts',(4.73474771699994,11.6,-9.53095599300001));
#165971=CARTESIAN_POINT('Ctrl Pts',(4.73619245199994,15.2,-9.53266521700002));
#165972=CARTESIAN_POINT('Ctrl Pts',(4.73619245199994,11.6,-9.53266521700002));
#165973=CARTESIAN_POINT('Ctrl Pts',(4.73764295999994,15.2,-9.53437820500002));
#165974=CARTESIAN_POINT('Ctrl Pts',(4.73764295999994,11.6,-9.53437820500002));
#165975=CARTESIAN_POINT('Ctrl Pts',(4.73909923899994,15.2,-9.53609493800002));
#165976=CARTESIAN_POINT('Ctrl Pts',(4.73909923899994,11.6,-9.53609493800002));
#165977=CARTESIAN_POINT('Ctrl Pts',(4.74056128899994,15.2,-9.53781539900002));
#165978=CARTESIAN_POINT('Ctrl Pts',(4.74056128899994,11.6,-9.53781539900002));
#165979=CARTESIAN_POINT('Ctrl Pts',(4.74202910999994,15.2,-9.53953957200002));
#165980=CARTESIAN_POINT('Ctrl Pts',(4.74202910999994,11.6,-9.53953957200002));
#165981=CARTESIAN_POINT('Ctrl Pts',(4.74350269999994,15.2,-9.54126744100002));
#165982=CARTESIAN_POINT('Ctrl Pts',(4.74350269999994,11.6,-9.54126744100002));
#165983=CARTESIAN_POINT('Ctrl Pts',(4.74498205799994,15.2,-9.54299898700001));
#165984=CARTESIAN_POINT('Ctrl Pts',(4.74498205799994,11.6,-9.54299898700001));
#165985=CARTESIAN_POINT('Ctrl Pts',(4.74646718399994,15.2,-9.54473419300001));
#165986=CARTESIAN_POINT('Ctrl Pts',(4.74646718399994,11.6,-9.54473419300001));
#165987=CARTESIAN_POINT('Ctrl Pts',(4.74795807699994,15.2,-9.54647304600002));
#165988=CARTESIAN_POINT('Ctrl Pts',(4.74795807699994,11.6,-9.54647304600002));
#165989=CARTESIAN_POINT('Ctrl Pts',(4.74945473399994,15.2,-9.54821552600002));
#165990=CARTESIAN_POINT('Ctrl Pts',(4.74945473399994,11.6,-9.54821552600002));
#165991=CARTESIAN_POINT('Ctrl Pts',(4.75095715699994,15.2,-9.54996161800001));
#165992=CARTESIAN_POINT('Ctrl Pts',(4.75095715699994,11.6,-9.54996161800001));
#165993=CARTESIAN_POINT('Ctrl Pts',(4.75246534399994,15.2,-9.55171130300002));
#165994=CARTESIAN_POINT('Ctrl Pts',(4.75246534399994,11.6,-9.55171130300002));
#165995=CARTESIAN_POINT('Ctrl Pts',(4.75397929399994,15.2,-9.55346456800001));
#165996=CARTESIAN_POINT('Ctrl Pts',(4.75397929399994,11.6,-9.55346456800001));
#165997=CARTESIAN_POINT('Ctrl Pts',(4.75549900499994,15.2,-9.55522139300001));
#165998=CARTESIAN_POINT('Ctrl Pts',(4.75549900499994,11.6,-9.55522139300001));
#165999=CARTESIAN_POINT('Ctrl Pts',(4.75702447799994,15.2,-9.55698176500002));
#166000=CARTESIAN_POINT('Ctrl Pts',(4.75702447799994,11.6,-9.55698176500002));
#166001=CARTESIAN_POINT('Ctrl Pts',(4.75855571099994,15.2,-9.55874566600002));
#166002=CARTESIAN_POINT('Ctrl Pts',(4.75855571099994,11.6,-9.55874566600002));
#166003=CARTESIAN_POINT('Ctrl Pts',(4.76009270299994,15.2,-9.56051308000001));
#166004=CARTESIAN_POINT('Ctrl Pts',(4.76009270299994,11.6,-9.56051308000001));
#166005=CARTESIAN_POINT('Ctrl Pts',(4.76163545499994,15.2,-9.56228399000001));
#166006=CARTESIAN_POINT('Ctrl Pts',(4.76163545499994,11.6,-9.56228399000001));
#166007=CARTESIAN_POINT('Ctrl Pts',(4.76318396199994,15.2,-9.56405838000002));
#166008=CARTESIAN_POINT('Ctrl Pts',(4.76318396199994,11.6,-9.56405838000002));
#166009=CARTESIAN_POINT('Ctrl Pts',(4.76473822699994,15.2,-9.56583623400002));
#166010=CARTESIAN_POINT('Ctrl Pts',(4.76473822699994,11.6,-9.56583623400002));
#166011=CARTESIAN_POINT('Ctrl Pts',(4.76629824599994,15.2,-9.56761753600002));
#166012=CARTESIAN_POINT('Ctrl Pts',(4.76629824599994,11.6,-9.56761753600002));
#166013=CARTESIAN_POINT('Ctrl Pts',(4.76786401999994,15.2,-9.56940227100001));
#166014=CARTESIAN_POINT('Ctrl Pts',(4.76786401999994,11.6,-9.56940227100001));
#166015=CARTESIAN_POINT('Ctrl Pts',(4.76943554699994,15.2,-9.57119042200001));
#166016=CARTESIAN_POINT('Ctrl Pts',(4.76943554699994,11.6,-9.57119042200001));
#166017=CARTESIAN_POINT('Ctrl Pts',(4.77101282699994,15.2,-9.57298197200002));
#166018=CARTESIAN_POINT('Ctrl Pts',(4.77101282699994,11.6,-9.57298197200002));
#166019=CARTESIAN_POINT('Ctrl Pts',(4.77259585799994,15.2,-9.57477690600001));
#166020=CARTESIAN_POINT('Ctrl Pts',(4.77259585799994,11.6,-9.57477690600001));
#166021=CARTESIAN_POINT('Ctrl Pts',(4.77418463899994,15.2,-9.57657520900002));
#166022=CARTESIAN_POINT('Ctrl Pts',(4.77418463899994,11.6,-9.57657520900002));
#166023=CARTESIAN_POINT('Ctrl Pts',(4.77577916999994,15.2,-9.57837686300002));
#166024=CARTESIAN_POINT('Ctrl Pts',(4.77577916999994,11.6,-9.57837686300002));
#166025=CARTESIAN_POINT('Ctrl Pts',(4.77737944799994,15.2,-9.58018185500002));
#166026=CARTESIAN_POINT('Ctrl Pts',(4.77737944799994,11.6,-9.58018185500002));
#166027=CARTESIAN_POINT('Ctrl Pts',(4.77898547399994,15.2,-9.58199016600001));
#166028=CARTESIAN_POINT('Ctrl Pts',(4.77898547399994,11.6,-9.58199016600001));
#166029=CARTESIAN_POINT('Ctrl Pts',(4.78059724599994,15.2,-9.58380178400001));
#166030=CARTESIAN_POINT('Ctrl Pts',(4.78059724599994,11.6,-9.58380178400001));
#166031=CARTESIAN_POINT('Ctrl Pts',(4.78221476399994,15.2,-9.58561669000002));
#166032=CARTESIAN_POINT('Ctrl Pts',(4.78221476399994,11.6,-9.58561669000002));
#166033=CARTESIAN_POINT('Ctrl Pts',(4.78383802499994,15.2,-9.58743487100002));
#166034=CARTESIAN_POINT('Ctrl Pts',(4.78383802499994,11.6,-9.58743487100002));
#166035=CARTESIAN_POINT('Ctrl Pts',(4.78546702799994,15.2,-9.58925631000002));
#166036=CARTESIAN_POINT('Ctrl Pts',(4.78546702799994,11.6,-9.58925631000002));
#166037=CARTESIAN_POINT('Ctrl Pts',(4.78710177399994,15.2,-9.59108099200002));
#166038=CARTESIAN_POINT('Ctrl Pts',(4.78710177399994,11.6,-9.59108099200002));
#166039=CARTESIAN_POINT('Ctrl Pts',(4.78874226099994,15.2,-9.59290890100002));
#166040=CARTESIAN_POINT('Ctrl Pts',(4.78874226099994,11.6,-9.59290890100002));
#166041=CARTESIAN_POINT('Ctrl Pts',(4.79038848599994,15.2,-9.59474002200002));
#166042=CARTESIAN_POINT('Ctrl Pts',(4.79038848599994,11.6,-9.59474002200002));
#166043=CARTESIAN_POINT('Ctrl Pts',(4.79204045099995,15.2,-9.59657434000002));
#166044=CARTESIAN_POINT('Ctrl Pts',(4.79204045099995,11.6,-9.59657434000002));
#166045=CARTESIAN_POINT('Ctrl Pts',(4.79369815299994,15.2,-9.59841183800001));
#166046=CARTESIAN_POINT('Ctrl Pts',(4.79369815299994,11.6,-9.59841183800001));
#166047=CARTESIAN_POINT('Ctrl Pts',(4.79536159199994,15.2,-9.60025250200001));
#166048=CARTESIAN_POINT('Ctrl Pts',(4.79536159199994,11.6,-9.60025250200001));
#166049=CARTESIAN_POINT('Ctrl Pts',(4.79703076399994,15.2,-9.60209631800002));
#166050=CARTESIAN_POINT('Ctrl Pts',(4.79703076399994,11.6,-9.60209631800002));
#166051=CARTESIAN_POINT('Ctrl Pts',(4.79870567099994,15.2,-9.60394326800002));
#166052=CARTESIAN_POINT('Ctrl Pts',(4.79870567099994,11.6,-9.60394326800002));
#166053=CARTESIAN_POINT('Ctrl Pts',(4.80038631199994,15.2,-9.60579333900002));
#166054=CARTESIAN_POINT('Ctrl Pts',(4.80038631199994,11.6,-9.60579333900002));
#166055=CARTESIAN_POINT('Ctrl Pts',(4.80207268399994,15.2,-9.60764651500002));
#166056=CARTESIAN_POINT('Ctrl Pts',(4.80207268399994,11.6,-9.60764651500002));
#166057=CARTESIAN_POINT('Ctrl Pts',(4.80376478599994,15.2,-9.60950278000002));
#166058=CARTESIAN_POINT('Ctrl Pts',(4.80376478599994,11.6,-9.60950278000002));
#166059=CARTESIAN_POINT('Ctrl Pts',(4.80546261699994,15.2,-9.61136212100002));
#166060=CARTESIAN_POINT('Ctrl Pts',(4.80546261699994,11.6,-9.61136212100002));
#166061=CARTESIAN_POINT('Ctrl Pts',(4.80716617699994,15.2,-9.61322452200001));
#166062=CARTESIAN_POINT('Ctrl Pts',(4.80716617699994,11.6,-9.61322452200001));
#166063=CARTESIAN_POINT('Ctrl Pts',(4.80887546399994,15.2,-9.61508996800001));
#166064=CARTESIAN_POINT('Ctrl Pts',(4.80887546399994,11.6,-9.61508996800001));
#166065=CARTESIAN_POINT('Ctrl Pts',(4.81059047599994,15.2,-9.61695844400002));
#166066=CARTESIAN_POINT('Ctrl Pts',(4.81059047599994,11.6,-9.61695844400002));
#166067=CARTESIAN_POINT('Ctrl Pts',(4.81231121399994,15.2,-9.61882993500002));
#166068=CARTESIAN_POINT('Ctrl Pts',(4.81231121399994,11.6,-9.61882993500002));
#166069=CARTESIAN_POINT('Ctrl Pts',(4.81403767399994,15.2,-9.62070442600002));
#166070=CARTESIAN_POINT('Ctrl Pts',(4.81403767399994,11.6,-9.62070442600002));
#166071=CARTESIAN_POINT('Ctrl Pts',(4.81576985699994,15.2,-9.62258190400001));
#166072=CARTESIAN_POINT('Ctrl Pts',(4.81576985699994,11.6,-9.62258190400001));
#166073=CARTESIAN_POINT('Ctrl Pts',(4.81750775999994,15.2,-9.62446235200002));
#166074=CARTESIAN_POINT('Ctrl Pts',(4.81750775999994,11.6,-9.62446235200002));
#166075=CARTESIAN_POINT('Ctrl Pts',(4.81925138399994,15.2,-9.62634575600001));
#166076=CARTESIAN_POINT('Ctrl Pts',(4.81925138399994,11.6,-9.62634575600001));
#166077=CARTESIAN_POINT('Ctrl Pts',(4.82100072499994,15.2,-9.62823210100002));
#166078=CARTESIAN_POINT('Ctrl Pts',(4.82100072499994,11.6,-9.62823210100002));
#166079=CARTESIAN_POINT('Ctrl Pts',(4.82275578399994,15.2,-9.63012137400002));
#166080=CARTESIAN_POINT('Ctrl Pts',(4.82275578399994,11.6,-9.63012137400002));
#166081=CARTESIAN_POINT('Ctrl Pts',(4.82451655899994,15.2,-9.63201355900001));
#166082=CARTESIAN_POINT('Ctrl Pts',(4.82451655899994,11.6,-9.63201355900001));
#166083=CARTESIAN_POINT('Ctrl Pts',(4.82628304799994,15.2,-9.63390864100001));
#166084=CARTESIAN_POINT('Ctrl Pts',(4.82628304799994,11.6,-9.63390864100001));
#166085=CARTESIAN_POINT('Ctrl Pts',(4.82805525099994,15.2,-9.63580660800002));
#166086=CARTESIAN_POINT('Ctrl Pts',(4.82805525099994,11.6,-9.63580660800002));
#166087=CARTESIAN_POINT('Ctrl Pts',(4.82983316599994,15.2,-9.63770744200002));
#166088=CARTESIAN_POINT('Ctrl Pts',(4.82983316599994,11.6,-9.63770744200002));
#166089=CARTESIAN_POINT('Ctrl Pts',(4.83161679299994,15.2,-9.63961113100002));
#166090=CARTESIAN_POINT('Ctrl Pts',(4.83161679299994,11.6,-9.63961113100002));
#166091=CARTESIAN_POINT('Ctrl Pts',(4.83340612799994,15.2,-9.64151766000001));
#166092=CARTESIAN_POINT('Ctrl Pts',(4.83340612799994,11.6,-9.64151766000001));
#166093=CARTESIAN_POINT('Ctrl Pts',(4.83520117199994,15.2,-9.64342701400002));
#166094=CARTESIAN_POINT('Ctrl Pts',(4.83520117199994,11.6,-9.64342701400002));
#166095=CARTESIAN_POINT('Ctrl Pts',(4.83700192299994,15.2,-9.64533918000001));
#166096=CARTESIAN_POINT('Ctrl Pts',(4.83700192299994,11.6,-9.64533918000001));
#166097=CARTESIAN_POINT('Ctrl Pts',(4.83880837899994,15.2,-9.64725414200002));
#166098=CARTESIAN_POINT('Ctrl Pts',(4.83880837899994,11.6,-9.64725414200002));
#166099=CARTESIAN_POINT('Ctrl Pts',(4.84062053999994,15.2,-9.64917188800002));
#166100=CARTESIAN_POINT('Ctrl Pts',(4.84062053999994,11.6,-9.64917188800002));
#166101=CARTESIAN_POINT('Ctrl Pts',(4.84243840399994,15.2,-9.65109240200002));
#166102=CARTESIAN_POINT('Ctrl Pts',(4.84243840399994,11.6,-9.65109240200002));
#166103=CARTESIAN_POINT('Ctrl Pts',(4.84426196999994,15.2,-9.65301567000001));
#166104=CARTESIAN_POINT('Ctrl Pts',(4.84426196999994,11.6,-9.65301567000001));
#166105=CARTESIAN_POINT('Ctrl Pts',(4.84609123599994,15.2,-9.65494167900001));
#166106=CARTESIAN_POINT('Ctrl Pts',(4.84609123599994,11.6,-9.65494167900001));
#166107=CARTESIAN_POINT('Ctrl Pts',(4.84792620099994,15.2,-9.65687041400001));
#166108=CARTESIAN_POINT('Ctrl Pts',(4.84792620099994,11.6,-9.65687041400001));
#166109=CARTESIAN_POINT('Ctrl Pts',(4.84976686399994,15.2,-9.65880186000001));
#166110=CARTESIAN_POINT('Ctrl Pts',(4.84976686399994,11.6,-9.65880186000001));
#166111=CARTESIAN_POINT('Ctrl Pts',(4.85161322299994,15.2,-9.66073600600001));
#166112=CARTESIAN_POINT('Ctrl Pts',(4.85161322299994,11.6,-9.66073600600001));
#166113=CARTESIAN_POINT('Ctrl Pts',(4.85346527699994,15.2,-9.66267283500001));
#166114=CARTESIAN_POINT('Ctrl Pts',(4.85346527699994,11.6,-9.66267283500001));
#166115=CARTESIAN_POINT('Ctrl Pts',(4.85532302399994,15.2,-9.66461233400001));
#166116=CARTESIAN_POINT('Ctrl Pts',(4.85532302399994,11.6,-9.66461233400001));
#166117=CARTESIAN_POINT('Ctrl Pts',(4.85718646499994,15.2,-9.66655449000001));
#166118=CARTESIAN_POINT('Ctrl Pts',(4.85718646499994,11.6,-9.66655449000001));
#166119=CARTESIAN_POINT('Ctrl Pts',(4.85905559499994,15.2,-9.66849928700001));
#166120=CARTESIAN_POINT('Ctrl Pts',(4.85905559499994,11.6,-9.66849928700001));
#166121=CARTESIAN_POINT('Ctrl Pts',(4.86093041599994,15.2,-9.67044671400001));
#166122=CARTESIAN_POINT('Ctrl Pts',(4.86093041599994,11.6,-9.67044671400001));
#166123=CARTESIAN_POINT('Ctrl Pts',(4.86281092399994,15.2,-9.67239675600001));
#166124=CARTESIAN_POINT('Ctrl Pts',(4.86281092399994,11.6,-9.67239675600001));
#166125=CARTESIAN_POINT('Ctrl Pts',(4.86469711899994,15.2,-9.67434939900001));
#166126=CARTESIAN_POINT('Ctrl Pts',(4.86469711899994,11.6,-9.67434939900001));
#166127=CARTESIAN_POINT('Ctrl Pts',(4.86658899899994,15.2,-9.67630462800001));
#166128=CARTESIAN_POINT('Ctrl Pts',(4.86658899899994,11.6,-9.67630462800001));
#166129=CARTESIAN_POINT('Ctrl Pts',(4.86848656299994,15.2,-9.67826243200001));
#166130=CARTESIAN_POINT('Ctrl Pts',(4.86848656299994,11.6,-9.67826243200001));
#166131=CARTESIAN_POINT('Ctrl Pts',(4.87038980999994,15.2,-9.68022279600001));
#166132=CARTESIAN_POINT('Ctrl Pts',(4.87038980999994,11.6,-9.68022279600001));
#166133=CARTESIAN_POINT('Ctrl Pts',(4.87229873699994,15.2,-9.68218570600001));
#166134=CARTESIAN_POINT('Ctrl Pts',(4.87229873699994,11.6,-9.68218570600001));
#166135=CARTESIAN_POINT('Ctrl Pts',(4.87421334399994,15.2,-9.68415114900001));
#166136=CARTESIAN_POINT('Ctrl Pts',(4.87421334399994,11.6,-9.68415114900001));
#166137=CARTESIAN_POINT('Ctrl Pts',(4.87613362999994,15.2,-9.68611911100002));
#166138=CARTESIAN_POINT('Ctrl Pts',(4.87613362999994,11.6,-9.68611911100002));
#166139=CARTESIAN_POINT('Ctrl Pts',(4.87805959199994,15.2,-9.68808957900001));
#166140=CARTESIAN_POINT('Ctrl Pts',(4.87805959199994,11.6,-9.68808957900001));
#166141=CARTESIAN_POINT('Ctrl Pts',(4.87999122899994,15.2,-9.69006253800002));
#166142=CARTESIAN_POINT('Ctrl Pts',(4.87999122899994,11.6,-9.69006253800002));
#166143=CARTESIAN_POINT('Ctrl Pts',(4.88192853999994,15.2,-9.69203797700001));
#166144=CARTESIAN_POINT('Ctrl Pts',(4.88192853999994,11.6,-9.69203797700001));
#166145=CARTESIAN_POINT('Ctrl Pts',(4.88387152299994,15.2,-9.69401588200001));
#166146=CARTESIAN_POINT('Ctrl Pts',(4.88387152299994,11.6,-9.69401588200001));
#166147=CARTESIAN_POINT('Ctrl Pts',(4.88582017699994,15.2,-9.69599623800001));
#166148=CARTESIAN_POINT('Ctrl Pts',(4.88582017699994,11.6,-9.69599623800001));
#166149=CARTESIAN_POINT('Ctrl Pts',(4.88777449999994,15.2,-9.69797903400002));
#166150=CARTESIAN_POINT('Ctrl Pts',(4.88777449999994,11.6,-9.69797903400002));
#166151=CARTESIAN_POINT('Ctrl Pts',(4.88973449199994,15.2,-9.69996425500001));
#166152=CARTESIAN_POINT('Ctrl Pts',(4.88973449199994,11.6,-9.69996425500001));
#166153=CARTESIAN_POINT('Ctrl Pts',(4.89170014899994,15.2,-9.70195188700002));
#166154=CARTESIAN_POINT('Ctrl Pts',(4.89170014899994,11.6,-9.70195188700002));
#166155=CARTESIAN_POINT('Ctrl Pts',(4.89367147099994,15.2,-9.70394192000001));
#166156=CARTESIAN_POINT('Ctrl Pts',(4.89367147099994,11.6,-9.70394192000001));
#166157=CARTESIAN_POINT('Ctrl Pts',(4.89564845699994,15.2,-9.70593433700001));
#166158=CARTESIAN_POINT('Ctrl Pts',(4.89564845699994,11.6,-9.70593433700001));
#166159=CARTESIAN_POINT('Ctrl Pts',(4.89763110499994,15.2,-9.70792912700001));
#166160=CARTESIAN_POINT('Ctrl Pts',(4.89763110499994,11.6,-9.70792912700001));
#166161=CARTESIAN_POINT('Ctrl Pts',(4.89961941299994,15.2,-9.70992627700001));
#166162=CARTESIAN_POINT('Ctrl Pts',(4.89961941299994,11.6,-9.70992627700001));
#166163=CARTESIAN_POINT('Ctrl Pts',(4.90161337899994,15.2,-9.71192577200001));
#166164=CARTESIAN_POINT('Ctrl Pts',(4.90161337899994,11.6,-9.71192577200001));
#166165=CARTESIAN_POINT('Ctrl Pts',(4.90361300299994,15.2,-9.71392760200001));
#166166=CARTESIAN_POINT('Ctrl Pts',(4.90361300299994,11.6,-9.71392760200001));
#166167=CARTESIAN_POINT('Ctrl Pts',(4.90561828399994,15.2,-9.71593175000001));
#166168=CARTESIAN_POINT('Ctrl Pts',(4.90561828399994,11.6,-9.71593175000001));
#166169=CARTESIAN_POINT('Ctrl Pts',(4.90762921799994,15.2,-9.71793820800001));
#166170=CARTESIAN_POINT('Ctrl Pts',(4.90762921799994,11.6,-9.71793820800001));
#166171=CARTESIAN_POINT('Ctrl Pts',(4.90964580399994,15.2,-9.71994695800001));
#166172=CARTESIAN_POINT('Ctrl Pts',(4.90964580399994,11.6,-9.71994695800001));
#166173=CARTESIAN_POINT('Ctrl Pts',(4.91166804199994,15.2,-9.72195799000001));
#166174=CARTESIAN_POINT('Ctrl Pts',(4.91166804199994,11.6,-9.72195799000001));
#166175=CARTESIAN_POINT('Ctrl Pts',(4.91369592899994,15.2,-9.72397129100001));
#166176=CARTESIAN_POINT('Ctrl Pts',(4.91369592899994,11.6,-9.72397129100001));
#166177=CARTESIAN_POINT('Ctrl Pts',(4.91572946499994,15.2,-9.72598684700001));
#166178=CARTESIAN_POINT('Ctrl Pts',(4.91572946499994,11.6,-9.72598684700001));
#166179=CARTESIAN_POINT('Ctrl Pts',(4.91776864699994,15.2,-9.72800464600001));
#166180=CARTESIAN_POINT('Ctrl Pts',(4.91776864699994,11.6,-9.72800464600001));
#166181=CARTESIAN_POINT('Ctrl Pts',(4.91981347399994,15.2,-9.73002467500001));
#166182=CARTESIAN_POINT('Ctrl Pts',(4.91981347399994,11.6,-9.73002467500001));
#166183=CARTESIAN_POINT('Ctrl Pts',(4.92186394399994,15.2,-9.73204692000001));
#166184=CARTESIAN_POINT('Ctrl Pts',(4.92186394399994,11.6,-9.73204692000001));
#166185=CARTESIAN_POINT('Ctrl Pts',(4.92392005599994,15.2,-9.73407137100001));
#166186=CARTESIAN_POINT('Ctrl Pts',(4.92392005599994,11.6,-9.73407137100001));
#166187=CARTESIAN_POINT('Ctrl Pts',(4.92598180799994,15.2,-9.73609801300001));
#166188=CARTESIAN_POINT('Ctrl Pts',(4.92598180799994,11.6,-9.73609801300001));
#166189=CARTESIAN_POINT('Ctrl Pts',(4.92804919799995,15.2,-9.73812683200001));
#166190=CARTESIAN_POINT('Ctrl Pts',(4.92804919799995,11.6,-9.73812683200001));
#166191=CARTESIAN_POINT('Ctrl Pts',(4.93012222499994,15.2,-9.74015782000001));
#166192=CARTESIAN_POINT('Ctrl Pts',(4.93012222499994,11.6,-9.74015782000001));
#166193=CARTESIAN_POINT('Ctrl Pts',(4.93220088799994,15.2,-9.74219096100001));
#166194=CARTESIAN_POINT('Ctrl Pts',(4.93220088799994,11.6,-9.74219096100001));
#166195=CARTESIAN_POINT('Ctrl Pts',(4.93428518399994,15.2,-9.74422624200001));
#166196=CARTESIAN_POINT('Ctrl Pts',(4.93428518399994,11.6,-9.74422624200001));
#166197=CARTESIAN_POINT('Ctrl Pts',(4.93637511199994,15.2,-9.74626365200001));
#166198=CARTESIAN_POINT('Ctrl Pts',(4.93637511199994,11.6,-9.74626365200001));
#166199=CARTESIAN_POINT('Ctrl Pts',(4.93847067099994,15.2,-9.74830317800001));
#166200=CARTESIAN_POINT('Ctrl Pts',(4.93847067099994,11.6,-9.74830317800001));
#166201=CARTESIAN_POINT('Ctrl Pts',(4.94057185799994,15.2,-9.75034480800001));
#166202=CARTESIAN_POINT('Ctrl Pts',(4.94057185799994,11.6,-9.75034480800001));
#166203=CARTESIAN_POINT('Ctrl Pts',(4.94267867199994,15.2,-9.75238852900001));
#166204=CARTESIAN_POINT('Ctrl Pts',(4.94267867199994,11.6,-9.75238852900001));
#166205=CARTESIAN_POINT('Ctrl Pts',(4.94479111299994,15.2,-9.75443432800001));
#166206=CARTESIAN_POINT('Ctrl Pts',(4.94479111299994,11.6,-9.75443432800001));
#166207=CARTESIAN_POINT('Ctrl Pts',(4.94690917699994,15.2,-9.75648219400002));
#166208=CARTESIAN_POINT('Ctrl Pts',(4.94690917699994,11.6,-9.75648219400002));
#166209=CARTESIAN_POINT('Ctrl Pts',(4.94903286299994,15.2,-9.75853211300001));
#166210=CARTESIAN_POINT('Ctrl Pts',(4.94903286299994,11.6,-9.75853211300001));
#166211=CARTESIAN_POINT('Ctrl Pts',(4.95116216899994,15.2,-9.76058407400001));
#166212=CARTESIAN_POINT('Ctrl Pts',(4.95116216899994,11.6,-9.76058407400001));
#166213=CARTESIAN_POINT('Ctrl Pts',(4.95329709499994,15.2,-9.76263806400001));
#166214=CARTESIAN_POINT('Ctrl Pts',(4.95329709499994,11.6,-9.76263806400001));
#166215=CARTESIAN_POINT('Ctrl Pts',(4.95543763799994,15.2,-9.76469407000001));
#166216=CARTESIAN_POINT('Ctrl Pts',(4.95543763799994,11.6,-9.76469407000001));
#166217=CARTESIAN_POINT('Ctrl Pts',(4.95758379699994,15.2,-9.76675208100001));
#166218=CARTESIAN_POINT('Ctrl Pts',(4.95758379699994,11.6,-9.76675208100001));
#166219=CARTESIAN_POINT('Ctrl Pts',(4.95973556799994,15.2,-9.76881208600001));
#166220=CARTESIAN_POINT('Ctrl Pts',(4.95973556799994,11.6,-9.76881208600001));
#166221=CARTESIAN_POINT('Ctrl Pts',(4.96189295299994,15.2,-9.77087406900001));
#166222=CARTESIAN_POINT('Ctrl Pts',(4.96189295299994,11.6,-9.77087406900001));
#166223=CARTESIAN_POINT('Ctrl Pts',(4.96405594799994,15.2,-9.77293802000001));
#166224=CARTESIAN_POINT('Ctrl Pts',(4.96405594799994,11.6,-9.77293802000001));
#166225=CARTESIAN_POINT('Ctrl Pts',(4.96622455099994,15.2,-9.77500392900001));
#166226=CARTESIAN_POINT('Ctrl Pts',(4.96622455099994,11.6,-9.77500392900001));
#166227=CARTESIAN_POINT('Ctrl Pts',(4.96839876099994,15.2,-9.77707177900001));
#166228=CARTESIAN_POINT('Ctrl Pts',(4.96839876099994,11.6,-9.77707177900001));
#166229=CARTESIAN_POINT('Ctrl Pts',(4.97057857799994,15.2,-9.77914156200001));
#166230=CARTESIAN_POINT('Ctrl Pts',(4.97057857799994,11.6,-9.77914156200001));
#166231=CARTESIAN_POINT('Ctrl Pts',(4.97276399699994,15.2,-9.78121326400001));
#166232=CARTESIAN_POINT('Ctrl Pts',(4.97276399699994,11.6,-9.78121326400001));
#166233=CARTESIAN_POINT('Ctrl Pts',(4.97495501799994,15.2,-9.78328687400001));
#166234=CARTESIAN_POINT('Ctrl Pts',(4.97495501799994,11.6,-9.78328687400001));
#166235=CARTESIAN_POINT('Ctrl Pts',(4.97715163999994,15.2,-9.78536237900001));
#166236=CARTESIAN_POINT('Ctrl Pts',(4.97715163999994,11.6,-9.78536237900001));
#166237=CARTESIAN_POINT('Ctrl Pts',(4.97935386099994,15.2,-9.78743976800001));
#166238=CARTESIAN_POINT('Ctrl Pts',(4.97935386099994,11.6,-9.78743976800001));
#166239=CARTESIAN_POINT('Ctrl Pts',(4.98156167699994,15.2,-9.78951902800001));
#166240=CARTESIAN_POINT('Ctrl Pts',(4.98156167699994,11.6,-9.78951902800001));
#166241=CARTESIAN_POINT('Ctrl Pts',(4.98377508799994,15.2,-9.79160014900001));
#166242=CARTESIAN_POINT('Ctrl Pts',(4.98377508799994,11.6,-9.79160014900001));
#166243=CARTESIAN_POINT('Ctrl Pts',(4.98599409399994,15.2,-9.79368311700001));
#166244=CARTESIAN_POINT('Ctrl Pts',(4.98599409399994,11.6,-9.79368311700001));
#166245=CARTESIAN_POINT('Ctrl Pts',(4.98821868999994,15.2,-9.79576792000001));
#166246=CARTESIAN_POINT('Ctrl Pts',(4.98821868999994,11.6,-9.79576792000001));
#166247=CARTESIAN_POINT('Ctrl Pts',(4.99044887699994,15.2,-9.79785454800002));
#166248=CARTESIAN_POINT('Ctrl Pts',(4.99044887699994,11.6,-9.79785454800002));
#166249=CARTESIAN_POINT('Ctrl Pts',(4.99268465099994,15.2,-9.79994298800001));
#166250=CARTESIAN_POINT('Ctrl Pts',(4.99268465099994,11.6,-9.79994298800001));
#166251=CARTESIAN_POINT('Ctrl Pts',(4.99492601099994,15.2,-9.80203322800001));
#166252=CARTESIAN_POINT('Ctrl Pts',(4.99492601099994,11.6,-9.80203322800001));
#166253=CARTESIAN_POINT('Ctrl Pts',(4.99717295499994,15.2,-9.80412525800001));
#166254=CARTESIAN_POINT('Ctrl Pts',(4.99717295499994,11.6,-9.80412525800001));
#166255=CARTESIAN_POINT('Ctrl Pts',(4.99942548199994,15.2,-9.80621906400001));
#166256=CARTESIAN_POINT('Ctrl Pts',(4.99942548199994,11.6,-9.80621906400001));
#166257=CARTESIAN_POINT('Ctrl Pts',(5.00168359099994,15.2,-9.80831463600001));
#166258=CARTESIAN_POINT('Ctrl Pts',(5.00168359099994,11.6,-9.80831463600001));
#166259=CARTESIAN_POINT('Ctrl Pts',(5.00394727799994,15.2,-9.81041196200001));
#166260=CARTESIAN_POINT('Ctrl Pts',(5.00394727799994,11.6,-9.81041196200001));
#166261=CARTESIAN_POINT('Ctrl Pts',(5.00621654199994,15.2,-9.81251102900002));
#166262=CARTESIAN_POINT('Ctrl Pts',(5.00621654199994,11.6,-9.81251102900002));
#166263=CARTESIAN_POINT('Ctrl Pts',(5.00849138299994,15.2,-9.81461182600001));
#166264=CARTESIAN_POINT('Ctrl Pts',(5.00849138299994,11.6,-9.81461182600001));
#166265=CARTESIAN_POINT('Ctrl Pts',(5.01077179499994,15.2,-9.81671434300001));
#166266=CARTESIAN_POINT('Ctrl Pts',(5.01077179499994,11.6,-9.81671434300001));
#166267=CARTESIAN_POINT('Ctrl Pts',(5.01305778099994,15.2,-9.81881856700001));
#166268=CARTESIAN_POINT('Ctrl Pts',(5.01305778099994,11.6,-9.81881856700001));
#166269=CARTESIAN_POINT('Ctrl Pts',(5.01534933699994,15.2,-9.82092448700001));
#166270=CARTESIAN_POINT('Ctrl Pts',(5.01534933699994,11.6,-9.82092448700001));
#166271=CARTESIAN_POINT('Ctrl Pts',(5.01764645999994,15.2,-9.82303209000001));
#166272=CARTESIAN_POINT('Ctrl Pts',(5.01764645999994,11.6,-9.82303209000001));
#166273=CARTESIAN_POINT('Ctrl Pts',(5.01994914999995,15.2,-9.82514136700001));
#166274=CARTESIAN_POINT('Ctrl Pts',(5.01994914999995,11.6,-9.82514136700001));
#166275=CARTESIAN_POINT('Ctrl Pts',(5.02225740499994,15.2,-9.82725230400001));
#166276=CARTESIAN_POINT('Ctrl Pts',(5.02225740499994,11.6,-9.82725230400001));
#166277=CARTESIAN_POINT('Ctrl Pts',(5.02457122199995,15.2,-9.82936489100001));
#166278=CARTESIAN_POINT('Ctrl Pts',(5.02457122199995,11.6,-9.82936489100001));
#166279=CARTESIAN_POINT('Ctrl Pts',(5.02689059999994,15.2,-9.83147911700001));
#166280=CARTESIAN_POINT('Ctrl Pts',(5.02689059999994,11.6,-9.83147911700001));
#166281=CARTESIAN_POINT('Ctrl Pts',(5.02921553699994,15.2,-9.83359496900001));
#166282=CARTESIAN_POINT('Ctrl Pts',(5.02921553699994,11.6,-9.83359496900001));
#166283=CARTESIAN_POINT('Ctrl Pts',(5.03154603199994,15.2,-9.83571243800001));
#166284=CARTESIAN_POINT('Ctrl Pts',(5.03154603199994,11.6,-9.83571243800001));
#166285=CARTESIAN_POINT('Ctrl Pts',(5.03388208199994,15.2,-9.83783151100001));
#166286=CARTESIAN_POINT('Ctrl Pts',(5.03388208199994,11.6,-9.83783151100001));
#166287=CARTESIAN_POINT('Ctrl Pts',(5.03622368499994,15.2,-9.83995217600001));
#166288=CARTESIAN_POINT('Ctrl Pts',(5.03622368499994,11.6,-9.83995217600001));
#166289=CARTESIAN_POINT('Ctrl Pts',(5.03857083999994,15.2,-9.84207442400001));
#166290=CARTESIAN_POINT('Ctrl Pts',(5.03857083999994,11.6,-9.84207442400001));
#166291=CARTESIAN_POINT('Ctrl Pts',(5.04092354399994,15.2,-9.84419824200001));
#166292=CARTESIAN_POINT('Ctrl Pts',(5.04092354399994,11.6,-9.84419824200001));
#166293=CARTESIAN_POINT('Ctrl Pts',(5.04328179699994,15.2,-9.84632361900001));
#166294=CARTESIAN_POINT('Ctrl Pts',(5.04328179699994,11.6,-9.84632361900001));
#166295=CARTESIAN_POINT('Ctrl Pts',(5.04564559499994,15.2,-9.84845054500001));
#166296=CARTESIAN_POINT('Ctrl Pts',(5.04564559499994,11.6,-9.84845054500001));
#166297=CARTESIAN_POINT('Ctrl Pts',(5.04801493799994,15.2,-9.85057900700001));
#166298=CARTESIAN_POINT('Ctrl Pts',(5.04801493799994,11.6,-9.85057900700001));
#166299=CARTESIAN_POINT('Ctrl Pts',(5.05038982199994,15.2,-9.85270899400001));
#166300=CARTESIAN_POINT('Ctrl Pts',(5.05038982199994,11.6,-9.85270899400001));
#166301=CARTESIAN_POINT('Ctrl Pts',(5.05277024799994,15.2,-9.85484049700001));
#166302=CARTESIAN_POINT('Ctrl Pts',(5.05277024799994,11.6,-9.85484049700001));
#166303=CARTESIAN_POINT('Ctrl Pts',(5.05515621199994,15.2,-9.85697350200001));
#166304=CARTESIAN_POINT('Ctrl Pts',(5.05515621199994,11.6,-9.85697350200001));
#166305=CARTESIAN_POINT('Ctrl Pts',(5.05754771099994,15.2,-9.85910800100001));
#166306=CARTESIAN_POINT('Ctrl Pts',(5.05754771099994,11.6,-9.85910800100001));
#166307=CARTESIAN_POINT('Ctrl Pts',(5.05994474599994,15.2,-9.86124398100001));
#166308=CARTESIAN_POINT('Ctrl Pts',(5.05994474599994,11.6,-9.86124398100001));
#166309=CARTESIAN_POINT('Ctrl Pts',(5.06234731399994,15.2,-9.86338143100001));
#166310=CARTESIAN_POINT('Ctrl Pts',(5.06234731399994,11.6,-9.86338143100001));
#166311=CARTESIAN_POINT('Ctrl Pts',(5.06475541199994,15.2,-9.86552034000001));
#166312=CARTESIAN_POINT('Ctrl Pts',(5.06475541199994,11.6,-9.86552034000001));
#166313=CARTESIAN_POINT('Ctrl Pts',(5.06716903899994,15.2,-9.86766069800001));
#166314=CARTESIAN_POINT('Ctrl Pts',(5.06716903899994,11.6,-9.86766069800001));
#166315=CARTESIAN_POINT('Ctrl Pts',(5.06958819299994,15.2,-9.86980249300001));
#166316=CARTESIAN_POINT('Ctrl Pts',(5.06958819299994,11.6,-9.86980249300001));
#166317=CARTESIAN_POINT('Ctrl Pts',(5.07201287199995,15.2,-9.87194571400001));
#166318=CARTESIAN_POINT('Ctrl Pts',(5.07201287199995,11.6,-9.87194571400001));
#166319=CARTESIAN_POINT('Ctrl Pts',(5.07444307399994,15.2,-9.87409035100001));
#166320=CARTESIAN_POINT('Ctrl Pts',(5.07444307399994,11.6,-9.87409035100001));
#166321=CARTESIAN_POINT('Ctrl Pts',(5.07687879599994,15.2,-9.87623639300001));
#166322=CARTESIAN_POINT('Ctrl Pts',(5.07687879599994,11.6,-9.87623639300001));
#166323=CARTESIAN_POINT('Ctrl Pts',(5.07932003899994,15.2,-9.87838382800001));
#166324=CARTESIAN_POINT('Ctrl Pts',(5.07932003899994,11.6,-9.87838382800001));
#166325=CARTESIAN_POINT('Ctrl Pts',(5.08176679799995,15.2,-9.88053264700001));
#166326=CARTESIAN_POINT('Ctrl Pts',(5.08176679799995,11.6,-9.88053264700001));
#166327=CARTESIAN_POINT('Ctrl Pts',(5.08421907399994,15.2,-9.88268283800001));
#166328=CARTESIAN_POINT('Ctrl Pts',(5.08421907399994,11.6,-9.88268283800001));
#166329=CARTESIAN_POINT('Ctrl Pts',(5.08667686199994,15.2,-9.88483438900001));
#166330=CARTESIAN_POINT('Ctrl Pts',(5.08667686199994,11.6,-9.88483438900001));
#166331=CARTESIAN_POINT('Ctrl Pts',(5.08914016199994,15.2,-9.88698729200001));
#166332=CARTESIAN_POINT('Ctrl Pts',(5.08914016199994,11.6,-9.88698729200001));
#166333=CARTESIAN_POINT('Ctrl Pts',(5.09160897099994,15.2,-9.88914153400001));
#166334=CARTESIAN_POINT('Ctrl Pts',(5.09160897099994,11.6,-9.88914153400001));
#166335=CARTESIAN_POINT('Ctrl Pts',(5.09408328699994,15.2,-9.89129710500001));
#166336=CARTESIAN_POINT('Ctrl Pts',(5.09408328699994,11.6,-9.89129710500001));
#166337=CARTESIAN_POINT('Ctrl Pts',(5.09656310899994,15.2,-9.89345399400001));
#166338=CARTESIAN_POINT('Ctrl Pts',(5.09656310899994,11.6,-9.89345399400001));
#166339=CARTESIAN_POINT('Ctrl Pts',(5.09904843499994,15.2,-9.89561219200001));
#166340=CARTESIAN_POINT('Ctrl Pts',(5.09904843499994,11.6,-9.89561219200001));
#166341=CARTESIAN_POINT('Ctrl Pts',(5.10153926199994,15.2,-9.89777168700001));
#166342=CARTESIAN_POINT('Ctrl Pts',(5.10153926199994,11.6,-9.89777168700001));
#166343=CARTESIAN_POINT('Ctrl Pts',(5.10403558799994,15.2,-9.89993246800001));
#166344=CARTESIAN_POINT('Ctrl Pts',(5.10403558799994,11.6,-9.89993246800001));
#166345=CARTESIAN_POINT('Ctrl Pts',(5.10653741199994,15.2,-9.90209452500001));
#166346=CARTESIAN_POINT('Ctrl Pts',(5.10653741199994,11.6,-9.90209452500001));
#166347=CARTESIAN_POINT('Ctrl Pts',(5.10904473099994,15.2,-9.90425784600001));
#166348=CARTESIAN_POINT('Ctrl Pts',(5.10904473099994,11.6,-9.90425784600001));
#166349=CARTESIAN_POINT('Ctrl Pts',(5.11155754399994,15.2,-9.90642242300001));
#166350=CARTESIAN_POINT('Ctrl Pts',(5.11155754399994,11.6,-9.90642242300001));
#166351=CARTESIAN_POINT('Ctrl Pts',(5.11407584799994,15.2,-9.90858824500001));
#166352=CARTESIAN_POINT('Ctrl Pts',(5.11407584799994,11.6,-9.90858824500001));
#166353=CARTESIAN_POINT('Ctrl Pts',(5.11659964299994,15.2,-9.91075529900001));
#166354=CARTESIAN_POINT('Ctrl Pts',(5.11659964299994,11.6,-9.91075529900001));
#166355=CARTESIAN_POINT('Ctrl Pts',(5.11912892399994,15.2,-9.91292357700001));
#166356=CARTESIAN_POINT('Ctrl Pts',(5.11912892399994,11.6,-9.91292357700001));
#166357=CARTESIAN_POINT('Ctrl Pts',(5.12166368999995,15.2,-9.91509306700001));
#166358=CARTESIAN_POINT('Ctrl Pts',(5.12166368999995,11.6,-9.91509306700001));
#166359=CARTESIAN_POINT('Ctrl Pts',(5.12420394099994,15.2,-9.91726376000001));
#166360=CARTESIAN_POINT('Ctrl Pts',(5.12420394099994,11.6,-9.91726376000001));
#166361=CARTESIAN_POINT('Ctrl Pts',(5.12674967199994,15.2,-9.91943564400001));
#166362=CARTESIAN_POINT('Ctrl Pts',(5.12674967199994,11.6,-9.91943564400001));
#166363=CARTESIAN_POINT('Ctrl Pts',(5.12930088299994,15.2,-9.92160871000001));
#166364=CARTESIAN_POINT('Ctrl Pts',(5.12930088299994,11.6,-9.92160871000001));
#166365=CARTESIAN_POINT('Ctrl Pts',(5.13185757099994,15.2,-9.92378294700002));
#166366=CARTESIAN_POINT('Ctrl Pts',(5.13185757099994,11.6,-9.92378294700002));
#166367=CARTESIAN_POINT('Ctrl Pts',(5.13441973599994,15.2,-9.92595834500001));
#166368=CARTESIAN_POINT('Ctrl Pts',(5.13441973599994,11.6,-9.92595834500001));
#166369=CARTESIAN_POINT('Ctrl Pts',(5.13698737199995,15.2,-9.92813489200001));
#166370=CARTESIAN_POINT('Ctrl Pts',(5.13698737199995,11.6,-9.92813489200001));
#166371=CARTESIAN_POINT('Ctrl Pts',(5.13956047999995,15.2,-9.93031258000001));
#166372=CARTESIAN_POINT('Ctrl Pts',(5.13956047999995,11.6,-9.93031258000001));
#166373=CARTESIAN_POINT('Ctrl Pts',(5.14213905699994,15.2,-9.93249139700001));
#166374=CARTESIAN_POINT('Ctrl Pts',(5.14213905699994,11.6,-9.93249139700001));
#166375=CARTESIAN_POINT('Ctrl Pts',(5.14472310199994,15.2,-9.93467133400001));
#166376=CARTESIAN_POINT('Ctrl Pts',(5.14472310199994,11.6,-9.93467133400001));
#166377=CARTESIAN_POINT('Ctrl Pts',(5.14731261099994,15.2,-9.93685238100001));
#166378=CARTESIAN_POINT('Ctrl Pts',(5.14731261099994,11.6,-9.93685238100001));
#166379=CARTESIAN_POINT('Ctrl Pts',(5.14990758299994,15.2,-9.93903452600001));
#166380=CARTESIAN_POINT('Ctrl Pts',(5.14990758299994,11.6,-9.93903452600001));
#166381=CARTESIAN_POINT('Ctrl Pts',(5.15250801599994,15.2,-9.94121776100001));
#166382=CARTESIAN_POINT('Ctrl Pts',(5.15250801599994,11.6,-9.94121776100001));
#166383=CARTESIAN_POINT('Ctrl Pts',(5.15511390699994,15.2,-9.94340207300001));
#166384=CARTESIAN_POINT('Ctrl Pts',(5.15511390699994,11.6,-9.94340207300001));
#166385=CARTESIAN_POINT('Ctrl Pts',(5.15772525599994,15.2,-9.94558745400001));
#166386=CARTESIAN_POINT('Ctrl Pts',(5.15772525599994,11.6,-9.94558745400001));
#166387=CARTESIAN_POINT('Ctrl Pts',(5.16034205999994,15.2,-9.94777389300001));
#166388=CARTESIAN_POINT('Ctrl Pts',(5.16034205999994,11.6,-9.94777389300001));
#166389=CARTESIAN_POINT('Ctrl Pts',(5.16296431499994,15.2,-9.94996138100001));
#166390=CARTESIAN_POINT('Ctrl Pts',(5.16296431499994,11.6,-9.94996138100001));
#166391=CARTESIAN_POINT('Ctrl Pts',(5.16559202199994,15.2,-9.95214990500001));
#166392=CARTESIAN_POINT('Ctrl Pts',(5.16559202199994,11.6,-9.95214990500001));
#166393=CARTESIAN_POINT('Ctrl Pts',(5.16822517599994,15.2,-9.95433945900001));
#166394=CARTESIAN_POINT('Ctrl Pts',(5.16822517599994,11.6,-9.95433945900001));
#166395=CARTESIAN_POINT('Ctrl Pts',(5.17086377599994,15.2,-9.95653003000001));
#166396=CARTESIAN_POINT('Ctrl Pts',(5.17086377599994,11.6,-9.95653003000001));
#166397=CARTESIAN_POINT('Ctrl Pts',(5.17350782199994,15.2,-9.95872160800001));
#166398=CARTESIAN_POINT('Ctrl Pts',(5.17350782199994,11.6,-9.95872160800001));
#166399=CARTESIAN_POINT('Ctrl Pts',(5.17615730899994,15.2,-9.96091418600001));
#166400=CARTESIAN_POINT('Ctrl Pts',(5.17615730899994,11.6,-9.96091418600001));
#166401=CARTESIAN_POINT('Ctrl Pts',(5.17881223599994,15.2,-9.96310775100001));
#166402=CARTESIAN_POINT('Ctrl Pts',(5.17881223599994,11.6,-9.96310775100001));
#166403=CARTESIAN_POINT('Ctrl Pts',(5.18147259999994,15.2,-9.96530229200001));
#166404=CARTESIAN_POINT('Ctrl Pts',(5.18147259999994,11.6,-9.96530229200001));
#166405=CARTESIAN_POINT('Ctrl Pts',(5.18413840099995,15.2,-9.96749780400001));
#166406=CARTESIAN_POINT('Ctrl Pts',(5.18413840099995,11.6,-9.96749780400001));
#166407=CARTESIAN_POINT('Ctrl Pts',(5.18680963499994,15.2,-9.96969427100001));
#166408=CARTESIAN_POINT('Ctrl Pts',(5.18680963499994,11.6,-9.96969427100001));
#166409=CARTESIAN_POINT('Ctrl Pts',(5.18948629999994,15.2,-9.97189168800001));
#166410=CARTESIAN_POINT('Ctrl Pts',(5.18948629999994,11.6,-9.97189168800001));
#166411=CARTESIAN_POINT('Ctrl Pts',(5.19216839499994,15.2,-9.97409004200001));
#166412=CARTESIAN_POINT('Ctrl Pts',(5.19216839499994,11.6,-9.97409004200001));
#166413=CARTESIAN_POINT('Ctrl Pts',(5.19485591699994,15.2,-9.97628932500001));
#166414=CARTESIAN_POINT('Ctrl Pts',(5.19485591699994,11.6,-9.97628932500001));
#166415=CARTESIAN_POINT('Ctrl Pts',(5.19754886399994,15.2,-9.97848952600001));
#166416=CARTESIAN_POINT('Ctrl Pts',(5.19754886399994,11.6,-9.97848952600001));
#166417=CARTESIAN_POINT('Ctrl Pts',(5.20024723299994,15.2,-9.98069063500001));
#166418=CARTESIAN_POINT('Ctrl Pts',(5.20024723299994,11.6,-9.98069063500001));
#166419=CARTESIAN_POINT('Ctrl Pts',(5.20295102399994,15.2,-9.98289264400001));
#166420=CARTESIAN_POINT('Ctrl Pts',(5.20295102399994,11.6,-9.98289264400001));
#166421=CARTESIAN_POINT('Ctrl Pts',(5.20566023399994,15.2,-9.98509554200002));
#166422=CARTESIAN_POINT('Ctrl Pts',(5.20566023399994,11.6,-9.98509554200002));
#166423=CARTESIAN_POINT('Ctrl Pts',(5.20837485899994,15.2,-9.98729931800001));
#166424=CARTESIAN_POINT('Ctrl Pts',(5.20837485899994,11.6,-9.98729931800001));
#166425=CARTESIAN_POINT('Ctrl Pts',(5.21109489899994,15.2,-9.98950396400001));
#166426=CARTESIAN_POINT('Ctrl Pts',(5.21109489899994,11.6,-9.98950396400001));
#166427=CARTESIAN_POINT('Ctrl Pts',(5.21382035099994,15.2,-9.99170947000001));
#166428=CARTESIAN_POINT('Ctrl Pts',(5.21382035099994,11.6,-9.99170947000001));
#166429=CARTESIAN_POINT('Ctrl Pts',(5.21655121299994,15.2,-9.99391582500001));
#166430=CARTESIAN_POINT('Ctrl Pts',(5.21655121299994,11.6,-9.99391582500001));
#166431=CARTESIAN_POINT('Ctrl Pts',(5.21928748199994,15.2,-9.99612302200001));
#166432=CARTESIAN_POINT('Ctrl Pts',(5.21928748199994,11.6,-9.99612302200001));
#166433=CARTESIAN_POINT('Ctrl Pts',(5.22202915799994,15.2,-9.99833104900001));
#166434=CARTESIAN_POINT('Ctrl Pts',(5.22202915799994,11.6,-9.99833104900001));
#166435=CARTESIAN_POINT('Ctrl Pts',(5.22477623599994,15.2,-10.000539896));
#166436=CARTESIAN_POINT('Ctrl Pts',(5.22477623599994,11.6,-10.000539896));
#166437=CARTESIAN_POINT('Ctrl Pts',(5.22752871599994,15.2,-10.002749554));
#166438=CARTESIAN_POINT('Ctrl Pts',(5.22752871599994,11.6,-10.002749554));
#166439=CARTESIAN_POINT('Ctrl Pts',(5.23028659499994,15.2,-10.004960015));
#166440=CARTESIAN_POINT('Ctrl Pts',(5.23028659499994,11.6,-10.004960015));
#166441=CARTESIAN_POINT('Ctrl Pts',(5.23304987099994,15.2,-10.007171267));
#166442=CARTESIAN_POINT('Ctrl Pts',(5.23304987099994,11.6,-10.007171267));
#166443=CARTESIAN_POINT('Ctrl Pts',(5.23581854099994,15.2,-10.009383302));
#166444=CARTESIAN_POINT('Ctrl Pts',(5.23581854099994,11.6,-10.009383302));
#166445=CARTESIAN_POINT('Ctrl Pts',(5.23859260399994,15.2,-10.01159611));
#166446=CARTESIAN_POINT('Ctrl Pts',(5.23859260399994,11.6,-10.01159611));
#166447=CARTESIAN_POINT('Ctrl Pts',(5.24137205699994,15.2,-10.013809682));
#166448=CARTESIAN_POINT('Ctrl Pts',(5.24137205699994,11.6,-10.013809682));
#166449=CARTESIAN_POINT('Ctrl Pts',(5.24415689799994,15.2,-10.016024008));
#166450=CARTESIAN_POINT('Ctrl Pts',(5.24415689799994,11.6,-10.016024008));
#166451=CARTESIAN_POINT('Ctrl Pts',(5.24694712499994,15.2,-10.018239077));
#166452=CARTESIAN_POINT('Ctrl Pts',(5.24694712499994,11.6,-10.018239077));
#166453=CARTESIAN_POINT('Ctrl Pts',(5.24974273599994,15.2,-10.020454881));
#166454=CARTESIAN_POINT('Ctrl Pts',(5.24974273599994,11.6,-10.020454881));
#166455=CARTESIAN_POINT('Ctrl Pts',(5.25254372799994,15.2,-10.022671411));
#166456=CARTESIAN_POINT('Ctrl Pts',(5.25254372799994,11.6,-10.022671411));
#166457=CARTESIAN_POINT('Ctrl Pts',(5.25535009899994,15.2,-10.024888657));
#166458=CARTESIAN_POINT('Ctrl Pts',(5.25535009899994,11.6,-10.024888657));
#166459=CARTESIAN_POINT('Ctrl Pts',(5.25816184699995,15.2,-10.02710661));
#166460=CARTESIAN_POINT('Ctrl Pts',(5.25816184699995,11.6,-10.02710661));
#166461=CARTESIAN_POINT('Ctrl Pts',(5.26097896999994,15.2,-10.029325259));
#166462=CARTESIAN_POINT('Ctrl Pts',(5.26097896999994,11.6,-10.029325259));
#166463=CARTESIAN_POINT('Ctrl Pts',(5.26380146599994,15.2,-10.031544597));
#166464=CARTESIAN_POINT('Ctrl Pts',(5.26380146599994,11.6,-10.031544597));
#166465=CARTESIAN_POINT('Ctrl Pts',(5.26662933099994,15.2,-10.033764612));
#166466=CARTESIAN_POINT('Ctrl Pts',(5.26662933099994,11.6,-10.033764612));
#166467=CARTESIAN_POINT('Ctrl Pts',(5.26946256499994,15.2,-10.035985297));
#166468=CARTESIAN_POINT('Ctrl Pts',(5.26946256499994,11.6,-10.035985297));
#166469=CARTESIAN_POINT('Ctrl Pts',(5.27230116399994,15.2,-10.038206641));
#166470=CARTESIAN_POINT('Ctrl Pts',(5.27230116399994,11.6,-10.038206641));
#166471=CARTESIAN_POINT('Ctrl Pts',(5.27514512699994,15.2,-10.040428636));
#166472=CARTESIAN_POINT('Ctrl Pts',(5.27514512699994,11.6,-10.040428636));
#166473=CARTESIAN_POINT('Ctrl Pts',(5.27799445099994,15.2,-10.042651271));
#166474=CARTESIAN_POINT('Ctrl Pts',(5.27799445099994,11.6,-10.042651271));
#166475=CARTESIAN_POINT('Ctrl Pts',(5.28084913499994,15.2,-10.04487454));
#166476=CARTESIAN_POINT('Ctrl Pts',(5.28084913499994,11.6,-10.04487454));
#166477=CARTESIAN_POINT('Ctrl Pts',(5.28370917499994,15.2,-10.047098429));
#166478=CARTESIAN_POINT('Ctrl Pts',(5.28370917499994,11.6,-10.047098429));
#166479=CARTESIAN_POINT('Ctrl Pts',(5.28657456899994,15.2,-10.049322933));
#166480=CARTESIAN_POINT('Ctrl Pts',(5.28657456899994,11.6,-10.049322933));
#166481=CARTESIAN_POINT('Ctrl Pts',(5.28944531599994,15.2,-10.05154804));
#166482=CARTESIAN_POINT('Ctrl Pts',(5.28944531599994,11.6,-10.05154804));
#166483=CARTESIAN_POINT('Ctrl Pts',(5.29232141299994,15.2,-10.053773742));
#166484=CARTESIAN_POINT('Ctrl Pts',(5.29232141299994,11.6,-10.053773742));
#166485=CARTESIAN_POINT('Ctrl Pts',(5.29520285699994,15.2,-10.05600003));
#166486=CARTESIAN_POINT('Ctrl Pts',(5.29520285699994,11.6,-10.05600003));
#166487=CARTESIAN_POINT('Ctrl Pts',(5.29808964699994,15.2,-10.058226894));
#166488=CARTESIAN_POINT('Ctrl Pts',(5.29808964699994,11.6,-10.058226894));
#166489=CARTESIAN_POINT('Ctrl Pts',(5.30098177999994,15.2,-10.060454326));
#166490=CARTESIAN_POINT('Ctrl Pts',(5.30098177999994,11.6,-10.060454326));
#166491=CARTESIAN_POINT('Ctrl Pts',(5.30387925399994,15.2,-10.062682315));
#166492=CARTESIAN_POINT('Ctrl Pts',(5.30387925399994,11.6,-10.062682315));
#166493=CARTESIAN_POINT('Ctrl Pts',(5.30678206599994,15.2,-10.064910853));
#166494=CARTESIAN_POINT('Ctrl Pts',(5.30678206599994,11.6,-10.064910853));
#166495=CARTESIAN_POINT('Ctrl Pts',(5.30969021499994,15.2,-10.067139933));
#166496=CARTESIAN_POINT('Ctrl Pts',(5.30969021499994,11.6,-10.067139933));
#166497=CARTESIAN_POINT('Ctrl Pts',(5.31260369799995,15.2,-10.069369542));
#166498=CARTESIAN_POINT('Ctrl Pts',(5.31260369799995,11.6,-10.069369542));
#166499=CARTESIAN_POINT('Ctrl Pts',(5.31552251199994,15.2,-10.071599674));
#166500=CARTESIAN_POINT('Ctrl Pts',(5.31552251199994,11.6,-10.071599674));
#166501=CARTESIAN_POINT('Ctrl Pts',(5.31844665599994,15.2,-10.073830318));
#166502=CARTESIAN_POINT('Ctrl Pts',(5.31844665599994,11.6,-10.073830318));
#166503=CARTESIAN_POINT('Ctrl Pts',(5.32137612699994,15.2,-10.076061466));
#166504=CARTESIAN_POINT('Ctrl Pts',(5.32137612699994,11.6,-10.076061466));
#166505=CARTESIAN_POINT('Ctrl Pts',(5.32431092299994,15.2,-10.078293108));
#166506=CARTESIAN_POINT('Ctrl Pts',(5.32431092299994,11.6,-10.078293108));
#166507=CARTESIAN_POINT('Ctrl Pts',(5.32725104099994,15.2,-10.080525236));
#166508=CARTESIAN_POINT('Ctrl Pts',(5.32725104099994,11.6,-10.080525236));
#166509=CARTESIAN_POINT('Ctrl Pts',(5.33019647899994,15.2,-10.08275784));
#166510=CARTESIAN_POINT('Ctrl Pts',(5.33019647899994,11.6,-10.08275784));
#166511=CARTESIAN_POINT('Ctrl Pts',(5.33314723499994,15.2,-10.084990912));
#166512=CARTESIAN_POINT('Ctrl Pts',(5.33314723499994,11.6,-10.084990912));
#166513=CARTESIAN_POINT('Ctrl Pts',(5.33610330699994,15.2,-10.087224444));
#166514=CARTESIAN_POINT('Ctrl Pts',(5.33610330699994,11.6,-10.087224444));
#166515=CARTESIAN_POINT('Ctrl Pts',(5.33906469099994,15.2,-10.089458425));
#166516=CARTESIAN_POINT('Ctrl Pts',(5.33906469099994,11.6,-10.089458425));
#166517=CARTESIAN_POINT('Ctrl Pts',(5.34203138799994,15.2,-10.091692847));
#166518=CARTESIAN_POINT('Ctrl Pts',(5.34203138799994,11.6,-10.091692847));
#166519=CARTESIAN_POINT('Ctrl Pts',(5.34500339199994,15.2,-10.093927703));
#166520=CARTESIAN_POINT('Ctrl Pts',(5.34500339199994,11.6,-10.093927703));
#166521=CARTESIAN_POINT('Ctrl Pts',(5.34798070299994,15.2,-10.096162981));
#166522=CARTESIAN_POINT('Ctrl Pts',(5.34798070299994,11.6,-10.096162981));
#166523=CARTESIAN_POINT('Ctrl Pts',(5.35096331799994,15.2,-10.098398674));
#166524=CARTESIAN_POINT('Ctrl Pts',(5.35096331799994,11.6,-10.098398674));
#166525=CARTESIAN_POINT('Ctrl Pts',(5.35395123399994,15.2,-10.100634772));
#166526=CARTESIAN_POINT('Ctrl Pts',(5.35395123399994,11.6,-10.100634772));
#166527=CARTESIAN_POINT('Ctrl Pts',(5.35694444999994,15.2,-10.102871266));
#166528=CARTESIAN_POINT('Ctrl Pts',(5.35694444999994,11.6,-10.102871266));
#166529=CARTESIAN_POINT('Ctrl Pts',(5.35994296099994,15.2,-10.105108146));
#166530=CARTESIAN_POINT('Ctrl Pts',(5.35994296099994,11.6,-10.105108146));
#166531=CARTESIAN_POINT('Ctrl Pts',(5.36294676699994,15.2,-10.107345404));
#166532=CARTESIAN_POINT('Ctrl Pts',(5.36294676699994,11.6,-10.107345404));
#166533=CARTESIAN_POINT('Ctrl Pts',(5.36595586499995,15.2,-10.109583032));
#166534=CARTESIAN_POINT('Ctrl Pts',(5.36595586499995,11.6,-10.109583032));
#166535=CARTESIAN_POINT('Ctrl Pts',(5.36897025299995,15.2,-10.111821023));
#166536=CARTESIAN_POINT('Ctrl Pts',(5.36897025299995,11.6,-10.111821023));
#166537=CARTESIAN_POINT('Ctrl Pts',(5.37198992799994,15.2,-10.114059367));
#166538=CARTESIAN_POINT('Ctrl Pts',(5.37198992799994,11.6,-10.114059367));
#166539=CARTESIAN_POINT('Ctrl Pts',(5.37501488899994,15.2,-10.116298058));
#166540=CARTESIAN_POINT('Ctrl Pts',(5.37501488899994,11.6,-10.116298058));
#166541=CARTESIAN_POINT('Ctrl Pts',(5.37804513399994,15.2,-10.118537086));
#166542=CARTESIAN_POINT('Ctrl Pts',(5.37804513399994,11.6,-10.118537086));
#166543=CARTESIAN_POINT('Ctrl Pts',(5.38108065899994,15.2,-10.120776443));
#166544=CARTESIAN_POINT('Ctrl Pts',(5.38108065899994,11.6,-10.120776443));
#166545=CARTESIAN_POINT('Ctrl Pts',(5.38412146299994,15.2,-10.123016119));
#166546=CARTESIAN_POINT('Ctrl Pts',(5.38412146299994,11.6,-10.123016119));
#166547=CARTESIAN_POINT('Ctrl Pts',(5.38716754099994,15.2,-10.125256102));
#166548=CARTESIAN_POINT('Ctrl Pts',(5.38716754099994,11.6,-10.125256102));
#166549=CARTESIAN_POINT('Ctrl Pts',(5.39021889199994,15.2,-10.127496383));
#166550=CARTESIAN_POINT('Ctrl Pts',(5.39021889199994,11.6,-10.127496383));
#166551=CARTESIAN_POINT('Ctrl Pts',(5.39327551199994,15.2,-10.129736951));
#166552=CARTESIAN_POINT('Ctrl Pts',(5.39327551199994,11.6,-10.129736951));
#166553=CARTESIAN_POINT('Ctrl Pts',(5.39633739999994,15.2,-10.131977796));
#166554=CARTESIAN_POINT('Ctrl Pts',(5.39633739999994,11.6,-10.131977796));
#166555=CARTESIAN_POINT('Ctrl Pts',(5.39940455199994,15.2,-10.13421891));
#166556=CARTESIAN_POINT('Ctrl Pts',(5.39940455199994,11.6,-10.13421891));
#166557=CARTESIAN_POINT('Ctrl Pts',(5.40247696699994,15.2,-10.136460289));
#166558=CARTESIAN_POINT('Ctrl Pts',(5.40247696699994,11.6,-10.136460289));
#166559=CARTESIAN_POINT('Ctrl Pts',(5.40555464399994,15.2,-10.138701926));
#166560=CARTESIAN_POINT('Ctrl Pts',(5.40555464399994,11.6,-10.138701926));
#166561=CARTESIAN_POINT('Ctrl Pts',(5.40863758099994,15.2,-10.140943823));
#166562=CARTESIAN_POINT('Ctrl Pts',(5.40863758099994,11.6,-10.140943823));
#166563=CARTESIAN_POINT('Ctrl Pts',(5.41110813999994,15.2,-10.142737544));
#166564=CARTESIAN_POINT('Ctrl Pts',(5.41110813999994,11.6,-10.142737544));
#166565=CARTESIAN_POINT('Ctrl Pts',(5.41296342599994,15.2,-10.14408295));
#166566=CARTESIAN_POINT('Ctrl Pts',(5.41296342599994,11.6,-10.14408295));
#166567=CARTESIAN_POINT('Ctrl Pts',(5.41420133599994,15.2,-10.144979939));
#166568=CARTESIAN_POINT('Ctrl Pts',(5.41420133599994,11.6,-10.144979939));
#166569=CARTESIAN_POINT('Ctrl Pts',(5.41482055299994,15.2,-10.145428447));
#166570=CARTESIAN_POINT('Ctrl Pts',(5.41482055299994,11.6,-10.145428447));
#166571=CARTESIAN_POINT('Ctrl Pts',(4.57383771099994,15.2,-9.31239140100002));
#166572=CARTESIAN_POINT('Ctrl Pts',(4.57476026769951,15.2,-9.31392144680197));
#166573=CARTESIAN_POINT('Ctrl Pts',(4.57571693070584,15.2,-9.31549767344764));
#166574=CARTESIAN_POINT('Ctrl Pts',(4.57670776760804,15.2,-9.31711891458905));
#166575=CARTESIAN_POINT('Ctrl Pts',(4.57770338282661,15.2,-9.31874797417473));
#166576=CARTESIAN_POINT('Ctrl Pts',(4.57873349763143,15.2,-9.32042248430923));
#166577=CARTESIAN_POINT('Ctrl Pts',(4.57979816282796,15.2,-9.32214130040799));
#166578=CARTESIAN_POINT('Ctrl Pts',(4.58086282792779,15.2,-9.32386011635063));
#166579=CARTESIAN_POINT('Ctrl Pts',(4.58196204049941,15.2,-9.32562323961556));
#166580=CARTESIAN_POINT('Ctrl Pts',(4.58309584770821,15.2,-9.32742955654993));
#166581=CARTESIAN_POINT('Ctrl Pts',(4.58422965491702,15.2,-9.32923587348429));
#166582=CARTESIAN_POINT('Ctrl Pts',(4.5853980563192,15.1999999999999,-9.33108538508538));
#166583=CARTESIAN_POINT('Ctrl Pts',(4.58660109166692,15.2,-9.33297701302539));
#166584=CARTESIAN_POINT('Ctrl Pts',(4.58780412712392,15.2,-9.33486864113721));
#166585=CARTESIAN_POINT('Ctrl Pts',(4.58904179768353,15.2,-9.33680238271311));
#166586=CARTESIAN_POINT('Ctrl Pts',(4.59031413808858,15.2,-9.33877718824021));
#166587=CARTESIAN_POINT('Ctrl Pts',(4.59158647837806,15.2,-9.34075199358794));
#166588=CARTESIAN_POINT('Ctrl Pts',(4.59289349004307,15.2,-9.34276786523282));
#166589=CARTESIAN_POINT('Ctrl Pts',(4.5942352060005,15.2,-9.34482377850088));
#166590=CARTESIAN_POINT('Ctrl Pts',(4.59557692195793,15.2,-9.34687969176897));
#166591=CARTESIAN_POINT('Ctrl Pts',(4.59695334073424,15.2,-9.34897564678802));
#166592=CARTESIAN_POINT('Ctrl Pts',(4.59836449093146,15.2,-9.35111065112542));
#166593=CARTESIAN_POINT('Ctrl Pts',(4.59977564125686,15.2,-9.35324565565676));
#166594=CARTESIAN_POINT('Ctrl Pts',(4.60122152409488,15.2,-9.35541970753459));
#166595=CARTESIAN_POINT('Ctrl Pts',(4.60270216417795,15.2,-9.35763183999108));
#166596=CARTESIAN_POINT('Ctrl Pts',(4.60418280412651,15.2,-9.35984397224663));
#166597=CARTESIAN_POINT('Ctrl Pts',(4.60569820106435,15.2,-9.36209418342296));
#166598=CARTESIAN_POINT('Ctrl Pts',(4.60724837709285,15.2,-9.36438152917477));
#166599=CARTESIAN_POINT('Ctrl Pts',(4.60879855312135,15.2,-9.36666887492659));
#166600=CARTESIAN_POINT('Ctrl Pts',(4.61038350778881,15.2,-9.36899335881716));
#166601=CARTESIAN_POINT('Ctrl Pts',(4.61200325789508,15.2,-9.37135405564644));
#166602=CARTESIAN_POINT('Ctrl Pts',(4.61362300800136,15.2,-9.37371475247571));
#166603=CARTESIAN_POINT('Ctrl Pts',(4.61527755797951,15.2,-9.3761116657423));
#166604=CARTESIAN_POINT('Ctrl Pts',(4.61696691708242,15.2,-9.37854389648485));
#166605=CARTESIAN_POINT('Ctrl Pts',(4.61865627633879,15.2,-9.38097612744834));
#166606=CARTESIAN_POINT('Ctrl Pts',(4.62038044630684,15.2,-9.38344367723195));
#166607=CARTESIAN_POINT('Ctrl Pts',(4.6221394413209,15.2,-9.38594566836979));
#166608=CARTESIAN_POINT('Ctrl Pts',(4.62389843617517,15.2,-9.38844765928039));
#166609=CARTESIAN_POINT('Ctrl Pts',(4.62569225239894,15.2,-9.39098409241392));
#166610=CARTESIAN_POINT('Ctrl Pts',(4.62752090125739,15.2,-9.39355411249879));
#166611=CARTESIAN_POINT('Ctrl Pts',(4.62965432503633,15.2,-9.39655246942013));
#166612=CARTESIAN_POINT('Ctrl Pts',(4.63183515898931,15.2,-9.39959654241051));
#166613=CARTESIAN_POINT('Ctrl Pts',(4.63406341059595,15.2,-9.4026850069196));
#166614=CARTESIAN_POINT('Ctrl Pts',(4.63597334044536,15.2,-9.40533226207569));
#166615=CARTESIAN_POINT('Ctrl Pts',(4.63791810759892,15.2,-9.40801213163555));
#166616=CARTESIAN_POINT('Ctrl Pts',(4.63989771385881,15.2,-9.41072380386897));
#166617=CARTESIAN_POINT('Ctrl Pts',(4.64187732011871,15.2,-9.4134354761024));
#166618=CARTESIAN_POINT('Ctrl Pts',(4.64389176767837,15.2,-9.41617895175048));
#166619=CARTESIAN_POINT('Ctrl Pts',(4.64594105451818,15.2,-9.41895343414755));
#166620=CARTESIAN_POINT('Ctrl Pts',(4.64799034154416,15.2,-9.42172791679664));
#166621=CARTESIAN_POINT('Ctrl Pts',(4.65007446671518,15.2,-9.42453340810711));
#166622=CARTESIAN_POINT('Ctrl Pts',(4.65219342783218,15.2,-9.42736913067964));
#166623=CARTESIAN_POINT('Ctrl Pts',(4.65431238875671,15.2,-9.43020485299459));
#166624=CARTESIAN_POINT('Ctrl Pts',(4.6564661859602,15.2,-9.43307080742409));
#166625=CARTESIAN_POINT('Ctrl Pts',(4.65865481280723,15.2,-9.43596623199865));
#166626=CARTESIAN_POINT('Ctrl Pts',(4.66084343965424,15.2,-9.43886165657323));
#166627=CARTESIAN_POINT('Ctrl Pts',(4.66306689596317,15.2,-9.4417865522873));
#166628=CARTESIAN_POINT('Ctrl Pts',(4.66532517296207,15.2,-9.44474017667803));
#166629=CARTESIAN_POINT('Ctrl Pts',(4.66758345016611,15.2,-9.44769380133706));
#166630=CARTESIAN_POINT('Ctrl Pts',(4.66987654967998,15.2,-9.45067615296685));
#166631=CARTESIAN_POINT('Ctrl Pts',(4.67220445892517,15.2,-9.45368650503292));
#166632=CARTESIAN_POINT('Ctrl Pts',(4.6745323679589,15.2,-9.45669685682556));
#166633=CARTESIAN_POINT('Ctrl Pts',(4.67689508671199,15.2,-9.45973520780302));
#166634=CARTESIAN_POINT('Ctrl Pts',(4.67929260254154,15.2,-9.46280084644163));
#166635=CARTESIAN_POINT('Ctrl Pts',(4.68169011837109,15.2,-9.46586648508024));
#166636=CARTESIAN_POINT('Ctrl Pts',(4.68412243150472,15.2,-9.46895940989898));
#166637=CARTESIAN_POINT('Ctrl Pts',(4.68658952378631,15.2,-9.47207892468993));
#166638=CARTESIAN_POINT('Ctrl Pts',(4.689056616292,15.2,-9.47519843976424));
#166639=CARTESIAN_POINT('Ctrl Pts',(4.69155849149409,15.2,-9.47834454267108));
#166640=CARTESIAN_POINT('Ctrl Pts',(4.69409512855138,15.2,-9.48151654984572));
#166641=CARTESIAN_POINT('Ctrl Pts',(4.69620899265059,15.2,-9.48415988901386));
#166642=CARTESIAN_POINT('Ctrl Pts',(4.69834699793628,15.2,-9.48682121918228));
#166643=CARTESIAN_POINT('Ctrl Pts',(4.70050913279937,15.2,-9.48950014835038));
#166644=CARTESIAN_POINT('Ctrl Pts',(4.70267126742678,15.2,-9.49217907722649));
#166645=CARTESIAN_POINT('Ctrl Pts',(4.70485753088146,15.2,-9.49487560747001));
#166646=CARTESIAN_POINT('Ctrl Pts',(4.70706790994411,15.2,-9.49758935543668));
#166647=CARTESIAN_POINT('Ctrl Pts',(4.70927828924768,15.2,-9.50030310369916));
#166648=CARTESIAN_POINT('Ctrl Pts',(4.71151278833977,15.2,-9.50303407011418));
#166649=CARTESIAN_POINT('Ctrl Pts',(4.71377138750447,15.2,-9.50578187914056));
#166650=CARTESIAN_POINT('Ctrl Pts',(4.71648170664982,15.2,-9.50907925015195));
#166651=CARTESIAN_POINT('Ctrl Pts',(4.71922673423483,15.2,-9.51240087193117));
#166652=CARTESIAN_POINT('Ctrl Pts',(4.7220064462772,15.2,-9.51574610653197));
#166653=CARTESIAN_POINT('Ctrl Pts',(4.72432287285293,15.2,-9.51853380188071));
#166654=CARTESIAN_POINT('Ctrl Pts',(4.72666338229611,15.2,-9.52133789668977));
#166655=CARTESIAN_POINT('Ctrl Pts',(4.72902796299251,15.2,-9.52415802592718));
#166656=CARTESIAN_POINT('Ctrl Pts',(4.73139254368892,15.2,-9.52697815516461));
#166657=CARTESIAN_POINT('Ctrl Pts',(4.73378119318574,15.2,-9.52981431736618));
#166658=CARTESIAN_POINT('Ctrl Pts',(4.7361938955488,15.2,-9.53266615833967));
#166659=CARTESIAN_POINT('Ctrl Pts',(4.73860659764888,15.2,-9.53551799900231));
#166660=CARTESIAN_POINT('Ctrl Pts',(4.74104335202599,15.2,-9.53838551687173));
#166661=CARTESIAN_POINT('Ctrl Pts',(4.74350414168635,15.2,-9.54126835988957));
#166662=CARTESIAN_POINT('Ctrl Pts',(4.74596493161494,15.2,-9.54415120322165));
#166663=CARTESIAN_POINT('Ctrl Pts',(4.7484497562237,15.2,-9.54704937064239));
#166664=CARTESIAN_POINT('Ctrl Pts',(4.75095859768007,15.2,-9.54996251591894));
#166665=CARTESIAN_POINT('Ctrl Pts',(4.75346743913642,15.2,-9.55287566119547));
#166666=CARTESIAN_POINT('Ctrl Pts',(4.75600029617711,15.2,-9.55580378354579));
#166667=CARTESIAN_POINT('Ctrl Pts',(4.75855715046982,15.2,-9.55874654390009));
#166668=CARTESIAN_POINT('Ctrl Pts',(4.76213674653536,15.2,-9.56286640846026));
#166669=CARTESIAN_POINT('Ctrl Pts',(4.76576337720379,15.2,-9.56701495697939));
#166670=CARTESIAN_POINT('Ctrl Pts',(4.76943698523321,15.2,-9.57119127176664));
#166671=CARTESIAN_POINT('Ctrl Pts',(4.77206099092766,15.2,-9.57417435371108));
#166672=CARTESIAN_POINT('Ctrl Pts',(4.77470896504431,15.2,-9.57717160112774));
#166673=CARTESIAN_POINT('Ctrl Pts',(4.77738088497488,15.2,-9.58018268480831));
#166674=CARTESIAN_POINT('Ctrl Pts',(4.78005280490545,15.2,-9.58319376848888));
#166675=CARTESIAN_POINT('Ctrl Pts',(4.78274867295005,15.2,-9.58621868871556));
#166676=CARTESIAN_POINT('Ctrl Pts',(4.78546846372637,15.2,-9.58925712074331));
#166677=CARTESIAN_POINT('Ctrl Pts',(4.78818825450268,15.2,-9.59229555277104));
#166678=CARTESIAN_POINT('Ctrl Pts',(4.79093197017425,15.2,-9.5953474966443));
#166679=CARTESIAN_POINT('Ctrl Pts',(4.7936995873977,15.2,-9.59841262970052));
#166680=CARTESIAN_POINT('Ctrl Pts',(4.79646720462116,15.2,-9.60147776275676));
#166681=CARTESIAN_POINT('Ctrl Pts',(4.79925872182179,15.2,-9.60455608865711));
#166682=CARTESIAN_POINT('Ctrl Pts',(4.80207411668416,15.2,-9.60764728747723));
#166683=CARTESIAN_POINT('Ctrl Pts',(4.80432643238992,15.2,-9.61012024633116));
#166684=CARTESIAN_POINT('Ctrl Pts',(4.80659402907221,15.2,-9.61260144555096));
#166685=CARTESIAN_POINT('Ctrl Pts',(4.80887689494432,15.2,-9.61509072513948));
#166686=CARTESIAN_POINT('Ctrl Pts',(4.81115976112746,15.2,-9.61758000506716));
#166687=CARTESIAN_POINT('Ctrl Pts',(4.81345789653985,15.2,-9.62007736431503));
#166688=CARTESIAN_POINT('Ctrl Pts',(4.81577128722248,15.2,-9.62258264672987));
#166689=CARTESIAN_POINT('Ctrl Pts',(4.81808467758992,15.2,-9.62508792880336));
#166690=CARTESIAN_POINT('Ctrl Pts',(4.82041332369872,15.2,-9.62760113152524));
#166691=CARTESIAN_POINT('Ctrl Pts',(4.82275721261667,15.2,-9.63012210159614));
#166692=CARTESIAN_POINT('Ctrl Pts',(4.82510110185397,15.2,-9.63264307201052));
#166693=CARTESIAN_POINT('Ctrl Pts',(4.82746023271683,15.2,-9.63517180841028));
#166694=CARTESIAN_POINT('Ctrl Pts',(4.82983459396817,15.2,-9.63770815572671));
#166695=CARTESIAN_POINT('Ctrl Pts',(4.832208954896,15.2,-9.64024450269757));
#166696=CARTESIAN_POINT('Ctrl Pts',(4.83459854451597,15.2,-9.64278846171439));
#166697=CARTESIAN_POINT('Ctrl Pts',(4.83700334887337,15.2,-9.64533987861616));
#166698=CARTESIAN_POINT('Ctrl Pts',(4.83940815355843,15.2,-9.64789129586556));
#166699=CARTESIAN_POINT('Ctrl Pts',(4.84182817370882,15.2,-9.65045017198234));
#166700=CARTESIAN_POINT('Ctrl Pts',(4.84426339500821,15.2,-9.65301635523332));
#166701=CARTESIAN_POINT('Ctrl Pts',(4.84669861630759,15.2,-9.65558253848429));
#166702=CARTESIAN_POINT('Ctrl Pts',(4.84914903850876,15.2,-9.65815602873055));
#166703=CARTESIAN_POINT('Ctrl Pts',(4.85161464714468,15.2,-9.66073667720525));
#166704=CARTESIAN_POINT('Ctrl Pts',(4.85408025544467,15.2,-9.66331732532834));
#166705=CARTESIAN_POINT('Ctrl Pts',(4.85656105066872,15.2,-9.6659051301097));
#166706=CARTESIAN_POINT('Ctrl Pts',(4.85905701769819,15.2,-9.66849994446489));
#166707=CARTESIAN_POINT('Ctrl Pts',(4.86155298506772,15.2,-9.67109475917362));
#166708=CARTESIAN_POINT('Ctrl Pts',(4.86406412438483,15.2,-9.67369658477809));
#166709=CARTESIAN_POINT('Ctrl Pts',(4.86659042041294,15.2,-9.67630527214317));
#166710=CARTESIAN_POINT('Ctrl Pts',(4.86974829027598,15.2,-9.67956613117182));
#166711=CARTESIAN_POINT('Ctrl Pts',(4.87292984304499,15.2,-9.68283771485622));
#166712=CARTESIAN_POINT('Ctrl Pts',(4.8761350494358,15.2,-9.68611973791261));
#166713=CARTESIAN_POINT('Ctrl Pts',(4.87869921433883,15.2,-9.68874535614309));
#166714=CARTESIAN_POINT('Ctrl Pts',(4.88127851644015,15.2,-9.69137765576307));
#166715=CARTESIAN_POINT('Ctrl Pts',(4.88387294073979,15.2,-9.69401649478152));
#166716=CARTESIAN_POINT('Ctrl Pts',(4.88646736539291,15.2,-9.69665533415952));
#166717=CARTESIAN_POINT('Ctrl Pts',(4.88907691291499,15.2,-9.69930071231338));
#166718=CARTESIAN_POINT('Ctrl Pts',(4.89170156567069,15.2,-9.70195248762522));
#166719=CARTESIAN_POINT('Ctrl Pts',(4.89498238143651,15.2,-9.70526720658438));
#166720=CARTESIAN_POINT('Ctrl Pts',(4.89828680232771,15.2,-9.708591920502));
#166721=CARTESIAN_POINT('Ctrl Pts',(4.90161479392686,15.2,-9.7119263561278));
#166722=CARTESIAN_POINT('Ctrl Pts',(4.90427718698853,15.2,-9.71459390441036));
#166723=CARTESIAN_POINT('Ctrl Pts',(4.90695466801434,15.2,-9.71726767529121));
#166724=CARTESIAN_POINT('Ctrl Pts',(4.90964721697305,15.2,-9.71994752847316));
#166725=CARTESIAN_POINT('Ctrl Pts',(4.91233976629863,15.2,-9.72262738202025));
#166726=CARTESIAN_POINT('Ctrl Pts',(4.9150473860368,15.2,-9.72531331995113));
#166727=CARTESIAN_POINT('Ctrl Pts',(4.91777005868672,15.2,-9.72800520393178));
#166728=CARTESIAN_POINT('Ctrl Pts',(4.92049273096567,15.2,-9.73069708754565));
#166729=CARTESIAN_POINT('Ctrl Pts',(4.92323045634267,15.2,-9.73339491785597));
#166730=CARTESIAN_POINT('Ctrl Pts',(4.92598321728332,15.2,-9.73609855707902));
#166731=CARTESIAN_POINT('Ctrl Pts',(4.92873597859904,15.2,-9.73880219667045));
#166732=CARTESIAN_POINT('Ctrl Pts',(4.9315037762229,15.2,-9.74151164834323));
#166733=CARTESIAN_POINT('Ctrl Pts',(4.93428659240377,15.2,-9.74422677462734));
#166734=CARTESIAN_POINT('Ctrl Pts',(4.93776511244029,15.2,-9.74762068229751));
#166735=CARTESIAN_POINT('Ctrl Pts',(4.941267098748,15.2,-9.75102345940662));
#166736=CARTESIAN_POINT('Ctrl Pts',(4.94479251923602,15.2,-9.7544348451712));
#166737=CARTESIAN_POINT('Ctrl Pts',(4.94831793972405,15.2,-9.7578462309358));
#166738=CARTESIAN_POINT('Ctrl Pts',(4.9518667911208,15.2,-9.76126622572552));
#166739=CARTESIAN_POINT('Ctrl Pts',(4.95543904244214,15.2,-9.76469457169842));
#166740=CARTESIAN_POINT('Ctrl Pts',(4.95829684326559,15.2,-9.76743724825253));
#166741=CARTESIAN_POINT('Ctrl Pts',(4.96116961839593,15.2,-9.77018527115238));
#166742=CARTESIAN_POINT('Ctrl Pts',(4.96405735000625,15.2,-9.77293850943978));
#166743=CARTESIAN_POINT('Ctrl Pts',(4.96694508201002,15.2,-9.77569174810231));
#166744=CARTESIAN_POINT('Ctrl Pts',(4.96984777119694,15.2,-9.77845020128403));
#166745=CARTESIAN_POINT('Ctrl Pts',(4.97276539796859,15.2,-9.78121374143516));
#166746=CARTESIAN_POINT('Ctrl Pts',(4.97641243123438,15.2,-9.7846681664358));
#166747=CARTESIAN_POINT('Ctrl Pts',(4.98008280670335,15.2,-9.78813053885881));
#166748=CARTESIAN_POINT('Ctrl Pts',(4.98377648719136,15.2,-9.79160061122055));
#166749=CARTESIAN_POINT('Ctrl Pts',(4.9867314313402,15.2,-9.794376668883));
#166750=CARTESIAN_POINT('Ctrl Pts',(4.98970129165934,15.2,-9.79715765257257));
#166751=CARTESIAN_POINT('Ctrl Pts',(4.99268604724769,15.2,-9.79994343778897));
#166752=CARTESIAN_POINT('Ctrl Pts',(4.99567080324272,15.2,-9.80272922338492));
#166753=CARTESIAN_POINT('Ctrl Pts',(4.99867045525731,15.2,-9.80551981066045));
#166754=CARTESIAN_POINT('Ctrl Pts',(5.00168498596239,15.2,-9.80831507489729));
#166755=CARTESIAN_POINT('Ctrl Pts',(5.00469951625674,15.2,-9.81111033875329));
#166756=CARTESIAN_POINT('Ctrl Pts',(5.00772892316488,15.2,-9.81391027710032));
#166757=CARTESIAN_POINT('Ctrl Pts',(5.01077318819283,15.2,-9.81671476953744));
#166758=CARTESIAN_POINT('Ctrl Pts',(5.01381745363556,15.2,-9.81951926235666));
#166759=CARTESIAN_POINT('Ctrl Pts',(5.01687657826893,15.2,-9.82232830744308));
#166760=CARTESIAN_POINT('Ctrl Pts',(5.01995054149299,15.2,-9.82514178226337));
#166761=CARTESIAN_POINT('Ctrl Pts',(5.02379299531365,15.2,-9.82865862559708));
#166762=CARTESIAN_POINT('Ctrl Pts',(5.02765863386107,15.2,-9.83218238931079));
#166763=CARTESIAN_POINT('Ctrl Pts',(5.03154742120973,15.2,-9.83571283941819));
#166764=CARTESIAN_POINT('Ctrl Pts',(5.03465845083434,15.2,-9.83853719927321));
#166765=CARTESIAN_POINT('Ctrl Pts',(5.03778429343989,15.2,-9.84136583625865));
#166766=CARTESIAN_POINT('Ctrl Pts',(5.04092493095995,15.2,-9.84419863152679));
#166767=CARTESIAN_POINT('Ctrl Pts',(5.04406556890792,15.2,-9.84703142718091));
#166768=CARTESIAN_POINT('Ctrl Pts',(5.04722100104379,15.2,-9.84986838097997));
#166769=CARTESIAN_POINT('Ctrl Pts',(5.05039120771752,15.2,-9.85270937319062));
#166770=CARTESIAN_POINT('Ctrl Pts',(5.05356141395932,15.2,-9.85555036501418));
#166771=CARTESIAN_POINT('Ctrl Pts',(5.05674639388866,15.2,-9.85839539606642));
#166772=CARTESIAN_POINT('Ctrl Pts',(5.05994612878567,15.2,-9.86124434808662));
#166773=CARTESIAN_POINT('Ctrl Pts',(5.06314586411864,15.2,-9.86409330049499));
#166774=CARTESIAN_POINT('Ctrl Pts',(5.06636035255929,15.2,-9.86694617341931));
#166775=CARTESIAN_POINT('Ctrl Pts',(5.06958957451402,15.2,-9.8698028497419));
#166776=CARTESIAN_POINT('Ctrl Pts',(5.07281879602876,15.2,-9.87265952567528));
#166777=CARTESIAN_POINT('Ctrl Pts',(5.07606275000721,15.2,-9.87552000557456));
#166778=CARTESIAN_POINT('Ctrl Pts',(5.0793214175171,15.2,-9.87838417350671));
#166779=CARTESIAN_POINT('Ctrl Pts',(5.08258008547098,15.2,-9.8812483418291));
#166780=CARTESIAN_POINT('Ctrl Pts',(5.08585346667739,15.2,-9.88411619788519));
#166781=CARTESIAN_POINT('Ctrl Pts',(5.08914153926046,15.2,-9.88698762677695));
#166782=CARTESIAN_POINT('Ctrl Pts',(5.09242961139553,15.2,-9.88985905527749));
#166783=CARTESIAN_POINT('Ctrl Pts',(5.09573237493298,15.2,-9.89273405530115));
#166784=CARTESIAN_POINT('Ctrl Pts',(5.09904980971583,15.2,-9.89561251578771));
#166785=CARTESIAN_POINT('Ctrl Pts',(5.10236724495068,15.2,-9.89849097666645));
#166786=CARTESIAN_POINT('Ctrl Pts',(5.10569934985637,15.2,-9.90137289553997));
#166787=CARTESIAN_POINT('Ctrl Pts',(5.10904610448321,15.2,-9.904258159975));
#166788=CARTESIAN_POINT('Ctrl Pts',(5.11239285911007,15.2,-9.90714342441002));
#166789=CARTESIAN_POINT('Ctrl Pts',(5.11575426434694,15.2,-9.91003203617322));
#166790=CARTESIAN_POINT('Ctrl Pts',(5.11913029581021,15.2,-9.91292388049782));
#166791=CARTESIAN_POINT('Ctrl Pts',(5.12166231917767,15.2,-9.91509276354427));
#166792=CARTESIAN_POINT('Ctrl Pts',(5.12420257155736,15.2,-9.9172634657072));
#166793=CARTESIAN_POINT('Ctrl Pts',(5.12675104246803,15.2,-9.91943593990367));
#166794=CARTESIAN_POINT('Ctrl Pts',(5.1292995133787,15.2,-9.92160841410014));
#166795=CARTESIAN_POINT('Ctrl Pts',(5.13185620388874,15.2,-9.92378266093279));
#166796=CARTESIAN_POINT('Ctrl Pts',(5.13442110408793,15.2,-9.92595863252054));
#166797=CARTESIAN_POINT('Ctrl Pts',(5.13698600428713,15.2,-9.9281346041083));
#166798=CARTESIAN_POINT('Ctrl Pts',(5.139559113277,15.2,-9.93031230086252));
#166799=CARTESIAN_POINT('Ctrl Pts',(5.14214042397488,15.2,-9.93249167699166));
#166800=CARTESIAN_POINT('Ctrl Pts',(5.14472173467275,15.2,-9.9346710531208));
#166801=CARTESIAN_POINT('Ctrl Pts',(5.14731124576196,15.2,-9.93685210917488));
#166802=CARTESIAN_POINT('Ctrl Pts',(5.14990894795854,15.2,-9.93903479822045));
#166803=CARTESIAN_POINT('Ctrl Pts',(5.15250665015513,15.2,-9.94121748726602));
#166804=CARTESIAN_POINT('Ctrl Pts',(5.15511254299286,15.2,-9.94340180889749));
#166805=CARTESIAN_POINT('Ctrl Pts',(5.15772661923588,15.2,-9.94558771809377));
#166806=CARTESIAN_POINT('Ctrl Pts',(5.16034069547889,15.2,-9.94777362729005));
#166807=CARTESIAN_POINT('Ctrl Pts',(5.16296295305647,15.2,-9.94996112383586));
#166808=CARTESIAN_POINT('Ctrl Pts',(5.1655933832098,15.2,-9.95215016196446));
#166809=CARTESIAN_POINT('Ctrl Pts',(5.16822381384098,15.2,-9.95433920049074));
#166810=CARTESIAN_POINT('Ctrl Pts',(5.17086241622444,15.2,-9.95652978094242));
#166811=CARTESIAN_POINT('Ctrl Pts',(5.17350918286022,15.2,-9.95872185842788));
#166812=CARTESIAN_POINT('Ctrl Pts',(5.17615594901517,15.2,-9.9609139355151));
#166813=CARTESIAN_POINT('Ctrl Pts',(5.17881087726968,15.2,-9.96310750935224));
#166814=CARTESIAN_POINT('Ctrl Pts',(5.18147395950697,15.2,-9.96530253489762));
#166815=CARTESIAN_POINT('Ctrl Pts',(5.18413704174425,15.2,-9.96749756044298));
#166816=CARTESIAN_POINT('Ctrl Pts',(5.18680827773747,15.2,-9.96969403773854));
#166817=CARTESIAN_POINT('Ctrl Pts',(5.18948765748565,15.2,-9.97189192229367));
#166818=CARTESIAN_POINT('Ctrl Pts',(5.19216703723384,15.2,-9.9740898068488));
#166819=CARTESIAN_POINT('Ctrl Pts',(5.19485456173318,15.2,-9.97628909883465));
#166820=CARTESIAN_POINT('Ctrl Pts',(5.19755021952244,15.2,-9.97848975301467));
#166821=CARTESIAN_POINT('Ctrl Pts',(5.2011444302346,15.2,-9.98142395885457));
#166822=CARTESIAN_POINT('Ctrl Pts',(5.20475310328501,15.2,-9.98436058880345));
#166823=CARTESIAN_POINT('Ctrl Pts',(5.20837621331727,15.2,-9.98729953596386));
#166824=CARTESIAN_POINT('Ctrl Pts',(5.21109354559466,15.2,-9.98950374613394));
#166825=CARTESIAN_POINT('Ctrl Pts',(5.2138189997966,15.2,-9.99170926057063));
#166826=CARTESIAN_POINT('Ctrl Pts',(5.21655256507298,15.2,-9.9939160356989));
#166827=CARTESIAN_POINT('Ctrl Pts',(5.21928613034937,15.2,-9.99612281082715));
#166828=CARTESIAN_POINT('Ctrl Pts',(5.22202780768977,15.2,-9.9983308470389));
#166829=CARTESIAN_POINT('Ctrl Pts',(5.22477758647739,15.2,-10.0005400987603));
#166830=CARTESIAN_POINT('Ctrl Pts',(5.22752736526501,15.2,-10.0027493504818));
#166831=CARTESIAN_POINT('Ctrl Pts',(5.23028524676868,15.2,-10.0049598200516));
#166832=CARTESIAN_POINT('Ctrl Pts',(5.23305121951404,15.2,-10.0071714627313));
#166833=CARTESIAN_POINT('Ctrl Pts',(5.23581719225941,15.2,-10.009383105411));
#166834=CARTESIAN_POINT('Ctrl Pts',(5.23859125696523,15.2,-10.0115959222059));
#166835=CARTESIAN_POINT('Ctrl Pts',(5.24137340369677,15.2,-10.0138098702504));
#166836=CARTESIAN_POINT('Ctrl Pts',(5.24415555042832,15.2,-10.0160238182948));
#166837=CARTESIAN_POINT('Ctrl Pts',(5.2469457794593,15.2,-10.0182388958809));
#166838=CARTESIAN_POINT('Ctrl Pts',(5.2497440806482,15.2,-10.0204550620086));
#166839=CARTESIAN_POINT('Ctrl Pts',(5.25254238234546,15.2,-10.0226712285388));
#166840=CARTESIAN_POINT('Ctrl Pts',(5.25534875561998,15.2,-10.0248884839444));
#166841=CARTESIAN_POINT('Ctrl Pts',(5.25816319136344,15.2,-10.0271067845169));
#166842=CARTESIAN_POINT('Ctrl Pts',(5.26097762659562,15.2,-10.0293250846865));
#166843=CARTESIAN_POINT('Ctrl Pts',(5.26380012429403,15.2,-10.0315444305393));
#166844=CARTESIAN_POINT('Ctrl Pts',(5.26663067352522,15.2,-10.0337647797087));
#166845=CARTESIAN_POINT('Ctrl Pts',(5.2694612227564,15.2,-10.0359851288781));
#166846=CARTESIAN_POINT('Ctrl Pts',(5.27229982402627,15.2,-10.0382064818227));
#166847=CARTESIAN_POINT('Ctrl Pts',(5.27514646726914,15.2,-10.0404287960437));
#166848=CARTESIAN_POINT('Ctrl Pts',(5.27799311051202,15.2,-10.0426511102647));
#166849=CARTESIAN_POINT('Ctrl Pts',(5.28084779672167,15.2,-10.0448743869687));
#166850=CARTESIAN_POINT('Ctrl Pts',(5.28371051350562,15.2,-10.0470985826897));
#166851=CARTESIAN_POINT('Ctrl Pts',(5.28657323028958,15.2,-10.0493227784106));
#166852=CARTESIAN_POINT('Ctrl Pts',(5.28944397922486,15.2,-10.0515478941217));
#166853=CARTESIAN_POINT('Ctrl Pts',(5.2923227494529,15.2,-10.0537738882491));
#166854=CARTESIAN_POINT('Ctrl Pts',(5.2961611101056,15.2,-10.0567418806885));
#166855=CARTESIAN_POINT('Ctrl Pts',(5.30001373151003,15.2,-10.0597114351726));
#166856=CARTESIAN_POINT('Ctrl Pts',(5.3038805888328,15.2,-10.0626824525012));
#166857=CARTESIAN_POINT('Ctrl Pts',(5.30678073156146,15.2,-10.0649107152953));
#166858=CARTESIAN_POINT('Ctrl Pts',(5.30968888252856,15.2,-10.0671398029896));
#166859=CARTESIAN_POINT('Ctrl Pts',(5.31260503076921,15.2,-10.0693696727104));
#166860=CARTESIAN_POINT('Ctrl Pts',(5.31552117900986,15.2,-10.0715995424311));
#166861=CARTESIAN_POINT('Ctrl Pts',(5.31844532504048,15.2,-10.0738301953356));
#166862=CARTESIAN_POINT('Ctrl Pts',(5.32137745823889,15.2,-10.0760615895146));
#166863=CARTESIAN_POINT('Ctrl Pts',(5.3243095914373,15.2,-10.0782929836937));
#166864=CARTESIAN_POINT('Ctrl Pts',(5.32724971145315,15.2,-10.0805251195045));
#166865=CARTESIAN_POINT('Ctrl Pts',(5.33019780817868,15.2,-10.0827579567566));
#166866=CARTESIAN_POINT('Ctrl Pts',(5.33314590490421,15.2,-10.0849907940088));
#166867=CARTESIAN_POINT('Ctrl Pts',(5.33610197836251,15.2,-10.0872243339776));
#166868=CARTESIAN_POINT('Ctrl Pts',(5.33906601854541,15.2,-10.0894585347713));
#166869=CARTESIAN_POINT('Ctrl Pts',(5.34203005926677,15.2,-10.0916927359709));
#166870=CARTESIAN_POINT('Ctrl Pts',(5.34500206646536,15.2,-10.0939276000957));
#166871=CARTESIAN_POINT('Ctrl Pts',(5.34798202964953,15.2,-10.0961630852123));
#166872=CARTESIAN_POINT('Ctrl Pts',(5.35096199229233,15.2,-10.0983985699229));
#166873=CARTESIAN_POINT('Ctrl Pts',(5.35394991103786,15.2,-10.1006346766689));
#166874=CARTESIAN_POINT('Ctrl Pts',(5.35694577437126,15.2,-10.1028713629494));
#166875=CARTESIAN_POINT('Ctrl Pts',(5.35994163770466,15.2,-10.10510804923));
#166876=CARTESIAN_POINT('Ctrl Pts',(5.36294544513703,15.2,-10.1073453142585));
#166877=CARTESIAN_POINT('Ctrl Pts',(5.36595718781997,15.2,-10.1095831229689));
#166878=CARTESIAN_POINT('Ctrl Pts',(5.3689689305029,15.2,-10.1118209316793));
#166879=CARTESIAN_POINT('Ctrl Pts',(5.37198860734323,15.2,-10.114059283598));
#166880=CARTESIAN_POINT('Ctrl Pts',(5.37501620998321,15.2,-10.1162981422667));
#166881=CARTESIAN_POINT('Ctrl Pts',(5.3780438126232,15.2,-10.1185370009353));
#166882=CARTESIAN_POINT('Ctrl Pts',(5.38107934056289,15.2,-10.1207763669873));
#166883=CARTESIAN_POINT('Ctrl Pts',(5.38412278120162,15.2,-10.1230161955309));
#166884=CARTESIAN_POINT('Ctrl Pts',(5.38716622184035,15.2,-10.1252560240745));
#166885=CARTESIAN_POINT('Ctrl Pts',(5.39021757455064,15.2,-10.1274963140527));
#166886=CARTESIAN_POINT('Ctrl Pts',(5.39327682838308,15.2,-10.1297370198332));
#166887=CARTESIAN_POINT('Ctrl Pts',(5.39633608221551,15.2,-10.1319777256136));
#166888=CARTESIAN_POINT('Ctrl Pts',(5.39940323605899,15.2,-10.1342188453762));
#166889=CARTESIAN_POINT('Ctrl Pts',(5.4024782818212,15.2,-10.1364603530864));
#166890=CARTESIAN_POINT('Ctrl Pts',(5.4065783432099,15.2,-10.1394490303047));
#166891=CARTESIAN_POINT('Ctrl Pts',(5.4106924385417,15.2,-10.1424383928519));
#166892=CARTESIAN_POINT('Ctrl Pts',(5.41482055299994,15.2,-10.145428447));
#166893=CARTESIAN_POINT('Ctrl Pts',(4.57383771099994,12.2,-9.31239140100002));
#166894=CARTESIAN_POINT('Ctrl Pts',(4.57476026769951,12.2,-9.31392144680197));
#166895=CARTESIAN_POINT('Ctrl Pts',(4.57571693070584,12.2,-9.31549767344764));
#166896=CARTESIAN_POINT('Ctrl Pts',(4.57670776760804,12.2,-9.31711891458905));
#166897=CARTESIAN_POINT('Ctrl Pts',(4.57770338282661,12.2,-9.31874797417473));
#166898=CARTESIAN_POINT('Ctrl Pts',(4.57873349763143,12.2,-9.32042248430923));
#166899=CARTESIAN_POINT('Ctrl Pts',(4.57979816282796,12.2,-9.32214130040799));
#166900=CARTESIAN_POINT('Ctrl Pts',(4.58086282792779,12.2,-9.32386011635063));
#166901=CARTESIAN_POINT('Ctrl Pts',(4.58196204049941,12.2,-9.32562323961556));
#166902=CARTESIAN_POINT('Ctrl Pts',(4.58309584770821,12.2,-9.32742955654993));
#166903=CARTESIAN_POINT('Ctrl Pts',(4.58422965491702,12.2,-9.32923587348429));
#166904=CARTESIAN_POINT('Ctrl Pts',(4.5853980563192,12.2,-9.33108538508538));
#166905=CARTESIAN_POINT('Ctrl Pts',(4.58660109166692,12.2,-9.33297701302539));
#166906=CARTESIAN_POINT('Ctrl Pts',(4.58780412712392,12.2,-9.33486864113721));
#166907=CARTESIAN_POINT('Ctrl Pts',(4.58904179768353,12.2,-9.33680238271311));
#166908=CARTESIAN_POINT('Ctrl Pts',(4.59031413808858,12.2,-9.33877718824021));
#166909=CARTESIAN_POINT('Ctrl Pts',(4.59158647837806,12.2,-9.34075199358794));
#166910=CARTESIAN_POINT('Ctrl Pts',(4.59289349004307,12.2,-9.34276786523282));
#166911=CARTESIAN_POINT('Ctrl Pts',(4.5942352060005,12.2,-9.34482377850088));
#166912=CARTESIAN_POINT('Ctrl Pts',(4.59557692195793,12.2,-9.34687969176897));
#166913=CARTESIAN_POINT('Ctrl Pts',(4.59695334073424,12.2,-9.34897564678802));
#166914=CARTESIAN_POINT('Ctrl Pts',(4.59836449093146,12.2,-9.35111065112542));
#166915=CARTESIAN_POINT('Ctrl Pts',(4.59977564125686,12.2,-9.35324565565676));
#166916=CARTESIAN_POINT('Ctrl Pts',(4.60122152409488,12.2,-9.35541970753459));
#166917=CARTESIAN_POINT('Ctrl Pts',(4.60270216417795,12.2,-9.35763183999108));
#166918=CARTESIAN_POINT('Ctrl Pts',(4.60418280412651,12.2,-9.35984397224663));
#166919=CARTESIAN_POINT('Ctrl Pts',(4.60569820106435,12.2,-9.36209418342296));
#166920=CARTESIAN_POINT('Ctrl Pts',(4.60724837709285,12.2,-9.36438152917477));
#166921=CARTESIAN_POINT('Ctrl Pts',(4.60879855312135,12.2,-9.36666887492659));
#166922=CARTESIAN_POINT('Ctrl Pts',(4.61038350778881,12.2,-9.36899335881716));
#166923=CARTESIAN_POINT('Ctrl Pts',(4.61200325789508,12.2,-9.37135405564644));
#166924=CARTESIAN_POINT('Ctrl Pts',(4.61362300800136,12.2,-9.37371475247571));
#166925=CARTESIAN_POINT('Ctrl Pts',(4.6152775579795,12.2,-9.3761116657423));
#166926=CARTESIAN_POINT('Ctrl Pts',(4.61696691708242,12.2,-9.37854389648485));
#166927=CARTESIAN_POINT('Ctrl Pts',(4.61865627633879,12.2,-9.38097612744834));
#166928=CARTESIAN_POINT('Ctrl Pts',(4.62038044630684,12.2,-9.38344367723194));
#166929=CARTESIAN_POINT('Ctrl Pts',(4.6221394413209,12.2,-9.38594566836979));
#166930=CARTESIAN_POINT('Ctrl Pts',(4.62389843617516,12.2,-9.38844765928039));
#166931=CARTESIAN_POINT('Ctrl Pts',(4.62569225239893,12.2,-9.39098409241391));
#166932=CARTESIAN_POINT('Ctrl Pts',(4.62752090125738,12.2,-9.39355411249878));
#166933=CARTESIAN_POINT('Ctrl Pts',(4.62965432503632,12.2,-9.39655246942012));
#166934=CARTESIAN_POINT('Ctrl Pts',(4.63183515898931,12.2,-9.39959654241051));
#166935=CARTESIAN_POINT('Ctrl Pts',(4.63406341059595,12.2,-9.4026850069196));
#166936=CARTESIAN_POINT('Ctrl Pts',(4.63597334044536,12.2,-9.40533226207569));
#166937=CARTESIAN_POINT('Ctrl Pts',(4.63791810759893,12.2,-9.40801213163557));
#166938=CARTESIAN_POINT('Ctrl Pts',(4.63989771385882,12.2,-9.41072380386899));
#166939=CARTESIAN_POINT('Ctrl Pts',(4.64187732011872,12.2,-9.41343547610242));
#166940=CARTESIAN_POINT('Ctrl Pts',(4.64389176767837,12.2,-9.41617895175048));
#166941=CARTESIAN_POINT('Ctrl Pts',(4.64594105451818,12.2,-9.41895343414755));
#166942=CARTESIAN_POINT('Ctrl Pts',(4.64799034154415,12.2,-9.42172791679664));
#166943=CARTESIAN_POINT('Ctrl Pts',(4.65007446671519,12.2,-9.42453340810711));
#166944=CARTESIAN_POINT('Ctrl Pts',(4.65219342783218,12.2,-9.42736913067964));
#166945=CARTESIAN_POINT('Ctrl Pts',(4.65431238875671,12.2,-9.43020485299459));
#166946=CARTESIAN_POINT('Ctrl Pts',(4.6564661859602,12.2,-9.43307080742409));
#166947=CARTESIAN_POINT('Ctrl Pts',(4.65865481280723,12.2,-9.43596623199865));
#166948=CARTESIAN_POINT('Ctrl Pts',(4.66084343965424,12.2,-9.43886165657323));
#166949=CARTESIAN_POINT('Ctrl Pts',(4.66306689596317,12.2,-9.4417865522873));
#166950=CARTESIAN_POINT('Ctrl Pts',(4.66532517296207,12.2,-9.44474017667803));
#166951=CARTESIAN_POINT('Ctrl Pts',(4.66758345016611,12.2,-9.44769380133706));
#166952=CARTESIAN_POINT('Ctrl Pts',(4.66987654967998,12.2,-9.45067615296685));
#166953=CARTESIAN_POINT('Ctrl Pts',(4.67220445892517,12.2,-9.45368650503292));
#166954=CARTESIAN_POINT('Ctrl Pts',(4.6745323679589,12.2,-9.45669685682556));
#166955=CARTESIAN_POINT('Ctrl Pts',(4.67689508671198,12.2,-9.45973520780301));
#166956=CARTESIAN_POINT('Ctrl Pts',(4.67929260254153,12.2,-9.46280084644161));
#166957=CARTESIAN_POINT('Ctrl Pts',(4.68169011837108,12.2,-9.46586648508022));
#166958=CARTESIAN_POINT('Ctrl Pts',(4.68412243150472,12.2,-9.46895940989898));
#166959=CARTESIAN_POINT('Ctrl Pts',(4.68658952378631,12.2,-9.47207892468993));
#166960=CARTESIAN_POINT('Ctrl Pts',(4.68864543409567,12.2,-9.47467852044351));
#166961=CARTESIAN_POINT('Ctrl Pts',(4.69072549915812,12.2,-9.4772965804064));
#166962=CARTESIAN_POINT('Ctrl Pts',(4.69282970658743,12.2,-9.47993270783602));
#166963=CARTESIAN_POINT('Ctrl Pts',(4.69493391401673,12.2,-9.48256883526565));
#166964=CARTESIAN_POINT('Ctrl Pts',(4.69706226372717,12.2,-9.48522303139291));
#166965=CARTESIAN_POINT('Ctrl Pts',(4.69921474685093,12.2,-9.48789490535034));
#166966=CARTESIAN_POINT('Ctrl Pts',(4.70136722997468,12.2,-9.49056677930778));
#166967=CARTESIAN_POINT('Ctrl Pts',(4.70354384427209,12.2,-9.49325633018069));
#166968=CARTESIAN_POINT('Ctrl Pts',(4.70574457678203,12.2,-9.49596317595684));
#166969=CARTESIAN_POINT('Ctrl Pts',(4.70794530929197,12.2,-9.49867002173299));
#166970=CARTESIAN_POINT('Ctrl Pts',(4.71017016234989,12.2,-9.50139416148887));
#166971=CARTESIAN_POINT('Ctrl Pts',(4.71241912047488,12.2,-9.50413521822497));
#166972=CARTESIAN_POINT('Ctrl Pts',(4.71466807859987,12.2,-9.50687627496106));
#166973=CARTESIAN_POINT('Ctrl Pts',(4.71694114156841,12.2,-9.50963424783884));
#166974=CARTESIAN_POINT('Ctrl Pts',(4.71923829650947,12.2,-9.51240876618482));
#166975=CARTESIAN_POINT('Ctrl Pts',(4.72153545145053,12.2,-9.51518328453081));
#166976=CARTESIAN_POINT('Ctrl Pts',(4.72385669858549,12.2,-9.51797434746616));
#166977=CARTESIAN_POINT('Ctrl Pts',(4.72620202087842,12.2,-9.52078159017534));
#166978=CARTESIAN_POINT('Ctrl Pts',(4.72854734317134,12.2,-9.52358883288451));
#166979=CARTESIAN_POINT('Ctrl Pts',(4.73091674152754,12.2,-9.5264122556905));
#166980=CARTESIAN_POINT('Ctrl Pts',(4.73331019888989,12.2,-9.52925149742742));
#166981=CARTESIAN_POINT('Ctrl Pts',(4.73570365625225,12.2,-9.53209073916435));
#166982=CARTESIAN_POINT('Ctrl Pts',(4.73812117286532,12.2,-9.53494580107768));
#166983=CARTESIAN_POINT('Ctrl Pts',(4.74056273201673,12.2,-9.53781632733326));
#166984=CARTESIAN_POINT('Ctrl Pts',(4.74300429116814,12.2,-9.54068685358883));
#166985=CARTESIAN_POINT('Ctrl Pts',(4.74546989343469,12.2,-9.54357284476711));
#166986=CARTESIAN_POINT('Ctrl Pts',(4.7479595183672,12.2,-9.54647395317112));
#166987=CARTESIAN_POINT('Ctrl Pts',(4.75044914329972,12.2,-9.54937506157513));
#166988=CARTESIAN_POINT('Ctrl Pts',(4.75296279254097,12.2,-9.55229128474327));
#166989=CARTESIAN_POINT('Ctrl Pts',(4.75550044580681,12.2,-9.55522228009169));
#166990=CARTESIAN_POINT('Ctrl Pts',(4.75803809879606,12.2,-9.55815327512063));
#166991=CARTESIAN_POINT('Ctrl Pts',(4.76059975812328,12.2,-9.56109904482553));
#166992=CARTESIAN_POINT('Ctrl Pts',(4.76318540110335,12.2,-9.56405924561279));
#166993=CARTESIAN_POINT('Ctrl Pts',(4.76628817318676,12.2,-9.56761148713828));
#166994=CARTESIAN_POINT('Ctrl Pts',(4.76942548359022,12.2,-9.57118451397422));
#166995=CARTESIAN_POINT('Ctrl Pts',(4.77259729568122,12.2,-9.57477774842089));
#166996=CARTESIAN_POINT('Ctrl Pts',(4.77524047227967,12.2,-9.57777211029659));
#166997=CARTESIAN_POINT('Ctrl Pts',(4.7779076078581,12.2,-9.58078050513585));
#166998=CARTESIAN_POINT('Ctrl Pts',(4.78059868265102,12.2,-9.5838026062477));
#166999=CARTESIAN_POINT('Ctrl Pts',(4.78328975744394,12.2,-9.58682470735954));
#167000=CARTESIAN_POINT('Ctrl Pts',(4.78600476912389,12.2,-9.58986051461742));
#167001=CARTESIAN_POINT('Ctrl Pts',(4.78874369585958,12.2,-9.59290970435399));
#167002=CARTESIAN_POINT('Ctrl Pts',(4.79148262259527,12.2,-9.59595889409057));
#167003=CARTESIAN_POINT('Ctrl Pts',(4.79424546551801,12.2,-9.59902146576233));
#167004=CARTESIAN_POINT('Ctrl Pts',(4.79703219808939,12.2,-9.60209710194394));
#167005=CARTESIAN_POINT('Ctrl Pts',(4.79926158396424,12.2,-9.60455761068807));
#167006=CARTESIAN_POINT('Ctrl Pts',(4.80150626298157,12.2,-9.60702647992004));
#167007=CARTESIAN_POINT('Ctrl Pts',(4.80376621807361,12.2,-9.60950354877256));
#167008=CARTESIAN_POINT('Ctrl Pts',(4.80602617347356,12.2,-9.61198061796259));
#167009=CARTESIAN_POINT('Ctrl Pts',(4.80830140771829,12.2,-9.6144658881857));
#167010=CARTESIAN_POINT('Ctrl Pts',(4.81059190779221,12.2,-9.6169591981135));
#167011=CARTESIAN_POINT('Ctrl Pts',(4.81345503272857,12.2,-9.6200758353534));
#167012=CARTESIAN_POINT('Ctrl Pts',(4.81634200971201,12.2,-9.62320503612101));
#167013=CARTESIAN_POINT('Ctrl Pts',(4.81925281367229,12.2,-9.62634649167755));
#167014=CARTESIAN_POINT('Ctrl Pts',(4.82158145665014,12.2,-9.62885965591734));
#167015=CARTESIAN_POINT('Ctrl Pts',(4.82392534859546,12.2,-9.63138066453388));
#167016=CARTESIAN_POINT('Ctrl Pts',(4.82628447629051,12.2,-9.63390936199334));
#167017=CARTESIAN_POINT('Ctrl Pts',(4.82864360430698,12.2,-9.63643805979733));
#167018=CARTESIAN_POINT('Ctrl Pts',(4.83101796937634,12.2,-9.638974445925));
#167019=CARTESIAN_POINT('Ctrl Pts',(4.83340755557171,12.2,-9.64151836663583));
#167020=CARTESIAN_POINT('Ctrl Pts',(4.8357971414415,12.2,-9.64406228700005));
#167021=CARTESIAN_POINT('Ctrl Pts',(4.83820194925935,12.2,-9.64661374168387));
#167022=CARTESIAN_POINT('Ctrl Pts',(4.84062196556053,12.2,-9.64917257980754));
#167023=CARTESIAN_POINT('Ctrl Pts',(4.84304198219142,12.2,-9.65173141827984));
#167024=CARTESIAN_POINT('Ctrl Pts',(4.84547720705748,12.2,-9.65429763929749));
#167025=CARTESIAN_POINT('Ctrl Pts',(4.84792762569202,12.2,-9.65687109199377));
#167026=CARTESIAN_POINT('Ctrl Pts',(4.85037804399269,12.2,-9.65944454433941));
#167027=CARTESIAN_POINT('Ctrl Pts',(4.85284365539239,12.2,-9.66202522954351));
#167028=CARTESIAN_POINT('Ctrl Pts',(4.85532444708999,12.2,-9.66461299784952));
#167029=CARTESIAN_POINT('Ctrl Pts',(4.8578052391256,12.2,-9.66720076650812));
#167030=CARTESIAN_POINT('Ctrl Pts',(4.86030121057858,12.2,-9.66979561792327));
#167031=CARTESIAN_POINT('Ctrl Pts',(4.86281234593865,12.2,-9.67239740645441));
#167032=CARTESIAN_POINT('Ctrl Pts',(4.86532348095657,12.2,-9.67499919463106));
#167033=CARTESIAN_POINT('Ctrl Pts',(4.86784978065201,12.2,-9.67760791779519));
#167034=CARTESIAN_POINT('Ctrl Pts',(4.87039122960937,12.2,-9.68022343208069));
#167035=CARTESIAN_POINT('Ctrl Pts',(4.87293267891299,12.2,-9.68283894672254));
#167036=CARTESIAN_POINT('Ctrl Pts',(4.87548927804419,12.2,-9.68546125174097));
#167037=CARTESIAN_POINT('Ctrl Pts',(4.87806101075164,12.2,-9.68809020178511));
#167038=CARTESIAN_POINT('Ctrl Pts',(4.88063274310869,12.2,-9.69071915147105));
#167039=CARTESIAN_POINT('Ctrl Pts',(4.88321960949983,12.2,-9.69335474786243));
#167040=CARTESIAN_POINT('Ctrl Pts',(4.88582159384114,12.2,-9.69599684753468));
#167041=CARTESIAN_POINT('Ctrl Pts',(4.88842357853696,12.2,-9.6986389475669));
#167042=CARTESIAN_POINT('Ctrl Pts',(4.89104068168142,12.2,-9.70128755079418));
#167043=CARTESIAN_POINT('Ctrl Pts',(4.89367288699155,12.2,-9.70394251604998));
#167044=CARTESIAN_POINT('Ctrl Pts',(4.89630509230166,12.2,-9.70659748130578));
#167045=CARTESIAN_POINT('Ctrl Pts',(4.89895240050244,12.2,-9.70925880748178));
#167046=CARTESIAN_POINT('Ctrl Pts',(4.90161479392686,12.2,-9.7119263561278));
#167047=CARTESIAN_POINT('Ctrl Pts',(4.90427718698853,12.2,-9.71459390441036));
#167048=CARTESIAN_POINT('Ctrl Pts',(4.90695466801434,12.2,-9.71726767529121));
#167049=CARTESIAN_POINT('Ctrl Pts',(4.90964721697305,12.2,-9.71994752847316));
#167050=CARTESIAN_POINT('Ctrl Pts',(4.91233976629863,12.2,-9.72262738202025));
#167051=CARTESIAN_POINT('Ctrl Pts',(4.9150473860368,12.2,-9.72531331995113));
#167052=CARTESIAN_POINT('Ctrl Pts',(4.91777005868672,12.2,-9.72800520393178));
#167053=CARTESIAN_POINT('Ctrl Pts',(4.92049273096567,12.2,-9.73069708754566));
#167054=CARTESIAN_POINT('Ctrl Pts',(4.92323045634267,12.2,-9.73339491785597));
#167055=CARTESIAN_POINT('Ctrl Pts',(4.92598321728332,12.2,-9.73609855707902));
#167056=CARTESIAN_POINT('Ctrl Pts',(4.92873597859904,12.2,-9.73880219667045));
#167057=CARTESIAN_POINT('Ctrl Pts',(4.9315037762229,12.2,-9.74151164834323));
#167058=CARTESIAN_POINT('Ctrl Pts',(4.93428659240377,12.2,-9.74422677462734));
#167059=CARTESIAN_POINT('Ctrl Pts',(4.93706940820549,12.2,-9.74694190054151));
#167060=CARTESIAN_POINT('Ctrl Pts',(4.93986724227323,12.2,-9.74966270318374));
#167061=CARTESIAN_POINT('Ctrl Pts',(4.94268007848674,12.2,-9.75238904829383));
#167062=CARTESIAN_POINT('Ctrl Pts',(4.94619612404108,12.2,-9.75579697996004));
#167063=CARTESIAN_POINT('Ctrl Pts',(4.94973560847935,12.2,-9.75921357279315));
#167064=CARTESIAN_POINT('Ctrl Pts',(4.95329849903368,12.2,-9.76263856779271));
#167065=CARTESIAN_POINT('Ctrl Pts',(4.95614881163249,12.2,-9.76537856394169));
#167066=CARTESIAN_POINT('Ctrl Pts',(4.95901410263243,12.2,-9.76812393955583));
#167067=CARTESIAN_POINT('Ctrl Pts',(4.96189435593458,12.2,-9.77087456139916));
#167068=CARTESIAN_POINT('Ctrl Pts',(4.96477460884431,12.2,-9.77362518286772));
#167069=CARTESIAN_POINT('Ctrl Pts',(4.9676698214871,12.2,-9.77638105316425));
#167070=CARTESIAN_POINT('Ctrl Pts',(4.97057997830379,12.2,-9.77914204154933));
#167071=CARTESIAN_POINT('Ctrl Pts',(4.97421767462202,12.2,-9.78259327731281));
#167072=CARTESIAN_POINT('Ctrl Pts',(4.97787871967697,12.2,-9.78605251049038));
#167073=CARTESIAN_POINT('Ctrl Pts',(4.98156307550907,12.2,-9.78951949298997));
#167074=CARTESIAN_POINT('Ctrl Pts',(4.98524743134117,12.2,-9.79298647548955));
#167075=CARTESIAN_POINT('Ctrl Pts',(4.98895510245724,12.2,-9.7964612059838));
#167076=CARTESIAN_POINT('Ctrl Pts',(4.99268604724769,12.2,-9.79994343778897));
#167077=CARTESIAN_POINT('Ctrl Pts',(4.99567080324272,12.2,-9.80272922338492));
#167078=CARTESIAN_POINT('Ctrl Pts',(4.99867045525731,12.2,-9.80551981066045));
#167079=CARTESIAN_POINT('Ctrl Pts',(5.00168498596239,12.2,-9.80831507489729));
#167080=CARTESIAN_POINT('Ctrl Pts',(5.00469951625674,12.2,-9.81111033875329));
#167081=CARTESIAN_POINT('Ctrl Pts',(5.00772892316488,12.2,-9.81391027710032));
#167082=CARTESIAN_POINT('Ctrl Pts',(5.01077318819283,12.2,-9.81671476953744));
#167083=CARTESIAN_POINT('Ctrl Pts',(5.01381745363556,12.2,-9.81951926235666));
#167084=CARTESIAN_POINT('Ctrl Pts',(5.01687657826894,12.2,-9.82232830744308));
#167085=CARTESIAN_POINT('Ctrl Pts',(5.019950541493,12.2,-9.82514178226338));
#167086=CARTESIAN_POINT('Ctrl Pts',(5.02302450429823,12.2,-9.82795525670034));
#167087=CARTESIAN_POINT('Ctrl Pts',(5.02611330502179,12.2,-9.83077316011948));
#167088=CARTESIAN_POINT('Ctrl Pts',(5.02921692603295,12.2,-9.83359537280717));
#167089=CARTESIAN_POINT('Ctrl Pts',(5.03232054746697,12.2,-9.83641758587938));
#167090=CARTESIAN_POINT('Ctrl Pts',(5.03543898819278,12.2,-9.83924410726024));
#167091=CARTESIAN_POINT('Ctrl Pts',(5.03857222753117,12.2,-9.84207481674811));
#167092=CARTESIAN_POINT('Ctrl Pts',(5.04170546644265,12.2,-9.8449055258503));
#167093=CARTESIAN_POINT('Ctrl Pts',(5.04485350520118,12.2,-9.8477404231461));
#167094=CARTESIAN_POINT('Ctrl Pts',(5.04801632277444,12.2,-9.85057938780249));
#167095=CARTESIAN_POINT('Ctrl Pts',(5.05117914077863,12.2,-9.85341835284568));
#167096=CARTESIAN_POINT('Ctrl Pts',(5.0543567388913,12.2,-9.85626138643381));
#167097=CARTESIAN_POINT('Ctrl Pts',(5.05754909496873,12.2,-9.85910837126861));
#167098=CARTESIAN_POINT('Ctrl Pts',(5.06153953984804,12.2,-9.86266710211814));
#167099=CARTESIAN_POINT('Ctrl Pts',(5.06555304729059,12.2,-9.86623200453327));
#167100=CARTESIAN_POINT('Ctrl Pts',(5.06958957451401,12.2,-9.8698028497419));
#167101=CARTESIAN_POINT('Ctrl Pts',(5.07281879602875,12.2,-9.87265952567528));
#167102=CARTESIAN_POINT('Ctrl Pts',(5.07606275000722,12.2,-9.87552000557456));
#167103=CARTESIAN_POINT('Ctrl Pts',(5.0793214175171,12.2,-9.87838417350671));
#167104=CARTESIAN_POINT('Ctrl Pts',(5.08258008547098,12.2,-9.8812483418291));
#167105=CARTESIAN_POINT('Ctrl Pts',(5.08585346667739,12.2,-9.88411619788519));
#167106=CARTESIAN_POINT('Ctrl Pts',(5.08914153926046,12.2,-9.88698762677695));
#167107=CARTESIAN_POINT('Ctrl Pts',(5.0932516297653,12.2,-9.89057691269605));
#167108=CARTESIAN_POINT('Ctrl Pts',(5.09738467640395,12.2,-9.89417178020187));
#167109=CARTESIAN_POINT('Ctrl Pts',(5.10154063703015,12.2,-9.89777200874382));
#167110=CARTESIAN_POINT('Ctrl Pts',(5.10486540525931,12.2,-9.90065219134192));
#167111=CARTESIAN_POINT('Ctrl Pts',(5.10820483866885,12.2,-9.90353580266432));
#167112=CARTESIAN_POINT('Ctrl Pts',(5.1115589162265,12.2,-9.90642273376132));
#167113=CARTESIAN_POINT('Ctrl Pts',(5.11491299424114,12.2,-9.90930966525166));
#167114=CARTESIAN_POINT('Ctrl Pts',(5.11828171662183,12.2,-9.91219991338946));
#167115=CARTESIAN_POINT('Ctrl Pts',(5.12166506121053,12.2,-9.91509336772697));
#167116=CARTESIAN_POINT('Ctrl Pts',(5.12420256942157,12.2,-9.91726345828299));
#167117=CARTESIAN_POINT('Ctrl Pts',(5.1267483029788,12.2,-9.91943535220047));
#167118=CARTESIAN_POINT('Ctrl Pts',(5.12930225227257,12.2,-9.92160900275636));
#167119=CARTESIAN_POINT('Ctrl Pts',(5.13185620156634,12.2,-9.92378265331226));
#167120=CARTESIAN_POINT('Ctrl Pts',(5.13441836786396,12.2,-9.92595806039197));
#167121=CARTESIAN_POINT('Ctrl Pts',(5.13698873968652,12.2,-9.92813517697939));
#167122=CARTESIAN_POINT('Ctrl Pts',(5.13955911150909,12.2,-9.93031229356681));
#167123=CARTESIAN_POINT('Ctrl Pts',(5.14213769076441,12.2,-9.9324911200041));
#167124=CARTESIAN_POINT('Ctrl Pts',(5.14472446746098,12.2,-9.93467161100799));
#167125=CARTESIAN_POINT('Ctrl Pts',(5.14731124462747,12.2,-9.93685210240799));
#167126=CARTESIAN_POINT('Ctrl Pts',(5.14990621883794,12.2,-9.93903425782513));
#167127=CARTESIAN_POINT('Ctrl Pts',(5.15250938109238,12.2,-9.94121803076773));
#167128=CARTESIAN_POINT('Ctrl Pts',(5.15511254287392,12.2,-9.94340180331361));
#167129=CARTESIAN_POINT('Ctrl Pts',(5.15772389388682,12.2,-9.9455871930265));
#167130=CARTESIAN_POINT('Ctrl Pts',(5.16034342329846,12.2,-9.94777415563981));
#167131=CARTESIAN_POINT('Ctrl Pts',(5.16296295271009,12.2,-9.94996111825313));
#167132=CARTESIAN_POINT('Ctrl Pts',(5.16559066093239,12.2,-9.95214965205152));
#167133=CARTESIAN_POINT('Ctrl Pts',(5.16822653779567,12.2,-9.95433971351375));
#167134=CARTESIAN_POINT('Ctrl Pts',(5.17086241465894,12.2,-9.95652977497597));
#167135=CARTESIAN_POINT('Ctrl Pts',(5.17350646224624,12.2,-9.95872136234635));
#167136=CARTESIAN_POINT('Ctrl Pts',(5.17615866898321,12.2,-9.96091443276667));
#167137=CARTESIAN_POINT('Ctrl Pts',(5.17881087572018,12.2,-9.96310750318699));
#167138=CARTESIAN_POINT('Ctrl Pts',(5.18147124182349,12.2,-9.96530205405724));
#167139=CARTESIAN_POINT('Ctrl Pts',(5.18413975897583,12.2,-9.96749804260233));
#167140=CARTESIAN_POINT('Ctrl Pts',(5.18680827612816,12.2,-9.96969403114742));
#167141=CARTESIAN_POINT('Ctrl Pts',(5.18948494291156,12.2,-9.97189145606147));
#167142=CARTESIAN_POINT('Ctrl Pts',(5.19216975123886,12.2,-9.9740902737996));
#167143=CARTESIAN_POINT('Ctrl Pts',(5.19574949600042,12.2,-9.97702203105007));
#167144=CARTESIAN_POINT('Ctrl Pts',(5.19934371189465,12.2,-9.97995626288546));
#167145=CARTESIAN_POINT('Ctrl Pts',(5.2029523790367,12.2,-9.98289286649009));
#167146=CARTESIAN_POINT('Ctrl Pts',(5.20565887914739,12.2,-9.98509531899352));
#167147=CARTESIAN_POINT('Ctrl Pts',(5.20837350631548,12.2,-9.98729910394679));
#167148=CARTESIAN_POINT('Ctrl Pts',(5.21109625200821,12.2,-9.98950417899167));
#167149=CARTESIAN_POINT('Ctrl Pts',(5.21381899770095,12.2,-9.99170925403654));
#167150=CARTESIAN_POINT('Ctrl Pts',(5.21654986121836,12.2,-9.99391561827304));
#167151=CARTESIAN_POINT('Ctrl Pts',(5.21928883340981,12.2,-9.99612322927606));
#167152=CARTESIAN_POINT('Ctrl Pts',(5.22202780560126,12.2,-9.99833084027908));
#167153=CARTESIAN_POINT('Ctrl Pts',(5.22477488589697,12.2,-10.0005396955924));
#167154=CARTESIAN_POINT('Ctrl Pts',(5.22753006522524,12.2,-10.0027497542891));
#167155=CARTESIAN_POINT('Ctrl Pts',(5.23028524455351,12.2,-10.0049598129857));
#167156=CARTESIAN_POINT('Ctrl Pts',(5.23304852239753,12.2,-10.0071710741482));
#167157=CARTESIAN_POINT('Ctrl Pts',(5.23581988862907,12.2,-10.009383494776));
#167158=CARTESIAN_POINT('Ctrl Pts',(5.23859125536407,12.2,-10.0115959158057));
#167159=CARTESIAN_POINT('Ctrl Pts',(5.24137071086803,12.2,-10.0138094972275));
#167160=CARTESIAN_POINT('Ctrl Pts',(5.24415824510758,12.2,-10.0160241942578));
#167161=CARTESIAN_POINT('Ctrl Pts',(5.24787495658297,12.2,-10.018977122961));
#167162=CARTESIAN_POINT('Ctrl Pts',(5.2516060308065,12.2,-10.0219320355112));
#167163=CARTESIAN_POINT('Ctrl Pts',(5.25535144294384,12.2,-10.0248888334916));
#167164=CARTESIAN_POINT('Ctrl Pts',(5.25816050217442,12.2,-10.0271064320776));
#167165=CARTESIAN_POINT('Ctrl Pts',(5.26097762743775,12.2,-10.0293250901802));
#167166=CARTESIAN_POINT('Ctrl Pts',(5.26380280766734,12.2,-10.0315447658078));
#167167=CARTESIAN_POINT('Ctrl Pts',(5.26662798841017,12.2,-10.0337644418386));
#167168=CARTESIAN_POINT('Ctrl Pts',(5.26946122435527,12.2,-10.035985135178));
#167169=CARTESIAN_POINT('Ctrl Pts',(5.27230250560263,12.2,-10.0382068042093));
#167170=CARTESIAN_POINT('Ctrl Pts',(5.27609087973883,12.2,-10.0411690289118));
#167171=CARTESIAN_POINT('Ctrl Pts',(5.27989355796704,12.2,-10.0441329885297));
#167172=CARTESIAN_POINT('Ctrl Pts',(5.28371051350562,12.2,-10.0470985826897));
#167173=CARTESIAN_POINT('Ctrl Pts',(5.28657323028958,12.2,-10.0493227784106));
#167174=CARTESIAN_POINT('Ctrl Pts',(5.28944397922486,12.2,-10.0515478941217));
#167175=CARTESIAN_POINT('Ctrl Pts',(5.2923227494529,12.2,-10.0537738882491));
#167176=CARTESIAN_POINT('Ctrl Pts',(5.29520151968094,12.2,-10.0559998823764));
#167177=CARTESIAN_POINT('Ctrl Pts',(5.2980883114251,12.2,-10.0582267551621));
#167178=CARTESIAN_POINT('Ctrl Pts',(5.3009831146105,12.2,-10.0604544647894));
#167179=CARTESIAN_POINT('Ctrl Pts',(5.30387791832178,12.2,-10.0626821748214));
#167180=CARTESIAN_POINT('Ctrl Pts',(5.30678073296032,12.2,-10.0649107217619));
#167181=CARTESIAN_POINT('Ctrl Pts',(5.30969154913446,12.2,-10.0671400657943));
#167182=CARTESIAN_POINT('Ctrl Pts',(5.31260236477979,12.2,-10.0693694094218));
#167183=CARTESIAN_POINT('Ctrl Pts',(5.31552118099209,12.2,-10.0715995491345));
#167184=CARTESIAN_POINT('Ctrl Pts',(5.31844798832456,12.2,-10.073830444415));
#167185=CARTESIAN_POINT('Ctrl Pts',(5.32137479565703,12.2,-10.0760613396954));
#167186=CARTESIAN_POINT('Ctrl Pts',(5.32430959359368,12.2,-10.0782929900911));
#167187=CARTESIAN_POINT('Ctrl Pts',(5.32725237132079,12.2,-10.08052535526));
#167188=CARTESIAN_POINT('Ctrl Pts',(5.33019514904789,12.2,-10.082757720429));
#167189=CARTESIAN_POINT('Ctrl Pts',(5.33314590727405,12.2,-10.0849908006478));
#167190=CARTESIAN_POINT('Ctrl Pts',(5.33610463504155,12.2,-10.087224556275));
#167191=CARTESIAN_POINT('Ctrl Pts',(5.34004960575655,12.2,-10.0902028973818));
#167192=CARTESIAN_POINT('Ctrl Pts',(5.34400874576488,12.2,-10.0931824386609));
#167193=CARTESIAN_POINT('Ctrl Pts',(5.34798202964953,12.2,-10.0961630852123));
#167194=CARTESIAN_POINT('Ctrl Pts',(5.35096199229234,12.2,-10.0983985699229));
#167195=CARTESIAN_POINT('Ctrl Pts',(5.35394991103786,12.2,-10.1006346766689));
#167196=CARTESIAN_POINT('Ctrl Pts',(5.35694577437126,12.2,-10.1028713629494));
#167197=CARTESIAN_POINT('Ctrl Pts',(5.35994163770465,12.2,-10.10510804923));
#167198=CARTESIAN_POINT('Ctrl Pts',(5.36294544513703,12.2,-10.1073453142585));
#167199=CARTESIAN_POINT('Ctrl Pts',(5.36595718781997,12.2,-10.1095831229689));
#167200=CARTESIAN_POINT('Ctrl Pts',(5.3689689305029,12.2,-10.1118209316793));
#167201=CARTESIAN_POINT('Ctrl Pts',(5.37198860734323,12.2,-10.114059283598));
#167202=CARTESIAN_POINT('Ctrl Pts',(5.37501620998322,12.2,-10.1162981422667));
#167203=CARTESIAN_POINT('Ctrl Pts',(5.3780438126232,12.2,-10.1185370009353));
#167204=CARTESIAN_POINT('Ctrl Pts',(5.38107934056289,12.2,-10.1207763669873));
#167205=CARTESIAN_POINT('Ctrl Pts',(5.38412278120162,12.2,-10.1230161955309));
#167206=CARTESIAN_POINT('Ctrl Pts',(5.38716622184035,12.2,-10.1252560240745));
#167207=CARTESIAN_POINT('Ctrl Pts',(5.39021757455064,12.2,-10.1274963140527));
#167208=CARTESIAN_POINT('Ctrl Pts',(5.39327682838308,12.2,-10.1297370198332));
#167209=CARTESIAN_POINT('Ctrl Pts',(5.39735583386349,12.2,-10.1327246278118));
#167210=CARTESIAN_POINT('Ctrl Pts',(5.40144888316411,12.2,-10.1357129685643));
#167211=CARTESIAN_POINT('Ctrl Pts',(5.40555595936562,12.2,-10.1387019911788));
#167212=CARTESIAN_POINT('Ctrl Pts',(5.40863626623696,12.2,-10.140943757936));
#167213=CARTESIAN_POINT('Ctrl Pts',(5.41172446743749,12.2,-10.1431859065926));
#167214=CARTESIAN_POINT('Ctrl Pts',(5.41482055299994,12.2,-10.145428447));
#167215=CARTESIAN_POINT('Origin',(-5.66257110645729E-14,15.2,-1.77635683940025E-14));
#167216=CARTESIAN_POINT('',(5.85257411399994,15.2,-8.56667970900002));
#167217=CARTESIAN_POINT('',(5.85257411399994,12.2,-8.56667970900002));
#167218=CARTESIAN_POINT('',(5.85257411399994,15.2,-8.56667970900002));
#167219=CARTESIAN_POINT('Origin',(-5.66257110645729E-14,12.2,-1.77635683940025E-14));
#167220=CARTESIAN_POINT('Origin',(-5.66257110645729E-14,15.2,-1.77635683940025E-14));
#167221=CARTESIAN_POINT('Origin',(-5.66257110645729E-14,15.2,-1.77635683940025E-14));
#167222=CARTESIAN_POINT('',(6.80355049614186,15.2,-9.27155330252674));
#167223=CARTESIAN_POINT('',(7.10901226899994,15.2,-9.03946594400002));
#167224=CARTESIAN_POINT('Origin',(-5.66257110645729E-14,15.2,-1.77635683940025E-14));
#167225=CARTESIAN_POINT('',(7.10901226899994,12.2,-9.03946594400002));
#167226=CARTESIAN_POINT('',(7.10901226899994,15.2,-9.03946594400002));
#167227=CARTESIAN_POINT('',(6.80355049614186,12.2,-9.27155330252674));
#167228=CARTESIAN_POINT('Origin',(-5.66257110645729E-14,12.2,-1.77635683940025E-14));
#167229=CARTESIAN_POINT('',(6.80355049599994,15.2,-9.27155330200002));
#167230=CARTESIAN_POINT('Ctrl Pts',(5.85257411399994,15.2,-8.56667970900002));
#167231=CARTESIAN_POINT('Ctrl Pts',(5.85257411399994,11.6,-8.56667970900002));
#167232=CARTESIAN_POINT('Ctrl Pts',(5.85268447799995,15.2,-8.56681469200002));
#167233=CARTESIAN_POINT('Ctrl Pts',(5.85268447799995,11.6,-8.56681469200002));
#167234=CARTESIAN_POINT('Ctrl Pts',(5.85290912899994,15.2,-8.56708931900002));
#167235=CARTESIAN_POINT('Ctrl Pts',(5.85290912899994,11.6,-8.56708931900002));
#167236=CARTESIAN_POINT('Ctrl Pts',(5.85324973299994,15.2,-8.56750527300001));
#167237=CARTESIAN_POINT('Ctrl Pts',(5.85324973299994,11.6,-8.56750527300001));
#167238=CARTESIAN_POINT('Ctrl Pts',(5.85370897499994,15.2,-8.56806526200002));
#167239=CARTESIAN_POINT('Ctrl Pts',(5.85370897499994,11.6,-8.56806526200002));
#167240=CARTESIAN_POINT('Ctrl Pts',(5.85429055399994,15.2,-8.56877298400001));
#167241=CARTESIAN_POINT('Ctrl Pts',(5.85429055399994,11.6,-8.56877298400001));
#167242=CARTESIAN_POINT('Ctrl Pts',(5.85488228099995,15.2,-8.56949158200001));
#167243=CARTESIAN_POINT('Ctrl Pts',(5.85488228099995,11.6,-8.56949158200001));
#167244=CARTESIAN_POINT('Ctrl Pts',(5.85548078499994,15.2,-8.57021692600001));
#167245=CARTESIAN_POINT('Ctrl Pts',(5.85548078499994,11.6,-8.57021692600001));
#167246=CARTESIAN_POINT('Ctrl Pts',(5.85608606099995,15.2,-8.57094898200002));
#167247=CARTESIAN_POINT('Ctrl Pts',(5.85608606099995,11.6,-8.57094898200002));
#167248=CARTESIAN_POINT('Ctrl Pts',(5.85669810699994,15.2,-8.57168771800002));
#167249=CARTESIAN_POINT('Ctrl Pts',(5.85669810699994,11.6,-8.57168771800002));
#167250=CARTESIAN_POINT('Ctrl Pts',(5.85731691799994,15.2,-8.57243310300002));
#167251=CARTESIAN_POINT('Ctrl Pts',(5.85731691799994,11.6,-8.57243310300002));
#167252=CARTESIAN_POINT('Ctrl Pts',(5.85794249299994,15.2,-8.57318510400002));
#167253=CARTESIAN_POINT('Ctrl Pts',(5.85794249299994,11.6,-8.57318510400002));
#167254=CARTESIAN_POINT('Ctrl Pts',(5.85857482799995,15.2,-8.57394368900002));
#167255=CARTESIAN_POINT('Ctrl Pts',(5.85857482799995,11.6,-8.57394368900002));
#167256=CARTESIAN_POINT('Ctrl Pts',(5.85921391899995,15.2,-8.57470882600002));
#167257=CARTESIAN_POINT('Ctrl Pts',(5.85921391899995,11.6,-8.57470882600002));
#167258=CARTESIAN_POINT('Ctrl Pts',(5.85985976499994,15.2,-8.57548048600002));
#167259=CARTESIAN_POINT('Ctrl Pts',(5.85985976499994,11.6,-8.57548048600002));
#167260=CARTESIAN_POINT('Ctrl Pts',(5.86051236099995,15.2,-8.57625863500001));
#167261=CARTESIAN_POINT('Ctrl Pts',(5.86051236099995,11.6,-8.57625863500001));
#167262=CARTESIAN_POINT('Ctrl Pts',(5.86117170399994,15.2,-8.57704324400002));
#167263=CARTESIAN_POINT('Ctrl Pts',(5.86117170399994,11.6,-8.57704324400002));
#167264=CARTESIAN_POINT('Ctrl Pts',(5.86183779199994,15.2,-8.57783428100002));
#167265=CARTESIAN_POINT('Ctrl Pts',(5.86183779199994,11.6,-8.57783428100002));
#167266=CARTESIAN_POINT('Ctrl Pts',(5.86251061899994,15.2,-8.57863171400002));
#167267=CARTESIAN_POINT('Ctrl Pts',(5.86251061899994,11.6,-8.57863171400002));
#167268=CARTESIAN_POINT('Ctrl Pts',(5.86319018499994,15.2,-8.57943551500002));
#167269=CARTESIAN_POINT('Ctrl Pts',(5.86319018499994,11.6,-8.57943551500002));
#167270=CARTESIAN_POINT('Ctrl Pts',(5.86387648599994,15.2,-8.58024565100001));
#167271=CARTESIAN_POINT('Ctrl Pts',(5.86387648599994,11.6,-8.58024565100001));
#167272=CARTESIAN_POINT('Ctrl Pts',(5.86456951799994,15.2,-8.58106209400002));
#167273=CARTESIAN_POINT('Ctrl Pts',(5.86456951799994,11.6,-8.58106209400002));
#167274=CARTESIAN_POINT('Ctrl Pts',(5.86526927899994,15.2,-8.58188481300001));
#167275=CARTESIAN_POINT('Ctrl Pts',(5.86526927899994,11.6,-8.58188481300001));
#167276=CARTESIAN_POINT('Ctrl Pts',(5.86597576599994,15.2,-8.58271377600002));
#167277=CARTESIAN_POINT('Ctrl Pts',(5.86597576599994,11.6,-8.58271377600002));
#167278=CARTESIAN_POINT('Ctrl Pts',(5.86668897299995,15.2,-8.58354895500002));
#167279=CARTESIAN_POINT('Ctrl Pts',(5.86668897299995,11.6,-8.58354895500002));
#167280=CARTESIAN_POINT('Ctrl Pts',(5.86740889999994,15.2,-8.58439031900001));
#167281=CARTESIAN_POINT('Ctrl Pts',(5.86740889999994,11.6,-8.58439031900001));
#167282=CARTESIAN_POINT('Ctrl Pts',(5.86813554199995,15.2,-8.58523784000001));
#167283=CARTESIAN_POINT('Ctrl Pts',(5.86813554199995,11.6,-8.58523784000001));
#167284=CARTESIAN_POINT('Ctrl Pts',(5.86886889699994,15.2,-8.58609148700002));
#167285=CARTESIAN_POINT('Ctrl Pts',(5.86886889699994,11.6,-8.58609148700002));
#167286=CARTESIAN_POINT('Ctrl Pts',(5.86960896099994,15.2,-8.58695123200001));
#167287=CARTESIAN_POINT('Ctrl Pts',(5.86960896099994,11.6,-8.58695123200001));
#167288=CARTESIAN_POINT('Ctrl Pts',(5.87035573299994,15.2,-8.58781704500002));
#167289=CARTESIAN_POINT('Ctrl Pts',(5.87035573299994,11.6,-8.58781704500002));
#167290=CARTESIAN_POINT('Ctrl Pts',(5.87110920599994,15.2,-8.58868889600001));
#167291=CARTESIAN_POINT('Ctrl Pts',(5.87110920599994,11.6,-8.58868889600001));
#167292=CARTESIAN_POINT('Ctrl Pts',(5.87186938099994,15.2,-8.58956675700002));
#167293=CARTESIAN_POINT('Ctrl Pts',(5.87186938099994,11.6,-8.58956675700002));
#167294=CARTESIAN_POINT('Ctrl Pts',(5.87263625099995,15.2,-8.59045059900001));
#167295=CARTESIAN_POINT('Ctrl Pts',(5.87263625099995,11.6,-8.59045059900001));
#167296=CARTESIAN_POINT('Ctrl Pts',(5.87340981499994,15.2,-8.59134039400002));
#167297=CARTESIAN_POINT('Ctrl Pts',(5.87340981499994,11.6,-8.59134039400002));
#167298=CARTESIAN_POINT('Ctrl Pts',(5.87419006999994,15.2,-8.59223611300001));
#167299=CARTESIAN_POINT('Ctrl Pts',(5.87419006999994,11.6,-8.59223611300001));
#167300=CARTESIAN_POINT('Ctrl Pts',(5.87497701299994,15.2,-8.59313772700002));
#167301=CARTESIAN_POINT('Ctrl Pts',(5.87497701299994,11.6,-8.59313772700002));
#167302=CARTESIAN_POINT('Ctrl Pts',(5.87577063899994,15.2,-8.59404520900002));
#167303=CARTESIAN_POINT('Ctrl Pts',(5.87577063899994,11.6,-8.59404520900002));
#167304=CARTESIAN_POINT('Ctrl Pts',(5.87657094599994,15.2,-8.59495852900002));
#167305=CARTESIAN_POINT('Ctrl Pts',(5.87657094599994,11.6,-8.59495852900002));
#167306=CARTESIAN_POINT('Ctrl Pts',(5.87737793199994,15.2,-8.59587766000002));
#167307=CARTESIAN_POINT('Ctrl Pts',(5.87737793199994,11.6,-8.59587766000002));
#167308=CARTESIAN_POINT('Ctrl Pts',(5.87819159199994,15.2,-8.59680257500001));
#167309=CARTESIAN_POINT('Ctrl Pts',(5.87819159199994,11.6,-8.59680257500001));
#167310=CARTESIAN_POINT('Ctrl Pts',(5.87901192399994,15.2,-8.59773324500001));
#167311=CARTESIAN_POINT('Ctrl Pts',(5.87901192399994,11.6,-8.59773324500001));
#167312=CARTESIAN_POINT('Ctrl Pts',(5.87983892499994,15.2,-8.59866964200002));
#167313=CARTESIAN_POINT('Ctrl Pts',(5.87983892499994,11.6,-8.59866964200002));
#167314=CARTESIAN_POINT('Ctrl Pts',(5.88067259099994,15.2,-8.59961174000002));
#167315=CARTESIAN_POINT('Ctrl Pts',(5.88067259099994,11.6,-8.59961174000002));
#167316=CARTESIAN_POINT('Ctrl Pts',(5.88151291899995,15.2,-8.60055951000002));
#167317=CARTESIAN_POINT('Ctrl Pts',(5.88151291899995,11.6,-8.60055951000002));
#167318=CARTESIAN_POINT('Ctrl Pts',(5.88235990599995,15.2,-8.60151292500002));
#167319=CARTESIAN_POINT('Ctrl Pts',(5.88235990599995,11.6,-8.60151292500002));
#167320=CARTESIAN_POINT('Ctrl Pts',(5.88321354999994,15.2,-8.60247195900002));
#167321=CARTESIAN_POINT('Ctrl Pts',(5.88321354999994,11.6,-8.60247195900002));
#167322=CARTESIAN_POINT('Ctrl Pts',(5.88407384499994,15.2,-8.60343658400001));
#167323=CARTESIAN_POINT('Ctrl Pts',(5.88407384499994,11.6,-8.60343658400001));
#167324=CARTESIAN_POINT('Ctrl Pts',(5.88494079099994,15.2,-8.60440677400002));
#167325=CARTESIAN_POINT('Ctrl Pts',(5.88494079099994,11.6,-8.60440677400002));
#167326=CARTESIAN_POINT('Ctrl Pts',(5.88581438299995,15.2,-8.60538250100002));
#167327=CARTESIAN_POINT('Ctrl Pts',(5.88581438299995,11.6,-8.60538250100002));
#167328=CARTESIAN_POINT('Ctrl Pts',(5.88669461899994,15.2,-8.60636373900002));
#167329=CARTESIAN_POINT('Ctrl Pts',(5.88669461899994,11.6,-8.60636373900002));
#167330=CARTESIAN_POINT('Ctrl Pts',(5.88758149499994,15.2,-8.60735046100002));
#167331=CARTESIAN_POINT('Ctrl Pts',(5.88758149499994,11.6,-8.60735046100002));
#167332=CARTESIAN_POINT('Ctrl Pts',(5.88847500799995,15.2,-8.60834264100001));
#167333=CARTESIAN_POINT('Ctrl Pts',(5.88847500799995,11.6,-8.60834264100001));
#167334=CARTESIAN_POINT('Ctrl Pts',(5.88937515499994,15.2,-8.60934025300002));
#167335=CARTESIAN_POINT('Ctrl Pts',(5.88937515499994,11.6,-8.60934025300002));
#167336=CARTESIAN_POINT('Ctrl Pts',(5.89028193299994,15.2,-8.61034327100001));
#167337=CARTESIAN_POINT('Ctrl Pts',(5.89028193299994,11.6,-8.61034327100001));
#167338=CARTESIAN_POINT('Ctrl Pts',(5.89119533899994,15.2,-8.61135166700001));
#167339=CARTESIAN_POINT('Ctrl Pts',(5.89119533899994,11.6,-8.61135166700001));
#167340=CARTESIAN_POINT('Ctrl Pts',(5.89211536799994,15.2,-8.61236541700002));
#167341=CARTESIAN_POINT('Ctrl Pts',(5.89211536799994,11.6,-8.61236541700002));
#167342=CARTESIAN_POINT('Ctrl Pts',(5.89304201999994,15.2,-8.61338449400002));
#167343=CARTESIAN_POINT('Ctrl Pts',(5.89304201999994,11.6,-8.61338449400002));
#167344=CARTESIAN_POINT('Ctrl Pts',(5.89397528899994,15.2,-8.61440887300001));
#167345=CARTESIAN_POINT('Ctrl Pts',(5.89397528899994,11.6,-8.61440887300001));
#167346=CARTESIAN_POINT('Ctrl Pts',(5.89491517399994,15.2,-8.61543852800001));
#167347=CARTESIAN_POINT('Ctrl Pts',(5.89491517399994,11.6,-8.61543852800001));
#167348=CARTESIAN_POINT('Ctrl Pts',(5.89586167099994,15.2,-8.61647343400002));
#167349=CARTESIAN_POINT('Ctrl Pts',(5.89586167099994,11.6,-8.61647343400002));
#167350=CARTESIAN_POINT('Ctrl Pts',(5.89681477699994,15.2,-8.61751356400001));
#167351=CARTESIAN_POINT('Ctrl Pts',(5.89681477699994,11.6,-8.61751356400001));
#167352=CARTESIAN_POINT('Ctrl Pts',(5.89777448799994,15.2,-8.61855889400001));
#167353=CARTESIAN_POINT('Ctrl Pts',(5.89777448799994,11.6,-8.61855889400001));
#167354=CARTESIAN_POINT('Ctrl Pts',(5.89874080199994,15.2,-8.61960939900002));
#167355=CARTESIAN_POINT('Ctrl Pts',(5.89874080199994,11.6,-8.61960939900002));
#167356=CARTESIAN_POINT('Ctrl Pts',(5.89971371499994,15.2,-8.62066505300002));
#167357=CARTESIAN_POINT('Ctrl Pts',(5.89971371499994,11.6,-8.62066505300002));
#167358=CARTESIAN_POINT('Ctrl Pts',(5.90069322499994,15.2,-8.62172583100002));
#167359=CARTESIAN_POINT('Ctrl Pts',(5.90069322499994,11.6,-8.62172583100002));
#167360=CARTESIAN_POINT('Ctrl Pts',(5.90167932799995,15.2,-8.62279170800001));
#167361=CARTESIAN_POINT('Ctrl Pts',(5.90167932799995,11.6,-8.62279170800001));
#167362=CARTESIAN_POINT('Ctrl Pts',(5.90267202099994,15.2,-8.62386266200001));
#167363=CARTESIAN_POINT('Ctrl Pts',(5.90267202099994,11.6,-8.62386266200001));
#167364=CARTESIAN_POINT('Ctrl Pts',(5.90367129999994,15.2,-8.62493866400002));
#167365=CARTESIAN_POINT('Ctrl Pts',(5.90367129999994,11.6,-8.62493866400002));
#167366=CARTESIAN_POINT('Ctrl Pts',(5.90467716299995,15.2,-8.62601969300002));
#167367=CARTESIAN_POINT('Ctrl Pts',(5.90467716299995,11.6,-8.62601969300002));
#167368=CARTESIAN_POINT('Ctrl Pts',(5.90568960799994,15.2,-8.62710572200001));
#167369=CARTESIAN_POINT('Ctrl Pts',(5.90568960799994,11.6,-8.62710572200001));
#167370=CARTESIAN_POINT('Ctrl Pts',(5.90670862899994,15.2,-8.62819672800001));
#167371=CARTESIAN_POINT('Ctrl Pts',(5.90670862899994,11.6,-8.62819672800001));
#167372=CARTESIAN_POINT('Ctrl Pts',(5.90773422399995,15.2,-8.62929268600002));
#167373=CARTESIAN_POINT('Ctrl Pts',(5.90773422399995,11.6,-8.62929268600002));
#167374=CARTESIAN_POINT('Ctrl Pts',(5.90876639199994,15.2,-8.63039357200002));
#167375=CARTESIAN_POINT('Ctrl Pts',(5.90876639199994,11.6,-8.63039357200002));
#167376=CARTESIAN_POINT('Ctrl Pts',(5.90980512599995,15.2,-8.63149936300001));
#167377=CARTESIAN_POINT('Ctrl Pts',(5.90980512599995,11.6,-8.63149936300001));
#167378=CARTESIAN_POINT('Ctrl Pts',(5.91085042599994,15.2,-8.63261003400002));
#167379=CARTESIAN_POINT('Ctrl Pts',(5.91085042599994,11.6,-8.63261003400002));
#167380=CARTESIAN_POINT('Ctrl Pts',(5.91190228799994,15.2,-8.63372556000002));
#167381=CARTESIAN_POINT('Ctrl Pts',(5.91190228799994,11.6,-8.63372556000002));
#167382=CARTESIAN_POINT('Ctrl Pts',(5.91296070699994,15.2,-8.63484591900002));
#167383=CARTESIAN_POINT('Ctrl Pts',(5.91296070699994,11.6,-8.63484591900002));
#167384=CARTESIAN_POINT('Ctrl Pts',(5.91402568199995,15.2,-8.63597108700001));
#167385=CARTESIAN_POINT('Ctrl Pts',(5.91402568199995,11.6,-8.63597108700001));
#167386=CARTESIAN_POINT('Ctrl Pts',(5.91509720999994,15.2,-8.63710104100001));
#167387=CARTESIAN_POINT('Ctrl Pts',(5.91509720999994,11.6,-8.63710104100001));
#167388=CARTESIAN_POINT('Ctrl Pts',(5.91617528699994,15.2,-8.63823575600002));
#167389=CARTESIAN_POINT('Ctrl Pts',(5.91617528699994,11.6,-8.63823575600002));
#167390=CARTESIAN_POINT('Ctrl Pts',(5.91725990899994,15.2,-8.63937520900001));
#167391=CARTESIAN_POINT('Ctrl Pts',(5.91725990899994,11.6,-8.63937520900001));
#167392=CARTESIAN_POINT('Ctrl Pts',(5.91835107499994,15.2,-8.64051937700001));
#167393=CARTESIAN_POINT('Ctrl Pts',(5.91835107499994,11.6,-8.64051937700001));
#167394=CARTESIAN_POINT('Ctrl Pts',(5.91944877999994,15.2,-8.64166823700002));
#167395=CARTESIAN_POINT('Ctrl Pts',(5.91944877999994,11.6,-8.64166823700002));
#167396=CARTESIAN_POINT('Ctrl Pts',(5.92055302199994,15.2,-8.64282176500001));
#167397=CARTESIAN_POINT('Ctrl Pts',(5.92055302199994,11.6,-8.64282176500001));
#167398=CARTESIAN_POINT('Ctrl Pts',(5.92166379799995,15.2,-8.64397994000001));
#167399=CARTESIAN_POINT('Ctrl Pts',(5.92166379799995,11.6,-8.64397994000001));
#167400=CARTESIAN_POINT('Ctrl Pts',(5.92278110299994,15.2,-8.64514273600001));
#167401=CARTESIAN_POINT('Ctrl Pts',(5.92278110299994,11.6,-8.64514273600001));
#167402=CARTESIAN_POINT('Ctrl Pts',(5.92390493499994,15.2,-8.64631013400002));
#167403=CARTESIAN_POINT('Ctrl Pts',(5.92390493499994,11.6,-8.64631013400002));
#167404=CARTESIAN_POINT('Ctrl Pts',(5.92503529199995,15.2,-8.64748210700002));
#167405=CARTESIAN_POINT('Ctrl Pts',(5.92503529199995,11.6,-8.64748210700002));
#167406=CARTESIAN_POINT('Ctrl Pts',(5.92617216899994,15.2,-8.64865863600001));
#167407=CARTESIAN_POINT('Ctrl Pts',(5.92617216899994,11.6,-8.64865863600001));
#167408=CARTESIAN_POINT('Ctrl Pts',(5.92731556399994,15.2,-8.64983969600001));
#167409=CARTESIAN_POINT('Ctrl Pts',(5.92731556399994,11.6,-8.64983969600001));
#167410=CARTESIAN_POINT('Ctrl Pts',(5.92846547399994,15.2,-8.65102526600002));
#167411=CARTESIAN_POINT('Ctrl Pts',(5.92846547399994,11.6,-8.65102526600002));
#167412=CARTESIAN_POINT('Ctrl Pts',(5.92962189399994,15.2,-8.65221532200002));
#167413=CARTESIAN_POINT('Ctrl Pts',(5.92962189399994,11.6,-8.65221532200002));
#167414=CARTESIAN_POINT('Ctrl Pts',(5.93078482299994,15.2,-8.65340984300002));
#167415=CARTESIAN_POINT('Ctrl Pts',(5.93078482299994,11.6,-8.65340984300002));
#167416=CARTESIAN_POINT('Ctrl Pts',(5.93195425599994,15.2,-8.65460880700001));
#167417=CARTESIAN_POINT('Ctrl Pts',(5.93195425599994,11.6,-8.65460880700001));
#167418=CARTESIAN_POINT('Ctrl Pts',(5.93313019299995,15.2,-8.65581219100001));
#167419=CARTESIAN_POINT('Ctrl Pts',(5.93313019299995,11.6,-8.65581219100001));
#167420=CARTESIAN_POINT('Ctrl Pts',(5.93431262699994,15.2,-8.65701997400001));
#167421=CARTESIAN_POINT('Ctrl Pts',(5.93431262699994,11.6,-8.65701997400001));
#167422=CARTESIAN_POINT('Ctrl Pts',(5.93550155699995,15.2,-8.65823213200001));
#167423=CARTESIAN_POINT('Ctrl Pts',(5.93550155699995,11.6,-8.65823213200001));
#167424=CARTESIAN_POINT('Ctrl Pts',(5.93669697899994,15.2,-8.65944864500002));
#167425=CARTESIAN_POINT('Ctrl Pts',(5.93669697899994,11.6,-8.65944864500002));
#167426=CARTESIAN_POINT('Ctrl Pts',(5.93789889099994,15.2,-8.66066949100002));
#167427=CARTESIAN_POINT('Ctrl Pts',(5.93789889099994,11.6,-8.66066949100002));
#167428=CARTESIAN_POINT('Ctrl Pts',(5.93910728799995,15.2,-8.66189464800001));
#167429=CARTESIAN_POINT('Ctrl Pts',(5.93910728799995,11.6,-8.66189464800001));
#167430=CARTESIAN_POINT('Ctrl Pts',(5.94032216899994,15.2,-8.66312409300001));
#167431=CARTESIAN_POINT('Ctrl Pts',(5.94032216899994,11.6,-8.66312409300001));
#167432=CARTESIAN_POINT('Ctrl Pts',(5.94154352899994,15.2,-8.66435780700002));
#167433=CARTESIAN_POINT('Ctrl Pts',(5.94154352899994,11.6,-8.66435780700002));
#167434=CARTESIAN_POINT('Ctrl Pts',(5.94277136499994,15.2,-8.66559576600002));
#167435=CARTESIAN_POINT('Ctrl Pts',(5.94277136499994,11.6,-8.66559576600002));
#167436=CARTESIAN_POINT('Ctrl Pts',(5.94400567599994,15.2,-8.66683795100002));
#167437=CARTESIAN_POINT('Ctrl Pts',(5.94400567599994,11.6,-8.66683795100002));
#167438=CARTESIAN_POINT('Ctrl Pts',(5.94524645699994,15.2,-8.66808434000001));
#167439=CARTESIAN_POINT('Ctrl Pts',(5.94524645699994,11.6,-8.66808434000001));
#167440=CARTESIAN_POINT('Ctrl Pts',(5.94649370399994,15.2,-8.66933491000001));
#167441=CARTESIAN_POINT('Ctrl Pts',(5.94649370399994,11.6,-8.66933491000001));
#167442=CARTESIAN_POINT('Ctrl Pts',(5.94774741599994,15.2,-8.67058964200002));
#167443=CARTESIAN_POINT('Ctrl Pts',(5.94774741599994,11.6,-8.67058964200002));
#167444=CARTESIAN_POINT('Ctrl Pts',(5.94900758799994,15.2,-8.67184851400001));
#167445=CARTESIAN_POINT('Ctrl Pts',(5.94900758799994,11.6,-8.67184851400001));
#167446=CARTESIAN_POINT('Ctrl Pts',(5.95027421799994,15.2,-8.67311150500001));
#167447=CARTESIAN_POINT('Ctrl Pts',(5.95027421799994,11.6,-8.67311150500001));
#167448=CARTESIAN_POINT('Ctrl Pts',(5.95154730199994,15.2,-8.67437859500002));
#167449=CARTESIAN_POINT('Ctrl Pts',(5.95154730199994,11.6,-8.67437859500002));
#167450=CARTESIAN_POINT('Ctrl Pts',(5.95282683699994,15.2,-8.67564976200002));
#167451=CARTESIAN_POINT('Ctrl Pts',(5.95282683699994,11.6,-8.67564976200002));
#167452=CARTESIAN_POINT('Ctrl Pts',(5.95411282099994,15.2,-8.67692498600002));
#167453=CARTESIAN_POINT('Ctrl Pts',(5.95411282099994,11.6,-8.67692498600002));
#167454=CARTESIAN_POINT('Ctrl Pts',(5.95540524899994,15.2,-8.67820424500002));
#167455=CARTESIAN_POINT('Ctrl Pts',(5.95540524899994,11.6,-8.67820424500002));
#167456=CARTESIAN_POINT('Ctrl Pts',(5.95670411999994,15.2,-8.67948752000002));
#167457=CARTESIAN_POINT('Ctrl Pts',(5.95670411999994,11.6,-8.67948752000002));
#167458=CARTESIAN_POINT('Ctrl Pts',(5.95800942899994,15.2,-8.68077479000002));
#167459=CARTESIAN_POINT('Ctrl Pts',(5.95800942899994,11.6,-8.68077479000002));
#167460=CARTESIAN_POINT('Ctrl Pts',(5.95932117299995,15.2,-8.68206603400001));
#167461=CARTESIAN_POINT('Ctrl Pts',(5.95932117299995,11.6,-8.68206603400001));
#167462=CARTESIAN_POINT('Ctrl Pts',(5.96063934899995,15.2,-8.68336123200002));
#167463=CARTESIAN_POINT('Ctrl Pts',(5.96063934899995,11.6,-8.68336123200002));
#167464=CARTESIAN_POINT('Ctrl Pts',(5.96196395499994,15.2,-8.68466036400001));
#167465=CARTESIAN_POINT('Ctrl Pts',(5.96196395499994,11.6,-8.68466036400001));
#167466=CARTESIAN_POINT('Ctrl Pts',(5.96329498499995,15.2,-8.68596340900002));
#167467=CARTESIAN_POINT('Ctrl Pts',(5.96329498499995,11.6,-8.68596340900002));
#167468=CARTESIAN_POINT('Ctrl Pts',(5.96463243999994,15.2,-8.68727034800001));
#167469=CARTESIAN_POINT('Ctrl Pts',(5.96463243999994,11.6,-8.68727034800001));
#167470=CARTESIAN_POINT('Ctrl Pts',(5.96597631299995,15.2,-8.68858116100002));
#167471=CARTESIAN_POINT('Ctrl Pts',(5.96597631299995,11.6,-8.68858116100002));
#167472=CARTESIAN_POINT('Ctrl Pts',(5.96732660299994,15.2,-8.68989582500001));
#167473=CARTESIAN_POINT('Ctrl Pts',(5.96732660299994,11.6,-8.68989582500001));
#167474=CARTESIAN_POINT('Ctrl Pts',(5.96868330599994,15.2,-8.69121432500001));
#167475=CARTESIAN_POINT('Ctrl Pts',(5.96868330599994,11.6,-8.69121432500001));
#167476=CARTESIAN_POINT('Ctrl Pts',(5.97004641899994,15.2,-8.69253663700002));
#167477=CARTESIAN_POINT('Ctrl Pts',(5.97004641899994,11.6,-8.69253663700002));
#167478=CARTESIAN_POINT('Ctrl Pts',(5.97141593799994,15.2,-8.69386274300001));
#167479=CARTESIAN_POINT('Ctrl Pts',(5.97141593799994,11.6,-8.69386274300001));
#167480=CARTESIAN_POINT('Ctrl Pts',(5.97279186099994,15.2,-8.69519262200001));
#167481=CARTESIAN_POINT('Ctrl Pts',(5.97279186099994,11.6,-8.69519262200001));
#167482=CARTESIAN_POINT('Ctrl Pts',(5.97417418499995,15.2,-8.69652625600001));
#167483=CARTESIAN_POINT('Ctrl Pts',(5.97417418499995,11.6,-8.69652625600001));
#167484=CARTESIAN_POINT('Ctrl Pts',(5.97556290599995,15.2,-8.69786362500001));
#167485=CARTESIAN_POINT('Ctrl Pts',(5.97556290599995,11.6,-8.69786362500001));
#167486=CARTESIAN_POINT('Ctrl Pts',(5.97695801999994,15.2,-8.69920470900002));
#167487=CARTESIAN_POINT('Ctrl Pts',(5.97695801999994,11.6,-8.69920470900002));
#167488=CARTESIAN_POINT('Ctrl Pts',(5.97835952599994,15.2,-8.70054948900002));
#167489=CARTESIAN_POINT('Ctrl Pts',(5.97835952599994,11.6,-8.70054948900002));
#167490=CARTESIAN_POINT('Ctrl Pts',(5.97976741899994,15.2,-8.70189794500002));
#167491=CARTESIAN_POINT('Ctrl Pts',(5.97976741899994,11.6,-8.70189794500002));
#167492=CARTESIAN_POINT('Ctrl Pts',(5.98118169699994,15.2,-8.70325005800002));
#167493=CARTESIAN_POINT('Ctrl Pts',(5.98118169699994,11.6,-8.70325005800002));
#167494=CARTESIAN_POINT('Ctrl Pts',(5.98260235599994,15.2,-8.70460581000001));
#167495=CARTESIAN_POINT('Ctrl Pts',(5.98260235599994,11.6,-8.70460581000001));
#167496=CARTESIAN_POINT('Ctrl Pts',(5.98402939199994,15.2,-8.70596518000001));
#167497=CARTESIAN_POINT('Ctrl Pts',(5.98402939199994,11.6,-8.70596518000001));
#167498=CARTESIAN_POINT('Ctrl Pts',(5.98546280499994,15.2,-8.70732814900002));
#167499=CARTESIAN_POINT('Ctrl Pts',(5.98546280499994,11.6,-8.70732814900002));
#167500=CARTESIAN_POINT('Ctrl Pts',(5.98690258799994,15.2,-8.70869469900001));
#167501=CARTESIAN_POINT('Ctrl Pts',(5.98690258799994,11.6,-8.70869469900001));
#167502=CARTESIAN_POINT('Ctrl Pts',(5.98834873999994,15.2,-8.71006481000002));
#167503=CARTESIAN_POINT('Ctrl Pts',(5.98834873999994,11.6,-8.71006481000002));
#167504=CARTESIAN_POINT('Ctrl Pts',(5.98980125799994,15.2,-8.71143846400001));
#167505=CARTESIAN_POINT('Ctrl Pts',(5.98980125799994,11.6,-8.71143846400001));
#167506=CARTESIAN_POINT('Ctrl Pts',(5.99126013699995,15.2,-8.71281564200002));
#167507=CARTESIAN_POINT('Ctrl Pts',(5.99126013699995,11.6,-8.71281564200002));
#167508=CARTESIAN_POINT('Ctrl Pts',(5.99272537499995,15.2,-8.71419632500002));
#167509=CARTESIAN_POINT('Ctrl Pts',(5.99272537499995,11.6,-8.71419632500002));
#167510=CARTESIAN_POINT('Ctrl Pts',(5.99419696899995,15.2,-8.71558049400001));
#167511=CARTESIAN_POINT('Ctrl Pts',(5.99419696899995,11.6,-8.71558049400001));
#167512=CARTESIAN_POINT('Ctrl Pts',(5.99567491499994,15.2,-8.71696813100002));
#167513=CARTESIAN_POINT('Ctrl Pts',(5.99567491499994,11.6,-8.71696813100002));
#167514=CARTESIAN_POINT('Ctrl Pts',(5.99715921199994,15.2,-8.71835921700002));
#167515=CARTESIAN_POINT('Ctrl Pts',(5.99715921199994,11.6,-8.71835921700002));
#167516=CARTESIAN_POINT('Ctrl Pts',(5.99864985299994,15.2,-8.71975373400002));
#167517=CARTESIAN_POINT('Ctrl Pts',(5.99864985299994,11.6,-8.71975373400002));
#167518=CARTESIAN_POINT('Ctrl Pts',(6.00014683699994,15.2,-8.72115166300001));
#167519=CARTESIAN_POINT('Ctrl Pts',(6.00014683699994,11.6,-8.72115166300001));
#167520=CARTESIAN_POINT('Ctrl Pts',(6.00165016199994,15.2,-8.72255298400002));
#167521=CARTESIAN_POINT('Ctrl Pts',(6.00165016199994,11.6,-8.72255298400002));
#167522=CARTESIAN_POINT('Ctrl Pts',(6.00315982299994,15.2,-8.72395768300001));
#167523=CARTESIAN_POINT('Ctrl Pts',(6.00315982299994,11.6,-8.72395768300001));
#167524=CARTESIAN_POINT('Ctrl Pts',(6.00467581699994,15.2,-8.72536573700001));
#167525=CARTESIAN_POINT('Ctrl Pts',(6.00467581699994,11.6,-8.72536573700001));
#167526=CARTESIAN_POINT('Ctrl Pts',(6.00619813999994,15.2,-8.72677713200002));
#167527=CARTESIAN_POINT('Ctrl Pts',(6.00619813999994,11.6,-8.72677713200002));
#167528=CARTESIAN_POINT('Ctrl Pts',(6.00772679099994,15.2,-8.72819184600001));
#167529=CARTESIAN_POINT('Ctrl Pts',(6.00772679099994,11.6,-8.72819184600001));
#167530=CARTESIAN_POINT('Ctrl Pts',(6.00926176599994,15.2,-8.72960986400001));
#167531=CARTESIAN_POINT('Ctrl Pts',(6.00926176599994,11.6,-8.72960986400001));
#167532=CARTESIAN_POINT('Ctrl Pts',(6.01080305999994,15.2,-8.73103116600002));
#167533=CARTESIAN_POINT('Ctrl Pts',(6.01080305999994,11.6,-8.73103116600002));
#167534=CARTESIAN_POINT('Ctrl Pts',(6.01235067299994,15.2,-8.73245573400002));
#167535=CARTESIAN_POINT('Ctrl Pts',(6.01235067299994,11.6,-8.73245573400002));
#167536=CARTESIAN_POINT('Ctrl Pts',(6.01390459799994,15.2,-8.73388355100002));
#167537=CARTESIAN_POINT('Ctrl Pts',(6.01390459799994,11.6,-8.73388355100002));
#167538=CARTESIAN_POINT('Ctrl Pts',(6.01546483399994,15.2,-8.73531460000001));
#167539=CARTESIAN_POINT('Ctrl Pts',(6.01546483399994,11.6,-8.73531460000001));
#167540=CARTESIAN_POINT('Ctrl Pts',(6.01703137899994,15.2,-8.73674886200002));
#167541=CARTESIAN_POINT('Ctrl Pts',(6.01703137899994,11.6,-8.73674886200002));
#167542=CARTESIAN_POINT('Ctrl Pts',(6.01860422799994,15.2,-8.73818631900001));
#167543=CARTESIAN_POINT('Ctrl Pts',(6.01860422799994,11.6,-8.73818631900001));
#167544=CARTESIAN_POINT('Ctrl Pts',(6.02018337599994,15.2,-8.73962695300002));
#167545=CARTESIAN_POINT('Ctrl Pts',(6.02018337599994,11.6,-8.73962695300002));
#167546=CARTESIAN_POINT('Ctrl Pts',(6.02176882399994,15.2,-8.74107074900002));
#167547=CARTESIAN_POINT('Ctrl Pts',(6.02176882399994,11.6,-8.74107074900002));
#167548=CARTESIAN_POINT('Ctrl Pts',(6.02336056599994,15.2,-8.74251768600002));
#167549=CARTESIAN_POINT('Ctrl Pts',(6.02336056599994,11.6,-8.74251768600002));
#167550=CARTESIAN_POINT('Ctrl Pts',(6.02495859899994,15.2,-8.74396774900001));
#167551=CARTESIAN_POINT('Ctrl Pts',(6.02495859899994,11.6,-8.74396774900001));
#167552=CARTESIAN_POINT('Ctrl Pts',(6.02656291999994,15.2,-8.74542091800001));
#167553=CARTESIAN_POINT('Ctrl Pts',(6.02656291999994,11.6,-8.74542091800001));
#167554=CARTESIAN_POINT('Ctrl Pts',(6.02817352699994,15.2,-8.74687718000001));
#167555=CARTESIAN_POINT('Ctrl Pts',(6.02817352699994,11.6,-8.74687718000001));
#167556=CARTESIAN_POINT('Ctrl Pts',(6.02979041499994,15.2,-8.74833651300002));
#167557=CARTESIAN_POINT('Ctrl Pts',(6.02979041499994,11.6,-8.74833651300002));
#167558=CARTESIAN_POINT('Ctrl Pts',(6.03141358199994,15.2,-8.74979890200001));
#167559=CARTESIAN_POINT('Ctrl Pts',(6.03141358199994,11.6,-8.74979890200001));
#167560=CARTESIAN_POINT('Ctrl Pts',(6.03304302299994,15.2,-8.75126433100002));
#167561=CARTESIAN_POINT('Ctrl Pts',(6.03304302299994,11.6,-8.75126433100002));
#167562=CARTESIAN_POINT('Ctrl Pts',(6.03467873699994,15.2,-8.75273277900002));
#167563=CARTESIAN_POINT('Ctrl Pts',(6.03467873699994,11.6,-8.75273277900002));
#167564=CARTESIAN_POINT('Ctrl Pts',(6.03632071899994,15.2,-8.75420423200002));
#167565=CARTESIAN_POINT('Ctrl Pts',(6.03632071899994,11.6,-8.75420423200002));
#167566=CARTESIAN_POINT('Ctrl Pts',(6.03796896799994,15.2,-8.75567867300001));
#167567=CARTESIAN_POINT('Ctrl Pts',(6.03796896799994,11.6,-8.75567867300001));
#167568=CARTESIAN_POINT('Ctrl Pts',(6.03962347799994,15.2,-8.75715608400002));
#167569=CARTESIAN_POINT('Ctrl Pts',(6.03962347799994,11.6,-8.75715608400002));
#167570=CARTESIAN_POINT('Ctrl Pts',(6.04128424699995,15.2,-8.75863644800001));
#167571=CARTESIAN_POINT('Ctrl Pts',(6.04128424699995,11.6,-8.75863644800001));
#167572=CARTESIAN_POINT('Ctrl Pts',(6.04295127299994,15.2,-8.76011974800001));
#167573=CARTESIAN_POINT('Ctrl Pts',(6.04295127299994,11.6,-8.76011974800001));
#167574=CARTESIAN_POINT('Ctrl Pts',(6.04462455099994,15.2,-8.76160596800002));
#167575=CARTESIAN_POINT('Ctrl Pts',(6.04462455099994,11.6,-8.76160596800002));
#167576=CARTESIAN_POINT('Ctrl Pts',(6.04630407799994,15.2,-8.76309509100002));
#167577=CARTESIAN_POINT('Ctrl Pts',(6.04630407799994,11.6,-8.76309509100002));
#167578=CARTESIAN_POINT('Ctrl Pts',(6.04798985099994,15.2,-8.76458710000002));
#167579=CARTESIAN_POINT('Ctrl Pts',(6.04798985099994,11.6,-8.76458710000002));
#167580=CARTESIAN_POINT('Ctrl Pts',(6.04968186699994,15.2,-8.76608197700002));
#167581=CARTESIAN_POINT('Ctrl Pts',(6.04968186699994,11.6,-8.76608197700002));
#167582=CARTESIAN_POINT('Ctrl Pts',(6.05138012199994,15.2,-8.76757970900002));
#167583=CARTESIAN_POINT('Ctrl Pts',(6.05138012199994,11.6,-8.76757970900002));
#167584=CARTESIAN_POINT('Ctrl Pts',(6.05308461499994,15.2,-8.76908027600001));
#167585=CARTESIAN_POINT('Ctrl Pts',(6.05308461499994,11.6,-8.76908027600001));
#167586=CARTESIAN_POINT('Ctrl Pts',(6.05479533999994,15.2,-8.77058366200002));
#167587=CARTESIAN_POINT('Ctrl Pts',(6.05479533999994,11.6,-8.77058366200002));
#167588=CARTESIAN_POINT('Ctrl Pts',(6.05651229499995,15.2,-8.77208985200001));
#167589=CARTESIAN_POINT('Ctrl Pts',(6.05651229499995,11.6,-8.77208985200001));
#167590=CARTESIAN_POINT('Ctrl Pts',(6.05823547599995,15.2,-8.77359882900001));
#167591=CARTESIAN_POINT('Ctrl Pts',(6.05823547599995,11.6,-8.77359882900001));
#167592=CARTESIAN_POINT('Ctrl Pts',(6.05996488099994,15.2,-8.77511057700002));
#167593=CARTESIAN_POINT('Ctrl Pts',(6.05996488099994,11.6,-8.77511057700002));
#167594=CARTESIAN_POINT('Ctrl Pts',(6.06170050599994,15.2,-8.77662507800002));
#167595=CARTESIAN_POINT('Ctrl Pts',(6.06170050599994,11.6,-8.77662507800002));
#167596=CARTESIAN_POINT('Ctrl Pts',(6.06344234899994,15.2,-8.77814231800001));
#167597=CARTESIAN_POINT('Ctrl Pts',(6.06344234899994,11.6,-8.77814231800001));
#167598=CARTESIAN_POINT('Ctrl Pts',(6.06519040399994,15.2,-8.77966227900002));
#167599=CARTESIAN_POINT('Ctrl Pts',(6.06519040399994,11.6,-8.77966227900002));
#167600=CARTESIAN_POINT('Ctrl Pts',(6.06694466899994,15.2,-8.78118494600002));
#167601=CARTESIAN_POINT('Ctrl Pts',(6.06694466899994,11.6,-8.78118494600002));
#167602=CARTESIAN_POINT('Ctrl Pts',(6.06870514199994,15.2,-8.78271030200001));
#167603=CARTESIAN_POINT('Ctrl Pts',(6.06870514199994,11.6,-8.78271030200001));
#167604=CARTESIAN_POINT('Ctrl Pts',(6.07047181899994,15.2,-8.78423833100002));
#167605=CARTESIAN_POINT('Ctrl Pts',(6.07047181899994,11.6,-8.78423833100002));
#167606=CARTESIAN_POINT('Ctrl Pts',(6.07224469599994,15.2,-8.78576901800002));
#167607=CARTESIAN_POINT('Ctrl Pts',(6.07224469599994,11.6,-8.78576901800002));
#167608=CARTESIAN_POINT('Ctrl Pts',(6.07402377099994,15.2,-8.78730234600001));
#167609=CARTESIAN_POINT('Ctrl Pts',(6.07402377099994,11.6,-8.78730234600001));
#167610=CARTESIAN_POINT('Ctrl Pts',(6.07580903899994,15.2,-8.78883830000002));
#167611=CARTESIAN_POINT('Ctrl Pts',(6.07580903899994,11.6,-8.78883830000002));
#167612=CARTESIAN_POINT('Ctrl Pts',(6.07760049799994,15.2,-8.79037686400002));
#167613=CARTESIAN_POINT('Ctrl Pts',(6.07760049799994,11.6,-8.79037686400002));
#167614=CARTESIAN_POINT('Ctrl Pts',(6.07939814499994,15.2,-8.79191802100001));
#167615=CARTESIAN_POINT('Ctrl Pts',(6.07939814499994,11.6,-8.79191802100001));
#167616=CARTESIAN_POINT('Ctrl Pts',(6.08120197499994,15.2,-8.79346175700002));
#167617=CARTESIAN_POINT('Ctrl Pts',(6.08120197499994,11.6,-8.79346175700002));
#167618=CARTESIAN_POINT('Ctrl Pts',(6.08301198699994,15.2,-8.79500805500001));
#167619=CARTESIAN_POINT('Ctrl Pts',(6.08301198699994,11.6,-8.79500805500001));
#167620=CARTESIAN_POINT('Ctrl Pts',(6.08482817699994,15.2,-8.79655689900002));
#167621=CARTESIAN_POINT('Ctrl Pts',(6.08482817699994,11.6,-8.79655689900002));
#167622=CARTESIAN_POINT('Ctrl Pts',(6.08665053999994,15.2,-8.79810827400001));
#167623=CARTESIAN_POINT('Ctrl Pts',(6.08665053999994,11.6,-8.79810827400001));
#167624=CARTESIAN_POINT('Ctrl Pts',(6.08847907499994,15.2,-8.79966216600002));
#167625=CARTESIAN_POINT('Ctrl Pts',(6.08847907499994,11.6,-8.79966216600002));
#167626=CARTESIAN_POINT('Ctrl Pts',(6.09031377799995,15.2,-8.80121855700001));
#167627=CARTESIAN_POINT('Ctrl Pts',(6.09031377799995,11.6,-8.80121855700001));
#167628=CARTESIAN_POINT('Ctrl Pts',(6.09215464499994,15.2,-8.80277743400002));
#167629=CARTESIAN_POINT('Ctrl Pts',(6.09215464499994,11.6,-8.80277743400002));
#167630=CARTESIAN_POINT('Ctrl Pts',(6.09400167399994,15.2,-8.80433877800002));
#167631=CARTESIAN_POINT('Ctrl Pts',(6.09400167399994,11.6,-8.80433877800002));
#167632=CARTESIAN_POINT('Ctrl Pts',(6.09585485999994,15.2,-8.80590257700002));
#167633=CARTESIAN_POINT('Ctrl Pts',(6.09585485999994,11.6,-8.80590257700002));
#167634=CARTESIAN_POINT('Ctrl Pts',(6.09771420199994,15.2,-8.80746881400002));
#167635=CARTESIAN_POINT('Ctrl Pts',(6.09771420199994,11.6,-8.80746881400002));
#167636=CARTESIAN_POINT('Ctrl Pts',(6.09957969399994,15.2,-8.80903747400002));
#167637=CARTESIAN_POINT('Ctrl Pts',(6.09957969399994,11.6,-8.80903747400002));
#167638=CARTESIAN_POINT('Ctrl Pts',(6.10145133499994,15.2,-8.81060854200001));
#167639=CARTESIAN_POINT('Ctrl Pts',(6.10145133499994,11.6,-8.81060854200001));
#167640=CARTESIAN_POINT('Ctrl Pts',(6.10332912099994,15.2,-8.81218200200001));
#167641=CARTESIAN_POINT('Ctrl Pts',(6.10332912099994,11.6,-8.81218200200001));
#167642=CARTESIAN_POINT('Ctrl Pts',(6.10521304799994,15.2,-8.81375784000002));
#167643=CARTESIAN_POINT('Ctrl Pts',(6.10521304799994,11.6,-8.81375784000002));
#167644=CARTESIAN_POINT('Ctrl Pts',(6.10710311299994,15.2,-8.81533604100002));
#167645=CARTESIAN_POINT('Ctrl Pts',(6.10710311299994,11.6,-8.81533604100002));
#167646=CARTESIAN_POINT('Ctrl Pts',(6.10899931399994,15.2,-8.81691658800002));
#167647=CARTESIAN_POINT('Ctrl Pts',(6.10899931399994,11.6,-8.81691658800002));
#167648=CARTESIAN_POINT('Ctrl Pts',(6.11090164599994,15.2,-8.81849946800001));
#167649=CARTESIAN_POINT('Ctrl Pts',(6.11090164599994,11.6,-8.81849946800001));
#167650=CARTESIAN_POINT('Ctrl Pts',(6.11281010699994,15.2,-8.82008466500002));
#167651=CARTESIAN_POINT('Ctrl Pts',(6.11281010699994,11.6,-8.82008466500002));
#167652=CARTESIAN_POINT('Ctrl Pts',(6.11472469299994,15.2,-8.82167216400001));
#167653=CARTESIAN_POINT('Ctrl Pts',(6.11472469299994,11.6,-8.82167216400001));
#167654=CARTESIAN_POINT('Ctrl Pts',(6.11664539999994,15.2,-8.82326195200001));
#167655=CARTESIAN_POINT('Ctrl Pts',(6.11664539999994,11.6,-8.82326195200001));
#167656=CARTESIAN_POINT('Ctrl Pts',(6.11857222599994,15.2,-8.82485401100002));
#167657=CARTESIAN_POINT('Ctrl Pts',(6.11857222599994,11.6,-8.82485401100002));
#167658=CARTESIAN_POINT('Ctrl Pts',(6.12050516699994,15.2,-8.82644832800001));
#167659=CARTESIAN_POINT('Ctrl Pts',(6.12050516699994,11.6,-8.82644832800001));
#167660=CARTESIAN_POINT('Ctrl Pts',(6.12244422199994,15.2,-8.82804488900002));
#167661=CARTESIAN_POINT('Ctrl Pts',(6.12244422199994,11.6,-8.82804488900002));
#167662=CARTESIAN_POINT('Ctrl Pts',(6.12438938299994,15.2,-8.82964367800002));
#167663=CARTESIAN_POINT('Ctrl Pts',(6.12438938299994,11.6,-8.82964367800002));
#167664=CARTESIAN_POINT('Ctrl Pts',(6.12634064999994,15.2,-8.83124468000002));
#167665=CARTESIAN_POINT('Ctrl Pts',(6.12634064999994,11.6,-8.83124468000002));
#167666=CARTESIAN_POINT('Ctrl Pts',(6.12829801999994,15.2,-8.83284788100001));
#167667=CARTESIAN_POINT('Ctrl Pts',(6.12829801999994,11.6,-8.83284788100001));
#167668=CARTESIAN_POINT('Ctrl Pts',(6.13026148799994,15.2,-8.83445326700001));
#167669=CARTESIAN_POINT('Ctrl Pts',(6.13026148799994,11.6,-8.83445326700001));
#167670=CARTESIAN_POINT('Ctrl Pts',(6.13223105199994,15.2,-8.83606082300001));
#167671=CARTESIAN_POINT('Ctrl Pts',(6.13223105199994,11.6,-8.83606082300001));
#167672=CARTESIAN_POINT('Ctrl Pts',(6.13420670699994,15.2,-8.83767053400002));
#167673=CARTESIAN_POINT('Ctrl Pts',(6.13420670699994,11.6,-8.83767053400002));
#167674=CARTESIAN_POINT('Ctrl Pts',(6.13618845099994,15.2,-8.83928238600001));
#167675=CARTESIAN_POINT('Ctrl Pts',(6.13618845099994,11.6,-8.83928238600001));
#167676=CARTESIAN_POINT('Ctrl Pts',(6.13817627999994,15.2,-8.84089636400001));
#167677=CARTESIAN_POINT('Ctrl Pts',(6.13817627999994,11.6,-8.84089636400001));
#167678=CARTESIAN_POINT('Ctrl Pts',(6.14017019199994,15.2,-8.84251245500002));
#167679=CARTESIAN_POINT('Ctrl Pts',(6.14017019199994,11.6,-8.84251245500002));
#167680=CARTESIAN_POINT('Ctrl Pts',(6.14217018299994,15.2,-8.84413064300002));
#167681=CARTESIAN_POINT('Ctrl Pts',(6.14217018299994,11.6,-8.84413064300002));
#167682=CARTESIAN_POINT('Ctrl Pts',(6.14417624999994,15.2,-8.84575091500002));
#167683=CARTESIAN_POINT('Ctrl Pts',(6.14417624999994,11.6,-8.84575091500002));
#167684=CARTESIAN_POINT('Ctrl Pts',(6.14618838899994,15.2,-8.84737325500002));
#167685=CARTESIAN_POINT('Ctrl Pts',(6.14618838899994,11.6,-8.84737325500002));
#167686=CARTESIAN_POINT('Ctrl Pts',(6.14820659699994,15.2,-8.84899765100002));
#167687=CARTESIAN_POINT('Ctrl Pts',(6.14820659699994,11.6,-8.84899765100002));
#167688=CARTESIAN_POINT('Ctrl Pts',(6.15023086899994,15.2,-8.85062408700002));
#167689=CARTESIAN_POINT('Ctrl Pts',(6.15023086899994,11.6,-8.85062408700002));
#167690=CARTESIAN_POINT('Ctrl Pts',(6.15226120499995,15.2,-8.85225255100002));
#167691=CARTESIAN_POINT('Ctrl Pts',(6.15226120499995,11.6,-8.85225255100002));
#167692=CARTESIAN_POINT('Ctrl Pts',(6.15429759899994,15.2,-8.85388302700001));
#167693=CARTESIAN_POINT('Ctrl Pts',(6.15429759899994,11.6,-8.85388302700001));
#167694=CARTESIAN_POINT('Ctrl Pts',(6.15634004999994,15.2,-8.85551550100002));
#167695=CARTESIAN_POINT('Ctrl Pts',(6.15634004999994,11.6,-8.85551550100002));
#167696=CARTESIAN_POINT('Ctrl Pts',(6.15838855099994,15.2,-8.85714995900001));
#167697=CARTESIAN_POINT('Ctrl Pts',(6.15838855099994,11.6,-8.85714995900001));
#167698=CARTESIAN_POINT('Ctrl Pts',(6.16044310199994,15.2,-8.85878638800002));
#167699=CARTESIAN_POINT('Ctrl Pts',(6.16044310199994,11.6,-8.85878638800002));
#167700=CARTESIAN_POINT('Ctrl Pts',(6.16250369999994,15.2,-8.86042477400002));
#167701=CARTESIAN_POINT('Ctrl Pts',(6.16250369999994,11.6,-8.86042477400002));
#167702=CARTESIAN_POINT('Ctrl Pts',(6.16457033899994,15.2,-8.86206510100001));
#167703=CARTESIAN_POINT('Ctrl Pts',(6.16457033899994,11.6,-8.86206510100001));
#167704=CARTESIAN_POINT('Ctrl Pts',(6.16664301799994,15.2,-8.86370735900002));
#167705=CARTESIAN_POINT('Ctrl Pts',(6.16664301799994,11.6,-8.86370735900002));
#167706=CARTESIAN_POINT('Ctrl Pts',(6.16872173199994,15.2,-8.86535153000001));
#167707=CARTESIAN_POINT('Ctrl Pts',(6.16872173199994,11.6,-8.86535153000001));
#167708=CARTESIAN_POINT('Ctrl Pts',(6.17080647799994,15.2,-8.86699760300001));
#167709=CARTESIAN_POINT('Ctrl Pts',(6.17080647799994,11.6,-8.86699760300001));
#167710=CARTESIAN_POINT('Ctrl Pts',(6.17289725299995,15.2,-8.86864556300001));
#167711=CARTESIAN_POINT('Ctrl Pts',(6.17289725299995,11.6,-8.86864556300001));
#167712=CARTESIAN_POINT('Ctrl Pts',(6.17499405399994,15.2,-8.87029539700002));
#167713=CARTESIAN_POINT('Ctrl Pts',(6.17499405399994,11.6,-8.87029539700002));
#167714=CARTESIAN_POINT('Ctrl Pts',(6.17709687799994,15.2,-8.87194709200001));
#167715=CARTESIAN_POINT('Ctrl Pts',(6.17709687799994,11.6,-8.87194709200001));
#167716=CARTESIAN_POINT('Ctrl Pts',(6.17920571999994,15.2,-8.87360063200001));
#167717=CARTESIAN_POINT('Ctrl Pts',(6.17920571999994,11.6,-8.87360063200001));
#167718=CARTESIAN_POINT('Ctrl Pts',(6.18132057899994,15.2,-8.87525600500001));
#167719=CARTESIAN_POINT('Ctrl Pts',(6.18132057899994,11.6,-8.87525600500001));
#167720=CARTESIAN_POINT('Ctrl Pts',(6.18344144899994,15.2,-8.87691319600002));
#167721=CARTESIAN_POINT('Ctrl Pts',(6.18344144899994,11.6,-8.87691319600002));
#167722=CARTESIAN_POINT('Ctrl Pts',(6.18556832799994,15.2,-8.87857219500002));
#167723=CARTESIAN_POINT('Ctrl Pts',(6.18556832799994,11.6,-8.87857219500002));
#167724=CARTESIAN_POINT('Ctrl Pts',(6.18770121399994,15.2,-8.88023298500002));
#167725=CARTESIAN_POINT('Ctrl Pts',(6.18770121399994,11.6,-8.88023298500002));
#167726=CARTESIAN_POINT('Ctrl Pts',(6.18984009999994,15.2,-8.88189555400002));
#167727=CARTESIAN_POINT('Ctrl Pts',(6.18984009999994,11.6,-8.88189555400002));
#167728=CARTESIAN_POINT('Ctrl Pts',(6.19198498599994,15.2,-8.88355988700001));
#167729=CARTESIAN_POINT('Ctrl Pts',(6.19198498599994,11.6,-8.88355988700001));
#167730=CARTESIAN_POINT('Ctrl Pts',(6.19413586799994,15.2,-8.88522597300001));
#167731=CARTESIAN_POINT('Ctrl Pts',(6.19413586799994,11.6,-8.88522597300001));
#167732=CARTESIAN_POINT('Ctrl Pts',(6.19629274299994,15.2,-8.88689379800002));
#167733=CARTESIAN_POINT('Ctrl Pts',(6.19629274299994,11.6,-8.88689379800002));
#167734=CARTESIAN_POINT('Ctrl Pts',(6.19845560599994,15.2,-8.88856334700002));
#167735=CARTESIAN_POINT('Ctrl Pts',(6.19845560599994,11.6,-8.88856334700002));
#167736=CARTESIAN_POINT('Ctrl Pts',(6.20062445399994,15.2,-8.89023460900002));
#167737=CARTESIAN_POINT('Ctrl Pts',(6.20062445399994,11.6,-8.89023460900002));
#167738=CARTESIAN_POINT('Ctrl Pts',(6.20279928499994,15.2,-8.89190757000001));
#167739=CARTESIAN_POINT('Ctrl Pts',(6.20279928499994,11.6,-8.89190757000001));
#167740=CARTESIAN_POINT('Ctrl Pts',(6.20498009499994,15.2,-8.89358221500002));
#167741=CARTESIAN_POINT('Ctrl Pts',(6.20498009499994,11.6,-8.89358221500002));
#167742=CARTESIAN_POINT('Ctrl Pts',(6.20716688099994,15.2,-8.89525853400002));
#167743=CARTESIAN_POINT('Ctrl Pts',(6.20716688099994,11.6,-8.89525853400002));
#167744=CARTESIAN_POINT('Ctrl Pts',(6.20935963799995,15.2,-8.89693651100002));
#167745=CARTESIAN_POINT('Ctrl Pts',(6.20935963799995,11.6,-8.89693651100002));
#167746=CARTESIAN_POINT('Ctrl Pts',(6.21155836399994,15.2,-8.89861613500001));
#167747=CARTESIAN_POINT('Ctrl Pts',(6.21155836399994,11.6,-8.89861613500001));
#167748=CARTESIAN_POINT('Ctrl Pts',(6.21376305499994,15.2,-8.90029739200001));
#167749=CARTESIAN_POINT('Ctrl Pts',(6.21376305499994,11.6,-8.90029739200001));
#167750=CARTESIAN_POINT('Ctrl Pts',(6.21597370899994,15.2,-8.90198026900002));
#167751=CARTESIAN_POINT('Ctrl Pts',(6.21597370899994,11.6,-8.90198026900002));
#167752=CARTESIAN_POINT('Ctrl Pts',(6.21819032199994,15.2,-8.90366475300001));
#167753=CARTESIAN_POINT('Ctrl Pts',(6.21819032199994,11.6,-8.90366475300001));
#167754=CARTESIAN_POINT('Ctrl Pts',(6.22041288899994,15.2,-8.90535083100002));
#167755=CARTESIAN_POINT('Ctrl Pts',(6.22041288899994,11.6,-8.90535083100002));
#167756=CARTESIAN_POINT('Ctrl Pts',(6.22264140799994,15.2,-8.90703849100002));
#167757=CARTESIAN_POINT('Ctrl Pts',(6.22264140799994,11.6,-8.90703849100002));
#167758=CARTESIAN_POINT('Ctrl Pts',(6.22487587699994,15.2,-8.90872771900002));
#167759=CARTESIAN_POINT('Ctrl Pts',(6.22487587699994,11.6,-8.90872771900002));
#167760=CARTESIAN_POINT('Ctrl Pts',(6.22711629099994,15.2,-8.91041850200001));
#167761=CARTESIAN_POINT('Ctrl Pts',(6.22711629099994,11.6,-8.91041850200001));
#167762=CARTESIAN_POINT('Ctrl Pts',(6.22936264599994,15.2,-8.91211082700002));
#167763=CARTESIAN_POINT('Ctrl Pts',(6.22936264599994,11.6,-8.91211082700002));
#167764=CARTESIAN_POINT('Ctrl Pts',(6.23161493899994,15.2,-8.91380468300002));
#167765=CARTESIAN_POINT('Ctrl Pts',(6.23161493899994,11.6,-8.91380468300002));
#167766=CARTESIAN_POINT('Ctrl Pts',(6.23387316899994,15.2,-8.91550005600001));
#167767=CARTESIAN_POINT('Ctrl Pts',(6.23387316899994,11.6,-8.91550005600001));
#167768=CARTESIAN_POINT('Ctrl Pts',(6.23613732999994,15.2,-8.91719693300002));
#167769=CARTESIAN_POINT('Ctrl Pts',(6.23613732999994,11.6,-8.91719693300002));
#167770=CARTESIAN_POINT('Ctrl Pts',(6.23840741799994,15.2,-8.91889530200002));
#167771=CARTESIAN_POINT('Ctrl Pts',(6.23840741799994,11.6,-8.91889530200002));
#167772=CARTESIAN_POINT('Ctrl Pts',(6.24068343299994,15.2,-8.92059515000001));
#167773=CARTESIAN_POINT('Ctrl Pts',(6.24068343299994,11.6,-8.92059515000001));
#167774=CARTESIAN_POINT('Ctrl Pts',(6.24296536899994,15.2,-8.92229646500001));
#167775=CARTESIAN_POINT('Ctrl Pts',(6.24296536899994,11.6,-8.92229646500001));
#167776=CARTESIAN_POINT('Ctrl Pts',(6.24525322299994,15.2,-8.92399923300001));
#167777=CARTESIAN_POINT('Ctrl Pts',(6.24525322299994,11.6,-8.92399923300001));
#167778=CARTESIAN_POINT('Ctrl Pts',(6.24754699199994,15.2,-8.92570344200001));
#167779=CARTESIAN_POINT('Ctrl Pts',(6.24754699199994,11.6,-8.92570344200001));
#167780=CARTESIAN_POINT('Ctrl Pts',(6.24984667299994,15.2,-8.92740908100001));
#167781=CARTESIAN_POINT('Ctrl Pts',(6.24984667299994,11.6,-8.92740908100001));
#167782=CARTESIAN_POINT('Ctrl Pts',(6.25215226099994,15.2,-8.92911613600001));
#167783=CARTESIAN_POINT('Ctrl Pts',(6.25215226099994,11.6,-8.92911613600001));
#167784=CARTESIAN_POINT('Ctrl Pts',(6.25446375499994,15.2,-8.93082459400001));
#167785=CARTESIAN_POINT('Ctrl Pts',(6.25446375499994,11.6,-8.93082459400001));
#167786=CARTESIAN_POINT('Ctrl Pts',(6.25678114899994,15.2,-8.93253444400001));
#167787=CARTESIAN_POINT('Ctrl Pts',(6.25678114899994,11.6,-8.93253444400001));
#167788=CARTESIAN_POINT('Ctrl Pts',(6.25910444299994,15.2,-8.93424567300002));
#167789=CARTESIAN_POINT('Ctrl Pts',(6.25910444299994,11.6,-8.93424567300002));
#167790=CARTESIAN_POINT('Ctrl Pts',(6.26143362999994,15.2,-8.93595826800002));
#167791=CARTESIAN_POINT('Ctrl Pts',(6.26143362999994,11.6,-8.93595826800002));
#167792=CARTESIAN_POINT('Ctrl Pts',(6.26376870799994,15.2,-8.93767221800001));
#167793=CARTESIAN_POINT('Ctrl Pts',(6.26376870799994,11.6,-8.93767221800001));
#167794=CARTESIAN_POINT('Ctrl Pts',(6.26610967499994,15.2,-8.93938751000002));
#167795=CARTESIAN_POINT('Ctrl Pts',(6.26610967499994,11.6,-8.93938751000002));
#167796=CARTESIAN_POINT('Ctrl Pts',(6.26845652499994,15.2,-8.94110413200002));
#167797=CARTESIAN_POINT('Ctrl Pts',(6.26845652499994,11.6,-8.94110413200002));
#167798=CARTESIAN_POINT('Ctrl Pts',(6.27080925699994,15.2,-8.94282207100002));
#167799=CARTESIAN_POINT('Ctrl Pts',(6.27080925699994,11.6,-8.94282207100002));
#167800=CARTESIAN_POINT('Ctrl Pts',(6.27316786699994,15.2,-8.94454131600002));
#167801=CARTESIAN_POINT('Ctrl Pts',(6.27316786699994,11.6,-8.94454131600002));
#167802=CARTESIAN_POINT('Ctrl Pts',(6.27553235099994,15.2,-8.94626185400002));
#167803=CARTESIAN_POINT('Ctrl Pts',(6.27553235099994,11.6,-8.94626185400002));
#167804=CARTESIAN_POINT('Ctrl Pts',(6.27790270499994,15.2,-8.94798367200002));
#167805=CARTESIAN_POINT('Ctrl Pts',(6.27790270499994,11.6,-8.94798367200002));
#167806=CARTESIAN_POINT('Ctrl Pts',(6.28027892799994,15.2,-8.94970676000002));
#167807=CARTESIAN_POINT('Ctrl Pts',(6.28027892799994,11.6,-8.94970676000002));
#167808=CARTESIAN_POINT('Ctrl Pts',(6.28266101299994,15.2,-8.95143110400002));
#167809=CARTESIAN_POINT('Ctrl Pts',(6.28266101299994,11.6,-8.95143110400002));
#167810=CARTESIAN_POINT('Ctrl Pts',(6.28504895899994,15.2,-8.95315669400001));
#167811=CARTESIAN_POINT('Ctrl Pts',(6.28504895899994,11.6,-8.95315669400001));
#167812=CARTESIAN_POINT('Ctrl Pts',(6.28744276399994,15.2,-8.95488351500001));
#167813=CARTESIAN_POINT('Ctrl Pts',(6.28744276399994,11.6,-8.95488351500001));
#167814=CARTESIAN_POINT('Ctrl Pts',(6.28984242199994,15.2,-8.95661155900001));
#167815=CARTESIAN_POINT('Ctrl Pts',(6.28984242199994,11.6,-8.95661155900001));
#167816=CARTESIAN_POINT('Ctrl Pts',(6.29224792999994,15.2,-8.95834081000002));
#167817=CARTESIAN_POINT('Ctrl Pts',(6.29224792999994,11.6,-8.95834081000002));
#167818=CARTESIAN_POINT('Ctrl Pts',(6.29465928599994,15.2,-8.96007125900002));
#167819=CARTESIAN_POINT('Ctrl Pts',(6.29465928599994,11.6,-8.96007125900002));
#167820=CARTESIAN_POINT('Ctrl Pts',(6.29707648499994,15.2,-8.96180289200002));
#167821=CARTESIAN_POINT('Ctrl Pts',(6.29707648499994,11.6,-8.96180289200002));
#167822=CARTESIAN_POINT('Ctrl Pts',(6.29949952399994,15.2,-8.96353569800001));
#167823=CARTESIAN_POINT('Ctrl Pts',(6.29949952399994,11.6,-8.96353569800001));
#167824=CARTESIAN_POINT('Ctrl Pts',(6.30192839999994,15.2,-8.96526966600002));
#167825=CARTESIAN_POINT('Ctrl Pts',(6.30192839999994,11.6,-8.96526966600002));
#167826=CARTESIAN_POINT('Ctrl Pts',(6.30436310999994,15.2,-8.96700478300002));
#167827=CARTESIAN_POINT('Ctrl Pts',(6.30436310999994,11.6,-8.96700478300002));
#167828=CARTESIAN_POINT('Ctrl Pts',(6.30680364899994,15.2,-8.96874103900002));
#167829=CARTESIAN_POINT('Ctrl Pts',(6.30680364899994,11.6,-8.96874103900002));
#167830=CARTESIAN_POINT('Ctrl Pts',(6.30925001499994,15.2,-8.97047842000001));
#167831=CARTESIAN_POINT('Ctrl Pts',(6.30925001499994,11.6,-8.97047842000001));
#167832=CARTESIAN_POINT('Ctrl Pts',(6.31170220399994,15.2,-8.97221691500001));
#167833=CARTESIAN_POINT('Ctrl Pts',(6.31170220399994,11.6,-8.97221691500001));
#167834=CARTESIAN_POINT('Ctrl Pts',(6.31416021399994,15.2,-8.97395651300002));
#167835=CARTESIAN_POINT('Ctrl Pts',(6.31416021399994,11.6,-8.97395651300002));
#167836=CARTESIAN_POINT('Ctrl Pts',(6.31662403899994,15.2,-8.97569720100002));
#167837=CARTESIAN_POINT('Ctrl Pts',(6.31662403899994,11.6,-8.97569720100002));
#167838=CARTESIAN_POINT('Ctrl Pts',(6.31909367699994,15.2,-8.97743896900002));
#167839=CARTESIAN_POINT('Ctrl Pts',(6.31909367699994,11.6,-8.97743896900002));
#167840=CARTESIAN_POINT('Ctrl Pts',(6.32156912499994,15.2,-8.97918180400002));
#167841=CARTESIAN_POINT('Ctrl Pts',(6.32156912499994,11.6,-8.97918180400002));
#167842=CARTESIAN_POINT('Ctrl Pts',(6.32405037899994,15.2,-8.98092569600001));
#167843=CARTESIAN_POINT('Ctrl Pts',(6.32405037899994,11.6,-8.98092569600001));
#167844=CARTESIAN_POINT('Ctrl Pts',(6.32653743599994,15.2,-8.98267063100001));
#167845=CARTESIAN_POINT('Ctrl Pts',(6.32653743599994,11.6,-8.98267063100001));
#167846=CARTESIAN_POINT('Ctrl Pts',(6.32903029199994,15.2,-8.98441660100002));
#167847=CARTESIAN_POINT('Ctrl Pts',(6.32903029199994,11.6,-8.98441660100002));
#167848=CARTESIAN_POINT('Ctrl Pts',(6.33152894299994,15.2,-8.98616359100001));
#167849=CARTESIAN_POINT('Ctrl Pts',(6.33152894299994,11.6,-8.98616359100001));
#167850=CARTESIAN_POINT('Ctrl Pts',(6.33403338799994,15.2,-8.98791159100002));
#167851=CARTESIAN_POINT('Ctrl Pts',(6.33403338799994,11.6,-8.98791159100002));
#167852=CARTESIAN_POINT('Ctrl Pts',(6.33654362099994,15.2,-8.98966059000001));
#167853=CARTESIAN_POINT('Ctrl Pts',(6.33654362099994,11.6,-8.98966059000001));
#167854=CARTESIAN_POINT('Ctrl Pts',(6.33905963999994,15.2,-8.99141057600002));
#167855=CARTESIAN_POINT('Ctrl Pts',(6.33905963999994,11.6,-8.99141057600002));
#167856=CARTESIAN_POINT('Ctrl Pts',(6.34158143999994,15.2,-8.99316153900001));
#167857=CARTESIAN_POINT('Ctrl Pts',(6.34158143999994,11.6,-8.99316153900001));
#167858=CARTESIAN_POINT('Ctrl Pts',(6.34410901999994,15.2,-8.99491346500002));
#167859=CARTESIAN_POINT('Ctrl Pts',(6.34410901999994,11.6,-8.99491346500002));
#167860=CARTESIAN_POINT('Ctrl Pts',(6.34664237499994,15.2,-8.99666634500001));
#167861=CARTESIAN_POINT('Ctrl Pts',(6.34664237499994,11.6,-8.99666634500001));
#167862=CARTESIAN_POINT('Ctrl Pts',(6.34918150099994,15.2,-8.99842016600001));
#167863=CARTESIAN_POINT('Ctrl Pts',(6.34918150099994,11.6,-8.99842016600001));
#167864=CARTESIAN_POINT('Ctrl Pts',(6.35172639699994,15.2,-9.00017491800002));
#167865=CARTESIAN_POINT('Ctrl Pts',(6.35172639699994,11.6,-9.00017491800002));
#167866=CARTESIAN_POINT('Ctrl Pts',(6.35427705599994,15.2,-9.00193058900001));
#167867=CARTESIAN_POINT('Ctrl Pts',(6.35427705599994,11.6,-9.00193058900001));
#167868=CARTESIAN_POINT('Ctrl Pts',(6.35683347799994,15.2,-9.00368716800001));
#167869=CARTESIAN_POINT('Ctrl Pts',(6.35683347799994,11.6,-9.00368716800001));
#167870=CARTESIAN_POINT('Ctrl Pts',(6.35939565699994,15.2,-9.00544464400001));
#167871=CARTESIAN_POINT('Ctrl Pts',(6.35939565699994,11.6,-9.00544464400001));
#167872=CARTESIAN_POINT('Ctrl Pts',(6.36196359199994,15.2,-9.00720300600002));
#167873=CARTESIAN_POINT('Ctrl Pts',(6.36196359199994,11.6,-9.00720300600002));
#167874=CARTESIAN_POINT('Ctrl Pts',(6.36453727799994,15.2,-9.00896224300002));
#167875=CARTESIAN_POINT('Ctrl Pts',(6.36453727799994,11.6,-9.00896224300002));
#167876=CARTESIAN_POINT('Ctrl Pts',(6.36711671099994,15.2,-9.01072234300001));
#167877=CARTESIAN_POINT('Ctrl Pts',(6.36711671099994,11.6,-9.01072234300001));
#167878=CARTESIAN_POINT('Ctrl Pts',(6.36970188799994,15.2,-9.01248329400002));
#167879=CARTESIAN_POINT('Ctrl Pts',(6.36970188799994,11.6,-9.01248329400002));
#167880=CARTESIAN_POINT('Ctrl Pts',(6.37229280699994,15.2,-9.01424508800002));
#167881=CARTESIAN_POINT('Ctrl Pts',(6.37229280699994,11.6,-9.01424508800002));
#167882=CARTESIAN_POINT('Ctrl Pts',(6.37488946299994,15.2,-9.01600771300001));
#167883=CARTESIAN_POINT('Ctrl Pts',(6.37488946299994,11.6,-9.01600771300001));
#167884=CARTESIAN_POINT('Ctrl Pts',(6.37749185299994,15.2,-9.01777115600002));
#167885=CARTESIAN_POINT('Ctrl Pts',(6.37749185299994,11.6,-9.01777115600002));
#167886=CARTESIAN_POINT('Ctrl Pts',(6.38009997299994,15.2,-9.01953540700001));
#167887=CARTESIAN_POINT('Ctrl Pts',(6.38009997299994,11.6,-9.01953540700001));
#167888=CARTESIAN_POINT('Ctrl Pts',(6.38271382099994,15.2,-9.02130045600002));
#167889=CARTESIAN_POINT('Ctrl Pts',(6.38271382099994,11.6,-9.02130045600002));
#167890=CARTESIAN_POINT('Ctrl Pts',(6.38533339199994,15.2,-9.02306629200002));
#167891=CARTESIAN_POINT('Ctrl Pts',(6.38533339199994,11.6,-9.02306629200002));
#167892=CARTESIAN_POINT('Ctrl Pts',(6.38795868399994,15.2,-9.02483290300001));
#167893=CARTESIAN_POINT('Ctrl Pts',(6.38795868399994,11.6,-9.02483290300001));
#167894=CARTESIAN_POINT('Ctrl Pts',(6.39058969199994,15.2,-9.02660027900002));
#167895=CARTESIAN_POINT('Ctrl Pts',(6.39058969199994,11.6,-9.02660027900002));
#167896=CARTESIAN_POINT('Ctrl Pts',(6.39322641399994,15.2,-9.02836840800001));
#167897=CARTESIAN_POINT('Ctrl Pts',(6.39322641399994,11.6,-9.02836840800001));
#167898=CARTESIAN_POINT('Ctrl Pts',(6.39586884499994,15.2,-9.03013728200002));
#167899=CARTESIAN_POINT('Ctrl Pts',(6.39586884499994,11.6,-9.03013728200002));
#167900=CARTESIAN_POINT('Ctrl Pts',(6.39851698299994,15.2,-9.03190688700001));
#167901=CARTESIAN_POINT('Ctrl Pts',(6.39851698299994,11.6,-9.03190688700001));
#167902=CARTESIAN_POINT('Ctrl Pts',(6.40117082299994,15.2,-9.03367721300001));
#167903=CARTESIAN_POINT('Ctrl Pts',(6.40117082299994,11.6,-9.03367721300001));
#167904=CARTESIAN_POINT('Ctrl Pts',(6.40383036299994,15.2,-9.03544825000001));
#167905=CARTESIAN_POINT('Ctrl Pts',(6.40383036299994,11.6,-9.03544825000001));
#167906=CARTESIAN_POINT('Ctrl Pts',(6.40649559999994,15.2,-9.03721998700002));
#167907=CARTESIAN_POINT('Ctrl Pts',(6.40649559999994,11.6,-9.03721998700002));
#167908=CARTESIAN_POINT('Ctrl Pts',(6.40916652899994,15.2,-9.03899241300002));
#167909=CARTESIAN_POINT('Ctrl Pts',(6.40916652899994,11.6,-9.03899241300002));
#167910=CARTESIAN_POINT('Ctrl Pts',(6.41184314599994,15.2,-9.04076551800001));
#167911=CARTESIAN_POINT('Ctrl Pts',(6.41184314599994,11.6,-9.04076551800001));
#167912=CARTESIAN_POINT('Ctrl Pts',(6.41452544999994,15.2,-9.04253929100001));
#167913=CARTESIAN_POINT('Ctrl Pts',(6.41452544999994,11.6,-9.04253929100001));
#167914=CARTESIAN_POINT('Ctrl Pts',(6.41721343599994,15.2,-9.04431372100002));
#167915=CARTESIAN_POINT('Ctrl Pts',(6.41721343599994,11.6,-9.04431372100002));
#167916=CARTESIAN_POINT('Ctrl Pts',(6.41990709999994,15.2,-9.04608879800002));
#167917=CARTESIAN_POINT('Ctrl Pts',(6.41990709999994,11.6,-9.04608879800002));
#167918=CARTESIAN_POINT('Ctrl Pts',(6.42260643999994,15.2,-9.04786451100002));
#167919=CARTESIAN_POINT('Ctrl Pts',(6.42260643999994,11.6,-9.04786451100002));
#167920=CARTESIAN_POINT('Ctrl Pts',(6.42531145199994,15.2,-9.04964084900002));
#167921=CARTESIAN_POINT('Ctrl Pts',(6.42531145199994,11.6,-9.04964084900002));
#167922=CARTESIAN_POINT('Ctrl Pts',(6.42802213199994,15.2,-9.05141780400001));
#167923=CARTESIAN_POINT('Ctrl Pts',(6.42802213199994,11.6,-9.05141780400001));
#167924=CARTESIAN_POINT('Ctrl Pts',(6.43073847599994,15.2,-9.05319536200002));
#167925=CARTESIAN_POINT('Ctrl Pts',(6.43073847599994,11.6,-9.05319536200002));
#167926=CARTESIAN_POINT('Ctrl Pts',(6.43346048199994,15.2,-9.05497351500001));
#167927=CARTESIAN_POINT('Ctrl Pts',(6.43346048199994,11.6,-9.05497351500001));
#167928=CARTESIAN_POINT('Ctrl Pts',(6.43618814599995,15.2,-9.05675225100002));
#167929=CARTESIAN_POINT('Ctrl Pts',(6.43618814599995,11.6,-9.05675225100002));
#167930=CARTESIAN_POINT('Ctrl Pts',(6.43892146399994,15.2,-9.05853156000001));
#167931=CARTESIAN_POINT('Ctrl Pts',(6.43892146399994,11.6,-9.05853156000001));
#167932=CARTESIAN_POINT('Ctrl Pts',(6.44166043299994,15.2,-9.06031143300002));
#167933=CARTESIAN_POINT('Ctrl Pts',(6.44166043299994,11.6,-9.06031143300002));
#167934=CARTESIAN_POINT('Ctrl Pts',(6.44440504999994,15.2,-9.06209185800002));
#167935=CARTESIAN_POINT('Ctrl Pts',(6.44440504999994,11.6,-9.06209185800002));
#167936=CARTESIAN_POINT('Ctrl Pts',(6.44715531099994,15.2,-9.06387282500001));
#167937=CARTESIAN_POINT('Ctrl Pts',(6.44715531099994,11.6,-9.06387282500001));
#167938=CARTESIAN_POINT('Ctrl Pts',(6.44991121199994,15.2,-9.06565432300001));
#167939=CARTESIAN_POINT('Ctrl Pts',(6.44991121199994,11.6,-9.06565432300001));
#167940=CARTESIAN_POINT('Ctrl Pts',(6.45267274999994,15.2,-9.06743634400001));
#167941=CARTESIAN_POINT('Ctrl Pts',(6.45267274999994,11.6,-9.06743634400001));
#167942=CARTESIAN_POINT('Ctrl Pts',(6.45543992299994,15.2,-9.06921887500001));
#167943=CARTESIAN_POINT('Ctrl Pts',(6.45543992299994,11.6,-9.06921887500001));
#167944=CARTESIAN_POINT('Ctrl Pts',(6.45821272399994,15.2,-9.07100190800002));
#167945=CARTESIAN_POINT('Ctrl Pts',(6.45821272399994,11.6,-9.07100190800002));
#167946=CARTESIAN_POINT('Ctrl Pts',(6.46099115299994,15.2,-9.07278543100002));
#167947=CARTESIAN_POINT('Ctrl Pts',(6.46099115299994,11.6,-9.07278543100002));
#167948=CARTESIAN_POINT('Ctrl Pts',(6.46377520499994,15.2,-9.07456943400001));
#167949=CARTESIAN_POINT('Ctrl Pts',(6.46377520499994,11.6,-9.07456943400001));
#167950=CARTESIAN_POINT('Ctrl Pts',(6.46656487599994,15.2,-9.07635390800002));
#167951=CARTESIAN_POINT('Ctrl Pts',(6.46656487599994,11.6,-9.07635390800002));
#167952=CARTESIAN_POINT('Ctrl Pts',(6.46936016299994,15.2,-9.07813884200002));
#167953=CARTESIAN_POINT('Ctrl Pts',(6.46936016299994,11.6,-9.07813884200002));
#167954=CARTESIAN_POINT('Ctrl Pts',(6.47216106399994,15.2,-9.07992422500002));
#167955=CARTESIAN_POINT('Ctrl Pts',(6.47216106399994,11.6,-9.07992422500002));
#167956=CARTESIAN_POINT('Ctrl Pts',(6.47496757199994,15.2,-9.08171004900002));
#167957=CARTESIAN_POINT('Ctrl Pts',(6.47496757199994,11.6,-9.08171004900002));
#167958=CARTESIAN_POINT('Ctrl Pts',(6.47777968799994,15.2,-9.08349630400001));
#167959=CARTESIAN_POINT('Ctrl Pts',(6.47777968799994,11.6,-9.08349630400001));
#167960=CARTESIAN_POINT('Ctrl Pts',(6.48059740499994,15.2,-9.08528297600002));
#167961=CARTESIAN_POINT('Ctrl Pts',(6.48059740499994,11.6,-9.08528297600002));
#167962=CARTESIAN_POINT('Ctrl Pts',(6.48342072099994,15.2,-9.08707005900002));
#167963=CARTESIAN_POINT('Ctrl Pts',(6.48342072099994,11.6,-9.08707005900002));
#167964=CARTESIAN_POINT('Ctrl Pts',(6.48624963199994,15.2,-9.08885754100002));
#167965=CARTESIAN_POINT('Ctrl Pts',(6.48624963199994,11.6,-9.08885754100002));
#167966=CARTESIAN_POINT('Ctrl Pts',(6.48908413499994,15.2,-9.09064541400002));
#167967=CARTESIAN_POINT('Ctrl Pts',(6.48908413499994,11.6,-9.09064541400002));
#167968=CARTESIAN_POINT('Ctrl Pts',(6.49192422599994,15.2,-9.09243366500002));
#167969=CARTESIAN_POINT('Ctrl Pts',(6.49192422599994,11.6,-9.09243366500002));
#167970=CARTESIAN_POINT('Ctrl Pts',(6.49476990199994,15.2,-9.09422228700001));
#167971=CARTESIAN_POINT('Ctrl Pts',(6.49476990199994,11.6,-9.09422228700001));
#167972=CARTESIAN_POINT('Ctrl Pts',(6.49762115899994,15.2,-9.09601126700002));
#167973=CARTESIAN_POINT('Ctrl Pts',(6.49762115899994,11.6,-9.09601126700002));
#167974=CARTESIAN_POINT('Ctrl Pts',(6.50047799399994,15.2,-9.09780059800001));
#167975=CARTESIAN_POINT('Ctrl Pts',(6.50047799399994,11.6,-9.09780059800001));
#167976=CARTESIAN_POINT('Ctrl Pts',(6.50334040299994,15.2,-9.09959026900001));
#167977=CARTESIAN_POINT('Ctrl Pts',(6.50334040299994,11.6,-9.09959026900001));
#167978=CARTESIAN_POINT('Ctrl Pts',(6.50620838199995,15.2,-9.10138026900002));
#167979=CARTESIAN_POINT('Ctrl Pts',(6.50620838199995,11.6,-9.10138026900002));
#167980=CARTESIAN_POINT('Ctrl Pts',(6.50908192999994,15.2,-9.10317059000001));
#167981=CARTESIAN_POINT('Ctrl Pts',(6.50908192999994,11.6,-9.10317059000001));
#167982=CARTESIAN_POINT('Ctrl Pts',(6.51196104099995,15.2,-9.10496122100002));
#167983=CARTESIAN_POINT('Ctrl Pts',(6.51196104099995,11.6,-9.10496122100002));
#167984=CARTESIAN_POINT('Ctrl Pts',(6.51484571099994,15.2,-9.10675215300002));
#167985=CARTESIAN_POINT('Ctrl Pts',(6.51484571099994,11.6,-9.10675215300002));
#167986=CARTESIAN_POINT('Ctrl Pts',(6.51773593899994,15.2,-9.10854337500002));
#167987=CARTESIAN_POINT('Ctrl Pts',(6.51773593899994,11.6,-9.10854337500002));
#167988=CARTESIAN_POINT('Ctrl Pts',(6.52063172099994,15.2,-9.11033487800001));
#167989=CARTESIAN_POINT('Ctrl Pts',(6.52063172099994,11.6,-9.11033487800001));
#167990=CARTESIAN_POINT('Ctrl Pts',(6.52353305099994,15.2,-9.11212665200001));
#167991=CARTESIAN_POINT('Ctrl Pts',(6.52353305099994,11.6,-9.11212665200001));
#167992=CARTESIAN_POINT('Ctrl Pts',(6.52643992799994,15.2,-9.11391868900001));
#167993=CARTESIAN_POINT('Ctrl Pts',(6.52643992799994,11.6,-9.11391868900001));
#167994=CARTESIAN_POINT('Ctrl Pts',(6.52935234699994,15.2,-9.11571097500002));
#167995=CARTESIAN_POINT('Ctrl Pts',(6.52935234699994,11.6,-9.11571097500002));
#167996=CARTESIAN_POINT('Ctrl Pts',(6.53227030599994,15.2,-9.11750350600002));
#167997=CARTESIAN_POINT('Ctrl Pts',(6.53227030599994,11.6,-9.11750350600002));
#167998=CARTESIAN_POINT('Ctrl Pts',(6.53519379999994,15.2,-9.11929626800001));
#167999=CARTESIAN_POINT('Ctrl Pts',(6.53519379999994,11.6,-9.11929626800001));
#168000=CARTESIAN_POINT('Ctrl Pts',(6.53812282699994,15.2,-9.12108925300002));
#168001=CARTESIAN_POINT('Ctrl Pts',(6.53812282699994,11.6,-9.12108925300002));
#168002=CARTESIAN_POINT('Ctrl Pts',(6.54105738299994,15.2,-9.12288245200001));
#168003=CARTESIAN_POINT('Ctrl Pts',(6.54105738299994,11.6,-9.12288245200001));
#168004=CARTESIAN_POINT('Ctrl Pts',(6.54399746299994,15.2,-9.12467585300002));
#168005=CARTESIAN_POINT('Ctrl Pts',(6.54399746299994,11.6,-9.12467585300002));
#168006=CARTESIAN_POINT('Ctrl Pts',(6.54694306499994,15.2,-9.12646944900001));
#168007=CARTESIAN_POINT('Ctrl Pts',(6.54694306499994,11.6,-9.12646944900001));
#168008=CARTESIAN_POINT('Ctrl Pts',(6.54989418399994,15.2,-9.12826322900001));
#168009=CARTESIAN_POINT('Ctrl Pts',(6.54989418399994,11.6,-9.12826322900001));
#168010=CARTESIAN_POINT('Ctrl Pts',(6.55285081899994,15.2,-9.13005718400001));
#168011=CARTESIAN_POINT('Ctrl Pts',(6.55285081899994,11.6,-9.13005718400001));
#168012=CARTESIAN_POINT('Ctrl Pts',(6.55581296599994,15.2,-9.13185130500001));
#168013=CARTESIAN_POINT('Ctrl Pts',(6.55581296599994,11.6,-9.13185130500001));
#168014=CARTESIAN_POINT('Ctrl Pts',(6.55878061899994,15.2,-9.13364558100002));
#168015=CARTESIAN_POINT('Ctrl Pts',(6.55878061899994,11.6,-9.13364558100002));
#168016=CARTESIAN_POINT('Ctrl Pts',(6.56175377599994,15.2,-9.13544000400002));
#168017=CARTESIAN_POINT('Ctrl Pts',(6.56175377599994,11.6,-9.13544000400002));
#168018=CARTESIAN_POINT('Ctrl Pts',(6.56473243399994,15.2,-9.13723456500002));
#168019=CARTESIAN_POINT('Ctrl Pts',(6.56473243399994,11.6,-9.13723456500002));
#168020=CARTESIAN_POINT('Ctrl Pts',(6.56771658899994,15.2,-9.13902925200002));
#168021=CARTESIAN_POINT('Ctrl Pts',(6.56771658899994,11.6,-9.13902925200002));
#168022=CARTESIAN_POINT('Ctrl Pts',(6.57070623699994,15.2,-9.14082405700002));
#168023=CARTESIAN_POINT('Ctrl Pts',(6.57070623699994,11.6,-9.14082405700002));
#168024=CARTESIAN_POINT('Ctrl Pts',(6.57370137599994,15.2,-9.14261897200002));
#168025=CARTESIAN_POINT('Ctrl Pts',(6.57370137599994,11.6,-9.14261897200002));
#168026=CARTESIAN_POINT('Ctrl Pts',(6.57670199999994,15.2,-9.14441398600001));
#168027=CARTESIAN_POINT('Ctrl Pts',(6.57670199999994,11.6,-9.14441398600001));
#168028=CARTESIAN_POINT('Ctrl Pts',(6.57970810799994,15.2,-9.14620908900002));
#168029=CARTESIAN_POINT('Ctrl Pts',(6.57970810799994,11.6,-9.14620908900002));
#168030=CARTESIAN_POINT('Ctrl Pts',(6.58271969499994,15.2,-9.14800427400002));
#168031=CARTESIAN_POINT('Ctrl Pts',(6.58271969499994,11.6,-9.14800427400002));
#168032=CARTESIAN_POINT('Ctrl Pts',(6.58573675799994,15.2,-9.14979953100002));
#168033=CARTESIAN_POINT('Ctrl Pts',(6.58573675799994,11.6,-9.14979953100002));
#168034=CARTESIAN_POINT('Ctrl Pts',(6.58875929299994,15.2,-9.15159484900002));
#168035=CARTESIAN_POINT('Ctrl Pts',(6.58875929299994,11.6,-9.15159484900002));
#168036=CARTESIAN_POINT('Ctrl Pts',(6.59178729699994,15.2,-9.15339022000002));
#168037=CARTESIAN_POINT('Ctrl Pts',(6.59178729699994,11.6,-9.15339022000002));
#168038=CARTESIAN_POINT('Ctrl Pts',(6.59482076499994,15.2,-9.15518563400001));
#168039=CARTESIAN_POINT('Ctrl Pts',(6.59482076499994,11.6,-9.15518563400001));
#168040=CARTESIAN_POINT('Ctrl Pts',(6.59785969599994,15.2,-9.15698108300001));
#168041=CARTESIAN_POINT('Ctrl Pts',(6.59785969599994,11.6,-9.15698108300001));
#168042=CARTESIAN_POINT('Ctrl Pts',(6.60090408599994,15.2,-9.15877655700001));
#168043=CARTESIAN_POINT('Ctrl Pts',(6.60090408599994,11.6,-9.15877655700001));
#168044=CARTESIAN_POINT('Ctrl Pts',(6.60395392899995,15.2,-9.16057204700002));
#168045=CARTESIAN_POINT('Ctrl Pts',(6.60395392899995,11.6,-9.16057204700002));
#168046=CARTESIAN_POINT('Ctrl Pts',(6.60700922399994,15.2,-9.16236754400002));
#168047=CARTESIAN_POINT('Ctrl Pts',(6.60700922399994,11.6,-9.16236754400002));
#168048=CARTESIAN_POINT('Ctrl Pts',(6.61006996599995,15.2,-9.16416303900002));
#168049=CARTESIAN_POINT('Ctrl Pts',(6.61006996599995,11.6,-9.16416303900002));
#168050=CARTESIAN_POINT('Ctrl Pts',(6.61313615199994,15.2,-9.16595852100002));
#168051=CARTESIAN_POINT('Ctrl Pts',(6.61313615199994,11.6,-9.16595852100002));
#168052=CARTESIAN_POINT('Ctrl Pts',(6.61620777899994,15.2,-9.16775398400001));
#168053=CARTESIAN_POINT('Ctrl Pts',(6.61620777899994,11.6,-9.16775398400001));
#168054=CARTESIAN_POINT('Ctrl Pts',(6.61928484299994,15.2,-9.16954941700002));
#168055=CARTESIAN_POINT('Ctrl Pts',(6.61928484299994,11.6,-9.16954941700002));
#168056=CARTESIAN_POINT('Ctrl Pts',(6.62236733999994,15.2,-9.17134481100002));
#168057=CARTESIAN_POINT('Ctrl Pts',(6.62236733999994,11.6,-9.17134481100002));
#168058=CARTESIAN_POINT('Ctrl Pts',(6.62545526699994,15.2,-9.17314015600001));
#168059=CARTESIAN_POINT('Ctrl Pts',(6.62545526699994,11.6,-9.17314015600001));
#168060=CARTESIAN_POINT('Ctrl Pts',(6.62854862099994,15.2,-9.17493544700001));
#168061=CARTESIAN_POINT('Ctrl Pts',(6.62854862099994,11.6,-9.17493544700001));
#168062=CARTESIAN_POINT('Ctrl Pts',(6.63164739699994,15.2,-9.17673067000001));
#168063=CARTESIAN_POINT('Ctrl Pts',(6.63164739699994,11.6,-9.17673067000001));
#168064=CARTESIAN_POINT('Ctrl Pts',(6.63475159199994,15.2,-9.17852581800001));
#168065=CARTESIAN_POINT('Ctrl Pts',(6.63475159199994,11.6,-9.17852581800001));
#168066=CARTESIAN_POINT('Ctrl Pts',(6.63786120299994,15.2,-9.18032088200002));
#168067=CARTESIAN_POINT('Ctrl Pts',(6.63786120299994,11.6,-9.18032088200002));
#168068=CARTESIAN_POINT('Ctrl Pts',(6.64097622599994,15.2,-9.18211585500002));
#168069=CARTESIAN_POINT('Ctrl Pts',(6.64097622599994,11.6,-9.18211585500002));
#168070=CARTESIAN_POINT('Ctrl Pts',(6.64409665799995,15.2,-9.18391072500001));
#168071=CARTESIAN_POINT('Ctrl Pts',(6.64409665799995,11.6,-9.18391072500001));
#168072=CARTESIAN_POINT('Ctrl Pts',(6.64722249499994,15.2,-9.18570548400002));
#168073=CARTESIAN_POINT('Ctrl Pts',(6.64722249499994,11.6,-9.18570548400002));
#168074=CARTESIAN_POINT('Ctrl Pts',(6.65035373299995,15.2,-9.18750012300002));
#168075=CARTESIAN_POINT('Ctrl Pts',(6.65035373299995,11.6,-9.18750012300002));
#168076=CARTESIAN_POINT('Ctrl Pts',(6.65349036899994,15.2,-9.18929463500002));
#168077=CARTESIAN_POINT('Ctrl Pts',(6.65349036899994,11.6,-9.18929463500002));
#168078=CARTESIAN_POINT('Ctrl Pts',(6.65663239999994,15.2,-9.19108900900002));
#168079=CARTESIAN_POINT('Ctrl Pts',(6.65663239999994,11.6,-9.19108900900002));
#168080=CARTESIAN_POINT('Ctrl Pts',(6.65977982099994,15.2,-9.19288323700002));
#168081=CARTESIAN_POINT('Ctrl Pts',(6.65977982099994,11.6,-9.19288323700002));
#168082=CARTESIAN_POINT('Ctrl Pts',(6.66293262999995,15.2,-9.19467731100001));
#168083=CARTESIAN_POINT('Ctrl Pts',(6.66293262999995,11.6,-9.19467731100001));
#168084=CARTESIAN_POINT('Ctrl Pts',(6.66609082299995,15.2,-9.19647121900002));
#168085=CARTESIAN_POINT('Ctrl Pts',(6.66609082299995,11.6,-9.19647121900002));
#168086=CARTESIAN_POINT('Ctrl Pts',(6.66925439499994,15.2,-9.19826495600002));
#168087=CARTESIAN_POINT('Ctrl Pts',(6.66925439499994,11.6,-9.19826495600002));
#168088=CARTESIAN_POINT('Ctrl Pts',(6.67242334399995,15.2,-9.20005851000001));
#168089=CARTESIAN_POINT('Ctrl Pts',(6.67242334399995,11.6,-9.20005851000001));
#168090=CARTESIAN_POINT('Ctrl Pts',(6.67559766699994,15.2,-9.20185187500002));
#168091=CARTESIAN_POINT('Ctrl Pts',(6.67559766699994,11.6,-9.20185187500002));
#168092=CARTESIAN_POINT('Ctrl Pts',(6.67877735899994,15.2,-9.20364504200002));
#168093=CARTESIAN_POINT('Ctrl Pts',(6.67877735899994,11.6,-9.20364504200002));
#168094=CARTESIAN_POINT('Ctrl Pts',(6.68196241599994,15.2,-9.20543800000001));
#168095=CARTESIAN_POINT('Ctrl Pts',(6.68196241599994,11.6,-9.20543800000001));
#168096=CARTESIAN_POINT('Ctrl Pts',(6.68515283699994,15.2,-9.20723074200002));
#168097=CARTESIAN_POINT('Ctrl Pts',(6.68515283699994,11.6,-9.20723074200002));
#168098=CARTESIAN_POINT('Ctrl Pts',(6.68834861499994,15.2,-9.20902325900002));
#168099=CARTESIAN_POINT('Ctrl Pts',(6.68834861499994,11.6,-9.20902325900002));
#168100=CARTESIAN_POINT('Ctrl Pts',(6.69154974999994,15.2,-9.21081554300001));
#168101=CARTESIAN_POINT('Ctrl Pts',(6.69154974999994,11.6,-9.21081554300001));
#168102=CARTESIAN_POINT('Ctrl Pts',(6.69475623599994,15.2,-9.21260758400001));
#168103=CARTESIAN_POINT('Ctrl Pts',(6.69475623599994,11.6,-9.21260758400001));
#168104=CARTESIAN_POINT('Ctrl Pts',(6.69796806999994,15.2,-9.21439937500002));
#168105=CARTESIAN_POINT('Ctrl Pts',(6.69796806999994,11.6,-9.21439937500002));
#168106=CARTESIAN_POINT('Ctrl Pts',(6.70118524799994,15.2,-9.21619090500002));
#168107=CARTESIAN_POINT('Ctrl Pts',(6.70118524799994,11.6,-9.21619090500002));
#168108=CARTESIAN_POINT('Ctrl Pts',(6.70440776799994,15.2,-9.21798216800001));
#168109=CARTESIAN_POINT('Ctrl Pts',(6.70440776799994,11.6,-9.21798216800001));
#168110=CARTESIAN_POINT('Ctrl Pts',(6.70763562499994,15.2,-9.21977315400002));
#168111=CARTESIAN_POINT('Ctrl Pts',(6.70763562499994,11.6,-9.21977315400002));
#168112=CARTESIAN_POINT('Ctrl Pts',(6.71086881499994,15.2,-9.22156385400001));
#168113=CARTESIAN_POINT('Ctrl Pts',(6.71086881499994,11.6,-9.22156385400001));
#168114=CARTESIAN_POINT('Ctrl Pts',(6.71410733699994,15.2,-9.22335426000001));
#168115=CARTESIAN_POINT('Ctrl Pts',(6.71410733699994,11.6,-9.22335426000001));
#168116=CARTESIAN_POINT('Ctrl Pts',(6.71735118499994,15.2,-9.22514436400002));
#168117=CARTESIAN_POINT('Ctrl Pts',(6.71735118499994,11.6,-9.22514436400002));
#168118=CARTESIAN_POINT('Ctrl Pts',(6.72060035499995,15.2,-9.22693415700002));
#168119=CARTESIAN_POINT('Ctrl Pts',(6.72060035499995,11.6,-9.22693415700002));
#168120=CARTESIAN_POINT('Ctrl Pts',(6.72385484599994,15.2,-9.22872363200002));
#168121=CARTESIAN_POINT('Ctrl Pts',(6.72385484599994,11.6,-9.22872363200002));
#168122=CARTESIAN_POINT('Ctrl Pts',(6.72711465299995,15.2,-9.23051277900001));
#168123=CARTESIAN_POINT('Ctrl Pts',(6.72711465299995,11.6,-9.23051277900001));
#168124=CARTESIAN_POINT('Ctrl Pts',(6.73037977199994,15.2,-9.23230159000001));
#168125=CARTESIAN_POINT('Ctrl Pts',(6.73037977199994,11.6,-9.23230159000001));
#168126=CARTESIAN_POINT('Ctrl Pts',(6.73365020099994,15.2,-9.23409005700002));
#168127=CARTESIAN_POINT('Ctrl Pts',(6.73365020099994,11.6,-9.23409005700002));
#168128=CARTESIAN_POINT('Ctrl Pts',(6.73692593399994,15.2,-9.23587817000002));
#168129=CARTESIAN_POINT('Ctrl Pts',(6.73692593399994,11.6,-9.23587817000002));
#168130=CARTESIAN_POINT('Ctrl Pts',(6.74020696799994,15.2,-9.23766592000002));
#168131=CARTESIAN_POINT('Ctrl Pts',(6.74020696799994,11.6,-9.23766592000002));
#168132=CARTESIAN_POINT('Ctrl Pts',(6.74349330199994,15.2,-9.23945330000001));
#168133=CARTESIAN_POINT('Ctrl Pts',(6.74349330199994,11.6,-9.23945330000001));
#168134=CARTESIAN_POINT('Ctrl Pts',(6.74678492799995,15.2,-9.24124030000002));
#168135=CARTESIAN_POINT('Ctrl Pts',(6.74678492799995,11.6,-9.24124030000002));
#168136=CARTESIAN_POINT('Ctrl Pts',(6.75008184499994,15.2,-9.24302691400002));
#168137=CARTESIAN_POINT('Ctrl Pts',(6.75008184499994,11.6,-9.24302691400002));
#168138=CARTESIAN_POINT('Ctrl Pts',(6.75338404999994,15.2,-9.24481313200002));
#168139=CARTESIAN_POINT('Ctrl Pts',(6.75338404999994,11.6,-9.24481313200002));
#168140=CARTESIAN_POINT('Ctrl Pts',(6.75669153899995,15.2,-9.24659894800002));
#168141=CARTESIAN_POINT('Ctrl Pts',(6.75669153899995,11.6,-9.24659894800002));
#168142=CARTESIAN_POINT('Ctrl Pts',(6.76000430999994,15.2,-9.24838435500002));
#168143=CARTESIAN_POINT('Ctrl Pts',(6.76000430999994,11.6,-9.24838435500002));
#168144=CARTESIAN_POINT('Ctrl Pts',(6.76332235699994,15.2,-9.25016934500002));
#168145=CARTESIAN_POINT('Ctrl Pts',(6.76332235699994,11.6,-9.25016934500002));
#168146=CARTESIAN_POINT('Ctrl Pts',(6.76664567999994,15.2,-9.25195390800001));
#168147=CARTESIAN_POINT('Ctrl Pts',(6.76664567999994,11.6,-9.25195390800001));
#168148=CARTESIAN_POINT('Ctrl Pts',(6.76997427099994,15.2,-9.25373803600002));
#168149=CARTESIAN_POINT('Ctrl Pts',(6.76997427099994,11.6,-9.25373803600002));
#168150=CARTESIAN_POINT('Ctrl Pts',(6.77330812799994,15.2,-9.25552171800001));
#168151=CARTESIAN_POINT('Ctrl Pts',(6.77330812799994,11.6,-9.25552171800001));
#168152=CARTESIAN_POINT('Ctrl Pts',(6.77664724599994,15.2,-9.25730494300002));
#168153=CARTESIAN_POINT('Ctrl Pts',(6.77664724599994,11.6,-9.25730494300002));
#168154=CARTESIAN_POINT('Ctrl Pts',(6.77999162099994,15.2,-9.25908770200002));
#168155=CARTESIAN_POINT('Ctrl Pts',(6.77999162099994,11.6,-9.25908770200002));
#168156=CARTESIAN_POINT('Ctrl Pts',(6.78334124799994,15.2,-9.26086998700002));
#168157=CARTESIAN_POINT('Ctrl Pts',(6.78334124799994,11.6,-9.26086998700002));
#168158=CARTESIAN_POINT('Ctrl Pts',(6.78669612399994,15.2,-9.26265178800002));
#168159=CARTESIAN_POINT('Ctrl Pts',(6.78669612399994,11.6,-9.26265178800002));
#168160=CARTESIAN_POINT('Ctrl Pts',(6.79005624699994,15.2,-9.26443310200002));
#168161=CARTESIAN_POINT('Ctrl Pts',(6.79005624699994,11.6,-9.26443310200002));
#168162=CARTESIAN_POINT('Ctrl Pts',(6.79342161599994,15.2,-9.26621392500002));
#168163=CARTESIAN_POINT('Ctrl Pts',(6.79342161599994,11.6,-9.26621392500002));
#168164=CARTESIAN_POINT('Ctrl Pts',(6.79679222899994,15.2,-9.26799425300001));
#168165=CARTESIAN_POINT('Ctrl Pts',(6.79679222899994,11.6,-9.26799425300001));
#168166=CARTESIAN_POINT('Ctrl Pts',(6.79949291499995,15.2,-9.26941812000001));
#168167=CARTESIAN_POINT('Ctrl Pts',(6.79949291499995,11.6,-9.26941812000001));
#168168=CARTESIAN_POINT('Ctrl Pts',(6.80152078799994,15.2,-9.27048579800001));
#168169=CARTESIAN_POINT('Ctrl Pts',(6.80152078799994,11.6,-9.27048579800001));
#168170=CARTESIAN_POINT('Ctrl Pts',(6.80287375199994,15.2,-9.27119748400001));
#168171=CARTESIAN_POINT('Ctrl Pts',(6.80287375199994,11.6,-9.27119748400001));
#168172=CARTESIAN_POINT('Ctrl Pts',(6.80355049599994,15.2,-9.27155330300002));
#168173=CARTESIAN_POINT('Ctrl Pts',(6.80355049599994,11.6,-9.27155330300002));
#168174=CARTESIAN_POINT('Ctrl Pts',(5.85257411399994,15.2,-8.56667970900002));
#168175=CARTESIAN_POINT('Ctrl Pts',(5.85268447799995,15.2,-8.56681469200002));
#168176=CARTESIAN_POINT('Ctrl Pts',(5.85290912899994,15.2,-8.56708931800001));
#168177=CARTESIAN_POINT('Ctrl Pts',(5.85324973299994,15.2,-8.56750527300001));
#168178=CARTESIAN_POINT('Ctrl Pts',(5.85370897399994,15.2,-8.56806526100002));
#168179=CARTESIAN_POINT('Ctrl Pts',(5.85429055399994,15.2,-8.56877298400001));
#168180=CARTESIAN_POINT('Ctrl Pts',(5.85488228099995,15.2,-8.56949158200001));
#168181=CARTESIAN_POINT('Ctrl Pts',(5.85548078499994,15.2,-8.57021692600001));
#168182=CARTESIAN_POINT('Ctrl Pts',(5.85608606099995,15.2,-8.57094898200002));
#168183=CARTESIAN_POINT('Ctrl Pts',(5.85669810699994,15.2,-8.57168771800002));
#168184=CARTESIAN_POINT('Ctrl Pts',(5.85731691799994,15.2,-8.57243310300002));
#168185=CARTESIAN_POINT('Ctrl Pts',(5.85794249299994,15.2,-8.57318510400002));
#168186=CARTESIAN_POINT('Ctrl Pts',(5.85857482799995,15.2,-8.57394368900002));
#168187=CARTESIAN_POINT('Ctrl Pts',(5.85921391899995,15.2,-8.57470882600002));
#168188=CARTESIAN_POINT('Ctrl Pts',(5.85985976499994,15.2,-8.57548048600002));
#168189=CARTESIAN_POINT('Ctrl Pts',(5.86051236099995,15.2,-8.57625863500001));
#168190=CARTESIAN_POINT('Ctrl Pts',(5.86117170399994,15.2,-8.57704324400002));
#168191=CARTESIAN_POINT('Ctrl Pts',(5.86183779199994,15.2,-8.57783428100002));
#168192=CARTESIAN_POINT('Ctrl Pts',(5.86251061899994,15.2,-8.57863171400002));
#168193=CARTESIAN_POINT('Ctrl Pts',(5.86319018499994,15.2,-8.57943551500002));
#168194=CARTESIAN_POINT('Ctrl Pts',(5.86387648599994,15.2,-8.58024565100001));
#168195=CARTESIAN_POINT('Ctrl Pts',(5.86456951799994,15.2,-8.58106209400002));
#168196=CARTESIAN_POINT('Ctrl Pts',(5.86526927899994,15.2,-8.58188481300001));
#168197=CARTESIAN_POINT('Ctrl Pts',(5.86597576599994,15.2,-8.58271377600002));
#168198=CARTESIAN_POINT('Ctrl Pts',(5.86668897299995,15.2,-8.58354895500002));
#168199=CARTESIAN_POINT('Ctrl Pts',(5.86740889999994,15.2,-8.58439031900001));
#168200=CARTESIAN_POINT('Ctrl Pts',(5.86813554199995,15.2,-8.58523784000001));
#168201=CARTESIAN_POINT('Ctrl Pts',(5.86886889699994,15.2,-8.58609148700002));
#168202=CARTESIAN_POINT('Ctrl Pts',(5.86960896099994,15.2,-8.58695123200001));
#168203=CARTESIAN_POINT('Ctrl Pts',(5.87035573299994,15.2,-8.58781704500002));
#168204=CARTESIAN_POINT('Ctrl Pts',(5.87110920599994,15.2,-8.58868889600001));
#168205=CARTESIAN_POINT('Ctrl Pts',(5.87186938099994,15.2,-8.58956675700002));
#168206=CARTESIAN_POINT('Ctrl Pts',(5.87263625099995,15.2,-8.59045059900001));
#168207=CARTESIAN_POINT('Ctrl Pts',(5.87340981499994,15.2,-8.59134039400002));
#168208=CARTESIAN_POINT('Ctrl Pts',(5.87419006999994,15.2,-8.59223611300001));
#168209=CARTESIAN_POINT('Ctrl Pts',(5.87497701299994,15.2,-8.59313772700002));
#168210=CARTESIAN_POINT('Ctrl Pts',(5.87577063899994,15.2,-8.59404520900002));
#168211=CARTESIAN_POINT('Ctrl Pts',(5.87657094599994,15.2,-8.59495852900002));
#168212=CARTESIAN_POINT('Ctrl Pts',(5.87737793199994,15.2,-8.59587766000002));
#168213=CARTESIAN_POINT('Ctrl Pts',(5.87819159199994,15.2,-8.59680257500001));
#168214=CARTESIAN_POINT('Ctrl Pts',(5.87901192399994,15.2,-8.59773324500001));
#168215=CARTESIAN_POINT('Ctrl Pts',(5.87983892499994,15.2,-8.59866964200002));
#168216=CARTESIAN_POINT('Ctrl Pts',(5.88067259099994,15.2,-8.59961174000002));
#168217=CARTESIAN_POINT('Ctrl Pts',(5.88151291899995,15.2,-8.60055951000002));
#168218=CARTESIAN_POINT('Ctrl Pts',(5.88235990599995,15.2,-8.60151292500002));
#168219=CARTESIAN_POINT('Ctrl Pts',(5.88321354999994,15.2,-8.60247195900002));
#168220=CARTESIAN_POINT('Ctrl Pts',(5.88407384499994,15.2,-8.60343658400001));
#168221=CARTESIAN_POINT('Ctrl Pts',(5.88494079099994,15.2,-8.60440677400002));
#168222=CARTESIAN_POINT('Ctrl Pts',(5.88581438299995,15.2,-8.60538250100002));
#168223=CARTESIAN_POINT('Ctrl Pts',(5.88669461899994,15.2,-8.60636373900002));
#168224=CARTESIAN_POINT('Ctrl Pts',(5.88758149499994,15.2,-8.60735046100002));
#168225=CARTESIAN_POINT('Ctrl Pts',(5.88847500799995,15.2,-8.60834264100001));
#168226=CARTESIAN_POINT('Ctrl Pts',(5.88937515499994,15.2,-8.60934025300002));
#168227=CARTESIAN_POINT('Ctrl Pts',(5.89028193299994,15.2,-8.61034327100001));
#168228=CARTESIAN_POINT('Ctrl Pts',(5.89119533899994,15.2,-8.61135166700001));
#168229=CARTESIAN_POINT('Ctrl Pts',(5.89211536799994,15.2,-8.61236541700002));
#168230=CARTESIAN_POINT('Ctrl Pts',(5.89304201999994,15.2,-8.61338449400002));
#168231=CARTESIAN_POINT('Ctrl Pts',(5.89397528899994,15.2,-8.61440887300001));
#168232=CARTESIAN_POINT('Ctrl Pts',(5.89491517399994,15.2,-8.61543852800001));
#168233=CARTESIAN_POINT('Ctrl Pts',(5.89586167099994,15.2,-8.61647343400002));
#168234=CARTESIAN_POINT('Ctrl Pts',(5.89681477699994,15.2,-8.61751356400001));
#168235=CARTESIAN_POINT('Ctrl Pts',(5.89777448799994,15.2,-8.61855889400001));
#168236=CARTESIAN_POINT('Ctrl Pts',(5.89874080199994,15.2,-8.61960939900002));
#168237=CARTESIAN_POINT('Ctrl Pts',(5.89971371499994,15.2,-8.62066505300002));
#168238=CARTESIAN_POINT('Ctrl Pts',(5.90069322499994,15.2,-8.62172583100002));
#168239=CARTESIAN_POINT('Ctrl Pts',(5.90167932799995,15.2,-8.62279170800001));
#168240=CARTESIAN_POINT('Ctrl Pts',(5.90267202099994,15.2,-8.62386266200001));
#168241=CARTESIAN_POINT('Ctrl Pts',(5.90367129999994,15.2,-8.62493866400002));
#168242=CARTESIAN_POINT('Ctrl Pts',(5.90467716299995,15.2,-8.62601969300002));
#168243=CARTESIAN_POINT('Ctrl Pts',(5.90568960799994,15.2,-8.62710572200001));
#168244=CARTESIAN_POINT('Ctrl Pts',(5.90670862899994,15.2,-8.62819672800001));
#168245=CARTESIAN_POINT('Ctrl Pts',(5.90773422399995,15.2,-8.62929268600002));
#168246=CARTESIAN_POINT('Ctrl Pts',(5.90876639199994,15.2,-8.63039357200002));
#168247=CARTESIAN_POINT('Ctrl Pts',(5.90980512599995,15.2,-8.63149936300001));
#168248=CARTESIAN_POINT('Ctrl Pts',(5.91085042599994,15.2,-8.63261003400002));
#168249=CARTESIAN_POINT('Ctrl Pts',(5.91190228799994,15.2,-8.63372556000002));
#168250=CARTESIAN_POINT('Ctrl Pts',(5.91296070699994,15.2,-8.63484591900002));
#168251=CARTESIAN_POINT('Ctrl Pts',(5.91402568199995,15.2,-8.63597108700001));
#168252=CARTESIAN_POINT('Ctrl Pts',(5.91509720999994,15.2,-8.63710104100001));
#168253=CARTESIAN_POINT('Ctrl Pts',(5.91617528699994,15.2,-8.63823575600002));
#168254=CARTESIAN_POINT('Ctrl Pts',(5.91725990899994,15.2,-8.63937520900001));
#168255=CARTESIAN_POINT('Ctrl Pts',(5.91835107499994,15.2,-8.64051937700001));
#168256=CARTESIAN_POINT('Ctrl Pts',(5.91944877999994,15.2,-8.64166823700002));
#168257=CARTESIAN_POINT('Ctrl Pts',(5.92055302199994,15.2,-8.64282176500001));
#168258=CARTESIAN_POINT('Ctrl Pts',(5.92166379799995,15.2,-8.64397994000001));
#168259=CARTESIAN_POINT('Ctrl Pts',(5.92278110299994,15.2,-8.64514273600001));
#168260=CARTESIAN_POINT('Ctrl Pts',(5.92390493499994,15.2,-8.64631013400002));
#168261=CARTESIAN_POINT('Ctrl Pts',(5.92503529199995,15.2,-8.64748210700002));
#168262=CARTESIAN_POINT('Ctrl Pts',(5.92617216899994,15.2,-8.64865863600001));
#168263=CARTESIAN_POINT('Ctrl Pts',(5.92731556399994,15.2,-8.64983969600001));
#168264=CARTESIAN_POINT('Ctrl Pts',(5.92846547399994,15.2,-8.65102526600002));
#168265=CARTESIAN_POINT('Ctrl Pts',(5.92962189399994,15.2,-8.65221532200002));
#168266=CARTESIAN_POINT('Ctrl Pts',(5.93078482299994,15.2,-8.65340984300002));
#168267=CARTESIAN_POINT('Ctrl Pts',(5.93195425599994,15.2,-8.65460880700001));
#168268=CARTESIAN_POINT('Ctrl Pts',(5.93313019299995,15.2,-8.65581219100001));
#168269=CARTESIAN_POINT('Ctrl Pts',(5.93431262699994,15.2,-8.65701997400001));
#168270=CARTESIAN_POINT('Ctrl Pts',(5.93550155699995,15.2,-8.65823213200001));
#168271=CARTESIAN_POINT('Ctrl Pts',(5.93669697899994,15.2,-8.65944864500002));
#168272=CARTESIAN_POINT('Ctrl Pts',(5.93789889099994,15.2,-8.66066949100002));
#168273=CARTESIAN_POINT('Ctrl Pts',(5.93910728799995,15.2,-8.66189464800001));
#168274=CARTESIAN_POINT('Ctrl Pts',(5.94032216899994,15.2,-8.66312409300001));
#168275=CARTESIAN_POINT('Ctrl Pts',(5.94154352899994,15.2,-8.66435780700002));
#168276=CARTESIAN_POINT('Ctrl Pts',(5.94277136499994,15.2,-8.66559576600002));
#168277=CARTESIAN_POINT('Ctrl Pts',(5.94400567599994,15.2,-8.66683795100002));
#168278=CARTESIAN_POINT('Ctrl Pts',(5.94524645699994,15.2,-8.66808434000001));
#168279=CARTESIAN_POINT('Ctrl Pts',(5.94649370399994,15.2,-8.66933491000001));
#168280=CARTESIAN_POINT('Ctrl Pts',(5.94774741599994,15.2,-8.67058964200002));
#168281=CARTESIAN_POINT('Ctrl Pts',(5.94900758799994,15.2,-8.67184851400001));
#168282=CARTESIAN_POINT('Ctrl Pts',(5.95027421799994,15.2,-8.67311150500001));
#168283=CARTESIAN_POINT('Ctrl Pts',(5.95154730199994,15.2,-8.67437859500002));
#168284=CARTESIAN_POINT('Ctrl Pts',(5.95282683699994,15.2,-8.67564976200002));
#168285=CARTESIAN_POINT('Ctrl Pts',(5.95411282099994,15.2,-8.67692498600002));
#168286=CARTESIAN_POINT('Ctrl Pts',(5.95540524899994,15.2,-8.67820424500002));
#168287=CARTESIAN_POINT('Ctrl Pts',(5.95670411999994,15.2,-8.67948752000002));
#168288=CARTESIAN_POINT('Ctrl Pts',(5.95800942899994,15.2,-8.68077479000002));
#168289=CARTESIAN_POINT('Ctrl Pts',(5.95932117299995,15.2,-8.68206603400001));
#168290=CARTESIAN_POINT('Ctrl Pts',(5.96063934899995,15.2,-8.68336123200002));
#168291=CARTESIAN_POINT('Ctrl Pts',(5.96196395499994,15.2,-8.68466036400001));
#168292=CARTESIAN_POINT('Ctrl Pts',(5.96329498499995,15.2,-8.68596340900002));
#168293=CARTESIAN_POINT('Ctrl Pts',(5.96463243999994,15.2,-8.68727034800001));
#168294=CARTESIAN_POINT('Ctrl Pts',(5.96597631299995,15.2,-8.68858116100002));
#168295=CARTESIAN_POINT('Ctrl Pts',(5.96732660299994,15.2,-8.68989582500001));
#168296=CARTESIAN_POINT('Ctrl Pts',(5.96868330599994,15.2,-8.69121432500001));
#168297=CARTESIAN_POINT('Ctrl Pts',(5.97004641899994,15.2,-8.69253663700002));
#168298=CARTESIAN_POINT('Ctrl Pts',(5.97141593799994,15.2,-8.69386274300001));
#168299=CARTESIAN_POINT('Ctrl Pts',(5.97279186099994,15.2,-8.69519262200001));
#168300=CARTESIAN_POINT('Ctrl Pts',(5.97417418499995,15.2,-8.69652625600001));
#168301=CARTESIAN_POINT('Ctrl Pts',(5.97556290599995,15.2,-8.69786362500001));
#168302=CARTESIAN_POINT('Ctrl Pts',(5.97695801999994,15.2,-8.69920470900002));
#168303=CARTESIAN_POINT('Ctrl Pts',(5.97835952599994,15.2,-8.70054948900002));
#168304=CARTESIAN_POINT('Ctrl Pts',(5.97976741899994,15.2,-8.70189794500002));
#168305=CARTESIAN_POINT('Ctrl Pts',(5.98118169699994,15.2,-8.70325005800002));
#168306=CARTESIAN_POINT('Ctrl Pts',(5.98260235599994,15.2,-8.70460581000001));
#168307=CARTESIAN_POINT('Ctrl Pts',(5.98402939199994,15.2,-8.70596518000001));
#168308=CARTESIAN_POINT('Ctrl Pts',(5.98546280499994,15.2,-8.70732814900002));
#168309=CARTESIAN_POINT('Ctrl Pts',(5.98690258799994,15.2,-8.70869469900001));
#168310=CARTESIAN_POINT('Ctrl Pts',(5.98834873999994,15.2,-8.71006481000002));
#168311=CARTESIAN_POINT('Ctrl Pts',(5.98980125799994,15.2,-8.71143846400001));
#168312=CARTESIAN_POINT('Ctrl Pts',(5.99126013699995,15.2,-8.71281564200002));
#168313=CARTESIAN_POINT('Ctrl Pts',(5.99272537499995,15.2,-8.71419632500002));
#168314=CARTESIAN_POINT('Ctrl Pts',(5.99419696899995,15.2,-8.71558049400001));
#168315=CARTESIAN_POINT('Ctrl Pts',(5.99567491499994,15.2,-8.71696813100002));
#168316=CARTESIAN_POINT('Ctrl Pts',(5.99715921199994,15.2,-8.71835921700002));
#168317=CARTESIAN_POINT('Ctrl Pts',(5.99864985299994,15.2,-8.71975373400002));
#168318=CARTESIAN_POINT('Ctrl Pts',(6.00014683699994,15.2,-8.72115166300001));
#168319=CARTESIAN_POINT('Ctrl Pts',(6.00165016199994,15.2,-8.72255298400002));
#168320=CARTESIAN_POINT('Ctrl Pts',(6.00315982299994,15.2,-8.72395768300001));
#168321=CARTESIAN_POINT('Ctrl Pts',(6.00467581699994,15.2,-8.72536573700001));
#168322=CARTESIAN_POINT('Ctrl Pts',(6.00619813999994,15.2,-8.72677713200002));
#168323=CARTESIAN_POINT('Ctrl Pts',(6.00772679099994,15.2,-8.72819184600001));
#168324=CARTESIAN_POINT('Ctrl Pts',(6.00926176599994,15.2,-8.72960986400001));
#168325=CARTESIAN_POINT('Ctrl Pts',(6.01080305999994,15.2,-8.73103116600002));
#168326=CARTESIAN_POINT('Ctrl Pts',(6.01235067299994,15.2,-8.73245573400002));
#168327=CARTESIAN_POINT('Ctrl Pts',(6.01390459799994,15.2,-8.73388355100002));
#168328=CARTESIAN_POINT('Ctrl Pts',(6.01546483399994,15.2,-8.73531460000001));
#168329=CARTESIAN_POINT('Ctrl Pts',(6.01703137899994,15.2,-8.73674886200002));
#168330=CARTESIAN_POINT('Ctrl Pts',(6.01860422799994,15.2,-8.73818631900001));
#168331=CARTESIAN_POINT('Ctrl Pts',(6.02018337599994,15.2,-8.73962695300002));
#168332=CARTESIAN_POINT('Ctrl Pts',(6.02176882399994,15.2,-8.74107074900002));
#168333=CARTESIAN_POINT('Ctrl Pts',(6.02336056599994,15.2,-8.74251768600002));
#168334=CARTESIAN_POINT('Ctrl Pts',(6.02495859899994,15.2,-8.74396774900001));
#168335=CARTESIAN_POINT('Ctrl Pts',(6.02656291999994,15.2,-8.74542091800001));
#168336=CARTESIAN_POINT('Ctrl Pts',(6.02817352699994,15.2,-8.74687718000001));
#168337=CARTESIAN_POINT('Ctrl Pts',(6.02979041499994,15.2,-8.74833651300002));
#168338=CARTESIAN_POINT('Ctrl Pts',(6.03141358199994,15.2,-8.74979890200001));
#168339=CARTESIAN_POINT('Ctrl Pts',(6.03304302299994,15.2,-8.75126433100002));
#168340=CARTESIAN_POINT('Ctrl Pts',(6.03467873699994,15.2,-8.75273277900002));
#168341=CARTESIAN_POINT('Ctrl Pts',(6.03632071899994,15.2,-8.75420423200002));
#168342=CARTESIAN_POINT('Ctrl Pts',(6.03796896799994,15.2,-8.75567867300001));
#168343=CARTESIAN_POINT('Ctrl Pts',(6.03962347799994,15.2,-8.75715608400002));
#168344=CARTESIAN_POINT('Ctrl Pts',(6.04128424699995,15.2,-8.75863644800001));
#168345=CARTESIAN_POINT('Ctrl Pts',(6.04295127299994,15.2,-8.76011974800001));
#168346=CARTESIAN_POINT('Ctrl Pts',(6.04462455099994,15.2,-8.76160596800002));
#168347=CARTESIAN_POINT('Ctrl Pts',(6.04630407799994,15.2,-8.76309509100002));
#168348=CARTESIAN_POINT('Ctrl Pts',(6.04798985099994,15.2,-8.76458710000002));
#168349=CARTESIAN_POINT('Ctrl Pts',(6.04968186699994,15.2,-8.76608197700002));
#168350=CARTESIAN_POINT('Ctrl Pts',(6.05138012199994,15.2,-8.76757970900002));
#168351=CARTESIAN_POINT('Ctrl Pts',(6.05308461499994,15.2,-8.76908027600001));
#168352=CARTESIAN_POINT('Ctrl Pts',(6.05479533999994,15.2,-8.77058366200002));
#168353=CARTESIAN_POINT('Ctrl Pts',(6.05651229499995,15.2,-8.77208985200001));
#168354=CARTESIAN_POINT('Ctrl Pts',(6.05823547599995,15.2,-8.77359882900001));
#168355=CARTESIAN_POINT('Ctrl Pts',(6.05996488099994,15.2,-8.77511057700002));
#168356=CARTESIAN_POINT('Ctrl Pts',(6.06170050599994,15.2,-8.77662507800002));
#168357=CARTESIAN_POINT('Ctrl Pts',(6.06344234899994,15.2,-8.77814231800001));
#168358=CARTESIAN_POINT('Ctrl Pts',(6.06519040399994,15.2,-8.77966227900002));
#168359=CARTESIAN_POINT('Ctrl Pts',(6.06694466899994,15.2,-8.78118494600002));
#168360=CARTESIAN_POINT('Ctrl Pts',(6.06870514199994,15.2,-8.78271030200001));
#168361=CARTESIAN_POINT('Ctrl Pts',(6.07047181899994,15.2,-8.78423833100002));
#168362=CARTESIAN_POINT('Ctrl Pts',(6.07224469599994,15.2,-8.78576901800002));
#168363=CARTESIAN_POINT('Ctrl Pts',(6.07402377099994,15.2,-8.78730234600001));
#168364=CARTESIAN_POINT('Ctrl Pts',(6.07580903899994,15.2,-8.78883830000002));
#168365=CARTESIAN_POINT('Ctrl Pts',(6.07760049799994,15.2,-8.79037686400002));
#168366=CARTESIAN_POINT('Ctrl Pts',(6.07939814499994,15.2,-8.79191802100001));
#168367=CARTESIAN_POINT('Ctrl Pts',(6.08120197499994,15.2,-8.79346175700002));
#168368=CARTESIAN_POINT('Ctrl Pts',(6.08301198699994,15.2,-8.79500805500001));
#168369=CARTESIAN_POINT('Ctrl Pts',(6.08482817699994,15.2,-8.79655689900002));
#168370=CARTESIAN_POINT('Ctrl Pts',(6.08665053999994,15.2,-8.79810827400001));
#168371=CARTESIAN_POINT('Ctrl Pts',(6.08847907499994,15.2,-8.79966216600002));
#168372=CARTESIAN_POINT('Ctrl Pts',(6.09031377799995,15.2,-8.80121855700001));
#168373=CARTESIAN_POINT('Ctrl Pts',(6.09215464499994,15.2,-8.80277743400002));
#168374=CARTESIAN_POINT('Ctrl Pts',(6.09400167399994,15.2,-8.80433877800002));
#168375=CARTESIAN_POINT('Ctrl Pts',(6.09585485999994,15.2,-8.80590257700002));
#168376=CARTESIAN_POINT('Ctrl Pts',(6.09771420199994,15.2,-8.80746881400002));
#168377=CARTESIAN_POINT('Ctrl Pts',(6.09957969399994,15.2,-8.80903747400002));
#168378=CARTESIAN_POINT('Ctrl Pts',(6.10145133499994,15.2,-8.81060854200001));
#168379=CARTESIAN_POINT('Ctrl Pts',(6.10332912099994,15.2,-8.81218200200001));
#168380=CARTESIAN_POINT('Ctrl Pts',(6.10521304799994,15.2,-8.81375784000002));
#168381=CARTESIAN_POINT('Ctrl Pts',(6.10710311299994,15.2,-8.81533604100002));
#168382=CARTESIAN_POINT('Ctrl Pts',(6.10899931399994,15.2,-8.81691658800002));
#168383=CARTESIAN_POINT('Ctrl Pts',(6.11090164599994,15.2,-8.81849946800001));
#168384=CARTESIAN_POINT('Ctrl Pts',(6.11281010699994,15.2,-8.82008466500002));
#168385=CARTESIAN_POINT('Ctrl Pts',(6.11472469299994,15.2,-8.82167216400001));
#168386=CARTESIAN_POINT('Ctrl Pts',(6.11664539999994,15.2,-8.82326195200001));
#168387=CARTESIAN_POINT('Ctrl Pts',(6.11857222599994,15.2,-8.82485401100002));
#168388=CARTESIAN_POINT('Ctrl Pts',(6.12050516699994,15.2,-8.82644832800001));
#168389=CARTESIAN_POINT('Ctrl Pts',(6.12244422199994,15.2,-8.82804488900002));
#168390=CARTESIAN_POINT('Ctrl Pts',(6.12438938299994,15.2,-8.82964367800002));
#168391=CARTESIAN_POINT('Ctrl Pts',(6.12634064999994,15.2,-8.83124468000002));
#168392=CARTESIAN_POINT('Ctrl Pts',(6.12829801999994,15.2,-8.83284788100001));
#168393=CARTESIAN_POINT('Ctrl Pts',(6.13026148799994,15.2,-8.83445326700001));
#168394=CARTESIAN_POINT('Ctrl Pts',(6.13223105199994,15.2,-8.83606082300001));
#168395=CARTESIAN_POINT('Ctrl Pts',(6.13420670699994,15.2,-8.83767053400002));
#168396=CARTESIAN_POINT('Ctrl Pts',(6.13618845099994,15.2,-8.83928238600001));
#168397=CARTESIAN_POINT('Ctrl Pts',(6.13817627999994,15.2,-8.84089636400001));
#168398=CARTESIAN_POINT('Ctrl Pts',(6.14017019199994,15.2,-8.84251245500002));
#168399=CARTESIAN_POINT('Ctrl Pts',(6.14217018299994,15.2,-8.84413064300002));
#168400=CARTESIAN_POINT('Ctrl Pts',(6.14417624999994,15.2,-8.84575091500002));
#168401=CARTESIAN_POINT('Ctrl Pts',(6.14618838899994,15.2,-8.84737325500002));
#168402=CARTESIAN_POINT('Ctrl Pts',(6.14820659699994,15.2,-8.84899765100002));
#168403=CARTESIAN_POINT('Ctrl Pts',(6.15023086899994,15.2,-8.85062408700002));
#168404=CARTESIAN_POINT('Ctrl Pts',(6.15226120499995,15.2,-8.85225255100002));
#168405=CARTESIAN_POINT('Ctrl Pts',(6.15429759899994,15.2,-8.85388302700001));
#168406=CARTESIAN_POINT('Ctrl Pts',(6.15634004999994,15.2,-8.85551550100002));
#168407=CARTESIAN_POINT('Ctrl Pts',(6.15838855099994,15.2,-8.85714995900001));
#168408=CARTESIAN_POINT('Ctrl Pts',(6.16044310199994,15.2,-8.85878638800002));
#168409=CARTESIAN_POINT('Ctrl Pts',(6.16250369999994,15.2,-8.86042477400002));
#168410=CARTESIAN_POINT('Ctrl Pts',(6.16457033899994,15.2,-8.86206510100001));
#168411=CARTESIAN_POINT('Ctrl Pts',(6.16664301799994,15.2,-8.86370735900002));
#168412=CARTESIAN_POINT('Ctrl Pts',(6.16872173199994,15.2,-8.86535153000001));
#168413=CARTESIAN_POINT('Ctrl Pts',(6.17080647799994,15.2,-8.86699760300001));
#168414=CARTESIAN_POINT('Ctrl Pts',(6.17289725299995,15.2,-8.86864556300001));
#168415=CARTESIAN_POINT('Ctrl Pts',(6.17499405399994,15.2,-8.87029539700002));
#168416=CARTESIAN_POINT('Ctrl Pts',(6.17709687799994,15.2,-8.87194709200001));
#168417=CARTESIAN_POINT('Ctrl Pts',(6.17920571999994,15.2,-8.87360063200001));
#168418=CARTESIAN_POINT('Ctrl Pts',(6.18132057899994,15.2,-8.87525600500001));
#168419=CARTESIAN_POINT('Ctrl Pts',(6.18344144899994,15.2,-8.87691319600002));
#168420=CARTESIAN_POINT('Ctrl Pts',(6.18556832799994,15.2,-8.87857219500002));
#168421=CARTESIAN_POINT('Ctrl Pts',(6.18770121399994,15.2,-8.88023298500002));
#168422=CARTESIAN_POINT('Ctrl Pts',(6.18984009999994,15.2,-8.88189555400002));
#168423=CARTESIAN_POINT('Ctrl Pts',(6.19198498599994,15.2,-8.88355988700001));
#168424=CARTESIAN_POINT('Ctrl Pts',(6.19413586799994,15.2,-8.88522597300001));
#168425=CARTESIAN_POINT('Ctrl Pts',(6.19629274299994,15.2,-8.88689379800002));
#168426=CARTESIAN_POINT('Ctrl Pts',(6.19845560599994,15.2,-8.88856334700002));
#168427=CARTESIAN_POINT('Ctrl Pts',(6.20062445399994,15.2,-8.89023460900002));
#168428=CARTESIAN_POINT('Ctrl Pts',(6.20279928499994,15.2,-8.89190757000001));
#168429=CARTESIAN_POINT('Ctrl Pts',(6.20498009499994,15.2,-8.89358221500002));
#168430=CARTESIAN_POINT('Ctrl Pts',(6.20716688099994,15.2,-8.89525853400002));
#168431=CARTESIAN_POINT('Ctrl Pts',(6.20935963799995,15.2,-8.89693651100002));
#168432=CARTESIAN_POINT('Ctrl Pts',(6.21155836399994,15.2,-8.89861613500001));
#168433=CARTESIAN_POINT('Ctrl Pts',(6.21376305499994,15.2,-8.90029739200001));
#168434=CARTESIAN_POINT('Ctrl Pts',(6.21597370899994,15.2,-8.90198026900002));
#168435=CARTESIAN_POINT('Ctrl Pts',(6.21819032199994,15.2,-8.90366475300001));
#168436=CARTESIAN_POINT('Ctrl Pts',(6.22041288899994,15.2,-8.90535083100002));
#168437=CARTESIAN_POINT('Ctrl Pts',(6.22264140799994,15.2,-8.90703849100002));
#168438=CARTESIAN_POINT('Ctrl Pts',(6.22487587699994,15.2,-8.90872771900002));
#168439=CARTESIAN_POINT('Ctrl Pts',(6.22711629099994,15.2,-8.91041850200001));
#168440=CARTESIAN_POINT('Ctrl Pts',(6.22936264599994,15.2,-8.91211082700002));
#168441=CARTESIAN_POINT('Ctrl Pts',(6.23161493899994,15.2,-8.91380468300002));
#168442=CARTESIAN_POINT('Ctrl Pts',(6.23387316899994,15.2,-8.91550005600001));
#168443=CARTESIAN_POINT('Ctrl Pts',(6.23613732999994,15.2,-8.91719693300002));
#168444=CARTESIAN_POINT('Ctrl Pts',(6.23840741799994,15.2,-8.91889530200002));
#168445=CARTESIAN_POINT('Ctrl Pts',(6.24068343299994,15.2,-8.92059515000001));
#168446=CARTESIAN_POINT('Ctrl Pts',(6.24296536899994,15.2,-8.92229646500001));
#168447=CARTESIAN_POINT('Ctrl Pts',(6.24525322299994,15.2,-8.92399923300001));
#168448=CARTESIAN_POINT('Ctrl Pts',(6.24754699199994,15.2,-8.92570344200001));
#168449=CARTESIAN_POINT('Ctrl Pts',(6.24984667299994,15.2,-8.92740908100001));
#168450=CARTESIAN_POINT('Ctrl Pts',(6.25215226099994,15.2,-8.92911613600001));
#168451=CARTESIAN_POINT('Ctrl Pts',(6.25446375499994,15.2,-8.93082459400001));
#168452=CARTESIAN_POINT('Ctrl Pts',(6.25678114899994,15.2,-8.93253444400001));
#168453=CARTESIAN_POINT('Ctrl Pts',(6.25910444299994,15.2,-8.93424567300002));
#168454=CARTESIAN_POINT('Ctrl Pts',(6.26143362999994,15.2,-8.93595826800002));
#168455=CARTESIAN_POINT('Ctrl Pts',(6.26376870799994,15.2,-8.93767221800001));
#168456=CARTESIAN_POINT('Ctrl Pts',(6.26610967499994,15.2,-8.93938751000002));
#168457=CARTESIAN_POINT('Ctrl Pts',(6.26845652499994,15.2,-8.94110413200002));
#168458=CARTESIAN_POINT('Ctrl Pts',(6.27080925699994,15.2,-8.94282207100002));
#168459=CARTESIAN_POINT('Ctrl Pts',(6.27316786699994,15.2,-8.94454131600002));
#168460=CARTESIAN_POINT('Ctrl Pts',(6.27553235099994,15.2,-8.94626185400002));
#168461=CARTESIAN_POINT('Ctrl Pts',(6.27790270499994,15.2,-8.94798367200002));
#168462=CARTESIAN_POINT('Ctrl Pts',(6.28027892799994,15.2,-8.94970676000002));
#168463=CARTESIAN_POINT('Ctrl Pts',(6.28266101299994,15.2,-8.95143110400002));
#168464=CARTESIAN_POINT('Ctrl Pts',(6.28504895899994,15.2,-8.95315669400001));
#168465=CARTESIAN_POINT('Ctrl Pts',(6.28744276399994,15.2,-8.95488351500001));
#168466=CARTESIAN_POINT('Ctrl Pts',(6.28984242199994,15.2,-8.95661155900001));
#168467=CARTESIAN_POINT('Ctrl Pts',(6.29224792999994,15.2,-8.95834081000002));
#168468=CARTESIAN_POINT('Ctrl Pts',(6.29465928599994,15.2,-8.96007125900002));
#168469=CARTESIAN_POINT('Ctrl Pts',(6.29707648499994,15.2,-8.96180289200002));
#168470=CARTESIAN_POINT('Ctrl Pts',(6.29949952399994,15.2,-8.96353569800001));
#168471=CARTESIAN_POINT('Ctrl Pts',(6.30192839999994,15.2,-8.96526966600002));
#168472=CARTESIAN_POINT('Ctrl Pts',(6.30436310999994,15.2,-8.96700478300002));
#168473=CARTESIAN_POINT('Ctrl Pts',(6.30680364899994,15.2,-8.96874103900002));
#168474=CARTESIAN_POINT('Ctrl Pts',(6.30925001499994,15.2,-8.97047842000001));
#168475=CARTESIAN_POINT('Ctrl Pts',(6.31170220399994,15.2,-8.97221691500001));
#168476=CARTESIAN_POINT('Ctrl Pts',(6.31416021399994,15.2,-8.97395651300002));
#168477=CARTESIAN_POINT('Ctrl Pts',(6.31662403899994,15.2,-8.97569720100002));
#168478=CARTESIAN_POINT('Ctrl Pts',(6.31909367699994,15.2,-8.97743896900002));
#168479=CARTESIAN_POINT('Ctrl Pts',(6.32156912499994,15.2,-8.97918180400002));
#168480=CARTESIAN_POINT('Ctrl Pts',(6.32405037899994,15.2,-8.98092569600001));
#168481=CARTESIAN_POINT('Ctrl Pts',(6.32653743599994,15.2,-8.98267063100001));
#168482=CARTESIAN_POINT('Ctrl Pts',(6.32903029199994,15.2,-8.98441660100002));
#168483=CARTESIAN_POINT('Ctrl Pts',(6.33152894299994,15.2,-8.98616359100001));
#168484=CARTESIAN_POINT('Ctrl Pts',(6.33403338799994,15.2,-8.98791159100002));
#168485=CARTESIAN_POINT('Ctrl Pts',(6.33654362099994,15.2,-8.98966059000001));
#168486=CARTESIAN_POINT('Ctrl Pts',(6.33905963999994,15.2,-8.99141057600002));
#168487=CARTESIAN_POINT('Ctrl Pts',(6.34158143999994,15.2,-8.99316153900001));
#168488=CARTESIAN_POINT('Ctrl Pts',(6.34410901999994,15.2,-8.99491346500002));
#168489=CARTESIAN_POINT('Ctrl Pts',(6.34664237499994,15.2,-8.99666634500001));
#168490=CARTESIAN_POINT('Ctrl Pts',(6.34918150099994,15.2,-8.99842016600001));
#168491=CARTESIAN_POINT('Ctrl Pts',(6.35172639699994,15.2,-9.00017491800002));
#168492=CARTESIAN_POINT('Ctrl Pts',(6.35427705599994,15.2,-9.00193058900001));
#168493=CARTESIAN_POINT('Ctrl Pts',(6.35683347799994,15.2,-9.00368716800001));
#168494=CARTESIAN_POINT('Ctrl Pts',(6.35939565699994,15.2,-9.00544464400001));
#168495=CARTESIAN_POINT('Ctrl Pts',(6.36196359199994,15.2,-9.00720300600002));
#168496=CARTESIAN_POINT('Ctrl Pts',(6.36453727799994,15.2,-9.00896224300002));
#168497=CARTESIAN_POINT('Ctrl Pts',(6.36711671099994,15.2,-9.01072234300001));
#168498=CARTESIAN_POINT('Ctrl Pts',(6.36970188799994,15.2,-9.01248329400002));
#168499=CARTESIAN_POINT('Ctrl Pts',(6.37229280699994,15.2,-9.01424508800002));
#168500=CARTESIAN_POINT('Ctrl Pts',(6.37488946299994,15.2,-9.01600771300001));
#168501=CARTESIAN_POINT('Ctrl Pts',(6.37749185299994,15.2,-9.01777115600002));
#168502=CARTESIAN_POINT('Ctrl Pts',(6.38009997299994,15.2,-9.01953540700001));
#168503=CARTESIAN_POINT('Ctrl Pts',(6.38271382099994,15.2,-9.02130045600002));
#168504=CARTESIAN_POINT('Ctrl Pts',(6.38533339199994,15.2,-9.02306629200002));
#168505=CARTESIAN_POINT('Ctrl Pts',(6.38795868399994,15.2,-9.02483290300001));
#168506=CARTESIAN_POINT('Ctrl Pts',(6.39058969199994,15.2,-9.02660027900002));
#168507=CARTESIAN_POINT('Ctrl Pts',(6.39322641399994,15.2,-9.02836840800001));
#168508=CARTESIAN_POINT('Ctrl Pts',(6.39586884499994,15.2,-9.03013728200002));
#168509=CARTESIAN_POINT('Ctrl Pts',(6.39851698299994,15.2,-9.03190688700001));
#168510=CARTESIAN_POINT('Ctrl Pts',(6.40117082299994,15.2,-9.03367721300001));
#168511=CARTESIAN_POINT('Ctrl Pts',(6.40383036299994,15.2,-9.03544825000001));
#168512=CARTESIAN_POINT('Ctrl Pts',(6.40649559999994,15.2,-9.03721998700002));
#168513=CARTESIAN_POINT('Ctrl Pts',(6.40916652899994,15.2,-9.03899241300002));
#168514=CARTESIAN_POINT('Ctrl Pts',(6.41184314599994,15.2,-9.04076551800001));
#168515=CARTESIAN_POINT('Ctrl Pts',(6.41452544999994,15.2,-9.04253929100001));
#168516=CARTESIAN_POINT('Ctrl Pts',(6.41721343599994,15.2,-9.04431372100002));
#168517=CARTESIAN_POINT('Ctrl Pts',(6.41990709999994,15.2,-9.04608879800002));
#168518=CARTESIAN_POINT('Ctrl Pts',(6.42260643999994,15.2,-9.04786451100002));
#168519=CARTESIAN_POINT('Ctrl Pts',(6.42531145199994,15.2,-9.04964084900002));
#168520=CARTESIAN_POINT('Ctrl Pts',(6.42802213199994,15.2,-9.05141780400001));
#168521=CARTESIAN_POINT('Ctrl Pts',(6.43073847599994,15.2,-9.05319536200002));
#168522=CARTESIAN_POINT('Ctrl Pts',(6.43346048199994,15.2,-9.05497351500001));
#168523=CARTESIAN_POINT('Ctrl Pts',(6.43618814599995,15.2,-9.05675225100002));
#168524=CARTESIAN_POINT('Ctrl Pts',(6.43892146399994,15.2,-9.05853156000001));
#168525=CARTESIAN_POINT('Ctrl Pts',(6.44166043299994,15.2,-9.06031143300002));
#168526=CARTESIAN_POINT('Ctrl Pts',(6.44440504999994,15.2,-9.06209185800002));
#168527=CARTESIAN_POINT('Ctrl Pts',(6.44715531099994,15.2,-9.06387282500001));
#168528=CARTESIAN_POINT('Ctrl Pts',(6.44991121199994,15.2,-9.06565432300001));
#168529=CARTESIAN_POINT('Ctrl Pts',(6.45267274999994,15.2,-9.06743634400001));
#168530=CARTESIAN_POINT('Ctrl Pts',(6.45543992299994,15.2,-9.06921887500001));
#168531=CARTESIAN_POINT('Ctrl Pts',(6.45821272399994,15.2,-9.07100190800002));
#168532=CARTESIAN_POINT('Ctrl Pts',(6.46099115299994,15.2,-9.07278543100002));
#168533=CARTESIAN_POINT('Ctrl Pts',(6.46377520499994,15.2,-9.07456943400001));
#168534=CARTESIAN_POINT('Ctrl Pts',(6.46656487599994,15.2,-9.07635390800002));
#168535=CARTESIAN_POINT('Ctrl Pts',(6.46936016299994,15.2,-9.07813884200002));
#168536=CARTESIAN_POINT('Ctrl Pts',(6.47216106399994,15.2,-9.07992422500002));
#168537=CARTESIAN_POINT('Ctrl Pts',(6.47496757199994,15.2,-9.08171004900002));
#168538=CARTESIAN_POINT('Ctrl Pts',(6.47777968799994,15.2,-9.08349630400001));
#168539=CARTESIAN_POINT('Ctrl Pts',(6.48059740499994,15.2,-9.08528297600002));
#168540=CARTESIAN_POINT('Ctrl Pts',(6.48342072099994,15.2,-9.08707005900002));
#168541=CARTESIAN_POINT('Ctrl Pts',(6.48624963199994,15.2,-9.08885754100002));
#168542=CARTESIAN_POINT('Ctrl Pts',(6.48908413499994,15.2,-9.09064541400002));
#168543=CARTESIAN_POINT('Ctrl Pts',(6.49192422599994,15.2,-9.09243366500002));
#168544=CARTESIAN_POINT('Ctrl Pts',(6.49476990199994,15.2,-9.09422228700001));
#168545=CARTESIAN_POINT('Ctrl Pts',(6.49762115899994,15.2,-9.09601126700002));
#168546=CARTESIAN_POINT('Ctrl Pts',(6.50047799399994,15.2,-9.09780059800001));
#168547=CARTESIAN_POINT('Ctrl Pts',(6.50334040299994,15.2,-9.09959026900001));
#168548=CARTESIAN_POINT('Ctrl Pts',(6.50620838199995,15.2,-9.10138026900002));
#168549=CARTESIAN_POINT('Ctrl Pts',(6.50908192999994,15.2,-9.10317059000001));
#168550=CARTESIAN_POINT('Ctrl Pts',(6.51196104099995,15.2,-9.10496122100002));
#168551=CARTESIAN_POINT('Ctrl Pts',(6.51484571099994,15.2,-9.10675215300002));
#168552=CARTESIAN_POINT('Ctrl Pts',(6.51773593899994,15.2,-9.10854337500002));
#168553=CARTESIAN_POINT('Ctrl Pts',(6.52063172099994,15.2,-9.11033487800001));
#168554=CARTESIAN_POINT('Ctrl Pts',(6.52353305099994,15.2,-9.11212665200001));
#168555=CARTESIAN_POINT('Ctrl Pts',(6.52643992799994,15.2,-9.11391868900001));
#168556=CARTESIAN_POINT('Ctrl Pts',(6.52935234699994,15.2,-9.11571097500002));
#168557=CARTESIAN_POINT('Ctrl Pts',(6.53227030599994,15.2,-9.11750350600002));
#168558=CARTESIAN_POINT('Ctrl Pts',(6.53519379999994,15.2,-9.11929626800001));
#168559=CARTESIAN_POINT('Ctrl Pts',(6.53812282699994,15.2,-9.12108925300002));
#168560=CARTESIAN_POINT('Ctrl Pts',(6.54105738299994,15.2,-9.12288245200001));
#168561=CARTESIAN_POINT('Ctrl Pts',(6.54399746299994,15.2,-9.12467585300002));
#168562=CARTESIAN_POINT('Ctrl Pts',(6.54694306499994,15.2,-9.12646944900001));
#168563=CARTESIAN_POINT('Ctrl Pts',(6.54989418399994,15.2,-9.12826322900001));
#168564=CARTESIAN_POINT('Ctrl Pts',(6.55285081899994,15.2,-9.13005718400001));
#168565=CARTESIAN_POINT('Ctrl Pts',(6.55581296599994,15.2,-9.13185130500001));
#168566=CARTESIAN_POINT('Ctrl Pts',(6.55878061899994,15.2,-9.13364558100002));
#168567=CARTESIAN_POINT('Ctrl Pts',(6.56175377599994,15.2,-9.13544000400002));
#168568=CARTESIAN_POINT('Ctrl Pts',(6.56473243399994,15.2,-9.13723456500002));
#168569=CARTESIAN_POINT('Ctrl Pts',(6.56771658899994,15.2,-9.13902925200002));
#168570=CARTESIAN_POINT('Ctrl Pts',(6.57070623699994,15.2,-9.14082405700002));
#168571=CARTESIAN_POINT('Ctrl Pts',(6.57370137599994,15.2,-9.14261897200002));
#168572=CARTESIAN_POINT('Ctrl Pts',(6.57670199999994,15.2,-9.14441398600001));
#168573=CARTESIAN_POINT('Ctrl Pts',(6.57970810799994,15.2,-9.14620908900002));
#168574=CARTESIAN_POINT('Ctrl Pts',(6.58271969499994,15.2,-9.14800427400002));
#168575=CARTESIAN_POINT('Ctrl Pts',(6.58573675799994,15.2,-9.14979953100002));
#168576=CARTESIAN_POINT('Ctrl Pts',(6.58875929299994,15.2,-9.15159484900002));
#168577=CARTESIAN_POINT('Ctrl Pts',(6.59178729699994,15.2,-9.15339022000002));
#168578=CARTESIAN_POINT('Ctrl Pts',(6.59482076499994,15.2,-9.15518563400001));
#168579=CARTESIAN_POINT('Ctrl Pts',(6.59785969599994,15.2,-9.15698108300001));
#168580=CARTESIAN_POINT('Ctrl Pts',(6.60090408599994,15.2,-9.15877655700001));
#168581=CARTESIAN_POINT('Ctrl Pts',(6.60395392899995,15.2,-9.16057204700002));
#168582=CARTESIAN_POINT('Ctrl Pts',(6.60700922399994,15.2,-9.16236754400002));
#168583=CARTESIAN_POINT('Ctrl Pts',(6.61006996599995,15.2,-9.16416303900002));
#168584=CARTESIAN_POINT('Ctrl Pts',(6.61313615199994,15.2,-9.16595852100002));
#168585=CARTESIAN_POINT('Ctrl Pts',(6.61620777899994,15.2,-9.16775398400001));
#168586=CARTESIAN_POINT('Ctrl Pts',(6.61928484299994,15.2,-9.16954941700002));
#168587=CARTESIAN_POINT('Ctrl Pts',(6.62236733999994,15.2,-9.17134481100002));
#168588=CARTESIAN_POINT('Ctrl Pts',(6.62545526699994,15.2,-9.17314015600001));
#168589=CARTESIAN_POINT('Ctrl Pts',(6.62854862099994,15.2,-9.17493544700001));
#168590=CARTESIAN_POINT('Ctrl Pts',(6.63164739699994,15.2,-9.17673067000001));
#168591=CARTESIAN_POINT('Ctrl Pts',(6.63475159199994,15.2,-9.17852581800001));
#168592=CARTESIAN_POINT('Ctrl Pts',(6.63786120299994,15.2,-9.18032088200002));
#168593=CARTESIAN_POINT('Ctrl Pts',(6.64097622599994,15.2,-9.18211585500002));
#168594=CARTESIAN_POINT('Ctrl Pts',(6.64409665799995,15.2,-9.18391072500001));
#168595=CARTESIAN_POINT('Ctrl Pts',(6.64722249499994,15.2,-9.18570548400002));
#168596=CARTESIAN_POINT('Ctrl Pts',(6.65035373299995,15.2,-9.18750012300002));
#168597=CARTESIAN_POINT('Ctrl Pts',(6.65349036899994,15.2,-9.18929463500002));
#168598=CARTESIAN_POINT('Ctrl Pts',(6.65663239999994,15.2,-9.19108900900002));
#168599=CARTESIAN_POINT('Ctrl Pts',(6.65977982099994,15.2,-9.19288323700002));
#168600=CARTESIAN_POINT('Ctrl Pts',(6.66293262999995,15.2,-9.19467731100001));
#168601=CARTESIAN_POINT('Ctrl Pts',(6.66609082299995,15.2,-9.19647121900002));
#168602=CARTESIAN_POINT('Ctrl Pts',(6.66925439499994,15.2,-9.19826495600002));
#168603=CARTESIAN_POINT('Ctrl Pts',(6.67242334399995,15.2,-9.20005851000001));
#168604=CARTESIAN_POINT('Ctrl Pts',(6.67559766699994,15.2,-9.20185187500002));
#168605=CARTESIAN_POINT('Ctrl Pts',(6.67877735899994,15.2,-9.20364504200002));
#168606=CARTESIAN_POINT('Ctrl Pts',(6.68196241599994,15.2,-9.20543800000001));
#168607=CARTESIAN_POINT('Ctrl Pts',(6.68515283699994,15.2,-9.20723074200002));
#168608=CARTESIAN_POINT('Ctrl Pts',(6.68834861499994,15.2,-9.20902325900002));
#168609=CARTESIAN_POINT('Ctrl Pts',(6.69154974999994,15.2,-9.21081554300001));
#168610=CARTESIAN_POINT('Ctrl Pts',(6.69475623599994,15.2,-9.21260758400001));
#168611=CARTESIAN_POINT('Ctrl Pts',(6.69796806999994,15.2,-9.21439937500002));
#168612=CARTESIAN_POINT('Ctrl Pts',(6.70118524799994,15.2,-9.21619090500002));
#168613=CARTESIAN_POINT('Ctrl Pts',(6.70440776799994,15.2,-9.21798216800001));
#168614=CARTESIAN_POINT('Ctrl Pts',(6.70763562499994,15.2,-9.21977315400002));
#168615=CARTESIAN_POINT('Ctrl Pts',(6.71086881499994,15.2,-9.22156385400001));
#168616=CARTESIAN_POINT('Ctrl Pts',(6.71410733699994,15.2,-9.22335426000001));
#168617=CARTESIAN_POINT('Ctrl Pts',(6.71735118499994,15.2,-9.22514436400002));
#168618=CARTESIAN_POINT('Ctrl Pts',(6.72060035499995,15.2,-9.22693415700002));
#168619=CARTESIAN_POINT('Ctrl Pts',(6.72385484599994,15.2,-9.22872363200002));
#168620=CARTESIAN_POINT('Ctrl Pts',(6.72711465299995,15.2,-9.23051277900001));
#168621=CARTESIAN_POINT('Ctrl Pts',(6.73037977199994,15.2,-9.23230159000001));
#168622=CARTESIAN_POINT('Ctrl Pts',(6.73365020099994,15.2,-9.23409005700002));
#168623=CARTESIAN_POINT('Ctrl Pts',(6.73692593399994,15.2,-9.23587817000002));
#168624=CARTESIAN_POINT('Ctrl Pts',(6.74020696799994,15.2,-9.23766592000002));
#168625=CARTESIAN_POINT('Ctrl Pts',(6.74349330199994,15.2,-9.23945330000001));
#168626=CARTESIAN_POINT('Ctrl Pts',(6.74678492799995,15.2,-9.24124030000002));
#168627=CARTESIAN_POINT('Ctrl Pts',(6.75008184499994,15.2,-9.24302691400002));
#168628=CARTESIAN_POINT('Ctrl Pts',(6.75338404999994,15.2,-9.24481313200002));
#168629=CARTESIAN_POINT('Ctrl Pts',(6.75669153899995,15.2,-9.24659894800002));
#168630=CARTESIAN_POINT('Ctrl Pts',(6.76000430999994,15.2,-9.24838435500002));
#168631=CARTESIAN_POINT('Ctrl Pts',(6.76332235699994,15.2,-9.25016934500002));
#168632=CARTESIAN_POINT('Ctrl Pts',(6.76664567999994,15.2,-9.25195390800001));
#168633=CARTESIAN_POINT('Ctrl Pts',(6.76997427099994,15.2,-9.25373803600002));
#168634=CARTESIAN_POINT('Ctrl Pts',(6.77330812799994,15.2,-9.25552171800001));
#168635=CARTESIAN_POINT('Ctrl Pts',(6.77664724599994,15.2,-9.25730494300002));
#168636=CARTESIAN_POINT('Ctrl Pts',(6.77999162099994,15.2,-9.25908770200002));
#168637=CARTESIAN_POINT('Ctrl Pts',(6.78334124799994,15.2,-9.26086998700002));
#168638=CARTESIAN_POINT('Ctrl Pts',(6.78669612399994,15.2,-9.26265178800002));
#168639=CARTESIAN_POINT('Ctrl Pts',(6.79005624699994,15.2,-9.26443310200002));
#168640=CARTESIAN_POINT('Ctrl Pts',(6.79342161599994,15.2,-9.26621392500002));
#168641=CARTESIAN_POINT('Ctrl Pts',(6.79679222899994,15.2,-9.26799425300001));
#168642=CARTESIAN_POINT('Ctrl Pts',(6.79949291499995,15.2,-9.26941812000001));
#168643=CARTESIAN_POINT('Ctrl Pts',(6.80152078799994,15.2,-9.27048579800001));
#168644=CARTESIAN_POINT('Ctrl Pts',(6.80287375199994,15.2,-9.27119748400001));
#168645=CARTESIAN_POINT('Ctrl Pts',(6.80355049599994,15.2,-9.27155330300002));
#168646=CARTESIAN_POINT('Ctrl Pts',(5.85257411399994,12.2,-8.56667970900002));
#168647=CARTESIAN_POINT('Ctrl Pts',(5.85268447799995,12.2,-8.56681469200002));
#168648=CARTESIAN_POINT('Ctrl Pts',(5.85290912899994,12.2,-8.56708931800001));
#168649=CARTESIAN_POINT('Ctrl Pts',(5.85324973299994,12.2,-8.56750527300001));
#168650=CARTESIAN_POINT('Ctrl Pts',(5.85370897399994,12.2,-8.56806526100002));
#168651=CARTESIAN_POINT('Ctrl Pts',(5.85429055399994,12.2,-8.56877298400001));
#168652=CARTESIAN_POINT('Ctrl Pts',(5.85488228099995,12.2,-8.56949158200001));
#168653=CARTESIAN_POINT('Ctrl Pts',(5.85548078499994,12.2,-8.57021692600001));
#168654=CARTESIAN_POINT('Ctrl Pts',(5.85608606099995,12.2,-8.57094898200002));
#168655=CARTESIAN_POINT('Ctrl Pts',(5.85669810699994,12.2,-8.57168771800002));
#168656=CARTESIAN_POINT('Ctrl Pts',(5.85731691799994,12.2,-8.57243310300002));
#168657=CARTESIAN_POINT('Ctrl Pts',(5.85794249299994,12.2,-8.57318510400002));
#168658=CARTESIAN_POINT('Ctrl Pts',(5.85857482799995,12.2,-8.57394368900002));
#168659=CARTESIAN_POINT('Ctrl Pts',(5.85921391899995,12.2,-8.57470882600002));
#168660=CARTESIAN_POINT('Ctrl Pts',(5.85985976499994,12.2,-8.57548048600002));
#168661=CARTESIAN_POINT('Ctrl Pts',(5.86051236099995,12.2,-8.57625863500001));
#168662=CARTESIAN_POINT('Ctrl Pts',(5.86117170399994,12.2,-8.57704324400002));
#168663=CARTESIAN_POINT('Ctrl Pts',(5.86183779199994,12.2,-8.57783428100002));
#168664=CARTESIAN_POINT('Ctrl Pts',(5.86251061899994,12.2,-8.57863171400002));
#168665=CARTESIAN_POINT('Ctrl Pts',(5.86319018499994,12.2,-8.57943551500002));
#168666=CARTESIAN_POINT('Ctrl Pts',(5.86387648599994,12.2,-8.58024565100001));
#168667=CARTESIAN_POINT('Ctrl Pts',(5.86456951799994,12.2,-8.58106209400002));
#168668=CARTESIAN_POINT('Ctrl Pts',(5.86526927899994,12.2,-8.58188481300001));
#168669=CARTESIAN_POINT('Ctrl Pts',(5.86597576599994,12.2,-8.58271377600002));
#168670=CARTESIAN_POINT('Ctrl Pts',(5.86668897299995,12.2,-8.58354895500002));
#168671=CARTESIAN_POINT('Ctrl Pts',(5.86740889999994,12.2,-8.58439031900001));
#168672=CARTESIAN_POINT('Ctrl Pts',(5.86813554199995,12.2,-8.58523784000001));
#168673=CARTESIAN_POINT('Ctrl Pts',(5.86886889699994,12.2,-8.58609148700002));
#168674=CARTESIAN_POINT('Ctrl Pts',(5.86960896099994,12.2,-8.58695123200001));
#168675=CARTESIAN_POINT('Ctrl Pts',(5.87035573299994,12.2,-8.58781704500002));
#168676=CARTESIAN_POINT('Ctrl Pts',(5.87110920599994,12.2,-8.58868889600001));
#168677=CARTESIAN_POINT('Ctrl Pts',(5.87186938099994,12.2,-8.58956675700002));
#168678=CARTESIAN_POINT('Ctrl Pts',(5.87263625099995,12.2,-8.59045059900001));
#168679=CARTESIAN_POINT('Ctrl Pts',(5.87340981499994,12.2,-8.59134039400002));
#168680=CARTESIAN_POINT('Ctrl Pts',(5.87419006999994,12.2,-8.59223611300001));
#168681=CARTESIAN_POINT('Ctrl Pts',(5.87497701299994,12.2,-8.59313772700002));
#168682=CARTESIAN_POINT('Ctrl Pts',(5.87577063899994,12.2,-8.59404520900002));
#168683=CARTESIAN_POINT('Ctrl Pts',(5.87657094599994,12.2,-8.59495852900002));
#168684=CARTESIAN_POINT('Ctrl Pts',(5.87737793199994,12.2,-8.59587766000002));
#168685=CARTESIAN_POINT('Ctrl Pts',(5.87819159199994,12.2,-8.59680257500001));
#168686=CARTESIAN_POINT('Ctrl Pts',(5.87901192399994,12.2,-8.59773324500001));
#168687=CARTESIAN_POINT('Ctrl Pts',(5.87983892499994,12.2,-8.59866964200002));
#168688=CARTESIAN_POINT('Ctrl Pts',(5.88067259099994,12.2,-8.59961174000002));
#168689=CARTESIAN_POINT('Ctrl Pts',(5.88151291899995,12.2,-8.60055951000002));
#168690=CARTESIAN_POINT('Ctrl Pts',(5.88235990599995,12.2,-8.60151292500002));
#168691=CARTESIAN_POINT('Ctrl Pts',(5.88321354999994,12.2,-8.60247195900002));
#168692=CARTESIAN_POINT('Ctrl Pts',(5.88407384499994,12.2,-8.60343658400001));
#168693=CARTESIAN_POINT('Ctrl Pts',(5.88494079099994,12.2,-8.60440677400002));
#168694=CARTESIAN_POINT('Ctrl Pts',(5.88581438299995,12.2,-8.60538250100002));
#168695=CARTESIAN_POINT('Ctrl Pts',(5.88669461899994,12.2,-8.60636373900002));
#168696=CARTESIAN_POINT('Ctrl Pts',(5.88758149499994,12.2,-8.60735046100002));
#168697=CARTESIAN_POINT('Ctrl Pts',(5.88847500799995,12.2,-8.60834264100001));
#168698=CARTESIAN_POINT('Ctrl Pts',(5.88937515499994,12.2,-8.60934025300002));
#168699=CARTESIAN_POINT('Ctrl Pts',(5.89028193299994,12.2,-8.61034327100001));
#168700=CARTESIAN_POINT('Ctrl Pts',(5.89119533899994,12.2,-8.61135166700001));
#168701=CARTESIAN_POINT('Ctrl Pts',(5.89211536799994,12.2,-8.61236541700002));
#168702=CARTESIAN_POINT('Ctrl Pts',(5.89304201999994,12.2,-8.61338449400002));
#168703=CARTESIAN_POINT('Ctrl Pts',(5.89397528899994,12.2,-8.61440887300001));
#168704=CARTESIAN_POINT('Ctrl Pts',(5.89491517399994,12.2,-8.61543852800001));
#168705=CARTESIAN_POINT('Ctrl Pts',(5.89586167099994,12.2,-8.61647343400002));
#168706=CARTESIAN_POINT('Ctrl Pts',(5.89681477699994,12.2,-8.61751356400001));
#168707=CARTESIAN_POINT('Ctrl Pts',(5.89777448799994,12.2,-8.61855889400001));
#168708=CARTESIAN_POINT('Ctrl Pts',(5.89874080199994,12.2,-8.61960939900002));
#168709=CARTESIAN_POINT('Ctrl Pts',(5.89971371499994,12.2,-8.62066505300002));
#168710=CARTESIAN_POINT('Ctrl Pts',(5.90069322499994,12.2,-8.62172583100002));
#168711=CARTESIAN_POINT('Ctrl Pts',(5.90167932799995,12.2,-8.62279170800001));
#168712=CARTESIAN_POINT('Ctrl Pts',(5.90267202099994,12.2,-8.62386266200001));
#168713=CARTESIAN_POINT('Ctrl Pts',(5.90367129999994,12.2,-8.62493866400002));
#168714=CARTESIAN_POINT('Ctrl Pts',(5.90467716299995,12.2,-8.62601969300002));
#168715=CARTESIAN_POINT('Ctrl Pts',(5.90568960799994,12.2,-8.62710572200001));
#168716=CARTESIAN_POINT('Ctrl Pts',(5.90670862899994,12.2,-8.62819672800001));
#168717=CARTESIAN_POINT('Ctrl Pts',(5.90773422399995,12.2,-8.62929268600002));
#168718=CARTESIAN_POINT('Ctrl Pts',(5.90876639199994,12.2,-8.63039357200002));
#168719=CARTESIAN_POINT('Ctrl Pts',(5.90980512599995,12.2,-8.63149936300001));
#168720=CARTESIAN_POINT('Ctrl Pts',(5.91085042599994,12.2,-8.63261003400002));
#168721=CARTESIAN_POINT('Ctrl Pts',(5.91190228799994,12.2,-8.63372556000002));
#168722=CARTESIAN_POINT('Ctrl Pts',(5.91296070699994,12.2,-8.63484591900002));
#168723=CARTESIAN_POINT('Ctrl Pts',(5.91402568199995,12.2,-8.63597108700001));
#168724=CARTESIAN_POINT('Ctrl Pts',(5.91509720999994,12.2,-8.63710104100001));
#168725=CARTESIAN_POINT('Ctrl Pts',(5.91617528699994,12.2,-8.63823575600002));
#168726=CARTESIAN_POINT('Ctrl Pts',(5.91725990899994,12.2,-8.63937520900001));
#168727=CARTESIAN_POINT('Ctrl Pts',(5.91835107499994,12.2,-8.64051937700001));
#168728=CARTESIAN_POINT('Ctrl Pts',(5.91944877999994,12.2,-8.64166823700002));
#168729=CARTESIAN_POINT('Ctrl Pts',(5.92055302199994,12.2,-8.64282176500001));
#168730=CARTESIAN_POINT('Ctrl Pts',(5.92166379799995,12.2,-8.64397994000001));
#168731=CARTESIAN_POINT('Ctrl Pts',(5.92278110299994,12.2,-8.64514273600001));
#168732=CARTESIAN_POINT('Ctrl Pts',(5.92390493499994,12.2,-8.64631013400002));
#168733=CARTESIAN_POINT('Ctrl Pts',(5.92503529199995,12.2,-8.64748210700002));
#168734=CARTESIAN_POINT('Ctrl Pts',(5.92617216899994,12.2,-8.64865863600001));
#168735=CARTESIAN_POINT('Ctrl Pts',(5.92731556399994,12.2,-8.64983969600001));
#168736=CARTESIAN_POINT('Ctrl Pts',(5.92846547399994,12.2,-8.65102526600002));
#168737=CARTESIAN_POINT('Ctrl Pts',(5.92962189399994,12.2,-8.65221532200002));
#168738=CARTESIAN_POINT('Ctrl Pts',(5.93078482299994,12.2,-8.65340984300002));
#168739=CARTESIAN_POINT('Ctrl Pts',(5.93195425599994,12.2,-8.65460880700001));
#168740=CARTESIAN_POINT('Ctrl Pts',(5.93313019299995,12.2,-8.65581219100001));
#168741=CARTESIAN_POINT('Ctrl Pts',(5.93431262699994,12.2,-8.65701997400001));
#168742=CARTESIAN_POINT('Ctrl Pts',(5.93550155699995,12.2,-8.65823213200001));
#168743=CARTESIAN_POINT('Ctrl Pts',(5.93669697899994,12.2,-8.65944864500002));
#168744=CARTESIAN_POINT('Ctrl Pts',(5.93789889099994,12.2,-8.66066949100002));
#168745=CARTESIAN_POINT('Ctrl Pts',(5.93910728799995,12.2,-8.66189464800001));
#168746=CARTESIAN_POINT('Ctrl Pts',(5.94032216899994,12.2,-8.66312409300001));
#168747=CARTESIAN_POINT('Ctrl Pts',(5.94154352899994,12.2,-8.66435780700002));
#168748=CARTESIAN_POINT('Ctrl Pts',(5.94277136499994,12.2,-8.66559576600002));
#168749=CARTESIAN_POINT('Ctrl Pts',(5.94400567599994,12.2,-8.66683795100002));
#168750=CARTESIAN_POINT('Ctrl Pts',(5.94524645699994,12.2,-8.66808434000001));
#168751=CARTESIAN_POINT('Ctrl Pts',(5.94649370399994,12.2,-8.66933491000001));
#168752=CARTESIAN_POINT('Ctrl Pts',(5.94774741599994,12.2,-8.67058964200002));
#168753=CARTESIAN_POINT('Ctrl Pts',(5.94900758799994,12.2,-8.67184851400001));
#168754=CARTESIAN_POINT('Ctrl Pts',(5.95027421799994,12.2,-8.67311150500001));
#168755=CARTESIAN_POINT('Ctrl Pts',(5.95154730199994,12.2,-8.67437859500002));
#168756=CARTESIAN_POINT('Ctrl Pts',(5.95282683699994,12.2,-8.67564976200002));
#168757=CARTESIAN_POINT('Ctrl Pts',(5.95411282099994,12.2,-8.67692498600002));
#168758=CARTESIAN_POINT('Ctrl Pts',(5.95540524899994,12.2,-8.67820424500002));
#168759=CARTESIAN_POINT('Ctrl Pts',(5.95670411999994,12.2,-8.67948752000002));
#168760=CARTESIAN_POINT('Ctrl Pts',(5.95800942899994,12.2,-8.68077479000002));
#168761=CARTESIAN_POINT('Ctrl Pts',(5.95932117299995,12.2,-8.68206603400001));
#168762=CARTESIAN_POINT('Ctrl Pts',(5.96063934899995,12.2,-8.68336123200002));
#168763=CARTESIAN_POINT('Ctrl Pts',(5.96196395499994,12.2,-8.68466036400001));
#168764=CARTESIAN_POINT('Ctrl Pts',(5.96329498499995,12.2,-8.68596340900002));
#168765=CARTESIAN_POINT('Ctrl Pts',(5.96463243999994,12.2,-8.68727034800001));
#168766=CARTESIAN_POINT('Ctrl Pts',(5.96597631299995,12.2,-8.68858116100002));
#168767=CARTESIAN_POINT('Ctrl Pts',(5.96732660299994,12.2,-8.68989582500001));
#168768=CARTESIAN_POINT('Ctrl Pts',(5.96868330599994,12.2,-8.69121432500001));
#168769=CARTESIAN_POINT('Ctrl Pts',(5.97004641899994,12.2,-8.69253663700002));
#168770=CARTESIAN_POINT('Ctrl Pts',(5.97141593799994,12.2,-8.69386274300001));
#168771=CARTESIAN_POINT('Ctrl Pts',(5.97279186099994,12.2,-8.69519262200001));
#168772=CARTESIAN_POINT('Ctrl Pts',(5.97417418499995,12.2,-8.69652625600001));
#168773=CARTESIAN_POINT('Ctrl Pts',(5.97556290599995,12.2,-8.69786362500001));
#168774=CARTESIAN_POINT('Ctrl Pts',(5.97695801999994,12.2,-8.69920470900002));
#168775=CARTESIAN_POINT('Ctrl Pts',(5.97835952599994,12.2,-8.70054948900002));
#168776=CARTESIAN_POINT('Ctrl Pts',(5.97976741899994,12.2,-8.70189794500002));
#168777=CARTESIAN_POINT('Ctrl Pts',(5.98118169699994,12.2,-8.70325005800002));
#168778=CARTESIAN_POINT('Ctrl Pts',(5.98260235599994,12.2,-8.70460581000001));
#168779=CARTESIAN_POINT('Ctrl Pts',(5.98402939199994,12.2,-8.70596518000001));
#168780=CARTESIAN_POINT('Ctrl Pts',(5.98546280499994,12.2,-8.70732814900002));
#168781=CARTESIAN_POINT('Ctrl Pts',(5.98690258799994,12.2,-8.70869469900001));
#168782=CARTESIAN_POINT('Ctrl Pts',(5.98834873999994,12.2,-8.71006481000002));
#168783=CARTESIAN_POINT('Ctrl Pts',(5.98980125799994,12.2,-8.71143846400001));
#168784=CARTESIAN_POINT('Ctrl Pts',(5.99126013699995,12.2,-8.71281564200002));
#168785=CARTESIAN_POINT('Ctrl Pts',(5.99272537499995,12.2,-8.71419632500002));
#168786=CARTESIAN_POINT('Ctrl Pts',(5.99419696899995,12.2,-8.71558049400001));
#168787=CARTESIAN_POINT('Ctrl Pts',(5.99567491499994,12.2,-8.71696813100002));
#168788=CARTESIAN_POINT('Ctrl Pts',(5.99715921199994,12.2,-8.71835921700002));
#168789=CARTESIAN_POINT('Ctrl Pts',(5.99864985299994,12.2,-8.71975373400002));
#168790=CARTESIAN_POINT('Ctrl Pts',(6.00014683699994,12.2,-8.72115166300001));
#168791=CARTESIAN_POINT('Ctrl Pts',(6.00165016199994,12.2,-8.72255298400002));
#168792=CARTESIAN_POINT('Ctrl Pts',(6.00315982299994,12.2,-8.72395768300001));
#168793=CARTESIAN_POINT('Ctrl Pts',(6.00467581699994,12.2,-8.72536573700001));
#168794=CARTESIAN_POINT('Ctrl Pts',(6.00619813999994,12.2,-8.72677713200002));
#168795=CARTESIAN_POINT('Ctrl Pts',(6.00772679099994,12.2,-8.72819184600001));
#168796=CARTESIAN_POINT('Ctrl Pts',(6.00926176599994,12.2,-8.72960986400001));
#168797=CARTESIAN_POINT('Ctrl Pts',(6.01080305999994,12.2,-8.73103116600002));
#168798=CARTESIAN_POINT('Ctrl Pts',(6.01235067299994,12.2,-8.73245573400002));
#168799=CARTESIAN_POINT('Ctrl Pts',(6.01390459799994,12.2,-8.73388355100002));
#168800=CARTESIAN_POINT('Ctrl Pts',(6.01546483399994,12.2,-8.73531460000001));
#168801=CARTESIAN_POINT('Ctrl Pts',(6.01703137899994,12.2,-8.73674886200002));
#168802=CARTESIAN_POINT('Ctrl Pts',(6.01860422799994,12.2,-8.73818631900001));
#168803=CARTESIAN_POINT('Ctrl Pts',(6.02018337599994,12.2,-8.73962695300002));
#168804=CARTESIAN_POINT('Ctrl Pts',(6.02176882399994,12.2,-8.74107074900002));
#168805=CARTESIAN_POINT('Ctrl Pts',(6.02336056599994,12.2,-8.74251768600002));
#168806=CARTESIAN_POINT('Ctrl Pts',(6.02495859899994,12.2,-8.74396774900001));
#168807=CARTESIAN_POINT('Ctrl Pts',(6.02656291999994,12.2,-8.74542091800001));
#168808=CARTESIAN_POINT('Ctrl Pts',(6.02817352699994,12.2,-8.74687718000001));
#168809=CARTESIAN_POINT('Ctrl Pts',(6.02979041499994,12.2,-8.74833651300002));
#168810=CARTESIAN_POINT('Ctrl Pts',(6.03141358199994,12.2,-8.74979890200001));
#168811=CARTESIAN_POINT('Ctrl Pts',(6.03304302299994,12.2,-8.75126433100002));
#168812=CARTESIAN_POINT('Ctrl Pts',(6.03467873699994,12.2,-8.75273277900002));
#168813=CARTESIAN_POINT('Ctrl Pts',(6.03632071899994,12.2,-8.75420423200002));
#168814=CARTESIAN_POINT('Ctrl Pts',(6.03796896799994,12.2,-8.75567867300001));
#168815=CARTESIAN_POINT('Ctrl Pts',(6.03962347799994,12.2,-8.75715608400002));
#168816=CARTESIAN_POINT('Ctrl Pts',(6.04128424699995,12.2,-8.75863644800001));
#168817=CARTESIAN_POINT('Ctrl Pts',(6.04295127299994,12.2,-8.76011974800001));
#168818=CARTESIAN_POINT('Ctrl Pts',(6.04462455099994,12.2,-8.76160596800002));
#168819=CARTESIAN_POINT('Ctrl Pts',(6.04630407799994,12.2,-8.76309509100002));
#168820=CARTESIAN_POINT('Ctrl Pts',(6.04798985099994,12.2,-8.76458710000002));
#168821=CARTESIAN_POINT('Ctrl Pts',(6.04968186699994,12.2,-8.76608197700002));
#168822=CARTESIAN_POINT('Ctrl Pts',(6.05138012199994,12.2,-8.76757970900002));
#168823=CARTESIAN_POINT('Ctrl Pts',(6.05308461499994,12.2,-8.76908027600001));
#168824=CARTESIAN_POINT('Ctrl Pts',(6.05479533999994,12.2,-8.77058366200002));
#168825=CARTESIAN_POINT('Ctrl Pts',(6.05651229499995,12.2,-8.77208985200001));
#168826=CARTESIAN_POINT('Ctrl Pts',(6.05823547599995,12.2,-8.77359882900001));
#168827=CARTESIAN_POINT('Ctrl Pts',(6.05996488099994,12.2,-8.77511057700002));
#168828=CARTESIAN_POINT('Ctrl Pts',(6.06170050599994,12.2,-8.77662507800002));
#168829=CARTESIAN_POINT('Ctrl Pts',(6.06344234899994,12.2,-8.77814231800001));
#168830=CARTESIAN_POINT('Ctrl Pts',(6.06519040399994,12.2,-8.77966227900002));
#168831=CARTESIAN_POINT('Ctrl Pts',(6.06694466899994,12.2,-8.78118494600002));
#168832=CARTESIAN_POINT('Ctrl Pts',(6.06870514199994,12.2,-8.78271030200001));
#168833=CARTESIAN_POINT('Ctrl Pts',(6.07047181899994,12.2,-8.78423833100002));
#168834=CARTESIAN_POINT('Ctrl Pts',(6.07224469599994,12.2,-8.78576901800002));
#168835=CARTESIAN_POINT('Ctrl Pts',(6.07402377099994,12.2,-8.78730234600001));
#168836=CARTESIAN_POINT('Ctrl Pts',(6.07580903899994,12.2,-8.78883830000002));
#168837=CARTESIAN_POINT('Ctrl Pts',(6.07760049799994,12.2,-8.79037686400002));
#168838=CARTESIAN_POINT('Ctrl Pts',(6.07939814499994,12.2,-8.79191802100001));
#168839=CARTESIAN_POINT('Ctrl Pts',(6.08120197499994,12.2,-8.79346175700002));
#168840=CARTESIAN_POINT('Ctrl Pts',(6.08301198699994,12.2,-8.79500805500001));
#168841=CARTESIAN_POINT('Ctrl Pts',(6.08482817699994,12.2,-8.79655689900002));
#168842=CARTESIAN_POINT('Ctrl Pts',(6.08665053999994,12.2,-8.79810827400001));
#168843=CARTESIAN_POINT('Ctrl Pts',(6.08847907499994,12.2,-8.79966216600002));
#168844=CARTESIAN_POINT('Ctrl Pts',(6.09031377799995,12.2,-8.80121855700001));
#168845=CARTESIAN_POINT('Ctrl Pts',(6.09215464499994,12.2,-8.80277743400002));
#168846=CARTESIAN_POINT('Ctrl Pts',(6.09400167399994,12.2,-8.80433877800002));
#168847=CARTESIAN_POINT('Ctrl Pts',(6.09585485999994,12.2,-8.80590257700002));
#168848=CARTESIAN_POINT('Ctrl Pts',(6.09771420199994,12.2,-8.80746881400002));
#168849=CARTESIAN_POINT('Ctrl Pts',(6.09957969399994,12.2,-8.80903747400002));
#168850=CARTESIAN_POINT('Ctrl Pts',(6.10145133499994,12.2,-8.81060854200001));
#168851=CARTESIAN_POINT('Ctrl Pts',(6.10332912099994,12.2,-8.81218200200001));
#168852=CARTESIAN_POINT('Ctrl Pts',(6.10521304799994,12.2,-8.81375784000002));
#168853=CARTESIAN_POINT('Ctrl Pts',(6.10710311299994,12.2,-8.81533604100002));
#168854=CARTESIAN_POINT('Ctrl Pts',(6.10899931399994,12.2,-8.81691658800002));
#168855=CARTESIAN_POINT('Ctrl Pts',(6.11090164599994,12.2,-8.81849946800001));
#168856=CARTESIAN_POINT('Ctrl Pts',(6.11281010699994,12.2,-8.82008466500002));
#168857=CARTESIAN_POINT('Ctrl Pts',(6.11472469299994,12.2,-8.82167216400001));
#168858=CARTESIAN_POINT('Ctrl Pts',(6.11664539999994,12.2,-8.82326195200001));
#168859=CARTESIAN_POINT('Ctrl Pts',(6.11857222599994,12.2,-8.82485401100002));
#168860=CARTESIAN_POINT('Ctrl Pts',(6.12050516699994,12.2,-8.82644832800001));
#168861=CARTESIAN_POINT('Ctrl Pts',(6.12244422199994,12.2,-8.82804488900002));
#168862=CARTESIAN_POINT('Ctrl Pts',(6.12438938299994,12.2,-8.82964367800002));
#168863=CARTESIAN_POINT('Ctrl Pts',(6.12634064999994,12.2,-8.83124468000002));
#168864=CARTESIAN_POINT('Ctrl Pts',(6.12829801999994,12.2,-8.83284788100001));
#168865=CARTESIAN_POINT('Ctrl Pts',(6.13026148799994,12.2,-8.83445326700001));
#168866=CARTESIAN_POINT('Ctrl Pts',(6.13223105199994,12.2,-8.83606082300001));
#168867=CARTESIAN_POINT('Ctrl Pts',(6.13420670699994,12.2,-8.83767053400002));
#168868=CARTESIAN_POINT('Ctrl Pts',(6.13618845099994,12.2,-8.83928238600001));
#168869=CARTESIAN_POINT('Ctrl Pts',(6.13817627999994,12.2,-8.84089636400001));
#168870=CARTESIAN_POINT('Ctrl Pts',(6.14017019199994,12.2,-8.84251245500002));
#168871=CARTESIAN_POINT('Ctrl Pts',(6.14217018299994,12.2,-8.84413064300002));
#168872=CARTESIAN_POINT('Ctrl Pts',(6.14417624999994,12.2,-8.84575091500002));
#168873=CARTESIAN_POINT('Ctrl Pts',(6.14618838899994,12.2,-8.84737325500002));
#168874=CARTESIAN_POINT('Ctrl Pts',(6.14820659699994,12.2,-8.84899765100002));
#168875=CARTESIAN_POINT('Ctrl Pts',(6.15023086899994,12.2,-8.85062408700002));
#168876=CARTESIAN_POINT('Ctrl Pts',(6.15226120499995,12.2,-8.85225255100002));
#168877=CARTESIAN_POINT('Ctrl Pts',(6.15429759899994,12.2,-8.85388302700001));
#168878=CARTESIAN_POINT('Ctrl Pts',(6.15634004999994,12.2,-8.85551550100002));
#168879=CARTESIAN_POINT('Ctrl Pts',(6.15838855099994,12.2,-8.85714995900001));
#168880=CARTESIAN_POINT('Ctrl Pts',(6.16044310199994,12.2,-8.85878638800002));
#168881=CARTESIAN_POINT('Ctrl Pts',(6.16250369999994,12.2,-8.86042477400002));
#168882=CARTESIAN_POINT('Ctrl Pts',(6.16457033899994,12.2,-8.86206510100001));
#168883=CARTESIAN_POINT('Ctrl Pts',(6.16664301799994,12.2,-8.86370735900002));
#168884=CARTESIAN_POINT('Ctrl Pts',(6.16872173199994,12.2,-8.86535153000001));
#168885=CARTESIAN_POINT('Ctrl Pts',(6.17080647799994,12.2,-8.86699760300001));
#168886=CARTESIAN_POINT('Ctrl Pts',(6.17289725299995,12.2,-8.86864556300001));
#168887=CARTESIAN_POINT('Ctrl Pts',(6.17499405399994,12.2,-8.87029539700002));
#168888=CARTESIAN_POINT('Ctrl Pts',(6.17709687799994,12.2,-8.87194709200001));
#168889=CARTESIAN_POINT('Ctrl Pts',(6.17920571999994,12.2,-8.87360063200001));
#168890=CARTESIAN_POINT('Ctrl Pts',(6.18132057899994,12.2,-8.87525600500001));
#168891=CARTESIAN_POINT('Ctrl Pts',(6.18344144899994,12.2,-8.87691319600002));
#168892=CARTESIAN_POINT('Ctrl Pts',(6.18556832799994,12.2,-8.87857219500002));
#168893=CARTESIAN_POINT('Ctrl Pts',(6.18770121399994,12.2,-8.88023298500002));
#168894=CARTESIAN_POINT('Ctrl Pts',(6.18984009999994,12.2,-8.88189555400002));
#168895=CARTESIAN_POINT('Ctrl Pts',(6.19198498599994,12.2,-8.88355988700001));
#168896=CARTESIAN_POINT('Ctrl Pts',(6.19413586799994,12.2,-8.88522597300001));
#168897=CARTESIAN_POINT('Ctrl Pts',(6.19629274299994,12.2,-8.88689379800002));
#168898=CARTESIAN_POINT('Ctrl Pts',(6.19845560599994,12.2,-8.88856334700002));
#168899=CARTESIAN_POINT('Ctrl Pts',(6.20062445399994,12.2,-8.89023460900002));
#168900=CARTESIAN_POINT('Ctrl Pts',(6.20279928499994,12.2,-8.89190757000001));
#168901=CARTESIAN_POINT('Ctrl Pts',(6.20498009499994,12.2,-8.89358221500002));
#168902=CARTESIAN_POINT('Ctrl Pts',(6.20716688099994,12.2,-8.89525853400002));
#168903=CARTESIAN_POINT('Ctrl Pts',(6.20935963799995,12.2,-8.89693651100002));
#168904=CARTESIAN_POINT('Ctrl Pts',(6.21155836399994,12.2,-8.89861613500001));
#168905=CARTESIAN_POINT('Ctrl Pts',(6.21376305499994,12.2,-8.90029739200001));
#168906=CARTESIAN_POINT('Ctrl Pts',(6.21597370899994,12.2,-8.90198026900002));
#168907=CARTESIAN_POINT('Ctrl Pts',(6.21819032199994,12.2,-8.90366475300001));
#168908=CARTESIAN_POINT('Ctrl Pts',(6.22041288899994,12.2,-8.90535083100002));
#168909=CARTESIAN_POINT('Ctrl Pts',(6.22264140799994,12.2,-8.90703849100002));
#168910=CARTESIAN_POINT('Ctrl Pts',(6.22487587699994,12.2,-8.90872771900002));
#168911=CARTESIAN_POINT('Ctrl Pts',(6.22711629099994,12.2,-8.91041850200001));
#168912=CARTESIAN_POINT('Ctrl Pts',(6.22936264599994,12.2,-8.91211082700002));
#168913=CARTESIAN_POINT('Ctrl Pts',(6.23161493899994,12.2,-8.91380468300002));
#168914=CARTESIAN_POINT('Ctrl Pts',(6.23387316899994,12.2,-8.91550005600001));
#168915=CARTESIAN_POINT('Ctrl Pts',(6.23613732999994,12.2,-8.91719693300002));
#168916=CARTESIAN_POINT('Ctrl Pts',(6.23840741799994,12.2,-8.91889530200002));
#168917=CARTESIAN_POINT('Ctrl Pts',(6.24068343299994,12.2,-8.92059515000001));
#168918=CARTESIAN_POINT('Ctrl Pts',(6.24296536899994,12.2,-8.92229646500001));
#168919=CARTESIAN_POINT('Ctrl Pts',(6.24525322299994,12.2,-8.92399923300001));
#168920=CARTESIAN_POINT('Ctrl Pts',(6.24754699199994,12.2,-8.92570344200001));
#168921=CARTESIAN_POINT('Ctrl Pts',(6.24984667299994,12.2,-8.92740908100001));
#168922=CARTESIAN_POINT('Ctrl Pts',(6.25215226099994,12.2,-8.92911613600001));
#168923=CARTESIAN_POINT('Ctrl Pts',(6.25446375499994,12.2,-8.93082459400001));
#168924=CARTESIAN_POINT('Ctrl Pts',(6.25678114899994,12.2,-8.93253444400001));
#168925=CARTESIAN_POINT('Ctrl Pts',(6.25910444299994,12.2,-8.93424567300002));
#168926=CARTESIAN_POINT('Ctrl Pts',(6.26143362999994,12.2,-8.93595826800002));
#168927=CARTESIAN_POINT('Ctrl Pts',(6.26376870799994,12.2,-8.93767221800001));
#168928=CARTESIAN_POINT('Ctrl Pts',(6.26610967499994,12.2,-8.93938751000002));
#168929=CARTESIAN_POINT('Ctrl Pts',(6.26845652499994,12.2,-8.94110413200002));
#168930=CARTESIAN_POINT('Ctrl Pts',(6.27080925699994,12.2,-8.94282207100002));
#168931=CARTESIAN_POINT('Ctrl Pts',(6.27316786699994,12.2,-8.94454131600002));
#168932=CARTESIAN_POINT('Ctrl Pts',(6.27553235099994,12.2,-8.94626185400002));
#168933=CARTESIAN_POINT('Ctrl Pts',(6.27790270499994,12.2,-8.94798367200002));
#168934=CARTESIAN_POINT('Ctrl Pts',(6.28027892799994,12.2,-8.94970676000002));
#168935=CARTESIAN_POINT('Ctrl Pts',(6.28266101299994,12.2,-8.95143110400002));
#168936=CARTESIAN_POINT('Ctrl Pts',(6.28504895899994,12.2,-8.95315669400001));
#168937=CARTESIAN_POINT('Ctrl Pts',(6.28744276399994,12.2,-8.95488351500001));
#168938=CARTESIAN_POINT('Ctrl Pts',(6.28984242199994,12.2,-8.95661155900001));
#168939=CARTESIAN_POINT('Ctrl Pts',(6.29224792999994,12.2,-8.95834081000002));
#168940=CARTESIAN_POINT('Ctrl Pts',(6.29465928599994,12.2,-8.96007125900002));
#168941=CARTESIAN_POINT('Ctrl Pts',(6.29707648499994,12.2,-8.96180289200002));
#168942=CARTESIAN_POINT('Ctrl Pts',(6.29949952399994,12.2,-8.96353569800001));
#168943=CARTESIAN_POINT('Ctrl Pts',(6.30192839999994,12.2,-8.96526966600002));
#168944=CARTESIAN_POINT('Ctrl Pts',(6.30436310999994,12.2,-8.96700478300002));
#168945=CARTESIAN_POINT('Ctrl Pts',(6.30680364899994,12.2,-8.96874103900002));
#168946=CARTESIAN_POINT('Ctrl Pts',(6.30925001499994,12.2,-8.97047842000001));
#168947=CARTESIAN_POINT('Ctrl Pts',(6.31170220399994,12.2,-8.97221691500001));
#168948=CARTESIAN_POINT('Ctrl Pts',(6.31416021399994,12.2,-8.97395651300002));
#168949=CARTESIAN_POINT('Ctrl Pts',(6.31662403899994,12.2,-8.97569720100002));
#168950=CARTESIAN_POINT('Ctrl Pts',(6.31909367699994,12.2,-8.97743896900002));
#168951=CARTESIAN_POINT('Ctrl Pts',(6.32156912499994,12.2,-8.97918180400002));
#168952=CARTESIAN_POINT('Ctrl Pts',(6.32405037899994,12.2,-8.98092569600001));
#168953=CARTESIAN_POINT('Ctrl Pts',(6.32653743599994,12.2,-8.98267063100001));
#168954=CARTESIAN_POINT('Ctrl Pts',(6.32903029199994,12.2,-8.98441660100002));
#168955=CARTESIAN_POINT('Ctrl Pts',(6.33152894299994,12.2,-8.98616359100001));
#168956=CARTESIAN_POINT('Ctrl Pts',(6.33403338799994,12.2,-8.98791159100002));
#168957=CARTESIAN_POINT('Ctrl Pts',(6.33654362099994,12.2,-8.98966059000001));
#168958=CARTESIAN_POINT('Ctrl Pts',(6.33905963999994,12.2,-8.99141057600002));
#168959=CARTESIAN_POINT('Ctrl Pts',(6.34158143999994,12.2,-8.99316153900001));
#168960=CARTESIAN_POINT('Ctrl Pts',(6.34410901999994,12.2,-8.99491346500002));
#168961=CARTESIAN_POINT('Ctrl Pts',(6.34664237499994,12.2,-8.99666634500001));
#168962=CARTESIAN_POINT('Ctrl Pts',(6.34918150099994,12.2,-8.99842016600001));
#168963=CARTESIAN_POINT('Ctrl Pts',(6.35172639699994,12.2,-9.00017491800002));
#168964=CARTESIAN_POINT('Ctrl Pts',(6.35427705599994,12.2,-9.00193058900001));
#168965=CARTESIAN_POINT('Ctrl Pts',(6.35683347799994,12.2,-9.00368716800001));
#168966=CARTESIAN_POINT('Ctrl Pts',(6.35939565699994,12.2,-9.00544464400001));
#168967=CARTESIAN_POINT('Ctrl Pts',(6.36196359199994,12.2,-9.00720300600002));
#168968=CARTESIAN_POINT('Ctrl Pts',(6.36453727799994,12.2,-9.00896224300002));
#168969=CARTESIAN_POINT('Ctrl Pts',(6.36711671099994,12.2,-9.01072234300001));
#168970=CARTESIAN_POINT('Ctrl Pts',(6.36970188799994,12.2,-9.01248329400002));
#168971=CARTESIAN_POINT('Ctrl Pts',(6.37229280699994,12.2,-9.01424508800002));
#168972=CARTESIAN_POINT('Ctrl Pts',(6.37488946299994,12.2,-9.01600771300001));
#168973=CARTESIAN_POINT('Ctrl Pts',(6.37749185299994,12.2,-9.01777115600002));
#168974=CARTESIAN_POINT('Ctrl Pts',(6.38009997299994,12.2,-9.01953540700001));
#168975=CARTESIAN_POINT('Ctrl Pts',(6.38271382099994,12.2,-9.02130045600002));
#168976=CARTESIAN_POINT('Ctrl Pts',(6.38533339199994,12.2,-9.02306629200002));
#168977=CARTESIAN_POINT('Ctrl Pts',(6.38795868399994,12.2,-9.02483290300001));
#168978=CARTESIAN_POINT('Ctrl Pts',(6.39058969199994,12.2,-9.02660027900002));
#168979=CARTESIAN_POINT('Ctrl Pts',(6.39322641399994,12.2,-9.02836840800001));
#168980=CARTESIAN_POINT('Ctrl Pts',(6.39586884499994,12.2,-9.03013728200002));
#168981=CARTESIAN_POINT('Ctrl Pts',(6.39851698299994,12.2,-9.03190688700001));
#168982=CARTESIAN_POINT('Ctrl Pts',(6.40117082299994,12.2,-9.03367721300001));
#168983=CARTESIAN_POINT('Ctrl Pts',(6.40383036299994,12.2,-9.03544825000001));
#168984=CARTESIAN_POINT('Ctrl Pts',(6.40649559999994,12.2,-9.03721998700002));
#168985=CARTESIAN_POINT('Ctrl Pts',(6.40916652899994,12.2,-9.03899241300002));
#168986=CARTESIAN_POINT('Ctrl Pts',(6.41184314599994,12.2,-9.04076551800001));
#168987=CARTESIAN_POINT('Ctrl Pts',(6.41452544999994,12.2,-9.04253929100001));
#168988=CARTESIAN_POINT('Ctrl Pts',(6.41721343599994,12.2,-9.04431372100002));
#168989=CARTESIAN_POINT('Ctrl Pts',(6.41990709999994,12.2,-9.04608879800002));
#168990=CARTESIAN_POINT('Ctrl Pts',(6.42260643999994,12.2,-9.04786451100002));
#168991=CARTESIAN_POINT('Ctrl Pts',(6.42531145199994,12.2,-9.04964084900002));
#168992=CARTESIAN_POINT('Ctrl Pts',(6.42802213199994,12.2,-9.05141780400001));
#168993=CARTESIAN_POINT('Ctrl Pts',(6.43073847599994,12.2,-9.05319536200002));
#168994=CARTESIAN_POINT('Ctrl Pts',(6.43346048199994,12.2,-9.05497351500001));
#168995=CARTESIAN_POINT('Ctrl Pts',(6.43618814599995,12.2,-9.05675225100002));
#168996=CARTESIAN_POINT('Ctrl Pts',(6.43892146399994,12.2,-9.05853156000001));
#168997=CARTESIAN_POINT('Ctrl Pts',(6.44166043299994,12.2,-9.06031143300002));
#168998=CARTESIAN_POINT('Ctrl Pts',(6.44440504999994,12.2,-9.06209185800002));
#168999=CARTESIAN_POINT('Ctrl Pts',(6.44715531099994,12.2,-9.06387282500001));
#169000=CARTESIAN_POINT('Ctrl Pts',(6.44991121199994,12.2,-9.06565432300001));
#169001=CARTESIAN_POINT('Ctrl Pts',(6.45267274999994,12.2,-9.06743634400001));
#169002=CARTESIAN_POINT('Ctrl Pts',(6.45543992299994,12.2,-9.06921887500001));
#169003=CARTESIAN_POINT('Ctrl Pts',(6.45821272399994,12.2,-9.07100190800002));
#169004=CARTESIAN_POINT('Ctrl Pts',(6.46099115299994,12.2,-9.07278543100002));
#169005=CARTESIAN_POINT('Ctrl Pts',(6.46377520499994,12.2,-9.07456943400001));
#169006=CARTESIAN_POINT('Ctrl Pts',(6.46656487599994,12.2,-9.07635390800002));
#169007=CARTESIAN_POINT('Ctrl Pts',(6.46936016299994,12.2,-9.07813884200002));
#169008=CARTESIAN_POINT('Ctrl Pts',(6.47216106399994,12.2,-9.07992422500002));
#169009=CARTESIAN_POINT('Ctrl Pts',(6.47496757199994,12.2,-9.08171004900002));
#169010=CARTESIAN_POINT('Ctrl Pts',(6.47777968799994,12.2,-9.08349630400001));
#169011=CARTESIAN_POINT('Ctrl Pts',(6.48059740499994,12.2,-9.08528297600002));
#169012=CARTESIAN_POINT('Ctrl Pts',(6.48342072099994,12.2,-9.08707005900002));
#169013=CARTESIAN_POINT('Ctrl Pts',(6.48624963199994,12.2,-9.08885754100002));
#169014=CARTESIAN_POINT('Ctrl Pts',(6.48908413499994,12.2,-9.09064541400002));
#169015=CARTESIAN_POINT('Ctrl Pts',(6.49192422599994,12.2,-9.09243366500002));
#169016=CARTESIAN_POINT('Ctrl Pts',(6.49476990199994,12.2,-9.09422228700001));
#169017=CARTESIAN_POINT('Ctrl Pts',(6.49762115899994,12.2,-9.09601126700002));
#169018=CARTESIAN_POINT('Ctrl Pts',(6.50047799399994,12.2,-9.09780059800001));
#169019=CARTESIAN_POINT('Ctrl Pts',(6.50334040299994,12.2,-9.09959026900001));
#169020=CARTESIAN_POINT('Ctrl Pts',(6.50620838199995,12.2,-9.10138026900002));
#169021=CARTESIAN_POINT('Ctrl Pts',(6.50908192999994,12.2,-9.10317059000001));
#169022=CARTESIAN_POINT('Ctrl Pts',(6.51196104099995,12.2,-9.10496122100002));
#169023=CARTESIAN_POINT('Ctrl Pts',(6.51484571099994,12.2,-9.10675215300002));
#169024=CARTESIAN_POINT('Ctrl Pts',(6.51773593899994,12.2,-9.10854337500002));
#169025=CARTESIAN_POINT('Ctrl Pts',(6.52063172099994,12.2,-9.11033487800001));
#169026=CARTESIAN_POINT('Ctrl Pts',(6.52353305099994,12.2,-9.11212665200001));
#169027=CARTESIAN_POINT('Ctrl Pts',(6.52643992799994,12.2,-9.11391868900001));
#169028=CARTESIAN_POINT('Ctrl Pts',(6.52935234699994,12.2,-9.11571097500002));
#169029=CARTESIAN_POINT('Ctrl Pts',(6.53227030599994,12.2,-9.11750350600002));
#169030=CARTESIAN_POINT('Ctrl Pts',(6.53519379999994,12.2,-9.11929626800001));
#169031=CARTESIAN_POINT('Ctrl Pts',(6.53812282699994,12.2,-9.12108925300002));
#169032=CARTESIAN_POINT('Ctrl Pts',(6.54105738299994,12.2,-9.12288245200001));
#169033=CARTESIAN_POINT('Ctrl Pts',(6.54399746299994,12.2,-9.12467585300002));
#169034=CARTESIAN_POINT('Ctrl Pts',(6.54694306499994,12.2,-9.12646944900001));
#169035=CARTESIAN_POINT('Ctrl Pts',(6.54989418399994,12.2,-9.12826322900001));
#169036=CARTESIAN_POINT('Ctrl Pts',(6.55285081899994,12.2,-9.13005718400001));
#169037=CARTESIAN_POINT('Ctrl Pts',(6.55581296599994,12.2,-9.13185130500001));
#169038=CARTESIAN_POINT('Ctrl Pts',(6.55878061899994,12.2,-9.13364558100002));
#169039=CARTESIAN_POINT('Ctrl Pts',(6.56175377599994,12.2,-9.13544000400002));
#169040=CARTESIAN_POINT('Ctrl Pts',(6.56473243399994,12.2,-9.13723456500002));
#169041=CARTESIAN_POINT('Ctrl Pts',(6.56771658899994,12.2,-9.13902925200002));
#169042=CARTESIAN_POINT('Ctrl Pts',(6.57070623699994,12.2,-9.14082405700002));
#169043=CARTESIAN_POINT('Ctrl Pts',(6.57370137599994,12.2,-9.14261897200002));
#169044=CARTESIAN_POINT('Ctrl Pts',(6.57670199999994,12.2,-9.14441398600001));
#169045=CARTESIAN_POINT('Ctrl Pts',(6.57970810799994,12.2,-9.14620908900002));
#169046=CARTESIAN_POINT('Ctrl Pts',(6.58271969499994,12.2,-9.14800427400002));
#169047=CARTESIAN_POINT('Ctrl Pts',(6.58573675799994,12.2,-9.14979953100002));
#169048=CARTESIAN_POINT('Ctrl Pts',(6.58875929299994,12.2,-9.15159484900002));
#169049=CARTESIAN_POINT('Ctrl Pts',(6.59178729699994,12.2,-9.15339022000002));
#169050=CARTESIAN_POINT('Ctrl Pts',(6.59482076499994,12.2,-9.15518563400001));
#169051=CARTESIAN_POINT('Ctrl Pts',(6.59785969599994,12.2,-9.15698108300001));
#169052=CARTESIAN_POINT('Ctrl Pts',(6.60090408599994,12.2,-9.15877655700001));
#169053=CARTESIAN_POINT('Ctrl Pts',(6.60395392899995,12.2,-9.16057204700002));
#169054=CARTESIAN_POINT('Ctrl Pts',(6.60700922399994,12.2,-9.16236754400002));
#169055=CARTESIAN_POINT('Ctrl Pts',(6.61006996599995,12.2,-9.16416303900002));
#169056=CARTESIAN_POINT('Ctrl Pts',(6.61313615199994,12.2,-9.16595852100002));
#169057=CARTESIAN_POINT('Ctrl Pts',(6.61620777899994,12.2,-9.16775398400001));
#169058=CARTESIAN_POINT('Ctrl Pts',(6.61928484299994,12.2,-9.16954941700002));
#169059=CARTESIAN_POINT('Ctrl Pts',(6.62236733999994,12.2,-9.17134481100002));
#169060=CARTESIAN_POINT('Ctrl Pts',(6.62545526699994,12.2,-9.17314015600001));
#169061=CARTESIAN_POINT('Ctrl Pts',(6.62854862099994,12.2,-9.17493544700001));
#169062=CARTESIAN_POINT('Ctrl Pts',(6.63164739699994,12.2,-9.17673067000001));
#169063=CARTESIAN_POINT('Ctrl Pts',(6.63475159199994,12.2,-9.17852581800001));
#169064=CARTESIAN_POINT('Ctrl Pts',(6.63786120299994,12.2,-9.18032088200002));
#169065=CARTESIAN_POINT('Ctrl Pts',(6.64097622599994,12.2,-9.18211585500002));
#169066=CARTESIAN_POINT('Ctrl Pts',(6.64409665799995,12.2,-9.18391072500001));
#169067=CARTESIAN_POINT('Ctrl Pts',(6.64722249499994,12.2,-9.18570548400002));
#169068=CARTESIAN_POINT('Ctrl Pts',(6.65035373299995,12.2,-9.18750012300002));
#169069=CARTESIAN_POINT('Ctrl Pts',(6.65349036899994,12.2,-9.18929463500002));
#169070=CARTESIAN_POINT('Ctrl Pts',(6.65663239999994,12.2,-9.19108900900002));
#169071=CARTESIAN_POINT('Ctrl Pts',(6.65977982099994,12.2,-9.19288323700002));
#169072=CARTESIAN_POINT('Ctrl Pts',(6.66293262999995,12.2,-9.19467731100001));
#169073=CARTESIAN_POINT('Ctrl Pts',(6.66609082299995,12.2,-9.19647121900002));
#169074=CARTESIAN_POINT('Ctrl Pts',(6.66925439499994,12.2,-9.19826495600002));
#169075=CARTESIAN_POINT('Ctrl Pts',(6.67242334399995,12.2,-9.20005851000001));
#169076=CARTESIAN_POINT('Ctrl Pts',(6.67559766699994,12.2,-9.20185187500002));
#169077=CARTESIAN_POINT('Ctrl Pts',(6.67877735899994,12.2,-9.20364504200002));
#169078=CARTESIAN_POINT('Ctrl Pts',(6.68196241599994,12.2,-9.20543800000001));
#169079=CARTESIAN_POINT('Ctrl Pts',(6.68515283699994,12.2,-9.20723074200002));
#169080=CARTESIAN_POINT('Ctrl Pts',(6.68834861499994,12.2,-9.20902325900002));
#169081=CARTESIAN_POINT('Ctrl Pts',(6.69154974999994,12.2,-9.21081554300001));
#169082=CARTESIAN_POINT('Ctrl Pts',(6.69475623599994,12.2,-9.21260758400001));
#169083=CARTESIAN_POINT('Ctrl Pts',(6.69796806999994,12.2,-9.21439937500002));
#169084=CARTESIAN_POINT('Ctrl Pts',(6.70118524799994,12.2,-9.21619090500002));
#169085=CARTESIAN_POINT('Ctrl Pts',(6.70440776799994,12.2,-9.21798216800001));
#169086=CARTESIAN_POINT('Ctrl Pts',(6.70763562499994,12.2,-9.21977315400002));
#169087=CARTESIAN_POINT('Ctrl Pts',(6.71086881499994,12.2,-9.22156385400001));
#169088=CARTESIAN_POINT('Ctrl Pts',(6.71410733699994,12.2,-9.22335426000001));
#169089=CARTESIAN_POINT('Ctrl Pts',(6.71735118499994,12.2,-9.22514436400002));
#169090=CARTESIAN_POINT('Ctrl Pts',(6.72060035499995,12.2,-9.22693415700002));
#169091=CARTESIAN_POINT('Ctrl Pts',(6.72385484599994,12.2,-9.22872363200002));
#169092=CARTESIAN_POINT('Ctrl Pts',(6.72711465299995,12.2,-9.23051277900001));
#169093=CARTESIAN_POINT('Ctrl Pts',(6.73037977199994,12.2,-9.23230159000001));
#169094=CARTESIAN_POINT('Ctrl Pts',(6.73365020099994,12.2,-9.23409005700002));
#169095=CARTESIAN_POINT('Ctrl Pts',(6.73692593399994,12.2,-9.23587817000002));
#169096=CARTESIAN_POINT('Ctrl Pts',(6.74020696799994,12.2,-9.23766592000002));
#169097=CARTESIAN_POINT('Ctrl Pts',(6.74349330199994,12.2,-9.23945330000001));
#169098=CARTESIAN_POINT('Ctrl Pts',(6.74678492799995,12.2,-9.24124030000002));
#169099=CARTESIAN_POINT('Ctrl Pts',(6.75008184499994,12.2,-9.24302691400002));
#169100=CARTESIAN_POINT('Ctrl Pts',(6.75338404999994,12.2,-9.24481313200002));
#169101=CARTESIAN_POINT('Ctrl Pts',(6.75669153899995,12.2,-9.24659894800002));
#169102=CARTESIAN_POINT('Ctrl Pts',(6.76000430999994,12.2,-9.24838435500002));
#169103=CARTESIAN_POINT('Ctrl Pts',(6.76332235699994,12.2,-9.25016934500002));
#169104=CARTESIAN_POINT('Ctrl Pts',(6.76664567999994,12.2,-9.25195390800001));
#169105=CARTESIAN_POINT('Ctrl Pts',(6.76997427099994,12.2,-9.25373803600002));
#169106=CARTESIAN_POINT('Ctrl Pts',(6.77330812799994,12.2,-9.25552171800001));
#169107=CARTESIAN_POINT('Ctrl Pts',(6.77664724599994,12.2,-9.25730494300002));
#169108=CARTESIAN_POINT('Ctrl Pts',(6.77999162099994,12.2,-9.25908770200002));
#169109=CARTESIAN_POINT('Ctrl Pts',(6.78334124799994,12.2,-9.26086998700002));
#169110=CARTESIAN_POINT('Ctrl Pts',(6.78669612399994,12.2,-9.26265178800002));
#169111=CARTESIAN_POINT('Ctrl Pts',(6.79005624699994,12.2,-9.26443310200002));
#169112=CARTESIAN_POINT('Ctrl Pts',(6.79342161599994,12.2,-9.26621392500002));
#169113=CARTESIAN_POINT('Ctrl Pts',(6.79679222899994,12.2,-9.26799425300001));
#169114=CARTESIAN_POINT('Ctrl Pts',(6.79949291499995,12.2,-9.26941812000001));
#169115=CARTESIAN_POINT('Ctrl Pts',(6.80152078799994,12.2,-9.27048579800001));
#169116=CARTESIAN_POINT('Ctrl Pts',(6.80287375199994,12.2,-9.27119748400001));
#169117=CARTESIAN_POINT('Ctrl Pts',(6.80355049599994,12.2,-9.27155330300002));
#169118=CARTESIAN_POINT('Ctrl Pts',(7.10901226899994,15.2,-9.03946594400002));
#169119=CARTESIAN_POINT('Ctrl Pts',(7.10901226899994,11.6,-9.03946594400002));
#169120=CARTESIAN_POINT('Ctrl Pts',(7.10885083699995,15.2,-9.03871859500001));
#169121=CARTESIAN_POINT('Ctrl Pts',(7.10885083699995,11.6,-9.03871859500001));
#169122=CARTESIAN_POINT('Ctrl Pts',(7.10852778299994,15.2,-9.03722439200001));
#169123=CARTESIAN_POINT('Ctrl Pts',(7.10852778299994,11.6,-9.03722439200001));
#169124=CARTESIAN_POINT('Ctrl Pts',(7.10804263899995,15.2,-9.03498456100002));
#169125=CARTESIAN_POINT('Ctrl Pts',(7.10804263899995,11.6,-9.03498456100002));
#169126=CARTESIAN_POINT('Ctrl Pts',(7.10739465099994,15.2,-9.03200107200002));
#169127=CARTESIAN_POINT('Ctrl Pts',(7.10739465099994,11.6,-9.03200107200002));
#169128=CARTESIAN_POINT('Ctrl Pts',(7.10658278299994,15.2,-9.02827662900001));
#169129=CARTESIAN_POINT('Ctrl Pts',(7.10658278299994,11.6,-9.02827662900001));
#169130=CARTESIAN_POINT('Ctrl Pts',(7.10576903499994,15.2,-9.02455710700002));
#169131=CARTESIAN_POINT('Ctrl Pts',(7.10576903499994,11.6,-9.02455710700002));
#169132=CARTESIAN_POINT('Ctrl Pts',(7.10495340799994,15.2,-9.02084250500002));
#169133=CARTESIAN_POINT('Ctrl Pts',(7.10495340799994,11.6,-9.02084250500002));
#169134=CARTESIAN_POINT('Ctrl Pts',(7.10413590299994,15.2,-9.01713282900002));
#169135=CARTESIAN_POINT('Ctrl Pts',(7.10413590299994,11.6,-9.01713282900002));
#169136=CARTESIAN_POINT('Ctrl Pts',(7.10331652799994,15.2,-9.01342808000001));
#169137=CARTESIAN_POINT('Ctrl Pts',(7.10331652799994,11.6,-9.01342808000001));
#169138=CARTESIAN_POINT('Ctrl Pts',(7.10249528699994,15.2,-9.00972826500002));
#169139=CARTESIAN_POINT('Ctrl Pts',(7.10249528699994,11.6,-9.00972826500002));
#169140=CARTESIAN_POINT('Ctrl Pts',(7.10167218799994,15.2,-9.00603338900002));
#169141=CARTESIAN_POINT('Ctrl Pts',(7.10167218799994,11.6,-9.00603338900002));
#169142=CARTESIAN_POINT('Ctrl Pts',(7.10084723999994,15.2,-9.00234345900002));
#169143=CARTESIAN_POINT('Ctrl Pts',(7.10084723999994,11.6,-9.00234345900002));
#169144=CARTESIAN_POINT('Ctrl Pts',(7.10002044999994,15.2,-8.99865848200001));
#169145=CARTESIAN_POINT('Ctrl Pts',(7.10002044999994,11.6,-8.99865848200001));
#169146=CARTESIAN_POINT('Ctrl Pts',(7.09919182999994,15.2,-8.99497846600001));
#169147=CARTESIAN_POINT('Ctrl Pts',(7.09919182999994,11.6,-8.99497846600001));
#169148=CARTESIAN_POINT('Ctrl Pts',(7.09836138399995,15.2,-8.99130341500002));
#169149=CARTESIAN_POINT('Ctrl Pts',(7.09836138399995,11.6,-8.99130341500002));
#169150=CARTESIAN_POINT('Ctrl Pts',(7.09752912199995,15.2,-8.98763333900002));
#169151=CARTESIAN_POINT('Ctrl Pts',(7.09752912199995,11.6,-8.98763333900002));
#169152=CARTESIAN_POINT('Ctrl Pts',(7.09669504999995,15.2,-8.98396824000002));
#169153=CARTESIAN_POINT('Ctrl Pts',(7.09669504999995,11.6,-8.98396824000002));
#169154=CARTESIAN_POINT('Ctrl Pts',(7.09585917499994,15.2,-8.98030812400001));
#169155=CARTESIAN_POINT('Ctrl Pts',(7.09585917499994,11.6,-8.98030812400001));
#169156=CARTESIAN_POINT('Ctrl Pts',(7.09502150299994,15.2,-8.97665299700002));
#169157=CARTESIAN_POINT('Ctrl Pts',(7.09502150299994,11.6,-8.97665299700002));
#169158=CARTESIAN_POINT('Ctrl Pts',(7.09418203899994,15.2,-8.97300286300002));
#169159=CARTESIAN_POINT('Ctrl Pts',(7.09418203899994,11.6,-8.97300286300002));
#169160=CARTESIAN_POINT('Ctrl Pts',(7.09334079199994,15.2,-8.96935772800001));
#169161=CARTESIAN_POINT('Ctrl Pts',(7.09334079199994,11.6,-8.96935772800001));
#169162=CARTESIAN_POINT('Ctrl Pts',(7.09249776599994,15.2,-8.96571759800001));
#169163=CARTESIAN_POINT('Ctrl Pts',(7.09249776599994,11.6,-8.96571759800001));
#169164=CARTESIAN_POINT('Ctrl Pts',(7.09165297099994,15.2,-8.96208247700002));
#169165=CARTESIAN_POINT('Ctrl Pts',(7.09165297099994,11.6,-8.96208247700002));
#169166=CARTESIAN_POINT('Ctrl Pts',(7.09080641499994,15.2,-8.95845237400002));
#169167=CARTESIAN_POINT('Ctrl Pts',(7.09080641499994,11.6,-8.95845237400002));
#169168=CARTESIAN_POINT('Ctrl Pts',(7.08995810299994,15.2,-8.95482729200002));
#169169=CARTESIAN_POINT('Ctrl Pts',(7.08995810299994,11.6,-8.95482729200002));
#169170=CARTESIAN_POINT('Ctrl Pts',(7.08910804199994,15.2,-8.95120723800002));
#169171=CARTESIAN_POINT('Ctrl Pts',(7.08910804199994,11.6,-8.95120723800002));
#169172=CARTESIAN_POINT('Ctrl Pts',(7.08825624299994,15.2,-8.94759221800001));
#169173=CARTESIAN_POINT('Ctrl Pts',(7.08825624299994,11.6,-8.94759221800001));
#169174=CARTESIAN_POINT('Ctrl Pts',(7.08740270999995,15.2,-8.94398223900001));
#169175=CARTESIAN_POINT('Ctrl Pts',(7.08740270999995,11.6,-8.94398223900001));
#169176=CARTESIAN_POINT('Ctrl Pts',(7.08654745099994,15.2,-8.94037730400001));
#169177=CARTESIAN_POINT('Ctrl Pts',(7.08654745099994,11.6,-8.94037730400001));
#169178=CARTESIAN_POINT('Ctrl Pts',(7.08569047499994,15.2,-8.93677742100002));
#169179=CARTESIAN_POINT('Ctrl Pts',(7.08569047499994,11.6,-8.93677742100002));
#169180=CARTESIAN_POINT('Ctrl Pts',(7.08483178599994,15.2,-8.93318259300001));
#169181=CARTESIAN_POINT('Ctrl Pts',(7.08483178599994,11.6,-8.93318259300001));
#169182=CARTESIAN_POINT('Ctrl Pts',(7.08397139199994,15.2,-8.92959282900001));
#169183=CARTESIAN_POINT('Ctrl Pts',(7.08397139199994,11.6,-8.92959282900001));
#169184=CARTESIAN_POINT('Ctrl Pts',(7.08310930199994,15.2,-8.92600813100002));
#169185=CARTESIAN_POINT('Ctrl Pts',(7.08310930199994,11.6,-8.92600813100002));
#169186=CARTESIAN_POINT('Ctrl Pts',(7.08224552099994,15.2,-8.92242850800002));
#169187=CARTESIAN_POINT('Ctrl Pts',(7.08224552099994,11.6,-8.92242850800002));
#169188=CARTESIAN_POINT('Ctrl Pts',(7.08138005899994,15.2,-8.91885396400001));
#169189=CARTESIAN_POINT('Ctrl Pts',(7.08138005899994,11.6,-8.91885396400001));
#169190=CARTESIAN_POINT('Ctrl Pts',(7.08051291999994,15.2,-8.91528450500001));
#169191=CARTESIAN_POINT('Ctrl Pts',(7.08051291999994,11.6,-8.91528450500001));
#169192=CARTESIAN_POINT('Ctrl Pts',(7.07964411499994,15.2,-8.91172013700002));
#169193=CARTESIAN_POINT('Ctrl Pts',(7.07964411499994,11.6,-8.91172013700002));
#169194=CARTESIAN_POINT('Ctrl Pts',(7.07877364899994,15.2,-8.90816086600001));
#169195=CARTESIAN_POINT('Ctrl Pts',(7.07877364899994,11.6,-8.90816086600001));
#169196=CARTESIAN_POINT('Ctrl Pts',(7.07790152999995,15.2,-8.90460669800002));
#169197=CARTESIAN_POINT('Ctrl Pts',(7.07790152999995,11.6,-8.90460669800002));
#169198=CARTESIAN_POINT('Ctrl Pts',(7.07702776499994,15.2,-8.90105763700002));
#169199=CARTESIAN_POINT('Ctrl Pts',(7.07702776499994,11.6,-8.90105763700002));
#169200=CARTESIAN_POINT('Ctrl Pts',(7.07615236299994,15.2,-8.89751369100001));
#169201=CARTESIAN_POINT('Ctrl Pts',(7.07615236299994,11.6,-8.89751369100001));
#169202=CARTESIAN_POINT('Ctrl Pts',(7.07527532899995,15.2,-8.89397486500001));
#169203=CARTESIAN_POINT('Ctrl Pts',(7.07527532899995,11.6,-8.89397486500001));
#169204=CARTESIAN_POINT('Ctrl Pts',(7.07439667399994,15.2,-8.89044116400001));
#169205=CARTESIAN_POINT('Ctrl Pts',(7.07439667399994,11.6,-8.89044116400001));
#169206=CARTESIAN_POINT('Ctrl Pts',(7.07351640099994,15.2,-8.88691259500002));
#169207=CARTESIAN_POINT('Ctrl Pts',(7.07351640099994,11.6,-8.88691259500002));
#169208=CARTESIAN_POINT('Ctrl Pts',(7.07263452099994,15.2,-8.88338916200002));
#169209=CARTESIAN_POINT('Ctrl Pts',(7.07263452099994,11.6,-8.88338916200002));
#169210=CARTESIAN_POINT('Ctrl Pts',(7.07175103999995,15.2,-8.87987087200001));
#169211=CARTESIAN_POINT('Ctrl Pts',(7.07175103999995,11.6,-8.87987087200001));
#169212=CARTESIAN_POINT('Ctrl Pts',(7.07086596699994,15.2,-8.87635773100002));
#169213=CARTESIAN_POINT('Ctrl Pts',(7.07086596699994,11.6,-8.87635773100002));
#169214=CARTESIAN_POINT('Ctrl Pts',(7.06997930699995,15.2,-8.87284974500002));
#169215=CARTESIAN_POINT('Ctrl Pts',(7.06997930699995,11.6,-8.87284974500002));
#169216=CARTESIAN_POINT('Ctrl Pts',(7.06909106899994,15.2,-8.86934691900001));
#169217=CARTESIAN_POINT('Ctrl Pts',(7.06909106899994,11.6,-8.86934691900001));
#169218=CARTESIAN_POINT('Ctrl Pts',(7.06820126099994,15.2,-8.86584925900002));
#169219=CARTESIAN_POINT('Ctrl Pts',(7.06820126099994,11.6,-8.86584925900002));
#169220=CARTESIAN_POINT('Ctrl Pts',(7.06730988999994,15.2,-8.86235676900002));
#169221=CARTESIAN_POINT('Ctrl Pts',(7.06730988999994,11.6,-8.86235676900002));
#169222=CARTESIAN_POINT('Ctrl Pts',(7.06641696399994,15.2,-8.85886945800002));
#169223=CARTESIAN_POINT('Ctrl Pts',(7.06641696399994,11.6,-8.85886945800002));
#169224=CARTESIAN_POINT('Ctrl Pts',(7.06552248999994,15.2,-8.85538733200002));
#169225=CARTESIAN_POINT('Ctrl Pts',(7.06552248999994,11.6,-8.85538733200002));
#169226=CARTESIAN_POINT('Ctrl Pts',(7.06462647799994,15.2,-8.85191039400001));
#169227=CARTESIAN_POINT('Ctrl Pts',(7.06462647799994,11.6,-8.85191039400001));
#169228=CARTESIAN_POINT('Ctrl Pts',(7.06372893199994,15.2,-8.84843865100001));
#169229=CARTESIAN_POINT('Ctrl Pts',(7.06372893199994,11.6,-8.84843865100001));
#169230=CARTESIAN_POINT('Ctrl Pts',(7.06282986099994,15.2,-8.84497210900001));
#169231=CARTESIAN_POINT('Ctrl Pts',(7.06282986099994,11.6,-8.84497210900001));
#169232=CARTESIAN_POINT('Ctrl Pts',(7.06192927499995,15.2,-8.84151077400002));
#169233=CARTESIAN_POINT('Ctrl Pts',(7.06192927499995,11.6,-8.84151077400002));
#169234=CARTESIAN_POINT('Ctrl Pts',(7.06102717799994,15.2,-8.83805465100002));
#169235=CARTESIAN_POINT('Ctrl Pts',(7.06102717799994,11.6,-8.83805465100002));
#169236=CARTESIAN_POINT('Ctrl Pts',(7.06012358099994,15.2,-8.83460374700002));
#169237=CARTESIAN_POINT('Ctrl Pts',(7.06012358099994,11.6,-8.83460374700002));
#169238=CARTESIAN_POINT('Ctrl Pts',(7.05921848999994,15.2,-8.83115806600001));
#169239=CARTESIAN_POINT('Ctrl Pts',(7.05921848999994,11.6,-8.83115806600001));
#169240=CARTESIAN_POINT('Ctrl Pts',(7.05831191399994,15.2,-8.82771761700001));
#169241=CARTESIAN_POINT('Ctrl Pts',(7.05831191399994,11.6,-8.82771761700001));
#169242=CARTESIAN_POINT('Ctrl Pts',(7.05740385899994,15.2,-8.82428240200002));
#169243=CARTESIAN_POINT('Ctrl Pts',(7.05740385899994,11.6,-8.82428240200002));
#169244=CARTESIAN_POINT('Ctrl Pts',(7.05649433399994,15.2,-8.82085243000001));
#169245=CARTESIAN_POINT('Ctrl Pts',(7.05649433399994,11.6,-8.82085243000001));
#169246=CARTESIAN_POINT('Ctrl Pts',(7.05558334699995,15.2,-8.81742770600002));
#169247=CARTESIAN_POINT('Ctrl Pts',(7.05558334699995,11.6,-8.81742770600002));
#169248=CARTESIAN_POINT('Ctrl Pts',(7.05467090599995,15.2,-8.81400823500002));
#169249=CARTESIAN_POINT('Ctrl Pts',(7.05467090599995,11.6,-8.81400823500002));
#169250=CARTESIAN_POINT('Ctrl Pts',(7.05375701899994,15.2,-8.81059402400002));
#169251=CARTESIAN_POINT('Ctrl Pts',(7.05375701899994,11.6,-8.81059402400002));
#169252=CARTESIAN_POINT('Ctrl Pts',(7.05284169299994,15.2,-8.80718507700001));
#169253=CARTESIAN_POINT('Ctrl Pts',(7.05284169299994,11.6,-8.80718507700001));
#169254=CARTESIAN_POINT('Ctrl Pts',(7.05192493599994,15.2,-8.80378140200002));
#169255=CARTESIAN_POINT('Ctrl Pts',(7.05192493599994,11.6,-8.80378140200002));
#169256=CARTESIAN_POINT('Ctrl Pts',(7.05100675599994,15.2,-8.80038300300001));
#169257=CARTESIAN_POINT('Ctrl Pts',(7.05100675599994,11.6,-8.80038300300001));
#169258=CARTESIAN_POINT('Ctrl Pts',(7.05008716199995,15.2,-8.79698988800002));
#169259=CARTESIAN_POINT('Ctrl Pts',(7.05008716199995,11.6,-8.79698988800002));
#169260=CARTESIAN_POINT('Ctrl Pts',(7.04916616099994,15.2,-8.79360206200002));
#169261=CARTESIAN_POINT('Ctrl Pts',(7.04916616099994,11.6,-8.79360206200002));
#169262=CARTESIAN_POINT('Ctrl Pts',(7.04824376099995,15.2,-8.79021953000001));
#169263=CARTESIAN_POINT('Ctrl Pts',(7.04824376099995,11.6,-8.79021953000001));
#169264=CARTESIAN_POINT('Ctrl Pts',(7.04731997099994,15.2,-8.78684229900001));
#169265=CARTESIAN_POINT('Ctrl Pts',(7.04731997099994,11.6,-8.78684229900001));
#169266=CARTESIAN_POINT('Ctrl Pts',(7.04639479699994,15.2,-8.78347037400001));
#169267=CARTESIAN_POINT('Ctrl Pts',(7.04639479699994,11.6,-8.78347037400001));
#169268=CARTESIAN_POINT('Ctrl Pts',(7.04546824999994,15.2,-8.78010376100002));
#169269=CARTESIAN_POINT('Ctrl Pts',(7.04546824999994,11.6,-8.78010376100002));
#169270=CARTESIAN_POINT('Ctrl Pts',(7.04454033599994,15.2,-8.77674246600002));
#169271=CARTESIAN_POINT('Ctrl Pts',(7.04454033599994,11.6,-8.77674246600002));
#169272=CARTESIAN_POINT('Ctrl Pts',(7.04361106199995,15.2,-8.77338649600001));
#169273=CARTESIAN_POINT('Ctrl Pts',(7.04361106199995,11.6,-8.77338649600001));
#169274=CARTESIAN_POINT('Ctrl Pts',(7.04268043899994,15.2,-8.77003585600002));
#169275=CARTESIAN_POINT('Ctrl Pts',(7.04268043899994,11.6,-8.77003585600002));
#169276=CARTESIAN_POINT('Ctrl Pts',(7.04174847399995,15.2,-8.76669055200002));
#169277=CARTESIAN_POINT('Ctrl Pts',(7.04174847399995,11.6,-8.76669055200002));
#169278=CARTESIAN_POINT('Ctrl Pts',(7.04081517499994,15.2,-8.76335058900001));
#169279=CARTESIAN_POINT('Ctrl Pts',(7.04081517499994,11.6,-8.76335058900001));
#169280=CARTESIAN_POINT('Ctrl Pts',(7.03988054999994,15.2,-8.76001597500002));
#169281=CARTESIAN_POINT('Ctrl Pts',(7.03988054999994,11.6,-8.76001597500002));
#169282=CARTESIAN_POINT('Ctrl Pts',(7.03894460699994,15.2,-8.75668671600002));
#169283=CARTESIAN_POINT('Ctrl Pts',(7.03894460699994,11.6,-8.75668671600002));
#169284=CARTESIAN_POINT('Ctrl Pts',(7.03800735599994,15.2,-8.75336281500001));
#169285=CARTESIAN_POINT('Ctrl Pts',(7.03800735599994,11.6,-8.75336281500001));
#169286=CARTESIAN_POINT('Ctrl Pts',(7.03706880199994,15.2,-8.75004428000001));
#169287=CARTESIAN_POINT('Ctrl Pts',(7.03706880199994,11.6,-8.75004428000001));
#169288=CARTESIAN_POINT('Ctrl Pts',(7.03612895599995,15.2,-8.74673111600002));
#169289=CARTESIAN_POINT('Ctrl Pts',(7.03612895599995,11.6,-8.74673111600002));
#169290=CARTESIAN_POINT('Ctrl Pts',(7.03518782499994,15.2,-8.74342333000002));
#169291=CARTESIAN_POINT('Ctrl Pts',(7.03518782499994,11.6,-8.74342333000002));
#169292=CARTESIAN_POINT('Ctrl Pts',(7.03424541799994,15.2,-8.74012092800001));
#169293=CARTESIAN_POINT('Ctrl Pts',(7.03424541799994,11.6,-8.74012092800001));
#169294=CARTESIAN_POINT('Ctrl Pts',(7.03330174299994,15.2,-8.73682391500001));
#169295=CARTESIAN_POINT('Ctrl Pts',(7.03330174299994,11.6,-8.73682391500001));
#169296=CARTESIAN_POINT('Ctrl Pts',(7.03235680899994,15.2,-8.73353229700001));
#169297=CARTESIAN_POINT('Ctrl Pts',(7.03235680899994,11.6,-8.73353229700001));
#169298=CARTESIAN_POINT('Ctrl Pts',(7.03141062299995,15.2,-8.73024608200001));
#169299=CARTESIAN_POINT('Ctrl Pts',(7.03141062299995,11.6,-8.73024608200001));
#169300=CARTESIAN_POINT('Ctrl Pts',(7.03046319299995,15.2,-8.72696527400001));
#169301=CARTESIAN_POINT('Ctrl Pts',(7.03046319299995,11.6,-8.72696527400001));
#169302=CARTESIAN_POINT('Ctrl Pts',(7.02951453099994,15.2,-8.72368987800002));
#169303=CARTESIAN_POINT('Ctrl Pts',(7.02951453099994,11.6,-8.72368987800002));
#169304=CARTESIAN_POINT('Ctrl Pts',(7.02856464099994,15.2,-8.72041990300002));
#169305=CARTESIAN_POINT('Ctrl Pts',(7.02856464099994,11.6,-8.72041990300002));
#169306=CARTESIAN_POINT('Ctrl Pts',(7.02761353399994,15.2,-8.71715535200002));
#169307=CARTESIAN_POINT('Ctrl Pts',(7.02761353399994,11.6,-8.71715535200002));
#169308=CARTESIAN_POINT('Ctrl Pts',(7.02666121799994,15.2,-8.71389623300002));
#169309=CARTESIAN_POINT('Ctrl Pts',(7.02666121799994,11.6,-8.71389623300002));
#169310=CARTESIAN_POINT('Ctrl Pts',(7.02570770099994,15.2,-8.71064255100002));
#169311=CARTESIAN_POINT('Ctrl Pts',(7.02570770099994,11.6,-8.71064255100002));
#169312=CARTESIAN_POINT('Ctrl Pts',(7.02475299199994,15.2,-8.70739431300001));
#169313=CARTESIAN_POINT('Ctrl Pts',(7.02475299199994,11.6,-8.70739431300001));
#169314=CARTESIAN_POINT('Ctrl Pts',(7.02379709999994,15.2,-8.70415152400002));
#169315=CARTESIAN_POINT('Ctrl Pts',(7.02379709999994,11.6,-8.70415152400002));
#169316=CARTESIAN_POINT('Ctrl Pts',(7.02284003299994,15.2,-8.70091419100002));
#169317=CARTESIAN_POINT('Ctrl Pts',(7.02284003299994,11.6,-8.70091419100002));
#169318=CARTESIAN_POINT('Ctrl Pts',(7.02188179799994,15.2,-8.69768231900002));
#169319=CARTESIAN_POINT('Ctrl Pts',(7.02188179799994,11.6,-8.69768231900002));
#169320=CARTESIAN_POINT('Ctrl Pts',(7.02092240599994,15.2,-8.69445591400002));
#169321=CARTESIAN_POINT('Ctrl Pts',(7.02092240599994,11.6,-8.69445591400002));
#169322=CARTESIAN_POINT('Ctrl Pts',(7.01996186499994,15.2,-8.69123498300001));
#169323=CARTESIAN_POINT('Ctrl Pts',(7.01996186499994,11.6,-8.69123498300001));
#169324=CARTESIAN_POINT('Ctrl Pts',(7.01900018299995,15.2,-8.68801953100002));
#169325=CARTESIAN_POINT('Ctrl Pts',(7.01900018299995,11.6,-8.68801953100002));
#169326=CARTESIAN_POINT('Ctrl Pts',(7.01803736899994,15.2,-8.68480956600001));
#169327=CARTESIAN_POINT('Ctrl Pts',(7.01803736899994,11.6,-8.68480956600001));
#169328=CARTESIAN_POINT('Ctrl Pts',(7.01707343299995,15.2,-8.68160509100001));
#169329=CARTESIAN_POINT('Ctrl Pts',(7.01707343299995,11.6,-8.68160509100001));
#169330=CARTESIAN_POINT('Ctrl Pts',(7.01610838099994,15.2,-8.67840611400002));
#169331=CARTESIAN_POINT('Ctrl Pts',(7.01610838099994,11.6,-8.67840611400002));
#169332=CARTESIAN_POINT('Ctrl Pts',(7.01514222399994,15.2,-8.67521264000001));
#169333=CARTESIAN_POINT('Ctrl Pts',(7.01514222399994,11.6,-8.67521264000001));
#169334=CARTESIAN_POINT('Ctrl Pts',(7.01417496999994,15.2,-8.67202467700002));
#169335=CARTESIAN_POINT('Ctrl Pts',(7.01417496999994,11.6,-8.67202467700002));
#169336=CARTESIAN_POINT('Ctrl Pts',(7.01320662599994,15.2,-8.66884222900002));
#169337=CARTESIAN_POINT('Ctrl Pts',(7.01320662599994,11.6,-8.66884222900002));
#169338=CARTESIAN_POINT('Ctrl Pts',(7.01223720399994,15.2,-8.66566530400002));
#169339=CARTESIAN_POINT('Ctrl Pts',(7.01223720399994,11.6,-8.66566530400002));
#169340=CARTESIAN_POINT('Ctrl Pts',(7.01126671099995,15.2,-8.66249390500002));
#169341=CARTESIAN_POINT('Ctrl Pts',(7.01126671099995,11.6,-8.66249390500002));
#169342=CARTESIAN_POINT('Ctrl Pts',(7.01029515599994,15.2,-8.65932804100002));
#169343=CARTESIAN_POINT('Ctrl Pts',(7.01029515599994,11.6,-8.65932804100002));
#169344=CARTESIAN_POINT('Ctrl Pts',(7.00932254799994,15.2,-8.65616771800001));
#169345=CARTESIAN_POINT('Ctrl Pts',(7.00932254799994,11.6,-8.65616771800001));
#169346=CARTESIAN_POINT('Ctrl Pts',(7.00834889699994,15.2,-8.65301294000002));
#169347=CARTESIAN_POINT('Ctrl Pts',(7.00834889699994,11.6,-8.65301294000002));
#169348=CARTESIAN_POINT('Ctrl Pts',(7.00737420899994,15.2,-8.64986371400001));
#169349=CARTESIAN_POINT('Ctrl Pts',(7.00737420899994,11.6,-8.64986371400001));
#169350=CARTESIAN_POINT('Ctrl Pts',(7.00639849599995,15.2,-8.64672004800001));
#169351=CARTESIAN_POINT('Ctrl Pts',(7.00639849599995,11.6,-8.64672004800001));
#169352=CARTESIAN_POINT('Ctrl Pts',(7.00542176599994,15.2,-8.64358194500002));
#169353=CARTESIAN_POINT('Ctrl Pts',(7.00542176599994,11.6,-8.64358194500002));
#169354=CARTESIAN_POINT('Ctrl Pts',(7.00444402699994,15.2,-8.64044941300002));
#169355=CARTESIAN_POINT('Ctrl Pts',(7.00444402699994,11.6,-8.64044941300002));
#169356=CARTESIAN_POINT('Ctrl Pts',(7.00346528799995,15.2,-8.63732245800002));
#169357=CARTESIAN_POINT('Ctrl Pts',(7.00346528799995,11.6,-8.63732245800002));
#169358=CARTESIAN_POINT('Ctrl Pts',(7.00248555899995,15.2,-8.63420108600002));
#169359=CARTESIAN_POINT('Ctrl Pts',(7.00248555899995,11.6,-8.63420108600002));
#169360=CARTESIAN_POINT('Ctrl Pts',(7.00150484899994,15.2,-8.63108530300002));
#169361=CARTESIAN_POINT('Ctrl Pts',(7.00150484899994,11.6,-8.63108530300002));
#169362=CARTESIAN_POINT('Ctrl Pts',(7.00052316699994,15.2,-8.62797511400002));
#169363=CARTESIAN_POINT('Ctrl Pts',(7.00052316699994,11.6,-8.62797511400002));
#169364=CARTESIAN_POINT('Ctrl Pts',(6.99954052099995,15.2,-8.62487052700001));
#169365=CARTESIAN_POINT('Ctrl Pts',(6.99954052099995,11.6,-8.62487052700001));
#169366=CARTESIAN_POINT('Ctrl Pts',(6.99855692199994,15.2,-8.62177154700002));
#169367=CARTESIAN_POINT('Ctrl Pts',(6.99855692199994,11.6,-8.62177154700002));
#169368=CARTESIAN_POINT('Ctrl Pts',(6.99757237899994,15.2,-8.61867818100002));
#169369=CARTESIAN_POINT('Ctrl Pts',(6.99757237899994,11.6,-8.61867818100002));
#169370=CARTESIAN_POINT('Ctrl Pts',(6.99658689799994,15.2,-8.61559043400002));
#169371=CARTESIAN_POINT('Ctrl Pts',(6.99658689799994,11.6,-8.61559043400002));
#169372=CARTESIAN_POINT('Ctrl Pts',(6.99560049199994,15.2,-8.61250831300002));
#169373=CARTESIAN_POINT('Ctrl Pts',(6.99560049199994,11.6,-8.61250831300002));
#169374=CARTESIAN_POINT('Ctrl Pts',(6.99461316799994,15.2,-8.60943182400002));
#169375=CARTESIAN_POINT('Ctrl Pts',(6.99461316799994,11.6,-8.60943182400002));
#169376=CARTESIAN_POINT('Ctrl Pts',(6.99362493699994,15.2,-8.60636097400001));
#169377=CARTESIAN_POINT('Ctrl Pts',(6.99362493699994,11.6,-8.60636097400001));
#169378=CARTESIAN_POINT('Ctrl Pts',(6.99263580599994,15.2,-8.60329576700002));
#169379=CARTESIAN_POINT('Ctrl Pts',(6.99263580599994,11.6,-8.60329576700002));
#169380=CARTESIAN_POINT('Ctrl Pts',(6.99164578499994,15.2,-8.60023621100002));
#169381=CARTESIAN_POINT('Ctrl Pts',(6.99164578499994,11.6,-8.60023621100002));
#169382=CARTESIAN_POINT('Ctrl Pts',(6.99065488599994,15.2,-8.59718231200001));
#169383=CARTESIAN_POINT('Ctrl Pts',(6.99065488599994,11.6,-8.59718231200001));
#169384=CARTESIAN_POINT('Ctrl Pts',(6.98966311399994,15.2,-8.59413407600002));
#169385=CARTESIAN_POINT('Ctrl Pts',(6.98966311399994,11.6,-8.59413407600002));
#169386=CARTESIAN_POINT('Ctrl Pts',(6.98867048099994,15.2,-8.59109150800002));
#169387=CARTESIAN_POINT('Ctrl Pts',(6.98867048099994,11.6,-8.59109150800002));
#169388=CARTESIAN_POINT('Ctrl Pts',(6.98767699599994,15.2,-8.58805461600002));
#169389=CARTESIAN_POINT('Ctrl Pts',(6.98767699599994,11.6,-8.58805461600002));
#169390=CARTESIAN_POINT('Ctrl Pts',(6.98668266799994,15.2,-8.58502340600002));
#169391=CARTESIAN_POINT('Ctrl Pts',(6.98668266799994,11.6,-8.58502340600002));
#169392=CARTESIAN_POINT('Ctrl Pts',(6.98568750699994,15.2,-8.58199788300002));
#169393=CARTESIAN_POINT('Ctrl Pts',(6.98568750699994,11.6,-8.58199788300002));
#169394=CARTESIAN_POINT('Ctrl Pts',(6.98469152199994,15.2,-8.57897805400002));
#169395=CARTESIAN_POINT('Ctrl Pts',(6.98469152199994,11.6,-8.57897805400002));
#169396=CARTESIAN_POINT('Ctrl Pts',(6.98369472199994,15.2,-8.57596392400002));
#169397=CARTESIAN_POINT('Ctrl Pts',(6.98369472199994,11.6,-8.57596392400002));
#169398=CARTESIAN_POINT('Ctrl Pts',(6.98269711799994,15.2,-8.57295550200002));
#169399=CARTESIAN_POINT('Ctrl Pts',(6.98269711799994,11.6,-8.57295550200002));
#169400=CARTESIAN_POINT('Ctrl Pts',(6.98169871799994,15.2,-8.56995279200002));
#169401=CARTESIAN_POINT('Ctrl Pts',(6.98169871799994,11.6,-8.56995279200002));
#169402=CARTESIAN_POINT('Ctrl Pts',(6.98069953199994,15.2,-8.56695580000002));
#169403=CARTESIAN_POINT('Ctrl Pts',(6.98069953199994,11.6,-8.56695580000002));
#169404=CARTESIAN_POINT('Ctrl Pts',(6.97969957099994,15.2,-8.56396453400002));
#169405=CARTESIAN_POINT('Ctrl Pts',(6.97969957099994,11.6,-8.56396453400002));
#169406=CARTESIAN_POINT('Ctrl Pts',(6.97869884199994,15.2,-8.56097899900002));
#169407=CARTESIAN_POINT('Ctrl Pts',(6.97869884199994,11.6,-8.56097899900002));
#169408=CARTESIAN_POINT('Ctrl Pts',(6.97769735699994,15.2,-8.55799920200001));
#169409=CARTESIAN_POINT('Ctrl Pts',(6.97769735699994,11.6,-8.55799920200001));
#169410=CARTESIAN_POINT('Ctrl Pts',(6.97669512399994,15.2,-8.55502514800002));
#169411=CARTESIAN_POINT('Ctrl Pts',(6.97669512399994,11.6,-8.55502514800002));
#169412=CARTESIAN_POINT('Ctrl Pts',(6.97569215299994,15.2,-8.55205684500002));
#169413=CARTESIAN_POINT('Ctrl Pts',(6.97569215299994,11.6,-8.55205684500002));
#169414=CARTESIAN_POINT('Ctrl Pts',(6.97468845399994,15.2,-8.54909429700001));
#169415=CARTESIAN_POINT('Ctrl Pts',(6.97468845399994,11.6,-8.54909429700001));
#169416=CARTESIAN_POINT('Ctrl Pts',(6.97368403699994,15.2,-8.54613751400001));
#169417=CARTESIAN_POINT('Ctrl Pts',(6.97368403699994,11.6,-8.54613751400001));
#169418=CARTESIAN_POINT('Ctrl Pts',(6.97267891199994,15.2,-8.54318649800001));
#169419=CARTESIAN_POINT('Ctrl Pts',(6.97267891199994,11.6,-8.54318649800001));
#169420=CARTESIAN_POINT('Ctrl Pts',(6.97167308699994,15.2,-8.54024125700001));
#169421=CARTESIAN_POINT('Ctrl Pts',(6.97167308699994,11.6,-8.54024125700001));
#169422=CARTESIAN_POINT('Ctrl Pts',(6.97066657399994,15.2,-8.53730179900002));
#169423=CARTESIAN_POINT('Ctrl Pts',(6.97066657399994,11.6,-8.53730179900002));
#169424=CARTESIAN_POINT('Ctrl Pts',(6.96965938299994,15.2,-8.53436812800001));
#169425=CARTESIAN_POINT('Ctrl Pts',(6.96965938299994,11.6,-8.53436812800001));
#169426=CARTESIAN_POINT('Ctrl Pts',(6.96865152099994,15.2,-8.53144025000002));
#169427=CARTESIAN_POINT('Ctrl Pts',(6.96865152099994,11.6,-8.53144025000002));
#169428=CARTESIAN_POINT('Ctrl Pts',(6.96764299999994,15.2,-8.52851817400002));
#169429=CARTESIAN_POINT('Ctrl Pts',(6.96764299999994,11.6,-8.52851817400002));
#169430=CARTESIAN_POINT('Ctrl Pts',(6.96663382999994,15.2,-8.52560190500002));
#169431=CARTESIAN_POINT('Ctrl Pts',(6.96663382999994,11.6,-8.52560190500002));
#169432=CARTESIAN_POINT('Ctrl Pts',(6.96562401999994,15.2,-8.52269144800001));
#169433=CARTESIAN_POINT('Ctrl Pts',(6.96562401999994,11.6,-8.52269144800001));
#169434=CARTESIAN_POINT('Ctrl Pts',(6.96461357999994,15.2,-8.51978681100002));
#169435=CARTESIAN_POINT('Ctrl Pts',(6.96461357999994,11.6,-8.51978681100002));
#169436=CARTESIAN_POINT('Ctrl Pts',(6.96360252099994,15.2,-8.51688800000002));
#169437=CARTESIAN_POINT('Ctrl Pts',(6.96360252099994,11.6,-8.51688800000002));
#169438=CARTESIAN_POINT('Ctrl Pts',(6.96259085299994,15.2,-8.51399502000002));
#169439=CARTESIAN_POINT('Ctrl Pts',(6.96259085299994,11.6,-8.51399502000002));
#169440=CARTESIAN_POINT('Ctrl Pts',(6.96157858499994,15.2,-8.51110787900001));
#169441=CARTESIAN_POINT('Ctrl Pts',(6.96157858499994,11.6,-8.51110787900001));
#169442=CARTESIAN_POINT('Ctrl Pts',(6.96056572699994,15.2,-8.50822658400002));
#169443=CARTESIAN_POINT('Ctrl Pts',(6.96056572699994,11.6,-8.50822658400002));
#169444=CARTESIAN_POINT('Ctrl Pts',(6.95955229099994,15.2,-8.50535113900002));
#169445=CARTESIAN_POINT('Ctrl Pts',(6.95955229099994,11.6,-8.50535113900002));
#169446=CARTESIAN_POINT('Ctrl Pts',(6.95853828499994,15.2,-8.50248155200001));
#169447=CARTESIAN_POINT('Ctrl Pts',(6.95853828499994,11.6,-8.50248155200001));
#169448=CARTESIAN_POINT('Ctrl Pts',(6.95752371999995,15.2,-8.49961782800002));
#169449=CARTESIAN_POINT('Ctrl Pts',(6.95752371999995,11.6,-8.49961782800002));
#169450=CARTESIAN_POINT('Ctrl Pts',(6.95650860599994,15.2,-8.49675997600002));
#169451=CARTESIAN_POINT('Ctrl Pts',(6.95650860599994,11.6,-8.49675997600002));
#169452=CARTESIAN_POINT('Ctrl Pts',(6.95549295399994,15.2,-8.49390799900002));
#169453=CARTESIAN_POINT('Ctrl Pts',(6.95549295399994,11.6,-8.49390799900002));
#169454=CARTESIAN_POINT('Ctrl Pts',(6.95447677299994,15.2,-8.49106190600001));
#169455=CARTESIAN_POINT('Ctrl Pts',(6.95447677299994,11.6,-8.49106190600001));
#169456=CARTESIAN_POINT('Ctrl Pts',(6.95346007499994,15.2,-8.48822170300001));
#169457=CARTESIAN_POINT('Ctrl Pts',(6.95346007499994,11.6,-8.48822170300001));
#169458=CARTESIAN_POINT('Ctrl Pts',(6.95244286799994,15.2,-8.48538739600002));
#169459=CARTESIAN_POINT('Ctrl Pts',(6.95244286799994,11.6,-8.48538739600002));
#169460=CARTESIAN_POINT('Ctrl Pts',(6.95142516299994,15.2,-8.48255899100002));
#169461=CARTESIAN_POINT('Ctrl Pts',(6.95142516299994,11.6,-8.48255899100002));
#169462=CARTESIAN_POINT('Ctrl Pts',(6.95040697199994,15.2,-8.47973649400002));
#169463=CARTESIAN_POINT('Ctrl Pts',(6.95040697199994,11.6,-8.47973649400002));
#169464=CARTESIAN_POINT('Ctrl Pts',(6.94938830399995,15.2,-8.47691991200002));
#169465=CARTESIAN_POINT('Ctrl Pts',(6.94938830399995,11.6,-8.47691991200002));
#169466=CARTESIAN_POINT('Ctrl Pts',(6.94836916999994,15.2,-8.47410925300002));
#169467=CARTESIAN_POINT('Ctrl Pts',(6.94836916999994,11.6,-8.47410925300002));
#169468=CARTESIAN_POINT('Ctrl Pts',(6.94734957799994,15.2,-8.47130452200001));
#169469=CARTESIAN_POINT('Ctrl Pts',(6.94734957799994,11.6,-8.47130452200001));
#169470=CARTESIAN_POINT('Ctrl Pts',(6.94632954299994,15.2,-8.46850572500001));
#169471=CARTESIAN_POINT('Ctrl Pts',(6.94632954299994,11.6,-8.46850572500001));
#169472=CARTESIAN_POINT('Ctrl Pts',(6.94530907199994,15.2,-8.46571286900001));
#169473=CARTESIAN_POINT('Ctrl Pts',(6.94530907199994,11.6,-8.46571286900001));
#169474=CARTESIAN_POINT('Ctrl Pts',(6.94428817599994,15.2,-8.46292596000002));
#169475=CARTESIAN_POINT('Ctrl Pts',(6.94428817599994,11.6,-8.46292596000002));
#169476=CARTESIAN_POINT('Ctrl Pts',(6.94326686599994,15.2,-8.46014500600001));
#169477=CARTESIAN_POINT('Ctrl Pts',(6.94326686599994,11.6,-8.46014500600001));
#169478=CARTESIAN_POINT('Ctrl Pts',(6.94224515399994,15.2,-8.45737001200002));
#169479=CARTESIAN_POINT('Ctrl Pts',(6.94224515399994,11.6,-8.45737001200002));
#169480=CARTESIAN_POINT('Ctrl Pts',(6.94122304799994,15.2,-8.45460098400002));
#169481=CARTESIAN_POINT('Ctrl Pts',(6.94122304799994,11.6,-8.45460098400002));
#169482=CARTESIAN_POINT('Ctrl Pts',(6.94020055999995,15.2,-8.45183793000002));
#169483=CARTESIAN_POINT('Ctrl Pts',(6.94020055999995,11.6,-8.45183793000002));
#169484=CARTESIAN_POINT('Ctrl Pts',(6.93917770099994,15.2,-8.44908085600002));
#169485=CARTESIAN_POINT('Ctrl Pts',(6.93917770099994,11.6,-8.44908085600002));
#169486=CARTESIAN_POINT('Ctrl Pts',(6.93815448099994,15.2,-8.44632976900002));
#169487=CARTESIAN_POINT('Ctrl Pts',(6.93815448099994,11.6,-8.44632976900002));
#169488=CARTESIAN_POINT('Ctrl Pts',(6.93713091199994,15.2,-8.44358467400001));
#169489=CARTESIAN_POINT('Ctrl Pts',(6.93713091199994,11.6,-8.44358467400001));
#169490=CARTESIAN_POINT('Ctrl Pts',(6.93610700299994,15.2,-8.44084557900001));
#169491=CARTESIAN_POINT('Ctrl Pts',(6.93610700299994,11.6,-8.44084557900001));
#169492=CARTESIAN_POINT('Ctrl Pts',(6.93508276499994,15.2,-8.43811248900002));
#169493=CARTESIAN_POINT('Ctrl Pts',(6.93508276499994,11.6,-8.43811248900002));
#169494=CARTESIAN_POINT('Ctrl Pts',(6.93405820999994,15.2,-8.43538541100001));
#169495=CARTESIAN_POINT('Ctrl Pts',(6.93405820999994,11.6,-8.43538541100001));
#169496=CARTESIAN_POINT('Ctrl Pts',(6.93303334799994,15.2,-8.43266435400002));
#169497=CARTESIAN_POINT('Ctrl Pts',(6.93303334799994,11.6,-8.43266435400002));
#169498=CARTESIAN_POINT('Ctrl Pts',(6.93200819099994,15.2,-8.42994932100002));
#169499=CARTESIAN_POINT('Ctrl Pts',(6.93200819099994,11.6,-8.42994932100002));
#169500=CARTESIAN_POINT('Ctrl Pts',(6.93098274699994,15.2,-8.42724032100002));
#169501=CARTESIAN_POINT('Ctrl Pts',(6.93098274699994,11.6,-8.42724032100002));
#169502=CARTESIAN_POINT('Ctrl Pts',(6.92995702999994,15.2,-8.42453735900002));
#169503=CARTESIAN_POINT('Ctrl Pts',(6.92995702999994,11.6,-8.42453735900002));
#169504=CARTESIAN_POINT('Ctrl Pts',(6.92893105099994,15.2,-8.42184044300001));
#169505=CARTESIAN_POINT('Ctrl Pts',(6.92893105099994,11.6,-8.42184044300001));
#169506=CARTESIAN_POINT('Ctrl Pts',(6.92790481799994,15.2,-8.41914957800002));
#169507=CARTESIAN_POINT('Ctrl Pts',(6.92790481799994,11.6,-8.41914957800002));
#169508=CARTESIAN_POINT('Ctrl Pts',(6.92687834499995,15.2,-8.41646477200002));
#169509=CARTESIAN_POINT('Ctrl Pts',(6.92687834499995,11.6,-8.41646477200002));
#169510=CARTESIAN_POINT('Ctrl Pts',(6.92585164099994,15.2,-8.41378603000001));
#169511=CARTESIAN_POINT('Ctrl Pts',(6.92585164099994,11.6,-8.41378603000001));
#169512=CARTESIAN_POINT('Ctrl Pts',(6.92482471899995,15.2,-8.41111336100001));
#169513=CARTESIAN_POINT('Ctrl Pts',(6.92482471899995,11.6,-8.41111336100001));
#169514=CARTESIAN_POINT('Ctrl Pts',(6.92379758999994,15.2,-8.40844676800002));
#169515=CARTESIAN_POINT('Ctrl Pts',(6.92379758999994,11.6,-8.40844676800002));
#169516=CARTESIAN_POINT('Ctrl Pts',(6.92277026199994,15.2,-8.40578626200001));
#169517=CARTESIAN_POINT('Ctrl Pts',(6.92277026199994,11.6,-8.40578626200001));
#169518=CARTESIAN_POINT('Ctrl Pts',(6.92174274999994,15.2,-8.40313184700002));
#169519=CARTESIAN_POINT('Ctrl Pts',(6.92174274999994,11.6,-8.40313184700002));
#169520=CARTESIAN_POINT('Ctrl Pts',(6.92071506399994,15.2,-8.40048352900002));
#169521=CARTESIAN_POINT('Ctrl Pts',(6.92071506399994,11.6,-8.40048352900002));
#169522=CARTESIAN_POINT('Ctrl Pts',(6.91968721499994,15.2,-8.39784131600002));
#169523=CARTESIAN_POINT('Ctrl Pts',(6.91968721499994,11.6,-8.39784131600002));
#169524=CARTESIAN_POINT('Ctrl Pts',(6.91865921499994,15.2,-8.39520521500001));
#169525=CARTESIAN_POINT('Ctrl Pts',(6.91865921499994,11.6,-8.39520521500001));
#169526=CARTESIAN_POINT('Ctrl Pts',(6.91763107299994,15.2,-8.39257523200001));
#169527=CARTESIAN_POINT('Ctrl Pts',(6.91763107299994,11.6,-8.39257523200001));
#169528=CARTESIAN_POINT('Ctrl Pts',(6.91660280299994,15.2,-8.38995137300002));
#169529=CARTESIAN_POINT('Ctrl Pts',(6.91660280299994,11.6,-8.38995137300002));
#169530=CARTESIAN_POINT('Ctrl Pts',(6.91557441499994,15.2,-8.38733364600002));
#169531=CARTESIAN_POINT('Ctrl Pts',(6.91557441499994,11.6,-8.38733364600002));
#169532=CARTESIAN_POINT('Ctrl Pts',(6.91454591999995,15.2,-8.38472205600001));
#169533=CARTESIAN_POINT('Ctrl Pts',(6.91454591999995,11.6,-8.38472205600001));
#169534=CARTESIAN_POINT('Ctrl Pts',(6.91351733199994,15.2,-8.38211661100001));
#169535=CARTESIAN_POINT('Ctrl Pts',(6.91351733199994,11.6,-8.38211661100001));
#169536=CARTESIAN_POINT('Ctrl Pts',(6.91248865999994,15.2,-8.37951731700001));
#169537=CARTESIAN_POINT('Ctrl Pts',(6.91248865999994,11.6,-8.37951731700001));
#169538=CARTESIAN_POINT('Ctrl Pts',(6.91145991499994,15.2,-8.37692418200002));
#169539=CARTESIAN_POINT('Ctrl Pts',(6.91145991499994,11.6,-8.37692418200002));
#169540=CARTESIAN_POINT('Ctrl Pts',(6.91043111099994,15.2,-8.37433721000002));
#169541=CARTESIAN_POINT('Ctrl Pts',(6.91043111099994,11.6,-8.37433721000002));
#169542=CARTESIAN_POINT('Ctrl Pts',(6.90940225899995,15.2,-8.37175641100002));
#169543=CARTESIAN_POINT('Ctrl Pts',(6.90940225899995,11.6,-8.37175641100002));
#169544=CARTESIAN_POINT('Ctrl Pts',(6.90837336899994,15.2,-8.36918179000002));
#169545=CARTESIAN_POINT('Ctrl Pts',(6.90837336899994,11.6,-8.36918179000002));
#169546=CARTESIAN_POINT('Ctrl Pts',(6.90734445199994,15.2,-8.36661335300001));
#169547=CARTESIAN_POINT('Ctrl Pts',(6.90734445199994,11.6,-8.36661335300001));
#169548=CARTESIAN_POINT('Ctrl Pts',(6.90631552399994,15.2,-8.36405110800002));
#169549=CARTESIAN_POINT('Ctrl Pts',(6.90631552399994,11.6,-8.36405110800002));
#169550=CARTESIAN_POINT('Ctrl Pts',(6.90528659299994,15.2,-8.36149506200002));
#169551=CARTESIAN_POINT('Ctrl Pts',(6.90528659299994,11.6,-8.36149506200002));
#169552=CARTESIAN_POINT('Ctrl Pts',(6.90425767199994,15.2,-8.35894522000002));
#169553=CARTESIAN_POINT('Ctrl Pts',(6.90425767199994,11.6,-8.35894522000002));
#169554=CARTESIAN_POINT('Ctrl Pts',(6.90322877199994,15.2,-8.35640159100001));
#169555=CARTESIAN_POINT('Ctrl Pts',(6.90322877199994,11.6,-8.35640159100001));
#169556=CARTESIAN_POINT('Ctrl Pts',(6.90219990499994,15.2,-8.35386418100001));
#169557=CARTESIAN_POINT('Ctrl Pts',(6.90219990499994,11.6,-8.35386418100001));
#169558=CARTESIAN_POINT('Ctrl Pts',(6.90117108399994,15.2,-8.35133299500002));
#169559=CARTESIAN_POINT('Ctrl Pts',(6.90117108399994,11.6,-8.35133299500002));
#169560=CARTESIAN_POINT('Ctrl Pts',(6.90014232099994,15.2,-8.34880804200001));
#169561=CARTESIAN_POINT('Ctrl Pts',(6.90014232099994,11.6,-8.34880804200001));
#169562=CARTESIAN_POINT('Ctrl Pts',(6.89911362499994,15.2,-8.34628932700002));
#169563=CARTESIAN_POINT('Ctrl Pts',(6.89911362499994,11.6,-8.34628932700002));
#169564=CARTESIAN_POINT('Ctrl Pts',(6.89808501099994,15.2,-8.34377685900002));
#169565=CARTESIAN_POINT('Ctrl Pts',(6.89808501099994,11.6,-8.34377685900002));
#169566=CARTESIAN_POINT('Ctrl Pts',(6.89705648999994,15.2,-8.34127064300001));
#169567=CARTESIAN_POINT('Ctrl Pts',(6.89705648999994,11.6,-8.34127064300001));
#169568=CARTESIAN_POINT('Ctrl Pts',(6.89602807299995,15.2,-8.33877068600002));
#169569=CARTESIAN_POINT('Ctrl Pts',(6.89602807299995,11.6,-8.33877068600002));
#169570=CARTESIAN_POINT('Ctrl Pts',(6.89499977499994,15.2,-8.33627699600001));
#169571=CARTESIAN_POINT('Ctrl Pts',(6.89499977499994,11.6,-8.33627699600001));
#169572=CARTESIAN_POINT('Ctrl Pts',(6.89397160499994,15.2,-8.33378957900001));
#169573=CARTESIAN_POINT('Ctrl Pts',(6.89397160499994,11.6,-8.33378957900001));
#169574=CARTESIAN_POINT('Ctrl Pts',(6.89294357699994,15.2,-8.33130844200002));
#169575=CARTESIAN_POINT('Ctrl Pts',(6.89294357699994,11.6,-8.33130844200002));
#169576=CARTESIAN_POINT('Ctrl Pts',(6.89191570099994,15.2,-8.32883359100002));
#169577=CARTESIAN_POINT('Ctrl Pts',(6.89191570099994,11.6,-8.32883359100002));
#169578=CARTESIAN_POINT('Ctrl Pts',(6.89088799199994,15.2,-8.32636503500002));
#169579=CARTESIAN_POINT('Ctrl Pts',(6.89088799199994,11.6,-8.32636503500002));
#169580=CARTESIAN_POINT('Ctrl Pts',(6.88986046099994,15.2,-8.32390277900002));
#169581=CARTESIAN_POINT('Ctrl Pts',(6.88986046099994,11.6,-8.32390277900002));
#169582=CARTESIAN_POINT('Ctrl Pts',(6.88883311899994,15.2,-8.32144682900001));
#169583=CARTESIAN_POINT('Ctrl Pts',(6.88883311899994,11.6,-8.32144682900001));
#169584=CARTESIAN_POINT('Ctrl Pts',(6.88780597999994,15.2,-8.31899719600001));
#169585=CARTESIAN_POINT('Ctrl Pts',(6.88780597999994,11.6,-8.31899719600001));
#169586=CARTESIAN_POINT('Ctrl Pts',(6.88677905699994,15.2,-8.31655388200002));
#169587=CARTESIAN_POINT('Ctrl Pts',(6.88677905699994,11.6,-8.31655388200002));
#169588=CARTESIAN_POINT('Ctrl Pts',(6.88575235999994,15.2,-8.31411689700002));
#169589=CARTESIAN_POINT('Ctrl Pts',(6.88575235999994,11.6,-8.31411689700002));
#169590=CARTESIAN_POINT('Ctrl Pts',(6.88472590399994,15.2,-8.31168624500001));
#169591=CARTESIAN_POINT('Ctrl Pts',(6.88472590399994,11.6,-8.31168624500001));
#169592=CARTESIAN_POINT('Ctrl Pts',(6.88369969899994,15.2,-8.30926193800002));
#169593=CARTESIAN_POINT('Ctrl Pts',(6.88369969899994,11.6,-8.30926193800002));
#169594=CARTESIAN_POINT('Ctrl Pts',(6.88267375899994,15.2,-8.30684397800002));
#169595=CARTESIAN_POINT('Ctrl Pts',(6.88267375899994,11.6,-8.30684397800002));
#169596=CARTESIAN_POINT('Ctrl Pts',(6.88164809599995,15.2,-8.30443237500001));
#169597=CARTESIAN_POINT('Ctrl Pts',(6.88164809599995,11.6,-8.30443237500001));
#169598=CARTESIAN_POINT('Ctrl Pts',(6.88062272399995,15.2,-8.30202713300002));
#169599=CARTESIAN_POINT('Ctrl Pts',(6.88062272399995,11.6,-8.30202713300002));
#169600=CARTESIAN_POINT('Ctrl Pts',(6.87959765299994,15.2,-8.29962826200001));
#169601=CARTESIAN_POINT('Ctrl Pts',(6.87959765299994,11.6,-8.29962826200001));
#169602=CARTESIAN_POINT('Ctrl Pts',(6.87857289699994,15.2,-8.29723576700001));
#169603=CARTESIAN_POINT('Ctrl Pts',(6.87857289699994,11.6,-8.29723576700001));
#169604=CARTESIAN_POINT('Ctrl Pts',(6.87754846999994,15.2,-8.29484965700001));
#169605=CARTESIAN_POINT('Ctrl Pts',(6.87754846999994,11.6,-8.29484965700001));
#169606=CARTESIAN_POINT('Ctrl Pts',(6.87652438199994,15.2,-8.29246993600002));
#169607=CARTESIAN_POINT('Ctrl Pts',(6.87652438199994,11.6,-8.29246993600002));
#169608=CARTESIAN_POINT('Ctrl Pts',(6.87550064899995,15.2,-8.29009661300002));
#169609=CARTESIAN_POINT('Ctrl Pts',(6.87550064899995,11.6,-8.29009661300002));
#169610=CARTESIAN_POINT('Ctrl Pts',(6.87447728099994,15.2,-8.28772969500001));
#169611=CARTESIAN_POINT('Ctrl Pts',(6.87447728099994,11.6,-8.28772969500001));
#169612=CARTESIAN_POINT('Ctrl Pts',(6.87345429199994,15.2,-8.28536918900001));
#169613=CARTESIAN_POINT('Ctrl Pts',(6.87345429199994,11.6,-8.28536918900001));
#169614=CARTESIAN_POINT('Ctrl Pts',(6.87243169499994,15.2,-8.28301510100001));
#169615=CARTESIAN_POINT('Ctrl Pts',(6.87243169499994,11.6,-8.28301510100001));
#169616=CARTESIAN_POINT('Ctrl Pts',(6.87140950299994,15.2,-8.28066743900001));
#169617=CARTESIAN_POINT('Ctrl Pts',(6.87140950299994,11.6,-8.28066743900001));
#169618=CARTESIAN_POINT('Ctrl Pts',(6.87038772899994,15.2,-8.27832621000002));
#169619=CARTESIAN_POINT('Ctrl Pts',(6.87038772899994,11.6,-8.27832621000002));
#169620=CARTESIAN_POINT('Ctrl Pts',(6.86936638499994,15.2,-8.27599142100001));
#169621=CARTESIAN_POINT('Ctrl Pts',(6.86936638499994,11.6,-8.27599142100001));
#169622=CARTESIAN_POINT('Ctrl Pts',(6.86834548499994,15.2,-8.27366307800002));
#169623=CARTESIAN_POINT('Ctrl Pts',(6.86834548499994,11.6,-8.27366307800002));
#169624=CARTESIAN_POINT('Ctrl Pts',(6.86732504299994,15.2,-8.27134119000002));
#169625=CARTESIAN_POINT('Ctrl Pts',(6.86732504299994,11.6,-8.27134119000002));
#169626=CARTESIAN_POINT('Ctrl Pts',(6.86630506999995,15.2,-8.26902576200002));
#169627=CARTESIAN_POINT('Ctrl Pts',(6.86630506999995,11.6,-8.26902576200002));
#169628=CARTESIAN_POINT('Ctrl Pts',(6.86528557999995,15.2,-8.26671680300001));
#169629=CARTESIAN_POINT('Ctrl Pts',(6.86528557999995,11.6,-8.26671680300001));
#169630=CARTESIAN_POINT('Ctrl Pts',(6.86426658699994,15.2,-8.26441431900001));
#169631=CARTESIAN_POINT('Ctrl Pts',(6.86426658699994,11.6,-8.26441431900001));
#169632=CARTESIAN_POINT('Ctrl Pts',(6.86324810299995,15.2,-8.26211831700002));
#169633=CARTESIAN_POINT('Ctrl Pts',(6.86324810299995,11.6,-8.26211831700002));
#169634=CARTESIAN_POINT('Ctrl Pts',(6.86223014199994,15.2,-8.25982880500002));
#169635=CARTESIAN_POINT('Ctrl Pts',(6.86223014199994,11.6,-8.25982880500002));
#169636=CARTESIAN_POINT('Ctrl Pts',(6.86121271699994,15.2,-8.25754578900002));
#169637=CARTESIAN_POINT('Ctrl Pts',(6.86121271699994,11.6,-8.25754578900002));
#169638=CARTESIAN_POINT('Ctrl Pts',(6.86019584299994,15.2,-8.25526927700002));
#169639=CARTESIAN_POINT('Ctrl Pts',(6.86019584299994,11.6,-8.25526927700002));
#169640=CARTESIAN_POINT('Ctrl Pts',(6.85917953099994,15.2,-8.25299927600001));
#169641=CARTESIAN_POINT('Ctrl Pts',(6.85917953099994,11.6,-8.25299927600001));
#169642=CARTESIAN_POINT('Ctrl Pts',(6.85816379599994,15.2,-8.25073579300001));
#169643=CARTESIAN_POINT('Ctrl Pts',(6.85816379599994,11.6,-8.25073579300001));
#169644=CARTESIAN_POINT('Ctrl Pts',(6.85714865199994,15.2,-8.24847883600001));
#169645=CARTESIAN_POINT('Ctrl Pts',(6.85714865199994,11.6,-8.24847883600001));
#169646=CARTESIAN_POINT('Ctrl Pts',(6.85613410999995,15.2,-8.24622841000001));
#169647=CARTESIAN_POINT('Ctrl Pts',(6.85613410999995,11.6,-8.24622841000001));
#169648=CARTESIAN_POINT('Ctrl Pts',(6.85512018599994,15.2,-8.24398452500001));
#169649=CARTESIAN_POINT('Ctrl Pts',(6.85512018599994,11.6,-8.24398452500001));
#169650=CARTESIAN_POINT('Ctrl Pts',(6.85410689299994,15.2,-8.24174718600002));
#169651=CARTESIAN_POINT('Ctrl Pts',(6.85410689299994,11.6,-8.24174718600002));
#169652=CARTESIAN_POINT('Ctrl Pts',(6.85309424499994,15.2,-8.23951640200002));
#169653=CARTESIAN_POINT('Ctrl Pts',(6.85309424499994,11.6,-8.23951640200002));
#169654=CARTESIAN_POINT('Ctrl Pts',(6.85208225499994,15.2,-8.23729217900001));
#169655=CARTESIAN_POINT('Ctrl Pts',(6.85208225499994,11.6,-8.23729217900001));
#169656=CARTESIAN_POINT('Ctrl Pts',(6.85107093599994,15.2,-8.23507452400002));
#169657=CARTESIAN_POINT('Ctrl Pts',(6.85107093599994,11.6,-8.23507452400002));
#169658=CARTESIAN_POINT('Ctrl Pts',(6.85006030399994,15.2,-8.23286344400002));
#169659=CARTESIAN_POINT('Ctrl Pts',(6.85006030399994,11.6,-8.23286344400002));
#169660=CARTESIAN_POINT('Ctrl Pts',(6.84905037099995,15.2,-8.23065895000001));
#169661=CARTESIAN_POINT('Ctrl Pts',(6.84905037099995,11.6,-8.23065895000001));
#169662=CARTESIAN_POINT('Ctrl Pts',(6.84804115199994,15.2,-8.22846104400002));
#169663=CARTESIAN_POINT('Ctrl Pts',(6.84804115199994,11.6,-8.22846104400002));
#169664=CARTESIAN_POINT('Ctrl Pts',(6.84703265999994,15.2,-8.22626973500002));
#169665=CARTESIAN_POINT('Ctrl Pts',(6.84703265999994,11.6,-8.22626973500002));
#169666=CARTESIAN_POINT('Ctrl Pts',(6.84602490999994,15.2,-8.22408503200002));
#169667=CARTESIAN_POINT('Ctrl Pts',(6.84602490999994,11.6,-8.22408503200002));
#169668=CARTESIAN_POINT('Ctrl Pts',(6.84501791499994,15.2,-8.22190694200001));
#169669=CARTESIAN_POINT('Ctrl Pts',(6.84501791499994,11.6,-8.22190694200001));
#169670=CARTESIAN_POINT('Ctrl Pts',(6.84401168999995,15.2,-8.21973547000002));
#169671=CARTESIAN_POINT('Ctrl Pts',(6.84401168999995,11.6,-8.21973547000002));
#169672=CARTESIAN_POINT('Ctrl Pts',(6.84300624899994,15.2,-8.21757062500001));
#169673=CARTESIAN_POINT('Ctrl Pts',(6.84300624899994,11.6,-8.21757062500001));
#169674=CARTESIAN_POINT('Ctrl Pts',(6.84200160499994,15.2,-8.21541241600002));
#169675=CARTESIAN_POINT('Ctrl Pts',(6.84200160499994,11.6,-8.21541241600002));
#169676=CARTESIAN_POINT('Ctrl Pts',(6.84099777399994,15.2,-8.21326084700001));
#169677=CARTESIAN_POINT('Ctrl Pts',(6.84099777399994,11.6,-8.21326084700001));
#169678=CARTESIAN_POINT('Ctrl Pts',(6.83999476999994,15.2,-8.21111592700002));
#169679=CARTESIAN_POINT('Ctrl Pts',(6.83999476999994,11.6,-8.21111592700002));
#169680=CARTESIAN_POINT('Ctrl Pts',(6.83899260499994,15.2,-8.20897766300002));
#169681=CARTESIAN_POINT('Ctrl Pts',(6.83899260499994,11.6,-8.20897766300002));
#169682=CARTESIAN_POINT('Ctrl Pts',(6.83799129699994,15.2,-8.20684606400001));
#169683=CARTESIAN_POINT('Ctrl Pts',(6.83799129699994,11.6,-8.20684606400001));
#169684=CARTESIAN_POINT('Ctrl Pts',(6.83699085699994,15.2,-8.20472113600001));
#169685=CARTESIAN_POINT('Ctrl Pts',(6.83699085699994,11.6,-8.20472113600001));
#169686=CARTESIAN_POINT('Ctrl Pts',(6.83599130199994,15.2,-8.20260288400002));
#169687=CARTESIAN_POINT('Ctrl Pts',(6.83599130199994,11.6,-8.20260288400002));
#169688=CARTESIAN_POINT('Ctrl Pts',(6.83499264499994,15.2,-8.20049132000002));
#169689=CARTESIAN_POINT('Ctrl Pts',(6.83499264499994,11.6,-8.20049132000002));
#169690=CARTESIAN_POINT('Ctrl Pts',(6.83399489999994,15.2,-8.19838644900001));
#169691=CARTESIAN_POINT('Ctrl Pts',(6.83399489999994,11.6,-8.19838644900001));
#169692=CARTESIAN_POINT('Ctrl Pts',(6.83299808299994,15.2,-8.19628827900001));
#169693=CARTESIAN_POINT('Ctrl Pts',(6.83299808299994,11.6,-8.19628827900001));
#169694=CARTESIAN_POINT('Ctrl Pts',(6.83200220999994,15.2,-8.19419681600002));
#169695=CARTESIAN_POINT('Ctrl Pts',(6.83200220999994,11.6,-8.19419681600002));
#169696=CARTESIAN_POINT('Ctrl Pts',(6.83100729199994,15.2,-8.19211207100001));
#169697=CARTESIAN_POINT('Ctrl Pts',(6.83100729199994,11.6,-8.19211207100001));
#169698=CARTESIAN_POINT('Ctrl Pts',(6.83001334499994,15.2,-8.19003404700002));
#169699=CARTESIAN_POINT('Ctrl Pts',(6.83001334499994,11.6,-8.19003404700002));
#169700=CARTESIAN_POINT('Ctrl Pts',(6.82902038699994,15.2,-8.18796275400001));
#169701=CARTESIAN_POINT('Ctrl Pts',(6.82902038699994,11.6,-8.18796275400001));
#169702=CARTESIAN_POINT('Ctrl Pts',(6.82802842799994,15.2,-8.18589820000001));
#169703=CARTESIAN_POINT('Ctrl Pts',(6.82802842799994,11.6,-8.18589820000001));
#169704=CARTESIAN_POINT('Ctrl Pts',(6.82703748599994,15.2,-8.18384039100001));
#169705=CARTESIAN_POINT('Ctrl Pts',(6.82703748599994,11.6,-8.18384039100001));
#169706=CARTESIAN_POINT('Ctrl Pts',(6.82604757499995,15.2,-8.18178933600001));
#169707=CARTESIAN_POINT('Ctrl Pts',(6.82604757499995,11.6,-8.18178933600001));
#169708=CARTESIAN_POINT('Ctrl Pts',(6.82505870999995,15.2,-8.17974504100001));
#169709=CARTESIAN_POINT('Ctrl Pts',(6.82505870999995,11.6,-8.17974504100001));
#169710=CARTESIAN_POINT('Ctrl Pts',(6.82407090599995,15.2,-8.17770751500002));
#169711=CARTESIAN_POINT('Ctrl Pts',(6.82407090599995,11.6,-8.17770751500002));
#169712=CARTESIAN_POINT('Ctrl Pts',(6.82308417899994,15.2,-8.17567676500002));
#169713=CARTESIAN_POINT('Ctrl Pts',(6.82308417899994,11.6,-8.17567676500002));
#169714=CARTESIAN_POINT('Ctrl Pts',(6.82209854199994,15.2,-8.17365279700002));
#169715=CARTESIAN_POINT('Ctrl Pts',(6.82209854199994,11.6,-8.17365279700002));
#169716=CARTESIAN_POINT('Ctrl Pts',(6.82111401199994,15.2,-8.17163562200001));
#169717=CARTESIAN_POINT('Ctrl Pts',(6.82111401199994,11.6,-8.17163562200001));
#169718=CARTESIAN_POINT('Ctrl Pts',(6.82013060499994,15.2,-8.16962524400001));
#169719=CARTESIAN_POINT('Ctrl Pts',(6.82013060499994,11.6,-8.16962524400001));
#169720=CARTESIAN_POINT('Ctrl Pts',(6.81914833299994,15.2,-8.16762167300002));
#169721=CARTESIAN_POINT('Ctrl Pts',(6.81914833299994,11.6,-8.16762167300002));
#169722=CARTESIAN_POINT('Ctrl Pts',(6.81816721399994,15.2,-8.16562491600001));
#169723=CARTESIAN_POINT('Ctrl Pts',(6.81816721399994,11.6,-8.16562491600001));
#169724=CARTESIAN_POINT('Ctrl Pts',(6.81718726299994,15.2,-8.16363498000002));
#169725=CARTESIAN_POINT('Ctrl Pts',(6.81718726299994,11.6,-8.16363498000002));
#169726=CARTESIAN_POINT('Ctrl Pts',(6.81620849499994,15.2,-8.16165187500001));
#169727=CARTESIAN_POINT('Ctrl Pts',(6.81620849499994,11.6,-8.16165187500001));
#169728=CARTESIAN_POINT('Ctrl Pts',(6.81523092699994,15.2,-8.15967560500001));
#169729=CARTESIAN_POINT('Ctrl Pts',(6.81523092699994,11.6,-8.15967560500001));
#169730=CARTESIAN_POINT('Ctrl Pts',(6.81425457199994,15.2,-8.15770618000002));
#169731=CARTESIAN_POINT('Ctrl Pts',(6.81425457199994,11.6,-8.15770618000002));
#169732=CARTESIAN_POINT('Ctrl Pts',(6.81327944699994,15.2,-8.15574360800002));
#169733=CARTESIAN_POINT('Ctrl Pts',(6.81327944699994,11.6,-8.15574360800002));
#169734=CARTESIAN_POINT('Ctrl Pts',(6.81230556799994,15.2,-8.15378789600001));
#169735=CARTESIAN_POINT('Ctrl Pts',(6.81230556799994,11.6,-8.15378789600001));
#169736=CARTESIAN_POINT('Ctrl Pts',(6.81133295099994,15.2,-8.15183905000002));
#169737=CARTESIAN_POINT('Ctrl Pts',(6.81133295099994,11.6,-8.15183905000002));
#169738=CARTESIAN_POINT('Ctrl Pts',(6.81036160899994,15.2,-8.14989708200001));
#169739=CARTESIAN_POINT('Ctrl Pts',(6.81036160899994,11.6,-8.14989708200001));
#169740=CARTESIAN_POINT('Ctrl Pts',(6.80939156199994,15.2,-8.14796199600002));
#169741=CARTESIAN_POINT('Ctrl Pts',(6.80939156199994,11.6,-8.14796199600002));
#169742=CARTESIAN_POINT('Ctrl Pts',(6.80842282199994,15.2,-8.14603380000002));
#169743=CARTESIAN_POINT('Ctrl Pts',(6.80842282199994,11.6,-8.14603380000002));
#169744=CARTESIAN_POINT('Ctrl Pts',(6.80745540699994,15.2,-8.14411250400001));
#169745=CARTESIAN_POINT('Ctrl Pts',(6.80745540699994,11.6,-8.14411250400001));
#169746=CARTESIAN_POINT('Ctrl Pts',(6.80648933299994,15.2,-8.14219811500001));
#169747=CARTESIAN_POINT('Ctrl Pts',(6.80648933299994,11.6,-8.14219811500001));
#169748=CARTESIAN_POINT('Ctrl Pts',(6.80552461599994,15.2,-8.14029063900002));
#169749=CARTESIAN_POINT('Ctrl Pts',(6.80552461599994,11.6,-8.14029063900002));
#169750=CARTESIAN_POINT('Ctrl Pts',(6.80456127099994,15.2,-8.13839008500001));
#169751=CARTESIAN_POINT('Ctrl Pts',(6.80456127099994,11.6,-8.13839008500001));
#169752=CARTESIAN_POINT('Ctrl Pts',(6.80359931599994,15.2,-8.13649646300002));
#169753=CARTESIAN_POINT('Ctrl Pts',(6.80359931599994,11.6,-8.13649646300002));
#169754=CARTESIAN_POINT('Ctrl Pts',(6.80263876599994,15.2,-8.13460977800002));
#169755=CARTESIAN_POINT('Ctrl Pts',(6.80263876599994,11.6,-8.13460977800002));
#169756=CARTESIAN_POINT('Ctrl Pts',(6.80167963599994,15.2,-8.13273003800001));
#169757=CARTESIAN_POINT('Ctrl Pts',(6.80167963599994,11.6,-8.13273003800001));
#169758=CARTESIAN_POINT('Ctrl Pts',(6.80072194599994,15.2,-8.13085725200001));
#169759=CARTESIAN_POINT('Ctrl Pts',(6.80072194599994,11.6,-8.13085725200001));
#169760=CARTESIAN_POINT('Ctrl Pts',(6.79976570799994,15.2,-8.12899142800001));
#169761=CARTESIAN_POINT('Ctrl Pts',(6.79976570799994,11.6,-8.12899142800001));
#169762=CARTESIAN_POINT('Ctrl Pts',(6.79881094199994,15.2,-8.12713257400001));
#169763=CARTESIAN_POINT('Ctrl Pts',(6.79881094199994,11.6,-8.12713257400001));
#169764=CARTESIAN_POINT('Ctrl Pts',(6.79785766299994,15.2,-8.12528069600001));
#169765=CARTESIAN_POINT('Ctrl Pts',(6.79785766299994,11.6,-8.12528069600001));
#169766=CARTESIAN_POINT('Ctrl Pts',(6.79690588799994,15.2,-8.12343580400002));
#169767=CARTESIAN_POINT('Ctrl Pts',(6.79690588799994,11.6,-8.12343580400002));
#169768=CARTESIAN_POINT('Ctrl Pts',(6.79595563299995,15.2,-8.12159790600001));
#169769=CARTESIAN_POINT('Ctrl Pts',(6.79595563299995,11.6,-8.12159790600001));
#169770=CARTESIAN_POINT('Ctrl Pts',(6.79500691399994,15.2,-8.11976700800002));
#169771=CARTESIAN_POINT('Ctrl Pts',(6.79500691399994,11.6,-8.11976700800002));
#169772=CARTESIAN_POINT('Ctrl Pts',(6.79405974999994,15.2,-8.11794312000002));
#169773=CARTESIAN_POINT('Ctrl Pts',(6.79405974999994,11.6,-8.11794312000002));
#169774=CARTESIAN_POINT('Ctrl Pts',(6.79311415699994,15.2,-8.11612625000001));
#169775=CARTESIAN_POINT('Ctrl Pts',(6.79311415699994,11.6,-8.11612625000001));
#169776=CARTESIAN_POINT('Ctrl Pts',(6.79217014999994,15.2,-8.11431640400002));
#169777=CARTESIAN_POINT('Ctrl Pts',(6.79217014999994,11.6,-8.11431640400002));
#169778=CARTESIAN_POINT('Ctrl Pts',(6.79122774799994,15.2,-8.11251359100002));
#169779=CARTESIAN_POINT('Ctrl Pts',(6.79122774799994,11.6,-8.11251359100002));
#169780=CARTESIAN_POINT('Ctrl Pts',(6.79028696699994,15.2,-8.11071782000001));
#169781=CARTESIAN_POINT('Ctrl Pts',(6.79028696699994,11.6,-8.11071782000001));
#169782=CARTESIAN_POINT('Ctrl Pts',(6.78934782399994,15.2,-8.10892909900002));
#169783=CARTESIAN_POINT('Ctrl Pts',(6.78934782399994,11.6,-8.10892909900002));
#169784=CARTESIAN_POINT('Ctrl Pts',(6.78841033799994,15.2,-8.10714743400002));
#169785=CARTESIAN_POINT('Ctrl Pts',(6.78841033799994,11.6,-8.10714743400002));
#169786=CARTESIAN_POINT('Ctrl Pts',(6.78747452299994,15.2,-8.10537283700001));
#169787=CARTESIAN_POINT('Ctrl Pts',(6.78747452299994,11.6,-8.10537283700001));
#169788=CARTESIAN_POINT('Ctrl Pts',(6.78654039799994,15.2,-8.10360531100002));
#169789=CARTESIAN_POINT('Ctrl Pts',(6.78654039799994,11.6,-8.10360531100002));
#169790=CARTESIAN_POINT('Ctrl Pts',(6.78560798099994,15.2,-8.10184486900001));
#169791=CARTESIAN_POINT('Ctrl Pts',(6.78560798099994,11.6,-8.10184486900001));
#169792=CARTESIAN_POINT('Ctrl Pts',(6.78467728799995,15.2,-8.10009151600001));
#169793=CARTESIAN_POINT('Ctrl Pts',(6.78467728799995,11.6,-8.10009151600001));
#169794=CARTESIAN_POINT('Ctrl Pts',(6.78374833699994,15.2,-8.09834526200002));
#169795=CARTESIAN_POINT('Ctrl Pts',(6.78374833699994,11.6,-8.09834526200002));
#169796=CARTESIAN_POINT('Ctrl Pts',(6.78282114499994,15.2,-8.09660611400002));
#169797=CARTESIAN_POINT('Ctrl Pts',(6.78282114499994,11.6,-8.09660611400002));
#169798=CARTESIAN_POINT('Ctrl Pts',(6.78189572999995,15.2,-8.09487408000002));
#169799=CARTESIAN_POINT('Ctrl Pts',(6.78189572999995,11.6,-8.09487408000002));
#169800=CARTESIAN_POINT('Ctrl Pts',(6.78097211099994,15.2,-8.09314916800002));
#169801=CARTESIAN_POINT('Ctrl Pts',(6.78097211099994,11.6,-8.09314916800002));
#169802=CARTESIAN_POINT('Ctrl Pts',(6.78005030299994,15.2,-8.09143138900002));
#169803=CARTESIAN_POINT('Ctrl Pts',(6.78005030299994,11.6,-8.09143138900002));
#169804=CARTESIAN_POINT('Ctrl Pts',(6.77913032499994,15.2,-8.08972074800002));
#169805=CARTESIAN_POINT('Ctrl Pts',(6.77913032499994,11.6,-8.08972074800002));
#169806=CARTESIAN_POINT('Ctrl Pts',(6.77821219499994,15.2,-8.08801725500001));
#169807=CARTESIAN_POINT('Ctrl Pts',(6.77821219499994,11.6,-8.08801725500001));
#169808=CARTESIAN_POINT('Ctrl Pts',(6.77729593099994,15.2,-8.08632091800002));
#169809=CARTESIAN_POINT('Ctrl Pts',(6.77729593099994,11.6,-8.08632091800002));
#169810=CARTESIAN_POINT('Ctrl Pts',(6.77638154999994,15.2,-8.08463174500002));
#169811=CARTESIAN_POINT('Ctrl Pts',(6.77638154999994,11.6,-8.08463174500002));
#169812=CARTESIAN_POINT('Ctrl Pts',(6.77546907099994,15.2,-8.08294974400001));
#169813=CARTESIAN_POINT('Ctrl Pts',(6.77546907099994,11.6,-8.08294974400001));
#169814=CARTESIAN_POINT('Ctrl Pts',(6.77455851199994,15.2,-8.08127492400001));
#169815=CARTESIAN_POINT('Ctrl Pts',(6.77455851199994,11.6,-8.08127492400001));
#169816=CARTESIAN_POINT('Ctrl Pts',(6.77364988999994,15.2,-8.07960729300002));
#169817=CARTESIAN_POINT('Ctrl Pts',(6.77364988999994,11.6,-8.07960729300002));
#169818=CARTESIAN_POINT('Ctrl Pts',(6.77274322499994,15.2,-8.07794686000002));
#169819=CARTESIAN_POINT('Ctrl Pts',(6.77274322499994,11.6,-8.07794686000002));
#169820=CARTESIAN_POINT('Ctrl Pts',(6.77183853299994,15.2,-8.07629363200002));
#169821=CARTESIAN_POINT('Ctrl Pts',(6.77183853299994,11.6,-8.07629363200002));
#169822=CARTESIAN_POINT('Ctrl Pts',(6.77093583499994,15.2,-8.07464761900002));
#169823=CARTESIAN_POINT('Ctrl Pts',(6.77093583499994,11.6,-8.07464761900002));
#169824=CARTESIAN_POINT('Ctrl Pts',(6.77003514699994,15.2,-8.07300882800002));
#169825=CARTESIAN_POINT('Ctrl Pts',(6.77003514699994,11.6,-8.07300882800002));
#169826=CARTESIAN_POINT('Ctrl Pts',(6.76913648999995,15.2,-8.07137726900002));
#169827=CARTESIAN_POINT('Ctrl Pts',(6.76913648999995,11.6,-8.07137726900002));
#169828=CARTESIAN_POINT('Ctrl Pts',(6.76823988099994,15.2,-8.06975294900001));
#169829=CARTESIAN_POINT('Ctrl Pts',(6.76823988099994,11.6,-8.06975294900001));
#169830=CARTESIAN_POINT('Ctrl Pts',(6.76734533799995,15.2,-8.06813587700002));
#169831=CARTESIAN_POINT('Ctrl Pts',(6.76734533799995,11.6,-8.06813587700002));
#169832=CARTESIAN_POINT('Ctrl Pts',(6.76645288099994,15.2,-8.06652606100002));
#169833=CARTESIAN_POINT('Ctrl Pts',(6.76645288099994,11.6,-8.06652606100002));
#169834=CARTESIAN_POINT('Ctrl Pts',(6.76556252799994,15.2,-8.06492351100001));
#169835=CARTESIAN_POINT('Ctrl Pts',(6.76556252799994,11.6,-8.06492351100001));
#169836=CARTESIAN_POINT('Ctrl Pts',(6.76467429899994,15.2,-8.06332823600002));
#169837=CARTESIAN_POINT('Ctrl Pts',(6.76467429899994,11.6,-8.06332823600002));
#169838=CARTESIAN_POINT('Ctrl Pts',(6.76378821099994,15.2,-8.06174024100001));
#169839=CARTESIAN_POINT('Ctrl Pts',(6.76378821099994,11.6,-8.06174024100001));
#169840=CARTESIAN_POINT('Ctrl Pts',(6.76290428599994,15.2,-8.06015953800001));
#169841=CARTESIAN_POINT('Ctrl Pts',(6.76290428599994,11.6,-8.06015953800001));
#169842=CARTESIAN_POINT('Ctrl Pts',(6.76202253899994,15.2,-8.05858613400002));
#169843=CARTESIAN_POINT('Ctrl Pts',(6.76202253899994,11.6,-8.05858613400002));
#169844=CARTESIAN_POINT('Ctrl Pts',(6.76114299199994,15.2,-8.05702003800001));
#169845=CARTESIAN_POINT('Ctrl Pts',(6.76114299199994,11.6,-8.05702003800001));
#169846=CARTESIAN_POINT('Ctrl Pts',(6.76026566399995,15.2,-8.05546125900002));
#169847=CARTESIAN_POINT('Ctrl Pts',(6.76026566399995,11.6,-8.05546125900002));
#169848=CARTESIAN_POINT('Ctrl Pts',(6.75939057299995,15.2,-8.05390980500002));
#169849=CARTESIAN_POINT('Ctrl Pts',(6.75939057299995,11.6,-8.05390980500002));
#169850=CARTESIAN_POINT('Ctrl Pts',(6.75851773999994,15.2,-8.05236568400002));
#169851=CARTESIAN_POINT('Ctrl Pts',(6.75851773999994,11.6,-8.05236568400002));
#169852=CARTESIAN_POINT('Ctrl Pts',(6.75764718299994,15.2,-8.05082890700002));
#169853=CARTESIAN_POINT('Ctrl Pts',(6.75764718299994,11.6,-8.05082890700002));
#169854=CARTESIAN_POINT('Ctrl Pts',(6.75677892299994,15.2,-8.04929948100002));
#169855=CARTESIAN_POINT('Ctrl Pts',(6.75677892299994,11.6,-8.04929948100002));
#169856=CARTESIAN_POINT('Ctrl Pts',(6.75591297799994,15.2,-8.04777741600001));
#169857=CARTESIAN_POINT('Ctrl Pts',(6.75591297799994,11.6,-8.04777741600001));
#169858=CARTESIAN_POINT('Ctrl Pts',(6.75504936899994,15.2,-8.04626271800002));
#169859=CARTESIAN_POINT('Ctrl Pts',(6.75504936899994,11.6,-8.04626271800002));
#169860=CARTESIAN_POINT('Ctrl Pts',(6.75418811399994,15.2,-8.04475539900002));
#169861=CARTESIAN_POINT('Ctrl Pts',(6.75418811399994,11.6,-8.04475539900002));
#169862=CARTESIAN_POINT('Ctrl Pts',(6.75332923499994,15.2,-8.04325546600002));
#169863=CARTESIAN_POINT('Ctrl Pts',(6.75332923499994,11.6,-8.04325546600002));
#169864=CARTESIAN_POINT('Ctrl Pts',(6.75247275099994,15.2,-8.04176292900001));
#169865=CARTESIAN_POINT('Ctrl Pts',(6.75247275099994,11.6,-8.04176292900001));
#169866=CARTESIAN_POINT('Ctrl Pts',(6.75161868199995,15.2,-8.04027779500002));
#169867=CARTESIAN_POINT('Ctrl Pts',(6.75161868199995,11.6,-8.04027779500002));
#169868=CARTESIAN_POINT('Ctrl Pts',(6.75076704799995,15.2,-8.03880007500002));
#169869=CARTESIAN_POINT('Ctrl Pts',(6.75076704799995,11.6,-8.03880007500002));
#169870=CARTESIAN_POINT('Ctrl Pts',(6.74991786899994,15.2,-8.03732977600001));
#169871=CARTESIAN_POINT('Ctrl Pts',(6.74991786899994,11.6,-8.03732977600001));
#169872=CARTESIAN_POINT('Ctrl Pts',(6.74907116499995,15.2,-8.03586690800002));
#169873=CARTESIAN_POINT('Ctrl Pts',(6.74907116499995,11.6,-8.03586690800002));
#169874=CARTESIAN_POINT('Ctrl Pts',(6.74822695699994,15.2,-8.03441148000001));
#169875=CARTESIAN_POINT('Ctrl Pts',(6.74822695699994,11.6,-8.03441148000001));
#169876=CARTESIAN_POINT('Ctrl Pts',(6.74738526499994,15.2,-8.03296350100002));
#169877=CARTESIAN_POINT('Ctrl Pts',(6.74738526499994,11.6,-8.03296350100002));
#169878=CARTESIAN_POINT('Ctrl Pts',(6.74654610999994,15.2,-8.03152298000001));
#169879=CARTESIAN_POINT('Ctrl Pts',(6.74654610999994,11.6,-8.03152298000001));
#169880=CARTESIAN_POINT('Ctrl Pts',(6.74570951199994,15.2,-8.03008992500001));
#169881=CARTESIAN_POINT('Ctrl Pts',(6.74570951199994,11.6,-8.03008992500001));
#169882=CARTESIAN_POINT('Ctrl Pts',(6.74487549099994,15.2,-8.02866434600002));
#169883=CARTESIAN_POINT('Ctrl Pts',(6.74487549099994,11.6,-8.02866434600002));
#169884=CARTESIAN_POINT('Ctrl Pts',(6.74404406899995,15.2,-8.02724625000002));
#169885=CARTESIAN_POINT('Ctrl Pts',(6.74404406899995,11.6,-8.02724625000002));
#169886=CARTESIAN_POINT('Ctrl Pts',(6.74321526699995,15.2,-8.02583564900001));
#169887=CARTESIAN_POINT('Ctrl Pts',(6.74321526699995,11.6,-8.02583564900001));
#169888=CARTESIAN_POINT('Ctrl Pts',(6.74238910499994,15.2,-8.02443255100002));
#169889=CARTESIAN_POINT('Ctrl Pts',(6.74238910499994,11.6,-8.02443255100002));
#169890=CARTESIAN_POINT('Ctrl Pts',(6.74156560399994,15.2,-8.02303696500001));
#169891=CARTESIAN_POINT('Ctrl Pts',(6.74156560399994,11.6,-8.02303696500001));
#169892=CARTESIAN_POINT('Ctrl Pts',(6.74074478399994,15.2,-8.02164890000002));
#169893=CARTESIAN_POINT('Ctrl Pts',(6.74074478399994,11.6,-8.02164890000002));
#169894=CARTESIAN_POINT('Ctrl Pts',(6.73992666899994,15.2,-8.02026836500002));
#169895=CARTESIAN_POINT('Ctrl Pts',(6.73992666899994,11.6,-8.02026836500002));
#169896=CARTESIAN_POINT('Ctrl Pts',(6.73911127899994,15.2,-8.01889537000001));
#169897=CARTESIAN_POINT('Ctrl Pts',(6.73911127899994,11.6,-8.01889537000001));
#169898=CARTESIAN_POINT('Ctrl Pts',(6.73829863399994,15.2,-8.01752992300001));
#169899=CARTESIAN_POINT('Ctrl Pts',(6.73829863399994,11.6,-8.01752992300001));
#169900=CARTESIAN_POINT('Ctrl Pts',(6.73748875699994,15.2,-8.01617203400001));
#169901=CARTESIAN_POINT('Ctrl Pts',(6.73748875699994,11.6,-8.01617203400001));
#169902=CARTESIAN_POINT('Ctrl Pts',(6.73668166999994,15.2,-8.01482171200002));
#169903=CARTESIAN_POINT('Ctrl Pts',(6.73668166999994,11.6,-8.01482171200002));
#169904=CARTESIAN_POINT('Ctrl Pts',(6.73587739199994,15.2,-8.01347896600002));
#169905=CARTESIAN_POINT('Ctrl Pts',(6.73587739199994,11.6,-8.01347896600002));
#169906=CARTESIAN_POINT('Ctrl Pts',(6.73507594699994,15.2,-8.01214380700002));
#169907=CARTESIAN_POINT('Ctrl Pts',(6.73507594699994,11.6,-8.01214380700002));
#169908=CARTESIAN_POINT('Ctrl Pts',(6.73427735599994,15.2,-8.01081624200001));
#169909=CARTESIAN_POINT('Ctrl Pts',(6.73427735599994,11.6,-8.01081624200001));
#169910=CARTESIAN_POINT('Ctrl Pts',(6.73348164099994,15.2,-8.00949628200001));
#169911=CARTESIAN_POINT('Ctrl Pts',(6.73348164099994,11.6,-8.00949628200001));
#169912=CARTESIAN_POINT('Ctrl Pts',(6.73268882399994,15.2,-8.00818393500002));
#169913=CARTESIAN_POINT('Ctrl Pts',(6.73268882399994,11.6,-8.00818393500002));
#169914=CARTESIAN_POINT('Ctrl Pts',(6.73189892699994,15.2,-8.00687921200002));
#169915=CARTESIAN_POINT('Ctrl Pts',(6.73189892699994,11.6,-8.00687921200002));
#169916=CARTESIAN_POINT('Ctrl Pts',(6.73111197299994,15.2,-8.00558212100002));
#169917=CARTESIAN_POINT('Ctrl Pts',(6.73111197299994,11.6,-8.00558212100002));
#169918=CARTESIAN_POINT('Ctrl Pts',(6.73032798299994,15.2,-8.00429267200002));
#169919=CARTESIAN_POINT('Ctrl Pts',(6.73032798299994,11.6,-8.00429267200002));
#169920=CARTESIAN_POINT('Ctrl Pts',(6.72954697899995,15.2,-8.00301087500002));
#169921=CARTESIAN_POINT('Ctrl Pts',(6.72954697899995,11.6,-8.00301087500002));
#169922=CARTESIAN_POINT('Ctrl Pts',(6.72876898499994,15.2,-8.00173673800002));
#169923=CARTESIAN_POINT('Ctrl Pts',(6.72876898499994,11.6,-8.00173673800002));
#169924=CARTESIAN_POINT('Ctrl Pts',(6.72799402199994,15.2,-8.00047027200002));
#169925=CARTESIAN_POINT('Ctrl Pts',(6.72799402199994,11.6,-8.00047027200002));
#169926=CARTESIAN_POINT('Ctrl Pts',(6.72722211399994,15.2,-7.99921148700002));
#169927=CARTESIAN_POINT('Ctrl Pts',(6.72722211399994,11.6,-7.99921148700002));
#169928=CARTESIAN_POINT('Ctrl Pts',(6.72645328299994,15.2,-7.99796039100002));
#169929=CARTESIAN_POINT('Ctrl Pts',(6.72645328299994,11.6,-7.99796039100002));
#169930=CARTESIAN_POINT('Ctrl Pts',(6.72568755199995,15.2,-7.99671699400001));
#169931=CARTESIAN_POINT('Ctrl Pts',(6.72568755199995,11.6,-7.99671699400001));
#169932=CARTESIAN_POINT('Ctrl Pts',(6.72492494399994,15.2,-7.99548130700002));
#169933=CARTESIAN_POINT('Ctrl Pts',(6.72492494399994,11.6,-7.99548130700002));
#169934=CARTESIAN_POINT('Ctrl Pts',(6.72416548199994,15.2,-7.99425333800002));
#169935=CARTESIAN_POINT('Ctrl Pts',(6.72416548199994,11.6,-7.99425333800002));
#169936=CARTESIAN_POINT('Ctrl Pts',(6.72340918899994,15.2,-7.99303309800001));
#169937=CARTESIAN_POINT('Ctrl Pts',(6.72340918899994,11.6,-7.99303309800001));
#169938=CARTESIAN_POINT('Ctrl Pts',(6.72265608899994,15.2,-7.99182059500002));
#169939=CARTESIAN_POINT('Ctrl Pts',(6.72265608899994,11.6,-7.99182059500002));
#169940=CARTESIAN_POINT('Ctrl Pts',(6.72190620499994,15.2,-7.99061584100001));
#169941=CARTESIAN_POINT('Ctrl Pts',(6.72190620499994,11.6,-7.99061584100001));
#169942=CARTESIAN_POINT('Ctrl Pts',(6.72115955899995,15.2,-7.98941884400002));
#169943=CARTESIAN_POINT('Ctrl Pts',(6.72115955899995,11.6,-7.98941884400002));
#169944=CARTESIAN_POINT('Ctrl Pts',(6.72041617599994,15.2,-7.98822961300001));
#169945=CARTESIAN_POINT('Ctrl Pts',(6.72041617599994,11.6,-7.98822961300001));
#169946=CARTESIAN_POINT('Ctrl Pts',(6.71967607999994,15.2,-7.98704816100001));
#169947=CARTESIAN_POINT('Ctrl Pts',(6.71967607999994,11.6,-7.98704816100001));
#169948=CARTESIAN_POINT('Ctrl Pts',(6.71893929399995,15.2,-7.98587449600002));
#169949=CARTESIAN_POINT('Ctrl Pts',(6.71893929399995,11.6,-7.98587449600002));
#169950=CARTESIAN_POINT('Ctrl Pts',(6.71820584199994,15.2,-7.98470862800002));
#169951=CARTESIAN_POINT('Ctrl Pts',(6.71820584199994,11.6,-7.98470862800002));
#169952=CARTESIAN_POINT('Ctrl Pts',(6.71747574699994,15.2,-7.98355056600002));
#169953=CARTESIAN_POINT('Ctrl Pts',(6.71747574699994,11.6,-7.98355056600002));
#169954=CARTESIAN_POINT('Ctrl Pts',(6.71674903499994,15.2,-7.98240032100002));
#169955=CARTESIAN_POINT('Ctrl Pts',(6.71674903499994,11.6,-7.98240032100002));
#169956=CARTESIAN_POINT('Ctrl Pts',(6.71602572899994,15.2,-7.98125790400002));
#169957=CARTESIAN_POINT('Ctrl Pts',(6.71602572899994,11.6,-7.98125790400002));
#169958=CARTESIAN_POINT('Ctrl Pts',(6.71530585299994,15.2,-7.98012332400001));
#169959=CARTESIAN_POINT('Ctrl Pts',(6.71530585299994,11.6,-7.98012332400001));
#169960=CARTESIAN_POINT('Ctrl Pts',(6.71458943199994,15.2,-7.97899659000001));
#169961=CARTESIAN_POINT('Ctrl Pts',(6.71458943199994,11.6,-7.97899659000001));
#169962=CARTESIAN_POINT('Ctrl Pts',(6.71387649099994,15.2,-7.97787771300002));
#169963=CARTESIAN_POINT('Ctrl Pts',(6.71387649099994,11.6,-7.97787771300002));
#169964=CARTESIAN_POINT('Ctrl Pts',(6.71316705499994,15.2,-7.97676670400002));
#169965=CARTESIAN_POINT('Ctrl Pts',(6.71316705499994,11.6,-7.97676670400002));
#169966=CARTESIAN_POINT('Ctrl Pts',(6.71246114699994,15.2,-7.97566357200001));
#169967=CARTESIAN_POINT('Ctrl Pts',(6.71246114699994,11.6,-7.97566357200001));
#169968=CARTESIAN_POINT('Ctrl Pts',(6.71175879199994,15.2,-7.97456832700002));
#169969=CARTESIAN_POINT('Ctrl Pts',(6.71175879199994,11.6,-7.97456832700002));
#169970=CARTESIAN_POINT('Ctrl Pts',(6.71106001699994,15.2,-7.97348098000001));
#169971=CARTESIAN_POINT('Ctrl Pts',(6.71106001699994,11.6,-7.97348098000001));
#169972=CARTESIAN_POINT('Ctrl Pts',(6.71036484499994,15.2,-7.97240154000002));
#169973=CARTESIAN_POINT('Ctrl Pts',(6.71036484499994,11.6,-7.97240154000002));
#169974=CARTESIAN_POINT('Ctrl Pts',(6.70967330099994,15.2,-7.97133002000002));
#169975=CARTESIAN_POINT('Ctrl Pts',(6.70967330099994,11.6,-7.97133002000002));
#169976=CARTESIAN_POINT('Ctrl Pts',(6.70898541199994,15.2,-7.97026642700001));
#169977=CARTESIAN_POINT('Ctrl Pts',(6.70898541199994,11.6,-7.97026642700001));
#169978=CARTESIAN_POINT('Ctrl Pts',(6.70830120299994,15.2,-7.96921077400001));
#169979=CARTESIAN_POINT('Ctrl Pts',(6.70830120299994,11.6,-7.96921077400001));
#169980=CARTESIAN_POINT('Ctrl Pts',(6.70762069999994,15.2,-7.96816306900002));
#169981=CARTESIAN_POINT('Ctrl Pts',(6.70762069999994,11.6,-7.96816306900002));
#169982=CARTESIAN_POINT('Ctrl Pts',(6.70694392699994,15.2,-7.96712332400002));
#169983=CARTESIAN_POINT('Ctrl Pts',(6.70694392699994,11.6,-7.96712332400002));
#169984=CARTESIAN_POINT('Ctrl Pts',(6.70627090999995,15.2,-7.96609155000001));
#169985=CARTESIAN_POINT('Ctrl Pts',(6.70627090999995,11.6,-7.96609155000001));
#169986=CARTESIAN_POINT('Ctrl Pts',(6.70560167699994,15.2,-7.96506775500001));
#169987=CARTESIAN_POINT('Ctrl Pts',(6.70560167699994,11.6,-7.96506775500001));
#169988=CARTESIAN_POINT('Ctrl Pts',(6.70493625199994,15.2,-7.96405195200002));
#169989=CARTESIAN_POINT('Ctrl Pts',(6.70493625199994,11.6,-7.96405195200002));
#169990=CARTESIAN_POINT('Ctrl Pts',(6.70427466299994,15.2,-7.96304415000002));
#169991=CARTESIAN_POINT('Ctrl Pts',(6.70427466299994,11.6,-7.96304415000002));
#169992=CARTESIAN_POINT('Ctrl Pts',(6.70361693399994,15.2,-7.96204436100002));
#169993=CARTESIAN_POINT('Ctrl Pts',(6.70361693399994,11.6,-7.96204436100002));
#169994=CARTESIAN_POINT('Ctrl Pts',(6.70296309299995,15.2,-7.96105259300001));
#169995=CARTESIAN_POINT('Ctrl Pts',(6.70296309299995,11.6,-7.96105259300001));
#169996=CARTESIAN_POINT('Ctrl Pts',(6.70231316599994,15.2,-7.96006886000002));
#169997=CARTESIAN_POINT('Ctrl Pts',(6.70231316599994,11.6,-7.96006886000002));
#169998=CARTESIAN_POINT('Ctrl Pts',(6.70166717899995,15.2,-7.95909317200002));
#169999=CARTESIAN_POINT('Ctrl Pts',(6.70166717899995,11.6,-7.95909317200002));
#170000=CARTESIAN_POINT('Ctrl Pts',(6.70102515999995,15.2,-7.95812553600002));
#170001=CARTESIAN_POINT('Ctrl Pts',(6.70102515999995,11.6,-7.95812553600002));
#170002=CARTESIAN_POINT('Ctrl Pts',(6.70038713599994,15.2,-7.95716596700001));
#170003=CARTESIAN_POINT('Ctrl Pts',(6.70038713599994,11.6,-7.95716596700001));
#170004=CARTESIAN_POINT('Ctrl Pts',(6.69975313299994,15.2,-7.95621447500002));
#170005=CARTESIAN_POINT('Ctrl Pts',(6.69975313299994,11.6,-7.95621447500002));
#170006=CARTESIAN_POINT('Ctrl Pts',(6.69912317899994,15.2,-7.95527107000002));
#170007=CARTESIAN_POINT('Ctrl Pts',(6.69912317899994,11.6,-7.95527107000002));
#170008=CARTESIAN_POINT('Ctrl Pts',(6.69849730099994,15.2,-7.95433576200002));
#170009=CARTESIAN_POINT('Ctrl Pts',(6.69849730099994,11.6,-7.95433576200002));
#170010=CARTESIAN_POINT('Ctrl Pts',(6.69787552599994,15.2,-7.95340856300002));
#170011=CARTESIAN_POINT('Ctrl Pts',(6.69787552599994,11.6,-7.95340856300002));
#170012=CARTESIAN_POINT('Ctrl Pts',(6.69725788299994,15.2,-7.95248948500002));
#170013=CARTESIAN_POINT('Ctrl Pts',(6.69725788299994,11.6,-7.95248948500002));
#170014=CARTESIAN_POINT('Ctrl Pts',(6.69664439799995,15.2,-7.95157853800001));
#170015=CARTESIAN_POINT('Ctrl Pts',(6.69664439799995,11.6,-7.95157853800001));
#170016=CARTESIAN_POINT('Ctrl Pts',(6.69603509999994,15.2,-7.95067573100001));
#170017=CARTESIAN_POINT('Ctrl Pts',(6.69603509999994,11.6,-7.95067573100001));
#170018=CARTESIAN_POINT('Ctrl Pts',(6.69543001599994,15.2,-7.94978107900001));
#170019=CARTESIAN_POINT('Ctrl Pts',(6.69543001599994,11.6,-7.94978107900001));
#170020=CARTESIAN_POINT('Ctrl Pts',(6.69482917499994,15.2,-7.94889459000002));
#170021=CARTESIAN_POINT('Ctrl Pts',(6.69482917499994,11.6,-7.94889459000002));
#170022=CARTESIAN_POINT('Ctrl Pts',(6.69423260499994,15.2,-7.94801627700001));
#170023=CARTESIAN_POINT('Ctrl Pts',(6.69423260499994,11.6,-7.94801627700001));
#170024=CARTESIAN_POINT('Ctrl Pts',(6.69364033499994,15.2,-7.94714614900002));
#170025=CARTESIAN_POINT('Ctrl Pts',(6.69364033499994,11.6,-7.94714614900002));
#170026=CARTESIAN_POINT('Ctrl Pts',(6.69305239199994,15.2,-7.94628422000001));
#170027=CARTESIAN_POINT('Ctrl Pts',(6.69305239199994,11.6,-7.94628422000001));
#170028=CARTESIAN_POINT('Ctrl Pts',(6.69246880599994,15.2,-7.94543049900001));
#170029=CARTESIAN_POINT('Ctrl Pts',(6.69246880599994,11.6,-7.94543049900001));
#170030=CARTESIAN_POINT('Ctrl Pts',(6.69188960599994,15.2,-7.94458500000002));
#170031=CARTESIAN_POINT('Ctrl Pts',(6.69188960599994,11.6,-7.94458500000002));
#170032=CARTESIAN_POINT('Ctrl Pts',(6.69131482099995,15.2,-7.94374773000002));
#170033=CARTESIAN_POINT('Ctrl Pts',(6.69131482099995,11.6,-7.94374773000002));
#170034=CARTESIAN_POINT('Ctrl Pts',(6.69074447799994,15.2,-7.94291870500002));
#170035=CARTESIAN_POINT('Ctrl Pts',(6.69074447799994,11.6,-7.94291870500002));
#170036=CARTESIAN_POINT('Ctrl Pts',(6.69017860899995,15.2,-7.94209793300002));
#170037=CARTESIAN_POINT('Ctrl Pts',(6.69017860899995,11.6,-7.94209793300002));
#170038=CARTESIAN_POINT('Ctrl Pts',(6.68961724099994,15.2,-7.94128542600002));
#170039=CARTESIAN_POINT('Ctrl Pts',(6.68961724099994,11.6,-7.94128542600002));
#170040=CARTESIAN_POINT('Ctrl Pts',(6.68906040599994,15.2,-7.94048119900002));
#170041=CARTESIAN_POINT('Ctrl Pts',(6.68906040599994,11.6,-7.94048119900002));
#170042=CARTESIAN_POINT('Ctrl Pts',(6.68850813299994,15.2,-7.93968525900001));
#170043=CARTESIAN_POINT('Ctrl Pts',(6.68850813299994,11.6,-7.93968525900001));
#170044=CARTESIAN_POINT('Ctrl Pts',(6.68796045099994,15.2,-7.93889762000001));
#170045=CARTESIAN_POINT('Ctrl Pts',(6.68796045099994,11.6,-7.93889762000001));
#170046=CARTESIAN_POINT('Ctrl Pts',(6.68741739099994,15.2,-7.93811829200001));
#170047=CARTESIAN_POINT('Ctrl Pts',(6.68741739099994,11.6,-7.93811829200001));
#170048=CARTESIAN_POINT('Ctrl Pts',(6.68687898199994,15.2,-7.93734729000001));
#170049=CARTESIAN_POINT('Ctrl Pts',(6.68687898199994,11.6,-7.93734729000001));
#170050=CARTESIAN_POINT('Ctrl Pts',(6.68634525499994,15.2,-7.93658462300002));
#170051=CARTESIAN_POINT('Ctrl Pts',(6.68634525499994,11.6,-7.93658462300002));
#170052=CARTESIAN_POINT('Ctrl Pts',(6.68581928699994,15.2,-7.93583464600002));
#170053=CARTESIAN_POINT('Ctrl Pts',(6.68581928699994,11.6,-7.93583464600002));
#170054=CARTESIAN_POINT('Ctrl Pts',(6.68540286299995,15.2,-7.93524212600002));
#170055=CARTESIAN_POINT('Ctrl Pts',(6.68540286299995,11.6,-7.93524212600002));
#170056=CARTESIAN_POINT('Ctrl Pts',(6.68509340699995,15.2,-7.93480250500001));
#170057=CARTESIAN_POINT('Ctrl Pts',(6.68509340699995,11.6,-7.93480250500001));
#170058=CARTESIAN_POINT('Ctrl Pts',(6.68488903399994,15.2,-7.93451247300001));
#170059=CARTESIAN_POINT('Ctrl Pts',(6.68488903399994,11.6,-7.93451247300001));
#170060=CARTESIAN_POINT('Ctrl Pts',(6.68478856699994,15.2,-7.93436996900001));
#170061=CARTESIAN_POINT('Ctrl Pts',(6.68478856699994,11.6,-7.93436996900001));
#170062=CARTESIAN_POINT('',(6.68478856699994,12.2,-7.93436996900001));
#170063=CARTESIAN_POINT('',(6.68478856699994,15.2,-7.93436996900001));
#170064=CARTESIAN_POINT('',(6.68478856699994,12.2,-7.93436996900001));
#170065=CARTESIAN_POINT('Ctrl Pts',(7.10901226899994,12.2,-9.03946594400002));
#170066=CARTESIAN_POINT('Ctrl Pts',(7.10885083699995,12.2,-9.03871859500001));
#170067=CARTESIAN_POINT('Ctrl Pts',(7.10852778299994,12.2,-9.03722439200001));
#170068=CARTESIAN_POINT('Ctrl Pts',(7.10804263899995,12.2,-9.03498456100002));
#170069=CARTESIAN_POINT('Ctrl Pts',(7.10739465099994,12.2,-9.03200107200002));
#170070=CARTESIAN_POINT('Ctrl Pts',(7.10658278299994,12.2,-9.02827662900001));
#170071=CARTESIAN_POINT('Ctrl Pts',(7.10576903499994,12.2,-9.02455710700002));
#170072=CARTESIAN_POINT('Ctrl Pts',(7.10495340799994,12.2,-9.02084250500002));
#170073=CARTESIAN_POINT('Ctrl Pts',(7.10413590299994,12.2,-9.01713282900002));
#170074=CARTESIAN_POINT('Ctrl Pts',(7.10331652799994,12.2,-9.01342808000001));
#170075=CARTESIAN_POINT('Ctrl Pts',(7.10249528699994,12.2,-9.00972826500002));
#170076=CARTESIAN_POINT('Ctrl Pts',(7.10167218799994,12.2,-9.00603338900002));
#170077=CARTESIAN_POINT('Ctrl Pts',(7.10084723999994,12.2,-9.00234345900002));
#170078=CARTESIAN_POINT('Ctrl Pts',(7.10002044999994,12.2,-8.99865848200001));
#170079=CARTESIAN_POINT('Ctrl Pts',(7.09919182999994,12.2,-8.99497846600001));
#170080=CARTESIAN_POINT('Ctrl Pts',(7.09836138399995,12.2,-8.99130341500002));
#170081=CARTESIAN_POINT('Ctrl Pts',(7.09752912199995,12.2,-8.98763333900002));
#170082=CARTESIAN_POINT('Ctrl Pts',(7.09669504999995,12.2,-8.98396824000002));
#170083=CARTESIAN_POINT('Ctrl Pts',(7.09585917499994,12.2,-8.98030812400001));
#170084=CARTESIAN_POINT('Ctrl Pts',(7.09502150299994,12.2,-8.97665299700002));
#170085=CARTESIAN_POINT('Ctrl Pts',(7.09418203899994,12.2,-8.97300286300002));
#170086=CARTESIAN_POINT('Ctrl Pts',(7.09334079199994,12.2,-8.96935772800001));
#170087=CARTESIAN_POINT('Ctrl Pts',(7.09249776599994,12.2,-8.96571759800001));
#170088=CARTESIAN_POINT('Ctrl Pts',(7.09165297099994,12.2,-8.96208247700002));
#170089=CARTESIAN_POINT('Ctrl Pts',(7.09080641499994,12.2,-8.95845237400002));
#170090=CARTESIAN_POINT('Ctrl Pts',(7.08995810299994,12.2,-8.95482729200002));
#170091=CARTESIAN_POINT('Ctrl Pts',(7.08910804199994,12.2,-8.95120723800002));
#170092=CARTESIAN_POINT('Ctrl Pts',(7.08825624299994,12.2,-8.94759221800001));
#170093=CARTESIAN_POINT('Ctrl Pts',(7.08740270999995,12.2,-8.94398223900001));
#170094=CARTESIAN_POINT('Ctrl Pts',(7.08654745099994,12.2,-8.94037730400001));
#170095=CARTESIAN_POINT('Ctrl Pts',(7.08569047499994,12.2,-8.93677742100002));
#170096=CARTESIAN_POINT('Ctrl Pts',(7.08483178599994,12.2,-8.93318259300001));
#170097=CARTESIAN_POINT('Ctrl Pts',(7.08397139199994,12.2,-8.92959282900001));
#170098=CARTESIAN_POINT('Ctrl Pts',(7.08310930199994,12.2,-8.92600813100002));
#170099=CARTESIAN_POINT('Ctrl Pts',(7.08224552099994,12.2,-8.92242850800002));
#170100=CARTESIAN_POINT('Ctrl Pts',(7.08138005899994,12.2,-8.91885396400001));
#170101=CARTESIAN_POINT('Ctrl Pts',(7.08051291999994,12.2,-8.91528450500001));
#170102=CARTESIAN_POINT('Ctrl Pts',(7.07964411499994,12.2,-8.91172013700002));
#170103=CARTESIAN_POINT('Ctrl Pts',(7.07877364899994,12.2,-8.90816086600001));
#170104=CARTESIAN_POINT('Ctrl Pts',(7.07790152999995,12.2,-8.90460669800002));
#170105=CARTESIAN_POINT('Ctrl Pts',(7.07702776499994,12.2,-8.90105763700002));
#170106=CARTESIAN_POINT('Ctrl Pts',(7.07615236299994,12.2,-8.89751369100001));
#170107=CARTESIAN_POINT('Ctrl Pts',(7.07527532899995,12.2,-8.89397486500001));
#170108=CARTESIAN_POINT('Ctrl Pts',(7.07439667399994,12.2,-8.89044116400001));
#170109=CARTESIAN_POINT('Ctrl Pts',(7.07351640099994,12.2,-8.88691259500002));
#170110=CARTESIAN_POINT('Ctrl Pts',(7.07263452099994,12.2,-8.88338916200002));
#170111=CARTESIAN_POINT('Ctrl Pts',(7.07175103999995,12.2,-8.87987087200001));
#170112=CARTESIAN_POINT('Ctrl Pts',(7.07086596699994,12.2,-8.87635773100002));
#170113=CARTESIAN_POINT('Ctrl Pts',(7.06997930699995,12.2,-8.87284974500002));
#170114=CARTESIAN_POINT('Ctrl Pts',(7.06909106899994,12.2,-8.86934691900001));
#170115=CARTESIAN_POINT('Ctrl Pts',(7.06820126099994,12.2,-8.86584925900002));
#170116=CARTESIAN_POINT('Ctrl Pts',(7.06730988999994,12.2,-8.86235676900002));
#170117=CARTESIAN_POINT('Ctrl Pts',(7.06641696399994,12.2,-8.85886945800002));
#170118=CARTESIAN_POINT('Ctrl Pts',(7.06552248999994,12.2,-8.85538733200002));
#170119=CARTESIAN_POINT('Ctrl Pts',(7.06462647799994,12.2,-8.85191039400001));
#170120=CARTESIAN_POINT('Ctrl Pts',(7.06372893199994,12.2,-8.84843865100001));
#170121=CARTESIAN_POINT('Ctrl Pts',(7.06282986099994,12.2,-8.84497210900001));
#170122=CARTESIAN_POINT('Ctrl Pts',(7.06192927499995,12.2,-8.84151077400002));
#170123=CARTESIAN_POINT('Ctrl Pts',(7.06102717799994,12.2,-8.83805465100002));
#170124=CARTESIAN_POINT('Ctrl Pts',(7.06012358099994,12.2,-8.83460374700002));
#170125=CARTESIAN_POINT('Ctrl Pts',(7.05921848999994,12.2,-8.83115806600001));
#170126=CARTESIAN_POINT('Ctrl Pts',(7.05831191399994,12.2,-8.82771761700001));
#170127=CARTESIAN_POINT('Ctrl Pts',(7.05740385899994,12.2,-8.82428240200002));
#170128=CARTESIAN_POINT('Ctrl Pts',(7.05649433399994,12.2,-8.82085243000001));
#170129=CARTESIAN_POINT('Ctrl Pts',(7.05558334699995,12.2,-8.81742770600002));
#170130=CARTESIAN_POINT('Ctrl Pts',(7.05467090599995,12.2,-8.81400823500002));
#170131=CARTESIAN_POINT('Ctrl Pts',(7.05375701899994,12.2,-8.81059402400002));
#170132=CARTESIAN_POINT('Ctrl Pts',(7.05284169299994,12.2,-8.80718507700001));
#170133=CARTESIAN_POINT('Ctrl Pts',(7.05192493599994,12.2,-8.80378140200002));
#170134=CARTESIAN_POINT('Ctrl Pts',(7.05100675599994,12.2,-8.80038300300001));
#170135=CARTESIAN_POINT('Ctrl Pts',(7.05008716199995,12.2,-8.79698988800002));
#170136=CARTESIAN_POINT('Ctrl Pts',(7.04916616099994,12.2,-8.79360206200002));
#170137=CARTESIAN_POINT('Ctrl Pts',(7.04824376099995,12.2,-8.79021953000001));
#170138=CARTESIAN_POINT('Ctrl Pts',(7.04731997099994,12.2,-8.78684229900001));
#170139=CARTESIAN_POINT('Ctrl Pts',(7.04639479699994,12.2,-8.78347037400001));
#170140=CARTESIAN_POINT('Ctrl Pts',(7.04546824999994,12.2,-8.78010376100002));
#170141=CARTESIAN_POINT('Ctrl Pts',(7.04454033599994,12.2,-8.77674246600002));
#170142=CARTESIAN_POINT('Ctrl Pts',(7.04361106199995,12.2,-8.77338649600001));
#170143=CARTESIAN_POINT('Ctrl Pts',(7.04268043899994,12.2,-8.77003585600002));
#170144=CARTESIAN_POINT('Ctrl Pts',(7.04174847399995,12.2,-8.76669055200002));
#170145=CARTESIAN_POINT('Ctrl Pts',(7.04081517499994,12.2,-8.76335058900001));
#170146=CARTESIAN_POINT('Ctrl Pts',(7.03988054999994,12.2,-8.76001597500002));
#170147=CARTESIAN_POINT('Ctrl Pts',(7.03894460699994,12.2,-8.75668671600002));
#170148=CARTESIAN_POINT('Ctrl Pts',(7.03800735599994,12.2,-8.75336281500001));
#170149=CARTESIAN_POINT('Ctrl Pts',(7.03706880199994,12.2,-8.75004428000001));
#170150=CARTESIAN_POINT('Ctrl Pts',(7.03612895599995,12.2,-8.74673111600002));
#170151=CARTESIAN_POINT('Ctrl Pts',(7.03518782499994,12.2,-8.74342333000002));
#170152=CARTESIAN_POINT('Ctrl Pts',(7.03424541799994,12.2,-8.74012092800001));
#170153=CARTESIAN_POINT('Ctrl Pts',(7.03330174299994,12.2,-8.73682391500001));
#170154=CARTESIAN_POINT('Ctrl Pts',(7.03235680899994,12.2,-8.73353229700001));
#170155=CARTESIAN_POINT('Ctrl Pts',(7.03141062299995,12.2,-8.73024608200001));
#170156=CARTESIAN_POINT('Ctrl Pts',(7.03046319299995,12.2,-8.72696527400001));
#170157=CARTESIAN_POINT('Ctrl Pts',(7.02951453099994,12.2,-8.72368987800002));
#170158=CARTESIAN_POINT('Ctrl Pts',(7.02856464099994,12.2,-8.72041990300002));
#170159=CARTESIAN_POINT('Ctrl Pts',(7.02761353399994,12.2,-8.71715535200002));
#170160=CARTESIAN_POINT('Ctrl Pts',(7.02666121799994,12.2,-8.71389623300002));
#170161=CARTESIAN_POINT('Ctrl Pts',(7.02570770099994,12.2,-8.71064255100002));
#170162=CARTESIAN_POINT('Ctrl Pts',(7.02475299199994,12.2,-8.70739431300001));
#170163=CARTESIAN_POINT('Ctrl Pts',(7.02379709999994,12.2,-8.70415152400002));
#170164=CARTESIAN_POINT('Ctrl Pts',(7.02284003299994,12.2,-8.70091419100002));
#170165=CARTESIAN_POINT('Ctrl Pts',(7.02188179799994,12.2,-8.69768231900002));
#170166=CARTESIAN_POINT('Ctrl Pts',(7.02092240599994,12.2,-8.69445591400002));
#170167=CARTESIAN_POINT('Ctrl Pts',(7.01996186499994,12.2,-8.69123498300001));
#170168=CARTESIAN_POINT('Ctrl Pts',(7.01900018299995,12.2,-8.68801953100002));
#170169=CARTESIAN_POINT('Ctrl Pts',(7.01803736899994,12.2,-8.68480956600001));
#170170=CARTESIAN_POINT('Ctrl Pts',(7.01707343299995,12.2,-8.68160509100001));
#170171=CARTESIAN_POINT('Ctrl Pts',(7.01610838099994,12.2,-8.67840611400002));
#170172=CARTESIAN_POINT('Ctrl Pts',(7.01514222399994,12.2,-8.67521264000001));
#170173=CARTESIAN_POINT('Ctrl Pts',(7.01417496999994,12.2,-8.67202467700002));
#170174=CARTESIAN_POINT('Ctrl Pts',(7.01320662599994,12.2,-8.66884222900002));
#170175=CARTESIAN_POINT('Ctrl Pts',(7.01223720399994,12.2,-8.66566530400002));
#170176=CARTESIAN_POINT('Ctrl Pts',(7.01126671099995,12.2,-8.66249390500002));
#170177=CARTESIAN_POINT('Ctrl Pts',(7.01029515599994,12.2,-8.65932804100002));
#170178=CARTESIAN_POINT('Ctrl Pts',(7.00932254799994,12.2,-8.65616771800001));
#170179=CARTESIAN_POINT('Ctrl Pts',(7.00834889699994,12.2,-8.65301294000002));
#170180=CARTESIAN_POINT('Ctrl Pts',(7.00737420899994,12.2,-8.64986371400001));
#170181=CARTESIAN_POINT('Ctrl Pts',(7.00639849599995,12.2,-8.64672004800001));
#170182=CARTESIAN_POINT('Ctrl Pts',(7.00542176599994,12.2,-8.64358194500002));
#170183=CARTESIAN_POINT('Ctrl Pts',(7.00444402699994,12.2,-8.64044941300002));
#170184=CARTESIAN_POINT('Ctrl Pts',(7.00346528799995,12.2,-8.63732245800002));
#170185=CARTESIAN_POINT('Ctrl Pts',(7.00248555899995,12.2,-8.63420108600002));
#170186=CARTESIAN_POINT('Ctrl Pts',(7.00150484899994,12.2,-8.63108530300002));
#170187=CARTESIAN_POINT('Ctrl Pts',(7.00052316699994,12.2,-8.62797511400002));
#170188=CARTESIAN_POINT('Ctrl Pts',(6.99954052099995,12.2,-8.62487052700001));
#170189=CARTESIAN_POINT('Ctrl Pts',(6.99855692199994,12.2,-8.62177154700002));
#170190=CARTESIAN_POINT('Ctrl Pts',(6.99757237899994,12.2,-8.61867818100002));
#170191=CARTESIAN_POINT('Ctrl Pts',(6.99658689799994,12.2,-8.61559043400002));
#170192=CARTESIAN_POINT('Ctrl Pts',(6.99560049199994,12.2,-8.61250831300002));
#170193=CARTESIAN_POINT('Ctrl Pts',(6.99461316799994,12.2,-8.60943182400002));
#170194=CARTESIAN_POINT('Ctrl Pts',(6.99362493699994,12.2,-8.60636097400001));
#170195=CARTESIAN_POINT('Ctrl Pts',(6.99263580599994,12.2,-8.60329576700002));
#170196=CARTESIAN_POINT('Ctrl Pts',(6.99164578499994,12.2,-8.60023621100002));
#170197=CARTESIAN_POINT('Ctrl Pts',(6.99065488599994,12.2,-8.59718231200001));
#170198=CARTESIAN_POINT('Ctrl Pts',(6.98966311399994,12.2,-8.59413407600002));
#170199=CARTESIAN_POINT('Ctrl Pts',(6.98867048099994,12.2,-8.59109150800002));
#170200=CARTESIAN_POINT('Ctrl Pts',(6.98767699599994,12.2,-8.58805461600002));
#170201=CARTESIAN_POINT('Ctrl Pts',(6.98668266799994,12.2,-8.58502340600002));
#170202=CARTESIAN_POINT('Ctrl Pts',(6.98568750699994,12.2,-8.58199788300002));
#170203=CARTESIAN_POINT('Ctrl Pts',(6.98469152199994,12.2,-8.57897805400002));
#170204=CARTESIAN_POINT('Ctrl Pts',(6.98369472199994,12.2,-8.57596392400002));
#170205=CARTESIAN_POINT('Ctrl Pts',(6.98269711799994,12.2,-8.57295550200002));
#170206=CARTESIAN_POINT('Ctrl Pts',(6.98169871799994,12.2,-8.56995279200002));
#170207=CARTESIAN_POINT('Ctrl Pts',(6.98069953199994,12.2,-8.56695580000002));
#170208=CARTESIAN_POINT('Ctrl Pts',(6.97969957099994,12.2,-8.56396453400002));
#170209=CARTESIAN_POINT('Ctrl Pts',(6.97869884199994,12.2,-8.56097899900002));
#170210=CARTESIAN_POINT('Ctrl Pts',(6.97769735699994,12.2,-8.55799920200001));
#170211=CARTESIAN_POINT('Ctrl Pts',(6.97669512399994,12.2,-8.55502514800002));
#170212=CARTESIAN_POINT('Ctrl Pts',(6.97569215299994,12.2,-8.55205684500002));
#170213=CARTESIAN_POINT('Ctrl Pts',(6.97468845399994,12.2,-8.54909429700001));
#170214=CARTESIAN_POINT('Ctrl Pts',(6.97368403699994,12.2,-8.54613751400001));
#170215=CARTESIAN_POINT('Ctrl Pts',(6.97267891199994,12.2,-8.54318649800001));
#170216=CARTESIAN_POINT('Ctrl Pts',(6.97167308699994,12.2,-8.54024125700001));
#170217=CARTESIAN_POINT('Ctrl Pts',(6.97066657399994,12.2,-8.53730179900002));
#170218=CARTESIAN_POINT('Ctrl Pts',(6.96965938299994,12.2,-8.53436812800001));
#170219=CARTESIAN_POINT('Ctrl Pts',(6.96865152099994,12.2,-8.53144025000002));
#170220=CARTESIAN_POINT('Ctrl Pts',(6.96764299999994,12.2,-8.52851817400002));
#170221=CARTESIAN_POINT('Ctrl Pts',(6.96663382999994,12.2,-8.52560190500002));
#170222=CARTESIAN_POINT('Ctrl Pts',(6.96562401999994,12.2,-8.52269144800001));
#170223=CARTESIAN_POINT('Ctrl Pts',(6.96461357999994,12.2,-8.51978681100002));
#170224=CARTESIAN_POINT('Ctrl Pts',(6.96360252099994,12.2,-8.51688800000002));
#170225=CARTESIAN_POINT('Ctrl Pts',(6.96259085299994,12.2,-8.51399502000002));
#170226=CARTESIAN_POINT('Ctrl Pts',(6.96157858499994,12.2,-8.51110787900001));
#170227=CARTESIAN_POINT('Ctrl Pts',(6.96056572699994,12.2,-8.50822658400002));
#170228=CARTESIAN_POINT('Ctrl Pts',(6.95955229099994,12.2,-8.50535113900002));
#170229=CARTESIAN_POINT('Ctrl Pts',(6.95853828499994,12.2,-8.50248155200001));
#170230=CARTESIAN_POINT('Ctrl Pts',(6.95752371999995,12.2,-8.49961782800002));
#170231=CARTESIAN_POINT('Ctrl Pts',(6.95650860599994,12.2,-8.49675997600002));
#170232=CARTESIAN_POINT('Ctrl Pts',(6.95549295399994,12.2,-8.49390799900002));
#170233=CARTESIAN_POINT('Ctrl Pts',(6.95447677299994,12.2,-8.49106190600001));
#170234=CARTESIAN_POINT('Ctrl Pts',(6.95346007499994,12.2,-8.48822170300001));
#170235=CARTESIAN_POINT('Ctrl Pts',(6.95244286799994,12.2,-8.48538739600002));
#170236=CARTESIAN_POINT('Ctrl Pts',(6.95142516299994,12.2,-8.48255899100002));
#170237=CARTESIAN_POINT('Ctrl Pts',(6.95040697199994,12.2,-8.47973649400002));
#170238=CARTESIAN_POINT('Ctrl Pts',(6.94938830399995,12.2,-8.47691991200002));
#170239=CARTESIAN_POINT('Ctrl Pts',(6.94836916999994,12.2,-8.47410925300002));
#170240=CARTESIAN_POINT('Ctrl Pts',(6.94734957799994,12.2,-8.47130452200001));
#170241=CARTESIAN_POINT('Ctrl Pts',(6.94632954299994,12.2,-8.46850572500001));
#170242=CARTESIAN_POINT('Ctrl Pts',(6.94530907199994,12.2,-8.46571286900001));
#170243=CARTESIAN_POINT('Ctrl Pts',(6.94428817599994,12.2,-8.46292596000002));
#170244=CARTESIAN_POINT('Ctrl Pts',(6.94326686599994,12.2,-8.46014500600001));
#170245=CARTESIAN_POINT('Ctrl Pts',(6.94224515399994,12.2,-8.45737001200002));
#170246=CARTESIAN_POINT('Ctrl Pts',(6.94122304799994,12.2,-8.45460098400002));
#170247=CARTESIAN_POINT('Ctrl Pts',(6.94020055999995,12.2,-8.45183793000002));
#170248=CARTESIAN_POINT('Ctrl Pts',(6.93917770099994,12.2,-8.44908085600002));
#170249=CARTESIAN_POINT('Ctrl Pts',(6.93815448099994,12.2,-8.44632976900002));
#170250=CARTESIAN_POINT('Ctrl Pts',(6.93713091199994,12.2,-8.44358467400001));
#170251=CARTESIAN_POINT('Ctrl Pts',(6.93610700299994,12.2,-8.44084557900001));
#170252=CARTESIAN_POINT('Ctrl Pts',(6.93508276499994,12.2,-8.43811248900002));
#170253=CARTESIAN_POINT('Ctrl Pts',(6.93405820999994,12.2,-8.43538541100001));
#170254=CARTESIAN_POINT('Ctrl Pts',(6.93303334799994,12.2,-8.43266435400002));
#170255=CARTESIAN_POINT('Ctrl Pts',(6.93200819099994,12.2,-8.42994932100002));
#170256=CARTESIAN_POINT('Ctrl Pts',(6.93098274699994,12.2,-8.42724032100002));
#170257=CARTESIAN_POINT('Ctrl Pts',(6.92995702999994,12.2,-8.42453735900002));
#170258=CARTESIAN_POINT('Ctrl Pts',(6.92893105099994,12.2,-8.42184044300001));
#170259=CARTESIAN_POINT('Ctrl Pts',(6.92790481799994,12.2,-8.41914957800002));
#170260=CARTESIAN_POINT('Ctrl Pts',(6.92687834499995,12.2,-8.41646477200002));
#170261=CARTESIAN_POINT('Ctrl Pts',(6.92585164099994,12.2,-8.41378603000001));
#170262=CARTESIAN_POINT('Ctrl Pts',(6.92482471899995,12.2,-8.41111336100001));
#170263=CARTESIAN_POINT('Ctrl Pts',(6.92379758999994,12.2,-8.40844676800002));
#170264=CARTESIAN_POINT('Ctrl Pts',(6.92277026199994,12.2,-8.40578626200001));
#170265=CARTESIAN_POINT('Ctrl Pts',(6.92174274999994,12.2,-8.40313184700002));
#170266=CARTESIAN_POINT('Ctrl Pts',(6.92071506399994,12.2,-8.40048352900002));
#170267=CARTESIAN_POINT('Ctrl Pts',(6.91968721499994,12.2,-8.39784131600002));
#170268=CARTESIAN_POINT('Ctrl Pts',(6.91865921499994,12.2,-8.39520521500001));
#170269=CARTESIAN_POINT('Ctrl Pts',(6.91763107299994,12.2,-8.39257523200001));
#170270=CARTESIAN_POINT('Ctrl Pts',(6.91660280299994,12.2,-8.38995137300002));
#170271=CARTESIAN_POINT('Ctrl Pts',(6.91557441499994,12.2,-8.38733364600002));
#170272=CARTESIAN_POINT('Ctrl Pts',(6.91454591999995,12.2,-8.38472205600001));
#170273=CARTESIAN_POINT('Ctrl Pts',(6.91351733199994,12.2,-8.38211661100001));
#170274=CARTESIAN_POINT('Ctrl Pts',(6.91248865999994,12.2,-8.37951731700001));
#170275=CARTESIAN_POINT('Ctrl Pts',(6.91145991499994,12.2,-8.37692418200002));
#170276=CARTESIAN_POINT('Ctrl Pts',(6.91043111099994,12.2,-8.37433721000002));
#170277=CARTESIAN_POINT('Ctrl Pts',(6.90940225899995,12.2,-8.37175641100002));
#170278=CARTESIAN_POINT('Ctrl Pts',(6.90837336899994,12.2,-8.36918179000002));
#170279=CARTESIAN_POINT('Ctrl Pts',(6.90734445199994,12.2,-8.36661335300001));
#170280=CARTESIAN_POINT('Ctrl Pts',(6.90631552399994,12.2,-8.36405110800002));
#170281=CARTESIAN_POINT('Ctrl Pts',(6.90528659299994,12.2,-8.36149506200002));
#170282=CARTESIAN_POINT('Ctrl Pts',(6.90425767199994,12.2,-8.35894522000002));
#170283=CARTESIAN_POINT('Ctrl Pts',(6.90322877199994,12.2,-8.35640159100001));
#170284=CARTESIAN_POINT('Ctrl Pts',(6.90219990499994,12.2,-8.35386418100001));
#170285=CARTESIAN_POINT('Ctrl Pts',(6.90117108399994,12.2,-8.35133299500002));
#170286=CARTESIAN_POINT('Ctrl Pts',(6.90014232099994,12.2,-8.34880804200001));
#170287=CARTESIAN_POINT('Ctrl Pts',(6.89911362499994,12.2,-8.34628932700002));
#170288=CARTESIAN_POINT('Ctrl Pts',(6.89808501099994,12.2,-8.34377685900002));
#170289=CARTESIAN_POINT('Ctrl Pts',(6.89705648999994,12.2,-8.34127064300001));
#170290=CARTESIAN_POINT('Ctrl Pts',(6.89602807299995,12.2,-8.33877068600002));
#170291=CARTESIAN_POINT('Ctrl Pts',(6.89499977499994,12.2,-8.33627699600001));
#170292=CARTESIAN_POINT('Ctrl Pts',(6.89397160499994,12.2,-8.33378957900001));
#170293=CARTESIAN_POINT('Ctrl Pts',(6.89294357699994,12.2,-8.33130844200002));
#170294=CARTESIAN_POINT('Ctrl Pts',(6.89191570099994,12.2,-8.32883359100002));
#170295=CARTESIAN_POINT('Ctrl Pts',(6.89088799199994,12.2,-8.32636503500002));
#170296=CARTESIAN_POINT('Ctrl Pts',(6.88986046099994,12.2,-8.32390277900002));
#170297=CARTESIAN_POINT('Ctrl Pts',(6.88883311899994,12.2,-8.32144682900001));
#170298=CARTESIAN_POINT('Ctrl Pts',(6.88780597999994,12.2,-8.31899719600001));
#170299=CARTESIAN_POINT('Ctrl Pts',(6.88677905699994,12.2,-8.31655388200002));
#170300=CARTESIAN_POINT('Ctrl Pts',(6.88575235999994,12.2,-8.31411689700002));
#170301=CARTESIAN_POINT('Ctrl Pts',(6.88472590399994,12.2,-8.31168624500001));
#170302=CARTESIAN_POINT('Ctrl Pts',(6.88369969899994,12.2,-8.30926193800002));
#170303=CARTESIAN_POINT('Ctrl Pts',(6.88267375899994,12.2,-8.30684397800002));
#170304=CARTESIAN_POINT('Ctrl Pts',(6.88164809599995,12.2,-8.30443237500001));
#170305=CARTESIAN_POINT('Ctrl Pts',(6.88062272399995,12.2,-8.30202713300002));
#170306=CARTESIAN_POINT('Ctrl Pts',(6.87959765299994,12.2,-8.29962826200001));
#170307=CARTESIAN_POINT('Ctrl Pts',(6.87857289699994,12.2,-8.29723576700001));
#170308=CARTESIAN_POINT('Ctrl Pts',(6.87754846999994,12.2,-8.29484965700001));
#170309=CARTESIAN_POINT('Ctrl Pts',(6.87652438199994,12.2,-8.29246993600002));
#170310=CARTESIAN_POINT('Ctrl Pts',(6.87550064899995,12.2,-8.29009661300002));
#170311=CARTESIAN_POINT('Ctrl Pts',(6.87447728099994,12.2,-8.28772969500001));
#170312=CARTESIAN_POINT('Ctrl Pts',(6.87345429199994,12.2,-8.28536918900001));
#170313=CARTESIAN_POINT('Ctrl Pts',(6.87243169499994,12.2,-8.28301510100001));
#170314=CARTESIAN_POINT('Ctrl Pts',(6.87140950299994,12.2,-8.28066743900001));
#170315=CARTESIAN_POINT('Ctrl Pts',(6.87038772899994,12.2,-8.27832621000002));
#170316=CARTESIAN_POINT('Ctrl Pts',(6.86936638499994,12.2,-8.27599142100001));
#170317=CARTESIAN_POINT('Ctrl Pts',(6.86834548499994,12.2,-8.27366307800002));
#170318=CARTESIAN_POINT('Ctrl Pts',(6.86732504299994,12.2,-8.27134119000002));
#170319=CARTESIAN_POINT('Ctrl Pts',(6.86630506999995,12.2,-8.26902576200002));
#170320=CARTESIAN_POINT('Ctrl Pts',(6.86528557999995,12.2,-8.26671680300001));
#170321=CARTESIAN_POINT('Ctrl Pts',(6.86426658699994,12.2,-8.26441431900001));
#170322=CARTESIAN_POINT('Ctrl Pts',(6.86324810299995,12.2,-8.26211831700002));
#170323=CARTESIAN_POINT('Ctrl Pts',(6.86223014199994,12.2,-8.25982880500002));
#170324=CARTESIAN_POINT('Ctrl Pts',(6.86121271699994,12.2,-8.25754578900002));
#170325=CARTESIAN_POINT('Ctrl Pts',(6.86019584299994,12.2,-8.25526927700002));
#170326=CARTESIAN_POINT('Ctrl Pts',(6.85917953099994,12.2,-8.25299927600001));
#170327=CARTESIAN_POINT('Ctrl Pts',(6.85816379599994,12.2,-8.25073579300001));
#170328=CARTESIAN_POINT('Ctrl Pts',(6.85714865199994,12.2,-8.24847883600001));
#170329=CARTESIAN_POINT('Ctrl Pts',(6.85613410999995,12.2,-8.24622841000001));
#170330=CARTESIAN_POINT('Ctrl Pts',(6.85512018599994,12.2,-8.24398452500001));
#170331=CARTESIAN_POINT('Ctrl Pts',(6.85410689299994,12.2,-8.24174718600002));
#170332=CARTESIAN_POINT('Ctrl Pts',(6.85309424499994,12.2,-8.23951640200002));
#170333=CARTESIAN_POINT('Ctrl Pts',(6.85208225499994,12.2,-8.23729217900001));
#170334=CARTESIAN_POINT('Ctrl Pts',(6.85107093599994,12.2,-8.23507452400002));
#170335=CARTESIAN_POINT('Ctrl Pts',(6.85006030399994,12.2,-8.23286344400002));
#170336=CARTESIAN_POINT('Ctrl Pts',(6.84905037099995,12.2,-8.23065895000001));
#170337=CARTESIAN_POINT('Ctrl Pts',(6.84804115199994,12.2,-8.22846104400002));
#170338=CARTESIAN_POINT('Ctrl Pts',(6.84703265999994,12.2,-8.22626973500002));
#170339=CARTESIAN_POINT('Ctrl Pts',(6.84602490999994,12.2,-8.22408503200002));
#170340=CARTESIAN_POINT('Ctrl Pts',(6.84501791499994,12.2,-8.22190694200001));
#170341=CARTESIAN_POINT('Ctrl Pts',(6.84401168999995,12.2,-8.21973547000002));
#170342=CARTESIAN_POINT('Ctrl Pts',(6.84300624899994,12.2,-8.21757062500001));
#170343=CARTESIAN_POINT('Ctrl Pts',(6.84200160499994,12.2,-8.21541241600002));
#170344=CARTESIAN_POINT('Ctrl Pts',(6.84099777399994,12.2,-8.21326084700001));
#170345=CARTESIAN_POINT('Ctrl Pts',(6.83999476999994,12.2,-8.21111592700002));
#170346=CARTESIAN_POINT('Ctrl Pts',(6.83899260499994,12.2,-8.20897766300002));
#170347=CARTESIAN_POINT('Ctrl Pts',(6.83799129699994,12.2,-8.20684606400001));
#170348=CARTESIAN_POINT('Ctrl Pts',(6.83699085699994,12.2,-8.20472113600001));
#170349=CARTESIAN_POINT('Ctrl Pts',(6.83599130199994,12.2,-8.20260288400002));
#170350=CARTESIAN_POINT('Ctrl Pts',(6.83499264499994,12.2,-8.20049132000002));
#170351=CARTESIAN_POINT('Ctrl Pts',(6.83399489999994,12.2,-8.19838644900001));
#170352=CARTESIAN_POINT('Ctrl Pts',(6.83299808299994,12.2,-8.19628827900001));
#170353=CARTESIAN_POINT('Ctrl Pts',(6.83200220999994,12.2,-8.19419681600002));
#170354=CARTESIAN_POINT('Ctrl Pts',(6.83100729199994,12.2,-8.19211207100001));
#170355=CARTESIAN_POINT('Ctrl Pts',(6.83001334499994,12.2,-8.19003404700002));
#170356=CARTESIAN_POINT('Ctrl Pts',(6.82902038699994,12.2,-8.18796275400001));
#170357=CARTESIAN_POINT('Ctrl Pts',(6.82802842799994,12.2,-8.18589820000001));
#170358=CARTESIAN_POINT('Ctrl Pts',(6.82703748599994,12.2,-8.18384039100001));
#170359=CARTESIAN_POINT('Ctrl Pts',(6.82604757499995,12.2,-8.18178933600001));
#170360=CARTESIAN_POINT('Ctrl Pts',(6.82505870999995,12.2,-8.17974504100001));
#170361=CARTESIAN_POINT('Ctrl Pts',(6.82407090599995,12.2,-8.17770751500002));
#170362=CARTESIAN_POINT('Ctrl Pts',(6.82308417899994,12.2,-8.17567676500002));
#170363=CARTESIAN_POINT('Ctrl Pts',(6.82209854199994,12.2,-8.17365279700002));
#170364=CARTESIAN_POINT('Ctrl Pts',(6.82111401199994,12.2,-8.17163562200001));
#170365=CARTESIAN_POINT('Ctrl Pts',(6.82013060499994,12.2,-8.16962524400001));
#170366=CARTESIAN_POINT('Ctrl Pts',(6.81914833299994,12.2,-8.16762167300002));
#170367=CARTESIAN_POINT('Ctrl Pts',(6.81816721399994,12.2,-8.16562491600001));
#170368=CARTESIAN_POINT('Ctrl Pts',(6.81718726299994,12.2,-8.16363498000002));
#170369=CARTESIAN_POINT('Ctrl Pts',(6.81620849499994,12.2,-8.16165187500001));
#170370=CARTESIAN_POINT('Ctrl Pts',(6.81523092699994,12.2,-8.15967560500001));
#170371=CARTESIAN_POINT('Ctrl Pts',(6.81425457199994,12.2,-8.15770618000002));
#170372=CARTESIAN_POINT('Ctrl Pts',(6.81327944699994,12.2,-8.15574360800002));
#170373=CARTESIAN_POINT('Ctrl Pts',(6.81230556799994,12.2,-8.15378789600001));
#170374=CARTESIAN_POINT('Ctrl Pts',(6.81133295099994,12.2,-8.15183905000002));
#170375=CARTESIAN_POINT('Ctrl Pts',(6.81036160899994,12.2,-8.14989708200001));
#170376=CARTESIAN_POINT('Ctrl Pts',(6.80939156199994,12.2,-8.14796199600002));
#170377=CARTESIAN_POINT('Ctrl Pts',(6.80842282199994,12.2,-8.14603380000002));
#170378=CARTESIAN_POINT('Ctrl Pts',(6.80745540699994,12.2,-8.14411250400001));
#170379=CARTESIAN_POINT('Ctrl Pts',(6.80648933299994,12.2,-8.14219811500001));
#170380=CARTESIAN_POINT('Ctrl Pts',(6.80552461599994,12.2,-8.14029063900002));
#170381=CARTESIAN_POINT('Ctrl Pts',(6.80456127099994,12.2,-8.13839008500001));
#170382=CARTESIAN_POINT('Ctrl Pts',(6.80359931599994,12.2,-8.13649646300002));
#170383=CARTESIAN_POINT('Ctrl Pts',(6.80263876599994,12.2,-8.13460977800002));
#170384=CARTESIAN_POINT('Ctrl Pts',(6.80167963599994,12.2,-8.13273003800001));
#170385=CARTESIAN_POINT('Ctrl Pts',(6.80072194599994,12.2,-8.13085725200001));
#170386=CARTESIAN_POINT('Ctrl Pts',(6.79976570799994,12.2,-8.12899142800001));
#170387=CARTESIAN_POINT('Ctrl Pts',(6.79881094199994,12.2,-8.12713257400001));
#170388=CARTESIAN_POINT('Ctrl Pts',(6.79785766299994,12.2,-8.12528069600001));
#170389=CARTESIAN_POINT('Ctrl Pts',(6.79690588799994,12.2,-8.12343580400002));
#170390=CARTESIAN_POINT('Ctrl Pts',(6.79595563299995,12.2,-8.12159790600001));
#170391=CARTESIAN_POINT('Ctrl Pts',(6.79500691399994,12.2,-8.11976700800002));
#170392=CARTESIAN_POINT('Ctrl Pts',(6.79405974999994,12.2,-8.11794312000002));
#170393=CARTESIAN_POINT('Ctrl Pts',(6.79311415699994,12.2,-8.11612625000001));
#170394=CARTESIAN_POINT('Ctrl Pts',(6.79217014999994,12.2,-8.11431640400002));
#170395=CARTESIAN_POINT('Ctrl Pts',(6.79122774799994,12.2,-8.11251359100002));
#170396=CARTESIAN_POINT('Ctrl Pts',(6.79028696699994,12.2,-8.11071782000001));
#170397=CARTESIAN_POINT('Ctrl Pts',(6.78934782399994,12.2,-8.10892909900002));
#170398=CARTESIAN_POINT('Ctrl Pts',(6.78841033799994,12.2,-8.10714743400002));
#170399=CARTESIAN_POINT('Ctrl Pts',(6.78747452299994,12.2,-8.10537283700001));
#170400=CARTESIAN_POINT('Ctrl Pts',(6.78654039799994,12.2,-8.10360531100002));
#170401=CARTESIAN_POINT('Ctrl Pts',(6.78560798099994,12.2,-8.10184486900001));
#170402=CARTESIAN_POINT('Ctrl Pts',(6.78467728799995,12.2,-8.10009151600001));
#170403=CARTESIAN_POINT('Ctrl Pts',(6.78374833699994,12.2,-8.09834526200002));
#170404=CARTESIAN_POINT('Ctrl Pts',(6.78282114499994,12.2,-8.09660611400002));
#170405=CARTESIAN_POINT('Ctrl Pts',(6.78189572999995,12.2,-8.09487408000002));
#170406=CARTESIAN_POINT('Ctrl Pts',(6.78097211099994,12.2,-8.09314916800002));
#170407=CARTESIAN_POINT('Ctrl Pts',(6.78005030299994,12.2,-8.09143138900002));
#170408=CARTESIAN_POINT('Ctrl Pts',(6.77913032499994,12.2,-8.08972074800002));
#170409=CARTESIAN_POINT('Ctrl Pts',(6.77821219499994,12.2,-8.08801725500001));
#170410=CARTESIAN_POINT('Ctrl Pts',(6.77729593099994,12.2,-8.08632091800002));
#170411=CARTESIAN_POINT('Ctrl Pts',(6.77638154999994,12.2,-8.08463174500002));
#170412=CARTESIAN_POINT('Ctrl Pts',(6.77546907099994,12.2,-8.08294974400001));
#170413=CARTESIAN_POINT('Ctrl Pts',(6.77455851199994,12.2,-8.08127492400001));
#170414=CARTESIAN_POINT('Ctrl Pts',(6.77364988999994,12.2,-8.07960729300002));
#170415=CARTESIAN_POINT('Ctrl Pts',(6.77274322499994,12.2,-8.07794686000002));
#170416=CARTESIAN_POINT('Ctrl Pts',(6.77183853299994,12.2,-8.07629363200002));
#170417=CARTESIAN_POINT('Ctrl Pts',(6.77093583499994,12.2,-8.07464761900002));
#170418=CARTESIAN_POINT('Ctrl Pts',(6.77003514699994,12.2,-8.07300882800002));
#170419=CARTESIAN_POINT('Ctrl Pts',(6.76913648999995,12.2,-8.07137726900002));
#170420=CARTESIAN_POINT('Ctrl Pts',(6.76823988099994,12.2,-8.06975294900001));
#170421=CARTESIAN_POINT('Ctrl Pts',(6.76734533799995,12.2,-8.06813587700002));
#170422=CARTESIAN_POINT('Ctrl Pts',(6.76645288099994,12.2,-8.06652606100002));
#170423=CARTESIAN_POINT('Ctrl Pts',(6.76556252799994,12.2,-8.06492351100001));
#170424=CARTESIAN_POINT('Ctrl Pts',(6.76467429899994,12.2,-8.06332823600002));
#170425=CARTESIAN_POINT('Ctrl Pts',(6.76378821099994,12.2,-8.06174024100001));
#170426=CARTESIAN_POINT('Ctrl Pts',(6.76290428599994,12.2,-8.06015953800001));
#170427=CARTESIAN_POINT('Ctrl Pts',(6.76202253899994,12.2,-8.05858613400002));
#170428=CARTESIAN_POINT('Ctrl Pts',(6.76114299199994,12.2,-8.05702003800001));
#170429=CARTESIAN_POINT('Ctrl Pts',(6.76026566399995,12.2,-8.05546125900002));
#170430=CARTESIAN_POINT('Ctrl Pts',(6.75939057299995,12.2,-8.05390980500002));
#170431=CARTESIAN_POINT('Ctrl Pts',(6.75851773999994,12.2,-8.05236568400002));
#170432=CARTESIAN_POINT('Ctrl Pts',(6.75764718299994,12.2,-8.05082890700002));
#170433=CARTESIAN_POINT('Ctrl Pts',(6.75677892299994,12.2,-8.04929948100002));
#170434=CARTESIAN_POINT('Ctrl Pts',(6.75591297799994,12.2,-8.04777741600001));
#170435=CARTESIAN_POINT('Ctrl Pts',(6.75504936899994,12.2,-8.04626271800002));
#170436=CARTESIAN_POINT('Ctrl Pts',(6.75418811399994,12.2,-8.04475539900002));
#170437=CARTESIAN_POINT('Ctrl Pts',(6.75332923499994,12.2,-8.04325546600002));
#170438=CARTESIAN_POINT('Ctrl Pts',(6.75247275099994,12.2,-8.04176292900001));
#170439=CARTESIAN_POINT('Ctrl Pts',(6.75161868199995,12.2,-8.04027779500002));
#170440=CARTESIAN_POINT('Ctrl Pts',(6.75076704799995,12.2,-8.03880007500002));
#170441=CARTESIAN_POINT('Ctrl Pts',(6.74991786899994,12.2,-8.03732977600001));
#170442=CARTESIAN_POINT('Ctrl Pts',(6.74907116499995,12.2,-8.03586690800002));
#170443=CARTESIAN_POINT('Ctrl Pts',(6.74822695699994,12.2,-8.03441148000001));
#170444=CARTESIAN_POINT('Ctrl Pts',(6.74738526499994,12.2,-8.03296350100002));
#170445=CARTESIAN_POINT('Ctrl Pts',(6.74654610999994,12.2,-8.03152298000001));
#170446=CARTESIAN_POINT('Ctrl Pts',(6.74570951199994,12.2,-8.03008992500001));
#170447=CARTESIAN_POINT('Ctrl Pts',(6.74487549099994,12.2,-8.02866434600002));
#170448=CARTESIAN_POINT('Ctrl Pts',(6.74404406899995,12.2,-8.02724625000002));
#170449=CARTESIAN_POINT('Ctrl Pts',(6.74321526699995,12.2,-8.02583564900001));
#170450=CARTESIAN_POINT('Ctrl Pts',(6.74238910499994,12.2,-8.02443255100002));
#170451=CARTESIAN_POINT('Ctrl Pts',(6.74156560399994,12.2,-8.02303696500001));
#170452=CARTESIAN_POINT('Ctrl Pts',(6.74074478399994,12.2,-8.02164890000002));
#170453=CARTESIAN_POINT('Ctrl Pts',(6.73992666899994,12.2,-8.02026836500002));
#170454=CARTESIAN_POINT('Ctrl Pts',(6.73911127899994,12.2,-8.01889537000001));
#170455=CARTESIAN_POINT('Ctrl Pts',(6.73829863399994,12.2,-8.01752992300001));
#170456=CARTESIAN_POINT('Ctrl Pts',(6.73748875699994,12.2,-8.01617203400001));
#170457=CARTESIAN_POINT('Ctrl Pts',(6.73668166999994,12.2,-8.01482171200002));
#170458=CARTESIAN_POINT('Ctrl Pts',(6.73587739199994,12.2,-8.01347896600002));
#170459=CARTESIAN_POINT('Ctrl Pts',(6.73507594699994,12.2,-8.01214380700002));
#170460=CARTESIAN_POINT('Ctrl Pts',(6.73427735599994,12.2,-8.01081624200001));
#170461=CARTESIAN_POINT('Ctrl Pts',(6.73348164099994,12.2,-8.00949628200001));
#170462=CARTESIAN_POINT('Ctrl Pts',(6.73268882399994,12.2,-8.00818393500002));
#170463=CARTESIAN_POINT('Ctrl Pts',(6.73189892699994,12.2,-8.00687921200002));
#170464=CARTESIAN_POINT('Ctrl Pts',(6.73111197299994,12.2,-8.00558212100002));
#170465=CARTESIAN_POINT('Ctrl Pts',(6.73032798299994,12.2,-8.00429267200002));
#170466=CARTESIAN_POINT('Ctrl Pts',(6.72954697899995,12.2,-8.00301087500002));
#170467=CARTESIAN_POINT('Ctrl Pts',(6.72876898499994,12.2,-8.00173673800002));
#170468=CARTESIAN_POINT('Ctrl Pts',(6.72799402199994,12.2,-8.00047027200002));
#170469=CARTESIAN_POINT('Ctrl Pts',(6.72722211399994,12.2,-7.99921148700002));
#170470=CARTESIAN_POINT('Ctrl Pts',(6.72645328299994,12.2,-7.99796039100002));
#170471=CARTESIAN_POINT('Ctrl Pts',(6.72568755199995,12.2,-7.99671699400001));
#170472=CARTESIAN_POINT('Ctrl Pts',(6.72492494399994,12.2,-7.99548130700002));
#170473=CARTESIAN_POINT('Ctrl Pts',(6.72416548199994,12.2,-7.99425333800002));
#170474=CARTESIAN_POINT('Ctrl Pts',(6.72340918899994,12.2,-7.99303309800001));
#170475=CARTESIAN_POINT('Ctrl Pts',(6.72265608899994,12.2,-7.99182059500002));
#170476=CARTESIAN_POINT('Ctrl Pts',(6.72190620499994,12.2,-7.99061584100001));
#170477=CARTESIAN_POINT('Ctrl Pts',(6.72115955899995,12.2,-7.98941884400002));
#170478=CARTESIAN_POINT('Ctrl Pts',(6.72041617599994,12.2,-7.98822961300001));
#170479=CARTESIAN_POINT('Ctrl Pts',(6.71967607999994,12.2,-7.98704816100001));
#170480=CARTESIAN_POINT('Ctrl Pts',(6.71893929399995,12.2,-7.98587449600002));
#170481=CARTESIAN_POINT('Ctrl Pts',(6.71820584199994,12.2,-7.98470862800002));
#170482=CARTESIAN_POINT('Ctrl Pts',(6.71747574699994,12.2,-7.98355056600002));
#170483=CARTESIAN_POINT('Ctrl Pts',(6.71674903499994,12.2,-7.98240032100002));
#170484=CARTESIAN_POINT('Ctrl Pts',(6.71602572899994,12.2,-7.98125790400002));
#170485=CARTESIAN_POINT('Ctrl Pts',(6.71530585299994,12.2,-7.98012332400001));
#170486=CARTESIAN_POINT('Ctrl Pts',(6.71458943199994,12.2,-7.97899659000001));
#170487=CARTESIAN_POINT('Ctrl Pts',(6.71387649099994,12.2,-7.97787771300002));
#170488=CARTESIAN_POINT('Ctrl Pts',(6.71316705499994,12.2,-7.97676670400002));
#170489=CARTESIAN_POINT('Ctrl Pts',(6.71246114699994,12.2,-7.97566357200001));
#170490=CARTESIAN_POINT('Ctrl Pts',(6.71175879199994,12.2,-7.97456832700002));
#170491=CARTESIAN_POINT('Ctrl Pts',(6.71106001699994,12.2,-7.97348098000001));
#170492=CARTESIAN_POINT('Ctrl Pts',(6.71036484499994,12.2,-7.97240154000002));
#170493=CARTESIAN_POINT('Ctrl Pts',(6.70967330099994,12.2,-7.97133002000002));
#170494=CARTESIAN_POINT('Ctrl Pts',(6.70898541199994,12.2,-7.97026642700001));
#170495=CARTESIAN_POINT('Ctrl Pts',(6.70830120299994,12.2,-7.96921077400001));
#170496=CARTESIAN_POINT('Ctrl Pts',(6.70762069999994,12.2,-7.96816306900002));
#170497=CARTESIAN_POINT('Ctrl Pts',(6.70694392699994,12.2,-7.96712332400002));
#170498=CARTESIAN_POINT('Ctrl Pts',(6.70627090999995,12.2,-7.96609155000001));
#170499=CARTESIAN_POINT('Ctrl Pts',(6.70560167699994,12.2,-7.96506775500001));
#170500=CARTESIAN_POINT('Ctrl Pts',(6.70493625199994,12.2,-7.96405195200002));
#170501=CARTESIAN_POINT('Ctrl Pts',(6.70427466299994,12.2,-7.96304415000002));
#170502=CARTESIAN_POINT('Ctrl Pts',(6.70361693399994,12.2,-7.96204436100002));
#170503=CARTESIAN_POINT('Ctrl Pts',(6.70296309299995,12.2,-7.96105259300001));
#170504=CARTESIAN_POINT('Ctrl Pts',(6.70231316599994,12.2,-7.96006886000002));
#170505=CARTESIAN_POINT('Ctrl Pts',(6.70166717899995,12.2,-7.95909317200002));
#170506=CARTESIAN_POINT('Ctrl Pts',(6.70102515999995,12.2,-7.95812553600002));
#170507=CARTESIAN_POINT('Ctrl Pts',(6.70038713599994,12.2,-7.95716596700001));
#170508=CARTESIAN_POINT('Ctrl Pts',(6.69975313299994,12.2,-7.95621447500002));
#170509=CARTESIAN_POINT('Ctrl Pts',(6.69912317899994,12.2,-7.95527107000002));
#170510=CARTESIAN_POINT('Ctrl Pts',(6.69849730099994,12.2,-7.95433576200002));
#170511=CARTESIAN_POINT('Ctrl Pts',(6.69787552599994,12.2,-7.95340856300002));
#170512=CARTESIAN_POINT('Ctrl Pts',(6.69725788299994,12.2,-7.95248948500002));
#170513=CARTESIAN_POINT('Ctrl Pts',(6.69664439799995,12.2,-7.95157853800001));
#170514=CARTESIAN_POINT('Ctrl Pts',(6.69603509999994,12.2,-7.95067573100001));
#170515=CARTESIAN_POINT('Ctrl Pts',(6.69543001599994,12.2,-7.94978107900001));
#170516=CARTESIAN_POINT('Ctrl Pts',(6.69482917499994,12.2,-7.94889459000002));
#170517=CARTESIAN_POINT('Ctrl Pts',(6.69423260499994,12.2,-7.94801627700001));
#170518=CARTESIAN_POINT('Ctrl Pts',(6.69364033499994,12.2,-7.94714614900002));
#170519=CARTESIAN_POINT('Ctrl Pts',(6.69305239199994,12.2,-7.94628422000001));
#170520=CARTESIAN_POINT('Ctrl Pts',(6.69246880599994,12.2,-7.94543049900001));
#170521=CARTESIAN_POINT('Ctrl Pts',(6.69188960599994,12.2,-7.94458500000002));
#170522=CARTESIAN_POINT('Ctrl Pts',(6.69131482099995,12.2,-7.94374773000002));
#170523=CARTESIAN_POINT('Ctrl Pts',(6.69074447799994,12.2,-7.94291870500002));
#170524=CARTESIAN_POINT('Ctrl Pts',(6.69017860899995,12.2,-7.94209793300002));
#170525=CARTESIAN_POINT('Ctrl Pts',(6.68961724099994,12.2,-7.94128542600002));
#170526=CARTESIAN_POINT('Ctrl Pts',(6.68906040599994,12.2,-7.94048119900002));
#170527=CARTESIAN_POINT('Ctrl Pts',(6.68850813299994,12.2,-7.93968525900001));
#170528=CARTESIAN_POINT('Ctrl Pts',(6.68796045099994,12.2,-7.93889762000001));
#170529=CARTESIAN_POINT('Ctrl Pts',(6.68741739099994,12.2,-7.93811829200001));
#170530=CARTESIAN_POINT('Ctrl Pts',(6.68687898199994,12.2,-7.93734729000001));
#170531=CARTESIAN_POINT('Ctrl Pts',(6.68634525499994,12.2,-7.93658462300002));
#170532=CARTESIAN_POINT('Ctrl Pts',(6.68581928699994,12.2,-7.93583464600002));
#170533=CARTESIAN_POINT('Ctrl Pts',(6.68540286299995,12.2,-7.93524212600002));
#170534=CARTESIAN_POINT('Ctrl Pts',(6.68509340699995,12.2,-7.93480250500001));
#170535=CARTESIAN_POINT('Ctrl Pts',(6.68488903399994,12.2,-7.93451247200001));
#170536=CARTESIAN_POINT('Ctrl Pts',(6.68478856699994,12.2,-7.93436996900001));
#170537=CARTESIAN_POINT('Ctrl Pts',(6.68478856699994,15.2,-7.93436996900001));
#170538=CARTESIAN_POINT('Ctrl Pts',(6.68488903399994,15.2,-7.93451247200001));
#170539=CARTESIAN_POINT('Ctrl Pts',(6.68509340699995,15.2,-7.93480250500001));
#170540=CARTESIAN_POINT('Ctrl Pts',(6.68540286299995,15.2,-7.93524212600002));
#170541=CARTESIAN_POINT('Ctrl Pts',(6.68581928699994,15.2,-7.93583464600002));
#170542=CARTESIAN_POINT('Ctrl Pts',(6.68634525499994,15.2,-7.93658462300002));
#170543=CARTESIAN_POINT('Ctrl Pts',(6.68687898199994,15.2,-7.93734729000001));
#170544=CARTESIAN_POINT('Ctrl Pts',(6.68741739099994,15.2,-7.93811829200001));
#170545=CARTESIAN_POINT('Ctrl Pts',(6.68796045099994,15.2,-7.93889762000001));
#170546=CARTESIAN_POINT('Ctrl Pts',(6.68850813299994,15.2,-7.93968525900001));
#170547=CARTESIAN_POINT('Ctrl Pts',(6.68906040599994,15.2,-7.94048119900002));
#170548=CARTESIAN_POINT('Ctrl Pts',(6.68961724099994,15.2,-7.94128542600002));
#170549=CARTESIAN_POINT('Ctrl Pts',(6.69017860899995,15.2,-7.94209793300002));
#170550=CARTESIAN_POINT('Ctrl Pts',(6.69074447799994,15.2,-7.94291870500002));
#170551=CARTESIAN_POINT('Ctrl Pts',(6.69131482099995,15.2,-7.94374773000002));
#170552=CARTESIAN_POINT('Ctrl Pts',(6.69188960599994,15.2,-7.94458500000002));
#170553=CARTESIAN_POINT('Ctrl Pts',(6.69246880599994,15.2,-7.94543049900001));
#170554=CARTESIAN_POINT('Ctrl Pts',(6.69305239199994,15.2,-7.94628422000001));
#170555=CARTESIAN_POINT('Ctrl Pts',(6.69364033499994,15.2,-7.94714614900002));
#170556=CARTESIAN_POINT('Ctrl Pts',(6.69423260499994,15.2,-7.94801627700001));
#170557=CARTESIAN_POINT('Ctrl Pts',(6.69482917499994,15.2,-7.94889459000002));
#170558=CARTESIAN_POINT('Ctrl Pts',(6.69543001599994,15.2,-7.94978107900001));
#170559=CARTESIAN_POINT('Ctrl Pts',(6.69603509999994,15.2,-7.95067573100001));
#170560=CARTESIAN_POINT('Ctrl Pts',(6.69664439799995,15.2,-7.95157853800001));
#170561=CARTESIAN_POINT('Ctrl Pts',(6.69725788299994,15.2,-7.95248948500002));
#170562=CARTESIAN_POINT('Ctrl Pts',(6.69787552599994,15.2,-7.95340856300002));
#170563=CARTESIAN_POINT('Ctrl Pts',(6.69849730099994,15.2,-7.95433576200002));
#170564=CARTESIAN_POINT('Ctrl Pts',(6.69912317899994,15.2,-7.95527107000002));
#170565=CARTESIAN_POINT('Ctrl Pts',(6.69975313299994,15.2,-7.95621447500002));
#170566=CARTESIAN_POINT('Ctrl Pts',(6.70038713599994,15.2,-7.95716596700001));
#170567=CARTESIAN_POINT('Ctrl Pts',(6.70102515999995,15.2,-7.95812553600002));
#170568=CARTESIAN_POINT('Ctrl Pts',(6.70166717899995,15.2,-7.95909317200002));
#170569=CARTESIAN_POINT('Ctrl Pts',(6.70231316599994,15.2,-7.96006886000002));
#170570=CARTESIAN_POINT('Ctrl Pts',(6.70296309299995,15.2,-7.96105259300001));
#170571=CARTESIAN_POINT('Ctrl Pts',(6.70361693399994,15.2,-7.96204436100002));
#170572=CARTESIAN_POINT('Ctrl Pts',(6.70427466299994,15.2,-7.96304415000002));
#170573=CARTESIAN_POINT('Ctrl Pts',(6.70493625199994,15.2,-7.96405195200002));
#170574=CARTESIAN_POINT('Ctrl Pts',(6.70560167699994,15.2,-7.96506775500001));
#170575=CARTESIAN_POINT('Ctrl Pts',(6.70627090999995,15.2,-7.96609155000001));
#170576=CARTESIAN_POINT('Ctrl Pts',(6.70694392699994,15.2,-7.96712332400002));
#170577=CARTESIAN_POINT('Ctrl Pts',(6.70762069999994,15.2,-7.96816306900002));
#170578=CARTESIAN_POINT('Ctrl Pts',(6.70830120299994,15.2,-7.96921077400001));
#170579=CARTESIAN_POINT('Ctrl Pts',(6.70898541199994,15.2,-7.97026642700001));
#170580=CARTESIAN_POINT('Ctrl Pts',(6.70967330099994,15.2,-7.97133002000002));
#170581=CARTESIAN_POINT('Ctrl Pts',(6.71036484499994,15.2,-7.97240154000002));
#170582=CARTESIAN_POINT('Ctrl Pts',(6.71106001699994,15.2,-7.97348098000001));
#170583=CARTESIAN_POINT('Ctrl Pts',(6.71175879199994,15.2,-7.97456832700002));
#170584=CARTESIAN_POINT('Ctrl Pts',(6.71246114699994,15.2,-7.97566357200001));
#170585=CARTESIAN_POINT('Ctrl Pts',(6.71316705499994,15.2,-7.97676670400002));
#170586=CARTESIAN_POINT('Ctrl Pts',(6.71387649099994,15.2,-7.97787771300002));
#170587=CARTESIAN_POINT('Ctrl Pts',(6.71458943199994,15.2,-7.97899659000001));
#170588=CARTESIAN_POINT('Ctrl Pts',(6.71530585299994,15.2,-7.98012332400001));
#170589=CARTESIAN_POINT('Ctrl Pts',(6.71602572899994,15.2,-7.98125790400002));
#170590=CARTESIAN_POINT('Ctrl Pts',(6.71674903499994,15.2,-7.98240032100002));
#170591=CARTESIAN_POINT('Ctrl Pts',(6.71747574699994,15.2,-7.98355056600002));
#170592=CARTESIAN_POINT('Ctrl Pts',(6.71820584199994,15.2,-7.98470862800002));
#170593=CARTESIAN_POINT('Ctrl Pts',(6.71893929399995,15.2,-7.98587449600002));
#170594=CARTESIAN_POINT('Ctrl Pts',(6.71967607999994,15.2,-7.98704816100001));
#170595=CARTESIAN_POINT('Ctrl Pts',(6.72041617599994,15.2,-7.98822961300001));
#170596=CARTESIAN_POINT('Ctrl Pts',(6.72115955899995,15.2,-7.98941884400002));
#170597=CARTESIAN_POINT('Ctrl Pts',(6.72190620499994,15.2,-7.99061584100001));
#170598=CARTESIAN_POINT('Ctrl Pts',(6.72265608899994,15.2,-7.99182059500002));
#170599=CARTESIAN_POINT('Ctrl Pts',(6.72340918899994,15.2,-7.99303309800001));
#170600=CARTESIAN_POINT('Ctrl Pts',(6.72416548199994,15.2,-7.99425333800002));
#170601=CARTESIAN_POINT('Ctrl Pts',(6.72492494399994,15.2,-7.99548130700002));
#170602=CARTESIAN_POINT('Ctrl Pts',(6.72568755199995,15.2,-7.99671699400001));
#170603=CARTESIAN_POINT('Ctrl Pts',(6.72645328299994,15.2,-7.99796039100002));
#170604=CARTESIAN_POINT('Ctrl Pts',(6.72722211399994,15.2,-7.99921148700002));
#170605=CARTESIAN_POINT('Ctrl Pts',(6.72799402199994,15.2,-8.00047027200002));
#170606=CARTESIAN_POINT('Ctrl Pts',(6.72876898499994,15.2,-8.00173673800002));
#170607=CARTESIAN_POINT('Ctrl Pts',(6.72954697899995,15.2,-8.00301087500002));
#170608=CARTESIAN_POINT('Ctrl Pts',(6.73032798299994,15.2,-8.00429267200002));
#170609=CARTESIAN_POINT('Ctrl Pts',(6.73111197299994,15.2,-8.00558212100002));
#170610=CARTESIAN_POINT('Ctrl Pts',(6.73189892699994,15.2,-8.00687921200002));
#170611=CARTESIAN_POINT('Ctrl Pts',(6.73268882399994,15.2,-8.00818393500002));
#170612=CARTESIAN_POINT('Ctrl Pts',(6.73348164099994,15.2,-8.00949628200001));
#170613=CARTESIAN_POINT('Ctrl Pts',(6.73427735599994,15.2,-8.01081624200001));
#170614=CARTESIAN_POINT('Ctrl Pts',(6.73507594699994,15.2,-8.01214380700002));
#170615=CARTESIAN_POINT('Ctrl Pts',(6.73587739199994,15.2,-8.01347896600002));
#170616=CARTESIAN_POINT('Ctrl Pts',(6.73668166999994,15.2,-8.01482171200002));
#170617=CARTESIAN_POINT('Ctrl Pts',(6.73748875699994,15.2,-8.01617203400001));
#170618=CARTESIAN_POINT('Ctrl Pts',(6.73829863399994,15.2,-8.01752992300001));
#170619=CARTESIAN_POINT('Ctrl Pts',(6.73911127899994,15.2,-8.01889537000001));
#170620=CARTESIAN_POINT('Ctrl Pts',(6.73992666899994,15.2,-8.02026836500002));
#170621=CARTESIAN_POINT('Ctrl Pts',(6.74074478399994,15.2,-8.02164890000002));
#170622=CARTESIAN_POINT('Ctrl Pts',(6.74156560399994,15.2,-8.02303696500001));
#170623=CARTESIAN_POINT('Ctrl Pts',(6.74238910499994,15.2,-8.02443255100002));
#170624=CARTESIAN_POINT('Ctrl Pts',(6.74321526699995,15.2,-8.02583564900001));
#170625=CARTESIAN_POINT('Ctrl Pts',(6.74404406899995,15.2,-8.02724625000002));
#170626=CARTESIAN_POINT('Ctrl Pts',(6.74487549099994,15.2,-8.02866434600002));
#170627=CARTESIAN_POINT('Ctrl Pts',(6.74570951199994,15.2,-8.03008992500001));
#170628=CARTESIAN_POINT('Ctrl Pts',(6.74654610999994,15.2,-8.03152298000001));
#170629=CARTESIAN_POINT('Ctrl Pts',(6.74738526499994,15.2,-8.03296350100002));
#170630=CARTESIAN_POINT('Ctrl Pts',(6.74822695699994,15.2,-8.03441148000001));
#170631=CARTESIAN_POINT('Ctrl Pts',(6.74907116499995,15.2,-8.03586690800002));
#170632=CARTESIAN_POINT('Ctrl Pts',(6.74991786899994,15.2,-8.03732977600001));
#170633=CARTESIAN_POINT('Ctrl Pts',(6.75076704799995,15.2,-8.03880007500002));
#170634=CARTESIAN_POINT('Ctrl Pts',(6.75161868199995,15.2,-8.04027779500002));
#170635=CARTESIAN_POINT('Ctrl Pts',(6.75247275099994,15.2,-8.04176292900001));
#170636=CARTESIAN_POINT('Ctrl Pts',(6.75332923499994,15.2,-8.04325546600002));
#170637=CARTESIAN_POINT('Ctrl Pts',(6.75418811399994,15.2,-8.04475539900002));
#170638=CARTESIAN_POINT('Ctrl Pts',(6.75504936899994,15.2,-8.04626271800002));
#170639=CARTESIAN_POINT('Ctrl Pts',(6.75591297799994,15.2,-8.04777741600001));
#170640=CARTESIAN_POINT('Ctrl Pts',(6.75677892299994,15.2,-8.04929948100002));
#170641=CARTESIAN_POINT('Ctrl Pts',(6.75764718299994,15.2,-8.05082890700002));
#170642=CARTESIAN_POINT('Ctrl Pts',(6.75851773999994,15.2,-8.05236568400002));
#170643=CARTESIAN_POINT('Ctrl Pts',(6.75939057299995,15.2,-8.05390980500002));
#170644=CARTESIAN_POINT('Ctrl Pts',(6.76026566399995,15.2,-8.05546125900002));
#170645=CARTESIAN_POINT('Ctrl Pts',(6.76114299199994,15.2,-8.05702003800001));
#170646=CARTESIAN_POINT('Ctrl Pts',(6.76202253899994,15.2,-8.05858613400002));
#170647=CARTESIAN_POINT('Ctrl Pts',(6.76290428599994,15.2,-8.06015953800001));
#170648=CARTESIAN_POINT('Ctrl Pts',(6.76378821099994,15.2,-8.06174024100001));
#170649=CARTESIAN_POINT('Ctrl Pts',(6.76467429899994,15.2,-8.06332823600002));
#170650=CARTESIAN_POINT('Ctrl Pts',(6.76556252799994,15.2,-8.06492351100001));
#170651=CARTESIAN_POINT('Ctrl Pts',(6.76645288099994,15.2,-8.06652606100002));
#170652=CARTESIAN_POINT('Ctrl Pts',(6.76734533799995,15.2,-8.06813587700002));
#170653=CARTESIAN_POINT('Ctrl Pts',(6.76823988099994,15.2,-8.06975294900001));
#170654=CARTESIAN_POINT('Ctrl Pts',(6.76913648999995,15.2,-8.07137726900002));
#170655=CARTESIAN_POINT('Ctrl Pts',(6.77003514699994,15.2,-8.07300882800002));
#170656=CARTESIAN_POINT('Ctrl Pts',(6.77093583499994,15.2,-8.07464761900002));
#170657=CARTESIAN_POINT('Ctrl Pts',(6.77183853299994,15.2,-8.07629363200002));
#170658=CARTESIAN_POINT('Ctrl Pts',(6.77274322499994,15.2,-8.07794686000002));
#170659=CARTESIAN_POINT('Ctrl Pts',(6.77364988999994,15.2,-8.07960729300002));
#170660=CARTESIAN_POINT('Ctrl Pts',(6.77455851199994,15.2,-8.08127492400001));
#170661=CARTESIAN_POINT('Ctrl Pts',(6.77546907099994,15.2,-8.08294974400001));
#170662=CARTESIAN_POINT('Ctrl Pts',(6.77638154999994,15.2,-8.08463174500002));
#170663=CARTESIAN_POINT('Ctrl Pts',(6.77729593099994,15.2,-8.08632091800002));
#170664=CARTESIAN_POINT('Ctrl Pts',(6.77821219499994,15.2,-8.08801725500001));
#170665=CARTESIAN_POINT('Ctrl Pts',(6.77913032499994,15.2,-8.08972074800002));
#170666=CARTESIAN_POINT('Ctrl Pts',(6.78005030299994,15.2,-8.09143138900002));
#170667=CARTESIAN_POINT('Ctrl Pts',(6.78097211099994,15.2,-8.09314916800002));
#170668=CARTESIAN_POINT('Ctrl Pts',(6.78189572999995,15.2,-8.09487408000002));
#170669=CARTESIAN_POINT('Ctrl Pts',(6.78282114499994,15.2,-8.09660611400002));
#170670=CARTESIAN_POINT('Ctrl Pts',(6.78374833699994,15.2,-8.09834526200002));
#170671=CARTESIAN_POINT('Ctrl Pts',(6.78467728799995,15.2,-8.10009151600001));
#170672=CARTESIAN_POINT('Ctrl Pts',(6.78560798099994,15.2,-8.10184486900001));
#170673=CARTESIAN_POINT('Ctrl Pts',(6.78654039799994,15.2,-8.10360531100002));
#170674=CARTESIAN_POINT('Ctrl Pts',(6.78747452299994,15.2,-8.10537283700001));
#170675=CARTESIAN_POINT('Ctrl Pts',(6.78841033799994,15.2,-8.10714743400002));
#170676=CARTESIAN_POINT('Ctrl Pts',(6.78934782399994,15.2,-8.10892909900002));
#170677=CARTESIAN_POINT('Ctrl Pts',(6.79028696699994,15.2,-8.11071782000001));
#170678=CARTESIAN_POINT('Ctrl Pts',(6.79122774799994,15.2,-8.11251359100002));
#170679=CARTESIAN_POINT('Ctrl Pts',(6.79217014999994,15.2,-8.11431640400002));
#170680=CARTESIAN_POINT('Ctrl Pts',(6.79311415699994,15.2,-8.11612625000001));
#170681=CARTESIAN_POINT('Ctrl Pts',(6.79405974999994,15.2,-8.11794312000002));
#170682=CARTESIAN_POINT('Ctrl Pts',(6.79500691399994,15.2,-8.11976700800002));
#170683=CARTESIAN_POINT('Ctrl Pts',(6.79595563299995,15.2,-8.12159790600001));
#170684=CARTESIAN_POINT('Ctrl Pts',(6.79690588799994,15.2,-8.12343580400002));
#170685=CARTESIAN_POINT('Ctrl Pts',(6.79785766299994,15.2,-8.12528069600001));
#170686=CARTESIAN_POINT('Ctrl Pts',(6.79881094199994,15.2,-8.12713257400001));
#170687=CARTESIAN_POINT('Ctrl Pts',(6.79976570799994,15.2,-8.12899142800001));
#170688=CARTESIAN_POINT('Ctrl Pts',(6.80072194599994,15.2,-8.13085725200001));
#170689=CARTESIAN_POINT('Ctrl Pts',(6.80167963599994,15.2,-8.13273003800001));
#170690=CARTESIAN_POINT('Ctrl Pts',(6.80263876599994,15.2,-8.13460977800002));
#170691=CARTESIAN_POINT('Ctrl Pts',(6.80359931599994,15.2,-8.13649646300002));
#170692=CARTESIAN_POINT('Ctrl Pts',(6.80456127099994,15.2,-8.13839008500001));
#170693=CARTESIAN_POINT('Ctrl Pts',(6.80552461599994,15.2,-8.14029063900002));
#170694=CARTESIAN_POINT('Ctrl Pts',(6.80648933299994,15.2,-8.14219811500001));
#170695=CARTESIAN_POINT('Ctrl Pts',(6.80745540699994,15.2,-8.14411250400001));
#170696=CARTESIAN_POINT('Ctrl Pts',(6.80842282199994,15.2,-8.14603380000002));
#170697=CARTESIAN_POINT('Ctrl Pts',(6.80939156199994,15.2,-8.14796199600002));
#170698=CARTESIAN_POINT('Ctrl Pts',(6.81036160899994,15.2,-8.14989708200001));
#170699=CARTESIAN_POINT('Ctrl Pts',(6.81133295099994,15.2,-8.15183905000002));
#170700=CARTESIAN_POINT('Ctrl Pts',(6.81230556799994,15.2,-8.15378789600001));
#170701=CARTESIAN_POINT('Ctrl Pts',(6.81327944699994,15.2,-8.15574360800002));
#170702=CARTESIAN_POINT('Ctrl Pts',(6.81425457199994,15.2,-8.15770618000002));
#170703=CARTESIAN_POINT('Ctrl Pts',(6.81523092699994,15.2,-8.15967560500001));
#170704=CARTESIAN_POINT('Ctrl Pts',(6.81620849499994,15.2,-8.16165187500001));
#170705=CARTESIAN_POINT('Ctrl Pts',(6.81718726299994,15.2,-8.16363498000002));
#170706=CARTESIAN_POINT('Ctrl Pts',(6.81816721399994,15.2,-8.16562491600001));
#170707=CARTESIAN_POINT('Ctrl Pts',(6.81914833299994,15.2,-8.16762167300002));
#170708=CARTESIAN_POINT('Ctrl Pts',(6.82013060499994,15.2,-8.16962524400001));
#170709=CARTESIAN_POINT('Ctrl Pts',(6.82111401199994,15.2,-8.17163562200001));
#170710=CARTESIAN_POINT('Ctrl Pts',(6.82209854199994,15.2,-8.17365279700002));
#170711=CARTESIAN_POINT('Ctrl Pts',(6.82308417899994,15.2,-8.17567676500002));
#170712=CARTESIAN_POINT('Ctrl Pts',(6.82407090599995,15.2,-8.17770751500002));
#170713=CARTESIAN_POINT('Ctrl Pts',(6.82505870999995,15.2,-8.17974504100001));
#170714=CARTESIAN_POINT('Ctrl Pts',(6.82604757499995,15.2,-8.18178933600001));
#170715=CARTESIAN_POINT('Ctrl Pts',(6.82703748599994,15.2,-8.18384039100001));
#170716=CARTESIAN_POINT('Ctrl Pts',(6.82802842799994,15.2,-8.18589820000001));
#170717=CARTESIAN_POINT('Ctrl Pts',(6.82902038699994,15.2,-8.18796275400001));
#170718=CARTESIAN_POINT('Ctrl Pts',(6.83001334499994,15.2,-8.19003404700002));
#170719=CARTESIAN_POINT('Ctrl Pts',(6.83100729199994,15.2,-8.19211207100001));
#170720=CARTESIAN_POINT('Ctrl Pts',(6.83200220999994,15.2,-8.19419681600002));
#170721=CARTESIAN_POINT('Ctrl Pts',(6.83299808299994,15.2,-8.19628827900001));
#170722=CARTESIAN_POINT('Ctrl Pts',(6.83399489999994,15.2,-8.19838644900001));
#170723=CARTESIAN_POINT('Ctrl Pts',(6.83499264499994,15.2,-8.20049132000002));
#170724=CARTESIAN_POINT('Ctrl Pts',(6.83599130199994,15.2,-8.20260288400002));
#170725=CARTESIAN_POINT('Ctrl Pts',(6.83699085699994,15.2,-8.20472113600001));
#170726=CARTESIAN_POINT('Ctrl Pts',(6.83799129699994,15.2,-8.20684606400001));
#170727=CARTESIAN_POINT('Ctrl Pts',(6.83899260499994,15.2,-8.20897766300002));
#170728=CARTESIAN_POINT('Ctrl Pts',(6.83999476999994,15.2,-8.21111592700002));
#170729=CARTESIAN_POINT('Ctrl Pts',(6.84099777399994,15.2,-8.21326084700001));
#170730=CARTESIAN_POINT('Ctrl Pts',(6.84200160499994,15.2,-8.21541241600002));
#170731=CARTESIAN_POINT('Ctrl Pts',(6.84300624899994,15.2,-8.21757062500001));
#170732=CARTESIAN_POINT('Ctrl Pts',(6.84401168999995,15.2,-8.21973547000002));
#170733=CARTESIAN_POINT('Ctrl Pts',(6.84501791499994,15.2,-8.22190694200001));
#170734=CARTESIAN_POINT('Ctrl Pts',(6.84602490999994,15.2,-8.22408503200002));
#170735=CARTESIAN_POINT('Ctrl Pts',(6.84703265999994,15.2,-8.22626973500002));
#170736=CARTESIAN_POINT('Ctrl Pts',(6.84804115199994,15.2,-8.22846104400002));
#170737=CARTESIAN_POINT('Ctrl Pts',(6.84905037099995,15.2,-8.23065895000001));
#170738=CARTESIAN_POINT('Ctrl Pts',(6.85006030399994,15.2,-8.23286344400002));
#170739=CARTESIAN_POINT('Ctrl Pts',(6.85107093599994,15.2,-8.23507452400002));
#170740=CARTESIAN_POINT('Ctrl Pts',(6.85208225499994,15.2,-8.23729217900001));
#170741=CARTESIAN_POINT('Ctrl Pts',(6.85309424499994,15.2,-8.23951640200002));
#170742=CARTESIAN_POINT('Ctrl Pts',(6.85410689299994,15.2,-8.24174718600002));
#170743=CARTESIAN_POINT('Ctrl Pts',(6.85512018599994,15.2,-8.24398452500001));
#170744=CARTESIAN_POINT('Ctrl Pts',(6.85613410999995,15.2,-8.24622841000001));
#170745=CARTESIAN_POINT('Ctrl Pts',(6.85714865199994,15.2,-8.24847883600001));
#170746=CARTESIAN_POINT('Ctrl Pts',(6.85816379599994,15.2,-8.25073579300001));
#170747=CARTESIAN_POINT('Ctrl Pts',(6.85917953099994,15.2,-8.25299927600001));
#170748=CARTESIAN_POINT('Ctrl Pts',(6.86019584299994,15.2,-8.25526927700002));
#170749=CARTESIAN_POINT('Ctrl Pts',(6.86121271699994,15.2,-8.25754578900002));
#170750=CARTESIAN_POINT('Ctrl Pts',(6.86223014199994,15.2,-8.25982880500002));
#170751=CARTESIAN_POINT('Ctrl Pts',(6.86324810299995,15.2,-8.26211831700002));
#170752=CARTESIAN_POINT('Ctrl Pts',(6.86426658699994,15.2,-8.26441431900001));
#170753=CARTESIAN_POINT('Ctrl Pts',(6.86528557999995,15.2,-8.26671680300001));
#170754=CARTESIAN_POINT('Ctrl Pts',(6.86630506999995,15.2,-8.26902576200002));
#170755=CARTESIAN_POINT('Ctrl Pts',(6.86732504299994,15.2,-8.27134119000002));
#170756=CARTESIAN_POINT('Ctrl Pts',(6.86834548499994,15.2,-8.27366307800002));
#170757=CARTESIAN_POINT('Ctrl Pts',(6.86936638499994,15.2,-8.27599142100001));
#170758=CARTESIAN_POINT('Ctrl Pts',(6.87038772899994,15.2,-8.27832621000002));
#170759=CARTESIAN_POINT('Ctrl Pts',(6.87140950299994,15.2,-8.28066743900001));
#170760=CARTESIAN_POINT('Ctrl Pts',(6.87243169499994,15.2,-8.28301510100001));
#170761=CARTESIAN_POINT('Ctrl Pts',(6.87345429199994,15.2,-8.28536918900001));
#170762=CARTESIAN_POINT('Ctrl Pts',(6.87447728099994,15.2,-8.28772969500001));
#170763=CARTESIAN_POINT('Ctrl Pts',(6.87550064899995,15.2,-8.29009661300002));
#170764=CARTESIAN_POINT('Ctrl Pts',(6.87652438199994,15.2,-8.29246993600002));
#170765=CARTESIAN_POINT('Ctrl Pts',(6.87754846999994,15.2,-8.29484965700001));
#170766=CARTESIAN_POINT('Ctrl Pts',(6.87857289699994,15.2,-8.29723576700001));
#170767=CARTESIAN_POINT('Ctrl Pts',(6.87959765299994,15.2,-8.29962826200001));
#170768=CARTESIAN_POINT('Ctrl Pts',(6.88062272399995,15.2,-8.30202713300002));
#170769=CARTESIAN_POINT('Ctrl Pts',(6.88164809599995,15.2,-8.30443237500001));
#170770=CARTESIAN_POINT('Ctrl Pts',(6.88267375899994,15.2,-8.30684397800002));
#170771=CARTESIAN_POINT('Ctrl Pts',(6.88369969899994,15.2,-8.30926193800002));
#170772=CARTESIAN_POINT('Ctrl Pts',(6.88472590399994,15.2,-8.31168624500001));
#170773=CARTESIAN_POINT('Ctrl Pts',(6.88575235999994,15.2,-8.31411689700002));
#170774=CARTESIAN_POINT('Ctrl Pts',(6.88677905699994,15.2,-8.31655388200002));
#170775=CARTESIAN_POINT('Ctrl Pts',(6.88780597999994,15.2,-8.31899719600001));
#170776=CARTESIAN_POINT('Ctrl Pts',(6.88883311899994,15.2,-8.32144682900001));
#170777=CARTESIAN_POINT('Ctrl Pts',(6.88986046099994,15.2,-8.32390277900002));
#170778=CARTESIAN_POINT('Ctrl Pts',(6.89088799199994,15.2,-8.32636503500002));
#170779=CARTESIAN_POINT('Ctrl Pts',(6.89191570099994,15.2,-8.32883359100002));
#170780=CARTESIAN_POINT('Ctrl Pts',(6.89294357699994,15.2,-8.33130844200002));
#170781=CARTESIAN_POINT('Ctrl Pts',(6.89397160499994,15.2,-8.33378957900001));
#170782=CARTESIAN_POINT('Ctrl Pts',(6.89499977499994,15.2,-8.33627699600001));
#170783=CARTESIAN_POINT('Ctrl Pts',(6.89602807299995,15.2,-8.33877068600002));
#170784=CARTESIAN_POINT('Ctrl Pts',(6.89705648999994,15.2,-8.34127064300001));
#170785=CARTESIAN_POINT('Ctrl Pts',(6.89808501099994,15.2,-8.34377685900002));
#170786=CARTESIAN_POINT('Ctrl Pts',(6.89911362499994,15.2,-8.34628932700002));
#170787=CARTESIAN_POINT('Ctrl Pts',(6.90014232099994,15.2,-8.34880804200001));
#170788=CARTESIAN_POINT('Ctrl Pts',(6.90117108399994,15.2,-8.35133299500002));
#170789=CARTESIAN_POINT('Ctrl Pts',(6.90219990499994,15.2,-8.35386418100001));
#170790=CARTESIAN_POINT('Ctrl Pts',(6.90322877199994,15.2,-8.35640159100001));
#170791=CARTESIAN_POINT('Ctrl Pts',(6.90425767199994,15.2,-8.35894522000002));
#170792=CARTESIAN_POINT('Ctrl Pts',(6.90528659299994,15.2,-8.36149506200002));
#170793=CARTESIAN_POINT('Ctrl Pts',(6.90631552399994,15.2,-8.36405110800002));
#170794=CARTESIAN_POINT('Ctrl Pts',(6.90734445199994,15.2,-8.36661335300001));
#170795=CARTESIAN_POINT('Ctrl Pts',(6.90837336899994,15.2,-8.36918179000002));
#170796=CARTESIAN_POINT('Ctrl Pts',(6.90940225899995,15.2,-8.37175641100002));
#170797=CARTESIAN_POINT('Ctrl Pts',(6.91043111099994,15.2,-8.37433721000002));
#170798=CARTESIAN_POINT('Ctrl Pts',(6.91145991499994,15.2,-8.37692418200002));
#170799=CARTESIAN_POINT('Ctrl Pts',(6.91248865999994,15.2,-8.37951731700001));
#170800=CARTESIAN_POINT('Ctrl Pts',(6.91351733199994,15.2,-8.38211661100001));
#170801=CARTESIAN_POINT('Ctrl Pts',(6.91454591999995,15.2,-8.38472205600001));
#170802=CARTESIAN_POINT('Ctrl Pts',(6.91557441499994,15.2,-8.38733364600002));
#170803=CARTESIAN_POINT('Ctrl Pts',(6.91660280299994,15.2,-8.38995137300002));
#170804=CARTESIAN_POINT('Ctrl Pts',(6.91763107299994,15.2,-8.39257523200001));
#170805=CARTESIAN_POINT('Ctrl Pts',(6.91865921499994,15.2,-8.39520521500001));
#170806=CARTESIAN_POINT('Ctrl Pts',(6.91968721499994,15.2,-8.39784131600002));
#170807=CARTESIAN_POINT('Ctrl Pts',(6.92071506399994,15.2,-8.40048352900002));
#170808=CARTESIAN_POINT('Ctrl Pts',(6.92174274999994,15.2,-8.40313184700002));
#170809=CARTESIAN_POINT('Ctrl Pts',(6.92277026199994,15.2,-8.40578626200001));
#170810=CARTESIAN_POINT('Ctrl Pts',(6.92379758999994,15.2,-8.40844676800002));
#170811=CARTESIAN_POINT('Ctrl Pts',(6.92482471899995,15.2,-8.41111336100001));
#170812=CARTESIAN_POINT('Ctrl Pts',(6.92585164099994,15.2,-8.41378603000001));
#170813=CARTESIAN_POINT('Ctrl Pts',(6.92687834499995,15.2,-8.41646477200002));
#170814=CARTESIAN_POINT('Ctrl Pts',(6.92790481799994,15.2,-8.41914957800002));
#170815=CARTESIAN_POINT('Ctrl Pts',(6.92893105099994,15.2,-8.42184044300001));
#170816=CARTESIAN_POINT('Ctrl Pts',(6.92995702999994,15.2,-8.42453735900002));
#170817=CARTESIAN_POINT('Ctrl Pts',(6.93098274699994,15.2,-8.42724032100002));
#170818=CARTESIAN_POINT('Ctrl Pts',(6.93200819099994,15.2,-8.42994932100002));
#170819=CARTESIAN_POINT('Ctrl Pts',(6.93303334799994,15.2,-8.43266435400002));
#170820=CARTESIAN_POINT('Ctrl Pts',(6.93405820999994,15.2,-8.43538541100001));
#170821=CARTESIAN_POINT('Ctrl Pts',(6.93508276499994,15.2,-8.43811248900002));
#170822=CARTESIAN_POINT('Ctrl Pts',(6.93610700299994,15.2,-8.44084557900001));
#170823=CARTESIAN_POINT('Ctrl Pts',(6.93713091199994,15.2,-8.44358467400001));
#170824=CARTESIAN_POINT('Ctrl Pts',(6.93815448099994,15.2,-8.44632976900002));
#170825=CARTESIAN_POINT('Ctrl Pts',(6.93917770099994,15.2,-8.44908085600002));
#170826=CARTESIAN_POINT('Ctrl Pts',(6.94020055999995,15.2,-8.45183793000002));
#170827=CARTESIAN_POINT('Ctrl Pts',(6.94122304799994,15.2,-8.45460098400002));
#170828=CARTESIAN_POINT('Ctrl Pts',(6.94224515399994,15.2,-8.45737001200002));
#170829=CARTESIAN_POINT('Ctrl Pts',(6.94326686599994,15.2,-8.46014500600001));
#170830=CARTESIAN_POINT('Ctrl Pts',(6.94428817599994,15.2,-8.46292596000002));
#170831=CARTESIAN_POINT('Ctrl Pts',(6.94530907199994,15.2,-8.46571286900001));
#170832=CARTESIAN_POINT('Ctrl Pts',(6.94632954299994,15.2,-8.46850572500001));
#170833=CARTESIAN_POINT('Ctrl Pts',(6.94734957799994,15.2,-8.47130452200001));
#170834=CARTESIAN_POINT('Ctrl Pts',(6.94836916999994,15.2,-8.47410925300002));
#170835=CARTESIAN_POINT('Ctrl Pts',(6.94938830399995,15.2,-8.47691991200002));
#170836=CARTESIAN_POINT('Ctrl Pts',(6.95040697199994,15.2,-8.47973649400002));
#170837=CARTESIAN_POINT('Ctrl Pts',(6.95142516299994,15.2,-8.48255899100002));
#170838=CARTESIAN_POINT('Ctrl Pts',(6.95244286799994,15.2,-8.48538739600002));
#170839=CARTESIAN_POINT('Ctrl Pts',(6.95346007499994,15.2,-8.48822170300001));
#170840=CARTESIAN_POINT('Ctrl Pts',(6.95447677299994,15.2,-8.49106190600001));
#170841=CARTESIAN_POINT('Ctrl Pts',(6.95549295399994,15.2,-8.49390799900002));
#170842=CARTESIAN_POINT('Ctrl Pts',(6.95650860599994,15.2,-8.49675997600002));
#170843=CARTESIAN_POINT('Ctrl Pts',(6.95752371999995,15.2,-8.49961782800002));
#170844=CARTESIAN_POINT('Ctrl Pts',(6.95853828499994,15.2,-8.50248155200001));
#170845=CARTESIAN_POINT('Ctrl Pts',(6.95955229099994,15.2,-8.50535113900002));
#170846=CARTESIAN_POINT('Ctrl Pts',(6.96056572699994,15.2,-8.50822658400002));
#170847=CARTESIAN_POINT('Ctrl Pts',(6.96157858499994,15.2,-8.51110787900001));
#170848=CARTESIAN_POINT('Ctrl Pts',(6.96259085299994,15.2,-8.51399502000002));
#170849=CARTESIAN_POINT('Ctrl Pts',(6.96360252099994,15.2,-8.51688800000002));
#170850=CARTESIAN_POINT('Ctrl Pts',(6.96461357999994,15.2,-8.51978681100002));
#170851=CARTESIAN_POINT('Ctrl Pts',(6.96562401999994,15.2,-8.52269144800001));
#170852=CARTESIAN_POINT('Ctrl Pts',(6.96663382999994,15.2,-8.52560190500002));
#170853=CARTESIAN_POINT('Ctrl Pts',(6.96764299999994,15.2,-8.52851817400002));
#170854=CARTESIAN_POINT('Ctrl Pts',(6.96865152099994,15.2,-8.53144025000002));
#170855=CARTESIAN_POINT('Ctrl Pts',(6.96965938299994,15.2,-8.53436812800001));
#170856=CARTESIAN_POINT('Ctrl Pts',(6.97066657399994,15.2,-8.53730179900002));
#170857=CARTESIAN_POINT('Ctrl Pts',(6.97167308699994,15.2,-8.54024125700001));
#170858=CARTESIAN_POINT('Ctrl Pts',(6.97267891199994,15.2,-8.54318649800001));
#170859=CARTESIAN_POINT('Ctrl Pts',(6.97368403699994,15.2,-8.54613751400001));
#170860=CARTESIAN_POINT('Ctrl Pts',(6.97468845399994,15.2,-8.54909429700001));
#170861=CARTESIAN_POINT('Ctrl Pts',(6.97569215299994,15.2,-8.55205684500002));
#170862=CARTESIAN_POINT('Ctrl Pts',(6.97669512399994,15.2,-8.55502514800002));
#170863=CARTESIAN_POINT('Ctrl Pts',(6.97769735699994,15.2,-8.55799920200001));
#170864=CARTESIAN_POINT('Ctrl Pts',(6.97869884199994,15.2,-8.56097899900002));
#170865=CARTESIAN_POINT('Ctrl Pts',(6.97969957099994,15.2,-8.56396453400002));
#170866=CARTESIAN_POINT('Ctrl Pts',(6.98069953199994,15.2,-8.56695580000002));
#170867=CARTESIAN_POINT('Ctrl Pts',(6.98169871799994,15.2,-8.56995279200002));
#170868=CARTESIAN_POINT('Ctrl Pts',(6.98269711799994,15.2,-8.57295550200002));
#170869=CARTESIAN_POINT('Ctrl Pts',(6.98369472199994,15.2,-8.57596392400002));
#170870=CARTESIAN_POINT('Ctrl Pts',(6.98469152199994,15.2,-8.57897805400002));
#170871=CARTESIAN_POINT('Ctrl Pts',(6.98568750699994,15.2,-8.58199788300002));
#170872=CARTESIAN_POINT('Ctrl Pts',(6.98668266799994,15.2,-8.58502340600002));
#170873=CARTESIAN_POINT('Ctrl Pts',(6.98767699599994,15.2,-8.58805461600002));
#170874=CARTESIAN_POINT('Ctrl Pts',(6.98867048099994,15.2,-8.59109150800002));
#170875=CARTESIAN_POINT('Ctrl Pts',(6.98966311399994,15.2,-8.59413407600002));
#170876=CARTESIAN_POINT('Ctrl Pts',(6.99065488599994,15.2,-8.59718231200001));
#170877=CARTESIAN_POINT('Ctrl Pts',(6.99164578499994,15.2,-8.60023621100002));
#170878=CARTESIAN_POINT('Ctrl Pts',(6.99263580599994,15.2,-8.60329576700002));
#170879=CARTESIAN_POINT('Ctrl Pts',(6.99362493699994,15.2,-8.60636097400001));
#170880=CARTESIAN_POINT('Ctrl Pts',(6.99461316799994,15.2,-8.60943182400002));
#170881=CARTESIAN_POINT('Ctrl Pts',(6.99560049199994,15.2,-8.61250831300002));
#170882=CARTESIAN_POINT('Ctrl Pts',(6.99658689799994,15.2,-8.61559043400002));
#170883=CARTESIAN_POINT('Ctrl Pts',(6.99757237899994,15.2,-8.61867818100002));
#170884=CARTESIAN_POINT('Ctrl Pts',(6.99855692199994,15.2,-8.62177154700002));
#170885=CARTESIAN_POINT('Ctrl Pts',(6.99954052099995,15.2,-8.62487052700001));
#170886=CARTESIAN_POINT('Ctrl Pts',(7.00052316699994,15.2,-8.62797511400002));
#170887=CARTESIAN_POINT('Ctrl Pts',(7.00150484899994,15.2,-8.63108530300002));
#170888=CARTESIAN_POINT('Ctrl Pts',(7.00248555899995,15.2,-8.63420108600002));
#170889=CARTESIAN_POINT('Ctrl Pts',(7.00346528799995,15.2,-8.63732245800002));
#170890=CARTESIAN_POINT('Ctrl Pts',(7.00444402699994,15.2,-8.64044941300002));
#170891=CARTESIAN_POINT('Ctrl Pts',(7.00542176599994,15.2,-8.64358194500002));
#170892=CARTESIAN_POINT('Ctrl Pts',(7.00639849599995,15.2,-8.64672004800001));
#170893=CARTESIAN_POINT('Ctrl Pts',(7.00737420899994,15.2,-8.64986371400001));
#170894=CARTESIAN_POINT('Ctrl Pts',(7.00834889699994,15.2,-8.65301294000002));
#170895=CARTESIAN_POINT('Ctrl Pts',(7.00932254799994,15.2,-8.65616771800001));
#170896=CARTESIAN_POINT('Ctrl Pts',(7.01029515599994,15.2,-8.65932804100002));
#170897=CARTESIAN_POINT('Ctrl Pts',(7.01126671099995,15.2,-8.66249390500002));
#170898=CARTESIAN_POINT('Ctrl Pts',(7.01223720399994,15.2,-8.66566530400002));
#170899=CARTESIAN_POINT('Ctrl Pts',(7.01320662599994,15.2,-8.66884222900002));
#170900=CARTESIAN_POINT('Ctrl Pts',(7.01417496999994,15.2,-8.67202467700002));
#170901=CARTESIAN_POINT('Ctrl Pts',(7.01514222399994,15.2,-8.67521264000001));
#170902=CARTESIAN_POINT('Ctrl Pts',(7.01610838099994,15.2,-8.67840611400002));
#170903=CARTESIAN_POINT('Ctrl Pts',(7.01707343299995,15.2,-8.68160509100001));
#170904=CARTESIAN_POINT('Ctrl Pts',(7.01803736899994,15.2,-8.68480956600001));
#170905=CARTESIAN_POINT('Ctrl Pts',(7.01900018299995,15.2,-8.68801953100002));
#170906=CARTESIAN_POINT('Ctrl Pts',(7.01996186499994,15.2,-8.69123498300001));
#170907=CARTESIAN_POINT('Ctrl Pts',(7.02092240599994,15.2,-8.69445591400002));
#170908=CARTESIAN_POINT('Ctrl Pts',(7.02188179799994,15.2,-8.69768231900002));
#170909=CARTESIAN_POINT('Ctrl Pts',(7.02284003299994,15.2,-8.70091419100002));
#170910=CARTESIAN_POINT('Ctrl Pts',(7.02379709999994,15.2,-8.70415152400002));
#170911=CARTESIAN_POINT('Ctrl Pts',(7.02475299199994,15.2,-8.70739431300001));
#170912=CARTESIAN_POINT('Ctrl Pts',(7.02570770099994,15.2,-8.71064255100002));
#170913=CARTESIAN_POINT('Ctrl Pts',(7.02666121799994,15.2,-8.71389623300002));
#170914=CARTESIAN_POINT('Ctrl Pts',(7.02761353399994,15.2,-8.71715535200002));
#170915=CARTESIAN_POINT('Ctrl Pts',(7.02856464099994,15.2,-8.72041990300002));
#170916=CARTESIAN_POINT('Ctrl Pts',(7.02951453099994,15.2,-8.72368987800002));
#170917=CARTESIAN_POINT('Ctrl Pts',(7.03046319299995,15.2,-8.72696527400001));
#170918=CARTESIAN_POINT('Ctrl Pts',(7.03141062299995,15.2,-8.73024608200001));
#170919=CARTESIAN_POINT('Ctrl Pts',(7.03235680899994,15.2,-8.73353229700001));
#170920=CARTESIAN_POINT('Ctrl Pts',(7.03330174299994,15.2,-8.73682391500001));
#170921=CARTESIAN_POINT('Ctrl Pts',(7.03424541799994,15.2,-8.74012092800001));
#170922=CARTESIAN_POINT('Ctrl Pts',(7.03518782499994,15.2,-8.74342333000002));
#170923=CARTESIAN_POINT('Ctrl Pts',(7.03612895599995,15.2,-8.74673111600002));
#170924=CARTESIAN_POINT('Ctrl Pts',(7.03706880199994,15.2,-8.75004428000001));
#170925=CARTESIAN_POINT('Ctrl Pts',(7.03800735599994,15.2,-8.75336281500001));
#170926=CARTESIAN_POINT('Ctrl Pts',(7.03894460699994,15.2,-8.75668671600002));
#170927=CARTESIAN_POINT('Ctrl Pts',(7.03988054999994,15.2,-8.76001597500002));
#170928=CARTESIAN_POINT('Ctrl Pts',(7.04081517499994,15.2,-8.76335058900001));
#170929=CARTESIAN_POINT('Ctrl Pts',(7.04174847399995,15.2,-8.76669055200002));
#170930=CARTESIAN_POINT('Ctrl Pts',(7.04268043899994,15.2,-8.77003585600002));
#170931=CARTESIAN_POINT('Ctrl Pts',(7.04361106199995,15.2,-8.77338649600001));
#170932=CARTESIAN_POINT('Ctrl Pts',(7.04454033599994,15.2,-8.77674246600002));
#170933=CARTESIAN_POINT('Ctrl Pts',(7.04546824999994,15.2,-8.78010376100002));
#170934=CARTESIAN_POINT('Ctrl Pts',(7.04639479699994,15.2,-8.78347037400001));
#170935=CARTESIAN_POINT('Ctrl Pts',(7.04731997099994,15.2,-8.78684229900001));
#170936=CARTESIAN_POINT('Ctrl Pts',(7.04824376099995,15.2,-8.79021953000001));
#170937=CARTESIAN_POINT('Ctrl Pts',(7.04916616099994,15.2,-8.79360206200002));
#170938=CARTESIAN_POINT('Ctrl Pts',(7.05008716199995,15.2,-8.79698988800002));
#170939=CARTESIAN_POINT('Ctrl Pts',(7.05100675599994,15.2,-8.80038300300001));
#170940=CARTESIAN_POINT('Ctrl Pts',(7.05192493599994,15.2,-8.80378140200002));
#170941=CARTESIAN_POINT('Ctrl Pts',(7.05284169299994,15.2,-8.80718507700001));
#170942=CARTESIAN_POINT('Ctrl Pts',(7.05375701899994,15.2,-8.81059402400002));
#170943=CARTESIAN_POINT('Ctrl Pts',(7.05467090599995,15.2,-8.81400823500002));
#170944=CARTESIAN_POINT('Ctrl Pts',(7.05558334699995,15.2,-8.81742770600002));
#170945=CARTESIAN_POINT('Ctrl Pts',(7.05649433399994,15.2,-8.82085243000001));
#170946=CARTESIAN_POINT('Ctrl Pts',(7.05740385899994,15.2,-8.82428240200002));
#170947=CARTESIAN_POINT('Ctrl Pts',(7.05831191399994,15.2,-8.82771761700001));
#170948=CARTESIAN_POINT('Ctrl Pts',(7.05921848999994,15.2,-8.83115806600001));
#170949=CARTESIAN_POINT('Ctrl Pts',(7.06012358099994,15.2,-8.83460374700002));
#170950=CARTESIAN_POINT('Ctrl Pts',(7.06102717799994,15.2,-8.83805465100002));
#170951=CARTESIAN_POINT('Ctrl Pts',(7.06192927499995,15.2,-8.84151077400002));
#170952=CARTESIAN_POINT('Ctrl Pts',(7.06282986099994,15.2,-8.84497210900001));
#170953=CARTESIAN_POINT('Ctrl Pts',(7.06372893199994,15.2,-8.84843865100001));
#170954=CARTESIAN_POINT('Ctrl Pts',(7.06462647799994,15.2,-8.85191039400001));
#170955=CARTESIAN_POINT('Ctrl Pts',(7.06552248999994,15.2,-8.85538733200002));
#170956=CARTESIAN_POINT('Ctrl Pts',(7.06641696399994,15.2,-8.85886945800002));
#170957=CARTESIAN_POINT('Ctrl Pts',(7.06730988999994,15.2,-8.86235676900002));
#170958=CARTESIAN_POINT('Ctrl Pts',(7.06820126099994,15.2,-8.86584925900002));
#170959=CARTESIAN_POINT('Ctrl Pts',(7.06909106899994,15.2,-8.86934691900001));
#170960=CARTESIAN_POINT('Ctrl Pts',(7.06997930699995,15.2,-8.87284974500002));
#170961=CARTESIAN_POINT('Ctrl Pts',(7.07086596699994,15.2,-8.87635773100002));
#170962=CARTESIAN_POINT('Ctrl Pts',(7.07175103999995,15.2,-8.87987087200001));
#170963=CARTESIAN_POINT('Ctrl Pts',(7.07263452099994,15.2,-8.88338916200002));
#170964=CARTESIAN_POINT('Ctrl Pts',(7.07351640099994,15.2,-8.88691259500002));
#170965=CARTESIAN_POINT('Ctrl Pts',(7.07439667399994,15.2,-8.89044116400001));
#170966=CARTESIAN_POINT('Ctrl Pts',(7.07527532899995,15.2,-8.89397486500001));
#170967=CARTESIAN_POINT('Ctrl Pts',(7.07615236299994,15.2,-8.89751369100001));
#170968=CARTESIAN_POINT('Ctrl Pts',(7.07702776499994,15.2,-8.90105763700002));
#170969=CARTESIAN_POINT('Ctrl Pts',(7.07790152999995,15.2,-8.90460669800002));
#170970=CARTESIAN_POINT('Ctrl Pts',(7.07877364899994,15.2,-8.90816086600001));
#170971=CARTESIAN_POINT('Ctrl Pts',(7.07964411499994,15.2,-8.91172013700002));
#170972=CARTESIAN_POINT('Ctrl Pts',(7.08051291999994,15.2,-8.91528450500001));
#170973=CARTESIAN_POINT('Ctrl Pts',(7.08138005899994,15.2,-8.91885396400001));
#170974=CARTESIAN_POINT('Ctrl Pts',(7.08224552099994,15.2,-8.92242850800002));
#170975=CARTESIAN_POINT('Ctrl Pts',(7.08310930199994,15.2,-8.92600813100002));
#170976=CARTESIAN_POINT('Ctrl Pts',(7.08397139199994,15.2,-8.92959282900001));
#170977=CARTESIAN_POINT('Ctrl Pts',(7.08483178599994,15.2,-8.93318259300001));
#170978=CARTESIAN_POINT('Ctrl Pts',(7.08569047499994,15.2,-8.93677742100002));
#170979=CARTESIAN_POINT('Ctrl Pts',(7.08654745099994,15.2,-8.94037730400001));
#170980=CARTESIAN_POINT('Ctrl Pts',(7.08740270999995,15.2,-8.94398223900001));
#170981=CARTESIAN_POINT('Ctrl Pts',(7.08825624299994,15.2,-8.94759221800001));
#170982=CARTESIAN_POINT('Ctrl Pts',(7.08910804199994,15.2,-8.95120723800002));
#170983=CARTESIAN_POINT('Ctrl Pts',(7.08995810299994,15.2,-8.95482729200002));
#170984=CARTESIAN_POINT('Ctrl Pts',(7.09080641499994,15.2,-8.95845237400002));
#170985=CARTESIAN_POINT('Ctrl Pts',(7.09165297099994,15.2,-8.96208247700002));
#170986=CARTESIAN_POINT('Ctrl Pts',(7.09249776599994,15.2,-8.96571759800001));
#170987=CARTESIAN_POINT('Ctrl Pts',(7.09334079199994,15.2,-8.96935772800001));
#170988=CARTESIAN_POINT('Ctrl Pts',(7.09418203899994,15.2,-8.97300286300002));
#170989=CARTESIAN_POINT('Ctrl Pts',(7.09502150299994,15.2,-8.97665299700002));
#170990=CARTESIAN_POINT('Ctrl Pts',(7.09585917499994,15.2,-8.98030812400001));
#170991=CARTESIAN_POINT('Ctrl Pts',(7.09669504999995,15.2,-8.98396824000002));
#170992=CARTESIAN_POINT('Ctrl Pts',(7.09752912199995,15.2,-8.98763333900002));
#170993=CARTESIAN_POINT('Ctrl Pts',(7.09836138399995,15.2,-8.99130341500002));
#170994=CARTESIAN_POINT('Ctrl Pts',(7.09919182999994,15.2,-8.99497846600001));
#170995=CARTESIAN_POINT('Ctrl Pts',(7.10002044999994,15.2,-8.99865848200001));
#170996=CARTESIAN_POINT('Ctrl Pts',(7.10084723999994,15.2,-9.00234345900002));
#170997=CARTESIAN_POINT('Ctrl Pts',(7.10167218799994,15.2,-9.00603338900002));
#170998=CARTESIAN_POINT('Ctrl Pts',(7.10249528699994,15.2,-9.00972826500002));
#170999=CARTESIAN_POINT('Ctrl Pts',(7.10331652799994,15.2,-9.01342808000001));
#171000=CARTESIAN_POINT('Ctrl Pts',(7.10413590299994,15.2,-9.01713282900002));
#171001=CARTESIAN_POINT('Ctrl Pts',(7.10495340799994,15.2,-9.02084250500002));
#171002=CARTESIAN_POINT('Ctrl Pts',(7.10576903499994,15.2,-9.02455710700002));
#171003=CARTESIAN_POINT('Ctrl Pts',(7.10658278299994,15.2,-9.02827662900001));
#171004=CARTESIAN_POINT('Ctrl Pts',(7.10739465099994,15.2,-9.03200107200002));
#171005=CARTESIAN_POINT('Ctrl Pts',(7.10804263899995,15.2,-9.03498456100002));
#171006=CARTESIAN_POINT('Ctrl Pts',(7.10852778299994,15.2,-9.03722439200001));
#171007=CARTESIAN_POINT('Ctrl Pts',(7.10885083699995,15.2,-9.03871859500001));
#171008=CARTESIAN_POINT('Ctrl Pts',(7.10901226899994,15.2,-9.03946594400002));
#171009=CARTESIAN_POINT('Origin',(-5.66257110645729E-14,15.2,-1.77635683940025E-14));
#171010=CARTESIAN_POINT('',(7.012168986001,15.2,-7.6465751233345));
#171011=CARTESIAN_POINT('',(7.012168986001,12.2,-7.6465751233345));
#171012=CARTESIAN_POINT('',(7.01216898599994,15.2,-7.64657512300002));
#171013=CARTESIAN_POINT('Origin',(-5.66257110645729E-14,12.2,-1.77635683940025E-14));
#171014=CARTESIAN_POINT('Origin',(-5.66257110645729E-14,15.2,-1.77635683940025E-14));
#171015=CARTESIAN_POINT('Origin',(-5.66257110645729E-14,15.2,-1.77635683940025E-14));
#171016=CARTESIAN_POINT('',(8.05377977099995,15.2,-8.20893607000002));
#171017=CARTESIAN_POINT('',(8.32310290799994,15.2,-7.93573928300002));
#171018=CARTESIAN_POINT('Origin',(-5.66257110645729E-14,15.2,-1.77635683940025E-14));
#171019=CARTESIAN_POINT('',(8.32310290799994,12.2,-7.93573928300002));
#171020=CARTESIAN_POINT('',(8.32310290799994,15.2,-7.93573928300002));
#171021=CARTESIAN_POINT('',(8.05377977099995,12.2,-8.20893607000002));
#171022=CARTESIAN_POINT('Origin',(-5.66257110645729E-14,12.2,-1.77635683940025E-14));
#171023=CARTESIAN_POINT('',(8.05377977099995,15.2,-8.20893607000002));
#171024=CARTESIAN_POINT('Ctrl Pts',(8.32310290799994,15.2,-7.93573928300002));
#171025=CARTESIAN_POINT('Ctrl Pts',(8.32310290799994,11.6,-7.93573928300002));
#171026=CARTESIAN_POINT('Ctrl Pts',(8.32283676099994,15.2,-7.93502251600002));
#171027=CARTESIAN_POINT('Ctrl Pts',(8.32283676099994,11.6,-7.93502251600002));
#171028=CARTESIAN_POINT('Ctrl Pts',(8.32230434799994,15.2,-7.93358949600002));
#171029=CARTESIAN_POINT('Ctrl Pts',(8.32230434799994,11.6,-7.93358949600002));
#171030=CARTESIAN_POINT('Ctrl Pts',(8.32150538099994,15.2,-7.93144150700002));
#171031=CARTESIAN_POINT('Ctrl Pts',(8.32150538099994,11.6,-7.93144150700002));
#171032=CARTESIAN_POINT('Ctrl Pts',(8.32043939299994,15.2,-7.92858060400001));
#171033=CARTESIAN_POINT('Ctrl Pts',(8.32043939299994,11.6,-7.92858060400001));
#171034=CARTESIAN_POINT('Ctrl Pts',(8.31910574599994,15.2,-7.92500961100002));
#171035=CARTESIAN_POINT('Ctrl Pts',(8.31910574599994,11.6,-7.92500961100002));
#171036=CARTESIAN_POINT('Ctrl Pts',(8.31777093699994,15.2,-7.92144375600002));
#171037=CARTESIAN_POINT('Ctrl Pts',(8.31777093699994,11.6,-7.92144375600002));
#171038=CARTESIAN_POINT('Ctrl Pts',(8.31643496899994,15.2,-7.91788304100002));
#171039=CARTESIAN_POINT('Ctrl Pts',(8.31643496899994,11.6,-7.91788304100002));
#171040=CARTESIAN_POINT('Ctrl Pts',(8.31509784399995,15.2,-7.91432746600002));
#171041=CARTESIAN_POINT('Ctrl Pts',(8.31509784399995,11.6,-7.91432746600002));
#171042=CARTESIAN_POINT('Ctrl Pts',(8.31375956699994,15.2,-7.91077703500001));
#171043=CARTESIAN_POINT('Ctrl Pts',(8.31375956699994,11.6,-7.91077703500001));
#171044=CARTESIAN_POINT('Ctrl Pts',(8.31242014699994,15.2,-7.90723175400001));
#171045=CARTESIAN_POINT('Ctrl Pts',(8.31242014699994,11.6,-7.90723175400001));
#171046=CARTESIAN_POINT('Ctrl Pts',(8.31107958999995,15.2,-7.90369162500002));
#171047=CARTESIAN_POINT('Ctrl Pts',(8.31107958999995,11.6,-7.90369162500002));
#171048=CARTESIAN_POINT('Ctrl Pts',(8.30973790699994,15.2,-7.90015665600002));
#171049=CARTESIAN_POINT('Ctrl Pts',(8.30973790699994,11.6,-7.90015665600002));
#171050=CARTESIAN_POINT('Ctrl Pts',(8.30839510599995,15.2,-7.89662685200001));
#171051=CARTESIAN_POINT('Ctrl Pts',(8.30839510599995,11.6,-7.89662685200001));
#171052=CARTESIAN_POINT('Ctrl Pts',(8.30705119799994,15.2,-7.89310221800001));
#171053=CARTESIAN_POINT('Ctrl Pts',(8.30705119799994,11.6,-7.89310221800001));
#171054=CARTESIAN_POINT('Ctrl Pts',(8.30570619199994,15.2,-7.88958275900002));
#171055=CARTESIAN_POINT('Ctrl Pts',(8.30570619199994,11.6,-7.88958275900002));
#171056=CARTESIAN_POINT('Ctrl Pts',(8.30436009499994,15.2,-7.88606848100001));
#171057=CARTESIAN_POINT('Ctrl Pts',(8.30436009499994,11.6,-7.88606848100001));
#171058=CARTESIAN_POINT('Ctrl Pts',(8.30301291399994,15.2,-7.88255938900001));
#171059=CARTESIAN_POINT('Ctrl Pts',(8.30301291399994,11.6,-7.88255938900001));
#171060=CARTESIAN_POINT('Ctrl Pts',(8.30166465799994,15.2,-7.87905548500002));
#171061=CARTESIAN_POINT('Ctrl Pts',(8.30166465799994,11.6,-7.87905548500002));
#171062=CARTESIAN_POINT('Ctrl Pts',(8.30031533299995,15.2,-7.87555677500002));
#171063=CARTESIAN_POINT('Ctrl Pts',(8.30031533299995,11.6,-7.87555677500002));
#171064=CARTESIAN_POINT('Ctrl Pts',(8.29896494599994,15.2,-7.87206326300002));
#171065=CARTESIAN_POINT('Ctrl Pts',(8.29896494599994,11.6,-7.87206326300002));
#171066=CARTESIAN_POINT('Ctrl Pts',(8.29761350399994,15.2,-7.86857495200002));
#171067=CARTESIAN_POINT('Ctrl Pts',(8.29761350399994,11.6,-7.86857495200002));
#171068=CARTESIAN_POINT('Ctrl Pts',(8.29626101599995,15.2,-7.86509184700002));
#171069=CARTESIAN_POINT('Ctrl Pts',(8.29626101599995,11.6,-7.86509184700002));
#171070=CARTESIAN_POINT('Ctrl Pts',(8.29490748799994,15.2,-7.86161395500002));
#171071=CARTESIAN_POINT('Ctrl Pts',(8.29490748799994,11.6,-7.86161395500002));
#171072=CARTESIAN_POINT('Ctrl Pts',(8.29355293099994,15.2,-7.85814127700001));
#171073=CARTESIAN_POINT('Ctrl Pts',(8.29355293099994,11.6,-7.85814127700001));
#171074=CARTESIAN_POINT('Ctrl Pts',(8.29219734999995,15.2,-7.85467382100002));
#171075=CARTESIAN_POINT('Ctrl Pts',(8.29219734999995,11.6,-7.85467382100002));
#171076=CARTESIAN_POINT('Ctrl Pts',(8.29084075499994,15.2,-7.85121159100001));
#171077=CARTESIAN_POINT('Ctrl Pts',(8.29084075499994,11.6,-7.85121159100001));
#171078=CARTESIAN_POINT('Ctrl Pts',(8.28948315499994,15.2,-7.84775459000001));
#171079=CARTESIAN_POINT('Ctrl Pts',(8.28948315499994,11.6,-7.84775459000001));
#171080=CARTESIAN_POINT('Ctrl Pts',(8.28812455599994,15.2,-7.84430282500002));
#171081=CARTESIAN_POINT('Ctrl Pts',(8.28812455599994,11.6,-7.84430282500002));
#171082=CARTESIAN_POINT('Ctrl Pts',(8.28676496699994,15.2,-7.84085630000002));
#171083=CARTESIAN_POINT('Ctrl Pts',(8.28676496699994,11.6,-7.84085630000002));
#171084=CARTESIAN_POINT('Ctrl Pts',(8.28540439599994,15.2,-7.83741501800002));
#171085=CARTESIAN_POINT('Ctrl Pts',(8.28540439599994,11.6,-7.83741501800002));
#171086=CARTESIAN_POINT('Ctrl Pts',(8.28404284999994,15.2,-7.83397898500001));
#171087=CARTESIAN_POINT('Ctrl Pts',(8.28404284999994,11.6,-7.83397898500001));
#171088=CARTESIAN_POINT('Ctrl Pts',(8.28268033699995,15.2,-7.83054820600002));
#171089=CARTESIAN_POINT('Ctrl Pts',(8.28268033699995,11.6,-7.83054820600002));
#171090=CARTESIAN_POINT('Ctrl Pts',(8.28131686599994,15.2,-7.82712268400001));
#171091=CARTESIAN_POINT('Ctrl Pts',(8.28131686599994,11.6,-7.82712268400001));
#171092=CARTESIAN_POINT('Ctrl Pts',(8.27995244399995,15.2,-7.82370242500001));
#171093=CARTESIAN_POINT('Ctrl Pts',(8.27995244399995,11.6,-7.82370242500001));
#171094=CARTESIAN_POINT('Ctrl Pts',(8.27858707899994,15.2,-7.82028743300001));
#171095=CARTESIAN_POINT('Ctrl Pts',(8.27858707899994,11.6,-7.82028743300001));
#171096=CARTESIAN_POINT('Ctrl Pts',(8.27722078099994,15.2,-7.81687771200002));
#171097=CARTESIAN_POINT('Ctrl Pts',(8.27722078099994,11.6,-7.81687771200002));
#171098=CARTESIAN_POINT('Ctrl Pts',(8.27585355599994,15.2,-7.81347326900002));
#171099=CARTESIAN_POINT('Ctrl Pts',(8.27585355599994,11.6,-7.81347326900002));
#171100=CARTESIAN_POINT('Ctrl Pts',(8.27448541299994,15.2,-7.81007410700001));
#171101=CARTESIAN_POINT('Ctrl Pts',(8.27448541299994,11.6,-7.81007410700001));
#171102=CARTESIAN_POINT('Ctrl Pts',(8.27311635999994,15.2,-7.80668023000001));
#171103=CARTESIAN_POINT('Ctrl Pts',(8.27311635999994,11.6,-7.80668023000001));
#171104=CARTESIAN_POINT('Ctrl Pts',(8.27174640499994,15.2,-7.80329164300002));
#171105=CARTESIAN_POINT('Ctrl Pts',(8.27174640499994,11.6,-7.80329164300002));
#171106=CARTESIAN_POINT('Ctrl Pts',(8.27037555599994,15.2,-7.79990835200002));
#171107=CARTESIAN_POINT('Ctrl Pts',(8.27037555599994,11.6,-7.79990835200002));
#171108=CARTESIAN_POINT('Ctrl Pts',(8.26900382399994,15.2,-7.79653036100001));
#171109=CARTESIAN_POINT('Ctrl Pts',(8.26900382399994,11.6,-7.79653036100001));
#171110=CARTESIAN_POINT('Ctrl Pts',(8.26763121199994,15.2,-7.79315767400002));
#171111=CARTESIAN_POINT('Ctrl Pts',(8.26763121199994,11.6,-7.79315767400002));
#171112=CARTESIAN_POINT('Ctrl Pts',(8.26625773199994,15.2,-7.78979029600002));
#171113=CARTESIAN_POINT('Ctrl Pts',(8.26625773199994,11.6,-7.78979029600002));
#171114=CARTESIAN_POINT('Ctrl Pts',(8.26488339199994,15.2,-7.78642823100002));
#171115=CARTESIAN_POINT('Ctrl Pts',(8.26488339199994,11.6,-7.78642823100002));
#171116=CARTESIAN_POINT('Ctrl Pts',(8.26350819799995,15.2,-7.78307148500001));
#171117=CARTESIAN_POINT('Ctrl Pts',(8.26350819799995,11.6,-7.78307148500001));
#171118=CARTESIAN_POINT('Ctrl Pts',(8.26213216099994,15.2,-7.77972006200002));
#171119=CARTESIAN_POINT('Ctrl Pts',(8.26213216099994,11.6,-7.77972006200002));
#171120=CARTESIAN_POINT('Ctrl Pts',(8.26075528799995,15.2,-7.77637396700002));
#171121=CARTESIAN_POINT('Ctrl Pts',(8.26075528799995,11.6,-7.77637396700002));
#171122=CARTESIAN_POINT('Ctrl Pts',(8.25937758699994,15.2,-7.77303320300001));
#171123=CARTESIAN_POINT('Ctrl Pts',(8.25937758699994,11.6,-7.77303320300001));
#171124=CARTESIAN_POINT('Ctrl Pts',(8.25799906799995,15.2,-7.76969777700002));
#171125=CARTESIAN_POINT('Ctrl Pts',(8.25799906799995,11.6,-7.76969777700002));
#171126=CARTESIAN_POINT('Ctrl Pts',(8.25661973699994,15.2,-7.76636769200002));
#171127=CARTESIAN_POINT('Ctrl Pts',(8.25661973699994,11.6,-7.76636769200002));
#171128=CARTESIAN_POINT('Ctrl Pts',(8.25523960299994,15.2,-7.76304295400001));
#171129=CARTESIAN_POINT('Ctrl Pts',(8.25523960299994,11.6,-7.76304295400001));
#171130=CARTESIAN_POINT('Ctrl Pts',(8.25385867499994,15.2,-7.75972356600001));
#171131=CARTESIAN_POINT('Ctrl Pts',(8.25385867499994,11.6,-7.75972356600001));
#171132=CARTESIAN_POINT('Ctrl Pts',(8.25247696199994,15.2,-7.75640953400002));
#171133=CARTESIAN_POINT('Ctrl Pts',(8.25247696199994,11.6,-7.75640953400002));
#171134=CARTESIAN_POINT('Ctrl Pts',(8.25109447199995,15.2,-7.75310086400002));
#171135=CARTESIAN_POINT('Ctrl Pts',(8.25109447199995,11.6,-7.75310086400002));
#171136=CARTESIAN_POINT('Ctrl Pts',(8.24971121199994,15.2,-7.74979755600001));
#171137=CARTESIAN_POINT('Ctrl Pts',(8.24971121199994,11.6,-7.74979755600001));
#171138=CARTESIAN_POINT('Ctrl Pts',(8.24832719199994,15.2,-7.74649962000002));
#171139=CARTESIAN_POINT('Ctrl Pts',(8.24832719199994,11.6,-7.74649962000002));
#171140=CARTESIAN_POINT('Ctrl Pts',(8.24694242099994,15.2,-7.74320705700001));
#171141=CARTESIAN_POINT('Ctrl Pts',(8.24694242099994,11.6,-7.74320705700001));
#171142=CARTESIAN_POINT('Ctrl Pts',(8.24555690699994,15.2,-7.73991987300001));
#171143=CARTESIAN_POINT('Ctrl Pts',(8.24555690699994,11.6,-7.73991987300001));
#171144=CARTESIAN_POINT('Ctrl Pts',(8.24417065699994,15.2,-7.73663807300002));
#171145=CARTESIAN_POINT('Ctrl Pts',(8.24417065699994,11.6,-7.73663807300002));
#171146=CARTESIAN_POINT('Ctrl Pts',(8.24278367999994,15.2,-7.73336166100002));
#171147=CARTESIAN_POINT('Ctrl Pts',(8.24278367999994,11.6,-7.73336166100002));
#171148=CARTESIAN_POINT('Ctrl Pts',(8.24139598699994,15.2,-7.73009064300001));
#171149=CARTESIAN_POINT('Ctrl Pts',(8.24139598699994,11.6,-7.73009064300001));
#171150=CARTESIAN_POINT('Ctrl Pts',(8.24000758299994,15.2,-7.72682502200002));
#171151=CARTESIAN_POINT('Ctrl Pts',(8.24000758299994,11.6,-7.72682502200002));
#171152=CARTESIAN_POINT('Ctrl Pts',(8.23861848099994,15.2,-7.72356480200001));
#171153=CARTESIAN_POINT('Ctrl Pts',(8.23861848099994,11.6,-7.72356480200001));
#171154=CARTESIAN_POINT('Ctrl Pts',(8.23722868599994,15.2,-7.72030999100001));
#171155=CARTESIAN_POINT('Ctrl Pts',(8.23722868599994,11.6,-7.72030999100001));
#171156=CARTESIAN_POINT('Ctrl Pts',(8.23583820599995,15.2,-7.71706059100002));
#171157=CARTESIAN_POINT('Ctrl Pts',(8.23583820599995,11.6,-7.71706059100002));
#171158=CARTESIAN_POINT('Ctrl Pts',(8.23444705399995,15.2,-7.71381660700002));
#171159=CARTESIAN_POINT('Ctrl Pts',(8.23444705399995,11.6,-7.71381660700002));
#171160=CARTESIAN_POINT('Ctrl Pts',(8.23305523399994,15.2,-7.71057804500002));
#171161=CARTESIAN_POINT('Ctrl Pts',(8.23305523399994,11.6,-7.71057804500002));
#171162=CARTESIAN_POINT('Ctrl Pts',(8.23166275799995,15.2,-7.70734490700002));
#171163=CARTESIAN_POINT('Ctrl Pts',(8.23166275799995,11.6,-7.70734490700002));
#171164=CARTESIAN_POINT('Ctrl Pts',(8.23026963299995,15.2,-7.70411720200002));
#171165=CARTESIAN_POINT('Ctrl Pts',(8.23026963299995,11.6,-7.70411720200002));
#171166=CARTESIAN_POINT('Ctrl Pts',(8.22887586899994,15.2,-7.70089492900001));
#171167=CARTESIAN_POINT('Ctrl Pts',(8.22887586899994,11.6,-7.70089492900001));
#171168=CARTESIAN_POINT('Ctrl Pts',(8.22748147299994,15.2,-7.69767809800002));
#171169=CARTESIAN_POINT('Ctrl Pts',(8.22748147299994,11.6,-7.69767809800002));
#171170=CARTESIAN_POINT('Ctrl Pts',(8.22608645599994,15.2,-7.69446671100001));
#171171=CARTESIAN_POINT('Ctrl Pts',(8.22608645599994,11.6,-7.69446671100001));
#171172=CARTESIAN_POINT('Ctrl Pts',(8.22469082399994,15.2,-7.69126077300001));
#171173=CARTESIAN_POINT('Ctrl Pts',(8.22469082399994,11.6,-7.69126077300001));
#171174=CARTESIAN_POINT('Ctrl Pts',(8.22329458799994,15.2,-7.68806029000002));
#171175=CARTESIAN_POINT('Ctrl Pts',(8.22329458799994,11.6,-7.68806029000002));
#171176=CARTESIAN_POINT('Ctrl Pts',(8.22189775699995,15.2,-7.68486526400002));
#171177=CARTESIAN_POINT('Ctrl Pts',(8.22189775699995,11.6,-7.68486526400002));
#171178=CARTESIAN_POINT('Ctrl Pts',(8.22050033799994,15.2,-7.68167570200001));
#171179=CARTESIAN_POINT('Ctrl Pts',(8.22050033799994,11.6,-7.68167570200001));
#171180=CARTESIAN_POINT('Ctrl Pts',(8.21910234199994,15.2,-7.67849160900001));
#171181=CARTESIAN_POINT('Ctrl Pts',(8.21910234199994,11.6,-7.67849160900001));
#171182=CARTESIAN_POINT('Ctrl Pts',(8.21770377699995,15.2,-7.67531298700002));
#171183=CARTESIAN_POINT('Ctrl Pts',(8.21770377699995,11.6,-7.67531298700002));
#171184=CARTESIAN_POINT('Ctrl Pts',(8.21630465099994,15.2,-7.67213984300002));
#171185=CARTESIAN_POINT('Ctrl Pts',(8.21630465099994,11.6,-7.67213984300002));
#171186=CARTESIAN_POINT('Ctrl Pts',(8.21490497299994,15.2,-7.66897218200001));
#171187=CARTESIAN_POINT('Ctrl Pts',(8.21490497299994,11.6,-7.66897218200001));
#171188=CARTESIAN_POINT('Ctrl Pts',(8.21350475399995,15.2,-7.66581000700001));
#171189=CARTESIAN_POINT('Ctrl Pts',(8.21350475399995,11.6,-7.66581000700001));
#171190=CARTESIAN_POINT('Ctrl Pts',(8.21210400199995,15.2,-7.66265332400001));
#171191=CARTESIAN_POINT('Ctrl Pts',(8.21210400199995,11.6,-7.66265332400001));
#171192=CARTESIAN_POINT('Ctrl Pts',(8.21070272499994,15.2,-7.65950213700001));
#171193=CARTESIAN_POINT('Ctrl Pts',(8.21070272499994,11.6,-7.65950213700001));
#171194=CARTESIAN_POINT('Ctrl Pts',(8.20930093299994,15.2,-7.65635645100001));
#171195=CARTESIAN_POINT('Ctrl Pts',(8.20930093299994,11.6,-7.65635645100001));
#171196=CARTESIAN_POINT('Ctrl Pts',(8.20789863399994,15.2,-7.65321627000001));
#171197=CARTESIAN_POINT('Ctrl Pts',(8.20789863399994,11.6,-7.65321627000001));
#171198=CARTESIAN_POINT('Ctrl Pts',(8.20649583899994,15.2,-7.65008160000002));
#171199=CARTESIAN_POINT('Ctrl Pts',(8.20649583899994,11.6,-7.65008160000002));
#171200=CARTESIAN_POINT('Ctrl Pts',(8.20509255499994,15.2,-7.64695244500002));
#171201=CARTESIAN_POINT('Ctrl Pts',(8.20509255499994,11.6,-7.64695244500002));
#171202=CARTESIAN_POINT('Ctrl Pts',(8.20368879299994,15.2,-7.64382880900002));
#171203=CARTESIAN_POINT('Ctrl Pts',(8.20368879299994,11.6,-7.64382880900002));
#171204=CARTESIAN_POINT('Ctrl Pts',(8.20228455999995,15.2,-7.64071069900002));
#171205=CARTESIAN_POINT('Ctrl Pts',(8.20228455999995,11.6,-7.64071069900002));
#171206=CARTESIAN_POINT('Ctrl Pts',(8.20087986699994,15.2,-7.63759811700002));
#171207=CARTESIAN_POINT('Ctrl Pts',(8.20087986699994,11.6,-7.63759811700002));
#171208=CARTESIAN_POINT('Ctrl Pts',(8.19947472199994,15.2,-7.63449107000002));
#171209=CARTESIAN_POINT('Ctrl Pts',(8.19947472199994,11.6,-7.63449107000002));
#171210=CARTESIAN_POINT('Ctrl Pts',(8.19806913599994,15.2,-7.63138956100001));
#171211=CARTESIAN_POINT('Ctrl Pts',(8.19806913599994,11.6,-7.63138956100001));
#171212=CARTESIAN_POINT('Ctrl Pts',(8.19666311599994,15.2,-7.62829359600002));
#171213=CARTESIAN_POINT('Ctrl Pts',(8.19666311599994,11.6,-7.62829359600002));
#171214=CARTESIAN_POINT('Ctrl Pts',(8.19525667099994,15.2,-7.62520317900002));
#171215=CARTESIAN_POINT('Ctrl Pts',(8.19525667099994,11.6,-7.62520317900002));
#171216=CARTESIAN_POINT('Ctrl Pts',(8.19384981299994,15.2,-7.62211831500001));
#171217=CARTESIAN_POINT('Ctrl Pts',(8.19384981299994,11.6,-7.62211831500001));
#171218=CARTESIAN_POINT('Ctrl Pts',(8.19244254899994,15.2,-7.61903900800001));
#171219=CARTESIAN_POINT('Ctrl Pts',(8.19244254899994,11.6,-7.61903900800001));
#171220=CARTESIAN_POINT('Ctrl Pts',(8.19103488899994,15.2,-7.61596526400002));
#171221=CARTESIAN_POINT('Ctrl Pts',(8.19103488899994,11.6,-7.61596526400002));
#171222=CARTESIAN_POINT('Ctrl Pts',(8.18962684199994,15.2,-7.61289708700001));
#171223=CARTESIAN_POINT('Ctrl Pts',(8.18962684199994,11.6,-7.61289708700001));
#171224=CARTESIAN_POINT('Ctrl Pts',(8.18821841799994,15.2,-7.60983448100002));
#171225=CARTESIAN_POINT('Ctrl Pts',(8.18821841799994,11.6,-7.60983448100002));
#171226=CARTESIAN_POINT('Ctrl Pts',(8.18680962599995,15.2,-7.60677745200002));
#171227=CARTESIAN_POINT('Ctrl Pts',(8.18680962599995,11.6,-7.60677745200002));
#171228=CARTESIAN_POINT('Ctrl Pts',(8.18540047699994,15.2,-7.60372600500002));
#171229=CARTESIAN_POINT('Ctrl Pts',(8.18540047699994,11.6,-7.60372600500002));
#171230=CARTESIAN_POINT('Ctrl Pts',(8.18399097599994,15.2,-7.60068014400002));
#171231=CARTESIAN_POINT('Ctrl Pts',(8.18399097599994,11.6,-7.60068014400002));
#171232=CARTESIAN_POINT('Ctrl Pts',(8.18258113699994,15.2,-7.59763987300002));
#171233=CARTESIAN_POINT('Ctrl Pts',(8.18258113699994,11.6,-7.59763987300002));
#171234=CARTESIAN_POINT('Ctrl Pts',(8.18117096699994,15.2,-7.59460519700002));
#171235=CARTESIAN_POINT('Ctrl Pts',(8.18117096699994,11.6,-7.59460519700002));
#171236=CARTESIAN_POINT('Ctrl Pts',(8.17976047699995,15.2,-7.59157612300001));
#171237=CARTESIAN_POINT('Ctrl Pts',(8.17976047699995,11.6,-7.59157612300001));
#171238=CARTESIAN_POINT('Ctrl Pts',(8.17834967399994,15.2,-7.58855265300002));
#171239=CARTESIAN_POINT('Ctrl Pts',(8.17834967399994,11.6,-7.58855265300002));
#171240=CARTESIAN_POINT('Ctrl Pts',(8.17693857099994,15.2,-7.58553479300001));
#171241=CARTESIAN_POINT('Ctrl Pts',(8.17693857099994,11.6,-7.58553479300001));
#171242=CARTESIAN_POINT('Ctrl Pts',(8.17552717499994,15.2,-7.58252254800002));
#171243=CARTESIAN_POINT('Ctrl Pts',(8.17552717499994,11.6,-7.58252254800002));
#171244=CARTESIAN_POINT('Ctrl Pts',(8.17411549699994,15.2,-7.57951592200002));
#171245=CARTESIAN_POINT('Ctrl Pts',(8.17411549699994,11.6,-7.57951592200002));
#171246=CARTESIAN_POINT('Ctrl Pts',(8.17270354399994,15.2,-7.57651491900001));
#171247=CARTESIAN_POINT('Ctrl Pts',(8.17270354399994,11.6,-7.57651491900001));
#171248=CARTESIAN_POINT('Ctrl Pts',(8.17129132899994,15.2,-7.57351954600002));
#171249=CARTESIAN_POINT('Ctrl Pts',(8.17129132899994,11.6,-7.57351954600002));
#171250=CARTESIAN_POINT('Ctrl Pts',(8.16987885999995,15.2,-7.57052980700001));
#171251=CARTESIAN_POINT('Ctrl Pts',(8.16987885999995,11.6,-7.57052980700001));
#171252=CARTESIAN_POINT('Ctrl Pts',(8.16846614699994,15.2,-7.56754570500001));
#171253=CARTESIAN_POINT('Ctrl Pts',(8.16846614699994,11.6,-7.56754570500001));
#171254=CARTESIAN_POINT('Ctrl Pts',(8.16705319899994,15.2,-7.56456724700002));
#171255=CARTESIAN_POINT('Ctrl Pts',(8.16705319899994,11.6,-7.56456724700002));
#171256=CARTESIAN_POINT('Ctrl Pts',(8.16564002699995,15.2,-7.56159443600002));
#171257=CARTESIAN_POINT('Ctrl Pts',(8.16564002699995,11.6,-7.56159443600002));
#171258=CARTESIAN_POINT('Ctrl Pts',(8.16422663899995,15.2,-7.55862727900002));
#171259=CARTESIAN_POINT('Ctrl Pts',(8.16422663899995,11.6,-7.55862727900002));
#171260=CARTESIAN_POINT('Ctrl Pts',(8.16281304699995,15.2,-7.55566577800002));
#171261=CARTESIAN_POINT('Ctrl Pts',(8.16281304699995,11.6,-7.55566577800002));
#171262=CARTESIAN_POINT('Ctrl Pts',(8.16139925799994,15.2,-7.55270994000002));
#171263=CARTESIAN_POINT('Ctrl Pts',(8.16139925799994,11.6,-7.55270994000002));
#171264=CARTESIAN_POINT('Ctrl Pts',(8.15998528399994,15.2,-7.54975976900001));
#171265=CARTESIAN_POINT('Ctrl Pts',(8.15998528399994,11.6,-7.54975976900001));
#171266=CARTESIAN_POINT('Ctrl Pts',(8.15857113399994,15.2,-7.54681526900002));
#171267=CARTESIAN_POINT('Ctrl Pts',(8.15857113399994,11.6,-7.54681526900002));
#171268=CARTESIAN_POINT('Ctrl Pts',(8.15715681899994,15.2,-7.54387644600002));
#171269=CARTESIAN_POINT('Ctrl Pts',(8.15715681899994,11.6,-7.54387644600002));
#171270=CARTESIAN_POINT('Ctrl Pts',(8.15574234599995,15.2,-7.54094330400001));
#171271=CARTESIAN_POINT('Ctrl Pts',(8.15574234599995,11.6,-7.54094330400001));
#171272=CARTESIAN_POINT('Ctrl Pts',(8.15432772699995,15.2,-7.53801584800001));
#171273=CARTESIAN_POINT('Ctrl Pts',(8.15432772699995,11.6,-7.53801584800001));
#171274=CARTESIAN_POINT('Ctrl Pts',(8.15291297199994,15.2,-7.53509408200002));
#171275=CARTESIAN_POINT('Ctrl Pts',(8.15291297199994,11.6,-7.53509408200002));
#171276=CARTESIAN_POINT('Ctrl Pts',(8.15149809099994,15.2,-7.53217801400002));
#171277=CARTESIAN_POINT('Ctrl Pts',(8.15149809099994,11.6,-7.53217801400002));
#171278=CARTESIAN_POINT('Ctrl Pts',(8.15008309399994,15.2,-7.52926764500002));
#171279=CARTESIAN_POINT('Ctrl Pts',(8.15008309399994,11.6,-7.52926764500002));
#171280=CARTESIAN_POINT('Ctrl Pts',(8.14866798999994,15.2,-7.52636298000001));
#171281=CARTESIAN_POINT('Ctrl Pts',(8.14866798999994,11.6,-7.52636298000001));
#171282=CARTESIAN_POINT('Ctrl Pts',(8.14725278899994,15.2,-7.52346402700002));
#171283=CARTESIAN_POINT('Ctrl Pts',(8.14725278899994,11.6,-7.52346402700002));
#171284=CARTESIAN_POINT('Ctrl Pts',(8.14583750199994,15.2,-7.52057078700001));
#171285=CARTESIAN_POINT('Ctrl Pts',(8.14583750199994,11.6,-7.52057078700001));
#171286=CARTESIAN_POINT('Ctrl Pts',(8.14442213799994,15.2,-7.51768326800001));
#171287=CARTESIAN_POINT('Ctrl Pts',(8.14442213799994,11.6,-7.51768326800001));
#171288=CARTESIAN_POINT('Ctrl Pts',(8.14300670799994,15.2,-7.51480147300001));
#171289=CARTESIAN_POINT('Ctrl Pts',(8.14300670799994,11.6,-7.51480147300001));
#171290=CARTESIAN_POINT('Ctrl Pts',(8.14159122299994,15.2,-7.51192540700002));
#171291=CARTESIAN_POINT('Ctrl Pts',(8.14159122299994,11.6,-7.51192540700002));
#171292=CARTESIAN_POINT('Ctrl Pts',(8.14017569099994,15.2,-7.50905507500002));
#171293=CARTESIAN_POINT('Ctrl Pts',(8.14017569099994,11.6,-7.50905507500002));
#171294=CARTESIAN_POINT('Ctrl Pts',(8.13876012299995,15.2,-7.50619048100001));
#171295=CARTESIAN_POINT('Ctrl Pts',(8.13876012299995,11.6,-7.50619048100001));
#171296=CARTESIAN_POINT('Ctrl Pts',(8.13734453099995,15.2,-7.50333163200001));
#171297=CARTESIAN_POINT('Ctrl Pts',(8.13734453099995,11.6,-7.50333163200001));
#171298=CARTESIAN_POINT('Ctrl Pts',(8.13592892199994,15.2,-7.50047853100002));
#171299=CARTESIAN_POINT('Ctrl Pts',(8.13592892199994,11.6,-7.50047853100002));
#171300=CARTESIAN_POINT('Ctrl Pts',(8.13451330699994,15.2,-7.49763118200002));
#171301=CARTESIAN_POINT('Ctrl Pts',(8.13451330699994,11.6,-7.49763118200002));
#171302=CARTESIAN_POINT('Ctrl Pts',(8.13309769899995,15.2,-7.49478959200002));
#171303=CARTESIAN_POINT('Ctrl Pts',(8.13309769899995,11.6,-7.49478959200002));
#171304=CARTESIAN_POINT('Ctrl Pts',(8.13168210599994,15.2,-7.49195376500002));
#171305=CARTESIAN_POINT('Ctrl Pts',(8.13168210599994,11.6,-7.49195376500002));
#171306=CARTESIAN_POINT('Ctrl Pts',(8.13026653799995,15.2,-7.48912370500002));
#171307=CARTESIAN_POINT('Ctrl Pts',(8.13026653799995,11.6,-7.48912370500002));
#171308=CARTESIAN_POINT('Ctrl Pts',(8.12885100599994,15.2,-7.48629941700001));
#171309=CARTESIAN_POINT('Ctrl Pts',(8.12885100599994,11.6,-7.48629941700001));
#171310=CARTESIAN_POINT('Ctrl Pts',(8.12743552099995,15.2,-7.48348090800001));
#171311=CARTESIAN_POINT('Ctrl Pts',(8.12743552099995,11.6,-7.48348090800001));
#171312=CARTESIAN_POINT('Ctrl Pts',(8.12602009199994,15.2,-7.48066818000002));
#171313=CARTESIAN_POINT('Ctrl Pts',(8.12602009199994,11.6,-7.48066818000002));
#171314=CARTESIAN_POINT('Ctrl Pts',(8.12460473099994,15.2,-7.47786123800001));
#171315=CARTESIAN_POINT('Ctrl Pts',(8.12460473099994,11.6,-7.47786123800001));
#171316=CARTESIAN_POINT('Ctrl Pts',(8.12318944699994,15.2,-7.47506008900002));
#171317=CARTESIAN_POINT('Ctrl Pts',(8.12318944699994,11.6,-7.47506008900002));
#171318=CARTESIAN_POINT('Ctrl Pts',(8.12177425199994,15.2,-7.47226473600002));
#171319=CARTESIAN_POINT('Ctrl Pts',(8.12177425199994,11.6,-7.47226473600002));
#171320=CARTESIAN_POINT('Ctrl Pts',(8.12035915499994,15.2,-7.46947518500002));
#171321=CARTESIAN_POINT('Ctrl Pts',(8.12035915499994,11.6,-7.46947518500002));
#171322=CARTESIAN_POINT('Ctrl Pts',(8.11894416699994,15.2,-7.46669144000002));
#171323=CARTESIAN_POINT('Ctrl Pts',(8.11894416699994,11.6,-7.46669144000002));
#171324=CARTESIAN_POINT('Ctrl Pts',(8.11752929899994,15.2,-7.46391350600002));
#171325=CARTESIAN_POINT('Ctrl Pts',(8.11752929899994,11.6,-7.46391350600002));
#171326=CARTESIAN_POINT('Ctrl Pts',(8.11611456099994,15.2,-7.46114138700002));
#171327=CARTESIAN_POINT('Ctrl Pts',(8.11611456099994,11.6,-7.46114138700002));
#171328=CARTESIAN_POINT('Ctrl Pts',(8.11469996399994,15.2,-7.45837509000002));
#171329=CARTESIAN_POINT('Ctrl Pts',(8.11469996399994,11.6,-7.45837509000002));
#171330=CARTESIAN_POINT('Ctrl Pts',(8.11328551799994,15.2,-7.45561461800002));
#171331=CARTESIAN_POINT('Ctrl Pts',(8.11328551799994,11.6,-7.45561461800002));
#171332=CARTESIAN_POINT('Ctrl Pts',(8.11187123599994,15.2,-7.45285997600002));
#171333=CARTESIAN_POINT('Ctrl Pts',(8.11187123599994,11.6,-7.45285997600002));
#171334=CARTESIAN_POINT('Ctrl Pts',(8.11045712499994,15.2,-7.45011117000002));
#171335=CARTESIAN_POINT('Ctrl Pts',(8.11045712499994,11.6,-7.45011117000002));
#171336=CARTESIAN_POINT('Ctrl Pts',(8.10904319799995,15.2,-7.44736820300002));
#171337=CARTESIAN_POINT('Ctrl Pts',(8.10904319799995,11.6,-7.44736820300002));
#171338=CARTESIAN_POINT('Ctrl Pts',(8.10762946499995,15.2,-7.44463108200001));
#171339=CARTESIAN_POINT('Ctrl Pts',(8.10762946499995,11.6,-7.44463108200001));
#171340=CARTESIAN_POINT('Ctrl Pts',(8.10621593799994,15.2,-7.44189981000002));
#171341=CARTESIAN_POINT('Ctrl Pts',(8.10621593799994,11.6,-7.44189981000002));
#171342=CARTESIAN_POINT('Ctrl Pts',(8.10480262699994,15.2,-7.43917439400001));
#171343=CARTESIAN_POINT('Ctrl Pts',(8.10480262699994,11.6,-7.43917439400001));
#171344=CARTESIAN_POINT('Ctrl Pts',(8.10338954199995,15.2,-7.43645483600002));
#171345=CARTESIAN_POINT('Ctrl Pts',(8.10338954199995,11.6,-7.43645483600002));
#171346=CARTESIAN_POINT('Ctrl Pts',(8.10197669399994,15.2,-7.43374114300002));
#171347=CARTESIAN_POINT('Ctrl Pts',(8.10197669399994,11.6,-7.43374114300002));
#171348=CARTESIAN_POINT('Ctrl Pts',(8.10056409499994,15.2,-7.43103331900001));
#171349=CARTESIAN_POINT('Ctrl Pts',(8.10056409499994,11.6,-7.43103331900001));
#171350=CARTESIAN_POINT('Ctrl Pts',(8.09915175599994,15.2,-7.42833136900002));
#171351=CARTESIAN_POINT('Ctrl Pts',(8.09915175599994,11.6,-7.42833136900002));
#171352=CARTESIAN_POINT('Ctrl Pts',(8.09773968599995,15.2,-7.42563529800002));
#171353=CARTESIAN_POINT('Ctrl Pts',(8.09773968599995,11.6,-7.42563529800002));
#171354=CARTESIAN_POINT('Ctrl Pts',(8.09632789799995,15.2,-7.42294511100001));
#171355=CARTESIAN_POINT('Ctrl Pts',(8.09632789799995,11.6,-7.42294511100001));
#171356=CARTESIAN_POINT('Ctrl Pts',(8.09491640099994,15.2,-7.42026081400001));
#171357=CARTESIAN_POINT('Ctrl Pts',(8.09491640099994,11.6,-7.42026081400001));
#171358=CARTESIAN_POINT('Ctrl Pts',(8.09350520799994,15.2,-7.41758240800002));
#171359=CARTESIAN_POINT('Ctrl Pts',(8.09350520799994,11.6,-7.41758240800002));
#171360=CARTESIAN_POINT('Ctrl Pts',(8.09209432999995,15.2,-7.41490990200001));
#171361=CARTESIAN_POINT('Ctrl Pts',(8.09209432999995,11.6,-7.41490990200001));
#171362=CARTESIAN_POINT('Ctrl Pts',(8.09068377599995,15.2,-7.41224329900002));
#171363=CARTESIAN_POINT('Ctrl Pts',(8.09068377599995,11.6,-7.41224329900002));
#171364=CARTESIAN_POINT('Ctrl Pts',(8.08927355799994,15.2,-7.40958260500002));
#171365=CARTESIAN_POINT('Ctrl Pts',(8.08927355799994,11.6,-7.40958260500002));
#171366=CARTESIAN_POINT('Ctrl Pts',(8.08786368899994,15.2,-7.40692782200002));
#171367=CARTESIAN_POINT('Ctrl Pts',(8.08786368899994,11.6,-7.40692782200002));
#171368=CARTESIAN_POINT('Ctrl Pts',(8.08645417899994,15.2,-7.40427895900002));
#171369=CARTESIAN_POINT('Ctrl Pts',(8.08645417899994,11.6,-7.40427895900002));
#171370=CARTESIAN_POINT('Ctrl Pts',(8.08504503799995,15.2,-7.40163601800001));
#171371=CARTESIAN_POINT('Ctrl Pts',(8.08504503799995,11.6,-7.40163601800001));
#171372=CARTESIAN_POINT('Ctrl Pts',(8.08363627799995,15.2,-7.39899900500002));
#171373=CARTESIAN_POINT('Ctrl Pts',(8.08363627799995,11.6,-7.39899900500002));
#171374=CARTESIAN_POINT('Ctrl Pts',(8.08222790999995,15.2,-7.39636792500002));
#171375=CARTESIAN_POINT('Ctrl Pts',(8.08222790999995,11.6,-7.39636792500002));
#171376=CARTESIAN_POINT('Ctrl Pts',(8.08081994599995,15.2,-7.39374278100002));
#171377=CARTESIAN_POINT('Ctrl Pts',(8.08081994599995,11.6,-7.39374278100002));
#171378=CARTESIAN_POINT('Ctrl Pts',(8.07941239799994,15.2,-7.39112358100002));
#171379=CARTESIAN_POINT('Ctrl Pts',(8.07941239799994,11.6,-7.39112358100002));
#171380=CARTESIAN_POINT('Ctrl Pts',(8.07800527499994,15.2,-7.38851032800002));
#171381=CARTESIAN_POINT('Ctrl Pts',(8.07800527499994,11.6,-7.38851032800002));
#171382=CARTESIAN_POINT('Ctrl Pts',(8.07659858999994,15.2,-7.38590302700001));
#171383=CARTESIAN_POINT('Ctrl Pts',(8.07659858999994,11.6,-7.38590302700001));
#171384=CARTESIAN_POINT('Ctrl Pts',(8.07519235299995,15.2,-7.38330168300001));
#171385=CARTESIAN_POINT('Ctrl Pts',(8.07519235299995,11.6,-7.38330168300001));
#171386=CARTESIAN_POINT('Ctrl Pts',(8.07378657799994,15.2,-7.38070630100002));
#171387=CARTESIAN_POINT('Ctrl Pts',(8.07378657799994,11.6,-7.38070630100002));
#171388=CARTESIAN_POINT('Ctrl Pts',(8.07238127399994,15.2,-7.37811688600001));
#171389=CARTESIAN_POINT('Ctrl Pts',(8.07238127399994,11.6,-7.37811688600001));
#171390=CARTESIAN_POINT('Ctrl Pts',(8.07097645399995,15.2,-7.37553344300002));
#171391=CARTESIAN_POINT('Ctrl Pts',(8.07097645399995,11.6,-7.37553344300002));
#171392=CARTESIAN_POINT('Ctrl Pts',(8.06957212799994,15.2,-7.37295597700002));
#171393=CARTESIAN_POINT('Ctrl Pts',(8.06957212799994,11.6,-7.37295597700002));
#171394=CARTESIAN_POINT('Ctrl Pts',(8.06816830899994,15.2,-7.37038449300002));
#171395=CARTESIAN_POINT('Ctrl Pts',(8.06816830899994,11.6,-7.37038449300002));
#171396=CARTESIAN_POINT('Ctrl Pts',(8.06676500799994,15.2,-7.36781899400002));
#171397=CARTESIAN_POINT('Ctrl Pts',(8.06676500799994,11.6,-7.36781899400002));
#171398=CARTESIAN_POINT('Ctrl Pts',(8.06536223699995,15.2,-7.36525948800002));
#171399=CARTESIAN_POINT('Ctrl Pts',(8.06536223699995,11.6,-7.36525948800002));
#171400=CARTESIAN_POINT('Ctrl Pts',(8.06396000599995,15.2,-7.36270597800001));
#171401=CARTESIAN_POINT('Ctrl Pts',(8.06396000599995,11.6,-7.36270597800001));
#171402=CARTESIAN_POINT('Ctrl Pts',(8.06255832899994,15.2,-7.36015847000001));
#171403=CARTESIAN_POINT('Ctrl Pts',(8.06255832899994,11.6,-7.36015847000001));
#171404=CARTESIAN_POINT('Ctrl Pts',(8.06115721599994,15.2,-7.35761696800001));
#171405=CARTESIAN_POINT('Ctrl Pts',(8.06115721599994,11.6,-7.35761696800001));
#171406=CARTESIAN_POINT('Ctrl Pts',(8.05975667999994,15.2,-7.35508147600001));
#171407=CARTESIAN_POINT('Ctrl Pts',(8.05975667999994,11.6,-7.35508147600001));
#171408=CARTESIAN_POINT('Ctrl Pts',(8.05835673199994,15.2,-7.35255200200001));
#171409=CARTESIAN_POINT('Ctrl Pts',(8.05835673199994,11.6,-7.35255200200001));
#171410=CARTESIAN_POINT('Ctrl Pts',(8.05695738399994,15.2,-7.35002854800002));
#171411=CARTESIAN_POINT('Ctrl Pts',(8.05695738399994,11.6,-7.35002854800002));
#171412=CARTESIAN_POINT('Ctrl Pts',(8.05555864699994,15.2,-7.34751112100002));
#171413=CARTESIAN_POINT('Ctrl Pts',(8.05555864699994,11.6,-7.34751112100002));
#171414=CARTESIAN_POINT('Ctrl Pts',(8.05416053399994,15.2,-7.34499972400001));
#171415=CARTESIAN_POINT('Ctrl Pts',(8.05416053399994,11.6,-7.34499972400001));
#171416=CARTESIAN_POINT('Ctrl Pts',(8.05276305599994,15.2,-7.34249436400002));
#171417=CARTESIAN_POINT('Ctrl Pts',(8.05276305599994,11.6,-7.34249436400002));
#171418=CARTESIAN_POINT('Ctrl Pts',(8.05136622599994,15.2,-7.33999504400002));
#171419=CARTESIAN_POINT('Ctrl Pts',(8.05136622599994,11.6,-7.33999504400002));
#171420=CARTESIAN_POINT('Ctrl Pts',(8.04997005499994,15.2,-7.33750177000001));
#171421=CARTESIAN_POINT('Ctrl Pts',(8.04997005499994,11.6,-7.33750177000001));
#171422=CARTESIAN_POINT('Ctrl Pts',(8.04857455599995,15.2,-7.33501454700002));
#171423=CARTESIAN_POINT('Ctrl Pts',(8.04857455599995,11.6,-7.33501454700002));
#171424=CARTESIAN_POINT('Ctrl Pts',(8.04717973999994,15.2,-7.33253338100001));
#171425=CARTESIAN_POINT('Ctrl Pts',(8.04717973999994,11.6,-7.33253338100001));
#171426=CARTESIAN_POINT('Ctrl Pts',(8.04578561899995,15.2,-7.33005827400002));
#171427=CARTESIAN_POINT('Ctrl Pts',(8.04578561899995,11.6,-7.33005827400002));
#171428=CARTESIAN_POINT('Ctrl Pts',(8.04439220499994,15.2,-7.32758923400001));
#171429=CARTESIAN_POINT('Ctrl Pts',(8.04439220499994,11.6,-7.32758923400001));
#171430=CARTESIAN_POINT('Ctrl Pts',(8.04299951199994,15.2,-7.32512626400001));
#171431=CARTESIAN_POINT('Ctrl Pts',(8.04299951199994,11.6,-7.32512626400001));
#171432=CARTESIAN_POINT('Ctrl Pts',(8.04160754999995,15.2,-7.32266936900002));
#171433=CARTESIAN_POINT('Ctrl Pts',(8.04160754999995,11.6,-7.32266936900002));
#171434=CARTESIAN_POINT('Ctrl Pts',(8.04021633199994,15.2,-7.32021855600002));
#171435=CARTESIAN_POINT('Ctrl Pts',(8.04021633199994,11.6,-7.32021855600002));
#171436=CARTESIAN_POINT('Ctrl Pts',(8.03882586899995,15.2,-7.31777382800002));
#171437=CARTESIAN_POINT('Ctrl Pts',(8.03882586899995,11.6,-7.31777382800002));
#171438=CARTESIAN_POINT('Ctrl Pts',(8.03743617699994,15.2,-7.31533519100001));
#171439=CARTESIAN_POINT('Ctrl Pts',(8.03743617699994,11.6,-7.31533519100001));
#171440=CARTESIAN_POINT('Ctrl Pts',(8.03604726399995,15.2,-7.31290264900001));
#171441=CARTESIAN_POINT('Ctrl Pts',(8.03604726399995,11.6,-7.31290264900001));
#171442=CARTESIAN_POINT('Ctrl Pts',(8.03465914399995,15.2,-7.31047620700001));
#171443=CARTESIAN_POINT('Ctrl Pts',(8.03465914399995,11.6,-7.31047620700001));
#171444=CARTESIAN_POINT('Ctrl Pts',(8.03327182899995,15.2,-7.30805587200001));
#171445=CARTESIAN_POINT('Ctrl Pts',(8.03327182899995,11.6,-7.30805587200001));
#171446=CARTESIAN_POINT('Ctrl Pts',(8.03188533199994,15.2,-7.30564164600001));
#171447=CARTESIAN_POINT('Ctrl Pts',(8.03188533199994,11.6,-7.30564164600001));
#171448=CARTESIAN_POINT('Ctrl Pts',(8.03049966599995,15.2,-7.30323353700002));
#171449=CARTESIAN_POINT('Ctrl Pts',(8.03049966599995,11.6,-7.30323353700002));
#171450=CARTESIAN_POINT('Ctrl Pts',(8.02911484199995,15.2,-7.30083154700001));
#171451=CARTESIAN_POINT('Ctrl Pts',(8.02911484199995,11.6,-7.30083154700001));
#171452=CARTESIAN_POINT('Ctrl Pts',(8.02773087299994,15.2,-7.29843568400002));
#171453=CARTESIAN_POINT('Ctrl Pts',(8.02773087299994,11.6,-7.29843568400002));
#171454=CARTESIAN_POINT('Ctrl Pts',(8.02634777099994,15.2,-7.29604595200002));
#171455=CARTESIAN_POINT('Ctrl Pts',(8.02634777099994,11.6,-7.29604595200002));
#171456=CARTESIAN_POINT('Ctrl Pts',(8.02496554899994,15.2,-7.29366235400001));
#171457=CARTESIAN_POINT('Ctrl Pts',(8.02496554899994,11.6,-7.29366235400001));
#171458=CARTESIAN_POINT('Ctrl Pts',(8.02358422099994,15.2,-7.29128489700001));
#171459=CARTESIAN_POINT('Ctrl Pts',(8.02358422099994,11.6,-7.29128489700001));
#171460=CARTESIAN_POINT('Ctrl Pts',(8.02220379799994,15.2,-7.28891358600002));
#171461=CARTESIAN_POINT('Ctrl Pts',(8.02220379799994,11.6,-7.28891358600002));
#171462=CARTESIAN_POINT('Ctrl Pts',(8.02082429299994,15.2,-7.28654842400001));
#171463=CARTESIAN_POINT('Ctrl Pts',(8.02082429299994,11.6,-7.28654842400001));
#171464=CARTESIAN_POINT('Ctrl Pts',(8.01944571799994,15.2,-7.28418941900002));
#171465=CARTESIAN_POINT('Ctrl Pts',(8.01944571799994,11.6,-7.28418941900002));
#171466=CARTESIAN_POINT('Ctrl Pts',(8.01806808699994,15.2,-7.28183657500002));
#171467=CARTESIAN_POINT('Ctrl Pts',(8.01806808699994,11.6,-7.28183657500002));
#171468=CARTESIAN_POINT('Ctrl Pts',(8.01669141199995,15.2,-7.27948989700002));
#171469=CARTESIAN_POINT('Ctrl Pts',(8.01669141199995,11.6,-7.27948989700002));
#171470=CARTESIAN_POINT('Ctrl Pts',(8.01531570699994,15.2,-7.27714938900001));
#171471=CARTESIAN_POINT('Ctrl Pts',(8.01531570699994,11.6,-7.27714938900001));
#171472=CARTESIAN_POINT('Ctrl Pts',(8.01394098199994,15.2,-7.27481505600001));
#171473=CARTESIAN_POINT('Ctrl Pts',(8.01394098199994,11.6,-7.27481505600001));
#171474=CARTESIAN_POINT('Ctrl Pts',(8.01256725299995,15.2,-7.27248690400002));
#171475=CARTESIAN_POINT('Ctrl Pts',(8.01256725299995,11.6,-7.27248690400002));
#171476=CARTESIAN_POINT('Ctrl Pts',(8.01119453199994,15.2,-7.27016493800001));
#171477=CARTESIAN_POINT('Ctrl Pts',(8.01119453199994,11.6,-7.27016493800001));
#171478=CARTESIAN_POINT('Ctrl Pts',(8.00982282999994,15.2,-7.26784916400002));
#171479=CARTESIAN_POINT('Ctrl Pts',(8.00982282999994,11.6,-7.26784916400002));
#171480=CARTESIAN_POINT('Ctrl Pts',(8.00845216399994,15.2,-7.26553958500002));
#171481=CARTESIAN_POINT('Ctrl Pts',(8.00845216399994,11.6,-7.26553958500002));
#171482=CARTESIAN_POINT('Ctrl Pts',(8.00708254199994,15.2,-7.26323620600001));
#171483=CARTESIAN_POINT('Ctrl Pts',(8.00708254199994,11.6,-7.26323620600001));
#171484=CARTESIAN_POINT('Ctrl Pts',(8.00571398099994,15.2,-7.26093903400002));
#171485=CARTESIAN_POINT('Ctrl Pts',(8.00571398099994,11.6,-7.26093903400002));
#171486=CARTESIAN_POINT('Ctrl Pts',(8.00434649299994,15.2,-7.25864807300002));
#171487=CARTESIAN_POINT('Ctrl Pts',(8.00434649299994,11.6,-7.25864807300002));
#171488=CARTESIAN_POINT('Ctrl Pts',(8.00298009099994,15.2,-7.25636332800002));
#171489=CARTESIAN_POINT('Ctrl Pts',(8.00298009099994,11.6,-7.25636332800002));
#171490=CARTESIAN_POINT('Ctrl Pts',(8.00161478799994,15.2,-7.25408480400001));
#171491=CARTESIAN_POINT('Ctrl Pts',(8.00161478799994,11.6,-7.25408480400001));
#171492=CARTESIAN_POINT('Ctrl Pts',(8.00025059599994,15.2,-7.25181250700001));
#171493=CARTESIAN_POINT('Ctrl Pts',(8.00025059599994,11.6,-7.25181250700001));
#171494=CARTESIAN_POINT('Ctrl Pts',(7.99888753099995,15.2,-7.24954644100002));
#171495=CARTESIAN_POINT('Ctrl Pts',(7.99888753099995,11.6,-7.24954644100002));
#171496=CARTESIAN_POINT('Ctrl Pts',(7.99752560499994,15.2,-7.24728661100002));
#171497=CARTESIAN_POINT('Ctrl Pts',(7.99752560499994,11.6,-7.24728661100002));
#171498=CARTESIAN_POINT('Ctrl Pts',(7.99616483099994,15.2,-7.24503302300001));
#171499=CARTESIAN_POINT('Ctrl Pts',(7.99616483099994,11.6,-7.24503302300001));
#171500=CARTESIAN_POINT('Ctrl Pts',(7.99480522199994,15.2,-7.24278568000001));
#171501=CARTESIAN_POINT('Ctrl Pts',(7.99480522199994,11.6,-7.24278568000001));
#171502=CARTESIAN_POINT('Ctrl Pts',(7.99344679099995,15.2,-7.24054459100002));
#171503=CARTESIAN_POINT('Ctrl Pts',(7.99344679099995,11.6,-7.24054459100002));
#171504=CARTESIAN_POINT('Ctrl Pts',(7.99208955399994,15.2,-7.23830975700002));
#171505=CARTESIAN_POINT('Ctrl Pts',(7.99208955399994,11.6,-7.23830975700002));
#171506=CARTESIAN_POINT('Ctrl Pts',(7.99073352199994,15.2,-7.23608118600002));
#171507=CARTESIAN_POINT('Ctrl Pts',(7.99073352199994,11.6,-7.23608118600002));
#171508=CARTESIAN_POINT('Ctrl Pts',(7.98937870999994,15.2,-7.23385888200001));
#171509=CARTESIAN_POINT('Ctrl Pts',(7.98937870999994,11.6,-7.23385888200001));
#171510=CARTESIAN_POINT('Ctrl Pts',(7.98802512999995,15.2,-7.23164284900002));
#171511=CARTESIAN_POINT('Ctrl Pts',(7.98802512999995,11.6,-7.23164284900002));
#171512=CARTESIAN_POINT('Ctrl Pts',(7.98667279799994,15.2,-7.22943309400002));
#171513=CARTESIAN_POINT('Ctrl Pts',(7.98667279799994,11.6,-7.22943309400002));
#171514=CARTESIAN_POINT('Ctrl Pts',(7.98532172499994,15.2,-7.22722962000002));
#171515=CARTESIAN_POINT('Ctrl Pts',(7.98532172499994,11.6,-7.22722962000002));
#171516=CARTESIAN_POINT('Ctrl Pts',(7.98397192599994,15.2,-7.22503243400002));
#171517=CARTESIAN_POINT('Ctrl Pts',(7.98397192599994,11.6,-7.22503243400002));
#171518=CARTESIAN_POINT('Ctrl Pts',(7.98262341399994,15.2,-7.22284154100001));
#171519=CARTESIAN_POINT('Ctrl Pts',(7.98262341399994,11.6,-7.22284154100001));
#171520=CARTESIAN_POINT('Ctrl Pts',(7.98127620499994,15.2,-7.22065694600002));
#171521=CARTESIAN_POINT('Ctrl Pts',(7.98127620499994,11.6,-7.22065694600002));
#171522=CARTESIAN_POINT('Ctrl Pts',(7.97993030999994,15.2,-7.21847865300001));
#171523=CARTESIAN_POINT('Ctrl Pts',(7.97993030999994,11.6,-7.21847865300001));
#171524=CARTESIAN_POINT('Ctrl Pts',(7.97858574299994,15.2,-7.21630666700002));
#171525=CARTESIAN_POINT('Ctrl Pts',(7.97858574299994,11.6,-7.21630666700002));
#171526=CARTESIAN_POINT('Ctrl Pts',(7.97724252099994,15.2,-7.21414099500001));
#171527=CARTESIAN_POINT('Ctrl Pts',(7.97724252099994,11.6,-7.21414099500001));
#171528=CARTESIAN_POINT('Ctrl Pts',(7.97590065499994,15.2,-7.21198164000001));
#171529=CARTESIAN_POINT('Ctrl Pts',(7.97590065499994,11.6,-7.21198164000001));
#171530=CARTESIAN_POINT('Ctrl Pts',(7.97456015899995,15.2,-7.20982861000002));
#171531=CARTESIAN_POINT('Ctrl Pts',(7.97456015899995,11.6,-7.20982861000002));
#171532=CARTESIAN_POINT('Ctrl Pts',(7.97322104799994,15.2,-7.20768190700002));
#171533=CARTESIAN_POINT('Ctrl Pts',(7.97322104799994,11.6,-7.20768190700002));
#171534=CARTESIAN_POINT('Ctrl Pts',(7.97188333599994,15.2,-7.20554153800002));
#171535=CARTESIAN_POINT('Ctrl Pts',(7.97188333599994,11.6,-7.20554153800002));
#171536=CARTESIAN_POINT('Ctrl Pts',(7.97054703699994,15.2,-7.20340750800001));
#171537=CARTESIAN_POINT('Ctrl Pts',(7.97054703699994,11.6,-7.20340750800001));
#171538=CARTESIAN_POINT('Ctrl Pts',(7.96921216599995,15.2,-7.20127982100002));
#171539=CARTESIAN_POINT('Ctrl Pts',(7.96921216599995,11.6,-7.20127982100002));
#171540=CARTESIAN_POINT('Ctrl Pts',(7.96787873499994,15.2,-7.19915848400002));
#171541=CARTESIAN_POINT('Ctrl Pts',(7.96787873499994,11.6,-7.19915848400002));
#171542=CARTESIAN_POINT('Ctrl Pts',(7.96654675899994,15.2,-7.19704350100002));
#171543=CARTESIAN_POINT('Ctrl Pts',(7.96654675899994,11.6,-7.19704350100002));
#171544=CARTESIAN_POINT('Ctrl Pts',(7.96521625299994,15.2,-7.19493487700002));
#171545=CARTESIAN_POINT('Ctrl Pts',(7.96521625299994,11.6,-7.19493487700002));
#171546=CARTESIAN_POINT('Ctrl Pts',(7.96388723099994,15.2,-7.19283261800002));
#171547=CARTESIAN_POINT('Ctrl Pts',(7.96388723099994,11.6,-7.19283261800002));
#171548=CARTESIAN_POINT('Ctrl Pts',(7.96255970799994,15.2,-7.19073672800001));
#171549=CARTESIAN_POINT('Ctrl Pts',(7.96255970799994,11.6,-7.19073672800001));
#171550=CARTESIAN_POINT('Ctrl Pts',(7.96123369799994,15.2,-7.18864721300001));
#171551=CARTESIAN_POINT('Ctrl Pts',(7.96123369799994,11.6,-7.18864721300001));
#171552=CARTESIAN_POINT('Ctrl Pts',(7.95990921399994,15.2,-7.18656407900002));
#171553=CARTESIAN_POINT('Ctrl Pts',(7.95990921399994,11.6,-7.18656407900002));
#171554=CARTESIAN_POINT('Ctrl Pts',(7.95858627199994,15.2,-7.18448732900002));
#171555=CARTESIAN_POINT('Ctrl Pts',(7.95858627199994,11.6,-7.18448732900002));
#171556=CARTESIAN_POINT('Ctrl Pts',(7.95726488599994,15.2,-7.18241697000002));
#171557=CARTESIAN_POINT('Ctrl Pts',(7.95726488599994,11.6,-7.18241697000002));
#171558=CARTESIAN_POINT('Ctrl Pts',(7.95594507099994,15.2,-7.18035300600001));
#171559=CARTESIAN_POINT('Ctrl Pts',(7.95594507099994,11.6,-7.18035300600001));
#171560=CARTESIAN_POINT('Ctrl Pts',(7.95462684099994,15.2,-7.17829544400002));
#171561=CARTESIAN_POINT('Ctrl Pts',(7.95462684099994,11.6,-7.17829544400002));
#171562=CARTESIAN_POINT('Ctrl Pts',(7.95331021099994,15.2,-7.17624428700002));
#171563=CARTESIAN_POINT('Ctrl Pts',(7.95331021099994,11.6,-7.17624428700002));
#171564=CARTESIAN_POINT('Ctrl Pts',(7.95199519599994,15.2,-7.17419954200002));
#171565=CARTESIAN_POINT('Ctrl Pts',(7.95199519599994,11.6,-7.17419954200002));
#171566=CARTESIAN_POINT('Ctrl Pts',(7.95068181099994,15.2,-7.17216121300002));
#171567=CARTESIAN_POINT('Ctrl Pts',(7.95068181099994,11.6,-7.17216121300002));
#171568=CARTESIAN_POINT('Ctrl Pts',(7.94937006899994,15.2,-7.17012930500001));
#171569=CARTESIAN_POINT('Ctrl Pts',(7.94937006899994,11.6,-7.17012930500001));
#171570=CARTESIAN_POINT('Ctrl Pts',(7.94805998699994,15.2,-7.16810382500002));
#171571=CARTESIAN_POINT('Ctrl Pts',(7.94805998699994,11.6,-7.16810382500002));
#171572=CARTESIAN_POINT('Ctrl Pts',(7.94675157799994,15.2,-7.16608477700002));
#171573=CARTESIAN_POINT('Ctrl Pts',(7.94675157799994,11.6,-7.16608477700002));
#171574=CARTESIAN_POINT('Ctrl Pts',(7.94544485899995,15.2,-7.16407216700001));
#171575=CARTESIAN_POINT('Ctrl Pts',(7.94544485899995,11.6,-7.16407216700001));
#171576=CARTESIAN_POINT('Ctrl Pts',(7.94413984299994,15.2,-7.16206599900002));
#171577=CARTESIAN_POINT('Ctrl Pts',(7.94413984299994,11.6,-7.16206599900002));
#171578=CARTESIAN_POINT('Ctrl Pts',(7.94283654599995,15.2,-7.16006627800001));
#171579=CARTESIAN_POINT('Ctrl Pts',(7.94283654599995,11.6,-7.16006627800001));
#171580=CARTESIAN_POINT('Ctrl Pts',(7.94153498399995,15.2,-7.15807301100002));
#171581=CARTESIAN_POINT('Ctrl Pts',(7.94153498399995,11.6,-7.15807301100002));
#171582=CARTESIAN_POINT('Ctrl Pts',(7.94023516999995,15.2,-7.15608620200002));
#171583=CARTESIAN_POINT('Ctrl Pts',(7.94023516999995,11.6,-7.15608620200002));
#171584=CARTESIAN_POINT('Ctrl Pts',(7.93893712099995,15.2,-7.15410585600001));
#171585=CARTESIAN_POINT('Ctrl Pts',(7.93893712099995,11.6,-7.15410585600001));
#171586=CARTESIAN_POINT('Ctrl Pts',(7.93764085099995,15.2,-7.15213198100002));
#171587=CARTESIAN_POINT('Ctrl Pts',(7.93764085099995,11.6,-7.15213198100002));
#171588=CARTESIAN_POINT('Ctrl Pts',(7.93634637499995,15.2,-7.15016457800001));
#171589=CARTESIAN_POINT('Ctrl Pts',(7.93634637499995,11.6,-7.15016457800001));
#171590=CARTESIAN_POINT('Ctrl Pts',(7.93505370999994,15.2,-7.14820365600002));
#171591=CARTESIAN_POINT('Ctrl Pts',(7.93505370999994,11.6,-7.14820365600002));
#171592=CARTESIAN_POINT('Ctrl Pts',(7.93376286999995,15.2,-7.14624921800001));
#171593=CARTESIAN_POINT('Ctrl Pts',(7.93376286999995,11.6,-7.14624921800001));
#171594=CARTESIAN_POINT('Ctrl Pts',(7.93247387099994,15.2,-7.14430127000002));
#171595=CARTESIAN_POINT('Ctrl Pts',(7.93247387099994,11.6,-7.14430127000002));
#171596=CARTESIAN_POINT('Ctrl Pts',(7.93118672799995,15.2,-7.14235981700002));
#171597=CARTESIAN_POINT('Ctrl Pts',(7.93118672799995,11.6,-7.14235981700002));
#171598=CARTESIAN_POINT('Ctrl Pts',(7.92990145699994,15.2,-7.14042486500002));
#171599=CARTESIAN_POINT('Ctrl Pts',(7.92990145699994,11.6,-7.14042486500002));
#171600=CARTESIAN_POINT('Ctrl Pts',(7.92861807299994,15.2,-7.13849641800002));
#171601=CARTESIAN_POINT('Ctrl Pts',(7.92861807299994,11.6,-7.13849641800002));
#171602=CARTESIAN_POINT('Ctrl Pts',(7.92733659099994,15.2,-7.13657448300002));
#171603=CARTESIAN_POINT('Ctrl Pts',(7.92733659099994,11.6,-7.13657448300002));
#171604=CARTESIAN_POINT('Ctrl Pts',(7.92605702899994,15.2,-7.13465906400002));
#171605=CARTESIAN_POINT('Ctrl Pts',(7.92605702899994,11.6,-7.13465906400002));
#171606=CARTESIAN_POINT('Ctrl Pts',(7.92477940099995,15.2,-7.13275016800001));
#171607=CARTESIAN_POINT('Ctrl Pts',(7.92477940099995,11.6,-7.13275016800001));
#171608=CARTESIAN_POINT('Ctrl Pts',(7.92350372299994,15.2,-7.13084779800001));
#171609=CARTESIAN_POINT('Ctrl Pts',(7.92350372299994,11.6,-7.13084779800001));
#171610=CARTESIAN_POINT('Ctrl Pts',(7.92223000999994,15.2,-7.12895196000002));
#171611=CARTESIAN_POINT('Ctrl Pts',(7.92223000999994,11.6,-7.12895196000002));
#171612=CARTESIAN_POINT('Ctrl Pts',(7.92095827899994,15.2,-7.12706266100002));
#171613=CARTESIAN_POINT('Ctrl Pts',(7.92095827899994,11.6,-7.12706266100002));
#171614=CARTESIAN_POINT('Ctrl Pts',(7.91968854599994,15.2,-7.12517990400002));
#171615=CARTESIAN_POINT('Ctrl Pts',(7.91968854599994,11.6,-7.12517990400002));
#171616=CARTESIAN_POINT('Ctrl Pts',(7.91842082599994,15.2,-7.12330369600001));
#171617=CARTESIAN_POINT('Ctrl Pts',(7.91842082599994,11.6,-7.12330369600001));
#171618=CARTESIAN_POINT('Ctrl Pts',(7.91715513599994,15.2,-7.12143404200001));
#171619=CARTESIAN_POINT('Ctrl Pts',(7.91715513599994,11.6,-7.12143404200001));
#171620=CARTESIAN_POINT('Ctrl Pts',(7.91589149199995,15.2,-7.11957094700002));
#171621=CARTESIAN_POINT('Ctrl Pts',(7.91589149199995,11.6,-7.11957094700002));
#171622=CARTESIAN_POINT('Ctrl Pts',(7.91462990899995,15.2,-7.11771441600002));
#171623=CARTESIAN_POINT('Ctrl Pts',(7.91462990899995,11.6,-7.11771441600002));
#171624=CARTESIAN_POINT('Ctrl Pts',(7.91337040399994,15.2,-7.11586445500001));
#171625=CARTESIAN_POINT('Ctrl Pts',(7.91337040399994,11.6,-7.11586445500001));
#171626=CARTESIAN_POINT('Ctrl Pts',(7.91211299299994,15.2,-7.11402106900002));
#171627=CARTESIAN_POINT('Ctrl Pts',(7.91211299299994,11.6,-7.11402106900002));
#171628=CARTESIAN_POINT('Ctrl Pts',(7.91085769199994,15.2,-7.11218426400002));
#171629=CARTESIAN_POINT('Ctrl Pts',(7.91085769199994,11.6,-7.11218426400002));
#171630=CARTESIAN_POINT('Ctrl Pts',(7.90960451799994,15.2,-7.11035404400001));
#171631=CARTESIAN_POINT('Ctrl Pts',(7.90960451799994,11.6,-7.11035404400001));
#171632=CARTESIAN_POINT('Ctrl Pts',(7.90835348799995,15.2,-7.10853041700001));
#171633=CARTESIAN_POINT('Ctrl Pts',(7.90835348799995,11.6,-7.10853041700001));
#171634=CARTESIAN_POINT('Ctrl Pts',(7.90710461699994,15.2,-7.10671338500001));
#171635=CARTESIAN_POINT('Ctrl Pts',(7.90710461699994,11.6,-7.10671338500001));
#171636=CARTESIAN_POINT('Ctrl Pts',(7.90585792199994,15.2,-7.10490295600002));
#171637=CARTESIAN_POINT('Ctrl Pts',(7.90585792199994,11.6,-7.10490295600002));
#171638=CARTESIAN_POINT('Ctrl Pts',(7.90461341899995,15.2,-7.10309913500001));
#171639=CARTESIAN_POINT('Ctrl Pts',(7.90461341899995,11.6,-7.10309913500001));
#171640=CARTESIAN_POINT('Ctrl Pts',(7.90337112499994,15.2,-7.10130192600002));
#171641=CARTESIAN_POINT('Ctrl Pts',(7.90337112499994,11.6,-7.10130192600002));
#171642=CARTESIAN_POINT('Ctrl Pts',(7.90213105799995,15.2,-7.09951133600002));
#171643=CARTESIAN_POINT('Ctrl Pts',(7.90213105799995,11.6,-7.09951133600002));
#171644=CARTESIAN_POINT('Ctrl Pts',(7.90089323199994,15.2,-7.09772736900002));
#171645=CARTESIAN_POINT('Ctrl Pts',(7.90089323199994,11.6,-7.09772736900002));
#171646=CARTESIAN_POINT('Ctrl Pts',(7.89965766699994,15.2,-7.09595003100001));
#171647=CARTESIAN_POINT('Ctrl Pts',(7.89965766699994,11.6,-7.09595003100001));
#171648=CARTESIAN_POINT('Ctrl Pts',(7.89842437699994,15.2,-7.09417932900001));
#171649=CARTESIAN_POINT('Ctrl Pts',(7.89842437699994,11.6,-7.09417932900001));
#171650=CARTESIAN_POINT('Ctrl Pts',(7.89719338099995,15.2,-7.09241526600002));
#171651=CARTESIAN_POINT('Ctrl Pts',(7.89719338099995,11.6,-7.09241526600002));
#171652=CARTESIAN_POINT('Ctrl Pts',(7.89596469399994,15.2,-7.09065784900002));
#171653=CARTESIAN_POINT('Ctrl Pts',(7.89596469399994,11.6,-7.09065784900002));
#171654=CARTESIAN_POINT('Ctrl Pts',(7.89473833399994,15.2,-7.08890708300002));
#171655=CARTESIAN_POINT('Ctrl Pts',(7.89473833399994,11.6,-7.08890708300002));
#171656=CARTESIAN_POINT('Ctrl Pts',(7.89351431799994,15.2,-7.08716297200001));
#171657=CARTESIAN_POINT('Ctrl Pts',(7.89351431799994,11.6,-7.08716297200001));
#171658=CARTESIAN_POINT('Ctrl Pts',(7.89229266299994,15.2,-7.08542552500001));
#171659=CARTESIAN_POINT('Ctrl Pts',(7.89229266299994,11.6,-7.08542552500001));
#171660=CARTESIAN_POINT('Ctrl Pts',(7.89107338599995,15.2,-7.08369474300002));
#171661=CARTESIAN_POINT('Ctrl Pts',(7.89107338599995,11.6,-7.08369474300002));
#171662=CARTESIAN_POINT('Ctrl Pts',(7.88985650599995,15.2,-7.08197063500001));
#171663=CARTESIAN_POINT('Ctrl Pts',(7.88985650599995,11.6,-7.08197063500001));
#171664=CARTESIAN_POINT('Ctrl Pts',(7.88864203699994,15.2,-7.08025320500001));
#171665=CARTESIAN_POINT('Ctrl Pts',(7.88864203699994,11.6,-7.08025320500001));
#171666=CARTESIAN_POINT('Ctrl Pts',(7.88742999899994,15.2,-7.07854245900001));
#171667=CARTESIAN_POINT('Ctrl Pts',(7.88742999899994,11.6,-7.07854245900001));
#171668=CARTESIAN_POINT('Ctrl Pts',(7.88622040799994,15.2,-7.07683840200002));
#171669=CARTESIAN_POINT('Ctrl Pts',(7.88622040799994,11.6,-7.07683840200002));
#171670=CARTESIAN_POINT('Ctrl Pts',(7.88501328299994,15.2,-7.07514104000002));
#171671=CARTESIAN_POINT('Ctrl Pts',(7.88501328299994,11.6,-7.07514104000002));
#171672=CARTESIAN_POINT('Ctrl Pts',(7.88380863899994,15.2,-7.07345037800001));
#171673=CARTESIAN_POINT('Ctrl Pts',(7.88380863899994,11.6,-7.07345037800001));
#171674=CARTESIAN_POINT('Ctrl Pts',(7.88260649599994,15.2,-7.07176642200002));
#171675=CARTESIAN_POINT('Ctrl Pts',(7.88260649599994,11.6,-7.07176642200002));
#171676=CARTESIAN_POINT('Ctrl Pts',(7.88140687099995,15.2,-7.07008917700002));
#171677=CARTESIAN_POINT('Ctrl Pts',(7.88140687099995,11.6,-7.07008917700002));
#171678=CARTESIAN_POINT('Ctrl Pts',(7.88020978099994,15.2,-7.06841865000002));
#171679=CARTESIAN_POINT('Ctrl Pts',(7.88020978099994,11.6,-7.06841865000002));
#171680=CARTESIAN_POINT('Ctrl Pts',(7.87901524399994,15.2,-7.06675484400002));
#171681=CARTESIAN_POINT('Ctrl Pts',(7.87901524399994,11.6,-7.06675484400002));
#171682=CARTESIAN_POINT('Ctrl Pts',(7.87782327799994,15.2,-7.06509776600001));
#171683=CARTESIAN_POINT('Ctrl Pts',(7.87782327799994,11.6,-7.06509776600001));
#171684=CARTESIAN_POINT('Ctrl Pts',(7.87663390099994,15.2,-7.06344742200002));
#171685=CARTESIAN_POINT('Ctrl Pts',(7.87663390099994,11.6,-7.06344742200002));
#171686=CARTESIAN_POINT('Ctrl Pts',(7.87544713199994,15.2,-7.06180381500002));
#171687=CARTESIAN_POINT('Ctrl Pts',(7.87544713199994,11.6,-7.06180381500002));
#171688=CARTESIAN_POINT('Ctrl Pts',(7.87426298699994,15.2,-7.06016695500002));
#171689=CARTESIAN_POINT('Ctrl Pts',(7.87426298699994,11.6,-7.06016695500002));
#171690=CARTESIAN_POINT('Ctrl Pts',(7.87308148499994,15.2,-7.05853684400001));
#171691=CARTESIAN_POINT('Ctrl Pts',(7.87308148499994,11.6,-7.05853684400001));
#171692=CARTESIAN_POINT('Ctrl Pts',(7.87190264399995,15.2,-7.05691348900002));
#171693=CARTESIAN_POINT('Ctrl Pts',(7.87190264399995,11.6,-7.05691348900002));
#171694=CARTESIAN_POINT('Ctrl Pts',(7.87072648199994,15.2,-7.05529689500001));
#171695=CARTESIAN_POINT('Ctrl Pts',(7.87072648199994,11.6,-7.05529689500001));
#171696=CARTESIAN_POINT('Ctrl Pts',(7.86955301799994,15.2,-7.05368706700002));
#171697=CARTESIAN_POINT('Ctrl Pts',(7.86955301799994,11.6,-7.05368706700002));
#171698=CARTESIAN_POINT('Ctrl Pts',(7.86838226999994,15.2,-7.05208401300002));
#171699=CARTESIAN_POINT('Ctrl Pts',(7.86838226999994,11.6,-7.05208401300002));
#171700=CARTESIAN_POINT('Ctrl Pts',(7.86721425699994,15.2,-7.05048773600002));
#171701=CARTESIAN_POINT('Ctrl Pts',(7.86721425699994,11.6,-7.05048773600002));
#171702=CARTESIAN_POINT('Ctrl Pts',(7.86604899599994,15.2,-7.04889824300002));
#171703=CARTESIAN_POINT('Ctrl Pts',(7.86604899599994,11.6,-7.04889824300002));
#171704=CARTESIAN_POINT('Ctrl Pts',(7.86488650699994,15.2,-7.04731553900002));
#171705=CARTESIAN_POINT('Ctrl Pts',(7.86488650699994,11.6,-7.04731553900002));
#171706=CARTESIAN_POINT('Ctrl Pts',(7.86372680699994,15.2,-7.04573963100002));
#171707=CARTESIAN_POINT('Ctrl Pts',(7.86372680699994,11.6,-7.04573963100002));
#171708=CARTESIAN_POINT('Ctrl Pts',(7.86256991599994,15.2,-7.04417052200002));
#171709=CARTESIAN_POINT('Ctrl Pts',(7.86256991599994,11.6,-7.04417052200002));
#171710=CARTESIAN_POINT('Ctrl Pts',(7.86141585299994,15.2,-7.04260821900001));
#171711=CARTESIAN_POINT('Ctrl Pts',(7.86141585299994,11.6,-7.04260821900001));
#171712=CARTESIAN_POINT('Ctrl Pts',(7.86026463599995,15.2,-7.04105272900001));
#171713=CARTESIAN_POINT('Ctrl Pts',(7.86026463599995,11.6,-7.04105272900001));
#171714=CARTESIAN_POINT('Ctrl Pts',(7.85911628399995,15.2,-7.03950405600001));
#171715=CARTESIAN_POINT('Ctrl Pts',(7.85911628399995,11.6,-7.03950405600001));
#171716=CARTESIAN_POINT('Ctrl Pts',(7.85797081499994,15.2,-7.03796220700001));
#171717=CARTESIAN_POINT('Ctrl Pts',(7.85797081499994,11.6,-7.03796220700001));
#171718=CARTESIAN_POINT('Ctrl Pts',(7.85682825099994,15.2,-7.03642718500002));
#171719=CARTESIAN_POINT('Ctrl Pts',(7.85682825099994,11.6,-7.03642718500002));
#171720=CARTESIAN_POINT('Ctrl Pts',(7.85568860799994,15.2,-7.03489899900001));
#171721=CARTESIAN_POINT('Ctrl Pts',(7.85568860799994,11.6,-7.03489899900001));
#171722=CARTESIAN_POINT('Ctrl Pts',(7.85455190599994,15.2,-7.03337765200001));
#171723=CARTESIAN_POINT('Ctrl Pts',(7.85455190599994,11.6,-7.03337765200001));
#171724=CARTESIAN_POINT('Ctrl Pts',(7.85341816499994,15.2,-7.03186315100002));
#171725=CARTESIAN_POINT('Ctrl Pts',(7.85341816499994,11.6,-7.03186315100002));
#171726=CARTESIAN_POINT('Ctrl Pts',(7.85228740299994,15.2,-7.03035550200001));
#171727=CARTESIAN_POINT('Ctrl Pts',(7.85228740299994,11.6,-7.03035550200001));
#171728=CARTESIAN_POINT('Ctrl Pts',(7.85115964099995,15.2,-7.02885471000001));
#171729=CARTESIAN_POINT('Ctrl Pts',(7.85115964099995,11.6,-7.02885471000001));
#171730=CARTESIAN_POINT('Ctrl Pts',(7.85003489699994,15.2,-7.02736078100001));
#171731=CARTESIAN_POINT('Ctrl Pts',(7.85003489699994,11.6,-7.02736078100001));
#171732=CARTESIAN_POINT('Ctrl Pts',(7.84891319099994,15.2,-7.02587372100002));
#171733=CARTESIAN_POINT('Ctrl Pts',(7.84891319099994,11.6,-7.02587372100002));
#171734=CARTESIAN_POINT('Ctrl Pts',(7.84779454299994,15.2,-7.02439353600001));
#171735=CARTESIAN_POINT('Ctrl Pts',(7.84779454299994,11.6,-7.02439353600001));
#171736=CARTESIAN_POINT('Ctrl Pts',(7.84667897299994,15.2,-7.02292023000001));
#171737=CARTESIAN_POINT('Ctrl Pts',(7.84667897299994,11.6,-7.02292023000001));
#171738=CARTESIAN_POINT('Ctrl Pts',(7.84556649899995,15.2,-7.02145381000002));
#171739=CARTESIAN_POINT('Ctrl Pts',(7.84556649899995,11.6,-7.02145381000002));
#171740=CARTESIAN_POINT('Ctrl Pts',(7.84445714199994,15.2,-7.01999428200001));
#171741=CARTESIAN_POINT('Ctrl Pts',(7.84445714199994,11.6,-7.01999428200001));
#171742=CARTESIAN_POINT('Ctrl Pts',(7.84335092199994,15.2,-7.01854165200002));
#171743=CARTESIAN_POINT('Ctrl Pts',(7.84335092199994,11.6,-7.01854165200002));
#171744=CARTESIAN_POINT('Ctrl Pts',(7.84224785899994,15.2,-7.01709592400002));
#171745=CARTESIAN_POINT('Ctrl Pts',(7.84224785899994,11.6,-7.01709592400002));
#171746=CARTESIAN_POINT('Ctrl Pts',(7.84114797199994,15.2,-7.01565710600002));
#171747=CARTESIAN_POINT('Ctrl Pts',(7.84114797199994,11.6,-7.01565710600002));
#171748=CARTESIAN_POINT('Ctrl Pts',(7.84005128199994,15.2,-7.01422520300002));
#171749=CARTESIAN_POINT('Ctrl Pts',(7.84005128199994,11.6,-7.01422520300002));
#171750=CARTESIAN_POINT('Ctrl Pts',(7.83895780899994,15.2,-7.01280021900001));
#171751=CARTESIAN_POINT('Ctrl Pts',(7.83895780899994,11.6,-7.01280021900001));
#171752=CARTESIAN_POINT('Ctrl Pts',(7.83786757299994,15.2,-7.01138216400001));
#171753=CARTESIAN_POINT('Ctrl Pts',(7.83786757299994,11.6,-7.01138216400001));
#171754=CARTESIAN_POINT('Ctrl Pts',(7.83678059499994,15.2,-7.00997103900002));
#171755=CARTESIAN_POINT('Ctrl Pts',(7.83678059499994,11.6,-7.00997103900002));
#171756=CARTESIAN_POINT('Ctrl Pts',(7.83569689499994,15.2,-7.00856685400002));
#171757=CARTESIAN_POINT('Ctrl Pts',(7.83569689499994,11.6,-7.00856685400002));
#171758=CARTESIAN_POINT('Ctrl Pts',(7.83461649299994,15.2,-7.00716961200002));
#171759=CARTESIAN_POINT('Ctrl Pts',(7.83461649299994,11.6,-7.00716961200002));
#171760=CARTESIAN_POINT('Ctrl Pts',(7.83353940999994,15.2,-7.00577931900002));
#171761=CARTESIAN_POINT('Ctrl Pts',(7.83353940999994,11.6,-7.00577931900002));
#171762=CARTESIAN_POINT('Ctrl Pts',(7.83246566699995,15.2,-7.00439598200001));
#171763=CARTESIAN_POINT('Ctrl Pts',(7.83246566699995,11.6,-7.00439598200001));
#171764=CARTESIAN_POINT('Ctrl Pts',(7.83139528399994,15.2,-7.00301960700001));
#171765=CARTESIAN_POINT('Ctrl Pts',(7.83139528399994,11.6,-7.00301960700001));
#171766=CARTESIAN_POINT('Ctrl Pts',(7.83032828199994,15.2,-7.00165020000002));
#171767=CARTESIAN_POINT('Ctrl Pts',(7.83032828199994,11.6,-7.00165020000002));
#171768=CARTESIAN_POINT('Ctrl Pts',(7.82926468199994,15.2,-7.00028776600002));
#171769=CARTESIAN_POINT('Ctrl Pts',(7.82926468199994,11.6,-7.00028776600002));
#171770=CARTESIAN_POINT('Ctrl Pts',(7.82820450599995,15.2,-6.99893231100001));
#171771=CARTESIAN_POINT('Ctrl Pts',(7.82820450599995,11.6,-6.99893231100001));
#171772=CARTESIAN_POINT('Ctrl Pts',(7.82714777299995,15.2,-6.99758384000001));
#171773=CARTESIAN_POINT('Ctrl Pts',(7.82714777299995,11.6,-6.99758384000001));
#171774=CARTESIAN_POINT('Ctrl Pts',(7.82609450599994,15.2,-6.99624236100002));
#171775=CARTESIAN_POINT('Ctrl Pts',(7.82609450599994,11.6,-6.99624236100002));
#171776=CARTESIAN_POINT('Ctrl Pts',(7.82504472499994,15.2,-6.99490787800002));
#171777=CARTESIAN_POINT('Ctrl Pts',(7.82504472499994,11.6,-6.99490787800002));
#171778=CARTESIAN_POINT('Ctrl Pts',(7.82399845099994,15.2,-6.99358039900002));
#171779=CARTESIAN_POINT('Ctrl Pts',(7.82399845099994,11.6,-6.99358039900002));
#171780=CARTESIAN_POINT('Ctrl Pts',(7.82295570699994,15.2,-6.99225992800002));
#171781=CARTESIAN_POINT('Ctrl Pts',(7.82295570699994,11.6,-6.99225992800002));
#171782=CARTESIAN_POINT('Ctrl Pts',(7.82191651399994,15.2,-6.99094647200001));
#171783=CARTESIAN_POINT('Ctrl Pts',(7.82191651399994,11.6,-6.99094647200001));
#171784=CARTESIAN_POINT('Ctrl Pts',(7.82088089199994,15.2,-6.98964003700001));
#171785=CARTESIAN_POINT('Ctrl Pts',(7.82088089199994,11.6,-6.98964003700001));
#171786=CARTESIAN_POINT('Ctrl Pts',(7.81984886499994,15.2,-6.98834063000002));
#171787=CARTESIAN_POINT('Ctrl Pts',(7.81984886499994,11.6,-6.98834063000002));
#171788=CARTESIAN_POINT('Ctrl Pts',(7.81882045199994,15.2,-6.98704825400001));
#171789=CARTESIAN_POINT('Ctrl Pts',(7.81882045199994,11.6,-6.98704825400001));
#171790=CARTESIAN_POINT('Ctrl Pts',(7.81779567699994,15.2,-6.98576291700002));
#171791=CARTESIAN_POINT('Ctrl Pts',(7.81779567699994,11.6,-6.98576291700002));
#171792=CARTESIAN_POINT('Ctrl Pts',(7.81677456099994,15.2,-6.98448462500001));
#171793=CARTESIAN_POINT('Ctrl Pts',(7.81677456099994,11.6,-6.98448462500001));
#171794=CARTESIAN_POINT('Ctrl Pts',(7.81575712599994,15.2,-6.98321338300002));
#171795=CARTESIAN_POINT('Ctrl Pts',(7.81575712599994,11.6,-6.98321338300002));
#171796=CARTESIAN_POINT('Ctrl Pts',(7.81474339499994,15.2,-6.98194919900001));
#171797=CARTESIAN_POINT('Ctrl Pts',(7.81474339499994,11.6,-6.98194919900001));
#171798=CARTESIAN_POINT('Ctrl Pts',(7.81373338799995,15.2,-6.98069207700001));
#171799=CARTESIAN_POINT('Ctrl Pts',(7.81373338799995,11.6,-6.98069207700001));
#171800=CARTESIAN_POINT('Ctrl Pts',(7.81272712999994,15.2,-6.97944202400001));
#171801=CARTESIAN_POINT('Ctrl Pts',(7.81272712999994,11.6,-6.97944202400001));
#171802=CARTESIAN_POINT('Ctrl Pts',(7.81172464099994,15.2,-6.97819904500002));
#171803=CARTESIAN_POINT('Ctrl Pts',(7.81172464099994,11.6,-6.97819904500002));
#171804=CARTESIAN_POINT('Ctrl Pts',(7.81072594399994,15.2,-6.97696314800002));
#171805=CARTESIAN_POINT('Ctrl Pts',(7.81072594399994,11.6,-6.97696314800002));
#171806=CARTESIAN_POINT('Ctrl Pts',(7.80973106299995,15.2,-6.97573433800001));
#171807=CARTESIAN_POINT('Ctrl Pts',(7.80973106299995,11.6,-6.97573433800001));
#171808=CARTESIAN_POINT('Ctrl Pts',(7.80874001999995,15.2,-6.97451262100002));
#171809=CARTESIAN_POINT('Ctrl Pts',(7.80874001999995,11.6,-6.97451262100002));
#171810=CARTESIAN_POINT('Ctrl Pts',(7.80775283599994,15.2,-6.97329800400002));
#171811=CARTESIAN_POINT('Ctrl Pts',(7.80775283599994,11.6,-6.97329800400002));
#171812=CARTESIAN_POINT('Ctrl Pts',(7.80676953599994,15.2,-6.97209049100002));
#171813=CARTESIAN_POINT('Ctrl Pts',(7.80676953599994,11.6,-6.97209049100002));
#171814=CARTESIAN_POINT('Ctrl Pts',(7.80579014099994,15.2,-6.97089009000001));
#171815=CARTESIAN_POINT('Ctrl Pts',(7.80579014099994,11.6,-6.97089009000001));
#171816=CARTESIAN_POINT('Ctrl Pts',(7.80481467499994,15.2,-6.96969680700001));
#171817=CARTESIAN_POINT('Ctrl Pts',(7.80481467499994,11.6,-6.96969680700001));
#171818=CARTESIAN_POINT('Ctrl Pts',(7.80384316099994,15.2,-6.96851064800001));
#171819=CARTESIAN_POINT('Ctrl Pts',(7.80384316099994,11.6,-6.96851064800001));
#171820=CARTESIAN_POINT('Ctrl Pts',(7.80287562299995,15.2,-6.96733161900001));
#171821=CARTESIAN_POINT('Ctrl Pts',(7.80287562299995,11.6,-6.96733161900001));
#171822=CARTESIAN_POINT('Ctrl Pts',(7.80191208299994,15.2,-6.96615972600001));
#171823=CARTESIAN_POINT('Ctrl Pts',(7.80191208299994,11.6,-6.96615972600001));
#171824=CARTESIAN_POINT('Ctrl Pts',(7.80095256499994,15.2,-6.96499497500002));
#171825=CARTESIAN_POINT('Ctrl Pts',(7.80095256499994,11.6,-6.96499497500002));
#171826=CARTESIAN_POINT('Ctrl Pts',(7.79999709199994,15.2,-6.96383737300001));
#171827=CARTESIAN_POINT('Ctrl Pts',(7.79999709199994,11.6,-6.96383737300001));
#171828=CARTESIAN_POINT('Ctrl Pts',(7.79904568799994,15.2,-6.96268692600002));
#171829=CARTESIAN_POINT('Ctrl Pts',(7.79904568799994,11.6,-6.96268692600002));
#171830=CARTESIAN_POINT('Ctrl Pts',(7.79809837699994,15.2,-6.96154364000002));
#171831=CARTESIAN_POINT('Ctrl Pts',(7.79809837699994,11.6,-6.96154364000002));
#171832=CARTESIAN_POINT('Ctrl Pts',(7.79715518199994,15.2,-6.96040752000001));
#171833=CARTESIAN_POINT('Ctrl Pts',(7.79715518199994,11.6,-6.96040752000001));
#171834=CARTESIAN_POINT('Ctrl Pts',(7.79621612699994,15.2,-6.95927857500001));
#171835=CARTESIAN_POINT('Ctrl Pts',(7.79621612699994,11.6,-6.95927857500001));
#171836=CARTESIAN_POINT('Ctrl Pts',(7.79528123699994,15.2,-6.95815681000001));
#171837=CARTESIAN_POINT('Ctrl Pts',(7.79528123699994,11.6,-6.95815681000001));
#171838=CARTESIAN_POINT('Ctrl Pts',(7.79435053399994,15.2,-6.95704223000002));
#171839=CARTESIAN_POINT('Ctrl Pts',(7.79435053399994,11.6,-6.95704223000002));
#171840=CARTESIAN_POINT('Ctrl Pts',(7.79342404399994,15.2,-6.95593484200002));
#171841=CARTESIAN_POINT('Ctrl Pts',(7.79342404399994,11.6,-6.95593484200002));
#171842=CARTESIAN_POINT('Ctrl Pts',(7.79250179099995,15.2,-6.95483465400001));
#171843=CARTESIAN_POINT('Ctrl Pts',(7.79250179099995,11.6,-6.95483465400001));
#171844=CARTESIAN_POINT('Ctrl Pts',(7.79158379899994,15.2,-6.95374167100002));
#171845=CARTESIAN_POINT('Ctrl Pts',(7.79158379899994,11.6,-6.95374167100002));
#171846=CARTESIAN_POINT('Ctrl Pts',(7.79067009299995,15.2,-6.95265589900002));
#171847=CARTESIAN_POINT('Ctrl Pts',(7.79067009299995,11.6,-6.95265589900002));
#171848=CARTESIAN_POINT('Ctrl Pts',(7.78976069699994,15.2,-6.95157734400001));
#171849=CARTESIAN_POINT('Ctrl Pts',(7.78976069699994,11.6,-6.95157734400001));
#171850=CARTESIAN_POINT('Ctrl Pts',(7.78885563499994,15.2,-6.95050601300002));
#171851=CARTESIAN_POINT('Ctrl Pts',(7.78885563499994,11.6,-6.95050601300002));
#171852=CARTESIAN_POINT('Ctrl Pts',(7.78795493299994,15.2,-6.94944191300002));
#171853=CARTESIAN_POINT('Ctrl Pts',(7.78795493299994,11.6,-6.94944191300002));
#171854=CARTESIAN_POINT('Ctrl Pts',(7.78705861699994,15.2,-6.94838504900002));
#171855=CARTESIAN_POINT('Ctrl Pts',(7.78705861699994,11.6,-6.94838504900002));
#171856=CARTESIAN_POINT('Ctrl Pts',(7.78616670899994,15.2,-6.94733542900002));
#171857=CARTESIAN_POINT('Ctrl Pts',(7.78616670899994,11.6,-6.94733542900002));
#171858=CARTESIAN_POINT('Ctrl Pts',(7.78527923799994,15.2,-6.94629305800002));
#171859=CARTESIAN_POINT('Ctrl Pts',(7.78527923799994,11.6,-6.94629305800002));
#171860=CARTESIAN_POINT('Ctrl Pts',(7.78439622499994,15.2,-6.94525794300001));
#171861=CARTESIAN_POINT('Ctrl Pts',(7.78439622499994,11.6,-6.94525794300001));
#171862=CARTESIAN_POINT('Ctrl Pts',(7.78351769799994,15.2,-6.94423009100002));
#171863=CARTESIAN_POINT('Ctrl Pts',(7.78351769799994,11.6,-6.94423009100002));
#171864=CARTESIAN_POINT('Ctrl Pts',(7.78264368299994,15.2,-6.94320950700002));
#171865=CARTESIAN_POINT('Ctrl Pts',(7.78264368299994,11.6,-6.94320950700002));
#171866=CARTESIAN_POINT('Ctrl Pts',(7.78177420299994,15.2,-6.94219620000001));
#171867=CARTESIAN_POINT('Ctrl Pts',(7.78177420299994,11.6,-6.94219620000001));
#171868=CARTESIAN_POINT('Ctrl Pts',(7.78090928599994,15.2,-6.94119017400002));
#171869=CARTESIAN_POINT('Ctrl Pts',(7.78090928599994,11.6,-6.94119017400002));
#171870=CARTESIAN_POINT('Ctrl Pts',(7.78004895599994,15.2,-6.94019143600002));
#171871=CARTESIAN_POINT('Ctrl Pts',(7.78004895599994,11.6,-6.94019143600002));
#171872=CARTESIAN_POINT('Ctrl Pts',(7.77919324199994,15.2,-6.93919999300002));
#171873=CARTESIAN_POINT('Ctrl Pts',(7.77919324199994,11.6,-6.93919999300002));
#171874=CARTESIAN_POINT('Ctrl Pts',(7.77834216699994,15.2,-6.93821585200002));
#171875=CARTESIAN_POINT('Ctrl Pts',(7.77834216699994,11.6,-6.93821585200002));
#171876=CARTESIAN_POINT('Ctrl Pts',(7.77749575799994,15.2,-6.93723901900002));
#171877=CARTESIAN_POINT('Ctrl Pts',(7.77749575799994,11.6,-6.93723901900002));
#171878=CARTESIAN_POINT('Ctrl Pts',(7.77665404199994,15.2,-6.93626950100001));
#171879=CARTESIAN_POINT('Ctrl Pts',(7.77665404199994,11.6,-6.93626950100001));
#171880=CARTESIAN_POINT('Ctrl Pts',(7.77581704399994,15.2,-6.93530730300001));
#171881=CARTESIAN_POINT('Ctrl Pts',(7.77581704399994,11.6,-6.93530730300001));
#171882=CARTESIAN_POINT('Ctrl Pts',(7.77498479199994,15.2,-6.93435243300002));
#171883=CARTESIAN_POINT('Ctrl Pts',(7.77498479199994,11.6,-6.93435243300002));
#171884=CARTESIAN_POINT('Ctrl Pts',(7.77415731199994,15.2,-6.93340489800002));
#171885=CARTESIAN_POINT('Ctrl Pts',(7.77415731199994,11.6,-6.93340489800002));
#171886=CARTESIAN_POINT('Ctrl Pts',(7.77333463099994,15.2,-6.93246470300001));
#171887=CARTESIAN_POINT('Ctrl Pts',(7.77333463099994,11.6,-6.93246470300001));
#171888=CARTESIAN_POINT('Ctrl Pts',(7.77251677499994,15.2,-6.93153185600002));
#171889=CARTESIAN_POINT('Ctrl Pts',(7.77251677499994,11.6,-6.93153185600002));
#171890=CARTESIAN_POINT('Ctrl Pts',(7.77170377299995,15.2,-6.93060636300002));
#171891=CARTESIAN_POINT('Ctrl Pts',(7.77170377299995,11.6,-6.93060636300002));
#171892=CARTESIAN_POINT('Ctrl Pts',(7.77089564999994,15.2,-6.92968823200002));
#171893=CARTESIAN_POINT('Ctrl Pts',(7.77089564999994,11.6,-6.92968823200002));
#171894=CARTESIAN_POINT('Ctrl Pts',(7.77009243399994,15.2,-6.92877746800002));
#171895=CARTESIAN_POINT('Ctrl Pts',(7.77009243399994,11.6,-6.92877746800002));
#171896=CARTESIAN_POINT('Ctrl Pts',(7.76929415399994,15.2,-6.92787407800001));
#171897=CARTESIAN_POINT('Ctrl Pts',(7.76929415399994,11.6,-6.92787407800001));
#171898=CARTESIAN_POINT('Ctrl Pts',(7.76850083499995,15.2,-6.92697807000001));
#171899=CARTESIAN_POINT('Ctrl Pts',(7.76850083499995,11.6,-6.92697807000001));
#171900=CARTESIAN_POINT('Ctrl Pts',(7.76771250599994,15.2,-6.92608944900002));
#171901=CARTESIAN_POINT('Ctrl Pts',(7.76771250599994,11.6,-6.92608944900002));
#171902=CARTESIAN_POINT('Ctrl Pts',(7.76692919399995,15.2,-6.92520822300001));
#171903=CARTESIAN_POINT('Ctrl Pts',(7.76692919399995,11.6,-6.92520822300001));
#171904=CARTESIAN_POINT('Ctrl Pts',(7.76615092799994,15.2,-6.92433439700002));
#171905=CARTESIAN_POINT('Ctrl Pts',(7.76615092799994,11.6,-6.92433439700002));
#171906=CARTESIAN_POINT('Ctrl Pts',(7.76537773499994,15.2,-6.92346798200001));
#171907=CARTESIAN_POINT('Ctrl Pts',(7.76537773499994,11.6,-6.92346798200001));
#171908=CARTESIAN_POINT('Ctrl Pts',(7.76460964399995,15.2,-6.92260898000002));
#171909=CARTESIAN_POINT('Ctrl Pts',(7.76460964399995,11.6,-6.92260898000002));
#171910=CARTESIAN_POINT('Ctrl Pts',(7.76384668299994,15.2,-6.92175740000001));
#171911=CARTESIAN_POINT('Ctrl Pts',(7.76384668299994,11.6,-6.92175740000001));
#171912=CARTESIAN_POINT('Ctrl Pts',(7.76308887999994,15.2,-6.92091324900002));
#171913=CARTESIAN_POINT('Ctrl Pts',(7.76308887999994,11.6,-6.92091324900002));
#171914=CARTESIAN_POINT('Ctrl Pts',(7.76233626399994,15.2,-6.92007653400001));
#171915=CARTESIAN_POINT('Ctrl Pts',(7.76233626399994,11.6,-6.92007653400001));
#171916=CARTESIAN_POINT('Ctrl Pts',(7.76158886399994,15.2,-6.91924726000002));
#171917=CARTESIAN_POINT('Ctrl Pts',(7.76158886399994,11.6,-6.91924726000002));
#171918=CARTESIAN_POINT('Ctrl Pts',(7.76084670899994,15.2,-6.91842543600002));
#171919=CARTESIAN_POINT('Ctrl Pts',(7.76084670899994,11.6,-6.91842543600002));
#171920=CARTESIAN_POINT('Ctrl Pts',(7.76010982699994,15.2,-6.91761106900002));
#171921=CARTESIAN_POINT('Ctrl Pts',(7.76010982699994,11.6,-6.91761106900002));
#171922=CARTESIAN_POINT('Ctrl Pts',(7.75937824799994,15.2,-6.91680416500001));
#171923=CARTESIAN_POINT('Ctrl Pts',(7.75937824799994,11.6,-6.91680416500001));
#171924=CARTESIAN_POINT('Ctrl Pts',(7.75865200099994,15.2,-6.91600473000002));
#171925=CARTESIAN_POINT('Ctrl Pts',(7.75865200099994,11.6,-6.91600473000002));
#171926=CARTESIAN_POINT('Ctrl Pts',(7.75793111599994,15.2,-6.91521277400001));
#171927=CARTESIAN_POINT('Ctrl Pts',(7.75793111599994,11.6,-6.91521277400001));
#171928=CARTESIAN_POINT('Ctrl Pts',(7.75721561999994,15.2,-6.91442830100002));
#171929=CARTESIAN_POINT('Ctrl Pts',(7.75721561999994,11.6,-6.91442830100002));
#171930=CARTESIAN_POINT('Ctrl Pts',(7.75650554599994,15.2,-6.91365131900002));
#171931=CARTESIAN_POINT('Ctrl Pts',(7.75650554599994,11.6,-6.91365131900002));
#171932=CARTESIAN_POINT('Ctrl Pts',(7.75580092299994,15.2,-6.91288183500002));
#171933=CARTESIAN_POINT('Ctrl Pts',(7.75580092299994,11.6,-6.91288183500002));
#171934=CARTESIAN_POINT('Ctrl Pts',(7.75510177999994,15.2,-6.91211985800001));
#171935=CARTESIAN_POINT('Ctrl Pts',(7.75510177999994,11.6,-6.91211985800001));
#171936=CARTESIAN_POINT('Ctrl Pts',(7.75440814899994,15.2,-6.91136539200001));
#171937=CARTESIAN_POINT('Ctrl Pts',(7.75440814899994,11.6,-6.91136539200001));
#171938=CARTESIAN_POINT('Ctrl Pts',(7.75372005699994,15.2,-6.91061844600001));
#171939=CARTESIAN_POINT('Ctrl Pts',(7.75372005699994,11.6,-6.91061844600001));
#171940=CARTESIAN_POINT('Ctrl Pts',(7.75303753799994,15.2,-6.90987902600002));
#171941=CARTESIAN_POINT('Ctrl Pts',(7.75303753799994,11.6,-6.90987902600002));
#171942=CARTESIAN_POINT('Ctrl Pts',(7.75236061999995,15.2,-6.90914714000002));
#171943=CARTESIAN_POINT('Ctrl Pts',(7.75236061999995,11.6,-6.90914714000002));
#171944=CARTESIAN_POINT('Ctrl Pts',(7.75168933499994,15.2,-6.90842279600002));
#171945=CARTESIAN_POINT('Ctrl Pts',(7.75168933499994,11.6,-6.90842279600002));
#171946=CARTESIAN_POINT('Ctrl Pts',(7.75102371399995,15.2,-6.90770599900001));
#171947=CARTESIAN_POINT('Ctrl Pts',(7.75102371399995,11.6,-6.90770599900001));
#171948=CARTESIAN_POINT('Ctrl Pts',(7.75036378799994,15.2,-6.90699675800002));
#171949=CARTESIAN_POINT('Ctrl Pts',(7.75036378799994,11.6,-6.90699675800002));
#171950=CARTESIAN_POINT('Ctrl Pts',(7.74970958799994,15.2,-6.90629507900002));
#171951=CARTESIAN_POINT('Ctrl Pts',(7.74970958799994,11.6,-6.90629507900002));
#171952=CARTESIAN_POINT('Ctrl Pts',(7.74906114399994,15.2,-6.90560097000001));
#171953=CARTESIAN_POINT('Ctrl Pts',(7.74906114399994,11.6,-6.90560097000001));
#171954=CARTESIAN_POINT('Ctrl Pts',(7.74841849099994,15.2,-6.90491443800001));
#171955=CARTESIAN_POINT('Ctrl Pts',(7.74841849099994,11.6,-6.90491443800001));
#171956=CARTESIAN_POINT('Ctrl Pts',(7.74778165799995,15.2,-6.90423549000001));
#171957=CARTESIAN_POINT('Ctrl Pts',(7.74778165799995,11.6,-6.90423549000001));
#171958=CARTESIAN_POINT('Ctrl Pts',(7.74715431199994,15.2,-6.90356800200002));
#171959=CARTESIAN_POINT('Ctrl Pts',(7.74715431199994,11.6,-6.90356800200002));
#171960=CARTESIAN_POINT('Ctrl Pts',(7.74665780199994,15.2,-6.90304077600001));
#171961=CARTESIAN_POINT('Ctrl Pts',(7.74665780199994,11.6,-6.90304077600001));
#171962=CARTESIAN_POINT('Ctrl Pts',(7.74628892999995,15.2,-6.90264967000001));
#171963=CARTESIAN_POINT('Ctrl Pts',(7.74628892999995,11.6,-6.90264967000001));
#171964=CARTESIAN_POINT('Ctrl Pts',(7.74604536199995,15.2,-6.90239167400001));
#171965=CARTESIAN_POINT('Ctrl Pts',(7.74604536199995,11.6,-6.90239167400001));
#171966=CARTESIAN_POINT('Ctrl Pts',(7.74592563699994,15.2,-6.90226492000001));
#171967=CARTESIAN_POINT('Ctrl Pts',(7.74592563699994,11.6,-6.90226492000001));
#171968=CARTESIAN_POINT('',(7.74592563699994,12.2,-6.90226492000001));
#171969=CARTESIAN_POINT('',(7.74592563699994,15.2,-6.90226492000001));
#171970=CARTESIAN_POINT('',(7.74592563699994,12.2,-6.90226492000001));
#171971=CARTESIAN_POINT('Ctrl Pts',(8.32310290799994,12.2,-7.93573928300002));
#171972=CARTESIAN_POINT('Ctrl Pts',(8.32283676099994,12.2,-7.93502251600002));
#171973=CARTESIAN_POINT('Ctrl Pts',(8.32230434799994,12.2,-7.93358949600002));
#171974=CARTESIAN_POINT('Ctrl Pts',(8.32150538099994,12.2,-7.93144150700002));
#171975=CARTESIAN_POINT('Ctrl Pts',(8.32043939299994,12.2,-7.92858060400001));
#171976=CARTESIAN_POINT('Ctrl Pts',(8.31910574599994,12.2,-7.92500961100002));
#171977=CARTESIAN_POINT('Ctrl Pts',(8.31777093699994,12.2,-7.92144375600002));
#171978=CARTESIAN_POINT('Ctrl Pts',(8.31643496899994,12.2,-7.91788304100002));
#171979=CARTESIAN_POINT('Ctrl Pts',(8.31509784399995,12.2,-7.91432746600002));
#171980=CARTESIAN_POINT('Ctrl Pts',(8.31375956699994,12.2,-7.91077703500001));
#171981=CARTESIAN_POINT('Ctrl Pts',(8.31242014699994,12.2,-7.90723175400001));
#171982=CARTESIAN_POINT('Ctrl Pts',(8.31107958999995,12.2,-7.90369162500002));
#171983=CARTESIAN_POINT('Ctrl Pts',(8.30973790699994,12.2,-7.90015665600002));
#171984=CARTESIAN_POINT('Ctrl Pts',(8.30812654585849,12.2,-7.89592089135391));
#171985=CARTESIAN_POINT('Ctrl Pts',(8.30651352407067,12.2,-7.89169288132307));
#171986=CARTESIAN_POINT('Ctrl Pts',(8.30489885992922,12.2,-7.88747263667696));
#171987=CARTESIAN_POINT('Ctrl Pts',(8.3032825651414,12.2,-7.88326016964612));
#171988=CARTESIAN_POINT('Ctrl Pts',(8.30166465799994,12.2,-7.87905548500002));
#171989=CARTESIAN_POINT('Ctrl Pts',(8.30031533299995,12.2,-7.87555677500002));
#171990=CARTESIAN_POINT('Ctrl Pts',(8.29896494599994,12.2,-7.87206326300002));
#171991=CARTESIAN_POINT('Ctrl Pts',(8.29761350399994,12.2,-7.86857495200002));
#171992=CARTESIAN_POINT('Ctrl Pts',(8.29626101599995,12.2,-7.86509184700002));
#171993=CARTESIAN_POINT('Ctrl Pts',(8.29490748799994,12.2,-7.86161395500002));
#171994=CARTESIAN_POINT('Ctrl Pts',(8.29355293099994,12.2,-7.85814127700001));
#171995=CARTESIAN_POINT('Ctrl Pts',(8.29219734999995,12.2,-7.85467382100002));
#171996=CARTESIAN_POINT('Ctrl Pts',(8.29084075499994,12.2,-7.85121159100001));
#171997=CARTESIAN_POINT('Ctrl Pts',(8.28948315499994,12.2,-7.84775459000001));
#171998=CARTESIAN_POINT('Ctrl Pts',(8.28812455599994,12.2,-7.84430282500002));
#171999=CARTESIAN_POINT('Ctrl Pts',(8.28676496699994,12.2,-7.84085630000002));
#172000=CARTESIAN_POINT('Ctrl Pts',(8.28540439599994,12.2,-7.83741501800002));
#172001=CARTESIAN_POINT('Ctrl Pts',(8.28404284999994,12.2,-7.83397898500001));
#172002=CARTESIAN_POINT('Ctrl Pts',(8.28268033699995,12.2,-7.83054820600002));
#172003=CARTESIAN_POINT('Ctrl Pts',(8.28131686599994,12.2,-7.82712268400001));
#172004=CARTESIAN_POINT('Ctrl Pts',(8.27995244399995,12.2,-7.82370242500001));
#172005=CARTESIAN_POINT('Ctrl Pts',(8.27858707899994,12.2,-7.82028743300001));
#172006=CARTESIAN_POINT('Ctrl Pts',(8.27722078099994,12.2,-7.81687771200002));
#172007=CARTESIAN_POINT('Ctrl Pts',(8.27585355599994,12.2,-7.81347326900002));
#172008=CARTESIAN_POINT('Ctrl Pts',(8.27448541299994,12.2,-7.81007410700001));
#172009=CARTESIAN_POINT('Ctrl Pts',(8.27311635999994,12.2,-7.80668023000001));
#172010=CARTESIAN_POINT('Ctrl Pts',(8.27174640499994,12.2,-7.80329164300002));
#172011=CARTESIAN_POINT('Ctrl Pts',(8.27037555599994,12.2,-7.79990835200002));
#172012=CARTESIAN_POINT('Ctrl Pts',(8.26900382399994,12.2,-7.79653036100001));
#172013=CARTESIAN_POINT('Ctrl Pts',(8.26763121199994,12.2,-7.79315767400002));
#172014=CARTESIAN_POINT('Ctrl Pts',(8.26625773199994,12.2,-7.78979029600002));
#172015=CARTESIAN_POINT('Ctrl Pts',(8.26488339199994,12.2,-7.78642823100002));
#172016=CARTESIAN_POINT('Ctrl Pts',(8.26350819799995,12.2,-7.78307148500001));
#172017=CARTESIAN_POINT('Ctrl Pts',(8.26213216099994,12.2,-7.77972006200002));
#172018=CARTESIAN_POINT('Ctrl Pts',(8.26075528799995,12.2,-7.77637396700002));
#172019=CARTESIAN_POINT('Ctrl Pts',(8.25937758699994,12.2,-7.77303320300001));
#172020=CARTESIAN_POINT('Ctrl Pts',(8.25799906799995,12.2,-7.76969777700002));
#172021=CARTESIAN_POINT('Ctrl Pts',(8.25661973699994,12.2,-7.76636769200002));
#172022=CARTESIAN_POINT('Ctrl Pts',(8.25523960299994,12.2,-7.76304295400001));
#172023=CARTESIAN_POINT('Ctrl Pts',(8.25385867499994,12.2,-7.75972356600001));
#172024=CARTESIAN_POINT('Ctrl Pts',(8.25247696199994,12.2,-7.75640953400002));
#172025=CARTESIAN_POINT('Ctrl Pts',(8.25109447199995,12.2,-7.75310086400002));
#172026=CARTESIAN_POINT('Ctrl Pts',(8.24971121199994,12.2,-7.74979755600001));
#172027=CARTESIAN_POINT('Ctrl Pts',(8.24832719199994,12.2,-7.74649962000002));
#172028=CARTESIAN_POINT('Ctrl Pts',(8.24694242099994,12.2,-7.74320705700001));
#172029=CARTESIAN_POINT('Ctrl Pts',(8.24555690699994,12.2,-7.73991987300001));
#172030=CARTESIAN_POINT('Ctrl Pts',(8.24417065699994,12.2,-7.73663807300002));
#172031=CARTESIAN_POINT('Ctrl Pts',(8.24278367999994,12.2,-7.73336166100002));
#172032=CARTESIAN_POINT('Ctrl Pts',(8.24139598699994,12.2,-7.73009064300001));
#172033=CARTESIAN_POINT('Ctrl Pts',(8.24000758299994,12.2,-7.72682502200002));
#172034=CARTESIAN_POINT('Ctrl Pts',(8.23861848099994,12.2,-7.72356480200001));
#172035=CARTESIAN_POINT('Ctrl Pts',(8.23722868599994,12.2,-7.72030999100001));
#172036=CARTESIAN_POINT('Ctrl Pts',(8.23583820599995,12.2,-7.71706059100002));
#172037=CARTESIAN_POINT('Ctrl Pts',(8.23444705399995,12.2,-7.71381660700002));
#172038=CARTESIAN_POINT('Ctrl Pts',(8.23305523399994,12.2,-7.71057804500002));
#172039=CARTESIAN_POINT('Ctrl Pts',(8.23166275799995,12.2,-7.70734490700002));
#172040=CARTESIAN_POINT('Ctrl Pts',(8.23026963299995,12.2,-7.70411720200002));
#172041=CARTESIAN_POINT('Ctrl Pts',(8.22887586899994,12.2,-7.70089492900001));
#172042=CARTESIAN_POINT('Ctrl Pts',(8.22748147299994,12.2,-7.69767809800002));
#172043=CARTESIAN_POINT('Ctrl Pts',(8.22608645599994,12.2,-7.69446671100001));
#172044=CARTESIAN_POINT('Ctrl Pts',(8.22469082399994,12.2,-7.69126077300001));
#172045=CARTESIAN_POINT('Ctrl Pts',(8.22329458799994,12.2,-7.68806029000002));
#172046=CARTESIAN_POINT('Ctrl Pts',(8.22189775699995,12.2,-7.68486526400002));
#172047=CARTESIAN_POINT('Ctrl Pts',(8.22050033799994,12.2,-7.68167570200001));
#172048=CARTESIAN_POINT('Ctrl Pts',(8.21910234199994,12.2,-7.67849160900001));
#172049=CARTESIAN_POINT('Ctrl Pts',(8.21770377699995,12.2,-7.67531298700002));
#172050=CARTESIAN_POINT('Ctrl Pts',(8.21630465099994,12.2,-7.67213984300002));
#172051=CARTESIAN_POINT('Ctrl Pts',(8.21490497299994,12.2,-7.66897218200001));
#172052=CARTESIAN_POINT('Ctrl Pts',(8.21350475399995,12.2,-7.66581000700001));
#172053=CARTESIAN_POINT('Ctrl Pts',(8.21210400199995,12.2,-7.66265332400001));
#172054=CARTESIAN_POINT('Ctrl Pts',(8.21070272499994,12.2,-7.65950213700001));
#172055=CARTESIAN_POINT('Ctrl Pts',(8.20930093299994,12.2,-7.65635645100001));
#172056=CARTESIAN_POINT('Ctrl Pts',(8.20789863399994,12.2,-7.65321627000001));
#172057=CARTESIAN_POINT('Ctrl Pts',(8.20649583899994,12.2,-7.65008160000002));
#172058=CARTESIAN_POINT('Ctrl Pts',(8.20509255499994,12.2,-7.64695244500002));
#172059=CARTESIAN_POINT('Ctrl Pts',(8.20368879299994,12.2,-7.64382880900002));
#172060=CARTESIAN_POINT('Ctrl Pts',(8.20228455999995,12.2,-7.64071069900002));
#172061=CARTESIAN_POINT('Ctrl Pts',(8.20087986699994,12.2,-7.63759811700002));
#172062=CARTESIAN_POINT('Ctrl Pts',(8.19947472199994,12.2,-7.63449107000002));
#172063=CARTESIAN_POINT('Ctrl Pts',(8.19806913599994,12.2,-7.63138956100001));
#172064=CARTESIAN_POINT('Ctrl Pts',(8.19666311599994,12.2,-7.62829359600002));
#172065=CARTESIAN_POINT('Ctrl Pts',(8.19525667099994,12.2,-7.62520317900002));
#172066=CARTESIAN_POINT('Ctrl Pts',(8.19384981299994,12.2,-7.62211831500001));
#172067=CARTESIAN_POINT('Ctrl Pts',(8.19244254899994,12.2,-7.61903900800001));
#172068=CARTESIAN_POINT('Ctrl Pts',(8.19103488899994,12.2,-7.61596526400002));
#172069=CARTESIAN_POINT('Ctrl Pts',(8.18962684199994,12.2,-7.61289708700001));
#172070=CARTESIAN_POINT('Ctrl Pts',(8.18821841799994,12.2,-7.60983448100002));
#172071=CARTESIAN_POINT('Ctrl Pts',(8.18680962599995,12.2,-7.60677745200002));
#172072=CARTESIAN_POINT('Ctrl Pts',(8.18540047699994,12.2,-7.60372600500002));
#172073=CARTESIAN_POINT('Ctrl Pts',(8.18399097599994,12.2,-7.60068014400002));
#172074=CARTESIAN_POINT('Ctrl Pts',(8.18258113699994,12.2,-7.59763987300002));
#172075=CARTESIAN_POINT('Ctrl Pts',(8.18117096699994,12.2,-7.59460519700002));
#172076=CARTESIAN_POINT('Ctrl Pts',(8.17976047699995,12.2,-7.59157612300001));
#172077=CARTESIAN_POINT('Ctrl Pts',(8.17834967399994,12.2,-7.58855265300002));
#172078=CARTESIAN_POINT('Ctrl Pts',(8.17693857099994,12.2,-7.58553479300001));
#172079=CARTESIAN_POINT('Ctrl Pts',(8.17552717499994,12.2,-7.58252254800002));
#172080=CARTESIAN_POINT('Ctrl Pts',(8.17411549699994,12.2,-7.57951592200002));
#172081=CARTESIAN_POINT('Ctrl Pts',(8.17270354399994,12.2,-7.57651491900001));
#172082=CARTESIAN_POINT('Ctrl Pts',(8.17129132899994,12.2,-7.57351954600002));
#172083=CARTESIAN_POINT('Ctrl Pts',(8.16987885999995,12.2,-7.57052980700001));
#172084=CARTESIAN_POINT('Ctrl Pts',(8.16846614699994,12.2,-7.56754570500001));
#172085=CARTESIAN_POINT('Ctrl Pts',(8.16705319899994,12.2,-7.56456724700002));
#172086=CARTESIAN_POINT('Ctrl Pts',(8.16564002699995,12.2,-7.56159443600002));
#172087=CARTESIAN_POINT('Ctrl Pts',(8.16422663899995,12.2,-7.55862727900002));
#172088=CARTESIAN_POINT('Ctrl Pts',(8.16281304699995,12.2,-7.55566577800002));
#172089=CARTESIAN_POINT('Ctrl Pts',(8.16139925799994,12.2,-7.55270994000002));
#172090=CARTESIAN_POINT('Ctrl Pts',(8.15998528399994,12.2,-7.54975976900001));
#172091=CARTESIAN_POINT('Ctrl Pts',(8.15857113399994,12.2,-7.54681526900002));
#172092=CARTESIAN_POINT('Ctrl Pts',(8.15715681899994,12.2,-7.54387644600002));
#172093=CARTESIAN_POINT('Ctrl Pts',(8.15574234599995,12.2,-7.54094330400001));
#172094=CARTESIAN_POINT('Ctrl Pts',(8.15432772699995,12.2,-7.53801584800001));
#172095=CARTESIAN_POINT('Ctrl Pts',(8.15291297199994,12.2,-7.53509408200002));
#172096=CARTESIAN_POINT('Ctrl Pts',(8.15149809099994,12.2,-7.53217801400002));
#172097=CARTESIAN_POINT('Ctrl Pts',(8.15008309399994,12.2,-7.52926764500002));
#172098=CARTESIAN_POINT('Ctrl Pts',(8.14866798999994,12.2,-7.52636298000001));
#172099=CARTESIAN_POINT('Ctrl Pts',(8.14725278899994,12.2,-7.52346402700002));
#172100=CARTESIAN_POINT('Ctrl Pts',(8.14583750199994,12.2,-7.52057078700001));
#172101=CARTESIAN_POINT('Ctrl Pts',(8.14442213799994,12.2,-7.51768326800001));
#172102=CARTESIAN_POINT('Ctrl Pts',(8.14300670799994,12.2,-7.51480147300001));
#172103=CARTESIAN_POINT('Ctrl Pts',(8.14159122299994,12.2,-7.51192540700002));
#172104=CARTESIAN_POINT('Ctrl Pts',(8.14017569099994,12.2,-7.50905507500002));
#172105=CARTESIAN_POINT('Ctrl Pts',(8.13876012299995,12.2,-7.50619048100001));
#172106=CARTESIAN_POINT('Ctrl Pts',(8.13734453099995,12.2,-7.50333163200001));
#172107=CARTESIAN_POINT('Ctrl Pts',(8.13592892199994,12.2,-7.50047853100002));
#172108=CARTESIAN_POINT('Ctrl Pts',(8.13423018390736,12.2,-7.4970617120138));
#172109=CARTESIAN_POINT('Ctrl Pts',(8.13253145646908,12.2,-7.49365353183833));
#172110=CARTESIAN_POINT('Ctrl Pts',(8.1308327555308,12.2,-7.4902539981617));
#172111=CARTESIAN_POINT('Ctrl Pts',(8.12913410293822,12.2,-7.48686311867665));
#172112=CARTESIAN_POINT('Ctrl Pts',(8.12743552099995,12.2,-7.48348090800001));
#172113=CARTESIAN_POINT('Ctrl Pts',(8.12602009199994,12.2,-7.48066818000002));
#172114=CARTESIAN_POINT('Ctrl Pts',(8.12460473099994,12.2,-7.47786123800001));
#172115=CARTESIAN_POINT('Ctrl Pts',(8.12318944699994,12.2,-7.47506008900002));
#172116=CARTESIAN_POINT('Ctrl Pts',(8.12177425199994,12.2,-7.47226473600002));
#172117=CARTESIAN_POINT('Ctrl Pts',(8.12035915499994,12.2,-7.46947518500002));
#172118=CARTESIAN_POINT('Ctrl Pts',(8.11894416699994,12.2,-7.46669144000002));
#172119=CARTESIAN_POINT('Ctrl Pts',(8.11752929899994,12.2,-7.46391350600002));
#172120=CARTESIAN_POINT('Ctrl Pts',(8.11611456099994,12.2,-7.46114138700002));
#172121=CARTESIAN_POINT('Ctrl Pts',(8.11469996399994,12.2,-7.45837509000002));
#172122=CARTESIAN_POINT('Ctrl Pts',(8.11328551799994,12.2,-7.45561461800002));
#172123=CARTESIAN_POINT('Ctrl Pts',(8.11187123599994,12.2,-7.45285997600002));
#172124=CARTESIAN_POINT('Ctrl Pts',(8.11045712499994,12.2,-7.45011117000002));
#172125=CARTESIAN_POINT('Ctrl Pts',(8.10904319799995,12.2,-7.44736820300002));
#172126=CARTESIAN_POINT('Ctrl Pts',(8.10762946499995,12.2,-7.44463108200001));
#172127=CARTESIAN_POINT('Ctrl Pts',(8.10621593799994,12.2,-7.44189981000002));
#172128=CARTESIAN_POINT('Ctrl Pts',(8.10480262699994,12.2,-7.43917439400001));
#172129=CARTESIAN_POINT('Ctrl Pts',(8.10338954199995,12.2,-7.43645483600002));
#172130=CARTESIAN_POINT('Ctrl Pts',(8.10197669399994,12.2,-7.43374114300002));
#172131=CARTESIAN_POINT('Ctrl Pts',(8.10056409499994,12.2,-7.43103331900001));
#172132=CARTESIAN_POINT('Ctrl Pts',(8.09915175599994,12.2,-7.42833136900002));
#172133=CARTESIAN_POINT('Ctrl Pts',(8.09773968599995,12.2,-7.42563529800002));
#172134=CARTESIAN_POINT('Ctrl Pts',(8.09632789799995,12.2,-7.42294511100001));
#172135=CARTESIAN_POINT('Ctrl Pts',(8.09491640099994,12.2,-7.42026081400001));
#172136=CARTESIAN_POINT('Ctrl Pts',(8.09350520799994,12.2,-7.41758240800002));
#172137=CARTESIAN_POINT('Ctrl Pts',(8.09209432999995,12.2,-7.41490990200001));
#172138=CARTESIAN_POINT('Ctrl Pts',(8.09068377599995,12.2,-7.41224329900002));
#172139=CARTESIAN_POINT('Ctrl Pts',(8.08927355799994,12.2,-7.40958260500002));
#172140=CARTESIAN_POINT('Ctrl Pts',(8.08786368899994,12.2,-7.40692782200002));
#172141=CARTESIAN_POINT('Ctrl Pts',(8.08645417899994,12.2,-7.40427895900002));
#172142=CARTESIAN_POINT('Ctrl Pts',(8.08504503799995,12.2,-7.40163601800001));
#172143=CARTESIAN_POINT('Ctrl Pts',(8.08363627799995,12.2,-7.39899900500002));
#172144=CARTESIAN_POINT('Ctrl Pts',(8.08222790999995,12.2,-7.39636792500002));
#172145=CARTESIAN_POINT('Ctrl Pts',(8.08081994599995,12.2,-7.39374278100002));
#172146=CARTESIAN_POINT('Ctrl Pts',(8.07941239799994,12.2,-7.39112358100002));
#172147=CARTESIAN_POINT('Ctrl Pts',(8.07800527499994,12.2,-7.38851032800002));
#172148=CARTESIAN_POINT('Ctrl Pts',(8.07659858999994,12.2,-7.38590302700001));
#172149=CARTESIAN_POINT('Ctrl Pts',(8.07519235299995,12.2,-7.38330168300001));
#172150=CARTESIAN_POINT('Ctrl Pts',(8.07378657799994,12.2,-7.38070630100002));
#172151=CARTESIAN_POINT('Ctrl Pts',(8.07238127399994,12.2,-7.37811688600001));
#172152=CARTESIAN_POINT('Ctrl Pts',(8.07097645399995,12.2,-7.37553344300002));
#172153=CARTESIAN_POINT('Ctrl Pts',(8.06957212799994,12.2,-7.37295597700002));
#172154=CARTESIAN_POINT('Ctrl Pts',(8.06816830899994,12.2,-7.37038449300002));
#172155=CARTESIAN_POINT('Ctrl Pts',(8.06676500799994,12.2,-7.36781899400002));
#172156=CARTESIAN_POINT('Ctrl Pts',(8.06536223699995,12.2,-7.36525948800002));
#172157=CARTESIAN_POINT('Ctrl Pts',(8.06396000599995,12.2,-7.36270597800001));
#172158=CARTESIAN_POINT('Ctrl Pts',(8.06255832899994,12.2,-7.36015847000001));
#172159=CARTESIAN_POINT('Ctrl Pts',(8.06115721599994,12.2,-7.35761696800001));
#172160=CARTESIAN_POINT('Ctrl Pts',(8.05975667999994,12.2,-7.35508147600001));
#172161=CARTESIAN_POINT('Ctrl Pts',(8.05835673199994,12.2,-7.35255200200001));
#172162=CARTESIAN_POINT('Ctrl Pts',(8.05695738399994,12.2,-7.35002854800002));
#172163=CARTESIAN_POINT('Ctrl Pts',(8.05555864699994,12.2,-7.34751112100002));
#172164=CARTESIAN_POINT('Ctrl Pts',(8.05416053399994,12.2,-7.34499972400001));
#172165=CARTESIAN_POINT('Ctrl Pts',(8.05276305599994,12.2,-7.34249436400002));
#172166=CARTESIAN_POINT('Ctrl Pts',(8.05136622599994,12.2,-7.33999504400002));
#172167=CARTESIAN_POINT('Ctrl Pts',(8.04997005499994,12.2,-7.33750177000001));
#172168=CARTESIAN_POINT('Ctrl Pts',(8.04857455599995,12.2,-7.33501454700002));
#172169=CARTESIAN_POINT('Ctrl Pts',(8.04717973999994,12.2,-7.33253338100001));
#172170=CARTESIAN_POINT('Ctrl Pts',(8.04578561899995,12.2,-7.33005827400002));
#172171=CARTESIAN_POINT('Ctrl Pts',(8.04439220499994,12.2,-7.32758923400001));
#172172=CARTESIAN_POINT('Ctrl Pts',(8.04299951199994,12.2,-7.32512626400001));
#172173=CARTESIAN_POINT('Ctrl Pts',(8.04160754999995,12.2,-7.32266936900002));
#172174=CARTESIAN_POINT('Ctrl Pts',(8.04021633199994,12.2,-7.32021855600002));
#172175=CARTESIAN_POINT('Ctrl Pts',(8.03882586899995,12.2,-7.31777382800002));
#172176=CARTESIAN_POINT('Ctrl Pts',(8.03743617699994,12.2,-7.31533519100001));
#172177=CARTESIAN_POINT('Ctrl Pts',(8.03604726399995,12.2,-7.31290264900001));
#172178=CARTESIAN_POINT('Ctrl Pts',(8.03465914399995,12.2,-7.31047620700001));
#172179=CARTESIAN_POINT('Ctrl Pts',(8.03327182899995,12.2,-7.30805587200001));
#172180=CARTESIAN_POINT('Ctrl Pts',(8.03188533199994,12.2,-7.30564164600001));
#172181=CARTESIAN_POINT('Ctrl Pts',(8.03049966599995,12.2,-7.30323353700002));
#172182=CARTESIAN_POINT('Ctrl Pts',(8.02911484199995,12.2,-7.30083154700001));
#172183=CARTESIAN_POINT('Ctrl Pts',(8.02773087299994,12.2,-7.29843568400002));
#172184=CARTESIAN_POINT('Ctrl Pts',(8.02634777099994,12.2,-7.29604595200002));
#172185=CARTESIAN_POINT('Ctrl Pts',(8.02496554899994,12.2,-7.29366235400001));
#172186=CARTESIAN_POINT('Ctrl Pts',(8.02358422099994,12.2,-7.29128489700001));
#172187=CARTESIAN_POINT('Ctrl Pts',(8.02220379799994,12.2,-7.28891358600002));
#172188=CARTESIAN_POINT('Ctrl Pts',(8.02082429299994,12.2,-7.28654842400001));
#172189=CARTESIAN_POINT('Ctrl Pts',(8.01944571799994,12.2,-7.28418941900002));
#172190=CARTESIAN_POINT('Ctrl Pts',(8.01806808699994,12.2,-7.28183657500002));
#172191=CARTESIAN_POINT('Ctrl Pts',(8.01669141199995,12.2,-7.27948989700002));
#172192=CARTESIAN_POINT('Ctrl Pts',(8.01531570699994,12.2,-7.27714938900001));
#172193=CARTESIAN_POINT('Ctrl Pts',(8.01394098199994,12.2,-7.27481505600001));
#172194=CARTESIAN_POINT('Ctrl Pts',(8.01256725299995,12.2,-7.27248690400002));
#172195=CARTESIAN_POINT('Ctrl Pts',(8.01119453199994,12.2,-7.27016493800001));
#172196=CARTESIAN_POINT('Ctrl Pts',(8.00982282999994,12.2,-7.26784916400002));
#172197=CARTESIAN_POINT('Ctrl Pts',(8.00845216399994,12.2,-7.26553958500002));
#172198=CARTESIAN_POINT('Ctrl Pts',(8.00708254199994,12.2,-7.26323620600001));
#172199=CARTESIAN_POINT('Ctrl Pts',(8.00571398099994,12.2,-7.26093903400002));
#172200=CARTESIAN_POINT('Ctrl Pts',(8.00434649299994,12.2,-7.25864807300002));
#172201=CARTESIAN_POINT('Ctrl Pts',(8.00298009099994,12.2,-7.25636332800002));
#172202=CARTESIAN_POINT('Ctrl Pts',(8.00161478799994,12.2,-7.25408480400001));
#172203=CARTESIAN_POINT('Ctrl Pts',(8.00025059599994,12.2,-7.25181250700001));
#172204=CARTESIAN_POINT('Ctrl Pts',(7.99888753099995,12.2,-7.24954644100002));
#172205=CARTESIAN_POINT('Ctrl Pts',(7.99752560499994,12.2,-7.24728661100002));
#172206=CARTESIAN_POINT('Ctrl Pts',(7.99616483099994,12.2,-7.24503302300001));
#172207=CARTESIAN_POINT('Ctrl Pts',(7.99480522199994,12.2,-7.24278568000001));
#172208=CARTESIAN_POINT('Ctrl Pts',(7.99344679099995,12.2,-7.24054459100002));
#172209=CARTESIAN_POINT('Ctrl Pts',(7.99208955399994,12.2,-7.23830975700002));
#172210=CARTESIAN_POINT('Ctrl Pts',(7.99073352199994,12.2,-7.23608118600002));
#172211=CARTESIAN_POINT('Ctrl Pts',(7.98937870999994,12.2,-7.23385888200001));
#172212=CARTESIAN_POINT('Ctrl Pts',(7.98802512999995,12.2,-7.23164284900002));
#172213=CARTESIAN_POINT('Ctrl Pts',(7.98667279799994,12.2,-7.22943309400002));
#172214=CARTESIAN_POINT('Ctrl Pts',(7.98532172499994,12.2,-7.22722962000002));
#172215=CARTESIAN_POINT('Ctrl Pts',(7.98397192599994,12.2,-7.22503243400002));
#172216=CARTESIAN_POINT('Ctrl Pts',(7.98262341399994,12.2,-7.22284154100001));
#172217=CARTESIAN_POINT('Ctrl Pts',(7.98127620499994,12.2,-7.22065694600002));
#172218=CARTESIAN_POINT('Ctrl Pts',(7.97993030999994,12.2,-7.21847865300001));
#172219=CARTESIAN_POINT('Ctrl Pts',(7.97858574299994,12.2,-7.21630666700002));
#172220=CARTESIAN_POINT('Ctrl Pts',(7.97724252099994,12.2,-7.21414099500001));
#172221=CARTESIAN_POINT('Ctrl Pts',(7.97590065499994,12.2,-7.21198164000001));
#172222=CARTESIAN_POINT('Ctrl Pts',(7.97456015899995,12.2,-7.20982861000002));
#172223=CARTESIAN_POINT('Ctrl Pts',(7.97322104799994,12.2,-7.20768190700002));
#172224=CARTESIAN_POINT('Ctrl Pts',(7.97188333599994,12.2,-7.20554153800002));
#172225=CARTESIAN_POINT('Ctrl Pts',(7.97054703699994,12.2,-7.20340750800001));
#172226=CARTESIAN_POINT('Ctrl Pts',(7.96921216599995,12.2,-7.20127982100002));
#172227=CARTESIAN_POINT('Ctrl Pts',(7.96787873499994,12.2,-7.19915848400002));
#172228=CARTESIAN_POINT('Ctrl Pts',(7.96654675899994,12.2,-7.19704350100002));
#172229=CARTESIAN_POINT('Ctrl Pts',(7.96521625299994,12.2,-7.19493487700002));
#172230=CARTESIAN_POINT('Ctrl Pts',(7.96388723099994,12.2,-7.19283261800002));
#172231=CARTESIAN_POINT('Ctrl Pts',(7.96255970799994,12.2,-7.19073672800001));
#172232=CARTESIAN_POINT('Ctrl Pts',(7.96123369799994,12.2,-7.18864721300001));
#172233=CARTESIAN_POINT('Ctrl Pts',(7.95990921399994,12.2,-7.18656407900002));
#172234=CARTESIAN_POINT('Ctrl Pts',(7.95858627199994,12.2,-7.18448732900002));
#172235=CARTESIAN_POINT('Ctrl Pts',(7.95726488599994,12.2,-7.18241697000002));
#172236=CARTESIAN_POINT('Ctrl Pts',(7.95594507099994,12.2,-7.18035300600001));
#172237=CARTESIAN_POINT('Ctrl Pts',(7.95462684099994,12.2,-7.17829544400002));
#172238=CARTESIAN_POINT('Ctrl Pts',(7.95331021099994,12.2,-7.17624428700002));
#172239=CARTESIAN_POINT('Ctrl Pts',(7.95199519599994,12.2,-7.17419954200002));
#172240=CARTESIAN_POINT('Ctrl Pts',(7.95068181099994,12.2,-7.17216121300002));
#172241=CARTESIAN_POINT('Ctrl Pts',(7.94937006899994,12.2,-7.17012930500001));
#172242=CARTESIAN_POINT('Ctrl Pts',(7.94805998699994,12.2,-7.16810382500002));
#172243=CARTESIAN_POINT('Ctrl Pts',(7.94675157799994,12.2,-7.16608477700002));
#172244=CARTESIAN_POINT('Ctrl Pts',(7.94544485899995,12.2,-7.16407216700001));
#172245=CARTESIAN_POINT('Ctrl Pts',(7.94413984299994,12.2,-7.16206599900002));
#172246=CARTESIAN_POINT('Ctrl Pts',(7.94283654599995,12.2,-7.16006627800001));
#172247=CARTESIAN_POINT('Ctrl Pts',(7.94153498399995,12.2,-7.15807301100002));
#172248=CARTESIAN_POINT('Ctrl Pts',(7.94023516999995,12.2,-7.15608620200002));
#172249=CARTESIAN_POINT('Ctrl Pts',(7.93893712099995,12.2,-7.15410585600001));
#172250=CARTESIAN_POINT('Ctrl Pts',(7.93764085099995,12.2,-7.15213198100002));
#172251=CARTESIAN_POINT('Ctrl Pts',(7.93634637499995,12.2,-7.15016457800001));
#172252=CARTESIAN_POINT('Ctrl Pts',(7.93505370999994,12.2,-7.14820365600002));
#172253=CARTESIAN_POINT('Ctrl Pts',(7.93376286999995,12.2,-7.14624921800001));
#172254=CARTESIAN_POINT('Ctrl Pts',(7.93247387099994,12.2,-7.14430127000002));
#172255=CARTESIAN_POINT('Ctrl Pts',(7.93118672799995,12.2,-7.14235981700002));
#172256=CARTESIAN_POINT('Ctrl Pts',(7.92990145699994,12.2,-7.14042486500002));
#172257=CARTESIAN_POINT('Ctrl Pts',(7.92861807299994,12.2,-7.13849641800002));
#172258=CARTESIAN_POINT('Ctrl Pts',(7.92733659099994,12.2,-7.13657448300002));
#172259=CARTESIAN_POINT('Ctrl Pts',(7.92605702899994,12.2,-7.13465906400002));
#172260=CARTESIAN_POINT('Ctrl Pts',(7.92477940099995,12.2,-7.13275016800001));
#172261=CARTESIAN_POINT('Ctrl Pts',(7.92350372299994,12.2,-7.13084779800001));
#172262=CARTESIAN_POINT('Ctrl Pts',(7.92223000999994,12.2,-7.12895196000002));
#172263=CARTESIAN_POINT('Ctrl Pts',(7.92095827899994,12.2,-7.12706266100002));
#172264=CARTESIAN_POINT('Ctrl Pts',(7.91968854599994,12.2,-7.12517990400002));
#172265=CARTESIAN_POINT('Ctrl Pts',(7.91842082599994,12.2,-7.12330369600001));
#172266=CARTESIAN_POINT('Ctrl Pts',(7.91715513599994,12.2,-7.12143404200001));
#172267=CARTESIAN_POINT('Ctrl Pts',(7.91589149199995,12.2,-7.11957094700002));
#172268=CARTESIAN_POINT('Ctrl Pts',(7.91462990899995,12.2,-7.11771441600002));
#172269=CARTESIAN_POINT('Ctrl Pts',(7.91337040399994,12.2,-7.11586445500001));
#172270=CARTESIAN_POINT('Ctrl Pts',(7.91211299299994,12.2,-7.11402106900002));
#172271=CARTESIAN_POINT('Ctrl Pts',(7.91085769199994,12.2,-7.11218426400002));
#172272=CARTESIAN_POINT('Ctrl Pts',(7.90960451799994,12.2,-7.11035404400001));
#172273=CARTESIAN_POINT('Ctrl Pts',(7.90835348799995,12.2,-7.10853041700001));
#172274=CARTESIAN_POINT('Ctrl Pts',(7.90710461699994,12.2,-7.10671338500001));
#172275=CARTESIAN_POINT('Ctrl Pts',(7.90585792199994,12.2,-7.10490295600002));
#172276=CARTESIAN_POINT('Ctrl Pts',(7.90461341899995,12.2,-7.10309913500001));
#172277=CARTESIAN_POINT('Ctrl Pts',(7.90337112499994,12.2,-7.10130192600002));
#172278=CARTESIAN_POINT('Ctrl Pts',(7.90213105799995,12.2,-7.09951133600002));
#172279=CARTESIAN_POINT('Ctrl Pts',(7.90089323199994,12.2,-7.09772736900002));
#172280=CARTESIAN_POINT('Ctrl Pts',(7.89965766699994,12.2,-7.09595003100001));
#172281=CARTESIAN_POINT('Ctrl Pts',(7.89842437699994,12.2,-7.09417932900001));
#172282=CARTESIAN_POINT('Ctrl Pts',(7.89719338099995,12.2,-7.09241526600002));
#172283=CARTESIAN_POINT('Ctrl Pts',(7.89596469399994,12.2,-7.09065784900002));
#172284=CARTESIAN_POINT('Ctrl Pts',(7.89473833399994,12.2,-7.08890708300002));
#172285=CARTESIAN_POINT('Ctrl Pts',(7.89351431799994,12.2,-7.08716297200001));
#172286=CARTESIAN_POINT('Ctrl Pts',(7.89229266299994,12.2,-7.08542552500001));
#172287=CARTESIAN_POINT('Ctrl Pts',(7.89107338599995,12.2,-7.08369474300002));
#172288=CARTESIAN_POINT('Ctrl Pts',(7.88985650599995,12.2,-7.08197063500001));
#172289=CARTESIAN_POINT('Ctrl Pts',(7.88864203699994,12.2,-7.08025320500001));
#172290=CARTESIAN_POINT('Ctrl Pts',(7.88742999899994,12.2,-7.07854245900001));
#172291=CARTESIAN_POINT('Ctrl Pts',(7.88622040799994,12.2,-7.07683840200002));
#172292=CARTESIAN_POINT('Ctrl Pts',(7.88501328299994,12.2,-7.07514104000002));
#172293=CARTESIAN_POINT('Ctrl Pts',(7.88380863899994,12.2,-7.07345037800001));
#172294=CARTESIAN_POINT('Ctrl Pts',(7.88260649599994,12.2,-7.07176642200002));
#172295=CARTESIAN_POINT('Ctrl Pts',(7.88140687099995,12.2,-7.07008917700002));
#172296=CARTESIAN_POINT('Ctrl Pts',(7.88020978099994,12.2,-7.06841865000002));
#172297=CARTESIAN_POINT('Ctrl Pts',(7.87901524399994,12.2,-7.06675484400002));
#172298=CARTESIAN_POINT('Ctrl Pts',(7.87782327799994,12.2,-7.06509776600001));
#172299=CARTESIAN_POINT('Ctrl Pts',(7.87663390099994,12.2,-7.06344742200002));
#172300=CARTESIAN_POINT('Ctrl Pts',(7.87544713199994,12.2,-7.06180381500002));
#172301=CARTESIAN_POINT('Ctrl Pts',(7.87426298699994,12.2,-7.06016695500002));
#172302=CARTESIAN_POINT('Ctrl Pts',(7.87308148499994,12.2,-7.05853684400001));
#172303=CARTESIAN_POINT('Ctrl Pts',(7.87190264399995,12.2,-7.05691348900002));
#172304=CARTESIAN_POINT('Ctrl Pts',(7.87072648199994,12.2,-7.05529689500001));
#172305=CARTESIAN_POINT('Ctrl Pts',(7.86955301799994,12.2,-7.05368706700002));
#172306=CARTESIAN_POINT('Ctrl Pts',(7.86838226999994,12.2,-7.05208401300002));
#172307=CARTESIAN_POINT('Ctrl Pts',(7.86721425699994,12.2,-7.05048773600002));
#172308=CARTESIAN_POINT('Ctrl Pts',(7.86604899599994,12.2,-7.04889824300002));
#172309=CARTESIAN_POINT('Ctrl Pts',(7.86488650699994,12.2,-7.04731553900002));
#172310=CARTESIAN_POINT('Ctrl Pts',(7.86372680699994,12.2,-7.04573963100002));
#172311=CARTESIAN_POINT('Ctrl Pts',(7.86256991599994,12.2,-7.04417052200002));
#172312=CARTESIAN_POINT('Ctrl Pts',(7.86141585299994,12.2,-7.04260821900001));
#172313=CARTESIAN_POINT('Ctrl Pts',(7.86026463599995,12.2,-7.04105272900001));
#172314=CARTESIAN_POINT('Ctrl Pts',(7.85911628399995,12.2,-7.03950405600001));
#172315=CARTESIAN_POINT('Ctrl Pts',(7.85797081499994,12.2,-7.03796220700001));
#172316=CARTESIAN_POINT('Ctrl Pts',(7.85682825099994,12.2,-7.03642718500002));
#172317=CARTESIAN_POINT('Ctrl Pts',(7.85568860799994,12.2,-7.03489899900001));
#172318=CARTESIAN_POINT('Ctrl Pts',(7.85455190599994,12.2,-7.03337765200001));
#172319=CARTESIAN_POINT('Ctrl Pts',(7.85341816499994,12.2,-7.03186315100002));
#172320=CARTESIAN_POINT('Ctrl Pts',(7.85228740299994,12.2,-7.03035550200001));
#172321=CARTESIAN_POINT('Ctrl Pts',(7.85115964099995,12.2,-7.02885471000001));
#172322=CARTESIAN_POINT('Ctrl Pts',(7.85003489699994,12.2,-7.02736078100001));
#172323=CARTESIAN_POINT('Ctrl Pts',(7.84891319099994,12.2,-7.02587372100002));
#172324=CARTESIAN_POINT('Ctrl Pts',(7.84779454299994,12.2,-7.02439353600001));
#172325=CARTESIAN_POINT('Ctrl Pts',(7.84667897299994,12.2,-7.02292023000001));
#172326=CARTESIAN_POINT('Ctrl Pts',(7.84556649899995,12.2,-7.02145381000002));
#172327=CARTESIAN_POINT('Ctrl Pts',(7.84445714199994,12.2,-7.01999428200001));
#172328=CARTESIAN_POINT('Ctrl Pts',(7.84335092199994,12.2,-7.01854165200002));
#172329=CARTESIAN_POINT('Ctrl Pts',(7.84224785899994,12.2,-7.01709592400002));
#172330=CARTESIAN_POINT('Ctrl Pts',(7.84114797199994,12.2,-7.01565710600002));
#172331=CARTESIAN_POINT('Ctrl Pts',(7.84005128199994,12.2,-7.01422520300002));
#172332=CARTESIAN_POINT('Ctrl Pts',(7.83895780899994,12.2,-7.01280021900001));
#172333=CARTESIAN_POINT('Ctrl Pts',(7.83786757299994,12.2,-7.01138216400001));
#172334=CARTESIAN_POINT('Ctrl Pts',(7.83656319944734,12.2,-7.00968881406154));
#172335=CARTESIAN_POINT('Ctrl Pts',(7.83526374289428,12.2,-7.00800587412212));
#172336=CARTESIAN_POINT('Ctrl Pts',(7.83396924322319,12.2,-7.00633335002984));
#172337=CARTESIAN_POINT('Ctrl Pts',(7.83267974367058,12.2,-7.00467125709134));
#172338=CARTESIAN_POINT('Ctrl Pts',(7.83139528399994,12.2,-7.00301960700001));
#172339=CARTESIAN_POINT('Ctrl Pts',(7.83032828199994,12.2,-7.00165020000002));
#172340=CARTESIAN_POINT('Ctrl Pts',(7.82926468199994,12.2,-7.00028776600002));
#172341=CARTESIAN_POINT('Ctrl Pts',(7.82820450599995,12.2,-6.99893231100001));
#172342=CARTESIAN_POINT('Ctrl Pts',(7.82714777299995,12.2,-6.99758384000001));
#172343=CARTESIAN_POINT('Ctrl Pts',(7.82609450599994,12.2,-6.99624236100002));
#172344=CARTESIAN_POINT('Ctrl Pts',(7.82504472499994,12.2,-6.99490787800002));
#172345=CARTESIAN_POINT('Ctrl Pts',(7.82399845099994,12.2,-6.99358039900002));
#172346=CARTESIAN_POINT('Ctrl Pts',(7.82295570699994,12.2,-6.99225992800002));
#172347=CARTESIAN_POINT('Ctrl Pts',(7.82191651399994,12.2,-6.99094647200001));
#172348=CARTESIAN_POINT('Ctrl Pts',(7.82088089199994,12.2,-6.98964003700001));
#172349=CARTESIAN_POINT('Ctrl Pts',(7.81984886499994,12.2,-6.98834063000002));
#172350=CARTESIAN_POINT('Ctrl Pts',(7.81882045199994,12.2,-6.98704825400001));
#172351=CARTESIAN_POINT('Ctrl Pts',(7.81779567699994,12.2,-6.98576291700002));
#172352=CARTESIAN_POINT('Ctrl Pts',(7.81677456099994,12.2,-6.98448462500001));
#172353=CARTESIAN_POINT('Ctrl Pts',(7.81575712599994,12.2,-6.98321338300002));
#172354=CARTESIAN_POINT('Ctrl Pts',(7.81474339499994,12.2,-6.98194919900001));
#172355=CARTESIAN_POINT('Ctrl Pts',(7.81373338799995,12.2,-6.98069207700001));
#172356=CARTESIAN_POINT('Ctrl Pts',(7.81272712999994,12.2,-6.97944202400001));
#172357=CARTESIAN_POINT('Ctrl Pts',(7.81172464099994,12.2,-6.97819904500002));
#172358=CARTESIAN_POINT('Ctrl Pts',(7.81072594399994,12.2,-6.97696314800002));
#172359=CARTESIAN_POINT('Ctrl Pts',(7.80973106299995,12.2,-6.97573433800001));
#172360=CARTESIAN_POINT('Ctrl Pts',(7.80874001999995,12.2,-6.97451262100002));
#172361=CARTESIAN_POINT('Ctrl Pts',(7.80775283599994,12.2,-6.97329800400002));
#172362=CARTESIAN_POINT('Ctrl Pts',(7.80676953599994,12.2,-6.97209049100002));
#172363=CARTESIAN_POINT('Ctrl Pts',(7.80579014099994,12.2,-6.97089009000001));
#172364=CARTESIAN_POINT('Ctrl Pts',(7.80481467499994,12.2,-6.96969680700001));
#172365=CARTESIAN_POINT('Ctrl Pts',(7.80384316099994,12.2,-6.96851064800001));
#172366=CARTESIAN_POINT('Ctrl Pts',(7.80287562299995,12.2,-6.96733161900001));
#172367=CARTESIAN_POINT('Ctrl Pts',(7.80191208299994,12.2,-6.96615972600001));
#172368=CARTESIAN_POINT('Ctrl Pts',(7.80095256499994,12.2,-6.96499497500002));
#172369=CARTESIAN_POINT('Ctrl Pts',(7.79999709199994,12.2,-6.96383737300001));
#172370=CARTESIAN_POINT('Ctrl Pts',(7.79904568799994,12.2,-6.96268692600002));
#172371=CARTESIAN_POINT('Ctrl Pts',(7.79809837699994,12.2,-6.96154364000002));
#172372=CARTESIAN_POINT('Ctrl Pts',(7.79715518199994,12.2,-6.96040752000001));
#172373=CARTESIAN_POINT('Ctrl Pts',(7.79621612699994,12.2,-6.95927857500001));
#172374=CARTESIAN_POINT('Ctrl Pts',(7.79528123699994,12.2,-6.95815681000001));
#172375=CARTESIAN_POINT('Ctrl Pts',(7.79435053399994,12.2,-6.95704223000002));
#172376=CARTESIAN_POINT('Ctrl Pts',(7.79342404399994,12.2,-6.95593484200002));
#172377=CARTESIAN_POINT('Ctrl Pts',(7.79250179099995,12.2,-6.95483465400001));
#172378=CARTESIAN_POINT('Ctrl Pts',(7.79158379899994,12.2,-6.95374167100002));
#172379=CARTESIAN_POINT('Ctrl Pts',(7.79067009299995,12.2,-6.95265589900002));
#172380=CARTESIAN_POINT('Ctrl Pts',(7.78976069699994,12.2,-6.95157734400001));
#172381=CARTESIAN_POINT('Ctrl Pts',(7.78885563499994,12.2,-6.95050601300002));
#172382=CARTESIAN_POINT('Ctrl Pts',(7.78795493299994,12.2,-6.94944191300002));
#172383=CARTESIAN_POINT('Ctrl Pts',(7.78705861699994,12.2,-6.94838504900002));
#172384=CARTESIAN_POINT('Ctrl Pts',(7.78616670899994,12.2,-6.94733542900002));
#172385=CARTESIAN_POINT('Ctrl Pts',(7.78527923799994,12.2,-6.94629305800002));
#172386=CARTESIAN_POINT('Ctrl Pts',(7.78439622499994,12.2,-6.94525794300001));
#172387=CARTESIAN_POINT('Ctrl Pts',(7.78351769799994,12.2,-6.94423009100002));
#172388=CARTESIAN_POINT('Ctrl Pts',(7.78264368299994,12.2,-6.94320950700002));
#172389=CARTESIAN_POINT('Ctrl Pts',(7.78177420299994,12.2,-6.94219620000001));
#172390=CARTESIAN_POINT('Ctrl Pts',(7.78090928599994,12.2,-6.94119017400002));
#172391=CARTESIAN_POINT('Ctrl Pts',(7.78004895599994,12.2,-6.94019143600002));
#172392=CARTESIAN_POINT('Ctrl Pts',(7.77919324199994,12.2,-6.93919999300002));
#172393=CARTESIAN_POINT('Ctrl Pts',(7.77834216699994,12.2,-6.93821585200002));
#172394=CARTESIAN_POINT('Ctrl Pts',(7.77749575799994,12.2,-6.93723901900002));
#172395=CARTESIAN_POINT('Ctrl Pts',(7.77665404199994,12.2,-6.93626950100001));
#172396=CARTESIAN_POINT('Ctrl Pts',(7.77581704399994,12.2,-6.93530730300001));
#172397=CARTESIAN_POINT('Ctrl Pts',(7.77498479199994,12.2,-6.93435243300002));
#172398=CARTESIAN_POINT('Ctrl Pts',(7.77415731199994,12.2,-6.93340489800002));
#172399=CARTESIAN_POINT('Ctrl Pts',(7.77333463099994,12.2,-6.93246470300001));
#172400=CARTESIAN_POINT('Ctrl Pts',(7.77251677499994,12.2,-6.93153185600002));
#172401=CARTESIAN_POINT('Ctrl Pts',(7.77170377299995,12.2,-6.93060636300002));
#172402=CARTESIAN_POINT('Ctrl Pts',(7.77089564999994,12.2,-6.92968823200002));
#172403=CARTESIAN_POINT('Ctrl Pts',(7.77009243399994,12.2,-6.92877746800002));
#172404=CARTESIAN_POINT('Ctrl Pts',(7.76929415399994,12.2,-6.92787407800001));
#172405=CARTESIAN_POINT('Ctrl Pts',(7.76850083499995,12.2,-6.92697807000001));
#172406=CARTESIAN_POINT('Ctrl Pts',(7.76771250599994,12.2,-6.92608944900002));
#172407=CARTESIAN_POINT('Ctrl Pts',(7.76692919399995,12.2,-6.92520822300001));
#172408=CARTESIAN_POINT('Ctrl Pts',(7.76615092799994,12.2,-6.92433439700002));
#172409=CARTESIAN_POINT('Ctrl Pts',(7.76537773499994,12.2,-6.92346798200001));
#172410=CARTESIAN_POINT('Ctrl Pts',(7.76460964399995,12.2,-6.92260898000002));
#172411=CARTESIAN_POINT('Ctrl Pts',(7.76384668299994,12.2,-6.92175740000001));
#172412=CARTESIAN_POINT('Ctrl Pts',(7.76308887999994,12.2,-6.92091324900002));
#172413=CARTESIAN_POINT('Ctrl Pts',(7.76233626399994,12.2,-6.92007653400001));
#172414=CARTESIAN_POINT('Ctrl Pts',(7.76158886399994,12.2,-6.91924726000002));
#172415=CARTESIAN_POINT('Ctrl Pts',(7.76084670899994,12.2,-6.91842543600002));
#172416=CARTESIAN_POINT('Ctrl Pts',(7.76010982699994,12.2,-6.91761106900002));
#172417=CARTESIAN_POINT('Ctrl Pts',(7.75937824799994,12.2,-6.91680416500001));
#172418=CARTESIAN_POINT('Ctrl Pts',(7.75865200099994,12.2,-6.91600473000002));
#172419=CARTESIAN_POINT('Ctrl Pts',(7.75793111599994,12.2,-6.91521277400001));
#172420=CARTESIAN_POINT('Ctrl Pts',(7.75721561999994,12.2,-6.91442830100002));
#172421=CARTESIAN_POINT('Ctrl Pts',(7.75650554599994,12.2,-6.91365131900002));
#172422=CARTESIAN_POINT('Ctrl Pts',(7.75580092299994,12.2,-6.91288183500002));
#172423=CARTESIAN_POINT('Ctrl Pts',(7.75510177999994,12.2,-6.91211985800001));
#172424=CARTESIAN_POINT('Ctrl Pts',(7.75440814899994,12.2,-6.91136539200001));
#172425=CARTESIAN_POINT('Ctrl Pts',(7.75372005699994,12.2,-6.91061844600001));
#172426=CARTESIAN_POINT('Ctrl Pts',(7.75303753799994,12.2,-6.90987902600002));
#172427=CARTESIAN_POINT('Ctrl Pts',(7.75236061999995,12.2,-6.90914714000002));
#172428=CARTESIAN_POINT('Ctrl Pts',(7.75168933499994,12.2,-6.90842279600002));
#172429=CARTESIAN_POINT('Ctrl Pts',(7.75102371399995,12.2,-6.90770599900001));
#172430=CARTESIAN_POINT('Ctrl Pts',(7.75036378799994,12.2,-6.90699675800002));
#172431=CARTESIAN_POINT('Ctrl Pts',(7.74970958799994,12.2,-6.90629507900002));
#172432=CARTESIAN_POINT('Ctrl Pts',(7.74906114399994,12.2,-6.90560097000001));
#172433=CARTESIAN_POINT('Ctrl Pts',(7.74841849099994,12.2,-6.90491443800001));
#172434=CARTESIAN_POINT('Ctrl Pts',(7.74778165799995,12.2,-6.90423549000001));
#172435=CARTESIAN_POINT('Ctrl Pts',(7.74715431199994,12.2,-6.90356800200002));
#172436=CARTESIAN_POINT('Ctrl Pts',(7.74665780099994,12.2,-6.90304077600001));
#172437=CARTESIAN_POINT('Ctrl Pts',(7.74628892999995,12.2,-6.90264967000001));
#172438=CARTESIAN_POINT('Ctrl Pts',(7.74604536199995,12.2,-6.90239167400001));
#172439=CARTESIAN_POINT('Ctrl Pts',(7.74592563699994,12.2,-6.90226492000001));
#172440=CARTESIAN_POINT('Ctrl Pts',(7.74592563699994,15.2,-6.90226492000001));
#172441=CARTESIAN_POINT('Ctrl Pts',(7.74604536199995,15.2,-6.90239167400001));
#172442=CARTESIAN_POINT('Ctrl Pts',(7.74628892999995,15.2,-6.90264967000001));
#172443=CARTESIAN_POINT('Ctrl Pts',(7.74665780099994,15.2,-6.90304077600001));
#172444=CARTESIAN_POINT('Ctrl Pts',(7.74715431199994,15.2,-6.90356800200002));
#172445=CARTESIAN_POINT('Ctrl Pts',(7.74778165799995,15.2,-6.90423549000001));
#172446=CARTESIAN_POINT('Ctrl Pts',(7.74841849099994,15.2,-6.90491443800001));
#172447=CARTESIAN_POINT('Ctrl Pts',(7.74906114399994,15.2,-6.90560097000001));
#172448=CARTESIAN_POINT('Ctrl Pts',(7.74970958799994,15.2,-6.90629507900002));
#172449=CARTESIAN_POINT('Ctrl Pts',(7.75036378799994,15.2,-6.90699675800002));
#172450=CARTESIAN_POINT('Ctrl Pts',(7.75102371399995,15.2,-6.90770599900001));
#172451=CARTESIAN_POINT('Ctrl Pts',(7.75168933499994,15.2,-6.90842279600002));
#172452=CARTESIAN_POINT('Ctrl Pts',(7.75236061999995,15.2,-6.90914714000002));
#172453=CARTESIAN_POINT('Ctrl Pts',(7.75303753799994,15.2,-6.90987902600002));
#172454=CARTESIAN_POINT('Ctrl Pts',(7.75372005699994,15.2,-6.91061844600001));
#172455=CARTESIAN_POINT('Ctrl Pts',(7.75440814899994,15.2,-6.91136539200001));
#172456=CARTESIAN_POINT('Ctrl Pts',(7.75510177999994,15.2,-6.91211985800001));
#172457=CARTESIAN_POINT('Ctrl Pts',(7.75580092299994,15.2,-6.91288183500002));
#172458=CARTESIAN_POINT('Ctrl Pts',(7.75650554599994,15.2,-6.91365131900002));
#172459=CARTESIAN_POINT('Ctrl Pts',(7.75721561999994,15.2,-6.91442830100002));
#172460=CARTESIAN_POINT('Ctrl Pts',(7.75793111599994,15.2,-6.91521277400001));
#172461=CARTESIAN_POINT('Ctrl Pts',(7.75865200099994,15.2,-6.91600473000002));
#172462=CARTESIAN_POINT('Ctrl Pts',(7.75937824799994,15.2,-6.91680416500001));
#172463=CARTESIAN_POINT('Ctrl Pts',(7.76010982699994,15.2,-6.91761106900002));
#172464=CARTESIAN_POINT('Ctrl Pts',(7.76084670899994,15.2,-6.91842543600002));
#172465=CARTESIAN_POINT('Ctrl Pts',(7.76158886399994,15.2,-6.91924726000002));
#172466=CARTESIAN_POINT('Ctrl Pts',(7.76233626399994,15.2,-6.92007653400001));
#172467=CARTESIAN_POINT('Ctrl Pts',(7.76308887999994,15.2,-6.92091324900002));
#172468=CARTESIAN_POINT('Ctrl Pts',(7.76384668299994,15.2,-6.92175740000001));
#172469=CARTESIAN_POINT('Ctrl Pts',(7.76460964399995,15.2,-6.92260898000002));
#172470=CARTESIAN_POINT('Ctrl Pts',(7.76537773499994,15.2,-6.92346798200001));
#172471=CARTESIAN_POINT('Ctrl Pts',(7.76615092799994,15.2,-6.92433439700002));
#172472=CARTESIAN_POINT('Ctrl Pts',(7.76692919399995,15.2,-6.92520822300001));
#172473=CARTESIAN_POINT('Ctrl Pts',(7.76771250599994,15.2,-6.92608944900002));
#172474=CARTESIAN_POINT('Ctrl Pts',(7.76850083499995,15.2,-6.92697807000001));
#172475=CARTESIAN_POINT('Ctrl Pts',(7.76929415399994,15.2,-6.92787407800001));
#172476=CARTESIAN_POINT('Ctrl Pts',(7.77009243399994,15.2,-6.92877746800002));
#172477=CARTESIAN_POINT('Ctrl Pts',(7.77089564999994,15.2,-6.92968823200002));
#172478=CARTESIAN_POINT('Ctrl Pts',(7.77170377299995,15.2,-6.93060636300002));
#172479=CARTESIAN_POINT('Ctrl Pts',(7.77251677499994,15.2,-6.93153185600002));
#172480=CARTESIAN_POINT('Ctrl Pts',(7.77333463099994,15.2,-6.93246470300001));
#172481=CARTESIAN_POINT('Ctrl Pts',(7.77415731199994,15.2,-6.93340489800002));
#172482=CARTESIAN_POINT('Ctrl Pts',(7.77498479199994,15.2,-6.93435243300002));
#172483=CARTESIAN_POINT('Ctrl Pts',(7.77581704399994,15.2,-6.93530730300001));
#172484=CARTESIAN_POINT('Ctrl Pts',(7.77665404199994,15.2,-6.93626950100001));
#172485=CARTESIAN_POINT('Ctrl Pts',(7.77749575799994,15.2,-6.93723901900002));
#172486=CARTESIAN_POINT('Ctrl Pts',(7.77834216699994,15.2,-6.93821585200002));
#172487=CARTESIAN_POINT('Ctrl Pts',(7.77919324199994,15.2,-6.93919999300002));
#172488=CARTESIAN_POINT('Ctrl Pts',(7.78004895599994,15.2,-6.94019143600002));
#172489=CARTESIAN_POINT('Ctrl Pts',(7.78090928599994,15.2,-6.94119017400002));
#172490=CARTESIAN_POINT('Ctrl Pts',(7.78177420299994,15.2,-6.94219620000001));
#172491=CARTESIAN_POINT('Ctrl Pts',(7.78264368299994,15.2,-6.94320950700002));
#172492=CARTESIAN_POINT('Ctrl Pts',(7.78351769799994,15.2,-6.94423009100002));
#172493=CARTESIAN_POINT('Ctrl Pts',(7.78439622499994,15.2,-6.94525794300001));
#172494=CARTESIAN_POINT('Ctrl Pts',(7.78527923799994,15.2,-6.94629305800002));
#172495=CARTESIAN_POINT('Ctrl Pts',(7.78616670899994,15.2,-6.94733542900002));
#172496=CARTESIAN_POINT('Ctrl Pts',(7.78705861699994,15.2,-6.94838504900002));
#172497=CARTESIAN_POINT('Ctrl Pts',(7.78795493299994,15.2,-6.94944191300002));
#172498=CARTESIAN_POINT('Ctrl Pts',(7.78885563499994,15.2,-6.95050601300002));
#172499=CARTESIAN_POINT('Ctrl Pts',(7.78976069699994,15.2,-6.95157734400001));
#172500=CARTESIAN_POINT('Ctrl Pts',(7.79067009299995,15.2,-6.95265589900002));
#172501=CARTESIAN_POINT('Ctrl Pts',(7.79158379899994,15.2,-6.95374167100002));
#172502=CARTESIAN_POINT('Ctrl Pts',(7.79250179099995,15.2,-6.95483465400001));
#172503=CARTESIAN_POINT('Ctrl Pts',(7.79342404399994,15.2,-6.95593484200002));
#172504=CARTESIAN_POINT('Ctrl Pts',(7.79435053399994,15.2,-6.95704223000002));
#172505=CARTESIAN_POINT('Ctrl Pts',(7.79528123699994,15.2,-6.95815681000001));
#172506=CARTESIAN_POINT('Ctrl Pts',(7.79621612699994,15.2,-6.95927857500001));
#172507=CARTESIAN_POINT('Ctrl Pts',(7.79715518199994,15.2,-6.96040752000001));
#172508=CARTESIAN_POINT('Ctrl Pts',(7.79809837699994,15.2,-6.96154364000002));
#172509=CARTESIAN_POINT('Ctrl Pts',(7.79904568799994,15.2,-6.96268692600002));
#172510=CARTESIAN_POINT('Ctrl Pts',(7.79999709199994,15.2,-6.96383737300001));
#172511=CARTESIAN_POINT('Ctrl Pts',(7.80095256499994,15.2,-6.96499497500002));
#172512=CARTESIAN_POINT('Ctrl Pts',(7.80191208299994,15.2,-6.96615972600001));
#172513=CARTESIAN_POINT('Ctrl Pts',(7.80287562299995,15.2,-6.96733161900001));
#172514=CARTESIAN_POINT('Ctrl Pts',(7.80384316099994,15.2,-6.96851064800001));
#172515=CARTESIAN_POINT('Ctrl Pts',(7.80481467499994,15.2,-6.96969680700001));
#172516=CARTESIAN_POINT('Ctrl Pts',(7.80579014099994,15.2,-6.97089009000001));
#172517=CARTESIAN_POINT('Ctrl Pts',(7.80676953599994,15.2,-6.97209049100002));
#172518=CARTESIAN_POINT('Ctrl Pts',(7.80775283599994,15.2,-6.97329800400002));
#172519=CARTESIAN_POINT('Ctrl Pts',(7.80874001999995,15.2,-6.97451262100002));
#172520=CARTESIAN_POINT('Ctrl Pts',(7.80973106299995,15.2,-6.97573433800001));
#172521=CARTESIAN_POINT('Ctrl Pts',(7.81072594399994,15.2,-6.97696314800002));
#172522=CARTESIAN_POINT('Ctrl Pts',(7.81172464099994,15.2,-6.97819904500002));
#172523=CARTESIAN_POINT('Ctrl Pts',(7.81272712999994,15.2,-6.97944202400001));
#172524=CARTESIAN_POINT('Ctrl Pts',(7.81373338799995,15.2,-6.98069207700001));
#172525=CARTESIAN_POINT('Ctrl Pts',(7.81474339499994,15.2,-6.98194919900001));
#172526=CARTESIAN_POINT('Ctrl Pts',(7.81575712599994,15.2,-6.98321338300002));
#172527=CARTESIAN_POINT('Ctrl Pts',(7.81677456099994,15.2,-6.98448462500001));
#172528=CARTESIAN_POINT('Ctrl Pts',(7.81779567699994,15.2,-6.98576291700002));
#172529=CARTESIAN_POINT('Ctrl Pts',(7.81882045199994,15.2,-6.98704825400001));
#172530=CARTESIAN_POINT('Ctrl Pts',(7.81984886499994,15.2,-6.98834063000002));
#172531=CARTESIAN_POINT('Ctrl Pts',(7.82088089199994,15.2,-6.98964003700001));
#172532=CARTESIAN_POINT('Ctrl Pts',(7.82191651399994,15.2,-6.99094647200001));
#172533=CARTESIAN_POINT('Ctrl Pts',(7.82295570699994,15.2,-6.99225992800002));
#172534=CARTESIAN_POINT('Ctrl Pts',(7.82399845099994,15.2,-6.99358039900002));
#172535=CARTESIAN_POINT('Ctrl Pts',(7.82504472499994,15.2,-6.99490787800002));
#172536=CARTESIAN_POINT('Ctrl Pts',(7.82609450599994,15.2,-6.99624236100002));
#172537=CARTESIAN_POINT('Ctrl Pts',(7.82714777299995,15.2,-6.99758384000001));
#172538=CARTESIAN_POINT('Ctrl Pts',(7.82820450599995,15.2,-6.99893231100001));
#172539=CARTESIAN_POINT('Ctrl Pts',(7.82926468199994,15.2,-7.00028776600002));
#172540=CARTESIAN_POINT('Ctrl Pts',(7.83032828199994,15.2,-7.00165020000002));
#172541=CARTESIAN_POINT('Ctrl Pts',(7.83139528399994,15.2,-7.00301960700001));
#172542=CARTESIAN_POINT('Ctrl Pts',(7.83267974366995,15.2,-7.00467125709003));
#172543=CARTESIAN_POINT('Ctrl Pts',(7.83396924322351,15.2,-7.0063333500305));
#172544=CARTESIAN_POINT('Ctrl Pts',(7.83526374289397,15.2,-7.00800587412146));
#172545=CARTESIAN_POINT('Ctrl Pts',(7.83656319944797,15.2,-7.00968881406286));
#172546=CARTESIAN_POINT('Ctrl Pts',(7.83786757299994,15.2,-7.01138216400001));
#172547=CARTESIAN_POINT('Ctrl Pts',(7.83895780899994,15.2,-7.01280021900001));
#172548=CARTESIAN_POINT('Ctrl Pts',(7.84005128199994,15.2,-7.01422520300002));
#172549=CARTESIAN_POINT('Ctrl Pts',(7.84114797199994,15.2,-7.01565710600002));
#172550=CARTESIAN_POINT('Ctrl Pts',(7.84224785899994,15.2,-7.01709592400002));
#172551=CARTESIAN_POINT('Ctrl Pts',(7.84335092199994,15.2,-7.01854165200002));
#172552=CARTESIAN_POINT('Ctrl Pts',(7.84445714199994,15.2,-7.01999428200001));
#172553=CARTESIAN_POINT('Ctrl Pts',(7.84556649899995,15.2,-7.02145381000002));
#172554=CARTESIAN_POINT('Ctrl Pts',(7.84667897299994,15.2,-7.02292023000001));
#172555=CARTESIAN_POINT('Ctrl Pts',(7.84779454299994,15.2,-7.02439353600001));
#172556=CARTESIAN_POINT('Ctrl Pts',(7.84891319099994,15.2,-7.02587372100002));
#172557=CARTESIAN_POINT('Ctrl Pts',(7.85003489699994,15.2,-7.02736078100001));
#172558=CARTESIAN_POINT('Ctrl Pts',(7.85115964099995,15.2,-7.02885471000001));
#172559=CARTESIAN_POINT('Ctrl Pts',(7.85228740299994,15.2,-7.03035550200001));
#172560=CARTESIAN_POINT('Ctrl Pts',(7.85341816499994,15.2,-7.03186315100002));
#172561=CARTESIAN_POINT('Ctrl Pts',(7.85455190599994,15.2,-7.03337765200001));
#172562=CARTESIAN_POINT('Ctrl Pts',(7.85568860799994,15.2,-7.03489899900001));
#172563=CARTESIAN_POINT('Ctrl Pts',(7.85682825099994,15.2,-7.03642718500002));
#172564=CARTESIAN_POINT('Ctrl Pts',(7.85797081499994,15.2,-7.03796220700001));
#172565=CARTESIAN_POINT('Ctrl Pts',(7.85911628399995,15.2,-7.03950405600001));
#172566=CARTESIAN_POINT('Ctrl Pts',(7.86026463599995,15.2,-7.04105272900001));
#172567=CARTESIAN_POINT('Ctrl Pts',(7.86141585299994,15.2,-7.04260821900001));
#172568=CARTESIAN_POINT('Ctrl Pts',(7.86256991599994,15.2,-7.04417052200002));
#172569=CARTESIAN_POINT('Ctrl Pts',(7.86372680699994,15.2,-7.04573963100002));
#172570=CARTESIAN_POINT('Ctrl Pts',(7.86488650699994,15.2,-7.04731553900002));
#172571=CARTESIAN_POINT('Ctrl Pts',(7.86604899599994,15.2,-7.04889824300002));
#172572=CARTESIAN_POINT('Ctrl Pts',(7.86721425699994,15.2,-7.05048773600002));
#172573=CARTESIAN_POINT('Ctrl Pts',(7.86838226999994,15.2,-7.05208401300002));
#172574=CARTESIAN_POINT('Ctrl Pts',(7.86955301799994,15.2,-7.05368706700002));
#172575=CARTESIAN_POINT('Ctrl Pts',(7.87072648199994,15.2,-7.05529689500001));
#172576=CARTESIAN_POINT('Ctrl Pts',(7.87190264399995,15.2,-7.05691348900002));
#172577=CARTESIAN_POINT('Ctrl Pts',(7.87308148499994,15.2,-7.05853684400001));
#172578=CARTESIAN_POINT('Ctrl Pts',(7.87426298699994,15.2,-7.06016695500002));
#172579=CARTESIAN_POINT('Ctrl Pts',(7.87544713199994,15.2,-7.06180381500002));
#172580=CARTESIAN_POINT('Ctrl Pts',(7.87663390099994,15.2,-7.06344742200002));
#172581=CARTESIAN_POINT('Ctrl Pts',(7.87782327799994,15.2,-7.06509776600001));
#172582=CARTESIAN_POINT('Ctrl Pts',(7.87901524399994,15.2,-7.06675484400002));
#172583=CARTESIAN_POINT('Ctrl Pts',(7.88020978099994,15.2,-7.06841865000002));
#172584=CARTESIAN_POINT('Ctrl Pts',(7.88140687099995,15.2,-7.07008917700002));
#172585=CARTESIAN_POINT('Ctrl Pts',(7.88260649599994,15.2,-7.07176642200002));
#172586=CARTESIAN_POINT('Ctrl Pts',(7.88380863899994,15.2,-7.07345037800001));
#172587=CARTESIAN_POINT('Ctrl Pts',(7.88501328299994,15.2,-7.07514104000002));
#172588=CARTESIAN_POINT('Ctrl Pts',(7.88622040799994,15.2,-7.07683840200002));
#172589=CARTESIAN_POINT('Ctrl Pts',(7.88742999899994,15.2,-7.07854245900001));
#172590=CARTESIAN_POINT('Ctrl Pts',(7.88864203699994,15.2,-7.08025320500001));
#172591=CARTESIAN_POINT('Ctrl Pts',(7.88985650599995,15.2,-7.08197063500001));
#172592=CARTESIAN_POINT('Ctrl Pts',(7.89107338599995,15.2,-7.08369474300002));
#172593=CARTESIAN_POINT('Ctrl Pts',(7.89229266299994,15.2,-7.08542552500001));
#172594=CARTESIAN_POINT('Ctrl Pts',(7.89351431799994,15.2,-7.08716297200001));
#172595=CARTESIAN_POINT('Ctrl Pts',(7.89473833399994,15.2,-7.08890708300002));
#172596=CARTESIAN_POINT('Ctrl Pts',(7.89596469399994,15.2,-7.09065784900002));
#172597=CARTESIAN_POINT('Ctrl Pts',(7.89719338099995,15.2,-7.09241526600002));
#172598=CARTESIAN_POINT('Ctrl Pts',(7.89842437699994,15.2,-7.09417932900001));
#172599=CARTESIAN_POINT('Ctrl Pts',(7.89965766699994,15.2,-7.09595003100001));
#172600=CARTESIAN_POINT('Ctrl Pts',(7.90089323199994,15.2,-7.09772736900002));
#172601=CARTESIAN_POINT('Ctrl Pts',(7.90213105799995,15.2,-7.09951133600002));
#172602=CARTESIAN_POINT('Ctrl Pts',(7.90337112499994,15.2,-7.10130192600002));
#172603=CARTESIAN_POINT('Ctrl Pts',(7.90461341899995,15.2,-7.10309913500001));
#172604=CARTESIAN_POINT('Ctrl Pts',(7.90585792199994,15.2,-7.10490295600002));
#172605=CARTESIAN_POINT('Ctrl Pts',(7.90710461699994,15.2,-7.10671338500001));
#172606=CARTESIAN_POINT('Ctrl Pts',(7.90835348799995,15.2,-7.10853041700001));
#172607=CARTESIAN_POINT('Ctrl Pts',(7.90960451799994,15.2,-7.11035404400001));
#172608=CARTESIAN_POINT('Ctrl Pts',(7.91085769199994,15.2,-7.11218426400002));
#172609=CARTESIAN_POINT('Ctrl Pts',(7.91211299299994,15.2,-7.11402106900002));
#172610=CARTESIAN_POINT('Ctrl Pts',(7.91337040399994,15.2,-7.11586445500001));
#172611=CARTESIAN_POINT('Ctrl Pts',(7.91462990899995,15.2,-7.11771441600002));
#172612=CARTESIAN_POINT('Ctrl Pts',(7.91589149199995,15.2,-7.11957094700002));
#172613=CARTESIAN_POINT('Ctrl Pts',(7.91715513599994,15.2,-7.12143404200001));
#172614=CARTESIAN_POINT('Ctrl Pts',(7.91842082599994,15.2,-7.12330369600001));
#172615=CARTESIAN_POINT('Ctrl Pts',(7.91968854599994,15.2,-7.12517990400002));
#172616=CARTESIAN_POINT('Ctrl Pts',(7.92095827899994,15.2,-7.12706266100002));
#172617=CARTESIAN_POINT('Ctrl Pts',(7.92223000999994,15.2,-7.12895196000002));
#172618=CARTESIAN_POINT('Ctrl Pts',(7.92350372299994,15.2,-7.13084779800001));
#172619=CARTESIAN_POINT('Ctrl Pts',(7.92477940099995,15.2,-7.13275016800001));
#172620=CARTESIAN_POINT('Ctrl Pts',(7.92605702899994,15.2,-7.13465906400002));
#172621=CARTESIAN_POINT('Ctrl Pts',(7.92733659099994,15.2,-7.13657448300002));
#172622=CARTESIAN_POINT('Ctrl Pts',(7.92861807299994,15.2,-7.13849641800002));
#172623=CARTESIAN_POINT('Ctrl Pts',(7.92990145699994,15.2,-7.14042486500002));
#172624=CARTESIAN_POINT('Ctrl Pts',(7.93118672799995,15.2,-7.14235981700002));
#172625=CARTESIAN_POINT('Ctrl Pts',(7.93247387099994,15.2,-7.14430127000002));
#172626=CARTESIAN_POINT('Ctrl Pts',(7.93376286999995,15.2,-7.14624921800001));
#172627=CARTESIAN_POINT('Ctrl Pts',(7.93505370999994,15.2,-7.14820365600002));
#172628=CARTESIAN_POINT('Ctrl Pts',(7.93634637499995,15.2,-7.15016457800001));
#172629=CARTESIAN_POINT('Ctrl Pts',(7.93764085099995,15.2,-7.15213198100002));
#172630=CARTESIAN_POINT('Ctrl Pts',(7.93893712099995,15.2,-7.15410585600001));
#172631=CARTESIAN_POINT('Ctrl Pts',(7.94023516999995,15.2,-7.15608620200002));
#172632=CARTESIAN_POINT('Ctrl Pts',(7.94153498399995,15.2,-7.15807301100002));
#172633=CARTESIAN_POINT('Ctrl Pts',(7.94283654599995,15.2,-7.16006627800001));
#172634=CARTESIAN_POINT('Ctrl Pts',(7.94413984299994,15.2,-7.16206599900002));
#172635=CARTESIAN_POINT('Ctrl Pts',(7.94544485899995,15.2,-7.16407216700001));
#172636=CARTESIAN_POINT('Ctrl Pts',(7.94675157799994,15.2,-7.16608477700002));
#172637=CARTESIAN_POINT('Ctrl Pts',(7.94805998699994,15.2,-7.16810382500002));
#172638=CARTESIAN_POINT('Ctrl Pts',(7.94937006899994,15.2,-7.17012930500001));
#172639=CARTESIAN_POINT('Ctrl Pts',(7.95068181099994,15.2,-7.17216121300002));
#172640=CARTESIAN_POINT('Ctrl Pts',(7.95199519599994,15.2,-7.17419954200002));
#172641=CARTESIAN_POINT('Ctrl Pts',(7.95331021099994,15.2,-7.17624428700002));
#172642=CARTESIAN_POINT('Ctrl Pts',(7.95462684099994,15.2,-7.17829544400002));
#172643=CARTESIAN_POINT('Ctrl Pts',(7.95594507099994,15.2,-7.18035300600001));
#172644=CARTESIAN_POINT('Ctrl Pts',(7.95726488599994,15.2,-7.18241697000002));
#172645=CARTESIAN_POINT('Ctrl Pts',(7.95858627199994,15.2,-7.18448732900002));
#172646=CARTESIAN_POINT('Ctrl Pts',(7.95990921399994,15.2,-7.18656407900002));
#172647=CARTESIAN_POINT('Ctrl Pts',(7.96123369799994,15.2,-7.18864721300001));
#172648=CARTESIAN_POINT('Ctrl Pts',(7.96255970799994,15.2,-7.19073672800001));
#172649=CARTESIAN_POINT('Ctrl Pts',(7.96388723099994,15.2,-7.19283261800002));
#172650=CARTESIAN_POINT('Ctrl Pts',(7.96521625299994,15.2,-7.19493487700002));
#172651=CARTESIAN_POINT('Ctrl Pts',(7.96654675899994,15.2,-7.19704350100002));
#172652=CARTESIAN_POINT('Ctrl Pts',(7.96787873499994,15.2,-7.19915848400002));
#172653=CARTESIAN_POINT('Ctrl Pts',(7.96921216599995,15.2,-7.20127982100002));
#172654=CARTESIAN_POINT('Ctrl Pts',(7.97054703699994,15.2,-7.20340750800001));
#172655=CARTESIAN_POINT('Ctrl Pts',(7.97188333599994,15.2,-7.20554153800002));
#172656=CARTESIAN_POINT('Ctrl Pts',(7.97322104799994,15.2,-7.20768190700002));
#172657=CARTESIAN_POINT('Ctrl Pts',(7.97456015899995,15.2,-7.20982861000002));
#172658=CARTESIAN_POINT('Ctrl Pts',(7.97590065499994,15.2,-7.21198164000001));
#172659=CARTESIAN_POINT('Ctrl Pts',(7.97724252099994,15.2,-7.21414099500001));
#172660=CARTESIAN_POINT('Ctrl Pts',(7.97858574299994,15.2,-7.21630666700002));
#172661=CARTESIAN_POINT('Ctrl Pts',(7.97993030999994,15.2,-7.21847865300001));
#172662=CARTESIAN_POINT('Ctrl Pts',(7.98127620499994,15.2,-7.22065694600002));
#172663=CARTESIAN_POINT('Ctrl Pts',(7.98262341399994,15.2,-7.22284154100001));
#172664=CARTESIAN_POINT('Ctrl Pts',(7.98397192599994,15.2,-7.22503243400002));
#172665=CARTESIAN_POINT('Ctrl Pts',(7.98532172499994,15.2,-7.22722962000002));
#172666=CARTESIAN_POINT('Ctrl Pts',(7.98667279799994,15.2,-7.22943309400002));
#172667=CARTESIAN_POINT('Ctrl Pts',(7.98802512999995,15.2,-7.23164284900002));
#172668=CARTESIAN_POINT('Ctrl Pts',(7.98937870999994,15.2,-7.23385888200001));
#172669=CARTESIAN_POINT('Ctrl Pts',(7.99073352199994,15.2,-7.23608118600002));
#172670=CARTESIAN_POINT('Ctrl Pts',(7.99208955399994,15.2,-7.23830975700002));
#172671=CARTESIAN_POINT('Ctrl Pts',(7.99344679099995,15.2,-7.24054459100002));
#172672=CARTESIAN_POINT('Ctrl Pts',(7.99480522199994,15.2,-7.24278568000001));
#172673=CARTESIAN_POINT('Ctrl Pts',(7.99616483099994,15.2,-7.24503302300001));
#172674=CARTESIAN_POINT('Ctrl Pts',(7.99752560499994,15.2,-7.24728661100002));
#172675=CARTESIAN_POINT('Ctrl Pts',(7.99888753099995,15.2,-7.24954644100002));
#172676=CARTESIAN_POINT('Ctrl Pts',(8.00025059599994,15.2,-7.25181250700001));
#172677=CARTESIAN_POINT('Ctrl Pts',(8.00161478799994,15.2,-7.25408480400001));
#172678=CARTESIAN_POINT('Ctrl Pts',(8.00298009099994,15.2,-7.25636332800002));
#172679=CARTESIAN_POINT('Ctrl Pts',(8.00434649299994,15.2,-7.25864807300002));
#172680=CARTESIAN_POINT('Ctrl Pts',(8.00571398099994,15.2,-7.26093903400002));
#172681=CARTESIAN_POINT('Ctrl Pts',(8.00708254199994,15.2,-7.26323620600001));
#172682=CARTESIAN_POINT('Ctrl Pts',(8.00845216399994,15.2,-7.26553958500002));
#172683=CARTESIAN_POINT('Ctrl Pts',(8.00982282999994,15.2,-7.26784916400002));
#172684=CARTESIAN_POINT('Ctrl Pts',(8.01119453199994,15.2,-7.27016493800001));
#172685=CARTESIAN_POINT('Ctrl Pts',(8.01256725299995,15.2,-7.27248690400002));
#172686=CARTESIAN_POINT('Ctrl Pts',(8.01394098199994,15.2,-7.27481505600001));
#172687=CARTESIAN_POINT('Ctrl Pts',(8.01531570699994,15.2,-7.27714938900001));
#172688=CARTESIAN_POINT('Ctrl Pts',(8.01669141199995,15.2,-7.27948989700002));
#172689=CARTESIAN_POINT('Ctrl Pts',(8.01806808699994,15.2,-7.28183657500002));
#172690=CARTESIAN_POINT('Ctrl Pts',(8.01944571799994,15.2,-7.28418941900002));
#172691=CARTESIAN_POINT('Ctrl Pts',(8.02082429299994,15.2,-7.28654842400001));
#172692=CARTESIAN_POINT('Ctrl Pts',(8.02220379799994,15.2,-7.28891358600002));
#172693=CARTESIAN_POINT('Ctrl Pts',(8.02358422099994,15.2,-7.29128489700001));
#172694=CARTESIAN_POINT('Ctrl Pts',(8.02496554899994,15.2,-7.29366235400001));
#172695=CARTESIAN_POINT('Ctrl Pts',(8.02634777099994,15.2,-7.29604595200002));
#172696=CARTESIAN_POINT('Ctrl Pts',(8.02773087299994,15.2,-7.29843568400002));
#172697=CARTESIAN_POINT('Ctrl Pts',(8.02911484199995,15.2,-7.30083154700001));
#172698=CARTESIAN_POINT('Ctrl Pts',(8.03049966599995,15.2,-7.30323353700002));
#172699=CARTESIAN_POINT('Ctrl Pts',(8.03188533199994,15.2,-7.30564164600001));
#172700=CARTESIAN_POINT('Ctrl Pts',(8.03327182899995,15.2,-7.30805587200001));
#172701=CARTESIAN_POINT('Ctrl Pts',(8.03465914399995,15.2,-7.31047620700001));
#172702=CARTESIAN_POINT('Ctrl Pts',(8.03604726399995,15.2,-7.31290264900001));
#172703=CARTESIAN_POINT('Ctrl Pts',(8.03743617699994,15.2,-7.31533519100001));
#172704=CARTESIAN_POINT('Ctrl Pts',(8.03882586899995,15.2,-7.31777382800002));
#172705=CARTESIAN_POINT('Ctrl Pts',(8.04021633199994,15.2,-7.32021855600002));
#172706=CARTESIAN_POINT('Ctrl Pts',(8.04160754999995,15.2,-7.32266936900002));
#172707=CARTESIAN_POINT('Ctrl Pts',(8.04299951199994,15.2,-7.32512626400001));
#172708=CARTESIAN_POINT('Ctrl Pts',(8.04439220499994,15.2,-7.32758923400001));
#172709=CARTESIAN_POINT('Ctrl Pts',(8.04578561899995,15.2,-7.33005827400002));
#172710=CARTESIAN_POINT('Ctrl Pts',(8.04717973999994,15.2,-7.33253338100001));
#172711=CARTESIAN_POINT('Ctrl Pts',(8.04857455599995,15.2,-7.33501454700002));
#172712=CARTESIAN_POINT('Ctrl Pts',(8.04997005499994,15.2,-7.33750177000001));
#172713=CARTESIAN_POINT('Ctrl Pts',(8.05136622599994,15.2,-7.33999504400002));
#172714=CARTESIAN_POINT('Ctrl Pts',(8.05276305599994,15.2,-7.34249436400002));
#172715=CARTESIAN_POINT('Ctrl Pts',(8.05416053399994,15.2,-7.34499972400001));
#172716=CARTESIAN_POINT('Ctrl Pts',(8.05555864699994,15.2,-7.34751112100002));
#172717=CARTESIAN_POINT('Ctrl Pts',(8.05695738399994,15.2,-7.35002854800002));
#172718=CARTESIAN_POINT('Ctrl Pts',(8.05835673199994,15.2,-7.35255200200001));
#172719=CARTESIAN_POINT('Ctrl Pts',(8.05975667999994,15.2,-7.35508147600001));
#172720=CARTESIAN_POINT('Ctrl Pts',(8.06115721599994,15.2,-7.35761696800001));
#172721=CARTESIAN_POINT('Ctrl Pts',(8.06255832899994,15.2,-7.36015847000001));
#172722=CARTESIAN_POINT('Ctrl Pts',(8.06396000599995,15.2,-7.36270597800001));
#172723=CARTESIAN_POINT('Ctrl Pts',(8.06536223699995,15.2,-7.36525948800002));
#172724=CARTESIAN_POINT('Ctrl Pts',(8.06676500799994,15.2,-7.36781899400002));
#172725=CARTESIAN_POINT('Ctrl Pts',(8.06816830899994,15.2,-7.37038449300002));
#172726=CARTESIAN_POINT('Ctrl Pts',(8.06957212799994,15.2,-7.37295597700002));
#172727=CARTESIAN_POINT('Ctrl Pts',(8.07097645399995,15.2,-7.37553344300002));
#172728=CARTESIAN_POINT('Ctrl Pts',(8.07238127399994,15.2,-7.37811688600001));
#172729=CARTESIAN_POINT('Ctrl Pts',(8.07378657799994,15.2,-7.38070630100002));
#172730=CARTESIAN_POINT('Ctrl Pts',(8.07519235299995,15.2,-7.38330168300001));
#172731=CARTESIAN_POINT('Ctrl Pts',(8.07659858999994,15.2,-7.38590302700001));
#172732=CARTESIAN_POINT('Ctrl Pts',(8.07800527499994,15.2,-7.38851032800002));
#172733=CARTESIAN_POINT('Ctrl Pts',(8.07941239799994,15.2,-7.39112358100002));
#172734=CARTESIAN_POINT('Ctrl Pts',(8.08081994599995,15.2,-7.39374278100002));
#172735=CARTESIAN_POINT('Ctrl Pts',(8.08222790999995,15.2,-7.39636792500002));
#172736=CARTESIAN_POINT('Ctrl Pts',(8.08363627799995,15.2,-7.39899900500002));
#172737=CARTESIAN_POINT('Ctrl Pts',(8.08504503799995,15.2,-7.40163601800001));
#172738=CARTESIAN_POINT('Ctrl Pts',(8.08645417899994,15.2,-7.40427895900002));
#172739=CARTESIAN_POINT('Ctrl Pts',(8.08786368899994,15.2,-7.40692782200002));
#172740=CARTESIAN_POINT('Ctrl Pts',(8.08927355799994,15.2,-7.40958260500002));
#172741=CARTESIAN_POINT('Ctrl Pts',(8.09068377599995,15.2,-7.41224329900002));
#172742=CARTESIAN_POINT('Ctrl Pts',(8.09209432999995,15.2,-7.41490990200001));
#172743=CARTESIAN_POINT('Ctrl Pts',(8.09350520799994,15.2,-7.41758240800002));
#172744=CARTESIAN_POINT('Ctrl Pts',(8.09491640099994,15.2,-7.42026081400001));
#172745=CARTESIAN_POINT('Ctrl Pts',(8.09632789799995,15.2,-7.42294511100001));
#172746=CARTESIAN_POINT('Ctrl Pts',(8.09773968599995,15.2,-7.42563529800002));
#172747=CARTESIAN_POINT('Ctrl Pts',(8.09915175599994,15.2,-7.42833136900002));
#172748=CARTESIAN_POINT('Ctrl Pts',(8.10056409499994,15.2,-7.43103331900001));
#172749=CARTESIAN_POINT('Ctrl Pts',(8.10197669399994,15.2,-7.43374114300002));
#172750=CARTESIAN_POINT('Ctrl Pts',(8.10338954199995,15.2,-7.43645483600002));
#172751=CARTESIAN_POINT('Ctrl Pts',(8.10480262699994,15.2,-7.43917439400001));
#172752=CARTESIAN_POINT('Ctrl Pts',(8.10621593799994,15.2,-7.44189981000002));
#172753=CARTESIAN_POINT('Ctrl Pts',(8.10762946499995,15.2,-7.44463108200001));
#172754=CARTESIAN_POINT('Ctrl Pts',(8.10904319799995,15.2,-7.44736820300002));
#172755=CARTESIAN_POINT('Ctrl Pts',(8.11045712499994,15.2,-7.45011117000002));
#172756=CARTESIAN_POINT('Ctrl Pts',(8.11187123599994,15.2,-7.45285997600002));
#172757=CARTESIAN_POINT('Ctrl Pts',(8.11328551799994,15.2,-7.45561461800002));
#172758=CARTESIAN_POINT('Ctrl Pts',(8.11469996399994,15.2,-7.45837509000002));
#172759=CARTESIAN_POINT('Ctrl Pts',(8.11611456099994,15.2,-7.46114138700002));
#172760=CARTESIAN_POINT('Ctrl Pts',(8.11752929899994,15.2,-7.46391350600002));
#172761=CARTESIAN_POINT('Ctrl Pts',(8.11894416699994,15.2,-7.46669144000002));
#172762=CARTESIAN_POINT('Ctrl Pts',(8.12035915499994,15.2,-7.46947518500002));
#172763=CARTESIAN_POINT('Ctrl Pts',(8.12177425199994,15.2,-7.47226473600002));
#172764=CARTESIAN_POINT('Ctrl Pts',(8.12318944699994,15.2,-7.47506008900002));
#172765=CARTESIAN_POINT('Ctrl Pts',(8.12460473099994,15.2,-7.47786123800001));
#172766=CARTESIAN_POINT('Ctrl Pts',(8.12602009199994,15.2,-7.48066818000002));
#172767=CARTESIAN_POINT('Ctrl Pts',(8.12743552099995,15.2,-7.48348090800001));
#172768=CARTESIAN_POINT('Ctrl Pts',(8.12913410293823,15.2,-7.48686311867713));
#172769=CARTESIAN_POINT('Ctrl Pts',(8.1308327555308,15.2,-7.49025399816146));
#172770=CARTESIAN_POINT('Ctrl Pts',(8.13253145646909,15.2,-7.49365353183857));
#172771=CARTESIAN_POINT('Ctrl Pts',(8.13423018390736,15.2,-7.49706171201332));
#172772=CARTESIAN_POINT('Ctrl Pts',(8.13592892199994,15.2,-7.50047853100002));
#172773=CARTESIAN_POINT('Ctrl Pts',(8.13734453099995,15.2,-7.50333163200001));
#172774=CARTESIAN_POINT('Ctrl Pts',(8.13876012299995,15.2,-7.50619048100001));
#172775=CARTESIAN_POINT('Ctrl Pts',(8.14017569099994,15.2,-7.50905507500002));
#172776=CARTESIAN_POINT('Ctrl Pts',(8.14159122299994,15.2,-7.51192540700002));
#172777=CARTESIAN_POINT('Ctrl Pts',(8.14300670799994,15.2,-7.51480147300001));
#172778=CARTESIAN_POINT('Ctrl Pts',(8.14442213799994,15.2,-7.51768326800001));
#172779=CARTESIAN_POINT('Ctrl Pts',(8.14583750199994,15.2,-7.52057078700001));
#172780=CARTESIAN_POINT('Ctrl Pts',(8.14725278899994,15.2,-7.52346402700002));
#172781=CARTESIAN_POINT('Ctrl Pts',(8.14866798999994,15.2,-7.52636298000001));
#172782=CARTESIAN_POINT('Ctrl Pts',(8.15008309399994,15.2,-7.52926764500002));
#172783=CARTESIAN_POINT('Ctrl Pts',(8.15149809099994,15.2,-7.53217801400002));
#172784=CARTESIAN_POINT('Ctrl Pts',(8.15291297199994,15.2,-7.53509408200002));
#172785=CARTESIAN_POINT('Ctrl Pts',(8.15432772699995,15.2,-7.53801584800001));
#172786=CARTESIAN_POINT('Ctrl Pts',(8.15574234599995,15.2,-7.54094330400001));
#172787=CARTESIAN_POINT('Ctrl Pts',(8.15715681899994,15.2,-7.54387644600002));
#172788=CARTESIAN_POINT('Ctrl Pts',(8.15857113399994,15.2,-7.54681526900002));
#172789=CARTESIAN_POINT('Ctrl Pts',(8.15998528399994,15.2,-7.54975976900001));
#172790=CARTESIAN_POINT('Ctrl Pts',(8.16139925799994,15.2,-7.55270994000002));
#172791=CARTESIAN_POINT('Ctrl Pts',(8.16281304699995,15.2,-7.55566577800002));
#172792=CARTESIAN_POINT('Ctrl Pts',(8.16422663899995,15.2,-7.55862727900002));
#172793=CARTESIAN_POINT('Ctrl Pts',(8.16564002699995,15.2,-7.56159443600002));
#172794=CARTESIAN_POINT('Ctrl Pts',(8.16705319899994,15.2,-7.56456724700002));
#172795=CARTESIAN_POINT('Ctrl Pts',(8.16846614699994,15.2,-7.56754570500001));
#172796=CARTESIAN_POINT('Ctrl Pts',(8.16987885999995,15.2,-7.57052980700001));
#172797=CARTESIAN_POINT('Ctrl Pts',(8.17129132899994,15.2,-7.57351954600002));
#172798=CARTESIAN_POINT('Ctrl Pts',(8.17270354399994,15.2,-7.57651491900001));
#172799=CARTESIAN_POINT('Ctrl Pts',(8.17411549699994,15.2,-7.57951592200002));
#172800=CARTESIAN_POINT('Ctrl Pts',(8.17552717499994,15.2,-7.58252254800002));
#172801=CARTESIAN_POINT('Ctrl Pts',(8.17693857099994,15.2,-7.58553479300001));
#172802=CARTESIAN_POINT('Ctrl Pts',(8.17834967399994,15.2,-7.58855265300002));
#172803=CARTESIAN_POINT('Ctrl Pts',(8.17976047699995,15.2,-7.59157612300001));
#172804=CARTESIAN_POINT('Ctrl Pts',(8.18117096699994,15.2,-7.59460519700002));
#172805=CARTESIAN_POINT('Ctrl Pts',(8.18258113699994,15.2,-7.59763987300002));
#172806=CARTESIAN_POINT('Ctrl Pts',(8.18399097599994,15.2,-7.60068014400002));
#172807=CARTESIAN_POINT('Ctrl Pts',(8.18540047699994,15.2,-7.60372600500002));
#172808=CARTESIAN_POINT('Ctrl Pts',(8.18680962599995,15.2,-7.60677745200002));
#172809=CARTESIAN_POINT('Ctrl Pts',(8.18821841799994,15.2,-7.60983448100002));
#172810=CARTESIAN_POINT('Ctrl Pts',(8.18962684199994,15.2,-7.61289708700001));
#172811=CARTESIAN_POINT('Ctrl Pts',(8.19103488899994,15.2,-7.61596526400002));
#172812=CARTESIAN_POINT('Ctrl Pts',(8.19244254899994,15.2,-7.61903900800001));
#172813=CARTESIAN_POINT('Ctrl Pts',(8.19384981299994,15.2,-7.62211831500001));
#172814=CARTESIAN_POINT('Ctrl Pts',(8.19525667099994,15.2,-7.62520317900002));
#172815=CARTESIAN_POINT('Ctrl Pts',(8.19666311599994,15.2,-7.62829359600002));
#172816=CARTESIAN_POINT('Ctrl Pts',(8.19806913599994,15.2,-7.63138956100001));
#172817=CARTESIAN_POINT('Ctrl Pts',(8.19947472199994,15.2,-7.63449107000002));
#172818=CARTESIAN_POINT('Ctrl Pts',(8.20087986699994,15.2,-7.63759811700002));
#172819=CARTESIAN_POINT('Ctrl Pts',(8.20228455999995,15.2,-7.64071069900002));
#172820=CARTESIAN_POINT('Ctrl Pts',(8.20368879299994,15.2,-7.64382880900002));
#172821=CARTESIAN_POINT('Ctrl Pts',(8.20509255499994,15.2,-7.64695244500002));
#172822=CARTESIAN_POINT('Ctrl Pts',(8.20649583899994,15.2,-7.65008160000002));
#172823=CARTESIAN_POINT('Ctrl Pts',(8.20789863399994,15.2,-7.65321627000001));
#172824=CARTESIAN_POINT('Ctrl Pts',(8.20930093299994,15.2,-7.65635645100001));
#172825=CARTESIAN_POINT('Ctrl Pts',(8.21070272499994,15.2,-7.65950213700001));
#172826=CARTESIAN_POINT('Ctrl Pts',(8.21210400199995,15.2,-7.66265332400001));
#172827=CARTESIAN_POINT('Ctrl Pts',(8.21350475399995,15.2,-7.66581000700001));
#172828=CARTESIAN_POINT('Ctrl Pts',(8.21490497299994,15.2,-7.66897218200001));
#172829=CARTESIAN_POINT('Ctrl Pts',(8.21630465099994,15.2,-7.67213984300002));
#172830=CARTESIAN_POINT('Ctrl Pts',(8.21770377699995,15.2,-7.67531298700002));
#172831=CARTESIAN_POINT('Ctrl Pts',(8.21910234199994,15.2,-7.67849160900001));
#172832=CARTESIAN_POINT('Ctrl Pts',(8.22050033799994,15.2,-7.68167570200001));
#172833=CARTESIAN_POINT('Ctrl Pts',(8.22189775699995,15.2,-7.68486526400002));
#172834=CARTESIAN_POINT('Ctrl Pts',(8.22329458799994,15.2,-7.68806029000002));
#172835=CARTESIAN_POINT('Ctrl Pts',(8.22469082399994,15.2,-7.69126077300001));
#172836=CARTESIAN_POINT('Ctrl Pts',(8.22608645599994,15.2,-7.69446671100001));
#172837=CARTESIAN_POINT('Ctrl Pts',(8.22748147299994,15.2,-7.69767809800002));
#172838=CARTESIAN_POINT('Ctrl Pts',(8.22887586899994,15.2,-7.70089492900001));
#172839=CARTESIAN_POINT('Ctrl Pts',(8.23026963299995,15.2,-7.70411720200002));
#172840=CARTESIAN_POINT('Ctrl Pts',(8.23166275799995,15.2,-7.70734490700002));
#172841=CARTESIAN_POINT('Ctrl Pts',(8.23305523399994,15.2,-7.71057804500002));
#172842=CARTESIAN_POINT('Ctrl Pts',(8.23444705399995,15.2,-7.71381660700002));
#172843=CARTESIAN_POINT('Ctrl Pts',(8.23583820599995,15.2,-7.71706059100002));
#172844=CARTESIAN_POINT('Ctrl Pts',(8.23722868599994,15.2,-7.72030999100001));
#172845=CARTESIAN_POINT('Ctrl Pts',(8.23861848099994,15.2,-7.72356480200001));
#172846=CARTESIAN_POINT('Ctrl Pts',(8.24000758299994,15.2,-7.72682502200002));
#172847=CARTESIAN_POINT('Ctrl Pts',(8.24139598699994,15.2,-7.73009064300001));
#172848=CARTESIAN_POINT('Ctrl Pts',(8.24278367999994,15.2,-7.73336166100002));
#172849=CARTESIAN_POINT('Ctrl Pts',(8.24417065699994,15.2,-7.73663807300002));
#172850=CARTESIAN_POINT('Ctrl Pts',(8.24555690699994,15.2,-7.73991987300001));
#172851=CARTESIAN_POINT('Ctrl Pts',(8.24694242099994,15.2,-7.74320705700001));
#172852=CARTESIAN_POINT('Ctrl Pts',(8.24832719199994,15.2,-7.74649962000002));
#172853=CARTESIAN_POINT('Ctrl Pts',(8.24971121199994,15.2,-7.74979755600001));
#172854=CARTESIAN_POINT('Ctrl Pts',(8.25109447199995,15.2,-7.75310086400002));
#172855=CARTESIAN_POINT('Ctrl Pts',(8.25247696199994,15.2,-7.75640953400002));
#172856=CARTESIAN_POINT('Ctrl Pts',(8.25385867499994,15.2,-7.75972356600001));
#172857=CARTESIAN_POINT('Ctrl Pts',(8.25523960299994,15.2,-7.76304295400001));
#172858=CARTESIAN_POINT('Ctrl Pts',(8.25661973699994,15.2,-7.76636769200002));
#172859=CARTESIAN_POINT('Ctrl Pts',(8.25799906799995,15.2,-7.76969777700002));
#172860=CARTESIAN_POINT('Ctrl Pts',(8.25937758699994,15.2,-7.77303320300001));
#172861=CARTESIAN_POINT('Ctrl Pts',(8.26075528799995,15.2,-7.77637396700002));
#172862=CARTESIAN_POINT('Ctrl Pts',(8.26213216099994,15.2,-7.77972006200002));
#172863=CARTESIAN_POINT('Ctrl Pts',(8.26350819799995,15.2,-7.78307148500001));
#172864=CARTESIAN_POINT('Ctrl Pts',(8.26488339199994,15.2,-7.78642823100002));
#172865=CARTESIAN_POINT('Ctrl Pts',(8.26625773199994,15.2,-7.78979029600002));
#172866=CARTESIAN_POINT('Ctrl Pts',(8.26763121199994,15.2,-7.79315767400002));
#172867=CARTESIAN_POINT('Ctrl Pts',(8.26900382399994,15.2,-7.79653036100001));
#172868=CARTESIAN_POINT('Ctrl Pts',(8.27037555599994,15.2,-7.79990835200002));
#172869=CARTESIAN_POINT('Ctrl Pts',(8.27174640499994,15.2,-7.80329164300002));
#172870=CARTESIAN_POINT('Ctrl Pts',(8.27311635999994,15.2,-7.80668023000001));
#172871=CARTESIAN_POINT('Ctrl Pts',(8.27448541299994,15.2,-7.81007410700001));
#172872=CARTESIAN_POINT('Ctrl Pts',(8.27585355599994,15.2,-7.81347326900002));
#172873=CARTESIAN_POINT('Ctrl Pts',(8.27722078099994,15.2,-7.81687771200002));
#172874=CARTESIAN_POINT('Ctrl Pts',(8.27858707899994,15.2,-7.82028743300001));
#172875=CARTESIAN_POINT('Ctrl Pts',(8.27995244399995,15.2,-7.82370242500001));
#172876=CARTESIAN_POINT('Ctrl Pts',(8.28131686599994,15.2,-7.82712268400001));
#172877=CARTESIAN_POINT('Ctrl Pts',(8.28268033699995,15.2,-7.83054820600002));
#172878=CARTESIAN_POINT('Ctrl Pts',(8.28404284999994,15.2,-7.83397898500001));
#172879=CARTESIAN_POINT('Ctrl Pts',(8.28540439599994,15.2,-7.83741501800002));
#172880=CARTESIAN_POINT('Ctrl Pts',(8.28676496699994,15.2,-7.84085630000002));
#172881=CARTESIAN_POINT('Ctrl Pts',(8.28812455599994,15.2,-7.84430282500002));
#172882=CARTESIAN_POINT('Ctrl Pts',(8.28948315499994,15.2,-7.84775459000001));
#172883=CARTESIAN_POINT('Ctrl Pts',(8.29084075499994,15.2,-7.85121159100001));
#172884=CARTESIAN_POINT('Ctrl Pts',(8.29219734999995,15.2,-7.85467382100002));
#172885=CARTESIAN_POINT('Ctrl Pts',(8.29355293099994,15.2,-7.85814127700001));
#172886=CARTESIAN_POINT('Ctrl Pts',(8.29490748799994,15.2,-7.86161395500002));
#172887=CARTESIAN_POINT('Ctrl Pts',(8.29626101599995,15.2,-7.86509184700002));
#172888=CARTESIAN_POINT('Ctrl Pts',(8.29761350399994,15.2,-7.86857495200002));
#172889=CARTESIAN_POINT('Ctrl Pts',(8.29896494599994,15.2,-7.87206326300002));
#172890=CARTESIAN_POINT('Ctrl Pts',(8.30031533299995,15.2,-7.87555677500002));
#172891=CARTESIAN_POINT('Ctrl Pts',(8.30166465799994,15.2,-7.87905548500002));
#172892=CARTESIAN_POINT('Ctrl Pts',(8.30328256514116,15.2,-7.88326016964724));
#172893=CARTESIAN_POINT('Ctrl Pts',(8.30489885992934,15.2,-7.8874726366764));
#172894=CARTESIAN_POINT('Ctrl Pts',(8.30651352407055,15.2,-7.89169288132363));
#172895=CARTESIAN_POINT('Ctrl Pts',(8.30812654585873,15.2,-7.89592089135279));
#172896=CARTESIAN_POINT('Ctrl Pts',(8.30973790699994,15.2,-7.90015665600002));
#172897=CARTESIAN_POINT('Ctrl Pts',(8.31107958999995,15.2,-7.90369162500002));
#172898=CARTESIAN_POINT('Ctrl Pts',(8.31242014699994,15.2,-7.90723175400001));
#172899=CARTESIAN_POINT('Ctrl Pts',(8.31375956699994,15.2,-7.91077703500001));
#172900=CARTESIAN_POINT('Ctrl Pts',(8.31509784399995,15.2,-7.91432746600002));
#172901=CARTESIAN_POINT('Ctrl Pts',(8.31643496899994,15.2,-7.91788304100002));
#172902=CARTESIAN_POINT('Ctrl Pts',(8.31777093699994,15.2,-7.92144375600002));
#172903=CARTESIAN_POINT('Ctrl Pts',(8.31910574599994,15.2,-7.92500961100002));
#172904=CARTESIAN_POINT('Ctrl Pts',(8.32043939299994,15.2,-7.92858060400001));
#172905=CARTESIAN_POINT('Ctrl Pts',(8.32150538099994,15.2,-7.93144150700002));
#172906=CARTESIAN_POINT('Ctrl Pts',(8.32230434799994,15.2,-7.93358949600002));
#172907=CARTESIAN_POINT('Ctrl Pts',(8.32283676099994,15.2,-7.93502251600002));
#172908=CARTESIAN_POINT('Ctrl Pts',(8.32310290799994,15.2,-7.93573928300002));
#172909=CARTESIAN_POINT('Ctrl Pts',(7.01216898599994,15.2,-7.64657512400002));
#172910=CARTESIAN_POINT('Ctrl Pts',(7.01216898599994,11.6,-7.64657512400002));
#172911=CARTESIAN_POINT('Ctrl Pts',(7.01229743599994,15.2,-7.64669302600002));
#172912=CARTESIAN_POINT('Ctrl Pts',(7.01229743599994,11.6,-7.64669302600002));
#172913=CARTESIAN_POINT('Ctrl Pts',(7.01255888299994,15.2,-7.64693288600002));
#172914=CARTESIAN_POINT('Ctrl Pts',(7.01255888299994,11.6,-7.64693288600002));
#172915=CARTESIAN_POINT('Ctrl Pts',(7.01295521699994,15.2,-7.64729613400001));
#172916=CARTESIAN_POINT('Ctrl Pts',(7.01295521699994,11.6,-7.64729613400001));
#172917=CARTESIAN_POINT('Ctrl Pts',(7.01348947999994,15.2,-7.64778506600001));
#172918=CARTESIAN_POINT('Ctrl Pts',(7.01348947999994,11.6,-7.64778506600001));
#172919=CARTESIAN_POINT('Ctrl Pts',(7.01416585899994,15.2,-7.64840281600002));
#172920=CARTESIAN_POINT('Ctrl Pts',(7.01416585899994,11.6,-7.64840281600002));
#172921=CARTESIAN_POINT('Ctrl Pts',(7.01485382999994,15.2,-7.64902988900002));
#172922=CARTESIAN_POINT('Ctrl Pts',(7.01485382999994,11.6,-7.64902988900002));
#172923=CARTESIAN_POINT('Ctrl Pts',(7.01554946899994,15.2,-7.64966267400002));
#172924=CARTESIAN_POINT('Ctrl Pts',(7.01554946899994,11.6,-7.64966267400002));
#172925=CARTESIAN_POINT('Ctrl Pts',(7.01625276599994,15.2,-7.65030114000002));
#172926=CARTESIAN_POINT('Ctrl Pts',(7.01625276599994,11.6,-7.65030114000002));
#172927=CARTESIAN_POINT('Ctrl Pts',(7.01696371599994,15.2,-7.65094525300002));
#172928=CARTESIAN_POINT('Ctrl Pts',(7.01696371599994,11.6,-7.65094525300002));
#172929=CARTESIAN_POINT('Ctrl Pts',(7.01768230799994,15.2,-7.65159498400001));
#172930=CARTESIAN_POINT('Ctrl Pts',(7.01768230799994,11.6,-7.65159498400001));
#172931=CARTESIAN_POINT('Ctrl Pts',(7.01840853599994,15.2,-7.65225030200002));
#172932=CARTESIAN_POINT('Ctrl Pts',(7.01840853599994,11.6,-7.65225030200002));
#172933=CARTESIAN_POINT('Ctrl Pts',(7.01914239299994,15.2,-7.65291117500002));
#172934=CARTESIAN_POINT('Ctrl Pts',(7.01914239299994,11.6,-7.65291117500002));
#172935=CARTESIAN_POINT('Ctrl Pts',(7.01988386999994,15.2,-7.65357757300002));
#172936=CARTESIAN_POINT('Ctrl Pts',(7.01988386999994,11.6,-7.65357757300002));
#172937=CARTESIAN_POINT('Ctrl Pts',(7.02063295999994,15.2,-7.65424946400002));
#172938=CARTESIAN_POINT('Ctrl Pts',(7.02063295999994,11.6,-7.65424946400002));
#172939=CARTESIAN_POINT('Ctrl Pts',(7.02138965599994,15.2,-7.65492682000002));
#172940=CARTESIAN_POINT('Ctrl Pts',(7.02138965599994,11.6,-7.65492682000002));
#172941=CARTESIAN_POINT('Ctrl Pts',(7.02215394899994,15.2,-7.65560960700002));
#172942=CARTESIAN_POINT('Ctrl Pts',(7.02215394899994,11.6,-7.65560960700002));
#172943=CARTESIAN_POINT('Ctrl Pts',(7.02292583299994,15.2,-7.65629779800002));
#172944=CARTESIAN_POINT('Ctrl Pts',(7.02292583299994,11.6,-7.65629779800002));
#172945=CARTESIAN_POINT('Ctrl Pts',(7.02370529899994,15.2,-7.65699136200002));
#172946=CARTESIAN_POINT('Ctrl Pts',(7.02370529899994,11.6,-7.65699136200002));
#172947=CARTESIAN_POINT('Ctrl Pts',(7.02449234199994,15.2,-7.65769026900001));
#172948=CARTESIAN_POINT('Ctrl Pts',(7.02449234199994,11.6,-7.65769026900001));
#172949=CARTESIAN_POINT('Ctrl Pts',(7.02528695099994,15.2,-7.65839448900002));
#172950=CARTESIAN_POINT('Ctrl Pts',(7.02528695099994,11.6,-7.65839448900002));
#172951=CARTESIAN_POINT('Ctrl Pts',(7.02608912099994,15.2,-7.65910399200001));
#172952=CARTESIAN_POINT('Ctrl Pts',(7.02608912099994,11.6,-7.65910399200001));
#172953=CARTESIAN_POINT('Ctrl Pts',(7.02689884399994,15.2,-7.65981875000002));
#172954=CARTESIAN_POINT('Ctrl Pts',(7.02689884399994,11.6,-7.65981875000002));
#172955=CARTESIAN_POINT('Ctrl Pts',(7.02771611299994,15.2,-7.66053873300002));
#172956=CARTESIAN_POINT('Ctrl Pts',(7.02771611299994,11.6,-7.66053873300002));
#172957=CARTESIAN_POINT('Ctrl Pts',(7.02854091899995,15.2,-7.66126391100002));
#172958=CARTESIAN_POINT('Ctrl Pts',(7.02854091899995,11.6,-7.66126391100002));
#172959=CARTESIAN_POINT('Ctrl Pts',(7.02937325699994,15.2,-7.66199425500002));
#172960=CARTESIAN_POINT('Ctrl Pts',(7.02937325699994,11.6,-7.66199425500002));
#172961=CARTESIAN_POINT('Ctrl Pts',(7.03021311799994,15.2,-7.66272973700002));
#172962=CARTESIAN_POINT('Ctrl Pts',(7.03021311799994,11.6,-7.66272973700002));
#172963=CARTESIAN_POINT('Ctrl Pts',(7.03106049599994,15.2,-7.66347032800001));
#172964=CARTESIAN_POINT('Ctrl Pts',(7.03106049599994,11.6,-7.66347032800001));
#172965=CARTESIAN_POINT('Ctrl Pts',(7.03191538199994,15.2,-7.66421599900001));
#172966=CARTESIAN_POINT('Ctrl Pts',(7.03191538199994,11.6,-7.66421599900001));
#172967=CARTESIAN_POINT('Ctrl Pts',(7.03277776899994,15.2,-7.66496672300002));
#172968=CARTESIAN_POINT('Ctrl Pts',(7.03277776899994,11.6,-7.66496672300002));
#172969=CARTESIAN_POINT('Ctrl Pts',(7.03364765099994,15.2,-7.66572247000001));
#172970=CARTESIAN_POINT('Ctrl Pts',(7.03364765099994,11.6,-7.66572247000001));
#172971=CARTESIAN_POINT('Ctrl Pts',(7.03452502099994,15.2,-7.66648321100002));
#172972=CARTESIAN_POINT('Ctrl Pts',(7.03452502099994,11.6,-7.66648321100002));
#172973=CARTESIAN_POINT('Ctrl Pts',(7.03540986899994,15.2,-7.66724892000001));
#172974=CARTESIAN_POINT('Ctrl Pts',(7.03540986899994,11.6,-7.66724892000001));
#172975=CARTESIAN_POINT('Ctrl Pts',(7.03630218999994,15.2,-7.66801956900002));
#172976=CARTESIAN_POINT('Ctrl Pts',(7.03630218999994,11.6,-7.66801956900002));
#172977=CARTESIAN_POINT('Ctrl Pts',(7.03720197799995,15.2,-7.66879512800001));
#172978=CARTESIAN_POINT('Ctrl Pts',(7.03720197799995,11.6,-7.66879512800001));
#172979=CARTESIAN_POINT('Ctrl Pts',(7.03810922299994,15.2,-7.66957557200002));
#172980=CARTESIAN_POINT('Ctrl Pts',(7.03810922299994,11.6,-7.66957557200002));
#172981=CARTESIAN_POINT('Ctrl Pts',(7.03902391899994,15.2,-7.67036087200001));
#172982=CARTESIAN_POINT('Ctrl Pts',(7.03902391899994,11.6,-7.67036087200001));
#172983=CARTESIAN_POINT('Ctrl Pts',(7.03994605999994,15.2,-7.67115100000002));
#172984=CARTESIAN_POINT('Ctrl Pts',(7.03994605999994,11.6,-7.67115100000002));
#172985=CARTESIAN_POINT('Ctrl Pts',(7.04087563899994,15.2,-7.67194593000001));
#172986=CARTESIAN_POINT('Ctrl Pts',(7.04087563899994,11.6,-7.67194593000001));
#172987=CARTESIAN_POINT('Ctrl Pts',(7.04181264599994,15.2,-7.67274563400001));
#172988=CARTESIAN_POINT('Ctrl Pts',(7.04181264599994,11.6,-7.67274563400001));
#172989=CARTESIAN_POINT('Ctrl Pts',(7.04275707599994,15.2,-7.67355008500001));
#172990=CARTESIAN_POINT('Ctrl Pts',(7.04275707599994,11.6,-7.67355008500001));
#172991=CARTESIAN_POINT('Ctrl Pts',(7.04370892199995,15.2,-7.67435925700001));
#172992=CARTESIAN_POINT('Ctrl Pts',(7.04370892199995,11.6,-7.67435925700001));
#172993=CARTESIAN_POINT('Ctrl Pts',(7.04466817699994,15.2,-7.67517312200001));
#172994=CARTESIAN_POINT('Ctrl Pts',(7.04466817699994,11.6,-7.67517312200001));
#172995=CARTESIAN_POINT('Ctrl Pts',(7.04563483299994,15.2,-7.67599165500001));
#172996=CARTESIAN_POINT('Ctrl Pts',(7.04563483299994,11.6,-7.67599165500001));
#172997=CARTESIAN_POINT('Ctrl Pts',(7.04660888399994,15.2,-7.67681482700001));
#172998=CARTESIAN_POINT('Ctrl Pts',(7.04660888399994,11.6,-7.67681482700001));
#172999=CARTESIAN_POINT('Ctrl Pts',(7.04759032399994,15.2,-7.67764261300002));
#173000=CARTESIAN_POINT('Ctrl Pts',(7.04759032399994,11.6,-7.67764261300002));
#173001=CARTESIAN_POINT('Ctrl Pts',(7.04857914399994,15.2,-7.67847498700001));
#173002=CARTESIAN_POINT('Ctrl Pts',(7.04857914399994,11.6,-7.67847498700001));
#173003=CARTESIAN_POINT('Ctrl Pts',(7.04957533699995,15.2,-7.67931192200002));
#173004=CARTESIAN_POINT('Ctrl Pts',(7.04957533699995,11.6,-7.67931192200002));
#173005=CARTESIAN_POINT('Ctrl Pts',(7.05057889899994,15.2,-7.68015339300002));
#173006=CARTESIAN_POINT('Ctrl Pts',(7.05057889899994,11.6,-7.68015339300002));
#173007=CARTESIAN_POINT('Ctrl Pts',(7.05158981999995,15.2,-7.68099937300001));
#173008=CARTESIAN_POINT('Ctrl Pts',(7.05158981999995,11.6,-7.68099937300001));
#173009=CARTESIAN_POINT('Ctrl Pts',(7.05260809399994,15.2,-7.68184983700002));
#173010=CARTESIAN_POINT('Ctrl Pts',(7.05260809399994,11.6,-7.68184983700002));
#173011=CARTESIAN_POINT('Ctrl Pts',(7.05363371299994,15.2,-7.68270475700002));
#173012=CARTESIAN_POINT('Ctrl Pts',(7.05363371299994,11.6,-7.68270475700002));
#173013=CARTESIAN_POINT('Ctrl Pts',(7.05466667299994,15.2,-7.68356411000001));
#173014=CARTESIAN_POINT('Ctrl Pts',(7.05466667299994,11.6,-7.68356411000001));
#173015=CARTESIAN_POINT('Ctrl Pts',(7.05570696599994,15.2,-7.68442787000001));
#173016=CARTESIAN_POINT('Ctrl Pts',(7.05570696599994,11.6,-7.68442787000001));
#173017=CARTESIAN_POINT('Ctrl Pts',(7.05675458399995,15.2,-7.68529601200001));
#173018=CARTESIAN_POINT('Ctrl Pts',(7.05675458399995,11.6,-7.68529601200001));
#173019=CARTESIAN_POINT('Ctrl Pts',(7.05780952099994,15.2,-7.68616850900001));
#173020=CARTESIAN_POINT('Ctrl Pts',(7.05780952099994,11.6,-7.68616850900001));
#173021=CARTESIAN_POINT('Ctrl Pts',(7.05887177099994,15.2,-7.68704533700002));
#173022=CARTESIAN_POINT('Ctrl Pts',(7.05887177099994,11.6,-7.68704533700002));
#173023=CARTESIAN_POINT('Ctrl Pts',(7.05994132499994,15.2,-7.68792647200002));
#173024=CARTESIAN_POINT('Ctrl Pts',(7.05994132499994,11.6,-7.68792647200002));
#173025=CARTESIAN_POINT('Ctrl Pts',(7.06101817799994,15.2,-7.68881188600002));
#173026=CARTESIAN_POINT('Ctrl Pts',(7.06101817799994,11.6,-7.68881188600002));
#173027=CARTESIAN_POINT('Ctrl Pts',(7.06210232399994,15.2,-7.68970155800002));
#173028=CARTESIAN_POINT('Ctrl Pts',(7.06210232399994,11.6,-7.68970155800002));
#173029=CARTESIAN_POINT('Ctrl Pts',(7.06319375299994,15.2,-7.69059545900002));
#173030=CARTESIAN_POINT('Ctrl Pts',(7.06319375299994,11.6,-7.69059545900002));
#173031=CARTESIAN_POINT('Ctrl Pts',(7.06429246299995,15.2,-7.69149356800002));
#173032=CARTESIAN_POINT('Ctrl Pts',(7.06429246299995,11.6,-7.69149356800002));
#173033=CARTESIAN_POINT('Ctrl Pts',(7.06539844399994,15.2,-7.69239585900002));
#173034=CARTESIAN_POINT('Ctrl Pts',(7.06539844399994,11.6,-7.69239585900002));
#173035=CARTESIAN_POINT('Ctrl Pts',(7.06651168899994,15.2,-7.69330230800002));
#173036=CARTESIAN_POINT('Ctrl Pts',(7.06651168899994,11.6,-7.69330230800002));
#173037=CARTESIAN_POINT('Ctrl Pts',(7.06763219399994,15.2,-7.69421289100002));
#173038=CARTESIAN_POINT('Ctrl Pts',(7.06763219399994,11.6,-7.69421289100002));
#173039=CARTESIAN_POINT('Ctrl Pts',(7.06875994999994,15.2,-7.69512758300002));
#173040=CARTESIAN_POINT('Ctrl Pts',(7.06875994999994,11.6,-7.69512758300002));
#173041=CARTESIAN_POINT('Ctrl Pts',(7.06989495099994,15.2,-7.69604636000001));
#173042=CARTESIAN_POINT('Ctrl Pts',(7.06989495099994,11.6,-7.69604636000001));
#173043=CARTESIAN_POINT('Ctrl Pts',(7.07103718999995,15.2,-7.69696919900002));
#173044=CARTESIAN_POINT('Ctrl Pts',(7.07103718999995,11.6,-7.69696919900002));
#173045=CARTESIAN_POINT('Ctrl Pts',(7.07218666199994,15.2,-7.69789607500002));
#173046=CARTESIAN_POINT('Ctrl Pts',(7.07218666199994,11.6,-7.69789607500002));
#173047=CARTESIAN_POINT('Ctrl Pts',(7.07334335899994,15.2,-7.69882696300002));
#173048=CARTESIAN_POINT('Ctrl Pts',(7.07334335899994,11.6,-7.69882696300002));
#173049=CARTESIAN_POINT('Ctrl Pts',(7.07450727399995,15.2,-7.69976184200001));
#173050=CARTESIAN_POINT('Ctrl Pts',(7.07450727399995,11.6,-7.69976184200001));
#173051=CARTESIAN_POINT('Ctrl Pts',(7.07567840199994,15.2,-7.70070068800001));
#173052=CARTESIAN_POINT('Ctrl Pts',(7.07567840199994,11.6,-7.70070068800001));
#173053=CARTESIAN_POINT('Ctrl Pts',(7.07685673499994,15.2,-7.70164347600002));
#173054=CARTESIAN_POINT('Ctrl Pts',(7.07685673499994,11.6,-7.70164347600002));
#173055=CARTESIAN_POINT('Ctrl Pts',(7.07804226699994,15.2,-7.70259018400001));
#173056=CARTESIAN_POINT('Ctrl Pts',(7.07804226699994,11.6,-7.70259018400001));
#173057=CARTESIAN_POINT('Ctrl Pts',(7.07923499199994,15.2,-7.70354078700001));
#173058=CARTESIAN_POINT('Ctrl Pts',(7.07923499199994,11.6,-7.70354078700001));
#173059=CARTESIAN_POINT('Ctrl Pts',(7.08043490299994,15.2,-7.70449526500002));
#173060=CARTESIAN_POINT('Ctrl Pts',(7.08043490299994,11.6,-7.70449526500002));
#173061=CARTESIAN_POINT('Ctrl Pts',(7.08164199399994,15.2,-7.70545359200002));
#173062=CARTESIAN_POINT('Ctrl Pts',(7.08164199399994,11.6,-7.70545359200002));
#173063=CARTESIAN_POINT('Ctrl Pts',(7.08285625699994,15.2,-7.70641574500001));
#173064=CARTESIAN_POINT('Ctrl Pts',(7.08285625699994,11.6,-7.70641574500001));
#173065=CARTESIAN_POINT('Ctrl Pts',(7.08407768699994,15.2,-7.70738170300002));
#173066=CARTESIAN_POINT('Ctrl Pts',(7.08407768699994,11.6,-7.70738170300002));
#173067=CARTESIAN_POINT('Ctrl Pts',(7.08530627699994,15.2,-7.70835144200002));
#173068=CARTESIAN_POINT('Ctrl Pts',(7.08530627699994,11.6,-7.70835144200002));
#173069=CARTESIAN_POINT('Ctrl Pts',(7.08654202199994,15.2,-7.70932493900002));
#173070=CARTESIAN_POINT('Ctrl Pts',(7.08654202199994,11.6,-7.70932493900002));
#173071=CARTESIAN_POINT('Ctrl Pts',(7.08778491199994,15.2,-7.71030217200002));
#173072=CARTESIAN_POINT('Ctrl Pts',(7.08778491199994,11.6,-7.71030217200002));
#173073=CARTESIAN_POINT('Ctrl Pts',(7.08903494499994,15.2,-7.71128311800001));
#173074=CARTESIAN_POINT('Ctrl Pts',(7.08903494499994,11.6,-7.71128311800001));
#173075=CARTESIAN_POINT('Ctrl Pts',(7.09029211099995,15.2,-7.71226775600002));
#173076=CARTESIAN_POINT('Ctrl Pts',(7.09029211099995,11.6,-7.71226775600002));
#173077=CARTESIAN_POINT('Ctrl Pts',(7.09155640599994,15.2,-7.71325606100002));
#173078=CARTESIAN_POINT('Ctrl Pts',(7.09155640599994,11.6,-7.71325606100002));
#173079=CARTESIAN_POINT('Ctrl Pts',(7.09282782099995,15.2,-7.71424801400002));
#173080=CARTESIAN_POINT('Ctrl Pts',(7.09282782099995,11.6,-7.71424801400002));
#173081=CARTESIAN_POINT('Ctrl Pts',(7.09410635299994,15.2,-7.71524359000002));
#173082=CARTESIAN_POINT('Ctrl Pts',(7.09410635299994,11.6,-7.71524359000002));
#173083=CARTESIAN_POINT('Ctrl Pts',(7.09539199299994,15.2,-7.71624276900001));
#173084=CARTESIAN_POINT('Ctrl Pts',(7.09539199299994,11.6,-7.71624276900001));
#173085=CARTESIAN_POINT('Ctrl Pts',(7.09668473699994,15.2,-7.71724552700002));
#173086=CARTESIAN_POINT('Ctrl Pts',(7.09668473699994,11.6,-7.71724552700002));
#173087=CARTESIAN_POINT('Ctrl Pts',(7.09798457499994,15.2,-7.71825184400001));
#173088=CARTESIAN_POINT('Ctrl Pts',(7.09798457499994,11.6,-7.71825184400001));
#173089=CARTESIAN_POINT('Ctrl Pts',(7.09929150499994,15.2,-7.71926169700001));
#173090=CARTESIAN_POINT('Ctrl Pts',(7.09929150499994,11.6,-7.71926169700001));
#173091=CARTESIAN_POINT('Ctrl Pts',(7.10060551799994,15.2,-7.72027506500002));
#173092=CARTESIAN_POINT('Ctrl Pts',(7.10060551799994,11.6,-7.72027506500002));
#173093=CARTESIAN_POINT('Ctrl Pts',(7.10192660699994,15.2,-7.72129192600002));
#173094=CARTESIAN_POINT('Ctrl Pts',(7.10192660699994,11.6,-7.72129192600002));
#173095=CARTESIAN_POINT('Ctrl Pts',(7.10325476799994,15.2,-7.72231225700001));
#173096=CARTESIAN_POINT('Ctrl Pts',(7.10325476799994,11.6,-7.72231225700001));
#173097=CARTESIAN_POINT('Ctrl Pts',(7.10458999399994,15.2,-7.72333604000002));
#173098=CARTESIAN_POINT('Ctrl Pts',(7.10458999399994,11.6,-7.72333604000002));
#173099=CARTESIAN_POINT('Ctrl Pts',(7.10593227899994,15.2,-7.72436325100001));
#173100=CARTESIAN_POINT('Ctrl Pts',(7.10593227899994,11.6,-7.72436325100001));
#173101=CARTESIAN_POINT('Ctrl Pts',(7.10728161499994,15.2,-7.72539386900001));
#173102=CARTESIAN_POINT('Ctrl Pts',(7.10728161499994,11.6,-7.72539386900001));
#173103=CARTESIAN_POINT('Ctrl Pts',(7.10863799699994,15.2,-7.72642787400001));
#173104=CARTESIAN_POINT('Ctrl Pts',(7.10863799699994,11.6,-7.72642787400001));
#173105=CARTESIAN_POINT('Ctrl Pts',(7.11000141999994,15.2,-7.72746524300001));
#173106=CARTESIAN_POINT('Ctrl Pts',(7.11000141999994,11.6,-7.72746524300001));
#173107=CARTESIAN_POINT('Ctrl Pts',(7.11137187499994,15.2,-7.72850595600002));
#173108=CARTESIAN_POINT('Ctrl Pts',(7.11137187499994,11.6,-7.72850595600002));
#173109=CARTESIAN_POINT('Ctrl Pts',(7.11274935899994,15.2,-7.72954999200002));
#173110=CARTESIAN_POINT('Ctrl Pts',(7.11274935899994,11.6,-7.72954999200002));
#173111=CARTESIAN_POINT('Ctrl Pts',(7.11413386299995,15.2,-7.73059733100002));
#173112=CARTESIAN_POINT('Ctrl Pts',(7.11413386299995,11.6,-7.73059733100002));
#173113=CARTESIAN_POINT('Ctrl Pts',(7.11552538199994,15.2,-7.73164795100002));
#173114=CARTESIAN_POINT('Ctrl Pts',(7.11552538199994,11.6,-7.73164795100002));
#173115=CARTESIAN_POINT('Ctrl Pts',(7.11692391099994,15.2,-7.73270183100002));
#173116=CARTESIAN_POINT('Ctrl Pts',(7.11692391099994,11.6,-7.73270183100002));
#173117=CARTESIAN_POINT('Ctrl Pts',(7.11832944099994,15.2,-7.73375895200001));
#173118=CARTESIAN_POINT('Ctrl Pts',(7.11832944099994,11.6,-7.73375895200001));
#173119=CARTESIAN_POINT('Ctrl Pts',(7.11974196799994,15.2,-7.73481929100001));
#173120=CARTESIAN_POINT('Ctrl Pts',(7.11974196799994,11.6,-7.73481929100001));
#173121=CARTESIAN_POINT('Ctrl Pts',(7.12116148499994,15.2,-7.73588283000001));
#173122=CARTESIAN_POINT('Ctrl Pts',(7.12116148499994,11.6,-7.73588283000001));
#173123=CARTESIAN_POINT('Ctrl Pts',(7.12258798699994,15.2,-7.73694954800002));
#173124=CARTESIAN_POINT('Ctrl Pts',(7.12258798699994,11.6,-7.73694954800002));
#173125=CARTESIAN_POINT('Ctrl Pts',(7.12402146699994,15.2,-7.73801942300001));
#173126=CARTESIAN_POINT('Ctrl Pts',(7.12402146699994,11.6,-7.73801942300001));
#173127=CARTESIAN_POINT('Ctrl Pts',(7.12546191799994,15.2,-7.73909243600002));
#173128=CARTESIAN_POINT('Ctrl Pts',(7.12546191799994,11.6,-7.73909243600002));
#173129=CARTESIAN_POINT('Ctrl Pts',(7.12690933599994,15.2,-7.74016856800002));
#173130=CARTESIAN_POINT('Ctrl Pts',(7.12690933599994,11.6,-7.74016856800002));
#173131=CARTESIAN_POINT('Ctrl Pts',(7.12836371399994,15.2,-7.74124779700001));
#173132=CARTESIAN_POINT('Ctrl Pts',(7.12836371399994,11.6,-7.74124779700001));
#173133=CARTESIAN_POINT('Ctrl Pts',(7.12982504399994,15.2,-7.74233010400001));
#173134=CARTESIAN_POINT('Ctrl Pts',(7.12982504399994,11.6,-7.74233010400001));
#173135=CARTESIAN_POINT('Ctrl Pts',(7.13129332299994,15.2,-7.74341546800001));
#173136=CARTESIAN_POINT('Ctrl Pts',(7.13129332299994,11.6,-7.74341546800001));
#173137=CARTESIAN_POINT('Ctrl Pts',(7.13276854299994,15.2,-7.74450387100002));
#173138=CARTESIAN_POINT('Ctrl Pts',(7.13276854299994,11.6,-7.74450387100002));
#173139=CARTESIAN_POINT('Ctrl Pts',(7.13425069899994,15.2,-7.74559529100002));
#173140=CARTESIAN_POINT('Ctrl Pts',(7.13425069899994,11.6,-7.74559529100002));
#173141=CARTESIAN_POINT('Ctrl Pts',(7.13573978399995,15.2,-7.74668971000001));
#173142=CARTESIAN_POINT('Ctrl Pts',(7.13573978399995,11.6,-7.74668971000001));
#173143=CARTESIAN_POINT('Ctrl Pts',(7.13723579299994,15.2,-7.74778710800001));
#173144=CARTESIAN_POINT('Ctrl Pts',(7.13723579299994,11.6,-7.74778710800001));
#173145=CARTESIAN_POINT('Ctrl Pts',(7.13873871899994,15.2,-7.74888746400002));
#173146=CARTESIAN_POINT('Ctrl Pts',(7.13873871899994,11.6,-7.74888746400002));
#173147=CARTESIAN_POINT('Ctrl Pts',(7.14024855599994,15.2,-7.74999076200002));
#173148=CARTESIAN_POINT('Ctrl Pts',(7.14024855599994,11.6,-7.74999076200002));
#173149=CARTESIAN_POINT('Ctrl Pts',(7.14176529899994,15.2,-7.75109697800002));
#173150=CARTESIAN_POINT('Ctrl Pts',(7.14176529899994,11.6,-7.75109697800002));
#173151=CARTESIAN_POINT('Ctrl Pts',(7.14328894099994,15.2,-7.75220609600002));
#173152=CARTESIAN_POINT('Ctrl Pts',(7.14328894099994,11.6,-7.75220609600002));
#173153=CARTESIAN_POINT('Ctrl Pts',(7.14481947699994,15.2,-7.75331809500001));
#173154=CARTESIAN_POINT('Ctrl Pts',(7.14481947699994,11.6,-7.75331809500001));
#173155=CARTESIAN_POINT('Ctrl Pts',(7.14635689999994,15.2,-7.75443295600001));
#173156=CARTESIAN_POINT('Ctrl Pts',(7.14635689999994,11.6,-7.75443295600001));
#173157=CARTESIAN_POINT('Ctrl Pts',(7.14790120399994,15.2,-7.75555066200001));
#173158=CARTESIAN_POINT('Ctrl Pts',(7.14790120399994,11.6,-7.75555066200001));
#173159=CARTESIAN_POINT('Ctrl Pts',(7.14945238399994,15.2,-7.75667119200002));
#173160=CARTESIAN_POINT('Ctrl Pts',(7.14945238399994,11.6,-7.75667119200002));
#173161=CARTESIAN_POINT('Ctrl Pts',(7.15101043299994,15.2,-7.75779452500001));
#173162=CARTESIAN_POINT('Ctrl Pts',(7.15101043299994,11.6,-7.75779452500001));
#173163=CARTESIAN_POINT('Ctrl Pts',(7.15257534599994,15.2,-7.75892064600002));
#173164=CARTESIAN_POINT('Ctrl Pts',(7.15257534599994,11.6,-7.75892064600002));
#173165=CARTESIAN_POINT('Ctrl Pts',(7.15414711699994,15.2,-7.76004953400002));
#173166=CARTESIAN_POINT('Ctrl Pts',(7.15414711699994,11.6,-7.76004953400002));
#173167=CARTESIAN_POINT('Ctrl Pts',(7.15572573899995,15.2,-7.76118117200002));
#173168=CARTESIAN_POINT('Ctrl Pts',(7.15572573899995,11.6,-7.76118117200002));
#173169=CARTESIAN_POINT('Ctrl Pts',(7.15731120799994,15.2,-7.76231553800002));
#173170=CARTESIAN_POINT('Ctrl Pts',(7.15731120799994,11.6,-7.76231553800002));
#173171=CARTESIAN_POINT('Ctrl Pts',(7.15890351499994,15.2,-7.76345261600002));
#173172=CARTESIAN_POINT('Ctrl Pts',(7.15890351499994,11.6,-7.76345261600002));
#173173=CARTESIAN_POINT('Ctrl Pts',(7.16050265799994,15.2,-7.76459238700002));
#173174=CARTESIAN_POINT('Ctrl Pts',(7.16050265799994,11.6,-7.76459238700002));
#173175=CARTESIAN_POINT('Ctrl Pts',(7.16210862799994,15.2,-7.76573483100002));
#173176=CARTESIAN_POINT('Ctrl Pts',(7.16210862799994,11.6,-7.76573483100002));
#173177=CARTESIAN_POINT('Ctrl Pts',(7.16372142099994,15.2,-7.76687993200002));
#173178=CARTESIAN_POINT('Ctrl Pts',(7.16372142099994,11.6,-7.76687993200002));
#173179=CARTESIAN_POINT('Ctrl Pts',(7.16534102999994,15.2,-7.76802767000002));
#173180=CARTESIAN_POINT('Ctrl Pts',(7.16534102999994,11.6,-7.76802767000002));
#173181=CARTESIAN_POINT('Ctrl Pts',(7.16696744899994,15.2,-7.76917802700002));
#173182=CARTESIAN_POINT('Ctrl Pts',(7.16696744899994,11.6,-7.76917802700002));
#173183=CARTESIAN_POINT('Ctrl Pts',(7.16860067299994,15.2,-7.77033098400001));
#173184=CARTESIAN_POINT('Ctrl Pts',(7.16860067299994,11.6,-7.77033098400001));
#173185=CARTESIAN_POINT('Ctrl Pts',(7.17024069599994,15.2,-7.77148652400002));
#173186=CARTESIAN_POINT('Ctrl Pts',(7.17024069599994,11.6,-7.77148652400002));
#173187=CARTESIAN_POINT('Ctrl Pts',(7.17188751299994,15.2,-7.77264462900002));
#173188=CARTESIAN_POINT('Ctrl Pts',(7.17188751299994,11.6,-7.77264462900002));
#173189=CARTESIAN_POINT('Ctrl Pts',(7.17354111499994,15.2,-7.77380527900001));
#173190=CARTESIAN_POINT('Ctrl Pts',(7.17354111499994,11.6,-7.77380527900001));
#173191=CARTESIAN_POINT('Ctrl Pts',(7.17520149999994,15.2,-7.77496845800002));
#173192=CARTESIAN_POINT('Ctrl Pts',(7.17520149999994,11.6,-7.77496845800002));
#173193=CARTESIAN_POINT('Ctrl Pts',(7.17686865999994,15.2,-7.77613414800002));
#173194=CARTESIAN_POINT('Ctrl Pts',(7.17686865999994,11.6,-7.77613414800002));
#173195=CARTESIAN_POINT('Ctrl Pts',(7.17854258999994,15.2,-7.77730233000002));
#173196=CARTESIAN_POINT('Ctrl Pts',(7.17854258999994,11.6,-7.77730233000002));
#173197=CARTESIAN_POINT('Ctrl Pts',(7.18022328299995,15.2,-7.77847298600002));
#173198=CARTESIAN_POINT('Ctrl Pts',(7.18022328299995,11.6,-7.77847298600002));
#173199=CARTESIAN_POINT('Ctrl Pts',(7.18191073399994,15.2,-7.77964610000001));
#173200=CARTESIAN_POINT('Ctrl Pts',(7.18191073399994,11.6,-7.77964610000001));
#173201=CARTESIAN_POINT('Ctrl Pts',(7.18360493799994,15.2,-7.78082165300002));
#173202=CARTESIAN_POINT('Ctrl Pts',(7.18360493799994,11.6,-7.78082165300002));
#173203=CARTESIAN_POINT('Ctrl Pts',(7.18530588899994,15.2,-7.78199962700001));
#173204=CARTESIAN_POINT('Ctrl Pts',(7.18530588899994,11.6,-7.78199962700001));
#173205=CARTESIAN_POINT('Ctrl Pts',(7.18701357999994,15.2,-7.78318000600001));
#173206=CARTESIAN_POINT('Ctrl Pts',(7.18701357999994,11.6,-7.78318000600001));
#173207=CARTESIAN_POINT('Ctrl Pts',(7.18872800599994,15.2,-7.78436277100001));
#173208=CARTESIAN_POINT('Ctrl Pts',(7.18872800599994,11.6,-7.78436277100001));
#173209=CARTESIAN_POINT('Ctrl Pts',(7.19044916199994,15.2,-7.78554790600002));
#173210=CARTESIAN_POINT('Ctrl Pts',(7.19044916199994,11.6,-7.78554790600002));
#173211=CARTESIAN_POINT('Ctrl Pts',(7.19217703999994,15.2,-7.78673539200001));
#173212=CARTESIAN_POINT('Ctrl Pts',(7.19217703999994,11.6,-7.78673539200001));
#173213=CARTESIAN_POINT('Ctrl Pts',(7.19391163699994,15.2,-7.78792521200002));
#173214=CARTESIAN_POINT('Ctrl Pts',(7.19391163699994,11.6,-7.78792521200002));
#173215=CARTESIAN_POINT('Ctrl Pts',(7.19565294499994,15.2,-7.78911735100002));
#173216=CARTESIAN_POINT('Ctrl Pts',(7.19565294499994,11.6,-7.78911735100002));
#173217=CARTESIAN_POINT('Ctrl Pts',(7.19740096099994,15.2,-7.79031178700002));
#173218=CARTESIAN_POINT('Ctrl Pts',(7.19740096099994,11.6,-7.79031178700002));
#173219=CARTESIAN_POINT('Ctrl Pts',(7.19915567599994,15.2,-7.79150850900002));
#173220=CARTESIAN_POINT('Ctrl Pts',(7.19915567599994,11.6,-7.79150850900002));
#173221=CARTESIAN_POINT('Ctrl Pts',(7.20091708699995,15.2,-7.79270749500002));
#173222=CARTESIAN_POINT('Ctrl Pts',(7.20091708699995,11.6,-7.79270749500002));
#173223=CARTESIAN_POINT('Ctrl Pts',(7.20268518599994,15.2,-7.79390872900001));
#173224=CARTESIAN_POINT('Ctrl Pts',(7.20268518599994,11.6,-7.79390872900001));
#173225=CARTESIAN_POINT('Ctrl Pts',(7.20445996999994,15.2,-7.79511219500002));
#173226=CARTESIAN_POINT('Ctrl Pts',(7.20445996999994,11.6,-7.79511219500002));
#173227=CARTESIAN_POINT('Ctrl Pts',(7.20624142999994,15.2,-7.79631787700002));
#173228=CARTESIAN_POINT('Ctrl Pts',(7.20624142999994,11.6,-7.79631787700002));
#173229=CARTESIAN_POINT('Ctrl Pts',(7.20802956399995,15.2,-7.79752575600002));
#173230=CARTESIAN_POINT('Ctrl Pts',(7.20802956399995,11.6,-7.79752575600002));
#173231=CARTESIAN_POINT('Ctrl Pts',(7.20982436399995,15.2,-7.79873581700001));
#173232=CARTESIAN_POINT('Ctrl Pts',(7.20982436399995,11.6,-7.79873581700001));
#173233=CARTESIAN_POINT('Ctrl Pts',(7.21162582299994,15.2,-7.79994804100002));
#173234=CARTESIAN_POINT('Ctrl Pts',(7.21162582299994,11.6,-7.79994804100002));
#173235=CARTESIAN_POINT('Ctrl Pts',(7.21343393899994,15.2,-7.80116241400002));
#173236=CARTESIAN_POINT('Ctrl Pts',(7.21343393899994,11.6,-7.80116241400002));
#173237=CARTESIAN_POINT('Ctrl Pts',(7.21524870299994,15.2,-7.80237891700001));
#173238=CARTESIAN_POINT('Ctrl Pts',(7.21524870299994,11.6,-7.80237891700001));
#173239=CARTESIAN_POINT('Ctrl Pts',(7.21707011099994,15.2,-7.80359753500001));
#173240=CARTESIAN_POINT('Ctrl Pts',(7.21707011099994,11.6,-7.80359753500001));
#173241=CARTESIAN_POINT('Ctrl Pts',(7.21889815899995,15.2,-7.80481825200001));
#173242=CARTESIAN_POINT('Ctrl Pts',(7.21889815899995,11.6,-7.80481825200001));
#173243=CARTESIAN_POINT('Ctrl Pts',(7.22073283799994,15.2,-7.80604104900001));
#173244=CARTESIAN_POINT('Ctrl Pts',(7.22073283799994,11.6,-7.80604104900001));
#173245=CARTESIAN_POINT('Ctrl Pts',(7.22257414399994,15.2,-7.80726591200001));
#173246=CARTESIAN_POINT('Ctrl Pts',(7.22257414399994,11.6,-7.80726591200001));
#173247=CARTESIAN_POINT('Ctrl Pts',(7.22442207099995,15.2,-7.80849282300002));
#173248=CARTESIAN_POINT('Ctrl Pts',(7.22442207099995,11.6,-7.80849282300002));
#173249=CARTESIAN_POINT('Ctrl Pts',(7.22627661399994,15.2,-7.80972176700002));
#173250=CARTESIAN_POINT('Ctrl Pts',(7.22627661399994,11.6,-7.80972176700002));
#173251=CARTESIAN_POINT('Ctrl Pts',(7.22813776799994,15.2,-7.81095272700002));
#173252=CARTESIAN_POINT('Ctrl Pts',(7.22813776799994,11.6,-7.81095272700002));
#173253=CARTESIAN_POINT('Ctrl Pts',(7.23000552399995,15.2,-7.81218568800002));
#173254=CARTESIAN_POINT('Ctrl Pts',(7.23000552399995,11.6,-7.81218568800002));
#173255=CARTESIAN_POINT('Ctrl Pts',(7.23187987999995,15.2,-7.81342063100002));
#173256=CARTESIAN_POINT('Ctrl Pts',(7.23187987999995,11.6,-7.81342063100002));
#173257=CARTESIAN_POINT('Ctrl Pts',(7.23376082999994,15.2,-7.81465754200001));
#173258=CARTESIAN_POINT('Ctrl Pts',(7.23376082999994,11.6,-7.81465754200001));
#173259=CARTESIAN_POINT('Ctrl Pts',(7.23564836799994,15.2,-7.81589640600002));
#173260=CARTESIAN_POINT('Ctrl Pts',(7.23564836799994,11.6,-7.81589640600002));
#173261=CARTESIAN_POINT('Ctrl Pts',(7.23754248699994,15.2,-7.81713720600001));
#173262=CARTESIAN_POINT('Ctrl Pts',(7.23754248699994,11.6,-7.81713720600001));
#173263=CARTESIAN_POINT('Ctrl Pts',(7.23944318299995,15.2,-7.81837992500002));
#173264=CARTESIAN_POINT('Ctrl Pts',(7.23944318299995,11.6,-7.81837992500002));
#173265=CARTESIAN_POINT('Ctrl Pts',(7.24135044899994,15.2,-7.81962454700002));
#173266=CARTESIAN_POINT('Ctrl Pts',(7.24135044899994,11.6,-7.81962454700002));
#173267=CARTESIAN_POINT('Ctrl Pts',(7.24326428099995,15.2,-7.82087105900001));
#173268=CARTESIAN_POINT('Ctrl Pts',(7.24326428099995,11.6,-7.82087105900001));
#173269=CARTESIAN_POINT('Ctrl Pts',(7.24518467299994,15.2,-7.82211944200002));
#173270=CARTESIAN_POINT('Ctrl Pts',(7.24518467299994,11.6,-7.82211944200002));
#173271=CARTESIAN_POINT('Ctrl Pts',(7.24711161899994,15.2,-7.82336968200001));
#173272=CARTESIAN_POINT('Ctrl Pts',(7.24711161899994,11.6,-7.82336968200001));
#173273=CARTESIAN_POINT('Ctrl Pts',(7.24904511399994,15.2,-7.82462176200001));
#173274=CARTESIAN_POINT('Ctrl Pts',(7.24904511399994,11.6,-7.82462176200001));
#173275=CARTESIAN_POINT('Ctrl Pts',(7.25098515199995,15.2,-7.82587566800002));
#173276=CARTESIAN_POINT('Ctrl Pts',(7.25098515199995,11.6,-7.82587566800002));
#173277=CARTESIAN_POINT('Ctrl Pts',(7.25293172799995,15.2,-7.82713138500001));
#173278=CARTESIAN_POINT('Ctrl Pts',(7.25293172799995,11.6,-7.82713138500001));
#173279=CARTESIAN_POINT('Ctrl Pts',(7.25488483599994,15.2,-7.82838889500002));
#173280=CARTESIAN_POINT('Ctrl Pts',(7.25488483599994,11.6,-7.82838889500002));
#173281=CARTESIAN_POINT('Ctrl Pts',(7.25684446999994,15.2,-7.82964818400002));
#173282=CARTESIAN_POINT('Ctrl Pts',(7.25684446999994,11.6,-7.82964818400002));
#173283=CARTESIAN_POINT('Ctrl Pts',(7.25881062599994,15.2,-7.83090923600002));
#173284=CARTESIAN_POINT('Ctrl Pts',(7.25881062599994,11.6,-7.83090923600002));
#173285=CARTESIAN_POINT('Ctrl Pts',(7.26078329799994,15.2,-7.83217203500002));
#173286=CARTESIAN_POINT('Ctrl Pts',(7.26078329799994,11.6,-7.83217203500002));
#173287=CARTESIAN_POINT('Ctrl Pts',(7.26276247899994,15.2,-7.83343656800002));
#173288=CARTESIAN_POINT('Ctrl Pts',(7.26276247899994,11.6,-7.83343656800002));
#173289=CARTESIAN_POINT('Ctrl Pts',(7.26474816499994,15.2,-7.83470281800002));
#173290=CARTESIAN_POINT('Ctrl Pts',(7.26474816499994,11.6,-7.83470281800002));
#173291=CARTESIAN_POINT('Ctrl Pts',(7.26674034999995,15.2,-7.83597077000002));
#173292=CARTESIAN_POINT('Ctrl Pts',(7.26674034999995,11.6,-7.83597077000002));
#173293=CARTESIAN_POINT('Ctrl Pts',(7.26873902899994,15.2,-7.83724040800001));
#173294=CARTESIAN_POINT('Ctrl Pts',(7.26873902899994,11.6,-7.83724040800001));
#173295=CARTESIAN_POINT('Ctrl Pts',(7.27074419499994,15.2,-7.83851172000002));
#173296=CARTESIAN_POINT('Ctrl Pts',(7.27074419499994,11.6,-7.83851172000002));
#173297=CARTESIAN_POINT('Ctrl Pts',(7.27275584499994,15.2,-7.83978468700001));
#173298=CARTESIAN_POINT('Ctrl Pts',(7.27275584499994,11.6,-7.83978468700001));
#173299=CARTESIAN_POINT('Ctrl Pts',(7.27477397199995,15.2,-7.84105929500001));
#173300=CARTESIAN_POINT('Ctrl Pts',(7.27477397199995,11.6,-7.84105929500001));
#173301=CARTESIAN_POINT('Ctrl Pts',(7.27679856999995,15.2,-7.84233553100002));
#173302=CARTESIAN_POINT('Ctrl Pts',(7.27679856999995,11.6,-7.84233553100002));
#173303=CARTESIAN_POINT('Ctrl Pts',(7.27882963499995,15.2,-7.84361337900001));
#173304=CARTESIAN_POINT('Ctrl Pts',(7.27882963499995,11.6,-7.84361337900001));
#173305=CARTESIAN_POINT('Ctrl Pts',(7.28086715999994,15.2,-7.84489282200001));
#173306=CARTESIAN_POINT('Ctrl Pts',(7.28086715999994,11.6,-7.84489282200001));
#173307=CARTESIAN_POINT('Ctrl Pts',(7.28291114199994,15.2,-7.84617384900002));
#173308=CARTESIAN_POINT('Ctrl Pts',(7.28291114199994,11.6,-7.84617384900002));
#173309=CARTESIAN_POINT('Ctrl Pts',(7.28496157299994,15.2,-7.84745644200001));
#173310=CARTESIAN_POINT('Ctrl Pts',(7.28496157299994,11.6,-7.84745644200001));
#173311=CARTESIAN_POINT('Ctrl Pts',(7.28701844799994,15.2,-7.84874058700002));
#173312=CARTESIAN_POINT('Ctrl Pts',(7.28701844799994,11.6,-7.84874058700002));
#173313=CARTESIAN_POINT('Ctrl Pts',(7.28908176299995,15.2,-7.85002627000001));
#173314=CARTESIAN_POINT('Ctrl Pts',(7.28908176299995,11.6,-7.85002627000001));
#173315=CARTESIAN_POINT('Ctrl Pts',(7.29115151099994,15.2,-7.85131347600001));
#173316=CARTESIAN_POINT('Ctrl Pts',(7.29115151099994,11.6,-7.85131347600001));
#173317=CARTESIAN_POINT('Ctrl Pts',(7.29322768799994,15.2,-7.85260219100002));
#173318=CARTESIAN_POINT('Ctrl Pts',(7.29322768799994,11.6,-7.85260219100002));
#173319=CARTESIAN_POINT('Ctrl Pts',(7.29531028699994,15.2,-7.85389239900002));
#173320=CARTESIAN_POINT('Ctrl Pts',(7.29531028699994,11.6,-7.85389239900002));
#173321=CARTESIAN_POINT('Ctrl Pts',(7.29739930399994,15.2,-7.85518408600002));
#173322=CARTESIAN_POINT('Ctrl Pts',(7.29739930399994,11.6,-7.85518408600002));
#173323=CARTESIAN_POINT('Ctrl Pts',(7.29949473199994,15.2,-7.85647723800002));
#173324=CARTESIAN_POINT('Ctrl Pts',(7.29949473199994,11.6,-7.85647723800002));
#173325=CARTESIAN_POINT('Ctrl Pts',(7.30159656799994,15.2,-7.85777184100001));
#173326=CARTESIAN_POINT('Ctrl Pts',(7.30159656799994,11.6,-7.85777184100001));
#173327=CARTESIAN_POINT('Ctrl Pts',(7.30370480499994,15.2,-7.85906787900001));
#173328=CARTESIAN_POINT('Ctrl Pts',(7.30370480499994,11.6,-7.85906787900001));
#173329=CARTESIAN_POINT('Ctrl Pts',(7.30581943699994,15.2,-7.86036533900001));
#173330=CARTESIAN_POINT('Ctrl Pts',(7.30581943699994,11.6,-7.86036533900001));
#173331=CARTESIAN_POINT('Ctrl Pts',(7.30794045899994,15.2,-7.86166420600001));
#173332=CARTESIAN_POINT('Ctrl Pts',(7.30794045899994,11.6,-7.86166420600001));
#173333=CARTESIAN_POINT('Ctrl Pts',(7.31006786699994,15.2,-7.86296446600002));
#173334=CARTESIAN_POINT('Ctrl Pts',(7.31006786699994,11.6,-7.86296446600002));
#173335=CARTESIAN_POINT('Ctrl Pts',(7.31220165399994,15.2,-7.86426610500002));
#173336=CARTESIAN_POINT('Ctrl Pts',(7.31220165399994,11.6,-7.86426610500002));
#173337=CARTESIAN_POINT('Ctrl Pts',(7.31434181599995,15.2,-7.86556910800002));
#173338=CARTESIAN_POINT('Ctrl Pts',(7.31434181599995,11.6,-7.86556910800002));
#173339=CARTESIAN_POINT('Ctrl Pts',(7.31648834699994,15.2,-7.86687346200001));
#173340=CARTESIAN_POINT('Ctrl Pts',(7.31648834699994,11.6,-7.86687346200001));
#173341=CARTESIAN_POINT('Ctrl Pts',(7.31864124199994,15.2,-7.86817915200002));
#173342=CARTESIAN_POINT('Ctrl Pts',(7.31864124199994,11.6,-7.86817915200002));
#173343=CARTESIAN_POINT('Ctrl Pts',(7.32080049399995,15.2,-7.86948616400001));
#173344=CARTESIAN_POINT('Ctrl Pts',(7.32080049399995,11.6,-7.86948616400001));
#173345=CARTESIAN_POINT('Ctrl Pts',(7.32296609999994,15.2,-7.87079448400001));
#173346=CARTESIAN_POINT('Ctrl Pts',(7.32296609999994,11.6,-7.87079448400001));
#173347=CARTESIAN_POINT('Ctrl Pts',(7.32513805299994,15.2,-7.87210409900001));
#173348=CARTESIAN_POINT('Ctrl Pts',(7.32513805299994,11.6,-7.87210409900001));
#173349=CARTESIAN_POINT('Ctrl Pts',(7.32731634799995,15.2,-7.87341499400001));
#173350=CARTESIAN_POINT('Ctrl Pts',(7.32731634799995,11.6,-7.87341499400001));
#173351=CARTESIAN_POINT('Ctrl Pts',(7.32950097899994,15.2,-7.87472715600002));
#173352=CARTESIAN_POINT('Ctrl Pts',(7.32950097899994,11.6,-7.87472715600002));
#173353=CARTESIAN_POINT('Ctrl Pts',(7.33169194399995,15.2,-7.87604056900002));
#173354=CARTESIAN_POINT('Ctrl Pts',(7.33169194399995,11.6,-7.87604056900002));
#173355=CARTESIAN_POINT('Ctrl Pts',(7.33388923299994,15.2,-7.87735522200002));
#173356=CARTESIAN_POINT('Ctrl Pts',(7.33388923299994,11.6,-7.87735522200002));
#173357=CARTESIAN_POINT('Ctrl Pts',(7.33609284399994,15.2,-7.87867109900001));
#173358=CARTESIAN_POINT('Ctrl Pts',(7.33609284399994,11.6,-7.87867109900001));
#173359=CARTESIAN_POINT('Ctrl Pts',(7.33830276899995,15.2,-7.87998818800002));
#173360=CARTESIAN_POINT('Ctrl Pts',(7.33830276899995,11.6,-7.87998818800002));
#173361=CARTESIAN_POINT('Ctrl Pts',(7.34051900599995,15.2,-7.88130647500001));
#173362=CARTESIAN_POINT('Ctrl Pts',(7.34051900599995,11.6,-7.88130647500001));
#173363=CARTESIAN_POINT('Ctrl Pts',(7.34274154699994,15.2,-7.88262594500001));
#173364=CARTESIAN_POINT('Ctrl Pts',(7.34274154699994,11.6,-7.88262594500001));
#173365=CARTESIAN_POINT('Ctrl Pts',(7.34497038799995,15.2,-7.88394658600001));
#173366=CARTESIAN_POINT('Ctrl Pts',(7.34497038799995,11.6,-7.88394658600001));
#173367=CARTESIAN_POINT('Ctrl Pts',(7.34720552299994,15.2,-7.88526838400001));
#173368=CARTESIAN_POINT('Ctrl Pts',(7.34720552299994,11.6,-7.88526838400001));
#173369=CARTESIAN_POINT('Ctrl Pts',(7.34944694599994,15.2,-7.88659132500002));
#173370=CARTESIAN_POINT('Ctrl Pts',(7.34944694599994,11.6,-7.88659132500002));
#173371=CARTESIAN_POINT('Ctrl Pts',(7.35169465499995,15.2,-7.88791539600001));
#173372=CARTESIAN_POINT('Ctrl Pts',(7.35169465499995,11.6,-7.88791539600001));
#173373=CARTESIAN_POINT('Ctrl Pts',(7.35394863999994,15.2,-7.88924058300001));
#173374=CARTESIAN_POINT('Ctrl Pts',(7.35394863999994,11.6,-7.88924058300001));
#173375=CARTESIAN_POINT('Ctrl Pts',(7.35620889899994,15.2,-7.89056687300001));
#173376=CARTESIAN_POINT('Ctrl Pts',(7.35620889899994,11.6,-7.89056687300001));
#173377=CARTESIAN_POINT('Ctrl Pts',(7.35847542699994,15.2,-7.89189425200002));
#173378=CARTESIAN_POINT('Ctrl Pts',(7.35847542699994,11.6,-7.89189425200002));
#173379=CARTESIAN_POINT('Ctrl Pts',(7.36074821699994,15.2,-7.89322270800002));
#173380=CARTESIAN_POINT('Ctrl Pts',(7.36074821699994,11.6,-7.89322270800002));
#173381=CARTESIAN_POINT('Ctrl Pts',(7.36302726299995,15.2,-7.89455222600001));
#173382=CARTESIAN_POINT('Ctrl Pts',(7.36302726299995,11.6,-7.89455222600001));
#173383=CARTESIAN_POINT('Ctrl Pts',(7.36531256299994,15.2,-7.89588279400002));
#173384=CARTESIAN_POINT('Ctrl Pts',(7.36531256299994,11.6,-7.89588279400002));
#173385=CARTESIAN_POINT('Ctrl Pts',(7.36760410799994,15.2,-7.89721439900001));
#173386=CARTESIAN_POINT('Ctrl Pts',(7.36760410799994,11.6,-7.89721439900001));
#173387=CARTESIAN_POINT('Ctrl Pts',(7.36990189499994,15.2,-7.89854702700002));
#173388=CARTESIAN_POINT('Ctrl Pts',(7.36990189499994,11.6,-7.89854702700002));
#173389=CARTESIAN_POINT('Ctrl Pts',(7.37220591899994,15.2,-7.89988066400002));
#173390=CARTESIAN_POINT('Ctrl Pts',(7.37220591899994,11.6,-7.89988066400002));
#173391=CARTESIAN_POINT('Ctrl Pts',(7.37451617399994,15.2,-7.90121530000001));
#173392=CARTESIAN_POINT('Ctrl Pts',(7.37451617399994,11.6,-7.90121530000001));
#173393=CARTESIAN_POINT('Ctrl Pts',(7.37683265399995,15.2,-7.90255091900002));
#173394=CARTESIAN_POINT('Ctrl Pts',(7.37683265399995,11.6,-7.90255091900002));
#173395=CARTESIAN_POINT('Ctrl Pts',(7.37915535499994,15.2,-7.90388750900001));
#173396=CARTESIAN_POINT('Ctrl Pts',(7.37915535499994,11.6,-7.90388750900001));
#173397=CARTESIAN_POINT('Ctrl Pts',(7.38148426999994,15.2,-7.90522505700002));
#173398=CARTESIAN_POINT('Ctrl Pts',(7.38148426999994,11.6,-7.90522505700002));
#173399=CARTESIAN_POINT('Ctrl Pts',(7.38381939699994,15.2,-7.90656355000002));
#173400=CARTESIAN_POINT('Ctrl Pts',(7.38381939699994,11.6,-7.90656355000002));
#173401=CARTESIAN_POINT('Ctrl Pts',(7.38616072799994,15.2,-7.90790297500001));
#173402=CARTESIAN_POINT('Ctrl Pts',(7.38616072799994,11.6,-7.90790297500001));
#173403=CARTESIAN_POINT('Ctrl Pts',(7.38850825799994,15.2,-7.90924331900002));
#173404=CARTESIAN_POINT('Ctrl Pts',(7.38850825799994,11.6,-7.90924331900002));
#173405=CARTESIAN_POINT('Ctrl Pts',(7.39086198299994,15.2,-7.91058457000001));
#173406=CARTESIAN_POINT('Ctrl Pts',(7.39086198299994,11.6,-7.91058457000001));
#173407=CARTESIAN_POINT('Ctrl Pts',(7.39322189599994,15.2,-7.91192671500001));
#173408=CARTESIAN_POINT('Ctrl Pts',(7.39322189599994,11.6,-7.91192671500001));
#173409=CARTESIAN_POINT('Ctrl Pts',(7.39558799399994,15.2,-7.91326974000001));
#173410=CARTESIAN_POINT('Ctrl Pts',(7.39558799399994,11.6,-7.91326974000001));
#173411=CARTESIAN_POINT('Ctrl Pts',(7.39796027099994,15.2,-7.91461363300002));
#173412=CARTESIAN_POINT('Ctrl Pts',(7.39796027099994,11.6,-7.91461363300002));
#173413=CARTESIAN_POINT('Ctrl Pts',(7.40033872099994,15.2,-7.91595838200001));
#173414=CARTESIAN_POINT('Ctrl Pts',(7.40033872099994,11.6,-7.91595838200001));
#173415=CARTESIAN_POINT('Ctrl Pts',(7.40272333899994,15.2,-7.91730397200002));
#173416=CARTESIAN_POINT('Ctrl Pts',(7.40272333899994,11.6,-7.91730397200002));
#173417=CARTESIAN_POINT('Ctrl Pts',(7.40511411999995,15.2,-7.91865039400002));
#173418=CARTESIAN_POINT('Ctrl Pts',(7.40511411999995,11.6,-7.91865039400002));
#173419=CARTESIAN_POINT('Ctrl Pts',(7.40751105899994,15.2,-7.91999763300002));
#173420=CARTESIAN_POINT('Ctrl Pts',(7.40751105899994,11.6,-7.91999763300002));
#173421=CARTESIAN_POINT('Ctrl Pts',(7.40991415099994,15.2,-7.92134567700002));
#173422=CARTESIAN_POINT('Ctrl Pts',(7.40991415099994,11.6,-7.92134567700002));
#173423=CARTESIAN_POINT('Ctrl Pts',(7.41232339099994,15.2,-7.92269451400001));
#173424=CARTESIAN_POINT('Ctrl Pts',(7.41232339099994,11.6,-7.92269451400001));
#173425=CARTESIAN_POINT('Ctrl Pts',(7.41473877199994,15.2,-7.92404412900002));
#173426=CARTESIAN_POINT('Ctrl Pts',(7.41473877199994,11.6,-7.92404412900002));
#173427=CARTESIAN_POINT('Ctrl Pts',(7.41716029099995,15.2,-7.92539451300001));
#173428=CARTESIAN_POINT('Ctrl Pts',(7.41716029099995,11.6,-7.92539451300001));
#173429=CARTESIAN_POINT('Ctrl Pts',(7.41958794199994,15.2,-7.92674565200001));
#173430=CARTESIAN_POINT('Ctrl Pts',(7.41958794199994,11.6,-7.92674565200001));
#173431=CARTESIAN_POINT('Ctrl Pts',(7.42202171899994,15.2,-7.92809753400002));
#173432=CARTESIAN_POINT('Ctrl Pts',(7.42202171899994,11.6,-7.92809753400002));
#173433=CARTESIAN_POINT('Ctrl Pts',(7.42446161799994,15.2,-7.92945014600001));
#173434=CARTESIAN_POINT('Ctrl Pts',(7.42446161799994,11.6,-7.92945014600001));
#173435=CARTESIAN_POINT('Ctrl Pts',(7.42690763399994,15.2,-7.93080347600001));
#173436=CARTESIAN_POINT('Ctrl Pts',(7.42690763399994,11.6,-7.93080347600001));
#173437=CARTESIAN_POINT('Ctrl Pts',(7.42935975999995,15.2,-7.93215751200002));
#173438=CARTESIAN_POINT('Ctrl Pts',(7.42935975999995,11.6,-7.93215751200002));
#173439=CARTESIAN_POINT('Ctrl Pts',(7.43181799299995,15.2,-7.93351224200002));
#173440=CARTESIAN_POINT('Ctrl Pts',(7.43181799299995,11.6,-7.93351224200002));
#173441=CARTESIAN_POINT('Ctrl Pts',(7.43428232699994,15.2,-7.93486765200001));
#173442=CARTESIAN_POINT('Ctrl Pts',(7.43428232699994,11.6,-7.93486765200001));
#173443=CARTESIAN_POINT('Ctrl Pts',(7.43675275699994,15.2,-7.93622373200002));
#173444=CARTESIAN_POINT('Ctrl Pts',(7.43675275699994,11.6,-7.93622373200002));
#173445=CARTESIAN_POINT('Ctrl Pts',(7.43922927599994,15.2,-7.93758046900002));
#173446=CARTESIAN_POINT('Ctrl Pts',(7.43922927599994,11.6,-7.93758046900002));
#173447=CARTESIAN_POINT('Ctrl Pts',(7.44171188299994,15.2,-7.93893785000002));
#173448=CARTESIAN_POINT('Ctrl Pts',(7.44171188299994,11.6,-7.93893785000002));
#173449=CARTESIAN_POINT('Ctrl Pts',(7.44420056799994,15.2,-7.94029586500002));
#173450=CARTESIAN_POINT('Ctrl Pts',(7.44420056799994,11.6,-7.94029586500002));
#173451=CARTESIAN_POINT('Ctrl Pts',(7.44669532899994,15.2,-7.94165450000002));
#173452=CARTESIAN_POINT('Ctrl Pts',(7.44669532899994,11.6,-7.94165450000002));
#173453=CARTESIAN_POINT('Ctrl Pts',(7.44919616099994,15.2,-7.94301374500002));
#173454=CARTESIAN_POINT('Ctrl Pts',(7.44919616099994,11.6,-7.94301374500002));
#173455=CARTESIAN_POINT('Ctrl Pts',(7.45170305699994,15.2,-7.94437358500002));
#173456=CARTESIAN_POINT('Ctrl Pts',(7.45170305699994,11.6,-7.94437358500002));
#173457=CARTESIAN_POINT('Ctrl Pts',(7.45421601299994,15.2,-7.94573401100001));
#173458=CARTESIAN_POINT('Ctrl Pts',(7.45421601299994,11.6,-7.94573401100001));
#173459=CARTESIAN_POINT('Ctrl Pts',(7.45673502399994,15.2,-7.94709501000002));
#173460=CARTESIAN_POINT('Ctrl Pts',(7.45673502399994,11.6,-7.94709501000002));
#173461=CARTESIAN_POINT('Ctrl Pts',(7.45926008499994,15.2,-7.94845657000002));
#173462=CARTESIAN_POINT('Ctrl Pts',(7.45926008499994,11.6,-7.94845657000002));
#173463=CARTESIAN_POINT('Ctrl Pts',(7.46179118999994,15.2,-7.94981867900002));
#173464=CARTESIAN_POINT('Ctrl Pts',(7.46179118999994,11.6,-7.94981867900002));
#173465=CARTESIAN_POINT('Ctrl Pts',(7.46432833399994,15.2,-7.95118132500002));
#173466=CARTESIAN_POINT('Ctrl Pts',(7.46432833399994,11.6,-7.95118132500002));
#173467=CARTESIAN_POINT('Ctrl Pts',(7.46687151199994,15.2,-7.95254449800002));
#173468=CARTESIAN_POINT('Ctrl Pts',(7.46687151199994,11.6,-7.95254449800002));
#173469=CARTESIAN_POINT('Ctrl Pts',(7.46942071999994,15.2,-7.95390818300002));
#173470=CARTESIAN_POINT('Ctrl Pts',(7.46942071999994,11.6,-7.95390818300002));
#173471=CARTESIAN_POINT('Ctrl Pts',(7.47197595099995,15.2,-7.95527237200002));
#173472=CARTESIAN_POINT('Ctrl Pts',(7.47197595099995,11.6,-7.95527237200002));
#173473=CARTESIAN_POINT('Ctrl Pts',(7.47453719999994,15.2,-7.95663705000001));
#173474=CARTESIAN_POINT('Ctrl Pts',(7.47453719999994,11.6,-7.95663705000001));
#173475=CARTESIAN_POINT('Ctrl Pts',(7.47710446499994,15.2,-7.95800220700002));
#173476=CARTESIAN_POINT('Ctrl Pts',(7.47710446499994,11.6,-7.95800220700002));
#173477=CARTESIAN_POINT('Ctrl Pts',(7.47967773699994,15.2,-7.95936783200001));
#173478=CARTESIAN_POINT('Ctrl Pts',(7.47967773699994,11.6,-7.95936783200001));
#173479=CARTESIAN_POINT('Ctrl Pts',(7.48225701299994,15.2,-7.96073391100002));
#173480=CARTESIAN_POINT('Ctrl Pts',(7.48225701299994,11.6,-7.96073391100002));
#173481=CARTESIAN_POINT('Ctrl Pts',(7.48484228799994,15.2,-7.96210043600002));
#173482=CARTESIAN_POINT('Ctrl Pts',(7.48484228799994,11.6,-7.96210043600002));
#173483=CARTESIAN_POINT('Ctrl Pts',(7.48743355699995,15.2,-7.96346739200001));
#173484=CARTESIAN_POINT('Ctrl Pts',(7.48743355699995,11.6,-7.96346739200001));
#173485=CARTESIAN_POINT('Ctrl Pts',(7.49003081299994,15.2,-7.96483476900002));
#173486=CARTESIAN_POINT('Ctrl Pts',(7.49003081299994,11.6,-7.96483476900002));
#173487=CARTESIAN_POINT('Ctrl Pts',(7.49263405299994,15.2,-7.96620255600001));
#173488=CARTESIAN_POINT('Ctrl Pts',(7.49263405299994,11.6,-7.96620255600001));
#173489=CARTESIAN_POINT('Ctrl Pts',(7.49524327099994,15.2,-7.96757074100002));
#173490=CARTESIAN_POINT('Ctrl Pts',(7.49524327099994,11.6,-7.96757074100002));
#173491=CARTESIAN_POINT('Ctrl Pts',(7.49785846099994,15.2,-7.96893931300002));
#173492=CARTESIAN_POINT('Ctrl Pts',(7.49785846099994,11.6,-7.96893931300002));
#173493=CARTESIAN_POINT('Ctrl Pts',(7.50047961999995,15.2,-7.97030826000002));
#173494=CARTESIAN_POINT('Ctrl Pts',(7.50047961999995,11.6,-7.97030826000002));
#173495=CARTESIAN_POINT('Ctrl Pts',(7.50310674299994,15.2,-7.97167757000001));
#173496=CARTESIAN_POINT('Ctrl Pts',(7.50310674299994,11.6,-7.97167757000001));
#173497=CARTESIAN_POINT('Ctrl Pts',(7.50573982199994,15.2,-7.97304723400002));
#173498=CARTESIAN_POINT('Ctrl Pts',(7.50573982199994,11.6,-7.97304723400002));
#173499=CARTESIAN_POINT('Ctrl Pts',(7.50837885499994,15.2,-7.97441723900001));
#173500=CARTESIAN_POINT('Ctrl Pts',(7.50837885499994,11.6,-7.97441723900001));
#173501=CARTESIAN_POINT('Ctrl Pts',(7.51102383599994,15.2,-7.97578757300001));
#173502=CARTESIAN_POINT('Ctrl Pts',(7.51102383599994,11.6,-7.97578757300001));
#173503=CARTESIAN_POINT('Ctrl Pts',(7.51367475799994,15.2,-7.97715822700001));
#173504=CARTESIAN_POINT('Ctrl Pts',(7.51367475799994,11.6,-7.97715822700001));
#173505=CARTESIAN_POINT('Ctrl Pts',(7.51633161799995,15.2,-7.97852918700002));
#173506=CARTESIAN_POINT('Ctrl Pts',(7.51633161799995,11.6,-7.97852918700002));
#173507=CARTESIAN_POINT('Ctrl Pts',(7.51899441199994,15.2,-7.97990044500001));
#173508=CARTESIAN_POINT('Ctrl Pts',(7.51899441199994,11.6,-7.97990044500001));
#173509=CARTESIAN_POINT('Ctrl Pts',(7.52166313299995,15.2,-7.98127198800002));
#173510=CARTESIAN_POINT('Ctrl Pts',(7.52166313299995,11.6,-7.98127198800002));
#173511=CARTESIAN_POINT('Ctrl Pts',(7.52433777599994,15.2,-7.98264380500001));
#173512=CARTESIAN_POINT('Ctrl Pts',(7.52433777599994,11.6,-7.98264380500001));
#173513=CARTESIAN_POINT('Ctrl Pts',(7.52701833599994,15.2,-7.98401588500001));
#173514=CARTESIAN_POINT('Ctrl Pts',(7.52701833599994,11.6,-7.98401588500001));
#173515=CARTESIAN_POINT('Ctrl Pts',(7.52970480999994,15.2,-7.98538821700002));
#173516=CARTESIAN_POINT('Ctrl Pts',(7.52970480999994,11.6,-7.98538821700002));
#173517=CARTESIAN_POINT('Ctrl Pts',(7.53239718999994,15.2,-7.98676079000002));
#173518=CARTESIAN_POINT('Ctrl Pts',(7.53239718999994,11.6,-7.98676079000002));
#173519=CARTESIAN_POINT('Ctrl Pts',(7.53509547299994,15.2,-7.98813359300001));
#173520=CARTESIAN_POINT('Ctrl Pts',(7.53509547299994,11.6,-7.98813359300001));
#173521=CARTESIAN_POINT('Ctrl Pts',(7.53779965199994,15.2,-7.98950661400001));
#173522=CARTESIAN_POINT('Ctrl Pts',(7.53779965199994,11.6,-7.98950661400001));
#173523=CARTESIAN_POINT('Ctrl Pts',(7.54050972499994,15.2,-7.99087984500002));
#173524=CARTESIAN_POINT('Ctrl Pts',(7.54050972499994,11.6,-7.99087984500002));
#173525=CARTESIAN_POINT('Ctrl Pts',(7.54322568399994,15.2,-7.99225327200002));
#173526=CARTESIAN_POINT('Ctrl Pts',(7.54322568399994,11.6,-7.99225327200002));
#173527=CARTESIAN_POINT('Ctrl Pts',(7.54594752699994,15.2,-7.99362688500001));
#173528=CARTESIAN_POINT('Ctrl Pts',(7.54594752699994,11.6,-7.99362688500001));
#173529=CARTESIAN_POINT('Ctrl Pts',(7.54867524599995,15.2,-7.99500067300002));
#173530=CARTESIAN_POINT('Ctrl Pts',(7.54867524599995,11.6,-7.99500067300002));
#173531=CARTESIAN_POINT('Ctrl Pts',(7.55140883599994,15.2,-7.99637462700002));
#173532=CARTESIAN_POINT('Ctrl Pts',(7.55140883599994,11.6,-7.99637462700002));
#173533=CARTESIAN_POINT('Ctrl Pts',(7.55414829499995,15.2,-7.99774873400001));
#173534=CARTESIAN_POINT('Ctrl Pts',(7.55414829499995,11.6,-7.99774873400001));
#173535=CARTESIAN_POINT('Ctrl Pts',(7.55689361499994,15.2,-7.99912298400002));
#173536=CARTESIAN_POINT('Ctrl Pts',(7.55689361499994,11.6,-7.99912298400002));
#173537=CARTESIAN_POINT('Ctrl Pts',(7.55964479299994,15.2,-8.00049736600002));
#173538=CARTESIAN_POINT('Ctrl Pts',(7.55964479299994,11.6,-8.00049736600002));
#173539=CARTESIAN_POINT('Ctrl Pts',(7.56240182199994,15.2,-8.00187187000001));
#173540=CARTESIAN_POINT('Ctrl Pts',(7.56240182199994,11.6,-8.00187187000001));
#173541=CARTESIAN_POINT('Ctrl Pts',(7.56516469899994,15.2,-8.00324648500002));
#173542=CARTESIAN_POINT('Ctrl Pts',(7.56516469899994,11.6,-8.00324648500002));
#173543=CARTESIAN_POINT('Ctrl Pts',(7.56793341799994,15.2,-8.00462119900001));
#173544=CARTESIAN_POINT('Ctrl Pts',(7.56793341799994,11.6,-8.00462119900001));
#173545=CARTESIAN_POINT('Ctrl Pts',(7.57070797399995,15.2,-8.00599600300002));
#173546=CARTESIAN_POINT('Ctrl Pts',(7.57070797399995,11.6,-8.00599600300002));
#173547=CARTESIAN_POINT('Ctrl Pts',(7.57348836199994,15.2,-8.00737088600001));
#173548=CARTESIAN_POINT('Ctrl Pts',(7.57348836199994,11.6,-8.00737088600001));
#173549=CARTESIAN_POINT('Ctrl Pts',(7.57627457699994,15.2,-8.00874583800002));
#173550=CARTESIAN_POINT('Ctrl Pts',(7.57627457699994,11.6,-8.00874583800002));
#173551=CARTESIAN_POINT('Ctrl Pts',(7.57906661499994,15.2,-8.01012084700002));
#173552=CARTESIAN_POINT('Ctrl Pts',(7.57906661499994,11.6,-8.01012084700002));
#173553=CARTESIAN_POINT('Ctrl Pts',(7.58186446999995,15.2,-8.01149590300002));
#173554=CARTESIAN_POINT('Ctrl Pts',(7.58186446999995,11.6,-8.01149590300002));
#173555=CARTESIAN_POINT('Ctrl Pts',(7.58466813599994,15.2,-8.01287099600002));
#173556=CARTESIAN_POINT('Ctrl Pts',(7.58466813599994,11.6,-8.01287099600002));
#173557=CARTESIAN_POINT('Ctrl Pts',(7.58747760999994,15.2,-8.01424611600002));
#173558=CARTESIAN_POINT('Ctrl Pts',(7.58747760999994,11.6,-8.01424611600002));
#173559=CARTESIAN_POINT('Ctrl Pts',(7.59029288699994,15.2,-8.01562125100002));
#173560=CARTESIAN_POINT('Ctrl Pts',(7.59029288699994,11.6,-8.01562125100002));
#173561=CARTESIAN_POINT('Ctrl Pts',(7.59311395999994,15.2,-8.01699639100002));
#173562=CARTESIAN_POINT('Ctrl Pts',(7.59311395999994,11.6,-8.01699639100002));
#173563=CARTESIAN_POINT('Ctrl Pts',(7.59594082499994,15.2,-8.01837152600001));
#173564=CARTESIAN_POINT('Ctrl Pts',(7.59594082499994,11.6,-8.01837152600001));
#173565=CARTESIAN_POINT('Ctrl Pts',(7.59877347799994,15.2,-8.01974664700002));
#173566=CARTESIAN_POINT('Ctrl Pts',(7.59877347799994,11.6,-8.01974664700002));
#173567=CARTESIAN_POINT('Ctrl Pts',(7.60161191199995,15.2,-8.02112174000002));
#173568=CARTESIAN_POINT('Ctrl Pts',(7.60161191199995,11.6,-8.02112174000002));
#173569=CARTESIAN_POINT('Ctrl Pts',(7.60445612499994,15.2,-8.02249679800001));
#173570=CARTESIAN_POINT('Ctrl Pts',(7.60445612499994,11.6,-8.02249679800001));
#173571=CARTESIAN_POINT('Ctrl Pts',(7.60730610999994,15.2,-8.02387181100002));
#173572=CARTESIAN_POINT('Ctrl Pts',(7.60730610999994,11.6,-8.02387181100002));
#173573=CARTESIAN_POINT('Ctrl Pts',(7.61016186199994,15.2,-8.02524676500001));
#173574=CARTESIAN_POINT('Ctrl Pts',(7.61016186199994,11.6,-8.02524676500001));
#173575=CARTESIAN_POINT('Ctrl Pts',(7.61302337699994,15.2,-8.02662165300001));
#173576=CARTESIAN_POINT('Ctrl Pts',(7.61302337699994,11.6,-8.02662165300001));
#173577=CARTESIAN_POINT('Ctrl Pts',(7.61589064899994,15.2,-8.02799646400001));
#173578=CARTESIAN_POINT('Ctrl Pts',(7.61589064899994,11.6,-8.02799646400001));
#173579=CARTESIAN_POINT('Ctrl Pts',(7.61876367299994,15.2,-8.02937118700001));
#173580=CARTESIAN_POINT('Ctrl Pts',(7.61876367299994,11.6,-8.02937118700001));
#173581=CARTESIAN_POINT('Ctrl Pts',(7.62164244499994,15.2,-8.03074581300002));
#173582=CARTESIAN_POINT('Ctrl Pts',(7.62164244499994,11.6,-8.03074581300002));
#173583=CARTESIAN_POINT('Ctrl Pts',(7.62452696099994,15.2,-8.03212033100002));
#173584=CARTESIAN_POINT('Ctrl Pts',(7.62452696099994,11.6,-8.03212033100002));
#173585=CARTESIAN_POINT('Ctrl Pts',(7.62741721299995,15.2,-8.03349473200001));
#173586=CARTESIAN_POINT('Ctrl Pts',(7.62741721299995,11.6,-8.03349473200001));
#173587=CARTESIAN_POINT('Ctrl Pts',(7.63031319799994,15.2,-8.03486900500002));
#173588=CARTESIAN_POINT('Ctrl Pts',(7.63031319799994,11.6,-8.03486900500002));
#173589=CARTESIAN_POINT('Ctrl Pts',(7.63321491099994,15.2,-8.03624314000002));
#173590=CARTESIAN_POINT('Ctrl Pts',(7.63321491099994,11.6,-8.03624314000002));
#173591=CARTESIAN_POINT('Ctrl Pts',(7.63612234699995,15.2,-8.03761712700001));
#173592=CARTESIAN_POINT('Ctrl Pts',(7.63612234699995,11.6,-8.03761712700001));
#173593=CARTESIAN_POINT('Ctrl Pts',(7.63903550099994,15.2,-8.03899095600002));
#173594=CARTESIAN_POINT('Ctrl Pts',(7.63903550099994,11.6,-8.03899095600002));
#173595=CARTESIAN_POINT('Ctrl Pts',(7.64195436699994,15.2,-8.04036461600001));
#173596=CARTESIAN_POINT('Ctrl Pts',(7.64195436699994,11.6,-8.04036461600001));
#173597=CARTESIAN_POINT('Ctrl Pts',(7.64487894199994,15.2,-8.04173809900002));
#173598=CARTESIAN_POINT('Ctrl Pts',(7.64487894199994,11.6,-8.04173809900002));
#173599=CARTESIAN_POINT('Ctrl Pts',(7.64780921899994,15.2,-8.04311139400001));
#173600=CARTESIAN_POINT('Ctrl Pts',(7.64780921899994,11.6,-8.04311139400001));
#173601=CARTESIAN_POINT('Ctrl Pts',(7.65074519499994,15.2,-8.04448449100001));
#173602=CARTESIAN_POINT('Ctrl Pts',(7.65074519499994,11.6,-8.04448449100001));
#173603=CARTESIAN_POINT('Ctrl Pts',(7.65368686399994,15.2,-8.04585738000002));
#173604=CARTESIAN_POINT('Ctrl Pts',(7.65368686399994,11.6,-8.04585738000002));
#173605=CARTESIAN_POINT('Ctrl Pts',(7.65663422099994,15.2,-8.04723005200002));
#173606=CARTESIAN_POINT('Ctrl Pts',(7.65663422099994,11.6,-8.04723005200002));
#173607=CARTESIAN_POINT('Ctrl Pts',(7.65958726299995,15.2,-8.04860249700001));
#173608=CARTESIAN_POINT('Ctrl Pts',(7.65958726299995,11.6,-8.04860249700001));
#173609=CARTESIAN_POINT('Ctrl Pts',(7.66254598199994,15.2,-8.04997470400002));
#173610=CARTESIAN_POINT('Ctrl Pts',(7.66254598199994,11.6,-8.04997470400002));
#173611=CARTESIAN_POINT('Ctrl Pts',(7.66551037499994,15.2,-8.05134666300001));
#173612=CARTESIAN_POINT('Ctrl Pts',(7.66551037499994,11.6,-8.05134666300001));
#173613=CARTESIAN_POINT('Ctrl Pts',(7.66848043599994,15.2,-8.05271836600001));
#173614=CARTESIAN_POINT('Ctrl Pts',(7.66848043599994,11.6,-8.05271836600001));
#173615=CARTESIAN_POINT('Ctrl Pts',(7.67145616099994,15.2,-8.05408980300001));
#173616=CARTESIAN_POINT('Ctrl Pts',(7.67145616099994,11.6,-8.05408980300001));
#173617=CARTESIAN_POINT('Ctrl Pts',(7.67443754499994,15.2,-8.05546096200001));
#173618=CARTESIAN_POINT('Ctrl Pts',(7.67443754499994,11.6,-8.05546096200001));
#173619=CARTESIAN_POINT('Ctrl Pts',(7.67742458199994,15.2,-8.05683183700001));
#173620=CARTESIAN_POINT('Ctrl Pts',(7.67742458199994,11.6,-8.05683183700001));
#173621=CARTESIAN_POINT('Ctrl Pts',(7.68041726999994,15.2,-8.05820241500001));
#173622=CARTESIAN_POINT('Ctrl Pts',(7.68041726999994,11.6,-8.05820241500001));
#173623=CARTESIAN_POINT('Ctrl Pts',(7.68341559999994,15.2,-8.05957268800002));
#173624=CARTESIAN_POINT('Ctrl Pts',(7.68341559999994,11.6,-8.05957268800002));
#173625=CARTESIAN_POINT('Ctrl Pts',(7.68641956999994,15.2,-8.06094264600001));
#173626=CARTESIAN_POINT('Ctrl Pts',(7.68641956999994,11.6,-8.06094264600001));
#173627=CARTESIAN_POINT('Ctrl Pts',(7.68942917399994,15.2,-8.06231227900001));
#173628=CARTESIAN_POINT('Ctrl Pts',(7.68942917399994,11.6,-8.06231227900001));
#173629=CARTESIAN_POINT('Ctrl Pts',(7.69244440799994,15.2,-8.06368157700001));
#173630=CARTESIAN_POINT('Ctrl Pts',(7.69244440799994,11.6,-8.06368157700001));
#173631=CARTESIAN_POINT('Ctrl Pts',(7.69546526599994,15.2,-8.06505053200001));
#173632=CARTESIAN_POINT('Ctrl Pts',(7.69546526599994,11.6,-8.06505053200001));
#173633=CARTESIAN_POINT('Ctrl Pts',(7.69849174399994,15.2,-8.06641913400002));
#173634=CARTESIAN_POINT('Ctrl Pts',(7.69849174399994,11.6,-8.06641913400002));
#173635=CARTESIAN_POINT('Ctrl Pts',(7.70152383599994,15.2,-8.06778737300002));
#173636=CARTESIAN_POINT('Ctrl Pts',(7.70152383599994,11.6,-8.06778737300002));
#173637=CARTESIAN_POINT('Ctrl Pts',(7.70456153899994,15.2,-8.06915523900001));
#173638=CARTESIAN_POINT('Ctrl Pts',(7.70456153899994,11.6,-8.06915523900001));
#173639=CARTESIAN_POINT('Ctrl Pts',(7.70760484499994,15.2,-8.07052272400002));
#173640=CARTESIAN_POINT('Ctrl Pts',(7.70760484499994,11.6,-8.07052272400002));
#173641=CARTESIAN_POINT('Ctrl Pts',(7.71065375199995,15.2,-8.07188981700002));
#173642=CARTESIAN_POINT('Ctrl Pts',(7.71065375199995,11.6,-8.07188981700002));
#173643=CARTESIAN_POINT('Ctrl Pts',(7.71370825399995,15.2,-8.07325651000001));
#173644=CARTESIAN_POINT('Ctrl Pts',(7.71370825399995,11.6,-8.07325651000001));
#173645=CARTESIAN_POINT('Ctrl Pts',(7.71676834699995,15.2,-8.07462279100001));
#173646=CARTESIAN_POINT('Ctrl Pts',(7.71676834699995,11.6,-8.07462279100001));
#173647=CARTESIAN_POINT('Ctrl Pts',(7.71983402499994,15.2,-8.07598865400001));
#173648=CARTESIAN_POINT('Ctrl Pts',(7.71983402499994,11.6,-8.07598865400001));
#173649=CARTESIAN_POINT('Ctrl Pts',(7.72290528299994,15.2,-8.07735408800001));
#173650=CARTESIAN_POINT('Ctrl Pts',(7.72290528299994,11.6,-8.07735408800001));
#173651=CARTESIAN_POINT('Ctrl Pts',(7.72598211699994,15.2,-8.07871908400001));
#173652=CARTESIAN_POINT('Ctrl Pts',(7.72598211699994,11.6,-8.07871908400001));
#173653=CARTESIAN_POINT('Ctrl Pts',(7.72906452199994,15.2,-8.08008363200001));
#173654=CARTESIAN_POINT('Ctrl Pts',(7.72906452199994,11.6,-8.08008363200001));
#173655=CARTESIAN_POINT('Ctrl Pts',(7.73215249199994,15.2,-8.08144772300002));
#173656=CARTESIAN_POINT('Ctrl Pts',(7.73215249199994,11.6,-8.08144772300002));
#173657=CARTESIAN_POINT('Ctrl Pts',(7.73524602399994,15.2,-8.08281134700002));
#173658=CARTESIAN_POINT('Ctrl Pts',(7.73524602399994,11.6,-8.08281134700002));
#173659=CARTESIAN_POINT('Ctrl Pts',(7.73834511099994,15.2,-8.08417449700002));
#173660=CARTESIAN_POINT('Ctrl Pts',(7.73834511099994,11.6,-8.08417449700002));
#173661=CARTESIAN_POINT('Ctrl Pts',(7.74144975099994,15.2,-8.08553716200001));
#173662=CARTESIAN_POINT('Ctrl Pts',(7.74144975099994,11.6,-8.08553716200001));
#173663=CARTESIAN_POINT('Ctrl Pts',(7.74455993599994,15.2,-8.08689933300002));
#173664=CARTESIAN_POINT('Ctrl Pts',(7.74455993599994,11.6,-8.08689933300002));
#173665=CARTESIAN_POINT('Ctrl Pts',(7.74767566299994,15.2,-8.08826100000001));
#173666=CARTESIAN_POINT('Ctrl Pts',(7.74767566299994,11.6,-8.08826100000001));
#173667=CARTESIAN_POINT('Ctrl Pts',(7.75079692599994,15.2,-8.08962215600001));
#173668=CARTESIAN_POINT('Ctrl Pts',(7.75079692599994,11.6,-8.08962215600001));
#173669=CARTESIAN_POINT('Ctrl Pts',(7.75392372099994,15.2,-8.09098279100001));
#173670=CARTESIAN_POINT('Ctrl Pts',(7.75392372099994,11.6,-8.09098279100001));
#173671=CARTESIAN_POINT('Ctrl Pts',(7.75705604399994,15.2,-8.09234289400001));
#173672=CARTESIAN_POINT('Ctrl Pts',(7.75705604399994,11.6,-8.09234289400001));
#173673=CARTESIAN_POINT('Ctrl Pts',(7.76019388899994,15.2,-8.09370245900002));
#173674=CARTESIAN_POINT('Ctrl Pts',(7.76019388899994,11.6,-8.09370245900002));
#173675=CARTESIAN_POINT('Ctrl Pts',(7.76333724999994,15.2,-8.09506147500001));
#173676=CARTESIAN_POINT('Ctrl Pts',(7.76333724999994,11.6,-8.09506147500001));
#173677=CARTESIAN_POINT('Ctrl Pts',(7.76648612399994,15.2,-8.09641993200002));
#173678=CARTESIAN_POINT('Ctrl Pts',(7.76648612399994,11.6,-8.09641993200002));
#173679=CARTESIAN_POINT('Ctrl Pts',(7.76964050599994,15.2,-8.09777782300002));
#173680=CARTESIAN_POINT('Ctrl Pts',(7.76964050599994,11.6,-8.09777782300002));
#173681=CARTESIAN_POINT('Ctrl Pts',(7.77280038999994,15.2,-8.09913513800002));
#173682=CARTESIAN_POINT('Ctrl Pts',(7.77280038999994,11.6,-8.09913513800002));
#173683=CARTESIAN_POINT('Ctrl Pts',(7.77596577299994,15.2,-8.10049186900001));
#173684=CARTESIAN_POINT('Ctrl Pts',(7.77596577299994,11.6,-8.10049186900001));
#173685=CARTESIAN_POINT('Ctrl Pts',(7.77913664799994,15.2,-8.10184800500002));
#173686=CARTESIAN_POINT('Ctrl Pts',(7.77913664799994,11.6,-8.10184800500002));
#173687=CARTESIAN_POINT('Ctrl Pts',(7.78231301099995,15.2,-8.10320354000002));
#173688=CARTESIAN_POINT('Ctrl Pts',(7.78231301099995,11.6,-8.10320354000002));
#173689=CARTESIAN_POINT('Ctrl Pts',(7.78549485799994,15.2,-8.10455846200002));
#173690=CARTESIAN_POINT('Ctrl Pts',(7.78549485799994,11.6,-8.10455846200002));
#173691=CARTESIAN_POINT('Ctrl Pts',(7.78868218299994,15.2,-8.10591276400002));
#173692=CARTESIAN_POINT('Ctrl Pts',(7.78868218299994,11.6,-8.10591276400002));
#173693=CARTESIAN_POINT('Ctrl Pts',(7.79187498299994,15.2,-8.10726643600002));
#173694=CARTESIAN_POINT('Ctrl Pts',(7.79187498299994,11.6,-8.10726643600002));
#173695=CARTESIAN_POINT('Ctrl Pts',(7.79507325099994,15.2,-8.10861947000001));
#173696=CARTESIAN_POINT('Ctrl Pts',(7.79507325099994,11.6,-8.10861947000001));
#173697=CARTESIAN_POINT('Ctrl Pts',(7.79827698299994,15.2,-8.10997185600002));
#173698=CARTESIAN_POINT('Ctrl Pts',(7.79827698299994,11.6,-8.10997185600002));
#173699=CARTESIAN_POINT('Ctrl Pts',(7.80148617399994,15.2,-8.11132358800002));
#173700=CARTESIAN_POINT('Ctrl Pts',(7.80148617399994,11.6,-8.11132358800002));
#173701=CARTESIAN_POINT('Ctrl Pts',(7.80470081999994,15.2,-8.11267465300002));
#173702=CARTESIAN_POINT('Ctrl Pts',(7.80470081999994,11.6,-8.11267465300002));
#173703=CARTESIAN_POINT('Ctrl Pts',(7.80792091399995,15.2,-8.11402504600002));
#173704=CARTESIAN_POINT('Ctrl Pts',(7.80792091399995,11.6,-8.11402504600002));
#173705=CARTESIAN_POINT('Ctrl Pts',(7.81114645399994,15.2,-8.11537475600002));
#173706=CARTESIAN_POINT('Ctrl Pts',(7.81114645399994,11.6,-8.11537475600002));
#173707=CARTESIAN_POINT('Ctrl Pts',(7.81437743299994,15.2,-8.11672377300001));
#173708=CARTESIAN_POINT('Ctrl Pts',(7.81437743299994,11.6,-8.11672377300001));
#173709=CARTESIAN_POINT('Ctrl Pts',(7.81761384899994,15.2,-8.11807209300002));
#173710=CARTESIAN_POINT('Ctrl Pts',(7.81761384899994,11.6,-8.11807209300002));
#173711=CARTESIAN_POINT('Ctrl Pts',(7.82085569299995,15.2,-8.11941970200002));
#173712=CARTESIAN_POINT('Ctrl Pts',(7.82085569299995,11.6,-8.11941970200002));
#173713=CARTESIAN_POINT('Ctrl Pts',(7.82410296399994,15.2,-8.12076659500002));
#173714=CARTESIAN_POINT('Ctrl Pts',(7.82410296399994,11.6,-8.12076659500002));
#173715=CARTESIAN_POINT('Ctrl Pts',(7.82735565499994,15.2,-8.12211276200001));
#173716=CARTESIAN_POINT('Ctrl Pts',(7.82735565499994,11.6,-8.12211276200001));
#173717=CARTESIAN_POINT('Ctrl Pts',(7.83061376199995,15.2,-8.12345819400001));
#173718=CARTESIAN_POINT('Ctrl Pts',(7.83061376199995,11.6,-8.12345819400001));
#173719=CARTESIAN_POINT('Ctrl Pts',(7.83387727999994,15.2,-8.12480288300002));
#173720=CARTESIAN_POINT('Ctrl Pts',(7.83387727999994,11.6,-8.12480288300002));
#173721=CARTESIAN_POINT('Ctrl Pts',(7.83714620399994,15.2,-8.12614682000002));
#173722=CARTESIAN_POINT('Ctrl Pts',(7.83714620399994,11.6,-8.12614682000002));
#173723=CARTESIAN_POINT('Ctrl Pts',(7.84042052999995,15.2,-8.12748999700002));
#173724=CARTESIAN_POINT('Ctrl Pts',(7.84042052999995,11.6,-8.12748999700002));
#173725=CARTESIAN_POINT('Ctrl Pts',(7.84370025199994,15.2,-8.12883240500001));
#173726=CARTESIAN_POINT('Ctrl Pts',(7.84370025199994,11.6,-8.12883240500001));
#173727=CARTESIAN_POINT('Ctrl Pts',(7.84698536499994,15.2,-8.13017403400002));
#173728=CARTESIAN_POINT('Ctrl Pts',(7.84698536499994,11.6,-8.13017403400002));
#173729=CARTESIAN_POINT('Ctrl Pts',(7.85027586699995,15.2,-8.13151487800001));
#173730=CARTESIAN_POINT('Ctrl Pts',(7.85027586699995,11.6,-8.13151487800001));
#173731=CARTESIAN_POINT('Ctrl Pts',(7.85357174999994,15.2,-8.13285492700001));
#173732=CARTESIAN_POINT('Ctrl Pts',(7.85357174999994,11.6,-8.13285492700001));
#173733=CARTESIAN_POINT('Ctrl Pts',(7.85687300999995,15.2,-8.13419417300001));
#173734=CARTESIAN_POINT('Ctrl Pts',(7.85687300999995,11.6,-8.13419417300001));
#173735=CARTESIAN_POINT('Ctrl Pts',(7.86017964299995,15.2,-8.13553260800001));
#173736=CARTESIAN_POINT('Ctrl Pts',(7.86017964299995,11.6,-8.13553260800001));
#173737=CARTESIAN_POINT('Ctrl Pts',(7.86349164399994,15.2,-8.13687022200002));
#173738=CARTESIAN_POINT('Ctrl Pts',(7.86349164399994,11.6,-8.13687022200002));
#173739=CARTESIAN_POINT('Ctrl Pts',(7.86680900699994,15.2,-8.13820700800001));
#173740=CARTESIAN_POINT('Ctrl Pts',(7.86680900699994,11.6,-8.13820700800001));
#173741=CARTESIAN_POINT('Ctrl Pts',(7.87013172899995,15.2,-8.13954295600002));
#173742=CARTESIAN_POINT('Ctrl Pts',(7.87013172899995,11.6,-8.13954295600002));
#173743=CARTESIAN_POINT('Ctrl Pts',(7.87345980499994,15.2,-8.14087806000002));
#173744=CARTESIAN_POINT('Ctrl Pts',(7.87345980499994,11.6,-8.14087806000002));
#173745=CARTESIAN_POINT('Ctrl Pts',(7.87679322899994,15.2,-8.14221230900002));
#173746=CARTESIAN_POINT('Ctrl Pts',(7.87679322899994,11.6,-8.14221230900002));
#173747=CARTESIAN_POINT('Ctrl Pts',(7.88013199699995,15.2,-8.14354569700001));
#173748=CARTESIAN_POINT('Ctrl Pts',(7.88013199699995,11.6,-8.14354569700001));
#173749=CARTESIAN_POINT('Ctrl Pts',(7.88347610399994,15.2,-8.14487821400002));
#173750=CARTESIAN_POINT('Ctrl Pts',(7.88347610399994,11.6,-8.14487821400002));
#173751=CARTESIAN_POINT('Ctrl Pts',(7.88682554499994,15.2,-8.14620985200002));
#173752=CARTESIAN_POINT('Ctrl Pts',(7.88682554499994,11.6,-8.14620985200002));
#173753=CARTESIAN_POINT('Ctrl Pts',(7.89018031499995,15.2,-8.14754060400002));
#173754=CARTESIAN_POINT('Ctrl Pts',(7.89018031499995,11.6,-8.14754060400002));
#173755=CARTESIAN_POINT('Ctrl Pts',(7.89354040999994,15.2,-8.14887046000001));
#173756=CARTESIAN_POINT('Ctrl Pts',(7.89354040999994,11.6,-8.14887046000001));
#173757=CARTESIAN_POINT('Ctrl Pts',(7.89690582599994,15.2,-8.15019941300001));
#173758=CARTESIAN_POINT('Ctrl Pts',(7.89690582599994,11.6,-8.15019941300001));
#173759=CARTESIAN_POINT('Ctrl Pts',(7.90027655699994,15.2,-8.15152745300002));
#173760=CARTESIAN_POINT('Ctrl Pts',(7.90027655699994,11.6,-8.15152745300002));
#173761=CARTESIAN_POINT('Ctrl Pts',(7.90365259799994,15.2,-8.15285457300002));
#173762=CARTESIAN_POINT('Ctrl Pts',(7.90365259799994,11.6,-8.15285457300002));
#173763=CARTESIAN_POINT('Ctrl Pts',(7.90703394399995,15.2,-8.15418076500002));
#173764=CARTESIAN_POINT('Ctrl Pts',(7.90703394399995,11.6,-8.15418076500002));
#173765=CARTESIAN_POINT('Ctrl Pts',(7.91042059099994,15.2,-8.15550602000001));
#173766=CARTESIAN_POINT('Ctrl Pts',(7.91042059099994,11.6,-8.15550602000001));
#173767=CARTESIAN_POINT('Ctrl Pts',(7.91381253499994,15.2,-8.15683033100001));
#173768=CARTESIAN_POINT('Ctrl Pts',(7.91381253499994,11.6,-8.15683033100001));
#173769=CARTESIAN_POINT('Ctrl Pts',(7.91720976999994,15.2,-8.15815368900001));
#173770=CARTESIAN_POINT('Ctrl Pts',(7.91720976999994,11.6,-8.15815368900001));
#173771=CARTESIAN_POINT('Ctrl Pts',(7.92061229099994,15.2,-8.15947608600002));
#173772=CARTESIAN_POINT('Ctrl Pts',(7.92061229099994,11.6,-8.15947608600002));
#173773=CARTESIAN_POINT('Ctrl Pts',(7.92402009399995,15.2,-8.16079751400002));
#173774=CARTESIAN_POINT('Ctrl Pts',(7.92402009399995,11.6,-8.16079751400002));
#173775=CARTESIAN_POINT('Ctrl Pts',(7.92743317499994,15.2,-8.16211796400001));
#173776=CARTESIAN_POINT('Ctrl Pts',(7.92743317499994,11.6,-8.16211796400001));
#173777=CARTESIAN_POINT('Ctrl Pts',(7.93085152599994,15.2,-8.16343743000001));
#173778=CARTESIAN_POINT('Ctrl Pts',(7.93085152599994,11.6,-8.16343743000001));
#173779=CARTESIAN_POINT('Ctrl Pts',(7.93427514599994,15.2,-8.16475590100002));
#173780=CARTESIAN_POINT('Ctrl Pts',(7.93427514599994,11.6,-8.16475590100002));
#173781=CARTESIAN_POINT('Ctrl Pts',(7.93770402899994,15.2,-8.16607337100002));
#173782=CARTESIAN_POINT('Ctrl Pts',(7.93770402899994,11.6,-8.16607337100002));
#173783=CARTESIAN_POINT('Ctrl Pts',(7.94113816999995,15.2,-8.16738983200001));
#173784=CARTESIAN_POINT('Ctrl Pts',(7.94113816999995,11.6,-8.16738983200001));
#173785=CARTESIAN_POINT('Ctrl Pts',(7.94457756299995,15.2,-8.16870527600001));
#173786=CARTESIAN_POINT('Ctrl Pts',(7.94457756299995,11.6,-8.16870527600001));
#173787=CARTESIAN_POINT('Ctrl Pts',(7.94802220599995,15.2,-8.17001969300001));
#173788=CARTESIAN_POINT('Ctrl Pts',(7.94802220599995,11.6,-8.17001969300001));
#173789=CARTESIAN_POINT('Ctrl Pts',(7.95147209099994,15.2,-8.17133307700002));
#173790=CARTESIAN_POINT('Ctrl Pts',(7.95147209099994,11.6,-8.17133307700002));
#173791=CARTESIAN_POINT('Ctrl Pts',(7.95492721599994,15.2,-8.17264542000002));
#173792=CARTESIAN_POINT('Ctrl Pts',(7.95492721599994,11.6,-8.17264542000002));
#173793=CARTESIAN_POINT('Ctrl Pts',(7.95838757499994,15.2,-8.17395671300002));
#173794=CARTESIAN_POINT('Ctrl Pts',(7.95838757499994,11.6,-8.17395671300002));
#173795=CARTESIAN_POINT('Ctrl Pts',(7.96185316299994,15.2,-8.17526694900002));
#173796=CARTESIAN_POINT('Ctrl Pts',(7.96185316299994,11.6,-8.17526694900002));
#173797=CARTESIAN_POINT('Ctrl Pts',(7.96532397699995,15.2,-8.17657611900002));
#173798=CARTESIAN_POINT('Ctrl Pts',(7.96532397699995,11.6,-8.17657611900002));
#173799=CARTESIAN_POINT('Ctrl Pts',(7.96880000999994,15.2,-8.17788421800002));
#173800=CARTESIAN_POINT('Ctrl Pts',(7.96880000999994,11.6,-8.17788421800002));
#173801=CARTESIAN_POINT('Ctrl Pts',(7.97228125899994,15.2,-8.17919123400002));
#173802=CARTESIAN_POINT('Ctrl Pts',(7.97228125899994,11.6,-8.17919123400002));
#173803=CARTESIAN_POINT('Ctrl Pts',(7.97576771799994,15.2,-8.18049716300001));
#173804=CARTESIAN_POINT('Ctrl Pts',(7.97576771799994,11.6,-8.18049716300001));
#173805=CARTESIAN_POINT('Ctrl Pts',(7.97925938299994,15.2,-8.18180199500001));
#173806=CARTESIAN_POINT('Ctrl Pts',(7.97925938299994,11.6,-8.18180199500001));
#173807=CARTESIAN_POINT('Ctrl Pts',(7.98275624999994,15.2,-8.18310572200001));
#173808=CARTESIAN_POINT('Ctrl Pts',(7.98275624999994,11.6,-8.18310572200001));
#173809=CARTESIAN_POINT('Ctrl Pts',(7.98625831199994,15.2,-8.18440833600001));
#173810=CARTESIAN_POINT('Ctrl Pts',(7.98625831199994,11.6,-8.18440833600001));
#173811=CARTESIAN_POINT('Ctrl Pts',(7.98976556499994,15.2,-8.18570982900001));
#173812=CARTESIAN_POINT('Ctrl Pts',(7.98976556499994,11.6,-8.18570982900001));
#173813=CARTESIAN_POINT('Ctrl Pts',(7.99327800399994,15.2,-8.18701019200001));
#173814=CARTESIAN_POINT('Ctrl Pts',(7.99327800399994,11.6,-8.18701019200001));
#173815=CARTESIAN_POINT('Ctrl Pts',(7.99679562499994,15.2,-8.18830942000002));
#173816=CARTESIAN_POINT('Ctrl Pts',(7.99679562499994,11.6,-8.18830942000002));
#173817=CARTESIAN_POINT('Ctrl Pts',(8.00031842399994,15.2,-8.18960750500001));
#173818=CARTESIAN_POINT('Ctrl Pts',(8.00031842399994,11.6,-8.18960750500001));
#173819=CARTESIAN_POINT('Ctrl Pts',(8.00384639599995,15.2,-8.19090444000001));
#173820=CARTESIAN_POINT('Ctrl Pts',(8.00384639599995,11.6,-8.19090444000001));
#173821=CARTESIAN_POINT('Ctrl Pts',(8.00737953699995,15.2,-8.19220021800002));
#173822=CARTESIAN_POINT('Ctrl Pts',(8.00737953699995,11.6,-8.19220021800002));
#173823=CARTESIAN_POINT('Ctrl Pts',(8.01091784199994,15.2,-8.19349483100002));
#173824=CARTESIAN_POINT('Ctrl Pts',(8.01091784199994,11.6,-8.19349483100002));
#173825=CARTESIAN_POINT('Ctrl Pts',(8.01446130799994,15.2,-8.19478827200001));
#173826=CARTESIAN_POINT('Ctrl Pts',(8.01446130799994,11.6,-8.19478827200001));
#173827=CARTESIAN_POINT('Ctrl Pts',(8.01800992599994,15.2,-8.19608053200002));
#173828=CARTESIAN_POINT('Ctrl Pts',(8.01800992599994,11.6,-8.19608053200002));
#173829=CARTESIAN_POINT('Ctrl Pts',(8.02156369399994,15.2,-8.19737160100001));
#173830=CARTESIAN_POINT('Ctrl Pts',(8.02156369399994,11.6,-8.19737160100001));
#173831=CARTESIAN_POINT('Ctrl Pts',(8.02512260399994,15.2,-8.19866147000001));
#173832=CARTESIAN_POINT('Ctrl Pts',(8.02512260399994,11.6,-8.19866147000001));
#173833=CARTESIAN_POINT('Ctrl Pts',(8.02868665099994,15.2,-8.19995012900002));
#173834=CARTESIAN_POINT('Ctrl Pts',(8.02868665099994,11.6,-8.19995012900002));
#173835=CARTESIAN_POINT('Ctrl Pts',(8.03225582899995,15.2,-8.20123757100001));
#173836=CARTESIAN_POINT('Ctrl Pts',(8.03225582899995,11.6,-8.20123757100001));
#173837=CARTESIAN_POINT('Ctrl Pts',(8.03583013499994,15.2,-8.20252378800001));
#173838=CARTESIAN_POINT('Ctrl Pts',(8.03583013499994,11.6,-8.20252378800001));
#173839=CARTESIAN_POINT('Ctrl Pts',(8.03940956399994,15.2,-8.20380877500002));
#173840=CARTESIAN_POINT('Ctrl Pts',(8.03940956399994,11.6,-8.20380877500002));
#173841=CARTESIAN_POINT('Ctrl Pts',(8.04299411599994,15.2,-8.20509252900001));
#173842=CARTESIAN_POINT('Ctrl Pts',(8.04299411599994,11.6,-8.20509252900001));
#173843=CARTESIAN_POINT('Ctrl Pts',(8.04658378799994,15.2,-8.20637504800001));
#173844=CARTESIAN_POINT('Ctrl Pts',(8.04658378799994,11.6,-8.20637504800001));
#173845=CARTESIAN_POINT('Ctrl Pts',(8.04945962199995,15.2,-8.20740007500002));
#173846=CARTESIAN_POINT('Ctrl Pts',(8.04945962199995,11.6,-8.20740007500002));
#173847=CARTESIAN_POINT('Ctrl Pts',(8.05161880099994,15.2,-8.20816828800002));
#173848=CARTESIAN_POINT('Ctrl Pts',(8.05161880099994,11.6,-8.20816828800002));
#173849=CARTESIAN_POINT('Ctrl Pts',(8.05305927699994,15.2,-8.20868018400001));
#173850=CARTESIAN_POINT('Ctrl Pts',(8.05305927699994,11.6,-8.20868018400001));
#173851=CARTESIAN_POINT('Ctrl Pts',(8.05377977099995,15.2,-8.20893607000002));
#173852=CARTESIAN_POINT('Ctrl Pts',(8.05377977099995,11.6,-8.20893607000002));
#173853=CARTESIAN_POINT('Ctrl Pts',(7.01216898599994,15.2,-7.64657512400002));
#173854=CARTESIAN_POINT('Ctrl Pts',(7.01348522039998,15.2,-7.64778327244868));
#173855=CARTESIAN_POINT('Ctrl Pts',(7.0148472207803,15.2,-7.64902613336841));
#173856=CARTESIAN_POINT('Ctrl Pts',(7.01625467904572,15.2,-7.65030255165183));
#173857=CARTESIAN_POINT('Ctrl Pts',(7.01766892478633,15.2,-7.65158512546942));
#173858=CARTESIAN_POINT('Ctrl Pts',(7.01912907680239,15.2,-7.6529015883544));
#173859=CARTESIAN_POINT('Ctrl Pts',(7.02063486162897,15.2,-7.65425083033056));
#173860=CARTESIAN_POINT('Ctrl Pts',(7.0221406463188,15.2,-7.65560007218416));
#173861=CARTESIAN_POINT('Ctrl Pts',(7.0236920633662,15.2,-7.65698209165132));
#173862=CARTESIAN_POINT('Ctrl Pts',(7.02528884122486,15.2,-7.65839580976662));
#173863=CARTESIAN_POINT('Ctrl Pts',(7.02688561908352,15.2,-7.65980952788194));
#173864=CARTESIAN_POINT('Ctrl Pts',(7.02852775929139,15.1999999999999,-7.66125494592225));
#173865=CARTESIAN_POINT('Ctrl Pts',(7.03021499706176,15.2,-7.66273101410725));
#173866=CARTESIAN_POINT('Ctrl Pts',(7.03190223498539,15.2,-7.66420708242633));
#173867=CARTESIAN_POINT('Ctrl Pts',(7.03363456925201,15.2,-7.66571380189834));
#173868=CARTESIAN_POINT('Ctrl Pts',(7.03541173743525,15.2,-7.66725015515077));
#173869=CARTESIAN_POINT('Ctrl Pts',(7.03718890545706,15.2,-7.66878650826362));
#173870=CARTESIAN_POINT('Ctrl Pts',(7.03901091135163,15.2,-7.67035249414299));
#173871=CARTESIAN_POINT('Ctrl Pts',(7.04087749604239,15.2,-7.67194712350903));
#173872=CARTESIAN_POINT('Ctrl Pts',(7.04274408073314,15.2,-7.67354175287507));
#173873=CARTESIAN_POINT('Ctrl Pts',(7.04465524144143,15.2,-7.67516502671293));
#173874=CARTESIAN_POINT('Ctrl Pts',(7.04661073111848,15.2,-7.67681598040177));
#173875=CARTESIAN_POINT('Ctrl Pts',(7.04856622097314,15.2,-7.67846693424055));
#173876=CARTESIAN_POINT('Ctrl Pts',(7.0505660383916,15.2,-7.68014557138276));
#173877=CARTESIAN_POINT('Ctrl Pts',(7.052609930506,15.2,-7.68185095122753));
#173878=CARTESIAN_POINT('Ctrl Pts',(7.05465382243473,15.2,-7.68355633091739));
#173879=CARTESIAN_POINT('Ctrl Pts',(7.0567417943918,15.2,-7.68528845520865));
#173880=CARTESIAN_POINT('Ctrl Pts',(7.05887359714957,15.2,-7.68704641381255));
#173881=CARTESIAN_POINT('Ctrl Pts',(7.06100539990735,15.2,-7.68880437241647));
#173882=CARTESIAN_POINT('Ctrl Pts',(7.06318103490329,15.2,-7.69058816246829));
#173883=CARTESIAN_POINT('Ctrl Pts',(7.06540025990411,15.2,-7.6923968984015));
#173884=CARTESIAN_POINT('Ctrl Pts',(7.06761948490493,15.2,-7.69420563433471));
#173885=CARTESIAN_POINT('Ctrl Pts',(7.0698823003436,15.2,-7.69603931773329));
#173886=CARTESIAN_POINT('Ctrl Pts',(7.07218846800684,15.2,-7.69789707783082));
#173887=CARTESIAN_POINT('Ctrl Pts',(7.07449463587956,15.2,-7.69975483809708));
#173888=CARTESIAN_POINT('Ctrl Pts',(7.07684415358985,15.2,-7.70163667853241));
#173889=CARTESIAN_POINT('Ctrl Pts',(7.07923678863878,15.2,-7.70354175580389));
#173890=CARTESIAN_POINT('Ctrl Pts',(7.08162942347036,15.2,-7.70544683290233));
#173891=CARTESIAN_POINT('Ctrl Pts',(7.08406517439433,15.2,-7.70737514680284));
#173892=CARTESIAN_POINT('Ctrl Pts',(7.08654380831541,15.2,-7.70932587299076));
#173893=CARTESIAN_POINT('Ctrl Pts',(7.0890224422365,15.2,-7.71127659917867));
#173894=CARTESIAN_POINT('Ctrl Pts',(7.09154395894146,15.2,-7.71324973923985));
#173895=CARTESIAN_POINT('Ctrl Pts',(7.09410812976205,15.2,-7.71524449049922));
#173896=CARTESIAN_POINT('Ctrl Pts',(7.09667230081556,15.2,-7.7172392419398));
#173897=CARTESIAN_POINT('Ctrl Pts',(7.09927912588989,15.2,-7.71925560495751));
#173898=CARTESIAN_POINT('Ctrl Pts',(7.10192837511943,15.2,-7.72129279365276));
#173899=CARTESIAN_POINT('Ctrl Pts',(7.10457762410833,15.2,-7.72332998216297));
#173900=CARTESIAN_POINT('Ctrl Pts',(7.10726930113564,15.2,-7.72538800047348));
#173901=CARTESIAN_POINT('Ctrl Pts',(7.11000317804863,15.2,-7.72746607899071));
#173902=CARTESIAN_POINT('Ctrl Pts',(7.11273705496164,15.2,-7.72954415750794));
#173903=CARTESIAN_POINT('Ctrl Pts',(7.11551313393964,15.2,-7.73164229980578));
#173904=CARTESIAN_POINT('Ctrl Pts',(7.11833118991771,15.2,-7.73375975631085));
#173905=CARTESIAN_POINT('Ctrl Pts',(7.12114924615177,15.2,-7.73587721300827));
#173906=CARTESIAN_POINT('Ctrl Pts',(7.12400928121682,15.2,-7.73801398467397));
#173907=CARTESIAN_POINT('Ctrl Pts',(7.12691107627235,15.2,-7.74016934248353));
#173908=CARTESIAN_POINT('Ctrl Pts',(7.12981287106431,15.2,-7.7423247000973));
#173909=CARTESIAN_POINT('Ctrl Pts',(7.13275642209166,15.2,-7.74449864123796));
#173910=CARTESIAN_POINT('Ctrl Pts',(7.1357415149832,15.2,-7.74669045474165));
#173911=CARTESIAN_POINT('Ctrl Pts',(7.13922412353743,15.2,-7.74924757062868));
#173912=CARTESIAN_POINT('Ctrl Pts',(7.14276327322082,15.2,-7.75182900945527));
#173913=CARTESIAN_POINT('Ctrl Pts',(7.14635862055642,15.2,-7.75443366743267));
#173914=CARTESIAN_POINT('Ctrl Pts',(7.14944034668413,15.2,-7.75666623129739));
#173915=CARTESIAN_POINT('Ctrl Pts',(7.15256336090648,15.2,-7.75891585329897));
#173916=CARTESIAN_POINT('Ctrl Pts',(7.1557274507082,15.2,-7.76118185404998));
#173917=CARTESIAN_POINT('Ctrl Pts',(7.15889154050992,15.2,-7.763447854801));
#173918=CARTESIAN_POINT('Ctrl Pts',(7.16209670506911,15.2,-7.76573023257232));
#173919=CARTESIAN_POINT('Ctrl Pts',(7.16534273219429,15.2,-7.76802832451938));
#173920=CARTESIAN_POINT('Ctrl Pts',(7.16804775489691,15.2,-7.76994340121152));
#173921=CARTESIAN_POINT('Ctrl Pts',(7.17078115538202,15.2,-7.77186938930173));
#173922=CARTESIAN_POINT('Ctrl Pts',(7.17354281051943,15.2,-7.77380591110674));
#173923=CARTESIAN_POINT('Ctrl Pts',(7.17630446565684,15.2,-7.77574243291174));
#173924=CARTESIAN_POINT('Ctrl Pts',(7.17909437698944,15.2,-7.77768948970035));
#173925=CARTESIAN_POINT('Ctrl Pts',(7.18191242205741,15.2,-7.77964670963038));
#173926=CARTESIAN_POINT('Ctrl Pts',(7.18473046712538,15.2,-7.7816039295604));
#173927=CARTESIAN_POINT('Ctrl Pts',(7.18757664829089,15.2,-7.78357131208995));
#173928=CARTESIAN_POINT('Ctrl Pts',(7.19045084253998,15.2,-7.78554849376558));
#173929=CARTESIAN_POINT('Ctrl Pts',(7.19332503678907,15.2,-7.78752567544121));
#173930=CARTESIAN_POINT('Ctrl Pts',(7.19622724572209,15.2,-7.78951265435554));
#173931=CARTESIAN_POINT('Ctrl Pts',(7.1991573499582,15.2,-7.79150907504999));
#173932=CARTESIAN_POINT('Ctrl Pts',(7.20208745419431,15.2,-7.79350549574444));
#173933=CARTESIAN_POINT('Ctrl Pts',(7.20504545320452,15.2,-7.79551135381969));
#173934=CARTESIAN_POINT('Ctrl Pts',(7.20803123050984,15.2,-7.79752630146776));
#173935=CARTESIAN_POINT('Ctrl Pts',(7.21101700781514,15.2,-7.79954124911583));
#173936=CARTESIAN_POINT('Ctrl Pts',(7.21403055872527,15.2,-7.80156528312143));
#173937=CARTESIAN_POINT('Ctrl Pts',(7.21707177115727,15.2,-7.80359805985799));
#173938=CARTESIAN_POINT('Ctrl Pts',(7.22011298358927,15.2,-7.80563083659455));
#173939=CARTESIAN_POINT('Ctrl Pts',(7.22318185372334,15.2,-7.80767235337257));
#173940=CARTESIAN_POINT('Ctrl Pts',(7.22627826691921,15.2,-7.80972227115078));
#173941=CARTESIAN_POINT('Ctrl Pts',(7.22937468011509,15.2,-7.81177218892899));
#173942=CARTESIAN_POINT('Ctrl Pts',(7.232498633412,15.2,-7.81383050583054));
#173943=CARTESIAN_POINT('Ctrl Pts',(7.2356500136408,15.2,-7.8158968902399));
#173944=CARTESIAN_POINT('Ctrl Pts',(7.2388013938696,15.2,-7.81796327464925));
#173945=CARTESIAN_POINT('Ctrl Pts',(7.24198019768924,15.2,-7.82003772281617));
#173946=CARTESIAN_POINT('Ctrl Pts',(7.24518631192758,15.2,-7.82211990649735));
#173947=CARTESIAN_POINT('Ctrl Pts',(7.24839242616592,15.2,-7.82420209017854));
#173948=CARTESIAN_POINT('Ctrl Pts',(7.25162585030193,15.2,-7.8262920095904));
#173949=CARTESIAN_POINT('Ctrl Pts',(7.25488646794304,15.2,-7.82838934000766));
#173950=CARTESIAN_POINT('Ctrl Pts',(7.25814708522875,15.2,-7.83048667019634));
#173951=CARTESIAN_POINT('Ctrl Pts',(7.26143489795205,15.2,-7.83259141059899));
#173952=CARTESIAN_POINT('Ctrl Pts',(7.26474978932463,15.2,-7.83470324321544));
#173953=CARTESIAN_POINT('Ctrl Pts',(7.26806468105854,15.2,-7.83681507606209));
#173954=CARTESIAN_POINT('Ctrl Pts',(7.27140665252256,15.2,-7.83893400037807));
#173955=CARTESIAN_POINT('Ctrl Pts',(7.27477558932589,15.2,-7.84105970169696));
#173956=CARTESIAN_POINT('Ctrl Pts',(7.27881831371023,15.2,-7.84361054341864));
#173957=CARTESIAN_POINT('Ctrl Pts',(7.28289986889003,15.2,-7.84617114590798));
#173958=CARTESIAN_POINT('Ctrl Pts',(7.28702005819959,15.2,-7.84874097163176));
#173959=CARTESIAN_POINT('Ctrl Pts',(7.29045354910377,15.2,-7.85088249295154));
#173960=CARTESIAN_POINT('Ctrl Pts',(7.29391387020648,15.2,-7.85303042183648));
#173961=CARTESIAN_POINT('Ctrl Pts',(7.2974009071881,15.2,-7.85518445250007));
#173962=CARTESIAN_POINT('Ctrl Pts',(7.30088794416971,15.2,-7.85733848316366));
#173963=CARTESIAN_POINT('Ctrl Pts',(7.30440169836636,15.2,-7.85949861731061));
#173964=CARTESIAN_POINT('Ctrl Pts',(7.30794205593796,15.2,-7.8616645545333));
#173965=CARTESIAN_POINT('Ctrl Pts',(7.3107743417637,15.2,-7.86339730416981));
#173966=CARTESIAN_POINT('Ctrl Pts',(7.31362365465114,15.2,-7.86513376828637));
#173967=CARTESIAN_POINT('Ctrl Pts',(7.31648993774905,15.2,-7.86687379586612));
#173968=CARTESIAN_POINT('Ctrl Pts',(7.31935622123749,15.2,-7.86861382368294));
#173969=CARTESIAN_POINT('Ctrl Pts',(7.32223947388583,15.2,-7.87035741397629));
#173970=CARTESIAN_POINT('Ctrl Pts',(7.32513963891247,15.2,-7.87210441927019));
#173971=CARTESIAN_POINT('Ctrl Pts',(7.32803980354397,15.2,-7.87385142432605));
#173972=CARTESIAN_POINT('Ctrl Pts',(7.33095688067336,15.2,-7.87560184292247));
#173973=CARTESIAN_POINT('Ctrl Pts',(7.33389081321019,15.2,-7.87735552789));
#173974=CARTESIAN_POINT('Ctrl Pts',(7.33682474614678,15.2,-7.87910921309649));
#173975=CARTESIAN_POINT('Ctrl Pts',(7.33977553461869,15.2,-7.88086616522557));
#173976=CARTESIAN_POINT('Ctrl Pts',(7.34274312222597,15.2,-7.88262623787725));
#173977=CARTESIAN_POINT('Ctrl Pts',(7.34571070942892,15.2,-7.88438631028913));
#173978=CARTESIAN_POINT('Ctrl Pts',(7.34869509506136,15.2,-7.88614950430848));
#173979=CARTESIAN_POINT('Ctrl Pts',(7.35169622363116,15.2,-7.88791567475207));
#173980=CARTESIAN_POINT('Ctrl Pts',(7.35469735260987,15.2,-7.88968184543631));
#173981=CARTESIAN_POINT('Ctrl Pts',(7.35771522422608,15.2,-7.89145099240646));
#173982=CARTESIAN_POINT('Ctrl Pts',(7.36074978128144,15.2,-7.89322297366989));
#173983=CARTESIAN_POINT('Ctrl Pts',(7.36378433792335,15.2,-7.89499495469188));
#173984=CARTESIAN_POINT('Ctrl Pts',(7.36683558060356,15.2,-7.89676977047163));
#173985=CARTESIAN_POINT('Ctrl Pts',(7.36990345373996,15.2,-7.89854727899272));
#173986=CARTESIAN_POINT('Ctrl Pts',(7.37450526407154,15.2,-7.90121354213762));
#173987=CARTESIAN_POINT('Ctrl Pts',(7.37914449107004,15.2,-7.90388586714569));
#173988=CARTESIAN_POINT('Ctrl Pts',(7.38382094847736,15.2,-7.90656378325908));
#173989=CARTESIAN_POINT('Ctrl Pts',(7.3877179961044,15.2,-7.9087953798986));
#173990=CARTESIAN_POINT('Ctrl Pts',(7.39164089426428,15.2,-7.91103086062592));
#173991=CARTESIAN_POINT('Ctrl Pts',(7.39558953926637,15.2,-7.91326995729288));
#173992=CARTESIAN_POINT('Ctrl Pts',(7.3987484550098,15.2,-7.91506123448001));
#173993=CARTESIAN_POINT('Ctrl Pts',(7.40192384672332,15.2,-7.91685482577517));
#173994=CARTESIAN_POINT('Ctrl Pts',(7.40511565923911,15.2,-7.91865059812822));
#173995=CARTESIAN_POINT('Ctrl Pts',(7.40830747218978,15.2,-7.92044637072596));
#173996=CARTESIAN_POINT('Ctrl Pts',(7.41151570710461,15.2,-7.92224432322578));
#173997=CARTESIAN_POINT('Ctrl Pts',(7.41474030694288,15.2,-7.92404432146954));
#173998=CARTESIAN_POINT('Ctrl Pts',(7.4179649063418,15.2,-7.92584431946806));
#173999=CARTESIAN_POINT('Ctrl Pts',(7.42120587123443,15.2,-7.92764636550015));
#174000=CARTESIAN_POINT('Ctrl Pts',(7.42446314696709,15.2,-7.92945032535255));
#174001=CARTESIAN_POINT('Ctrl Pts',(7.42772042314354,15.2,-7.93125428545074));
#174002=CARTESIAN_POINT('Ctrl Pts',(7.43099400907197,15.2,-7.93306016080194));
#174003=CARTESIAN_POINT('Ctrl Pts',(7.43428385125231,15.2,-7.9348678196228));
#174004=CARTESIAN_POINT('Ctrl Pts',(7.43839615375362,15.2,-7.93712739302571));
#174005=CARTESIAN_POINT('Ctrl Pts',(7.4425338536735,15.2,-7.93938975434406));
#174006=CARTESIAN_POINT('Ctrl Pts',(7.44669684721657,15.2,-7.94165465272127));
#174007=CARTESIAN_POINT('Ctrl Pts',(7.45002724177875,15.2,-7.94346657127492));
#174008=CARTESIAN_POINT('Ctrl Pts',(7.45337382243719,15.2,-7.94528011225012));
#174009=CARTESIAN_POINT('Ctrl Pts',(7.4567365362168,15.2,-7.94709515010164));
#174010=CARTESIAN_POINT('Ctrl Pts',(7.46009925045458,15.2,-7.94891018820047));
#174011=CARTESIAN_POINT('Ctrl Pts',(7.46347809617761,15.2,-7.95072672205225));
#174012=CARTESIAN_POINT('Ctrl Pts',(7.46687301975257,15.2,-7.95254462620697));
#174013=CARTESIAN_POINT('Ctrl Pts',(7.47026794286497,15.2,-7.954362530114));
#174014=CARTESIAN_POINT('Ctrl Pts',(7.47367894241303,15.2,-7.95618180382438));
#174015=CARTESIAN_POINT('Ctrl Pts',(7.47710596630269,15.2,-7.95800232371085));
#174016=CARTESIAN_POINT('Ctrl Pts',(7.48053299065928,15.2,-7.95982284384536));
#174017=CARTESIAN_POINT('Ctrl Pts',(7.48397603776546,15.2,-7.96164460979129));
#174018=CARTESIAN_POINT('Ctrl Pts',(7.48743505406614,15.2,-7.96346749739071));
#174019=CARTESIAN_POINT('Ctrl Pts',(7.49089406989552,15.2,-7.96529038474176));
#174020=CARTESIAN_POINT('Ctrl Pts',(7.49436905406058,15.2,-7.96711439526759));
#174021=CARTESIAN_POINT('Ctrl Pts',(7.49785995266246,15.2,-7.96893940645163));
#174022=CARTESIAN_POINT('Ctrl Pts',(7.50135085173997,15.2,-7.97076441788432));
#174023=CARTESIAN_POINT('Ctrl Pts',(7.50485766650815,15.2,-7.9725904296684));
#174024=CARTESIAN_POINT('Ctrl Pts',(7.50838034199395,15.2,-7.97441732127625));
#174025=CARTESIAN_POINT('Ctrl Pts',(7.51190301699978,15.2,-7.9762442126352));
#174026=CARTESIAN_POINT('Ctrl Pts',(7.51544155081094,15.2,-7.97807198345061));
#174027=CARTESIAN_POINT('Ctrl Pts',(7.51899589318542,15.2,-7.97990051596771));
#174028=CARTESIAN_POINT('Ctrl Pts',(7.52255023604418,15.2,-7.98172904873396));
#174029=CARTESIAN_POINT('Ctrl Pts',(7.52612038429057,15.2,-7.98355834170584));
#174030=CARTESIAN_POINT('Ctrl Pts',(7.52970628654155,15.2,-7.98538827725001));
#174031=CARTESIAN_POINT('Ctrl Pts',(7.53418866411098,15.2,-7.98767569655557));
#174032=CARTESIAN_POINT('Ctrl Pts',(7.53869565397767,15.2,-7.98996411995003));
#174033=CARTESIAN_POINT('Ctrl Pts',(7.54322715494988,15.2,-7.99225331849168));
#174034=CARTESIAN_POINT('Ctrl Pts',(7.54685235592522,15.2,-7.99408467742482));
#174035=CARTESIAN_POINT('Ctrl Pts',(7.5504932419663,15.2,-7.99591653310803));
#174036=CARTESIAN_POINT('Ctrl Pts',(7.5541497608894,15.2,-7.99774877004125));
#174037=CARTESIAN_POINT('Ctrl Pts',(7.5578062793143,15.2,-7.99958100672483));
#174038=CARTESIAN_POINT('Ctrl Pts',(7.56147842973493,15.2,-8.00141362508195));
#174039=CARTESIAN_POINT('Ctrl Pts',(7.56516615950571,15.2,-8.00324650977377));
#174040=CARTESIAN_POINT('Ctrl Pts',(7.56885388977894,15.2,-8.00507939471531));
#174041=CARTESIAN_POINT('Ctrl Pts',(7.57255719835921,15.2,-8.00691254635538));
#174042=CARTESIAN_POINT('Ctrl Pts',(7.57627603334126,15.2,-8.00874585256643));
#174043=CARTESIAN_POINT('Ctrl Pts',(7.58092457681545,15.2,-8.01103748520534));
#174044=CARTESIAN_POINT('Ctrl Pts',(7.58559737906784,15.2,-8.01332935810536));
#174045=CARTESIAN_POINT('Ctrl Pts',(7.59029433663925,15.2,-8.01562125254979));
#174046=CARTESIAN_POINT('Ctrl Pts',(7.5940519023892,15.2,-8.01745476795546));
#174047=CARTESIAN_POINT('Ctrl Pts',(7.59782492616485,15.2,-8.01928829830977));
#174048=CARTESIAN_POINT('Ctrl Pts',(7.60161335670564,15.2,-8.02112173122377));
#174049=CARTESIAN_POINT('Ctrl Pts',(7.6054017877626,15.2,-8.02295516438757));
#174050=CARTESIAN_POINT('Ctrl Pts',(7.60920562595072,15.2,-8.0247885025054));
#174051=CARTESIAN_POINT('Ctrl Pts',(7.61302481688267,15.2,-8.02662163404973));
#174052=CARTESIAN_POINT('Ctrl Pts',(7.61684400729424,15.2,-8.0284547653443));
#174053=CARTESIAN_POINT('Ctrl Pts',(7.62067855032046,15.2,-8.03028769017776));
#174054=CARTESIAN_POINT('Ctrl Pts',(7.62452839472697,15.2,-8.03212030158353));
#174055=CARTESIAN_POINT('Ctrl Pts',(7.62837823965803,15.2,-8.033952913239));
#174056=CARTESIAN_POINT('Ctrl Pts',(7.63224338392581,15.2,-8.0357852113995));
#174057=CARTESIAN_POINT('Ctrl Pts',(7.63612377705471,15.2,-8.0376170877575));
#174058=CARTESIAN_POINT('Ctrl Pts',(7.64000416965489,15.2,-8.03944896386589));
#174059=CARTESIAN_POINT('Ctrl Pts',(7.64389980889269,15.2,-8.04128041761109));
#174060=CARTESIAN_POINT('Ctrl Pts',(7.64781064340532,15.2,-8.04311134435034));
#174061=CARTESIAN_POINT('Ctrl Pts',(7.65172147845082,15.2,-8.04494227133905));
#174062=CARTESIAN_POINT('Ctrl Pts',(7.65564750900921,15.2,-8.04677267072491));
#174063=CARTESIAN_POINT('Ctrl Pts',(7.65958868261389,15.2,-8.04860243765793));
#174064=CARTESIAN_POINT('Ctrl Pts',(7.66352985568157,15.2,-8.05043220434163));
#174065=CARTESIAN_POINT('Ctrl Pts',(7.66748616990403,15.2,-8.05226133700944));
#174066=CARTESIAN_POINT('Ctrl Pts',(7.67145757516536,15.2,-8.0540897332847));
#174067=CARTESIAN_POINT('Ctrl Pts',(7.67542898096779,15.2,-8.05591812980909));
#174068=CARTESIAN_POINT('Ctrl Pts',(7.67941547718586,15.2,-8.05774578974429));
#174069=CARTESIAN_POINT('Ctrl Pts',(7.68341701029382,15.2,-8.05957260939935));
#174070=CARTESIAN_POINT('Ctrl Pts',(7.68741854285656,15.2,-8.06139942880551));
#174071=CARTESIAN_POINT('Ctrl Pts',(7.69143511387739,15.2,-8.06322540671183));
#174072=CARTESIAN_POINT('Ctrl Pts',(7.69546667032407,15.2,-8.06505044345163));
#174073=CARTESIAN_POINT('Ctrl Pts',(7.69949822732004,15.2,-8.06687548044008));
#174074=CARTESIAN_POINT('Ctrl Pts',(7.70354477009058,15.2,-8.06869957497418));
#174075=CARTESIAN_POINT('Ctrl Pts',(7.70760624521932,15.2,-8.07052262602626));
#174076=CARTESIAN_POINT('Ctrl Pts',(7.71166771979469,15.2,-8.07234567682996));
#174077=CARTESIAN_POINT('Ctrl Pts',(7.71574412950861,15.2,-8.07416768306215));
#174078=CARTESIAN_POINT('Ctrl Pts',(7.7198354193393,15.2,-8.07598854646898));
#174079=CARTESIAN_POINT('Ctrl Pts',(7.72290388740911,15.2,-8.07735419433421));
#174080=CARTESIAN_POINT('Ctrl Pts',(7.72598072637295,15.2,-8.07871919913259));
#174081=CARTESIAN_POINT('Ctrl Pts',(7.72906591394746,15.2,-8.08008351803911));
#174082=CARTESIAN_POINT('Ctrl Pts',(7.7321511009615,15.2,-8.08144783669778));
#174083=CARTESIAN_POINT('Ctrl Pts',(7.73524463656677,15.2,-8.08281146929815));
#174084=CARTESIAN_POINT('Ctrl Pts',(7.73834649953813,15.2,-8.08417437591523));
#174085=CARTESIAN_POINT('Ctrl Pts',(7.74144836250949,15.2,-8.08553728253232));
#174086=CARTESIAN_POINT('Ctrl Pts',(7.74455855253516,15.2,-8.08689946147788));
#174087=CARTESIAN_POINT('Ctrl Pts',(7.74767704701939,15.2,-8.08826087222626));
#174088=CARTESIAN_POINT('Ctrl Pts',(7.75183503947618,15.2,-8.09007608647499));
#174089=CARTESIAN_POINT('Ctrl Pts',(7.75600779751741,15.2,-8.09188993544337));
#174090=CARTESIAN_POINT('Ctrl Pts',(7.76019526734024,15.2,-8.09370232146203));
#174091=CARTESIAN_POINT('Ctrl Pts',(7.76333587042055,15.2,-8.09506161128469));
#174092=CARTESIAN_POINT('Ctrl Pts',(7.76648474912819,15.2,-8.09642007686546));
#174093=CARTESIAN_POINT('Ctrl Pts',(7.76964188221315,15.2,-8.09777767931265));
#174094=CARTESIAN_POINT('Ctrl Pts',(7.77279901472456,15.2,-8.0991352815132));
#174095=CARTESIAN_POINT('Ctrl Pts',(7.77596440179388,15.2,-8.10049202014713));
#174096=CARTESIAN_POINT('Ctrl Pts',(7.77913802034595,15.2,-8.10184785484779));
#174097=CARTESIAN_POINT('Ctrl Pts',(7.78231163889802,15.2,-8.10320368954846));
#174098=CARTESIAN_POINT('Ctrl Pts',(7.7854934897375,15.2,-8.10455862031097));
#174099=CARTESIAN_POINT('Ctrl Pts',(7.78868355171945,15.2,-8.10591260651792));
#174100=CARTESIAN_POINT('Ctrl Pts',(7.79187361370141,15.2,-8.10726659272487));
#174101=CARTESIAN_POINT('Ctrl Pts',(7.79507188673229,15.2,-8.1086196342751));
#174102=CARTESIAN_POINT('Ctrl Pts',(7.79827834775531,15.2,-8.10997169244046));
#174103=CARTESIAN_POINT('Ctrl Pts',(7.80148480877833,15.2,-8.11132375060581));
#174104=CARTESIAN_POINT('Ctrl Pts',(7.80469945859988,15.2,-8.11267482453515));
#174105=CARTESIAN_POINT('Ctrl Pts',(7.80792227510707,15.2,-8.11402487511118));
#174106=CARTESIAN_POINT('Ctrl Pts',(7.81114509161427,15.2,-8.11537492568722));
#174107=CARTESIAN_POINT('Ctrl Pts',(7.8143760758959,15.2,-8.11672395137166));
#174108=CARTESIAN_POINT('Ctrl Pts',(7.81761520536043,15.2,-8.11807191503117));
#174109=CARTESIAN_POINT('Ctrl Pts',(7.82085433541341,15.2,-8.11941987893555));
#174110=CARTESIAN_POINT('Ctrl Pts',(7.82410161060201,15.2,-8.12076677956464));
#174111=CARTESIAN_POINT('Ctrl Pts',(7.82735700970124,15.2,-8.12211257855174));
#174112=CARTESIAN_POINT('Ctrl Pts',(7.83061240820906,15.2,-8.12345837729435));
#174113=CARTESIAN_POINT('Ctrl Pts',(7.83387593048743,15.2,-8.12480307394178));
#174114=CARTESIAN_POINT('Ctrl Pts',(7.83714755511628,15.2,-8.12614663025162));
#174115=CARTESIAN_POINT('Ctrl Pts',(7.84041917974513,15.2,-8.12749018656146));
#174116=CARTESIAN_POINT('Ctrl Pts',(7.84369890559382,15.2,-8.12883260207837));
#174117=CARTESIAN_POINT('Ctrl Pts',(7.84698671255839,15.2,-8.13017383786286));
#174118=CARTESIAN_POINT('Ctrl Pts',(7.85027451952297,15.2,-8.13151507364736));
#174119=CARTESIAN_POINT('Ctrl Pts',(7.8535704072366,15.2,-8.132855130532));
#174120=CARTESIAN_POINT('Ctrl Pts',(7.85687435324155,15.2,-8.13419397023335));
#174121=CARTESIAN_POINT('Ctrl Pts',(7.86127961498163,15.2,-8.13597908999731));
#174122=CARTESIAN_POINT('Ctrl Pts',(7.86569920325117,15.2,-8.13776204476379));
#174123=CARTESIAN_POINT('Ctrl Pts',(7.8701330682165,15.2,-8.1395427452495));
#174124=CARTESIAN_POINT('Ctrl Pts',(7.87345846663844,15.2,-8.14087827049248));
#174125=CARTESIAN_POINT('Ctrl Pts',(7.87679189515162,15.2,-8.14221252771051));
#174126=CARTESIAN_POINT('Ctrl Pts',(7.88013333211424,15.2,-8.14354547941196));
#174127=CARTESIAN_POINT('Ctrl Pts',(7.88347476907685,15.2,-8.1448784311134));
#174128=CARTESIAN_POINT('Ctrl Pts',(7.88682421419297,15.2,-8.14621007677687));
#174129=CARTESIAN_POINT('Ctrl Pts',(7.89018164625294,15.2,-8.14754038002623));
#174130=CARTESIAN_POINT('Ctrl Pts',(7.89353907831292,15.2,-8.1488706832756));
#174131=CARTESIAN_POINT('Ctrl Pts',(7.89690449902077,15.2,-8.15019964365768));
#174132=CARTESIAN_POINT('Ctrl Pts',(7.90027788449683,15.2,-8.15152722299049));
#174133=CARTESIAN_POINT('Ctrl Pts',(7.90365126997288,15.2,-8.15285480232329));
#174134=CARTESIAN_POINT('Ctrl Pts',(7.90703261990442,15.2,-8.15418100155361));
#174135=CARTESIAN_POINT('Ctrl Pts',(7.91042191486392,15.2,-8.15550578383893));
#174136=CARTESIAN_POINT('Ctrl Pts',(7.91381120982342,15.2,-8.15683056612426));
#174137=CARTESIAN_POINT('Ctrl Pts',(7.9172084492157,15.2,-8.15815393170967));
#174138=CARTESIAN_POINT('Ctrl Pts',(7.92061361075757,15.2,-8.15947584345351));
#174139=CARTESIAN_POINT('Ctrl Pts',(7.92401877291804,15.2,-8.1607977554375));
#174140=CARTESIAN_POINT('Ctrl Pts',(7.92743185824741,15.2,-8.16211821359607));
#174141=CARTESIAN_POINT('Ctrl Pts',(7.93085284395401,15.2,-8.16343718157922));
#174142=CARTESIAN_POINT('Ctrl Pts',(7.93427382903912,15.2,-8.16475614932277));
#174143=CARTESIAN_POINT('Ctrl Pts',(7.93770271698383,15.2,-8.16607362622019));
#174144=CARTESIAN_POINT('Ctrl Pts',(7.94113948369823,15.2,-8.16738957798795));
#174145=CARTESIAN_POINT('Ctrl Pts',(7.94457625041264,15.2,-8.1687055297557));
#174146=CARTESIAN_POINT('Ctrl Pts',(7.94802089680109,15.2,-8.17001995414094));
#174147=CARTESIAN_POINT('Ctrl Pts',(7.95147340134301,15.2,-8.17133281688477));
#174148=CARTESIAN_POINT('Ctrl Pts',(7.95492590588493,15.2,-8.1726456796286));
#174149=CARTESIAN_POINT('Ctrl Pts',(7.95838626900923,15.2,-8.17395698016428));
#174150=CARTESIAN_POINT('Ctrl Pts',(7.96185446946655,15.2,-8.17526668253336));
#174151=CARTESIAN_POINT('Ctrl Pts',(7.96532266992388,15.2,-8.17657638490244));
#174152=CARTESIAN_POINT('Ctrl Pts',(7.96879870768088,15.2,-8.17788449018826));
#174153=CARTESIAN_POINT('Ctrl Pts',(7.97228256113695,15.2,-8.17919096205759));
#174154=CARTESIAN_POINT('Ctrl Pts',(7.97576641459302,15.2,-8.18049743392693));
#174155=CARTESIAN_POINT('Ctrl Pts',(7.97925808400946,15.2,-8.18180227364659));
#174156=CARTESIAN_POINT('Ctrl Pts',(7.98275754809791,15.2,-8.18310544349788));
#174157=CARTESIAN_POINT('Ctrl Pts',(7.98742350063965,15.2,-8.18484300345741));
#174158=CARTESIAN_POINT('Ctrl Pts',(7.99210330678536,15.2,-8.18657759313905));
#174159=CARTESIAN_POINT('Ctrl Pts',(7.99679691987539,15.2,-8.18830913439989));
#174160=CARTESIAN_POINT('Ctrl Pts',(8.00031712937317,15.2,-8.18960779022755));
#174161=CARTESIAN_POINT('Ctrl Pts',(8.00384510547836,15.2,-8.19090473193042));
#174162=CARTESIAN_POINT('Ctrl Pts',(8.00738082801655,15.2,-8.19219992675836));
#174163=CARTESIAN_POINT('Ctrl Pts',(8.01091655055476,15.2,-8.19349512158631));
#174164=CARTESIAN_POINT('Ctrl Pts',(8.0144600206093,15.2,-8.19478857045598));
#174165=CARTESIAN_POINT('Ctrl Pts',(8.01801121306294,15.2,-8.19608023411754));
#174166=CARTESIAN_POINT('Ctrl Pts',(8.02156240551658,15.2,-8.1973718977791));
#174167=CARTESIAN_POINT('Ctrl Pts',(8.02512132091221,15.2,-8.19866177459971));
#174168=CARTESIAN_POINT('Ctrl Pts',(8.02868793308492,15.2,-8.19994982449247));
#174169=CARTESIAN_POINT('Ctrl Pts',(8.03225454525763,15.2,-8.20123787438524));
#174170=CARTESIAN_POINT('Ctrl Pts',(8.03582885370021,15.2,-8.20252409623311));
#174171=CARTESIAN_POINT('Ctrl Pts',(8.03941084394403,15.2,-8.20380846647837));
#174172=CARTESIAN_POINT('Ctrl Pts',(8.04418683136959,15.2,-8.20552096029426));
#174173=CARTESIAN_POINT('Ctrl Pts',(8.04897647635771,15.2,-8.20723016286848));
#174174=CARTESIAN_POINT('Ctrl Pts',(8.05377977099995,15.2,-8.20893607000002));
#174175=CARTESIAN_POINT('Ctrl Pts',(7.01216898599994,12.2,-7.64657512400002));
#174176=CARTESIAN_POINT('Ctrl Pts',(7.01348522039998,12.2,-7.64778327244868));
#174177=CARTESIAN_POINT('Ctrl Pts',(7.0148472207803,12.2,-7.64902613336841));
#174178=CARTESIAN_POINT('Ctrl Pts',(7.01625467904572,12.2,-7.65030255165183));
#174179=CARTESIAN_POINT('Ctrl Pts',(7.01766892478633,12.2,-7.65158512546942));
#174180=CARTESIAN_POINT('Ctrl Pts',(7.01912907680239,12.2,-7.6529015883544));
#174181=CARTESIAN_POINT('Ctrl Pts',(7.02063486162897,12.2,-7.65425083033056));
#174182=CARTESIAN_POINT('Ctrl Pts',(7.0221406463188,12.2,-7.65560007218416));
#174183=CARTESIAN_POINT('Ctrl Pts',(7.0236920633662,12.2,-7.65698209165132));
#174184=CARTESIAN_POINT('Ctrl Pts',(7.02528884122486,12.2,-7.65839580976662));
#174185=CARTESIAN_POINT('Ctrl Pts',(7.02688561908352,12.2,-7.65980952788194));
#174186=CARTESIAN_POINT('Ctrl Pts',(7.02852775929138,12.2,-7.66125494592225));
#174187=CARTESIAN_POINT('Ctrl Pts',(7.03021499706176,12.2,-7.66273101410724));
#174188=CARTESIAN_POINT('Ctrl Pts',(7.03190223498538,12.2,-7.66420708242633));
#174189=CARTESIAN_POINT('Ctrl Pts',(7.03363456925201,12.2,-7.66571380189834));
#174190=CARTESIAN_POINT('Ctrl Pts',(7.03541173743525,12.2,-7.66725015515077));
#174191=CARTESIAN_POINT('Ctrl Pts',(7.03718890545706,12.2,-7.66878650826362));
#174192=CARTESIAN_POINT('Ctrl Pts',(7.03901091135163,12.2,-7.67035249414299));
#174193=CARTESIAN_POINT('Ctrl Pts',(7.04087749604239,12.2,-7.67194712350903));
#174194=CARTESIAN_POINT('Ctrl Pts',(7.04274408073314,12.2,-7.67354175287507));
#174195=CARTESIAN_POINT('Ctrl Pts',(7.04465524144143,12.2,-7.67516502671293));
#174196=CARTESIAN_POINT('Ctrl Pts',(7.04661073111848,12.2,-7.67681598040177));
#174197=CARTESIAN_POINT('Ctrl Pts',(7.04856622097314,12.2,-7.67846693424055));
#174198=CARTESIAN_POINT('Ctrl Pts',(7.0505660383916,12.2,-7.68014557138276));
#174199=CARTESIAN_POINT('Ctrl Pts',(7.052609930506,12.2,-7.68185095122753));
#174200=CARTESIAN_POINT('Ctrl Pts',(7.05465382243473,12.2,-7.68355633091739));
#174201=CARTESIAN_POINT('Ctrl Pts',(7.0567417943918,12.2,-7.68528845520865));
#174202=CARTESIAN_POINT('Ctrl Pts',(7.05887359714957,12.2,-7.68704641381255));
#174203=CARTESIAN_POINT('Ctrl Pts',(7.06100539990735,12.2,-7.68880437241647));
#174204=CARTESIAN_POINT('Ctrl Pts',(7.06318103490329,12.2,-7.69058816246829));
#174205=CARTESIAN_POINT('Ctrl Pts',(7.06540025990411,12.2,-7.6923968984015));
#174206=CARTESIAN_POINT('Ctrl Pts',(7.06761948490493,12.2,-7.69420563433471));
#174207=CARTESIAN_POINT('Ctrl Pts',(7.0698823003436,12.2,-7.69603931773329));
#174208=CARTESIAN_POINT('Ctrl Pts',(7.07218846800684,12.2,-7.69789707783082));
#174209=CARTESIAN_POINT('Ctrl Pts',(7.07449463587956,12.2,-7.69975483809708));
#174210=CARTESIAN_POINT('Ctrl Pts',(7.07684415358985,12.2,-7.7016366785324));
#174211=CARTESIAN_POINT('Ctrl Pts',(7.07923678863878,12.2,-7.70354175580389));
#174212=CARTESIAN_POINT('Ctrl Pts',(7.08162942347036,12.2,-7.70544683290233));
#174213=CARTESIAN_POINT('Ctrl Pts',(7.08406517439434,12.2,-7.70737514680284));
#174214=CARTESIAN_POINT('Ctrl Pts',(7.08654380831542,12.2,-7.70932587299076));
#174215=CARTESIAN_POINT('Ctrl Pts',(7.0890224422365,12.2,-7.71127659917867));
#174216=CARTESIAN_POINT('Ctrl Pts',(7.09154395894146,12.2,-7.71324973923985));
#174217=CARTESIAN_POINT('Ctrl Pts',(7.09410812976205,12.2,-7.71524449049922));
#174218=CARTESIAN_POINT('Ctrl Pts',(7.09667230081556,12.2,-7.7172392419398));
#174219=CARTESIAN_POINT('Ctrl Pts',(7.09927912588989,12.2,-7.71925560495751));
#174220=CARTESIAN_POINT('Ctrl Pts',(7.10192837511943,12.2,-7.72129279365276));
#174221=CARTESIAN_POINT('Ctrl Pts',(7.10457762410833,12.2,-7.72332998216297));
#174222=CARTESIAN_POINT('Ctrl Pts',(7.10726930113565,12.2,-7.72538800047348));
#174223=CARTESIAN_POINT('Ctrl Pts',(7.11000317804864,12.2,-7.72746607899071));
#174224=CARTESIAN_POINT('Ctrl Pts',(7.11273705496165,12.2,-7.72954415750795));
#174225=CARTESIAN_POINT('Ctrl Pts',(7.11551313393964,12.2,-7.73164229980578));
#174226=CARTESIAN_POINT('Ctrl Pts',(7.11833118991771,12.2,-7.73375975631085));
#174227=CARTESIAN_POINT('Ctrl Pts',(7.12114924615177,12.2,-7.73587721300827));
#174228=CARTESIAN_POINT('Ctrl Pts',(7.12400928121682,12.2,-7.73801398467397));
#174229=CARTESIAN_POINT('Ctrl Pts',(7.12691107627235,12.2,-7.74016934248353));
#174230=CARTESIAN_POINT('Ctrl Pts',(7.1298128710643,12.2,-7.7423247000973));
#174231=CARTESIAN_POINT('Ctrl Pts',(7.13275642209165,12.2,-7.74449864123795));
#174232=CARTESIAN_POINT('Ctrl Pts',(7.13574151498319,12.2,-7.74669045474164));
#174233=CARTESIAN_POINT('Ctrl Pts',(7.13872660787473,12.2,-7.74888226824533));
#174234=CARTESIAN_POINT('Ctrl Pts',(7.14175324050544,12.2,-7.75109195327193));
#174235=CARTESIAN_POINT('Ctrl Pts',(7.14482119846152,12.2,-7.75331881030127));
#174236=CARTESIAN_POINT('Ctrl Pts',(7.14788915669627,12.2,-7.7555456675329));
#174237=CARTESIAN_POINT('Ctrl Pts',(7.15099843786044,12.2,-7.75778969883038));
#174238=CARTESIAN_POINT('Ctrl Pts',(7.15414883011829,12.2,-7.76005022170473));
#174239=CARTESIAN_POINT('Ctrl Pts',(7.15729922208998,12.2,-7.76231074437373));
#174240=CARTESIAN_POINT('Ctrl Pts',(7.16049072419569,12.2,-7.76458775550723));
#174241=CARTESIAN_POINT('Ctrl Pts',(7.16372312500968,12.2,-7.7668805912677));
#174242=CARTESIAN_POINT('Ctrl Pts',(7.16695552582367,12.2,-7.76917342702817));
#174243=CARTESIAN_POINT('Ctrl Pts',(7.17022882447495,12.2,-7.77148208502517));
#174244=CARTESIAN_POINT('Ctrl Pts',(7.17354281051944,12.2,-7.77380591110674));
#174245=CARTESIAN_POINT('Ctrl Pts',(7.17630446565685,12.2,-7.77574243291175));
#174246=CARTESIAN_POINT('Ctrl Pts',(7.17909437698944,12.2,-7.77768948970035));
#174247=CARTESIAN_POINT('Ctrl Pts',(7.18191242205741,12.2,-7.77964670963038));
#174248=CARTESIAN_POINT('Ctrl Pts',(7.18473046712538,12.2,-7.7816039295604));
#174249=CARTESIAN_POINT('Ctrl Pts',(7.18757664829088,12.2,-7.78357131208995));
#174250=CARTESIAN_POINT('Ctrl Pts',(7.19045084253998,12.2,-7.78554849376558));
#174251=CARTESIAN_POINT('Ctrl Pts',(7.19332503678907,12.2,-7.78752567544121));
#174252=CARTESIAN_POINT('Ctrl Pts',(7.19622724572209,12.2,-7.78951265435554));
#174253=CARTESIAN_POINT('Ctrl Pts',(7.1991573499582,12.2,-7.79150907504999));
#174254=CARTESIAN_POINT('Ctrl Pts',(7.20208745419431,12.2,-7.79350549574444));
#174255=CARTESIAN_POINT('Ctrl Pts',(7.20504545320452,12.2,-7.79551135381969));
#174256=CARTESIAN_POINT('Ctrl Pts',(7.20803123050984,12.2,-7.79752630146776));
#174257=CARTESIAN_POINT('Ctrl Pts',(7.21101700781514,12.2,-7.79954124911583));
#174258=CARTESIAN_POINT('Ctrl Pts',(7.21403055872526,12.2,-7.80156528312142));
#174259=CARTESIAN_POINT('Ctrl Pts',(7.21707177115726,12.2,-7.80359805985798));
#174260=CARTESIAN_POINT('Ctrl Pts',(7.22011298358926,12.2,-7.80563083659454));
#174261=CARTESIAN_POINT('Ctrl Pts',(7.22318185372333,12.2,-7.80767235337257));
#174262=CARTESIAN_POINT('Ctrl Pts',(7.22627826691921,12.2,-7.80972227115077));
#174263=CARTESIAN_POINT('Ctrl Pts',(7.22937468011509,12.2,-7.81177218892898));
#174264=CARTESIAN_POINT('Ctrl Pts',(7.232498633412,12.2,-7.81383050583054));
#174265=CARTESIAN_POINT('Ctrl Pts',(7.2356500136408,12.2,-7.8158968902399));
#174266=CARTESIAN_POINT('Ctrl Pts',(7.2388013938696,12.2,-7.81796327464925));
#174267=CARTESIAN_POINT('Ctrl Pts',(7.24198019768924,12.2,-7.82003772281617));
#174268=CARTESIAN_POINT('Ctrl Pts',(7.24518631192758,12.2,-7.82211990649735));
#174269=CARTESIAN_POINT('Ctrl Pts',(7.24839242616592,12.2,-7.82420209017854));
#174270=CARTESIAN_POINT('Ctrl Pts',(7.25162585030193,12.2,-7.8262920095904));
#174271=CARTESIAN_POINT('Ctrl Pts',(7.25488646794304,12.2,-7.82838934000766));
#174272=CARTESIAN_POINT('Ctrl Pts',(7.25814708522875,12.2,-7.83048667019634));
#174273=CARTESIAN_POINT('Ctrl Pts',(7.26143489795204,12.2,-7.83259141059899));
#174274=CARTESIAN_POINT('Ctrl Pts',(7.26474978932463,12.2,-7.83470324321544));
#174275=CARTESIAN_POINT('Ctrl Pts',(7.26806468105854,12.2,-7.83681507606209));
#174276=CARTESIAN_POINT('Ctrl Pts',(7.27140665252256,12.2,-7.83893400037807));
#174277=CARTESIAN_POINT('Ctrl Pts',(7.27477558932589,12.2,-7.84105970169696));
#174278=CARTESIAN_POINT('Ctrl Pts',(7.27881831371023,12.2,-7.84361054341865));
#174279=CARTESIAN_POINT('Ctrl Pts',(7.28289986889003,12.2,-7.84617114590798));
#174280=CARTESIAN_POINT('Ctrl Pts',(7.28702005819959,12.2,-7.84874097163176));
#174281=CARTESIAN_POINT('Ctrl Pts',(7.29045354910377,12.2,-7.85088249295154));
#174282=CARTESIAN_POINT('Ctrl Pts',(7.29391387020648,12.2,-7.85303042183648));
#174283=CARTESIAN_POINT('Ctrl Pts',(7.2974009071881,12.2,-7.85518445250007));
#174284=CARTESIAN_POINT('Ctrl Pts',(7.30088794416971,12.2,-7.85733848316366));
#174285=CARTESIAN_POINT('Ctrl Pts',(7.30440169836636,12.2,-7.85949861731061));
#174286=CARTESIAN_POINT('Ctrl Pts',(7.30794205593796,12.2,-7.8616645545333));
#174287=CARTESIAN_POINT('Ctrl Pts',(7.3107743417637,12.2,-7.86339730416981));
#174288=CARTESIAN_POINT('Ctrl Pts',(7.31362365465114,12.2,-7.86513376828637));
#174289=CARTESIAN_POINT('Ctrl Pts',(7.31648993774905,12.2,-7.86687379586612));
#174290=CARTESIAN_POINT('Ctrl Pts',(7.31935622123749,12.2,-7.86861382368294));
#174291=CARTESIAN_POINT('Ctrl Pts',(7.32223947388583,12.2,-7.87035741397629));
#174292=CARTESIAN_POINT('Ctrl Pts',(7.32513963891247,12.2,-7.87210441927019));
#174293=CARTESIAN_POINT('Ctrl Pts',(7.32803980354397,12.2,-7.87385142432605));
#174294=CARTESIAN_POINT('Ctrl Pts',(7.33095688067336,12.2,-7.87560184292247));
#174295=CARTESIAN_POINT('Ctrl Pts',(7.33389081321019,12.2,-7.87735552789));
#174296=CARTESIAN_POINT('Ctrl Pts',(7.33755822918106,12.2,-7.87954763427864));
#174297=CARTESIAN_POINT('Ctrl Pts',(7.34125198209144,12.2,-7.88174484455071));
#174298=CARTESIAN_POINT('Ctrl Pts',(7.34497196125675,12.2,-7.88394687510602));
#174299=CARTESIAN_POINT('Ctrl Pts',(7.34794794475119,12.2,-7.88570849964627));
#174300=CARTESIAN_POINT('Ctrl Pts',(7.35094071298473,12.2,-7.88747320897994));
#174301=CARTESIAN_POINT('Ctrl Pts',(7.35395020891167,12.2,-7.88924085899819));
#174302=CARTESIAN_POINT('Ctrl Pts',(7.35695970442857,12.2,-7.89100850877559));
#174303=CARTESIAN_POINT('Ctrl Pts',(7.35998592972057,12.2,-7.8927790992141));
#174304=CARTESIAN_POINT('Ctrl Pts',(7.36302882619295,12.2,-7.89455248834672));
#174305=CARTESIAN_POINT('Ctrl Pts',(7.36607172307993,12.2,-7.89632587772097));
#174306=CARTESIAN_POINT('Ctrl Pts',(7.36913129149947,12.2,-7.89810206652612));
#174307=CARTESIAN_POINT('Ctrl Pts',(7.37220747700153,12.2,-7.89988091384546));
#174308=CARTESIAN_POINT('Ctrl Pts',(7.37528366208447,12.2,-7.90165976092243));
#174309=CARTESIAN_POINT('Ctrl Pts',(7.37837646182128,12.2,-7.90344126715918));
#174310=CARTESIAN_POINT('Ctrl Pts',(7.38148582249879,12.2,-7.90522529299115));
#174311=CARTESIAN_POINT('Ctrl Pts',(7.38459518359994,12.2,-7.90700931906619));
#174312=CARTESIAN_POINT('Ctrl Pts',(7.38772110534015,12.2,-7.90879586437362));
#174313=CARTESIAN_POINT('Ctrl Pts',(7.39086353029026,12.2,-7.91058479363794));
#174314=CARTESIAN_POINT('Ctrl Pts',(7.39400595481222,12.2,-7.91237372265852));
#174315=CARTESIAN_POINT('Ctrl Pts',(7.39716488463087,12.2,-7.91416503415361));
#174316=CARTESIAN_POINT('Ctrl Pts',(7.40034026248071,12.2,-7.91595859200676));
#174317=CARTESIAN_POINT('Ctrl Pts',(7.40351564076321,12.2,-7.91775215010429));
#174318=CARTESIAN_POINT('Ctrl Pts',(7.40670746712928,12.2,-7.91954795595341));
#174319=CARTESIAN_POINT('Ctrl Pts',(7.4099156879854,12.2,-7.92134587522623));
#174320=CARTESIAN_POINT('Ctrl Pts',(7.4131239084044,12.2,-7.92314379425408));
#174321=CARTESIAN_POINT('Ctrl Pts',(7.41634852180882,12.2,-7.92494382498344));
#174322=CARTESIAN_POINT('Ctrl Pts',(7.41958947298666,12.2,-7.92674583744705));
#174323=CARTESIAN_POINT('Ctrl Pts',(7.42283042460608,12.2,-7.92854785015617));
#174324=CARTESIAN_POINT('Ctrl Pts',(7.4260877143798,12.2,-7.93035184282937));
#174325=CARTESIAN_POINT('Ctrl Pts',(7.42936128672487,12.2,-7.93215768548334));
#174326=CARTESIAN_POINT('Ctrl Pts',(7.43263485906994,12.2,-7.93396352813731));
#174327=CARTESIAN_POINT('Ctrl Pts',(7.4359247148947,12.2,-7.93577121949983));
#174328=CARTESIAN_POINT('Ctrl Pts',(7.43923079846543,12.2,-7.93758063032085));
#174329=CARTESIAN_POINT('Ctrl Pts',(7.44253688158571,12.2,-7.93939004089532));
#174330=CARTESIAN_POINT('Ctrl Pts',(7.4458591925582,12.2,-7.94120117193874));
#174331=CARTESIAN_POINT('Ctrl Pts',(7.44919767702261,12.2,-7.94301389379877));
#174332=CARTESIAN_POINT('Ctrl Pts',(7.45253616194188,12.2,-7.94482661590579));
#174333=CARTESIAN_POINT('Ctrl Pts',(7.45589081965178,12.2,-7.94664092944779));
#174334=CARTESIAN_POINT('Ctrl Pts',(7.45926159655934,12.2,-7.94845670754689));
#174335=CARTESIAN_POINT('Ctrl Pts',(7.46263237300765,12.2,-7.95027248539859));
#174336=CARTESIAN_POINT('Ctrl Pts',(7.46601926710107,12.2,-7.95208972755287));
#174337=CARTESIAN_POINT('Ctrl Pts',(7.46942222548851,12.2,-7.95390830879302));
#174338=CARTESIAN_POINT('Ctrl Pts',(7.47282518433961,12.2,-7.95572689028095));
#174339=CARTESIAN_POINT('Ctrl Pts',(7.47624420656598,12.2,-7.95754681084617));
#174340=CARTESIAN_POINT('Ctrl Pts',(7.47967923848175,12.2,-7.95936794581428));
#174341=CARTESIAN_POINT('Ctrl Pts',(7.48311426992949,12.2,-7.96118908053426));
#174342=CARTESIAN_POINT('Ctrl Pts',(7.48656531214274,12.2,-7.96301143010287));
#174343=CARTESIAN_POINT('Ctrl Pts',(7.49003230869161,12.2,-7.96483487134262));
#174344=CARTESIAN_POINT('Ctrl Pts',(7.49349930571284,12.2,-7.96665831283081));
#174345=CARTESIAN_POINT('Ctrl Pts',(7.49698225712489,12.2,-7.96848284732471));
#174346=CARTESIAN_POINT('Ctrl Pts',(7.50048111126106,12.2,-7.97030835092426));
#174347=CARTESIAN_POINT('Ctrl Pts',(7.50397996492053,12.2,-7.97213385427508));
#174348=CARTESIAN_POINT('Ctrl Pts',(7.50749471944015,12.2,-7.97396032869579));
#174349=CARTESIAN_POINT('Ctrl Pts',(7.51102532077099,12.2,-7.9757876526932));
#174350=CARTESIAN_POINT('Ctrl Pts',(7.51455592258288,12.2,-7.97761497693956));
#174351=CARTESIAN_POINT('Ctrl Pts',(7.51810237148497,12.2,-7.97944315110537));
#174352=CARTESIAN_POINT('Ctrl Pts',(7.52166461379125,12.2,-7.98127205664953));
#174353=CARTESIAN_POINT('Ctrl Pts',(7.52522685561217,12.2,-7.98310096194451));
#174354=CARTESIAN_POINT('Ctrl Pts',(7.52880489064658,12.2,-7.98493059795321));
#174355=CARTESIAN_POINT('Ctrl Pts',(7.53239866512897,12.2,-7.98676084719243));
#174356=CARTESIAN_POINT('Ctrl Pts',(7.535992440101,12.2,-7.98859109668101));
#174357=CARTESIAN_POINT('Ctrl Pts',(7.53960195397454,12.2,-7.99042195955855));
#174358=CARTESIAN_POINT('Ctrl Pts',(7.54322715494989,12.2,-7.99225331849168));
#174359=CARTESIAN_POINT('Ctrl Pts',(7.54685235592523,12.2,-7.99408467742483));
#174360=CARTESIAN_POINT('Ctrl Pts',(7.55049324196629,12.2,-7.99591653310802));
#174361=CARTESIAN_POINT('Ctrl Pts',(7.55414976088939,12.2,-7.99774877004125));
#174362=CARTESIAN_POINT('Ctrl Pts',(7.55780627931429,12.2,-7.99958100672483));
#174363=CARTESIAN_POINT('Ctrl Pts',(7.56147842973493,12.2,-8.00141362508195));
#174364=CARTESIAN_POINT('Ctrl Pts',(7.56516615950571,12.2,-8.00324650977377));
#174365=CARTESIAN_POINT('Ctrl Pts',(7.56885388977894,12.2,-8.00507939471531));
#174366=CARTESIAN_POINT('Ctrl Pts',(7.57255719835921,12.2,-8.00691254635538));
#174367=CARTESIAN_POINT('Ctrl Pts',(7.57627603334126,12.2,-8.00874585256643));
#174368=CARTESIAN_POINT('Ctrl Pts',(7.5799948678166,12.2,-8.01057915852768));
#174369=CARTESIAN_POINT('Ctrl Pts',(7.58372922740104,12.2,-8.01241261765558));
#174370=CARTESIAN_POINT('Ctrl Pts',(7.58747906042681,12.2,-8.01424611961679));
#174371=CARTESIAN_POINT('Ctrl Pts',(7.59216635209222,12.2,-8.01653799725567));
#174372=CARTESIAN_POINT('Ctrl Pts',(7.59687781814253,12.2,-8.01882993989391));
#174373=CARTESIAN_POINT('Ctrl Pts',(7.60161335670564,12.2,-8.02112173122377));
#174374=CARTESIAN_POINT('Ctrl Pts',(7.6054017877626,12.2,-8.02295516438757));
#174375=CARTESIAN_POINT('Ctrl Pts',(7.60920562595072,12.2,-8.0247885025054));
#174376=CARTESIAN_POINT('Ctrl Pts',(7.61302481688267,12.2,-8.02662163404973));
#174377=CARTESIAN_POINT('Ctrl Pts',(7.61684400729424,12.2,-8.0284547653443));
#174378=CARTESIAN_POINT('Ctrl Pts',(7.62067855032046,12.2,-8.03028769017776));
#174379=CARTESIAN_POINT('Ctrl Pts',(7.62452839472697,12.2,-8.03212030158353));
#174380=CARTESIAN_POINT('Ctrl Pts',(7.62837823965803,12.2,-8.033952913239));
#174381=CARTESIAN_POINT('Ctrl Pts',(7.63224338392581,12.2,-8.0357852113995));
#174382=CARTESIAN_POINT('Ctrl Pts',(7.63612377705471,12.2,-8.0376170877575));
#174383=CARTESIAN_POINT('Ctrl Pts',(7.64000416965489,12.2,-8.03944896386589));
#174384=CARTESIAN_POINT('Ctrl Pts',(7.64389980889268,12.2,-8.04128041761109));
#174385=CARTESIAN_POINT('Ctrl Pts',(7.64781064340532,12.2,-8.04311134435034));
#174386=CARTESIAN_POINT('Ctrl Pts',(7.65172147845082,12.2,-8.04494227133905));
#174387=CARTESIAN_POINT('Ctrl Pts',(7.65564750900921,12.2,-8.04677267072491));
#174388=CARTESIAN_POINT('Ctrl Pts',(7.65958868261389,12.2,-8.04860243765793));
#174389=CARTESIAN_POINT('Ctrl Pts',(7.66352985568157,12.2,-8.05043220434163));
#174390=CARTESIAN_POINT('Ctrl Pts',(7.66748616990403,12.2,-8.05226133700944));
#174391=CARTESIAN_POINT('Ctrl Pts',(7.67145757516536,12.2,-8.0540897332847));
#174392=CARTESIAN_POINT('Ctrl Pts',(7.67542898096779,12.2,-8.05591812980909));
#174393=CARTESIAN_POINT('Ctrl Pts',(7.67941547718586,12.2,-8.05774578974429));
#174394=CARTESIAN_POINT('Ctrl Pts',(7.68341701029382,12.2,-8.05957260939935));
#174395=CARTESIAN_POINT('Ctrl Pts',(7.68741854285656,12.2,-8.06139942880551));
#174396=CARTESIAN_POINT('Ctrl Pts',(7.6914351138774,12.2,-8.06322540671183));
#174397=CARTESIAN_POINT('Ctrl Pts',(7.69546667032408,12.2,-8.06505044345163));
#174398=CARTESIAN_POINT('Ctrl Pts',(7.69949822732005,12.2,-8.06687548044008));
#174399=CARTESIAN_POINT('Ctrl Pts',(7.70354477009057,12.2,-8.06869957497417));
#174400=CARTESIAN_POINT('Ctrl Pts',(7.70760624521931,12.2,-8.07052262602626));
#174401=CARTESIAN_POINT('Ctrl Pts',(7.71065235128918,12.2,-8.07188991419113));
#174402=CARTESIAN_POINT('Ctrl Pts',(7.71370685831119,12.2,-8.07325661520887));
#174403=CARTESIAN_POINT('Ctrl Pts',(7.71676974325544,12.2,-8.07462268645711));
#174404=CARTESIAN_POINT('Ctrl Pts',(7.71983262819969,12.2,-8.07598875770535));
#174405=CARTESIAN_POINT('Ctrl Pts',(7.72290389047696,12.2,-8.07735420070077));
#174406=CARTESIAN_POINT('Ctrl Pts',(7.72598350940601,12.2,-8.07871897185958));
#174407=CARTESIAN_POINT('Ctrl Pts',(7.72906312833507,12.2,-8.08008374301838));
#174408=CARTESIAN_POINT('Ctrl Pts',(7.7321511031052,12.2,-8.08144784196891));
#174409=CARTESIAN_POINT('Ctrl Pts',(7.73524741211657,12.2,-8.08281122816947));
#174410=CARTESIAN_POINT('Ctrl Pts',(7.73834372169042,12.2,-8.08417461461772));
#174411=CARTESIAN_POINT('Ctrl Pts',(7.74144836607497,12.2,-8.08553728883243));
#174412=CARTESIAN_POINT('Ctrl Pts',(7.74456132215352,12.2,-8.08689920732192));
#174413=CARTESIAN_POINT('Ctrl Pts',(7.74871192931572,12.2,-8.08871509822889));
#174414=CARTESIAN_POINT('Ctrl Pts',(7.7528773134865,12.2,-8.09052964854155));
#174415=CARTESIAN_POINT('Ctrl Pts',(7.75705742449704,12.2,-8.09234275945712));
#174416=CARTESIAN_POINT('Ctrl Pts',(7.76019250789733,12.2,-8.09370259270556));
#174417=CARTESIAN_POINT('Ctrl Pts',(7.76333587322172,12.2,-8.09506161708457));
#174418=CARTESIAN_POINT('Ctrl Pts',(7.76648750064817,12.2,-8.09641979032697));
#174419=CARTESIAN_POINT('Ctrl Pts',(7.76963912807461,12.2,-8.09777796356937));
#174420=CARTESIAN_POINT('Ctrl Pts',(7.77279901690881,12.2,-8.09913528725348));
#174421=CARTESIAN_POINT('Ctrl Pts',(7.77596714533424,12.2,-8.10049171999599));
#174422=CARTESIAN_POINT('Ctrl Pts',(7.77913527433522,12.2,-8.1018481529849));
#174423=CARTESIAN_POINT('Ctrl Pts',(7.7823116421302,12.2,-8.10320369578193));
#174424=CARTESIAN_POINT('Ctrl Pts',(7.78549622821913,12.2,-8.10455830727033));
#174425=CARTESIAN_POINT('Ctrl Pts',(7.78868081372953,12.2,-8.10591291851264));
#174426=CARTESIAN_POINT('Ctrl Pts',(7.79187361794138,12.2,-8.10726659894341));
#174427=CARTESIAN_POINT('Ctrl Pts',(7.79507461761095,12.2,-8.10861930829506));
#174428=CARTESIAN_POINT('Ctrl Pts',(7.79934261697653,12.2,-8.11042292068202));
#174429=CARTESIAN_POINT('Ctrl Pts',(7.80362518662598,12.2,-8.11222480775822));
#174430=CARTESIAN_POINT('Ctrl Pts',(7.80792227510707,12.2,-8.11402487511118));
#174431=CARTESIAN_POINT('Ctrl Pts',(7.81114509161427,12.2,-8.11537492568722));
#174432=CARTESIAN_POINT('Ctrl Pts',(7.8143760758959,12.2,-8.11672395137166));
#174433=CARTESIAN_POINT('Ctrl Pts',(7.81761520536043,12.2,-8.11807191503117));
#174434=CARTESIAN_POINT('Ctrl Pts',(7.82085433541341,12.2,-8.11941987893555));
#174435=CARTESIAN_POINT('Ctrl Pts',(7.82410161060201,12.2,-8.12076677956464));
#174436=CARTESIAN_POINT('Ctrl Pts',(7.82735700970124,12.2,-8.12211257855174));
#174437=CARTESIAN_POINT('Ctrl Pts',(7.83061240820906,12.2,-8.12345837729435));
#174438=CARTESIAN_POINT('Ctrl Pts',(7.83387593048743,12.2,-8.12480307394178));
#174439=CARTESIAN_POINT('Ctrl Pts',(7.83714755511628,12.2,-8.12614663025162));
#174440=CARTESIAN_POINT('Ctrl Pts',(7.84041917974513,12.2,-8.12749018656146));
#174441=CARTESIAN_POINT('Ctrl Pts',(7.84369890559382,12.2,-8.12883260207837));
#174442=CARTESIAN_POINT('Ctrl Pts',(7.84698671255839,12.2,-8.13017383786286));
#174443=CARTESIAN_POINT('Ctrl Pts',(7.85027451952297,12.2,-8.13151507364736));
#174444=CARTESIAN_POINT('Ctrl Pts',(7.8535704072366,12.2,-8.132855130532));
#174445=CARTESIAN_POINT('Ctrl Pts',(7.85687435324155,12.2,-8.13419397023335));
#174446=CARTESIAN_POINT('Ctrl Pts',(7.8601782992465,12.2,-8.13553280993471));
#174447=CARTESIAN_POINT('Ctrl Pts',(7.86349030432613,12.2,-8.13687043210278));
#174448=CARTESIAN_POINT('Ctrl Pts',(7.86681034637147,12.2,-8.13820679838767));
#174449=CARTESIAN_POINT('Ctrl Pts',(7.87013038841681,12.2,-8.13954316467256));
#174450=CARTESIAN_POINT('Ctrl Pts',(7.8734584687616,12.2,-8.14087827564088));
#174451=CARTESIAN_POINT('Ctrl Pts',(7.8767945642643,12.2,-8.14221209342592));
#174452=CARTESIAN_POINT('Ctrl Pts',(7.88013066037304,12.2,-8.14354591145326));
#174453=CARTESIAN_POINT('Ctrl Pts',(7.88347477237572,12.2,-8.14487843628027));
#174454=CARTESIAN_POINT('Ctrl Pts',(7.88682687798899,12.2,-8.14620963076522));
#174455=CARTESIAN_POINT('Ctrl Pts',(7.89017898299329,12.2,-8.14754082500835));
#174456=CARTESIAN_POINT('Ctrl Pts',(7.89353908232146,12.2,-8.14887068922244));
#174457=CARTESIAN_POINT('Ctrl Pts',(7.89690715540994,12.2,-8.15019918503204));
#174458=CARTESIAN_POINT('Ctrl Pts',(7.90027522849842,12.2,-8.15152768084165));
#174459=CARTESIAN_POINT('Ctrl Pts',(7.90365127357448,12.2,-8.15285480812613));
#174460=CARTESIAN_POINT('Ctrl Pts',(7.90703526961888,12.2,-8.15418053091117));
#174461=CARTESIAN_POINT('Ctrl Pts',(7.91154726413984,12.2,-8.15594816121095));
#174462=CARTESIAN_POINT('Ctrl Pts',(7.91607339557461,12.2,-8.15771329454178));
#174463=CARTESIAN_POINT('Ctrl Pts',(7.92061361075757,12.2,-8.15947584345351));
#174464=CARTESIAN_POINT('Ctrl Pts',(7.92515382655913,12.2,-8.16123839260539));
#174465=CARTESIAN_POINT('Ctrl Pts',(7.92970812676935,12.2,-8.16299835740859));
#174466=CARTESIAN_POINT('Ctrl Pts',(7.93427646176133,12.2,-8.16475565073456));
#174467=CARTESIAN_POINT('Ctrl Pts',(7.9377027126941,12.2,-8.16607362060932));
#174468=CARTESIAN_POINT('Ctrl Pts',(7.94113685797289,12.2,-8.16739008949063));
#174469=CARTESIAN_POINT('Ctrl Pts',(7.94457887544676,12.2,-8.16870501928216));
#174470=CARTESIAN_POINT('Ctrl Pts',(7.94802089292064,12.2,-8.1700199490737));
#174471=CARTESIAN_POINT('Ctrl Pts',(7.95147078271611,12.2,-8.17133334008787));
#174472=CARTESIAN_POINT('Ctrl Pts',(7.95492852413146,12.2,-8.17264515737368));
#174473=CARTESIAN_POINT('Ctrl Pts',(7.95838626554681,12.2,-8.17395697465949));
#174474=CARTESIAN_POINT('Ctrl Pts',(7.96185185806996,12.2,-8.17526721716206));
#174475=CARTESIAN_POINT('Ctrl Pts',(7.96532528102603,12.2,-8.17657585090641));
#174476=CARTESIAN_POINT('Ctrl Pts',(7.96995651205477,12.2,-8.17832069605736));
#174477=CARTESIAN_POINT('Ctrl Pts',(7.97460166248075,12.2,-8.18006268020411));
#174478=CARTESIAN_POINT('Ctrl Pts',(7.97926068347808,12.2,-8.18180171875121));
#174479=CARTESIAN_POINT('Ctrl Pts',(7.98275494890868,12.2,-8.18310599754308));
#174480=CARTESIAN_POINT('Ctrl Pts',(7.98625701599166,12.2,-8.18440861915686));
#174481=CARTESIAN_POINT('Ctrl Pts',(7.98976686150504,12.2,-8.18570954653218));
#174482=CARTESIAN_POINT('Ctrl Pts',(7.99444665594795,12.2,-8.18744411652349));
#174483=CARTESIAN_POINT('Ctrl Pts',(7.99914028058659,12.2,-8.18917567643041));
#174484=CARTESIAN_POINT('Ctrl Pts',(8.00384768901123,12.2,-8.1909041510243));
#174485=CARTESIAN_POINT('Ctrl Pts',(8.007378245009,12.2,-8.19220050685196));
#174486=CARTESIAN_POINT('Ctrl Pts',(8.01091655503138,12.2,-8.19349512722138));
#174487=CARTESIAN_POINT('Ctrl Pts',(8.01446259644487,12.2,-8.19478797688259));
#174488=CARTESIAN_POINT('Ctrl Pts',(8.01800863785837,12.2,-8.19608082654379));
#174489=CARTESIAN_POINT('Ctrl Pts',(8.02156241031632,12.2,-8.19737190427552));
#174490=CARTESIAN_POINT('Ctrl Pts',(8.0251238882448,12.2,-8.1986611675262));
#174491=CARTESIAN_POINT('Ctrl Pts',(8.03105968500793,12.2,-8.20080993968872));
#174492=CARTESIAN_POINT('Ctrl Pts',(8.03701687660465,12.2,-8.20295365973189));
#174493=CARTESIAN_POINT('Ctrl Pts',(8.04299539641855,12.2,-8.20509222040386));
#174494=CARTESIAN_POINT('Ctrl Pts',(8.04658250817656,12.2,-8.20637535676042));
#174495=CARTESIAN_POINT('Ctrl Pts',(8.05017730034549,12.2,-8.20765663976758));
#174496=CARTESIAN_POINT('Ctrl Pts',(8.05377977099995,12.2,-8.20893607000002));
#174497=CARTESIAN_POINT('Origin',(-5.66257110645729E-14,15.2,-1.77635683940025E-14));
#174498=CARTESIAN_POINT('',(8.02901631833639,15.2,-6.57080831866923));
#174499=CARTESIAN_POINT('',(8.02901631833639,12.2,-6.57080831866923));
#174500=CARTESIAN_POINT('',(8.02901631799994,15.2,-6.57080831900001));
#174501=CARTESIAN_POINT('Origin',(-5.66257110645729E-14,12.2,-1.77635683940025E-14));
#174502=CARTESIAN_POINT('Origin',(-5.66257110645729E-14,15.2,-1.77635683940025E-14));
#174503=CARTESIAN_POINT('Origin',(-5.66257110645729E-14,15.2,-1.77635683940025E-14));
#174504=CARTESIAN_POINT('',(9.14005731399994,15.2,-6.97920857100002));
#174505=CARTESIAN_POINT('',(9.36775917399994,15.2,-6.67046385500001));
#174506=CARTESIAN_POINT('Origin',(-5.66257110645729E-14,15.2,-1.77635683940025E-14));
#174507=CARTESIAN_POINT('',(9.36775917399994,12.2,-6.67046385500001));
#174508=CARTESIAN_POINT('',(9.36775917399994,15.2,-6.67046385500001));
#174509=CARTESIAN_POINT('',(9.14005731399994,12.2,-6.97920857100002));
#174510=CARTESIAN_POINT('Origin',(-5.66257110645729E-14,12.2,-1.77635683940025E-14));
#174511=CARTESIAN_POINT('',(9.14005731399994,15.2,-6.97920857100002));
#174512=CARTESIAN_POINT('Ctrl Pts',(8.02901631899994,15.2,-6.57080831800001));
#174513=CARTESIAN_POINT('Ctrl Pts',(8.02901631899994,11.6,-6.57080831800001));
#174514=CARTESIAN_POINT('Ctrl Pts',(8.02916024099994,15.2,-6.57090674100001));
#174515=CARTESIAN_POINT('Ctrl Pts',(8.02916024099994,11.6,-6.57090674100001));
#174516=CARTESIAN_POINT('Ctrl Pts',(8.02945316199994,15.2,-6.57110695200001));
#174517=CARTESIAN_POINT('Ctrl Pts',(8.02945316199994,11.6,-6.57110695200001));
#174518=CARTESIAN_POINT('Ctrl Pts',(8.02989715799994,15.2,-6.57141009900001));
#174519=CARTESIAN_POINT('Ctrl Pts',(8.02989715799994,11.6,-6.57141009900001));
#174520=CARTESIAN_POINT('Ctrl Pts',(8.03049556399994,15.2,-6.57181801900002));
#174521=CARTESIAN_POINT('Ctrl Pts',(8.03049556399994,11.6,-6.57181801900002));
#174522=CARTESIAN_POINT('Ctrl Pts',(8.03125297399994,15.2,-6.57233322300002));
#174523=CARTESIAN_POINT('Ctrl Pts',(8.03125297399994,11.6,-6.57233322300002));
#174524=CARTESIAN_POINT('Ctrl Pts',(8.03202318499994,15.2,-6.57285600500002));
#174525=CARTESIAN_POINT('Ctrl Pts',(8.03202318499994,11.6,-6.57285600500002));
#174526=CARTESIAN_POINT('Ctrl Pts',(8.03280179799994,15.2,-6.57338335000002));
#174527=CARTESIAN_POINT('Ctrl Pts',(8.03280179799994,11.6,-6.57338335000002));
#174528=CARTESIAN_POINT('Ctrl Pts',(8.03358879899994,15.2,-6.57391522700002));
#174529=CARTESIAN_POINT('Ctrl Pts',(8.03358879899994,11.6,-6.57391522700002));
#174530=CARTESIAN_POINT('Ctrl Pts',(8.03438417899994,15.2,-6.57445160500002));
#174531=CARTESIAN_POINT('Ctrl Pts',(8.03438417899994,11.6,-6.57445160500002));
#174532=CARTESIAN_POINT('Ctrl Pts',(8.03518792399995,15.2,-6.57499245800001));
#174533=CARTESIAN_POINT('Ctrl Pts',(8.03518792399995,11.6,-6.57499245800001));
#174534=CARTESIAN_POINT('Ctrl Pts',(8.03600002099994,15.2,-6.57553775100002));
#174535=CARTESIAN_POINT('Ctrl Pts',(8.03600002099994,11.6,-6.57553775100002));
#174536=CARTESIAN_POINT('Ctrl Pts',(8.03682045999994,15.2,-6.57608745900002));
#174537=CARTESIAN_POINT('Ctrl Pts',(8.03682045999994,11.6,-6.57608745900002));
#174538=CARTESIAN_POINT('Ctrl Pts',(8.03764922899994,15.2,-6.57664155100001));
#174539=CARTESIAN_POINT('Ctrl Pts',(8.03764922899994,11.6,-6.57664155100001));
#174540=CARTESIAN_POINT('Ctrl Pts',(8.03848631399994,15.2,-6.57719999700002));
#174541=CARTESIAN_POINT('Ctrl Pts',(8.03848631399994,11.6,-6.57719999700002));
#174542=CARTESIAN_POINT('Ctrl Pts',(8.03933170499995,15.2,-6.57776276800002));
#174543=CARTESIAN_POINT('Ctrl Pts',(8.03933170499995,11.6,-6.57776276800002));
#174544=CARTESIAN_POINT('Ctrl Pts',(8.04018539099994,15.2,-6.57832983600001));
#174545=CARTESIAN_POINT('Ctrl Pts',(8.04018539099994,11.6,-6.57832983600001));
#174546=CARTESIAN_POINT('Ctrl Pts',(8.04104735699994,15.2,-6.57890117200001));
#174547=CARTESIAN_POINT('Ctrl Pts',(8.04104735699994,11.6,-6.57890117200001));
#174548=CARTESIAN_POINT('Ctrl Pts',(8.04191759399994,15.2,-6.57947674700001));
#174549=CARTESIAN_POINT('Ctrl Pts',(8.04191759399994,11.6,-6.57947674700001));
#174550=CARTESIAN_POINT('Ctrl Pts',(8.04279608999994,15.2,-6.58005653200001));
#174551=CARTESIAN_POINT('Ctrl Pts',(8.04279608999994,11.6,-6.58005653200001));
#174552=CARTESIAN_POINT('Ctrl Pts',(8.04368283299995,15.2,-6.58064049900001));
#174553=CARTESIAN_POINT('Ctrl Pts',(8.04368283299995,11.6,-6.58064049900001));
#174554=CARTESIAN_POINT('Ctrl Pts',(8.04457780999994,15.2,-6.58122862000001));
#174555=CARTESIAN_POINT('Ctrl Pts',(8.04457780999994,11.6,-6.58122862000001));
#174556=CARTESIAN_POINT('Ctrl Pts',(8.04548101299994,15.2,-6.58182086700001));
#174557=CARTESIAN_POINT('Ctrl Pts',(8.04548101299994,11.6,-6.58182086700001));
#174558=CARTESIAN_POINT('Ctrl Pts',(8.04639242599994,15.2,-6.58241721200002));
#174559=CARTESIAN_POINT('Ctrl Pts',(8.04639242599994,11.6,-6.58241721200002));
#174560=CARTESIAN_POINT('Ctrl Pts',(8.04731204199994,15.2,-6.58301762600002));
#174561=CARTESIAN_POINT('Ctrl Pts',(8.04731204199994,11.6,-6.58301762600002));
#174562=CARTESIAN_POINT('Ctrl Pts',(8.04823984699994,15.2,-6.58362208200002));
#174563=CARTESIAN_POINT('Ctrl Pts',(8.04823984699994,11.6,-6.58362208200002));
#174564=CARTESIAN_POINT('Ctrl Pts',(8.04917582899994,15.2,-6.58423055400001));
#174565=CARTESIAN_POINT('Ctrl Pts',(8.04917582899994,11.6,-6.58423055400001));
#174566=CARTESIAN_POINT('Ctrl Pts',(8.05011997799994,15.2,-6.58484301200001));
#174567=CARTESIAN_POINT('Ctrl Pts',(8.05011997799994,11.6,-6.58484301200001));
#174568=CARTESIAN_POINT('Ctrl Pts',(8.05107228299994,15.2,-6.58545943100001));
#174569=CARTESIAN_POINT('Ctrl Pts',(8.05107228299994,11.6,-6.58545943100001));
#174570=CARTESIAN_POINT('Ctrl Pts',(8.05203273199995,15.2,-6.58607978300001));
#174571=CARTESIAN_POINT('Ctrl Pts',(8.05203273199995,11.6,-6.58607978300001));
#174572=CARTESIAN_POINT('Ctrl Pts',(8.05300131399994,15.2,-6.58670403900001));
#174573=CARTESIAN_POINT('Ctrl Pts',(8.05300131399994,11.6,-6.58670403900001));
#174574=CARTESIAN_POINT('Ctrl Pts',(8.05397801699994,15.2,-6.58733217500002));
#174575=CARTESIAN_POINT('Ctrl Pts',(8.05397801699994,11.6,-6.58733217500002));
#174576=CARTESIAN_POINT('Ctrl Pts',(8.05496283099994,15.2,-6.58796416400002));
#174577=CARTESIAN_POINT('Ctrl Pts',(8.05496283099994,11.6,-6.58796416400002));
#174578=CARTESIAN_POINT('Ctrl Pts',(8.05595574499994,15.2,-6.58859997700001));
#174579=CARTESIAN_POINT('Ctrl Pts',(8.05595574499994,11.6,-6.58859997700001));
#174580=CARTESIAN_POINT('Ctrl Pts',(8.05695674699994,15.2,-6.58923959000001));
#174581=CARTESIAN_POINT('Ctrl Pts',(8.05695674699994,11.6,-6.58923959000001));
#174582=CARTESIAN_POINT('Ctrl Pts',(8.05796582599994,15.2,-6.58988297500001));
#174583=CARTESIAN_POINT('Ctrl Pts',(8.05796582599994,11.6,-6.58988297500001));
#174584=CARTESIAN_POINT('Ctrl Pts',(8.05898297299994,15.2,-6.59053010600001));
#174585=CARTESIAN_POINT('Ctrl Pts',(8.05898297299994,11.6,-6.59053010600001));
#174586=CARTESIAN_POINT('Ctrl Pts',(8.06000817399994,15.2,-6.59118095800002));
#174587=CARTESIAN_POINT('Ctrl Pts',(8.06000817399994,11.6,-6.59118095800002));
#174588=CARTESIAN_POINT('Ctrl Pts',(8.06104142099995,15.2,-6.59183550400002));
#174589=CARTESIAN_POINT('Ctrl Pts',(8.06104142099995,11.6,-6.59183550400002));
#174590=CARTESIAN_POINT('Ctrl Pts',(8.06208269999994,15.2,-6.59249371900002));
#174591=CARTESIAN_POINT('Ctrl Pts',(8.06208269999994,11.6,-6.59249371900002));
#174592=CARTESIAN_POINT('Ctrl Pts',(8.06313200299994,15.2,-6.59315557600002));
#174593=CARTESIAN_POINT('Ctrl Pts',(8.06313200299994,11.6,-6.59315557600002));
#174594=CARTESIAN_POINT('Ctrl Pts',(8.06418931899995,15.2,-6.59382104900001));
#174595=CARTESIAN_POINT('Ctrl Pts',(8.06418931899995,11.6,-6.59382104900001));
#174596=CARTESIAN_POINT('Ctrl Pts',(8.06525463399994,15.2,-6.59449011500002));
#174597=CARTESIAN_POINT('Ctrl Pts',(8.06525463399994,11.6,-6.59449011500002));
#174598=CARTESIAN_POINT('Ctrl Pts',(8.06632794099994,15.2,-6.59516274600002));
#174599=CARTESIAN_POINT('Ctrl Pts',(8.06632794099994,11.6,-6.59516274600002));
#174600=CARTESIAN_POINT('Ctrl Pts',(8.06740922699994,15.2,-6.59583891700001));
#174601=CARTESIAN_POINT('Ctrl Pts',(8.06740922699994,11.6,-6.59583891700001));
#174602=CARTESIAN_POINT('Ctrl Pts',(8.06849848299994,15.2,-6.59651860500002));
#174603=CARTESIAN_POINT('Ctrl Pts',(8.06849848299994,11.6,-6.59651860500002));
#174604=CARTESIAN_POINT('Ctrl Pts',(8.06959569799995,15.2,-6.59720178200002));
#174605=CARTESIAN_POINT('Ctrl Pts',(8.06959569799995,11.6,-6.59720178200002));
#174606=CARTESIAN_POINT('Ctrl Pts',(8.07070085999994,15.2,-6.59788842600002));
#174607=CARTESIAN_POINT('Ctrl Pts',(8.07070085999994,11.6,-6.59788842600002));
#174608=CARTESIAN_POINT('Ctrl Pts',(8.07181395999994,15.2,-6.59857851000002));
#174609=CARTESIAN_POINT('Ctrl Pts',(8.07181395999994,11.6,-6.59857851000002));
#174610=CARTESIAN_POINT('Ctrl Pts',(8.07293498599994,15.2,-6.59927200900002));
#174611=CARTESIAN_POINT('Ctrl Pts',(8.07293498599994,11.6,-6.59927200900002));
#174612=CARTESIAN_POINT('Ctrl Pts',(8.07406392899994,15.2,-6.59996890000001));
#174613=CARTESIAN_POINT('Ctrl Pts',(8.07406392899994,11.6,-6.59996890000001));
#174614=CARTESIAN_POINT('Ctrl Pts',(8.07520077799994,15.2,-6.60066915900002));
#174615=CARTESIAN_POINT('Ctrl Pts',(8.07520077799994,11.6,-6.60066915900002));
#174616=CARTESIAN_POINT('Ctrl Pts',(8.07634552199995,15.2,-6.60137276000002));
#174617=CARTESIAN_POINT('Ctrl Pts',(8.07634552199995,11.6,-6.60137276000002));
#174618=CARTESIAN_POINT('Ctrl Pts',(8.07749815199994,15.2,-6.60207968000002));
#174619=CARTESIAN_POINT('Ctrl Pts',(8.07749815199994,11.6,-6.60207968000002));
#174620=CARTESIAN_POINT('Ctrl Pts',(8.07865865699995,15.2,-6.60278989300001));
#174621=CARTESIAN_POINT('Ctrl Pts',(8.07865865699995,11.6,-6.60278989300001));
#174622=CARTESIAN_POINT('Ctrl Pts',(8.07982702499995,15.2,-6.60350337600002));
#174623=CARTESIAN_POINT('Ctrl Pts',(8.07982702499995,11.6,-6.60350337600002));
#174624=CARTESIAN_POINT('Ctrl Pts',(8.08100324799994,15.2,-6.60422010600002));
#174625=CARTESIAN_POINT('Ctrl Pts',(8.08100324799994,11.6,-6.60422010600002));
#174626=CARTESIAN_POINT('Ctrl Pts',(8.08218731399995,15.2,-6.60494005800001));
#174627=CARTESIAN_POINT('Ctrl Pts',(8.08218731399995,11.6,-6.60494005800001));
#174628=CARTESIAN_POINT('Ctrl Pts',(8.08337921499995,15.2,-6.60566320800001));
#174629=CARTESIAN_POINT('Ctrl Pts',(8.08337921499995,11.6,-6.60566320800001));
#174630=CARTESIAN_POINT('Ctrl Pts',(8.08457893799994,15.2,-6.60638953300002));
#174631=CARTESIAN_POINT('Ctrl Pts',(8.08457893799994,11.6,-6.60638953300002));
#174632=CARTESIAN_POINT('Ctrl Pts',(8.08578647499994,15.2,-6.60711901000001));
#174633=CARTESIAN_POINT('Ctrl Pts',(8.08578647499994,11.6,-6.60711901000001));
#174634=CARTESIAN_POINT('Ctrl Pts',(8.08700181499994,15.2,-6.60785161500002));
#174635=CARTESIAN_POINT('Ctrl Pts',(8.08700181499994,11.6,-6.60785161500002));
#174636=CARTESIAN_POINT('Ctrl Pts',(8.08822494799994,15.2,-6.60858732400002));
#174637=CARTESIAN_POINT('Ctrl Pts',(8.08822494799994,11.6,-6.60858732400002));
#174638=CARTESIAN_POINT('Ctrl Pts',(8.08945586299994,15.2,-6.60932611600002));
#174639=CARTESIAN_POINT('Ctrl Pts',(8.08945586299994,11.6,-6.60932611600002));
#174640=CARTESIAN_POINT('Ctrl Pts',(8.09069455099995,15.2,-6.61006796600002));
#174641=CARTESIAN_POINT('Ctrl Pts',(8.09069455099995,11.6,-6.61006796600002));
#174642=CARTESIAN_POINT('Ctrl Pts',(8.09194100299995,15.2,-6.61081285000002));
#174643=CARTESIAN_POINT('Ctrl Pts',(8.09194100299995,11.6,-6.61081285000002));
#174644=CARTESIAN_POINT('Ctrl Pts',(8.09319520699994,15.2,-6.61156074800001));
#174645=CARTESIAN_POINT('Ctrl Pts',(8.09319520699994,11.6,-6.61156074800001));
#174646=CARTESIAN_POINT('Ctrl Pts',(8.09445715399994,15.2,-6.61231163600001));
#174647=CARTESIAN_POINT('Ctrl Pts',(8.09445715399994,11.6,-6.61231163600001));
#174648=CARTESIAN_POINT('Ctrl Pts',(8.09572683299994,15.2,-6.61306549100001));
#174649=CARTESIAN_POINT('Ctrl Pts',(8.09572683299994,11.6,-6.61306549100001));
#174650=CARTESIAN_POINT('Ctrl Pts',(8.09700423599995,15.2,-6.61382228900001));
#174651=CARTESIAN_POINT('Ctrl Pts',(8.09700423599995,11.6,-6.61382228900001));
#174652=CARTESIAN_POINT('Ctrl Pts',(8.09828935199995,15.2,-6.61458201000002));
#174653=CARTESIAN_POINT('Ctrl Pts',(8.09828935199995,11.6,-6.61458201000002));
#174654=CARTESIAN_POINT('Ctrl Pts',(8.09958216999994,15.2,-6.61534463100002));
#174655=CARTESIAN_POINT('Ctrl Pts',(8.09958216999994,11.6,-6.61534463100002));
#174656=CARTESIAN_POINT('Ctrl Pts',(8.10088268299994,15.2,-6.61611012900002));
#174657=CARTESIAN_POINT('Ctrl Pts',(8.10088268299994,11.6,-6.61611012900002));
#174658=CARTESIAN_POINT('Ctrl Pts',(8.10219087899995,15.2,-6.61687848200001));
#174659=CARTESIAN_POINT('Ctrl Pts',(8.10219087899995,11.6,-6.61687848200001));
#174660=CARTESIAN_POINT('Ctrl Pts',(8.10350674899994,15.2,-6.61764966700002));
#174661=CARTESIAN_POINT('Ctrl Pts',(8.10350674899994,11.6,-6.61764966700002));
#174662=CARTESIAN_POINT('Ctrl Pts',(8.10483028199994,15.2,-6.61842366300001));
#174663=CARTESIAN_POINT('Ctrl Pts',(8.10483028199994,11.6,-6.61842366300001));
#174664=CARTESIAN_POINT('Ctrl Pts',(8.10616147099994,15.2,-6.61920044900001));
#174665=CARTESIAN_POINT('Ctrl Pts',(8.10616147099994,11.6,-6.61920044900001));
#174666=CARTESIAN_POINT('Ctrl Pts',(8.10750030299995,15.2,-6.61998000200001));
#174667=CARTESIAN_POINT('Ctrl Pts',(8.10750030299995,11.6,-6.61998000200001));
#174668=CARTESIAN_POINT('Ctrl Pts',(8.10884677199994,15.2,-6.62076229900002));
#174669=CARTESIAN_POINT('Ctrl Pts',(8.10884677199994,11.6,-6.62076229900002));
#174670=CARTESIAN_POINT('Ctrl Pts',(8.11020086499994,15.2,-6.62154732200002));
#174671=CARTESIAN_POINT('Ctrl Pts',(8.11020086499994,11.6,-6.62154732200002));
#174672=CARTESIAN_POINT('Ctrl Pts',(8.11156257299994,15.2,-6.62233504500002));
#174673=CARTESIAN_POINT('Ctrl Pts',(8.11156257299994,11.6,-6.62233504500002));
#174674=CARTESIAN_POINT('Ctrl Pts',(8.11293188799995,15.2,-6.62312544900002));
#174675=CARTESIAN_POINT('Ctrl Pts',(8.11293188799995,11.6,-6.62312544900002));
#174676=CARTESIAN_POINT('Ctrl Pts',(8.11430879999994,15.2,-6.62391851300002));
#174677=CARTESIAN_POINT('Ctrl Pts',(8.11430879999994,11.6,-6.62391851300002));
#174678=CARTESIAN_POINT('Ctrl Pts',(8.11569329999994,15.2,-6.62471421500002));
#174679=CARTESIAN_POINT('Ctrl Pts',(8.11569329999994,11.6,-6.62471421500002));
#174680=CARTESIAN_POINT('Ctrl Pts',(8.11708537499995,15.2,-6.62551253400002));
#174681=CARTESIAN_POINT('Ctrl Pts',(8.11708537499995,11.6,-6.62551253400002));
#174682=CARTESIAN_POINT('Ctrl Pts',(8.11848501999994,15.2,-6.62631344700002));
#174683=CARTESIAN_POINT('Ctrl Pts',(8.11848501999994,11.6,-6.62631344700002));
#174684=CARTESIAN_POINT('Ctrl Pts',(8.11989222299994,15.2,-6.62711693700002));
#174685=CARTESIAN_POINT('Ctrl Pts',(8.11989222299994,11.6,-6.62711693700002));
#174686=CARTESIAN_POINT('Ctrl Pts',(8.12130697599994,15.2,-6.62792297900002));
#174687=CARTESIAN_POINT('Ctrl Pts',(8.12130697599994,11.6,-6.62792297900002));
#174688=CARTESIAN_POINT('Ctrl Pts',(8.12272926799994,15.2,-6.62873155500002));
#174689=CARTESIAN_POINT('Ctrl Pts',(8.12272926799994,11.6,-6.62873155500002));
#174690=CARTESIAN_POINT('Ctrl Pts',(8.12415908999995,15.2,-6.62954264200001));
#174691=CARTESIAN_POINT('Ctrl Pts',(8.12415908999995,11.6,-6.62954264200001));
#174692=CARTESIAN_POINT('Ctrl Pts',(8.12559643299995,15.2,-6.63035622100002));
#174693=CARTESIAN_POINT('Ctrl Pts',(8.12559643299995,11.6,-6.63035622100002));
#174694=CARTESIAN_POINT('Ctrl Pts',(8.12704128799994,15.2,-6.63117227000001));
#174695=CARTESIAN_POINT('Ctrl Pts',(8.12704128799994,11.6,-6.63117227000001));
#174696=CARTESIAN_POINT('Ctrl Pts',(8.12849364599994,15.2,-6.63199077000002));
#174697=CARTESIAN_POINT('Ctrl Pts',(8.12849364599994,11.6,-6.63199077000002));
#174698=CARTESIAN_POINT('Ctrl Pts',(8.12995349699994,15.2,-6.63281170000002));
#174699=CARTESIAN_POINT('Ctrl Pts',(8.12995349699994,11.6,-6.63281170000002));
#174700=CARTESIAN_POINT('Ctrl Pts',(8.13142083099994,15.2,-6.63363503900002));
#174701=CARTESIAN_POINT('Ctrl Pts',(8.13142083099994,11.6,-6.63363503900002));
#174702=CARTESIAN_POINT('Ctrl Pts',(8.13289563999994,15.2,-6.63446076700002));
#174703=CARTESIAN_POINT('Ctrl Pts',(8.13289563999994,11.6,-6.63446076700002));
#174704=CARTESIAN_POINT('Ctrl Pts',(8.13437791499994,15.2,-6.63528886500002));
#174705=CARTESIAN_POINT('Ctrl Pts',(8.13437791499994,11.6,-6.63528886500002));
#174706=CARTESIAN_POINT('Ctrl Pts',(8.13586764499994,15.2,-6.63611931100001));
#174707=CARTESIAN_POINT('Ctrl Pts',(8.13586764499994,11.6,-6.63611931100001));
#174708=CARTESIAN_POINT('Ctrl Pts',(8.13736482299995,15.2,-6.63695208700001));
#174709=CARTESIAN_POINT('Ctrl Pts',(8.13736482299995,11.6,-6.63695208700001));
#174710=CARTESIAN_POINT('Ctrl Pts',(8.13886943899995,15.2,-6.63778717100002));
#174711=CARTESIAN_POINT('Ctrl Pts',(8.13886943899995,11.6,-6.63778717100002));
#174712=CARTESIAN_POINT('Ctrl Pts',(8.14038148299994,15.2,-6.63862454400002));
#174713=CARTESIAN_POINT('Ctrl Pts',(8.14038148299994,11.6,-6.63862454400002));
#174714=CARTESIAN_POINT('Ctrl Pts',(8.14190094599994,15.2,-6.63946418600001));
#174715=CARTESIAN_POINT('Ctrl Pts',(8.14190094599994,11.6,-6.63946418600001));
#174716=CARTESIAN_POINT('Ctrl Pts',(8.14342782099994,15.2,-6.64030607900001));
#174717=CARTESIAN_POINT('Ctrl Pts',(8.14342782099994,11.6,-6.64030607900001));
#174718=CARTESIAN_POINT('Ctrl Pts',(8.14496209699995,15.2,-6.64115020100001));
#174719=CARTESIAN_POINT('Ctrl Pts',(8.14496209699995,11.6,-6.64115020100001));
#174720=CARTESIAN_POINT('Ctrl Pts',(8.14650376499995,15.2,-6.64199653400001));
#174721=CARTESIAN_POINT('Ctrl Pts',(8.14650376499995,11.6,-6.64199653400001));
#174722=CARTESIAN_POINT('Ctrl Pts',(8.14805281799994,15.2,-6.64284505700002));
#174723=CARTESIAN_POINT('Ctrl Pts',(8.14805281799994,11.6,-6.64284505700002));
#174724=CARTESIAN_POINT('Ctrl Pts',(8.14960924299994,15.2,-6.64369575200002));
#174725=CARTESIAN_POINT('Ctrl Pts',(8.14960924299994,11.6,-6.64369575200002));
#174726=CARTESIAN_POINT('Ctrl Pts',(8.15117303599994,15.2,-6.64454860000002));
#174727=CARTESIAN_POINT('Ctrl Pts',(8.15117303599994,11.6,-6.64454860000002));
#174728=CARTESIAN_POINT('Ctrl Pts',(8.15274418299994,15.2,-6.64540358000002));
#174729=CARTESIAN_POINT('Ctrl Pts',(8.15274418299994,11.6,-6.64540358000002));
#174730=CARTESIAN_POINT('Ctrl Pts',(8.15432267899994,15.2,-6.64626067400001));
#174731=CARTESIAN_POINT('Ctrl Pts',(8.15432267899994,11.6,-6.64626067400001));
#174732=CARTESIAN_POINT('Ctrl Pts',(8.15590851399994,15.2,-6.64711986300001));
#174733=CARTESIAN_POINT('Ctrl Pts',(8.15590851399994,11.6,-6.64711986300001));
#174734=CARTESIAN_POINT('Ctrl Pts',(8.15750167799994,15.2,-6.64798112700002));
#174735=CARTESIAN_POINT('Ctrl Pts',(8.15750167799994,11.6,-6.64798112700002));
#174736=CARTESIAN_POINT('Ctrl Pts',(8.15910216299994,15.2,-6.64884444900002));
#174737=CARTESIAN_POINT('Ctrl Pts',(8.15910216299994,11.6,-6.64884444900002));
#174738=CARTESIAN_POINT('Ctrl Pts',(8.16070995999995,15.2,-6.64970980800001));
#174739=CARTESIAN_POINT('Ctrl Pts',(8.16070995999995,11.6,-6.64970980800001));
#174740=CARTESIAN_POINT('Ctrl Pts',(8.16232505999994,15.2,-6.65057718600002));
#174741=CARTESIAN_POINT('Ctrl Pts',(8.16232505999994,11.6,-6.65057718600002));
#174742=CARTESIAN_POINT('Ctrl Pts',(8.16394745599995,15.2,-6.65144656500001));
#174743=CARTESIAN_POINT('Ctrl Pts',(8.16394745599995,11.6,-6.65144656500001));
#174744=CARTESIAN_POINT('Ctrl Pts',(8.16557713499994,15.2,-6.65231792500002));
#174745=CARTESIAN_POINT('Ctrl Pts',(8.16557713499994,11.6,-6.65231792500002));
#174746=CARTESIAN_POINT('Ctrl Pts',(8.16721409299995,15.2,-6.65319124900002));
#174747=CARTESIAN_POINT('Ctrl Pts',(8.16721409299995,11.6,-6.65319124900002));
#174748=CARTESIAN_POINT('Ctrl Pts',(8.16885831799994,15.2,-6.65406651700001));
#174749=CARTESIAN_POINT('Ctrl Pts',(8.16885831799994,11.6,-6.65406651700001));
#174750=CARTESIAN_POINT('Ctrl Pts',(8.17050980299994,15.2,-6.65494371200002));
#174751=CARTESIAN_POINT('Ctrl Pts',(8.17050980299994,11.6,-6.65494371200002));
#174752=CARTESIAN_POINT('Ctrl Pts',(8.17216853799994,15.2,-6.65582281300001));
#174753=CARTESIAN_POINT('Ctrl Pts',(8.17216853799994,11.6,-6.65582281300001));
#174754=CARTESIAN_POINT('Ctrl Pts',(8.17383451599994,15.2,-6.65670380500002));
#174755=CARTESIAN_POINT('Ctrl Pts',(8.17383451599994,11.6,-6.65670380500002));
#174756=CARTESIAN_POINT('Ctrl Pts',(8.17550772699994,15.2,-6.65758666800001));
#174757=CARTESIAN_POINT('Ctrl Pts',(8.17550772699994,11.6,-6.65758666800001));
#174758=CARTESIAN_POINT('Ctrl Pts',(8.17718816199994,15.2,-6.65847138400002));
#174759=CARTESIAN_POINT('Ctrl Pts',(8.17718816199994,11.6,-6.65847138400002));
#174760=CARTESIAN_POINT('Ctrl Pts',(8.17887581399994,15.2,-6.65935793500001));
#174761=CARTESIAN_POINT('Ctrl Pts',(8.17887581399994,11.6,-6.65935793500001));
#174762=CARTESIAN_POINT('Ctrl Pts',(8.18057067299995,15.2,-6.66024630300001));
#174763=CARTESIAN_POINT('Ctrl Pts',(8.18057067299995,11.6,-6.66024630300001));
#174764=CARTESIAN_POINT('Ctrl Pts',(8.18227273099994,15.2,-6.66113646900002));
#174765=CARTESIAN_POINT('Ctrl Pts',(8.18227273099994,11.6,-6.66113646900002));
#174766=CARTESIAN_POINT('Ctrl Pts',(8.18398197899995,15.2,-6.66202841800001));
#174767=CARTESIAN_POINT('Ctrl Pts',(8.18398197899995,11.6,-6.66202841800001));
#174768=CARTESIAN_POINT('Ctrl Pts',(8.18569840899994,15.2,-6.66292212900002));
#174769=CARTESIAN_POINT('Ctrl Pts',(8.18569840899994,11.6,-6.66292212900002));
#174770=CARTESIAN_POINT('Ctrl Pts',(8.18742201199994,15.2,-6.66381758700001));
#174771=CARTESIAN_POINT('Ctrl Pts',(8.18742201199994,11.6,-6.66381758700001));
#174772=CARTESIAN_POINT('Ctrl Pts',(8.18915277999994,15.2,-6.66471477100002));
#174773=CARTESIAN_POINT('Ctrl Pts',(8.18915277999994,11.6,-6.66471477100002));
#174774=CARTESIAN_POINT('Ctrl Pts',(8.19089070299994,15.2,-6.66561366600002));
#174775=CARTESIAN_POINT('Ctrl Pts',(8.19089070299994,11.6,-6.66561366600002));
#174776=CARTESIAN_POINT('Ctrl Pts',(8.19263577499994,15.2,-6.66651425400002));
#174777=CARTESIAN_POINT('Ctrl Pts',(8.19263577499994,11.6,-6.66651425400002));
#174778=CARTESIAN_POINT('Ctrl Pts',(8.19438798599995,15.2,-6.66741651700002));
#174779=CARTESIAN_POINT('Ctrl Pts',(8.19438798599995,11.6,-6.66741651700002));
#174780=CARTESIAN_POINT('Ctrl Pts',(8.19614732799994,15.2,-6.66832043800002));
#174781=CARTESIAN_POINT('Ctrl Pts',(8.19614732799994,11.6,-6.66832043800002));
#174782=CARTESIAN_POINT('Ctrl Pts',(8.19791379199994,15.2,-6.66922599900002));
#174783=CARTESIAN_POINT('Ctrl Pts',(8.19791379199994,11.6,-6.66922599900002));
#174784=CARTESIAN_POINT('Ctrl Pts',(8.19968736899994,15.2,-6.67013318300001));
#174785=CARTESIAN_POINT('Ctrl Pts',(8.19968736899994,11.6,-6.67013318300001));
#174786=CARTESIAN_POINT('Ctrl Pts',(8.20146805299995,15.2,-6.67104197300001));
#174787=CARTESIAN_POINT('Ctrl Pts',(8.20146805299995,11.6,-6.67104197300001));
#174788=CARTESIAN_POINT('Ctrl Pts',(8.20325583299994,15.2,-6.67195235100002));
#174789=CARTESIAN_POINT('Ctrl Pts',(8.20325583299994,11.6,-6.67195235100002));
#174790=CARTESIAN_POINT('Ctrl Pts',(8.20505070199994,15.2,-6.67286430200001));
#174791=CARTESIAN_POINT('Ctrl Pts',(8.20505070199994,11.6,-6.67286430200001));
#174792=CARTESIAN_POINT('Ctrl Pts',(8.20685265099995,15.2,-6.67377780700001));
#174793=CARTESIAN_POINT('Ctrl Pts',(8.20685265099995,11.6,-6.67377780700001));
#174794=CARTESIAN_POINT('Ctrl Pts',(8.20866167299994,15.2,-6.67469284900001));
#174795=CARTESIAN_POINT('Ctrl Pts',(8.20866167299994,11.6,-6.67469284900001));
#174796=CARTESIAN_POINT('Ctrl Pts',(8.21047775899994,15.2,-6.67560941200002));
#174797=CARTESIAN_POINT('Ctrl Pts',(8.21047775899994,11.6,-6.67560941200002));
#174798=CARTESIAN_POINT('Ctrl Pts',(8.21230089999995,15.2,-6.67652747800001));
#174799=CARTESIAN_POINT('Ctrl Pts',(8.21230089999995,11.6,-6.67652747800001));
#174800=CARTESIAN_POINT('Ctrl Pts',(8.21413108799995,15.2,-6.67744703200002));
#174801=CARTESIAN_POINT('Ctrl Pts',(8.21413108799995,11.6,-6.67744703200002));
#174802=CARTESIAN_POINT('Ctrl Pts',(8.21596831499994,15.2,-6.67836805600002));
#174803=CARTESIAN_POINT('Ctrl Pts',(8.21596831499994,11.6,-6.67836805600002));
#174804=CARTESIAN_POINT('Ctrl Pts',(8.21781257299994,15.2,-6.67929053200002));
#174805=CARTESIAN_POINT('Ctrl Pts',(8.21781257299994,11.6,-6.67929053200002));
#174806=CARTESIAN_POINT('Ctrl Pts',(8.21966385399995,15.2,-6.68021444700001));
#174807=CARTESIAN_POINT('Ctrl Pts',(8.21966385399995,11.6,-6.68021444700001));
#174808=CARTESIAN_POINT('Ctrl Pts',(8.22152214799994,15.2,-6.68113978100001));
#174809=CARTESIAN_POINT('Ctrl Pts',(8.22152214799994,11.6,-6.68113978100001));
#174810=CARTESIAN_POINT('Ctrl Pts',(8.22338744899995,15.2,-6.68206651900002));
#174811=CARTESIAN_POINT('Ctrl Pts',(8.22338744899995,11.6,-6.68206651900002));
#174812=CARTESIAN_POINT('Ctrl Pts',(8.22525974799994,15.2,-6.68299464400001));
#174813=CARTESIAN_POINT('Ctrl Pts',(8.22525974799994,11.6,-6.68299464400001));
#174814=CARTESIAN_POINT('Ctrl Pts',(8.22713903599994,15.2,-6.68392414100002));
#174815=CARTESIAN_POINT('Ctrl Pts',(8.22713903599994,11.6,-6.68392414100002));
#174816=CARTESIAN_POINT('Ctrl Pts',(8.22902530599994,15.2,-6.68485499200001));
#174817=CARTESIAN_POINT('Ctrl Pts',(8.22902530599994,11.6,-6.68485499200001));
#174818=CARTESIAN_POINT('Ctrl Pts',(8.23091854999995,15.2,-6.68578718100001));
#174819=CARTESIAN_POINT('Ctrl Pts',(8.23091854999995,11.6,-6.68578718100001));
#174820=CARTESIAN_POINT('Ctrl Pts',(8.23281875799994,15.2,-6.68672069200002));
#174821=CARTESIAN_POINT('Ctrl Pts',(8.23281875799994,11.6,-6.68672069200002));
#174822=CARTESIAN_POINT('Ctrl Pts',(8.23472592499994,15.2,-6.68765551000002));
#174823=CARTESIAN_POINT('Ctrl Pts',(8.23472592499994,11.6,-6.68765551000002));
#174824=CARTESIAN_POINT('Ctrl Pts',(8.23664004099994,15.2,-6.68859161700002));
#174825=CARTESIAN_POINT('Ctrl Pts',(8.23664004099994,11.6,-6.68859161700002));
#174826=CARTESIAN_POINT('Ctrl Pts',(8.23856109699994,15.2,-6.68952899800002));
#174827=CARTESIAN_POINT('Ctrl Pts',(8.23856109699994,11.6,-6.68952899800002));
#174828=CARTESIAN_POINT('Ctrl Pts',(8.24048908699995,15.2,-6.69046763800001));
#174829=CARTESIAN_POINT('Ctrl Pts',(8.24048908699995,11.6,-6.69046763800001));
#174830=CARTESIAN_POINT('Ctrl Pts',(8.24242400099994,15.2,-6.69140751800001));
#174831=CARTESIAN_POINT('Ctrl Pts',(8.24242400099994,11.6,-6.69140751800001));
#174832=CARTESIAN_POINT('Ctrl Pts',(8.24436583299994,15.2,-6.69234862500002));
#174833=CARTESIAN_POINT('Ctrl Pts',(8.24436583299994,11.6,-6.69234862500002));
#174834=CARTESIAN_POINT('Ctrl Pts',(8.24631457299994,15.2,-6.69329094200001));
#174835=CARTESIAN_POINT('Ctrl Pts',(8.24631457299994,11.6,-6.69329094200001));
#174836=CARTESIAN_POINT('Ctrl Pts',(8.24827021499994,15.2,-6.69423445400002));
#174837=CARTESIAN_POINT('Ctrl Pts',(8.24827021499994,11.6,-6.69423445400002));
#174838=CARTESIAN_POINT('Ctrl Pts',(8.25023274999995,15.2,-6.69517914500001));
#174839=CARTESIAN_POINT('Ctrl Pts',(8.25023274999995,11.6,-6.69517914500001));
#174840=CARTESIAN_POINT('Ctrl Pts',(8.25220216899995,15.2,-6.69612499700002));
#174841=CARTESIAN_POINT('Ctrl Pts',(8.25220216899995,11.6,-6.69612499700002));
#174842=CARTESIAN_POINT('Ctrl Pts',(8.25417846599995,15.2,-6.69707199800002));
#174843=CARTESIAN_POINT('Ctrl Pts',(8.25417846599995,11.6,-6.69707199800002));
#174844=CARTESIAN_POINT('Ctrl Pts',(8.25616163199994,15.2,-6.69802013100002));
#174845=CARTESIAN_POINT('Ctrl Pts',(8.25616163199994,11.6,-6.69802013100002));
#174846=CARTESIAN_POINT('Ctrl Pts',(8.25815165799994,15.2,-6.69896938100001));
#174847=CARTESIAN_POINT('Ctrl Pts',(8.25815165799994,11.6,-6.69896938100001));
#174848=CARTESIAN_POINT('Ctrl Pts',(8.26014853899995,15.2,-6.69991973000001));
#174849=CARTESIAN_POINT('Ctrl Pts',(8.26014853899995,11.6,-6.69991973000001));
#174850=CARTESIAN_POINT('Ctrl Pts',(8.26215226399994,15.2,-6.70087116600002));
#174851=CARTESIAN_POINT('Ctrl Pts',(8.26215226399994,11.6,-6.70087116600002));
#174852=CARTESIAN_POINT('Ctrl Pts',(8.26416282699994,15.2,-6.70182367200002));
#174853=CARTESIAN_POINT('Ctrl Pts',(8.26416282699994,11.6,-6.70182367200002));
#174854=CARTESIAN_POINT('Ctrl Pts',(8.26618022099994,15.2,-6.70277723300002));
#174855=CARTESIAN_POINT('Ctrl Pts',(8.26618022099994,11.6,-6.70277723300002));
#174856=CARTESIAN_POINT('Ctrl Pts',(8.26820443599994,15.2,-6.70373183400002));
#174857=CARTESIAN_POINT('Ctrl Pts',(8.26820443599994,11.6,-6.70373183400002));
#174858=CARTESIAN_POINT('Ctrl Pts',(8.27023546499994,15.2,-6.70468746000001));
#174859=CARTESIAN_POINT('Ctrl Pts',(8.27023546499994,11.6,-6.70468746000001));
#174860=CARTESIAN_POINT('Ctrl Pts',(8.27227329999995,15.2,-6.70564409400002));
#174861=CARTESIAN_POINT('Ctrl Pts',(8.27227329999995,11.6,-6.70564409400002));
#174862=CARTESIAN_POINT('Ctrl Pts',(8.27431793299995,15.2,-6.70660172400002));
#174863=CARTESIAN_POINT('Ctrl Pts',(8.27431793299995,11.6,-6.70660172400002));
#174864=CARTESIAN_POINT('Ctrl Pts',(8.27636935699994,15.2,-6.70756033100002));
#174865=CARTESIAN_POINT('Ctrl Pts',(8.27636935699994,11.6,-6.70756033100002));
#174866=CARTESIAN_POINT('Ctrl Pts',(8.27842756399994,15.2,-6.70851990500001));
#174867=CARTESIAN_POINT('Ctrl Pts',(8.27842756399994,11.6,-6.70851990500001));
#174868=CARTESIAN_POINT('Ctrl Pts',(8.28049254599994,15.2,-6.70948042700001));
#174869=CARTESIAN_POINT('Ctrl Pts',(8.28049254599994,11.6,-6.70948042700001));
#174870=CARTESIAN_POINT('Ctrl Pts',(8.28256429399995,15.2,-6.71044188300002));
#174871=CARTESIAN_POINT('Ctrl Pts',(8.28256429399995,11.6,-6.71044188300002));
#174872=CARTESIAN_POINT('Ctrl Pts',(8.28464280299994,15.2,-6.71140425900001));
#174873=CARTESIAN_POINT('Ctrl Pts',(8.28464280299994,11.6,-6.71140425900001));
#174874=CARTESIAN_POINT('Ctrl Pts',(8.28672806299994,15.2,-6.71236754000001));
#174875=CARTESIAN_POINT('Ctrl Pts',(8.28672806299994,11.6,-6.71236754000001));
#174876=CARTESIAN_POINT('Ctrl Pts',(8.28882006799994,15.2,-6.71333171200001));
#174877=CARTESIAN_POINT('Ctrl Pts',(8.28882006799994,11.6,-6.71333171200001));
#174878=CARTESIAN_POINT('Ctrl Pts',(8.29091880799994,15.2,-6.71429675900002));
#174879=CARTESIAN_POINT('Ctrl Pts',(8.29091880799994,11.6,-6.71429675900002));
#174880=CARTESIAN_POINT('Ctrl Pts',(8.29302427799994,15.2,-6.71526266700001));
#174881=CARTESIAN_POINT('Ctrl Pts',(8.29302427799994,11.6,-6.71526266700001));
#174882=CARTESIAN_POINT('Ctrl Pts',(8.29513646899994,15.2,-6.71622942100001));
#174883=CARTESIAN_POINT('Ctrl Pts',(8.29513646899994,11.6,-6.71622942100001));
#174884=CARTESIAN_POINT('Ctrl Pts',(8.29725537199994,15.2,-6.71719700700002));
#174885=CARTESIAN_POINT('Ctrl Pts',(8.29725537199994,11.6,-6.71719700700002));
#174886=CARTESIAN_POINT('Ctrl Pts',(8.29938098199994,15.2,-6.71816541100001));
#174887=CARTESIAN_POINT('Ctrl Pts',(8.29938098199994,11.6,-6.71816541100001));
#174888=CARTESIAN_POINT('Ctrl Pts',(8.30151328999994,15.2,-6.71913461700001));
#174889=CARTESIAN_POINT('Ctrl Pts',(8.30151328999994,11.6,-6.71913461700001));
#174890=CARTESIAN_POINT('Ctrl Pts',(8.30365228799994,15.2,-6.72010461100002));
#174891=CARTESIAN_POINT('Ctrl Pts',(8.30365228799994,11.6,-6.72010461100002));
#174892=CARTESIAN_POINT('Ctrl Pts',(8.30579796699995,15.2,-6.72107538000001));
#174893=CARTESIAN_POINT('Ctrl Pts',(8.30579796699995,11.6,-6.72107538000001));
#174894=CARTESIAN_POINT('Ctrl Pts',(8.30795032399994,15.2,-6.72204690800001));
#174895=CARTESIAN_POINT('Ctrl Pts',(8.30795032399994,11.6,-6.72204690800001));
#174896=CARTESIAN_POINT('Ctrl Pts',(8.31010934699994,15.2,-6.72301918300001));
#174897=CARTESIAN_POINT('Ctrl Pts',(8.31010934699994,11.6,-6.72301918300001));
#174898=CARTESIAN_POINT('Ctrl Pts',(8.31227502999995,15.2,-6.72399218800001));
#174899=CARTESIAN_POINT('Ctrl Pts',(8.31227502999995,11.6,-6.72399218800001));
#174900=CARTESIAN_POINT('Ctrl Pts',(8.31444736699994,15.2,-6.72496591100002));
#174901=CARTESIAN_POINT('Ctrl Pts',(8.31444736699994,11.6,-6.72496591100002));
#174902=CARTESIAN_POINT('Ctrl Pts',(8.31662634799994,15.2,-6.72594033700002));
#174903=CARTESIAN_POINT('Ctrl Pts',(8.31662634799994,11.6,-6.72594033700002));
#174904=CARTESIAN_POINT('Ctrl Pts',(8.31881196599995,15.2,-6.72691545200002));
#174905=CARTESIAN_POINT('Ctrl Pts',(8.31881196599995,11.6,-6.72691545200002));
#174906=CARTESIAN_POINT('Ctrl Pts',(8.32100421399995,15.2,-6.72789124100002));
#174907=CARTESIAN_POINT('Ctrl Pts',(8.32100421399995,11.6,-6.72789124100002));
#174908=CARTESIAN_POINT('Ctrl Pts',(8.32320308399994,15.2,-6.72886769200002));
#174909=CARTESIAN_POINT('Ctrl Pts',(8.32320308399994,11.6,-6.72886769200002));
#174910=CARTESIAN_POINT('Ctrl Pts',(8.32540856899995,15.2,-6.72984479000001));
#174911=CARTESIAN_POINT('Ctrl Pts',(8.32540856899995,11.6,-6.72984479000001));
#174912=CARTESIAN_POINT('Ctrl Pts',(8.32762066299994,15.2,-6.73082252200001));
#174913=CARTESIAN_POINT('Ctrl Pts',(8.32762066299994,11.6,-6.73082252200001));
#174914=CARTESIAN_POINT('Ctrl Pts',(8.32983935499995,15.2,-6.73180087200001));
#174915=CARTESIAN_POINT('Ctrl Pts',(8.32983935499995,11.6,-6.73180087200001));
#174916=CARTESIAN_POINT('Ctrl Pts',(8.33206463999994,15.2,-6.73277982900002));
#174917=CARTESIAN_POINT('Ctrl Pts',(8.33206463999994,11.6,-6.73277982900002));
#174918=CARTESIAN_POINT('Ctrl Pts',(8.33429650899994,15.2,-6.73375937700002));
#174919=CARTESIAN_POINT('Ctrl Pts',(8.33429650899994,11.6,-6.73375937700002));
#174920=CARTESIAN_POINT('Ctrl Pts',(8.33653495599994,15.2,-6.73473950400002));
#174921=CARTESIAN_POINT('Ctrl Pts',(8.33653495599994,11.6,-6.73473950400002));
#174922=CARTESIAN_POINT('Ctrl Pts',(8.33877997299994,15.2,-6.73572019500002));
#174923=CARTESIAN_POINT('Ctrl Pts',(8.33877997299994,11.6,-6.73572019500002));
#174924=CARTESIAN_POINT('Ctrl Pts',(8.34103155399994,15.2,-6.73670143600001));
#174925=CARTESIAN_POINT('Ctrl Pts',(8.34103155399994,11.6,-6.73670143600001));
#174926=CARTESIAN_POINT('Ctrl Pts',(8.34328968799994,15.2,-6.73768321600001));
#174927=CARTESIAN_POINT('Ctrl Pts',(8.34328968799994,11.6,-6.73768321600001));
#174928=CARTESIAN_POINT('Ctrl Pts',(8.34555437099995,15.2,-6.73866551800002));
#174929=CARTESIAN_POINT('Ctrl Pts',(8.34555437099995,11.6,-6.73866551800002));
#174930=CARTESIAN_POINT('Ctrl Pts',(8.34782559499994,15.2,-6.73964833200002));
#174931=CARTESIAN_POINT('Ctrl Pts',(8.34782559499994,11.6,-6.73964833200002));
#174932=CARTESIAN_POINT('Ctrl Pts',(8.35010335099994,15.2,-6.74063164200001));
#174933=CARTESIAN_POINT('Ctrl Pts',(8.35010335099994,11.6,-6.74063164200001));
#174934=CARTESIAN_POINT('Ctrl Pts',(8.35238763299994,15.2,-6.74161543600002));
#174935=CARTESIAN_POINT('Ctrl Pts',(8.35238763299994,11.6,-6.74161543600002));
#174936=CARTESIAN_POINT('Ctrl Pts',(8.35467843299995,15.2,-6.74259969900002));
#174937=CARTESIAN_POINT('Ctrl Pts',(8.35467843299995,11.6,-6.74259969900002));
#174938=CARTESIAN_POINT('Ctrl Pts',(8.35697574399994,15.2,-6.74358442000001));
#174939=CARTESIAN_POINT('Ctrl Pts',(8.35697574399994,11.6,-6.74358442000001));
#174940=CARTESIAN_POINT('Ctrl Pts',(8.35927955899994,15.2,-6.74456958300001));
#174941=CARTESIAN_POINT('Ctrl Pts',(8.35927955899994,11.6,-6.74456958300001));
#174942=CARTESIAN_POINT('Ctrl Pts',(8.36158986899994,15.2,-6.74555517700002));
#174943=CARTESIAN_POINT('Ctrl Pts',(8.36158986899994,11.6,-6.74555517700002));
#174944=CARTESIAN_POINT('Ctrl Pts',(8.36390666999994,15.2,-6.74654118800002));
#174945=CARTESIAN_POINT('Ctrl Pts',(8.36390666999994,11.6,-6.74654118800002));
#174946=CARTESIAN_POINT('Ctrl Pts',(8.36622995199994,15.2,-6.74752760300001));
#174947=CARTESIAN_POINT('Ctrl Pts',(8.36622995199994,11.6,-6.74752760300001));
#174948=CARTESIAN_POINT('Ctrl Pts',(8.36855970799994,15.2,-6.74851440900002));
#174949=CARTESIAN_POINT('Ctrl Pts',(8.36855970799994,11.6,-6.74851440900002));
#174950=CARTESIAN_POINT('Ctrl Pts',(8.37089593099994,15.2,-6.74950159200002));
#174951=CARTESIAN_POINT('Ctrl Pts',(8.37089593099994,11.6,-6.74950159200002));
#174952=CARTESIAN_POINT('Ctrl Pts',(8.37323861399994,15.2,-6.75048914100002));
#174953=CARTESIAN_POINT('Ctrl Pts',(8.37323861399994,11.6,-6.75048914100002));
#174954=CARTESIAN_POINT('Ctrl Pts',(8.37558774999994,15.2,-6.75147704100001));
#174955=CARTESIAN_POINT('Ctrl Pts',(8.37558774999994,11.6,-6.75147704100001));
#174956=CARTESIAN_POINT('Ctrl Pts',(8.37794332999995,15.2,-6.75246527900002));
#174957=CARTESIAN_POINT('Ctrl Pts',(8.37794332999995,11.6,-6.75246527900002));
#174958=CARTESIAN_POINT('Ctrl Pts',(8.38030534899995,15.2,-6.75345384400002));
#174959=CARTESIAN_POINT('Ctrl Pts',(8.38030534899995,11.6,-6.75345384400002));
#174960=CARTESIAN_POINT('Ctrl Pts',(8.38267379899994,15.2,-6.75444272200002));
#174961=CARTESIAN_POINT('Ctrl Pts',(8.38267379899994,11.6,-6.75444272200002));
#174962=CARTESIAN_POINT('Ctrl Pts',(8.38504867299994,15.2,-6.75543189900001));
#174963=CARTESIAN_POINT('Ctrl Pts',(8.38504867299994,11.6,-6.75543189900001));
#174964=CARTESIAN_POINT('Ctrl Pts',(8.38742996299995,15.2,-6.75642136400001));
#174965=CARTESIAN_POINT('Ctrl Pts',(8.38742996299995,11.6,-6.75642136400001));
#174966=CARTESIAN_POINT('Ctrl Pts',(8.38981766199994,15.2,-6.75741110400002));
#174967=CARTESIAN_POINT('Ctrl Pts',(8.38981766199994,11.6,-6.75741110400002));
#174968=CARTESIAN_POINT('Ctrl Pts',(8.39221176299995,15.2,-6.75840110500002));
#174969=CARTESIAN_POINT('Ctrl Pts',(8.39221176299995,11.6,-6.75840110500002));
#174970=CARTESIAN_POINT('Ctrl Pts',(8.39461225899995,15.2,-6.75939135600002));
#174971=CARTESIAN_POINT('Ctrl Pts',(8.39461225899995,11.6,-6.75939135600002));
#174972=CARTESIAN_POINT('Ctrl Pts',(8.39701914299994,15.2,-6.76038184300002));
#174973=CARTESIAN_POINT('Ctrl Pts',(8.39701914299994,11.6,-6.76038184300002));
#174974=CARTESIAN_POINT('Ctrl Pts',(8.39943240599995,15.2,-6.76137255500001));
#174975=CARTESIAN_POINT('Ctrl Pts',(8.39943240599995,11.6,-6.76137255500001));
#174976=CARTESIAN_POINT('Ctrl Pts',(8.40185204399994,15.2,-6.76236347800002));
#174977=CARTESIAN_POINT('Ctrl Pts',(8.40185204399994,11.6,-6.76236347800002));
#174978=CARTESIAN_POINT('Ctrl Pts',(8.40427804899995,15.2,-6.76335459900002));
#174979=CARTESIAN_POINT('Ctrl Pts',(8.40427804899995,11.6,-6.76335459900002));
#174980=CARTESIAN_POINT('Ctrl Pts',(8.40671041099995,15.2,-6.76434590800002));
#174981=CARTESIAN_POINT('Ctrl Pts',(8.40671041099995,11.6,-6.76434590800002));
#174982=CARTESIAN_POINT('Ctrl Pts',(8.40914912599995,15.2,-6.76533739000002));
#174983=CARTESIAN_POINT('Ctrl Pts',(8.40914912599995,11.6,-6.76533739000002));
#174984=CARTESIAN_POINT('Ctrl Pts',(8.41159418599995,15.2,-6.76632903300002));
#174985=CARTESIAN_POINT('Ctrl Pts',(8.41159418599995,11.6,-6.76632903300002));
#174986=CARTESIAN_POINT('Ctrl Pts',(8.41404558399995,15.2,-6.76732082600001));
#174987=CARTESIAN_POINT('Ctrl Pts',(8.41404558399995,11.6,-6.76732082600001));
#174988=CARTESIAN_POINT('Ctrl Pts',(8.41650331199994,15.2,-6.76831275600002));
#174989=CARTESIAN_POINT('Ctrl Pts',(8.41650331199994,11.6,-6.76831275600002));
#174990=CARTESIAN_POINT('Ctrl Pts',(8.41896736399995,15.2,-6.76930481000002));
#174991=CARTESIAN_POINT('Ctrl Pts',(8.41896736399995,11.6,-6.76930481000002));
#174992=CARTESIAN_POINT('Ctrl Pts',(8.42143773199994,15.2,-6.77029697800001));
#174993=CARTESIAN_POINT('Ctrl Pts',(8.42143773199994,11.6,-6.77029697800001));
#174994=CARTESIAN_POINT('Ctrl Pts',(8.42391440899994,15.2,-6.77128924400002));
#174995=CARTESIAN_POINT('Ctrl Pts',(8.42391440899994,11.6,-6.77128924400002));
#174996=CARTESIAN_POINT('Ctrl Pts',(8.42639738999994,15.2,-6.77228159900002));
#174997=CARTESIAN_POINT('Ctrl Pts',(8.42639738999994,11.6,-6.77228159900002));
#174998=CARTESIAN_POINT('Ctrl Pts',(8.42888666599995,15.2,-6.77327402900002));
#174999=CARTESIAN_POINT('Ctrl Pts',(8.42888666599995,11.6,-6.77327402900002));
#175000=CARTESIAN_POINT('Ctrl Pts',(8.43138222999994,15.2,-6.77426652400002));
#175001=CARTESIAN_POINT('Ctrl Pts',(8.43138222999994,11.6,-6.77426652400002));
#175002=CARTESIAN_POINT('Ctrl Pts',(8.43388407399994,15.2,-6.77525907100001));
#175003=CARTESIAN_POINT('Ctrl Pts',(8.43388407399994,11.6,-6.77525907100001));
#175004=CARTESIAN_POINT('Ctrl Pts',(8.43639219399994,15.2,-6.77625165600002));
#175005=CARTESIAN_POINT('Ctrl Pts',(8.43639219399994,11.6,-6.77625165600002));
#175006=CARTESIAN_POINT('Ctrl Pts',(8.43890658199994,15.2,-6.77724426900002));
#175007=CARTESIAN_POINT('Ctrl Pts',(8.43890658199994,11.6,-6.77724426900002));
#175008=CARTESIAN_POINT('Ctrl Pts',(8.44142722799995,15.2,-6.77823689800002));
#175009=CARTESIAN_POINT('Ctrl Pts',(8.44142722799995,11.6,-6.77823689800002));
#175010=CARTESIAN_POINT('Ctrl Pts',(8.44395412799994,15.2,-6.77922953000002));
#175011=CARTESIAN_POINT('Ctrl Pts',(8.44395412799994,11.6,-6.77922953000002));
#175012=CARTESIAN_POINT('Ctrl Pts',(8.44648727499994,15.2,-6.78022215500001));
#175013=CARTESIAN_POINT('Ctrl Pts',(8.44648727499994,11.6,-6.78022215500001));
#175014=CARTESIAN_POINT('Ctrl Pts',(8.44902666199994,15.2,-6.78121475900002));
#175015=CARTESIAN_POINT('Ctrl Pts',(8.44902666199994,11.6,-6.78121475900002));
#175016=CARTESIAN_POINT('Ctrl Pts',(8.45157227999995,15.2,-6.78220733100002));
#175017=CARTESIAN_POINT('Ctrl Pts',(8.45157227999995,11.6,-6.78220733100002));
#175018=CARTESIAN_POINT('Ctrl Pts',(8.45412412299994,15.2,-6.78319985900002));
#175019=CARTESIAN_POINT('Ctrl Pts',(8.45412412299994,11.6,-6.78319985900002));
#175020=CARTESIAN_POINT('Ctrl Pts',(8.45668218599995,15.2,-6.78419233300002));
#175021=CARTESIAN_POINT('Ctrl Pts',(8.45668218599995,11.6,-6.78419233300002));
#175022=CARTESIAN_POINT('Ctrl Pts',(8.45924645999995,15.2,-6.78518473800001));
#175023=CARTESIAN_POINT('Ctrl Pts',(8.45924645999995,11.6,-6.78518473800001));
#175024=CARTESIAN_POINT('Ctrl Pts',(8.46181693799995,15.2,-6.78617706500001));
#175025=CARTESIAN_POINT('Ctrl Pts',(8.46181693799995,11.6,-6.78617706500001));
#175026=CARTESIAN_POINT('Ctrl Pts',(8.46439361399994,15.2,-6.78716930200002));
#175027=CARTESIAN_POINT('Ctrl Pts',(8.46439361399994,11.6,-6.78716930200002));
#175028=CARTESIAN_POINT('Ctrl Pts',(8.46697648099994,15.2,-6.78816143700002));
#175029=CARTESIAN_POINT('Ctrl Pts',(8.46697648099994,11.6,-6.78816143700002));
#175030=CARTESIAN_POINT('Ctrl Pts',(8.46956553199994,15.2,-6.78915345800001));
#175031=CARTESIAN_POINT('Ctrl Pts',(8.46956553199994,11.6,-6.78915345800001));
#175032=CARTESIAN_POINT('Ctrl Pts',(8.47216075899994,15.2,-6.79014535300002));
#175033=CARTESIAN_POINT('Ctrl Pts',(8.47216075899994,11.6,-6.79014535300002));
#175034=CARTESIAN_POINT('Ctrl Pts',(8.47476215699994,15.2,-6.79113711200002));
#175035=CARTESIAN_POINT('Ctrl Pts',(8.47476215699994,11.6,-6.79113711200002));
#175036=CARTESIAN_POINT('Ctrl Pts',(8.47736971999994,15.2,-6.79212872300001));
#175037=CARTESIAN_POINT('Ctrl Pts',(8.47736971999994,11.6,-6.79212872300001));
#175038=CARTESIAN_POINT('Ctrl Pts',(8.47998343699994,15.2,-6.79312017300001));
#175039=CARTESIAN_POINT('Ctrl Pts',(8.47998343699994,11.6,-6.79312017300001));
#175040=CARTESIAN_POINT('Ctrl Pts',(8.48260330399994,15.2,-6.79411145300002));
#175041=CARTESIAN_POINT('Ctrl Pts',(8.48260330399994,11.6,-6.79411145300002));
#175042=CARTESIAN_POINT('Ctrl Pts',(8.48522931299994,15.2,-6.79510255000002));
#175043=CARTESIAN_POINT('Ctrl Pts',(8.48522931299994,11.6,-6.79510255000002));
#175044=CARTESIAN_POINT('Ctrl Pts',(8.48786145799994,15.2,-6.79609345300002));
#175045=CARTESIAN_POINT('Ctrl Pts',(8.48786145799994,11.6,-6.79609345300002));
#175046=CARTESIAN_POINT('Ctrl Pts',(8.49049973399995,15.2,-6.79708415100002));
#175047=CARTESIAN_POINT('Ctrl Pts',(8.49049973399995,11.6,-6.79708415100002));
#175048=CARTESIAN_POINT('Ctrl Pts',(8.49314412999994,15.2,-6.79807463300002));
#175049=CARTESIAN_POINT('Ctrl Pts',(8.49314412999994,11.6,-6.79807463300002));
#175050=CARTESIAN_POINT('Ctrl Pts',(8.49579464199994,15.2,-6.79906488700002));
#175051=CARTESIAN_POINT('Ctrl Pts',(8.49579464199994,11.6,-6.79906488700002));
#175052=CARTESIAN_POINT('Ctrl Pts',(8.49845126199994,15.2,-6.80005490200001));
#175053=CARTESIAN_POINT('Ctrl Pts',(8.49845126199994,11.6,-6.80005490200001));
#175054=CARTESIAN_POINT('Ctrl Pts',(8.50111398399994,15.2,-6.80104466700002));
#175055=CARTESIAN_POINT('Ctrl Pts',(8.50111398399994,11.6,-6.80104466700002));
#175056=CARTESIAN_POINT('Ctrl Pts',(8.50378280199994,15.2,-6.80203417000002));
#175057=CARTESIAN_POINT('Ctrl Pts',(8.50378280199994,11.6,-6.80203417000002));
#175058=CARTESIAN_POINT('Ctrl Pts',(8.50645770599994,15.2,-6.80302340200001));
#175059=CARTESIAN_POINT('Ctrl Pts',(8.50645770599994,11.6,-6.80302340200001));
#175060=CARTESIAN_POINT('Ctrl Pts',(8.50913869399994,15.2,-6.80401235000001));
#175061=CARTESIAN_POINT('Ctrl Pts',(8.50913869399994,11.6,-6.80401235000001));
#175062=CARTESIAN_POINT('Ctrl Pts',(8.51182575499994,15.2,-6.80500100300002));
#175063=CARTESIAN_POINT('Ctrl Pts',(8.51182575499994,11.6,-6.80500100300002));
#175064=CARTESIAN_POINT('Ctrl Pts',(8.51451888399994,15.2,-6.80598935000001));
#175065=CARTESIAN_POINT('Ctrl Pts',(8.51451888399994,11.6,-6.80598935000001));
#175066=CARTESIAN_POINT('Ctrl Pts',(8.51721807399995,15.2,-6.80697738100001));
#175067=CARTESIAN_POINT('Ctrl Pts',(8.51721807399995,11.6,-6.80697738100001));
#175068=CARTESIAN_POINT('Ctrl Pts',(8.51992331799994,15.2,-6.80796508400002));
#175069=CARTESIAN_POINT('Ctrl Pts',(8.51992331799994,11.6,-6.80796508400002));
#175070=CARTESIAN_POINT('Ctrl Pts',(8.52263460999995,15.2,-6.80895244900002));
#175071=CARTESIAN_POINT('Ctrl Pts',(8.52263460999995,11.6,-6.80895244900002));
#175072=CARTESIAN_POINT('Ctrl Pts',(8.52535194299995,15.2,-6.80993946500001));
#175073=CARTESIAN_POINT('Ctrl Pts',(8.52535194299995,11.6,-6.80993946500001));
#175074=CARTESIAN_POINT('Ctrl Pts',(8.52807530999995,15.2,-6.81092612000001));
#175075=CARTESIAN_POINT('Ctrl Pts',(8.52807530999995,11.6,-6.81092612000001));
#175076=CARTESIAN_POINT('Ctrl Pts',(8.53080470399994,15.2,-6.81191240500001));
#175077=CARTESIAN_POINT('Ctrl Pts',(8.53080470399994,11.6,-6.81191240500001));
#175078=CARTESIAN_POINT('Ctrl Pts',(8.53354011899994,15.2,-6.81289830700001));
#175079=CARTESIAN_POINT('Ctrl Pts',(8.53354011899994,11.6,-6.81289830700001));
#175080=CARTESIAN_POINT('Ctrl Pts',(8.53628154899994,15.2,-6.81388381600001));
#175081=CARTESIAN_POINT('Ctrl Pts',(8.53628154899994,11.6,-6.81388381600001));
#175082=CARTESIAN_POINT('Ctrl Pts',(8.53902898399994,15.2,-6.81486892200001));
#175083=CARTESIAN_POINT('Ctrl Pts',(8.53902898399994,11.6,-6.81486892200001));
#175084=CARTESIAN_POINT('Ctrl Pts',(8.54178242199995,15.2,-6.81585361400002));
#175085=CARTESIAN_POINT('Ctrl Pts',(8.54178242199995,11.6,-6.81585361400002));
#175086=CARTESIAN_POINT('Ctrl Pts',(8.54454185299995,15.2,-6.81683788100001));
#175087=CARTESIAN_POINT('Ctrl Pts',(8.54454185299995,11.6,-6.81683788100001));
#175088=CARTESIAN_POINT('Ctrl Pts',(8.54730727099994,15.2,-6.81782171200001));
#175089=CARTESIAN_POINT('Ctrl Pts',(8.54730727099994,11.6,-6.81782171200001));
#175090=CARTESIAN_POINT('Ctrl Pts',(8.55007866999994,15.2,-6.81880509700001));
#175091=CARTESIAN_POINT('Ctrl Pts',(8.55007866999994,11.6,-6.81880509700001));
#175092=CARTESIAN_POINT('Ctrl Pts',(8.55285604299995,15.2,-6.81978802600002));
#175093=CARTESIAN_POINT('Ctrl Pts',(8.55285604299995,11.6,-6.81978802600002));
#175094=CARTESIAN_POINT('Ctrl Pts',(8.55563938299994,15.2,-6.82077048700001));
#175095=CARTESIAN_POINT('Ctrl Pts',(8.55563938299994,11.6,-6.82077048700001));
#175096=CARTESIAN_POINT('Ctrl Pts',(8.55842868299994,15.2,-6.82175247000002));
#175097=CARTESIAN_POINT('Ctrl Pts',(8.55842868299994,11.6,-6.82175247000002));
#175098=CARTESIAN_POINT('Ctrl Pts',(8.56122393899994,15.2,-6.82273396400002));
#175099=CARTESIAN_POINT('Ctrl Pts',(8.56122393899994,11.6,-6.82273396400002));
#175100=CARTESIAN_POINT('Ctrl Pts',(8.56402513999994,15.2,-6.82371496000002));
#175101=CARTESIAN_POINT('Ctrl Pts',(8.56402513999994,11.6,-6.82371496000002));
#175102=CARTESIAN_POINT('Ctrl Pts',(8.56683228399995,15.2,-6.82469544700002));
#175103=CARTESIAN_POINT('Ctrl Pts',(8.56683228399995,11.6,-6.82469544700002));
#175104=CARTESIAN_POINT('Ctrl Pts',(8.56964536099994,15.2,-6.82567541400001));
#175105=CARTESIAN_POINT('Ctrl Pts',(8.56964536099994,11.6,-6.82567541400001));
#175106=CARTESIAN_POINT('Ctrl Pts',(8.57246436599995,15.2,-6.82665485000002));
#175107=CARTESIAN_POINT('Ctrl Pts',(8.57246436599995,11.6,-6.82665485000002));
#175108=CARTESIAN_POINT('Ctrl Pts',(8.57528929199994,15.2,-6.82763374600002));
#175109=CARTESIAN_POINT('Ctrl Pts',(8.57528929199994,11.6,-6.82763374600002));
#175110=CARTESIAN_POINT('Ctrl Pts',(8.57812013199995,15.2,-6.82861209100002));
#175111=CARTESIAN_POINT('Ctrl Pts',(8.57812013199995,11.6,-6.82861209100002));
#175112=CARTESIAN_POINT('Ctrl Pts',(8.58095687899995,15.2,-6.82958987500002));
#175113=CARTESIAN_POINT('Ctrl Pts',(8.58095687899995,11.6,-6.82958987500002));
#175114=CARTESIAN_POINT('Ctrl Pts',(8.58379952799995,15.2,-6.83056708700001));
#175115=CARTESIAN_POINT('Ctrl Pts',(8.58379952799995,11.6,-6.83056708700001));
#175116=CARTESIAN_POINT('Ctrl Pts',(8.58664807299995,15.2,-6.83154371800001));
#175117=CARTESIAN_POINT('Ctrl Pts',(8.58664807299995,11.6,-6.83154371800001));
#175118=CARTESIAN_POINT('Ctrl Pts',(8.58950250399995,15.2,-6.83251975700002));
#175119=CARTESIAN_POINT('Ctrl Pts',(8.58950250399995,11.6,-6.83251975700002));
#175120=CARTESIAN_POINT('Ctrl Pts',(8.59236281799994,15.2,-6.83349519300001));
#175121=CARTESIAN_POINT('Ctrl Pts',(8.59236281799994,11.6,-6.83349519300001));
#175122=CARTESIAN_POINT('Ctrl Pts',(8.59522900599995,15.2,-6.83447001700002));
#175123=CARTESIAN_POINT('Ctrl Pts',(8.59522900599995,11.6,-6.83447001700002));
#175124=CARTESIAN_POINT('Ctrl Pts',(8.59810106299994,15.2,-6.83544421800002));
#175125=CARTESIAN_POINT('Ctrl Pts',(8.59810106299994,11.6,-6.83544421800002));
#175126=CARTESIAN_POINT('Ctrl Pts',(8.60097898199994,15.2,-6.83641778800002));
#175127=CARTESIAN_POINT('Ctrl Pts',(8.60097898199994,11.6,-6.83641778800002));
#175128=CARTESIAN_POINT('Ctrl Pts',(8.60386275599994,15.2,-6.83739071300002));
#175129=CARTESIAN_POINT('Ctrl Pts',(8.60386275599994,11.6,-6.83739071300002));
#175130=CARTESIAN_POINT('Ctrl Pts',(8.60675237799994,15.2,-6.83836298700002));
#175131=CARTESIAN_POINT('Ctrl Pts',(8.60675237799994,11.6,-6.83836298700002));
#175132=CARTESIAN_POINT('Ctrl Pts',(8.60964784399994,15.2,-6.83933459800001));
#175133=CARTESIAN_POINT('Ctrl Pts',(8.60964784399994,11.6,-6.83933459800001));
#175134=CARTESIAN_POINT('Ctrl Pts',(8.61254914499994,15.2,-6.84030553500002));
#175135=CARTESIAN_POINT('Ctrl Pts',(8.61254914499994,11.6,-6.84030553500002));
#175136=CARTESIAN_POINT('Ctrl Pts',(8.61545627499994,15.2,-6.84127579100001));
#175137=CARTESIAN_POINT('Ctrl Pts',(8.61545627499994,11.6,-6.84127579100001));
#175138=CARTESIAN_POINT('Ctrl Pts',(8.61836922799995,15.2,-6.84224535300002));
#175139=CARTESIAN_POINT('Ctrl Pts',(8.61836922799995,11.6,-6.84224535300002));
#175140=CARTESIAN_POINT('Ctrl Pts',(8.62128799699994,15.2,-6.84321421300002));
#175141=CARTESIAN_POINT('Ctrl Pts',(8.62128799699994,11.6,-6.84321421300002));
#175142=CARTESIAN_POINT('Ctrl Pts',(8.62421257699994,15.2,-6.84418236000001));
#175143=CARTESIAN_POINT('Ctrl Pts',(8.62421257699994,11.6,-6.84418236000001));
#175144=CARTESIAN_POINT('Ctrl Pts',(8.62714295899995,15.2,-6.84514978400002));
#175145=CARTESIAN_POINT('Ctrl Pts',(8.62714295899995,11.6,-6.84514978400002));
#175146=CARTESIAN_POINT('Ctrl Pts',(8.63007913999994,15.2,-6.84611647700001));
#175147=CARTESIAN_POINT('Ctrl Pts',(8.63007913999994,11.6,-6.84611647700001));
#175148=CARTESIAN_POINT('Ctrl Pts',(8.63302110999994,15.2,-6.84708242700002));
#175149=CARTESIAN_POINT('Ctrl Pts',(8.63302110999994,11.6,-6.84708242700002));
#175150=CARTESIAN_POINT('Ctrl Pts',(8.63596886299994,15.2,-6.84804762500002));
#175151=CARTESIAN_POINT('Ctrl Pts',(8.63596886299994,11.6,-6.84804762500002));
#175152=CARTESIAN_POINT('Ctrl Pts',(8.63892239499994,15.2,-6.84901206200001));
#175153=CARTESIAN_POINT('Ctrl Pts',(8.63892239499994,11.6,-6.84901206200001));
#175154=CARTESIAN_POINT('Ctrl Pts',(8.64188169699995,15.2,-6.84997572700001));
#175155=CARTESIAN_POINT('Ctrl Pts',(8.64188169699995,11.6,-6.84997572700001));
#175156=CARTESIAN_POINT('Ctrl Pts',(8.64484676499995,15.2,-6.85093861100002));
#175157=CARTESIAN_POINT('Ctrl Pts',(8.64484676499995,11.6,-6.85093861100002));
#175158=CARTESIAN_POINT('Ctrl Pts',(8.64781759099994,15.2,-6.85190070400001));
#175159=CARTESIAN_POINT('Ctrl Pts',(8.64781759099994,11.6,-6.85190070400001));
#175160=CARTESIAN_POINT('Ctrl Pts',(8.65079416799994,15.2,-6.85286199700001));
#175161=CARTESIAN_POINT('Ctrl Pts',(8.65079416799994,11.6,-6.85286199700001));
#175162=CARTESIAN_POINT('Ctrl Pts',(8.65377649099995,15.2,-6.85382247900002));
#175163=CARTESIAN_POINT('Ctrl Pts',(8.65377649099995,11.6,-6.85382247900002));
#175164=CARTESIAN_POINT('Ctrl Pts',(8.65676455199995,15.2,-6.85478214300002));
#175165=CARTESIAN_POINT('Ctrl Pts',(8.65676455199995,11.6,-6.85478214300002));
#175166=CARTESIAN_POINT('Ctrl Pts',(8.65975834599995,15.2,-6.85574097600002));
#175167=CARTESIAN_POINT('Ctrl Pts',(8.65975834599995,11.6,-6.85574097600002));
#175168=CARTESIAN_POINT('Ctrl Pts',(8.66275786699994,15.2,-6.85669897000002));
#175169=CARTESIAN_POINT('Ctrl Pts',(8.66275786699994,11.6,-6.85669897000002));
#175170=CARTESIAN_POINT('Ctrl Pts',(8.66576310799994,15.2,-6.85765611600001));
#175171=CARTESIAN_POINT('Ctrl Pts',(8.66576310799994,11.6,-6.85765611600001));
#175172=CARTESIAN_POINT('Ctrl Pts',(8.66877406099994,15.2,-6.85861240500002));
#175173=CARTESIAN_POINT('Ctrl Pts',(8.66877406099994,11.6,-6.85861240500002));
#175174=CARTESIAN_POINT('Ctrl Pts',(8.67179072199994,15.2,-6.85956782600002));
#175175=CARTESIAN_POINT('Ctrl Pts',(8.67179072199994,11.6,-6.85956782600002));
#175176=CARTESIAN_POINT('Ctrl Pts',(8.67481308299995,15.2,-6.86052237000002));
#175177=CARTESIAN_POINT('Ctrl Pts',(8.67481308299995,11.6,-6.86052237000002));
#175178=CARTESIAN_POINT('Ctrl Pts',(8.67784113899994,15.2,-6.86147602700002));
#175179=CARTESIAN_POINT('Ctrl Pts',(8.67784113899994,11.6,-6.86147602700002));
#175180=CARTESIAN_POINT('Ctrl Pts',(8.68087488199994,15.2,-6.86242879000002));
#175181=CARTESIAN_POINT('Ctrl Pts',(8.68087488199994,11.6,-6.86242879000002));
#175182=CARTESIAN_POINT('Ctrl Pts',(8.68391430599995,15.2,-6.86338064600001));
#175183=CARTESIAN_POINT('Ctrl Pts',(8.68391430599995,11.6,-6.86338064600001));
#175184=CARTESIAN_POINT('Ctrl Pts',(8.68695940699994,15.2,-6.86433158800002));
#175185=CARTESIAN_POINT('Ctrl Pts',(8.68695940699994,11.6,-6.86433158800002));
#175186=CARTESIAN_POINT('Ctrl Pts',(8.69001017599994,15.2,-6.86528160700002));
#175187=CARTESIAN_POINT('Ctrl Pts',(8.69001017599994,11.6,-6.86528160700002));
#175188=CARTESIAN_POINT('Ctrl Pts',(8.69306660699994,15.2,-6.86623069300002));
#175189=CARTESIAN_POINT('Ctrl Pts',(8.69306660699994,11.6,-6.86623069300002));
#175190=CARTESIAN_POINT('Ctrl Pts',(8.69612869499995,15.2,-6.86717883500001));
#175191=CARTESIAN_POINT('Ctrl Pts',(8.69612869499995,11.6,-6.86717883500001));
#175192=CARTESIAN_POINT('Ctrl Pts',(8.69919643199994,15.2,-6.86812602700002));
#175193=CARTESIAN_POINT('Ctrl Pts',(8.69919643199994,11.6,-6.86812602700002));
#175194=CARTESIAN_POINT('Ctrl Pts',(8.70226981399994,15.2,-6.86907225700002));
#175195=CARTESIAN_POINT('Ctrl Pts',(8.70226981399994,11.6,-6.86907225700002));
#175196=CARTESIAN_POINT('Ctrl Pts',(8.70534883099995,15.2,-6.87001751700001));
#175197=CARTESIAN_POINT('Ctrl Pts',(8.70534883099995,11.6,-6.87001751700001));
#175198=CARTESIAN_POINT('Ctrl Pts',(8.70843347999994,15.2,-6.87096179800001));
#175199=CARTESIAN_POINT('Ctrl Pts',(8.70843347999994,11.6,-6.87096179800001));
#175200=CARTESIAN_POINT('Ctrl Pts',(8.71152375499994,15.2,-6.87190509100001));
#175201=CARTESIAN_POINT('Ctrl Pts',(8.71152375499994,11.6,-6.87190509100001));
#175202=CARTESIAN_POINT('Ctrl Pts',(8.71461964599994,15.2,-6.87284738500002));
#175203=CARTESIAN_POINT('Ctrl Pts',(8.71461964599994,11.6,-6.87284738500002));
#175204=CARTESIAN_POINT('Ctrl Pts',(8.71772114999994,15.2,-6.87378867300002));
#175205=CARTESIAN_POINT('Ctrl Pts',(8.71772114999994,11.6,-6.87378867300002));
#175206=CARTESIAN_POINT('Ctrl Pts',(8.72082825999994,15.2,-6.87472894600001));
#175207=CARTESIAN_POINT('Ctrl Pts',(8.72082825999994,11.6,-6.87472894600001));
#175208=CARTESIAN_POINT('Ctrl Pts',(8.72394096899994,15.2,-6.87566819200002));
#175209=CARTESIAN_POINT('Ctrl Pts',(8.72394096899994,11.6,-6.87566819200002));
#175210=CARTESIAN_POINT('Ctrl Pts',(8.72705927099994,15.2,-6.87660640600001));
#175211=CARTESIAN_POINT('Ctrl Pts',(8.72705927099994,11.6,-6.87660640600001));
#175212=CARTESIAN_POINT('Ctrl Pts',(8.73018315999994,15.2,-6.87754357600002));
#175213=CARTESIAN_POINT('Ctrl Pts',(8.73018315999994,11.6,-6.87754357600002));
#175214=CARTESIAN_POINT('Ctrl Pts',(8.73331262999994,15.2,-6.87847969400002));
#175215=CARTESIAN_POINT('Ctrl Pts',(8.73331262999994,11.6,-6.87847969400002));
#175216=CARTESIAN_POINT('Ctrl Pts',(8.73644767399994,15.2,-6.87941475100001));
#175217=CARTESIAN_POINT('Ctrl Pts',(8.73644767399994,11.6,-6.87941475100001));
#175218=CARTESIAN_POINT('Ctrl Pts',(8.73958828699994,15.2,-6.88034873900002));
#175219=CARTESIAN_POINT('Ctrl Pts',(8.73958828699994,11.6,-6.88034873900002));
#175220=CARTESIAN_POINT('Ctrl Pts',(8.74273446099994,15.2,-6.88128164700001));
#175221=CARTESIAN_POINT('Ctrl Pts',(8.74273446099994,11.6,-6.88128164700001));
#175222=CARTESIAN_POINT('Ctrl Pts',(8.74588619099994,15.2,-6.88221346800002));
#175223=CARTESIAN_POINT('Ctrl Pts',(8.74588619099994,11.6,-6.88221346800002));
#175224=CARTESIAN_POINT('Ctrl Pts',(8.74904346899994,15.2,-6.88314419200001));
#175225=CARTESIAN_POINT('Ctrl Pts',(8.74904346899994,11.6,-6.88314419200001));
#175226=CARTESIAN_POINT('Ctrl Pts',(8.75220629199994,15.2,-6.88407381000002));
#175227=CARTESIAN_POINT('Ctrl Pts',(8.75220629199994,11.6,-6.88407381000002));
#175228=CARTESIAN_POINT('Ctrl Pts',(8.75537464999995,15.2,-6.88500231400001));
#175229=CARTESIAN_POINT('Ctrl Pts',(8.75537464999995,11.6,-6.88500231400001));
#175230=CARTESIAN_POINT('Ctrl Pts',(8.75854853999994,15.2,-6.88592969500001));
#175231=CARTESIAN_POINT('Ctrl Pts',(8.75854853999994,11.6,-6.88592969500001));
#175232=CARTESIAN_POINT('Ctrl Pts',(8.76172795499994,15.2,-6.88685594400001));
#175233=CARTESIAN_POINT('Ctrl Pts',(8.76172795499994,11.6,-6.88685594400001));
#175234=CARTESIAN_POINT('Ctrl Pts',(8.76491288799994,15.2,-6.88778105200001));
#175235=CARTESIAN_POINT('Ctrl Pts',(8.76491288799994,11.6,-6.88778105200001));
#175236=CARTESIAN_POINT('Ctrl Pts',(8.76810333299994,15.2,-6.88870501000002));
#175237=CARTESIAN_POINT('Ctrl Pts',(8.76810333299994,11.6,-6.88870501000002));
#175238=CARTESIAN_POINT('Ctrl Pts',(8.77129928299994,15.2,-6.88962781100001));
#175239=CARTESIAN_POINT('Ctrl Pts',(8.77129928299994,11.6,-6.88962781100001));
#175240=CARTESIAN_POINT('Ctrl Pts',(8.77450073399995,15.2,-6.89054944400001));
#175241=CARTESIAN_POINT('Ctrl Pts',(8.77450073399995,11.6,-6.89054944400001));
#175242=CARTESIAN_POINT('Ctrl Pts',(8.77770767799994,15.2,-6.89146990200002));
#175243=CARTESIAN_POINT('Ctrl Pts',(8.77770767799994,11.6,-6.89146990200002));
#175244=CARTESIAN_POINT('Ctrl Pts',(8.78092010799995,15.2,-6.89238917500001));
#175245=CARTESIAN_POINT('Ctrl Pts',(8.78092010799995,11.6,-6.89238917500001));
#175246=CARTESIAN_POINT('Ctrl Pts',(8.78413802099994,15.2,-6.89330725600002));
#175247=CARTESIAN_POINT('Ctrl Pts',(8.78413802099994,11.6,-6.89330725600002));
#175248=CARTESIAN_POINT('Ctrl Pts',(8.78736140799995,15.2,-6.89422413400001));
#175249=CARTESIAN_POINT('Ctrl Pts',(8.78736140799995,11.6,-6.89422413400001));
#175250=CARTESIAN_POINT('Ctrl Pts',(8.79059026399995,15.2,-6.89513980300001));
#175251=CARTESIAN_POINT('Ctrl Pts',(8.79059026399995,11.6,-6.89513980300001));
#175252=CARTESIAN_POINT('Ctrl Pts',(8.79382458299995,15.2,-6.89605425400002));
#175253=CARTESIAN_POINT('Ctrl Pts',(8.79382458299995,11.6,-6.89605425400002));
#175254=CARTESIAN_POINT('Ctrl Pts',(8.79706435899994,15.2,-6.89696747700002));
#175255=CARTESIAN_POINT('Ctrl Pts',(8.79706435899994,11.6,-6.89696747700002));
#175256=CARTESIAN_POINT('Ctrl Pts',(8.80030958499994,15.2,-6.89787946300001));
#175257=CARTESIAN_POINT('Ctrl Pts',(8.80030958499994,11.6,-6.89787946300001));
#175258=CARTESIAN_POINT('Ctrl Pts',(8.80356025499994,15.2,-6.89879020600002));
#175259=CARTESIAN_POINT('Ctrl Pts',(8.80356025499994,11.6,-6.89879020600002));
#175260=CARTESIAN_POINT('Ctrl Pts',(8.80681636199995,15.2,-6.89969969500002));
#175261=CARTESIAN_POINT('Ctrl Pts',(8.80681636199995,11.6,-6.89969969500002));
#175262=CARTESIAN_POINT('Ctrl Pts',(8.81007790199994,15.2,-6.90060792400002));
#175263=CARTESIAN_POINT('Ctrl Pts',(8.81007790199994,11.6,-6.90060792400002));
#175264=CARTESIAN_POINT('Ctrl Pts',(8.81334486699994,15.2,-6.90151488300002));
#175265=CARTESIAN_POINT('Ctrl Pts',(8.81334486699994,11.6,-6.90151488300002));
#175266=CARTESIAN_POINT('Ctrl Pts',(8.81661725299994,15.2,-6.90242056300002));
#175267=CARTESIAN_POINT('Ctrl Pts',(8.81661725299994,11.6,-6.90242056300002));
#175268=CARTESIAN_POINT('Ctrl Pts',(8.81989505199994,15.2,-6.90332495700002));
#175269=CARTESIAN_POINT('Ctrl Pts',(8.81989505199994,11.6,-6.90332495700002));
#175270=CARTESIAN_POINT('Ctrl Pts',(8.82317825799994,15.2,-6.90422805600001));
#175271=CARTESIAN_POINT('Ctrl Pts',(8.82317825799994,11.6,-6.90422805600001));
#175272=CARTESIAN_POINT('Ctrl Pts',(8.82646686599994,15.2,-6.90512985200002));
#175273=CARTESIAN_POINT('Ctrl Pts',(8.82646686599994,11.6,-6.90512985200002));
#175274=CARTESIAN_POINT('Ctrl Pts',(8.82976086799994,15.2,-6.90603033500001));
#175275=CARTESIAN_POINT('Ctrl Pts',(8.82976086799994,11.6,-6.90603033500001));
#175276=CARTESIAN_POINT('Ctrl Pts',(8.83306025999994,15.2,-6.90692950000001));
#175277=CARTESIAN_POINT('Ctrl Pts',(8.83306025999994,11.6,-6.90692950000001));
#175278=CARTESIAN_POINT('Ctrl Pts',(8.83636503499994,15.2,-6.90782733500001));
#175279=CARTESIAN_POINT('Ctrl Pts',(8.83636503499994,11.6,-6.90782733500001));
#175280=CARTESIAN_POINT('Ctrl Pts',(8.83967518699994,15.2,-6.90872383400002));
#175281=CARTESIAN_POINT('Ctrl Pts',(8.83967518699994,11.6,-6.90872383400002));
#175282=CARTESIAN_POINT('Ctrl Pts',(8.84299070999995,15.2,-6.90961898900002));
#175283=CARTESIAN_POINT('Ctrl Pts',(8.84299070999995,11.6,-6.90961898900002));
#175284=CARTESIAN_POINT('Ctrl Pts',(8.84631159699994,15.2,-6.91051279100002));
#175285=CARTESIAN_POINT('Ctrl Pts',(8.84631159699994,11.6,-6.91051279100002));
#175286=CARTESIAN_POINT('Ctrl Pts',(8.84963784299994,15.2,-6.91140523000002));
#175287=CARTESIAN_POINT('Ctrl Pts',(8.84963784299994,11.6,-6.91140523000002));
#175288=CARTESIAN_POINT('Ctrl Pts',(8.85296944199995,15.2,-6.91229630100001));
#175289=CARTESIAN_POINT('Ctrl Pts',(8.85296944199995,11.6,-6.91229630100001));
#175290=CARTESIAN_POINT('Ctrl Pts',(8.85630638699994,15.2,-6.91318599400002));
#175291=CARTESIAN_POINT('Ctrl Pts',(8.85630638699994,11.6,-6.91318599400002));
#175292=CARTESIAN_POINT('Ctrl Pts',(8.85964867399995,15.2,-6.91407430100002));
#175293=CARTESIAN_POINT('Ctrl Pts',(8.85964867399995,11.6,-6.91407430100002));
#175294=CARTESIAN_POINT('Ctrl Pts',(8.86299629299995,15.2,-6.91496121400001));
#175295=CARTESIAN_POINT('Ctrl Pts',(8.86299629299995,11.6,-6.91496121400001));
#175296=CARTESIAN_POINT('Ctrl Pts',(8.86634924199995,15.2,-6.91584672500002));
#175297=CARTESIAN_POINT('Ctrl Pts',(8.86634924199995,11.6,-6.91584672500002));
#175298=CARTESIAN_POINT('Ctrl Pts',(8.86970751299994,15.2,-6.91673082700002));
#175299=CARTESIAN_POINT('Ctrl Pts',(8.86970751299994,11.6,-6.91673082700002));
#175300=CARTESIAN_POINT('Ctrl Pts',(8.87307109999995,15.2,-6.91761350900002));
#175301=CARTESIAN_POINT('Ctrl Pts',(8.87307109999995,11.6,-6.91761350900002));
#175302=CARTESIAN_POINT('Ctrl Pts',(8.87643999799994,15.2,-6.91849476600002));
#175303=CARTESIAN_POINT('Ctrl Pts',(8.87643999799994,11.6,-6.91849476600002));
#175304=CARTESIAN_POINT('Ctrl Pts',(8.87981419899995,15.2,-6.91937458800002));
#175305=CARTESIAN_POINT('Ctrl Pts',(8.87981419899995,11.6,-6.91937458800002));
#175306=CARTESIAN_POINT('Ctrl Pts',(8.88319369999994,15.2,-6.92025296700002));
#175307=CARTESIAN_POINT('Ctrl Pts',(8.88319369999994,11.6,-6.92025296700002));
#175308=CARTESIAN_POINT('Ctrl Pts',(8.88657849099994,15.2,-6.92112989800002));
#175309=CARTESIAN_POINT('Ctrl Pts',(8.88657849099994,11.6,-6.92112989800002));
#175310=CARTESIAN_POINT('Ctrl Pts',(8.88996856999994,15.2,-6.92200536900001));
#175311=CARTESIAN_POINT('Ctrl Pts',(8.88996856999994,11.6,-6.92200536900001));
#175312=CARTESIAN_POINT('Ctrl Pts',(8.89336392799994,15.2,-6.92287937400001));
#175313=CARTESIAN_POINT('Ctrl Pts',(8.89336392799994,11.6,-6.92287937400001));
#175314=CARTESIAN_POINT('Ctrl Pts',(8.89676456199994,15.2,-6.92375190400002));
#175315=CARTESIAN_POINT('Ctrl Pts',(8.89676456199994,11.6,-6.92375190400002));
#175316=CARTESIAN_POINT('Ctrl Pts',(8.90017046199995,15.2,-6.92462295300002));
#175317=CARTESIAN_POINT('Ctrl Pts',(8.90017046199995,11.6,-6.92462295300002));
#175318=CARTESIAN_POINT('Ctrl Pts',(8.90358162499994,15.2,-6.92549251100001));
#175319=CARTESIAN_POINT('Ctrl Pts',(8.90358162499994,11.6,-6.92549251100001));
#175320=CARTESIAN_POINT('Ctrl Pts',(8.90699804399994,15.2,-6.92636057100002));
#175321=CARTESIAN_POINT('Ctrl Pts',(8.90699804399994,11.6,-6.92636057100002));
#175322=CARTESIAN_POINT('Ctrl Pts',(8.91041971299994,15.2,-6.92722712600002));
#175323=CARTESIAN_POINT('Ctrl Pts',(8.91041971299994,11.6,-6.92722712600002));
#175324=CARTESIAN_POINT('Ctrl Pts',(8.91384662699994,15.2,-6.92809216800002));
#175325=CARTESIAN_POINT('Ctrl Pts',(8.91384662699994,11.6,-6.92809216800002));
#175326=CARTESIAN_POINT('Ctrl Pts',(8.91727877799994,15.2,-6.92895568800001));
#175327=CARTESIAN_POINT('Ctrl Pts',(8.91727877799994,11.6,-6.92895568800001));
#175328=CARTESIAN_POINT('Ctrl Pts',(8.92071616199994,15.2,-6.92981767800001));
#175329=CARTESIAN_POINT('Ctrl Pts',(8.92071616199994,11.6,-6.92981767800001));
#175330=CARTESIAN_POINT('Ctrl Pts',(8.92415877199995,15.2,-6.93067813200001));
#175331=CARTESIAN_POINT('Ctrl Pts',(8.92415877199995,11.6,-6.93067813200001));
#175332=CARTESIAN_POINT('Ctrl Pts',(8.92760660199994,15.2,-6.93153704100002));
#175333=CARTESIAN_POINT('Ctrl Pts',(8.92760660199994,11.6,-6.93153704100002));
#175334=CARTESIAN_POINT('Ctrl Pts',(8.93105964599994,15.2,-6.93239439700001));
#175335=CARTESIAN_POINT('Ctrl Pts',(8.93105964599994,11.6,-6.93239439700001));
#175336=CARTESIAN_POINT('Ctrl Pts',(8.93451789999994,15.2,-6.93325019300002));
#175337=CARTESIAN_POINT('Ctrl Pts',(8.93451789999994,11.6,-6.93325019300002));
#175338=CARTESIAN_POINT('Ctrl Pts',(8.93798135499994,15.2,-6.93410442100002));
#175339=CARTESIAN_POINT('Ctrl Pts',(8.93798135499994,11.6,-6.93410442100002));
#175340=CARTESIAN_POINT('Ctrl Pts',(8.94145000699995,15.2,-6.93495707400002));
#175341=CARTESIAN_POINT('Ctrl Pts',(8.94145000699995,11.6,-6.93495707400002));
#175342=CARTESIAN_POINT('Ctrl Pts',(8.94492384899995,15.2,-6.93580814300002));
#175343=CARTESIAN_POINT('Ctrl Pts',(8.94492384899995,11.6,-6.93580814300002));
#175344=CARTESIAN_POINT('Ctrl Pts',(8.94840287499994,15.2,-6.93665762100002));
#175345=CARTESIAN_POINT('Ctrl Pts',(8.94840287499994,11.6,-6.93665762100002));
#175346=CARTESIAN_POINT('Ctrl Pts',(8.95188708099995,15.2,-6.93750550000001));
#175347=CARTESIAN_POINT('Ctrl Pts',(8.95188708099995,11.6,-6.93750550000001));
#175348=CARTESIAN_POINT('Ctrl Pts',(8.95537645899994,15.2,-6.93835177400001));
#175349=CARTESIAN_POINT('Ctrl Pts',(8.95537645899994,11.6,-6.93835177400001));
#175350=CARTESIAN_POINT('Ctrl Pts',(8.95887100399994,15.2,-6.93919643400001));
#175351=CARTESIAN_POINT('Ctrl Pts',(8.95887100399994,11.6,-6.93919643400001));
#175352=CARTESIAN_POINT('Ctrl Pts',(8.96237070999995,15.2,-6.94003947100001));
#175353=CARTESIAN_POINT('Ctrl Pts',(8.96237070999995,11.6,-6.94003947100001));
#175354=CARTESIAN_POINT('Ctrl Pts',(8.96587556999994,15.2,-6.94088088000001));
#175355=CARTESIAN_POINT('Ctrl Pts',(8.96587556999994,11.6,-6.94088088000001));
#175356=CARTESIAN_POINT('Ctrl Pts',(8.96938557999994,15.2,-6.94172065300001));
#175357=CARTESIAN_POINT('Ctrl Pts',(8.96938557999994,11.6,-6.94172065300001));
#175358=CARTESIAN_POINT('Ctrl Pts',(8.97290073199994,15.2,-6.94255878100002));
#175359=CARTESIAN_POINT('Ctrl Pts',(8.97290073199994,11.6,-6.94255878100002));
#175360=CARTESIAN_POINT('Ctrl Pts',(8.97642102299994,15.2,-6.94339525900002));
#175361=CARTESIAN_POINT('Ctrl Pts',(8.97642102299994,11.6,-6.94339525900002));
#175362=CARTESIAN_POINT('Ctrl Pts',(8.97994644299994,15.2,-6.94423007600002));
#175363=CARTESIAN_POINT('Ctrl Pts',(8.97994644299994,11.6,-6.94423007600002));
#175364=CARTESIAN_POINT('Ctrl Pts',(8.98347698999994,15.2,-6.94506322800001));
#175365=CARTESIAN_POINT('Ctrl Pts',(8.98347698999994,11.6,-6.94506322800001));
#175366=CARTESIAN_POINT('Ctrl Pts',(8.98701265699994,15.2,-6.94589470600001));
#175367=CARTESIAN_POINT('Ctrl Pts',(8.98701265699994,11.6,-6.94589470600001));
#175368=CARTESIAN_POINT('Ctrl Pts',(8.99055343599995,15.2,-6.94672450200001));
#175369=CARTESIAN_POINT('Ctrl Pts',(8.99055343599995,11.6,-6.94672450200001));
#175370=CARTESIAN_POINT('Ctrl Pts',(8.99409932299994,15.2,-6.94755260900001));
#175371=CARTESIAN_POINT('Ctrl Pts',(8.99409932299994,11.6,-6.94755260900001));
#175372=CARTESIAN_POINT('Ctrl Pts',(8.99765031299994,15.2,-6.94837902000002));
#175373=CARTESIAN_POINT('Ctrl Pts',(8.99765031299994,11.6,-6.94837902000002));
#175374=CARTESIAN_POINT('Ctrl Pts',(9.00120639799994,15.2,-6.94920372700001));
#175375=CARTESIAN_POINT('Ctrl Pts',(9.00120639799994,11.6,-6.94920372700001));
#175376=CARTESIAN_POINT('Ctrl Pts',(9.00476757299994,15.2,-6.95002672400002));
#175377=CARTESIAN_POINT('Ctrl Pts',(9.00476757299994,11.6,-6.95002672400002));
#175378=CARTESIAN_POINT('Ctrl Pts',(9.00833383199994,15.2,-6.95084800200001));
#175379=CARTESIAN_POINT('Ctrl Pts',(9.00833383199994,11.6,-6.95084800200001));
#175380=CARTESIAN_POINT('Ctrl Pts',(9.01190517099994,15.2,-6.95166755500002));
#175381=CARTESIAN_POINT('Ctrl Pts',(9.01190517099994,11.6,-6.95166755500002));
#175382=CARTESIAN_POINT('Ctrl Pts',(9.01548158099994,15.2,-6.95248537400002));
#175383=CARTESIAN_POINT('Ctrl Pts',(9.01548158099994,11.6,-6.95248537400002));
#175384=CARTESIAN_POINT('Ctrl Pts',(9.01906305899994,15.2,-6.95330145400002));
#175385=CARTESIAN_POINT('Ctrl Pts',(9.01906305899994,11.6,-6.95330145400002));
#175386=CARTESIAN_POINT('Ctrl Pts',(9.02264959699994,15.2,-6.95411578600002));
#175387=CARTESIAN_POINT('Ctrl Pts',(9.02264959699994,11.6,-6.95411578600002));
#175388=CARTESIAN_POINT('Ctrl Pts',(9.02624118899995,15.2,-6.95492836400001));
#175389=CARTESIAN_POINT('Ctrl Pts',(9.02624118899995,11.6,-6.95492836400001));
#175390=CARTESIAN_POINT('Ctrl Pts',(9.02983783099994,15.2,-6.95573917900001));
#175391=CARTESIAN_POINT('Ctrl Pts',(9.02983783099994,11.6,-6.95573917900001));
#175392=CARTESIAN_POINT('Ctrl Pts',(9.03343951599994,15.2,-6.95654822400002));
#175393=CARTESIAN_POINT('Ctrl Pts',(9.03343951599994,11.6,-6.95654822400002));
#175394=CARTESIAN_POINT('Ctrl Pts',(9.03704623799995,15.2,-6.95735549300001));
#175395=CARTESIAN_POINT('Ctrl Pts',(9.03704623799995,11.6,-6.95735549300001));
#175396=CARTESIAN_POINT('Ctrl Pts',(9.04065799199994,15.2,-6.95816097800002));
#175397=CARTESIAN_POINT('Ctrl Pts',(9.04065799199994,11.6,-6.95816097800002));
#175398=CARTESIAN_POINT('Ctrl Pts',(9.04427477099994,15.2,-6.95896467300001));
#175399=CARTESIAN_POINT('Ctrl Pts',(9.04427477099994,11.6,-6.95896467300001));
#175400=CARTESIAN_POINT('Ctrl Pts',(9.04789657099995,15.2,-6.95976657000001));
#175401=CARTESIAN_POINT('Ctrl Pts',(9.04789657099995,11.6,-6.95976657000001));
#175402=CARTESIAN_POINT('Ctrl Pts',(9.05152338599994,15.2,-6.96056666300001));
#175403=CARTESIAN_POINT('Ctrl Pts',(9.05152338599994,11.6,-6.96056666300001));
#175404=CARTESIAN_POINT('Ctrl Pts',(9.05515520799994,15.2,-6.96136494300001));
#175405=CARTESIAN_POINT('Ctrl Pts',(9.05515520799994,11.6,-6.96136494300001));
#175406=CARTESIAN_POINT('Ctrl Pts',(9.05879203399994,15.2,-6.96216140500002));
#175407=CARTESIAN_POINT('Ctrl Pts',(9.05879203399994,11.6,-6.96216140500002));
#175408=CARTESIAN_POINT('Ctrl Pts',(9.06243385699995,15.2,-6.96295603900002));
#175409=CARTESIAN_POINT('Ctrl Pts',(9.06243385699995,11.6,-6.96295603900002));
#175410=CARTESIAN_POINT('Ctrl Pts',(9.06608066899994,15.2,-6.96374884000001));
#175411=CARTESIAN_POINT('Ctrl Pts',(9.06608066899994,11.6,-6.96374884000001));
#175412=CARTESIAN_POINT('Ctrl Pts',(9.06973246699994,15.2,-6.96453980000002));
#175413=CARTESIAN_POINT('Ctrl Pts',(9.06973246699994,11.6,-6.96453980000002));
#175414=CARTESIAN_POINT('Ctrl Pts',(9.07338924199994,15.2,-6.96532891100002));
#175415=CARTESIAN_POINT('Ctrl Pts',(9.07338924199994,11.6,-6.96532891100002));
#175416=CARTESIAN_POINT('Ctrl Pts',(9.07705099099994,15.2,-6.96611616700002));
#175417=CARTESIAN_POINT('Ctrl Pts',(9.07705099099994,11.6,-6.96611616700002));
#175418=CARTESIAN_POINT('Ctrl Pts',(9.08071770699994,15.2,-6.96690156100002));
#175419=CARTESIAN_POINT('Ctrl Pts',(9.08071770699994,11.6,-6.96690156100002));
#175420=CARTESIAN_POINT('Ctrl Pts',(9.08438938599994,15.2,-6.96768508700002));
#175421=CARTESIAN_POINT('Ctrl Pts',(9.08438938599994,11.6,-6.96768508700002));
#175422=CARTESIAN_POINT('Ctrl Pts',(9.08806602099994,15.2,-6.96846673800002));
#175423=CARTESIAN_POINT('Ctrl Pts',(9.08806602099994,11.6,-6.96846673800002));
#175424=CARTESIAN_POINT('Ctrl Pts',(9.09174760799995,15.2,-6.96924650800002));
#175425=CARTESIAN_POINT('Ctrl Pts',(9.09174760799995,11.6,-6.96924650800002));
#175426=CARTESIAN_POINT('Ctrl Pts',(9.09543414099995,15.2,-6.97002439100002));
#175427=CARTESIAN_POINT('Ctrl Pts',(9.09543414099995,11.6,-6.97002439100002));
#175428=CARTESIAN_POINT('Ctrl Pts',(9.09912561399995,15.2,-6.97080037900002));
#175429=CARTESIAN_POINT('Ctrl Pts',(9.09912561399995,11.6,-6.97080037900002));
#175430=CARTESIAN_POINT('Ctrl Pts',(9.10282202199994,15.2,-6.97157446400002));
#175431=CARTESIAN_POINT('Ctrl Pts',(9.10282202199994,11.6,-6.97157446400002));
#175432=CARTESIAN_POINT('Ctrl Pts',(9.10652335599995,15.2,-6.97234663800002));
#175433=CARTESIAN_POINT('Ctrl Pts',(9.10652335599995,11.6,-6.97234663800002));
#175434=CARTESIAN_POINT('Ctrl Pts',(9.11022960799994,15.2,-6.97311689200002));
#175435=CARTESIAN_POINT('Ctrl Pts',(9.11022960799994,11.6,-6.97311689200002));
#175436=CARTESIAN_POINT('Ctrl Pts',(9.11394077299994,15.2,-6.97388521800002));
#175437=CARTESIAN_POINT('Ctrl Pts',(9.11394077299994,11.6,-6.97388521800002));
#175438=CARTESIAN_POINT('Ctrl Pts',(9.11765684399995,15.2,-6.97465160800002));
#175439=CARTESIAN_POINT('Ctrl Pts',(9.11765684399995,11.6,-6.97465160800002));
#175440=CARTESIAN_POINT('Ctrl Pts',(9.12137781599995,15.2,-6.97541605700001));
#175441=CARTESIAN_POINT('Ctrl Pts',(9.12137781599995,11.6,-6.97541605700001));
#175442=CARTESIAN_POINT('Ctrl Pts',(9.12510368599994,15.2,-6.97617855800001));
#175443=CARTESIAN_POINT('Ctrl Pts',(9.12510368599994,11.6,-6.97617855800001));
#175444=CARTESIAN_POINT('Ctrl Pts',(9.12883444799995,15.2,-6.97693911100002));
#175445=CARTESIAN_POINT('Ctrl Pts',(9.12883444799995,11.6,-6.97693911100002));
#175446=CARTESIAN_POINT('Ctrl Pts',(9.13257010499994,15.2,-6.97769771200001));
#175447=CARTESIAN_POINT('Ctrl Pts',(9.13257010499994,11.6,-6.97769771200001));
#175448=CARTESIAN_POINT('Ctrl Pts',(9.13556254299994,15.2,-6.97830303200002));
#175449=CARTESIAN_POINT('Ctrl Pts',(9.13556254299994,11.6,-6.97830303200002));
#175450=CARTESIAN_POINT('Ctrl Pts',(9.13780907299994,15.2,-6.97875614300001));
#175451=CARTESIAN_POINT('Ctrl Pts',(9.13780907299994,11.6,-6.97875614300001));
#175452=CARTESIAN_POINT('Ctrl Pts',(9.13930773799994,15.2,-6.97905782700002));
#175453=CARTESIAN_POINT('Ctrl Pts',(9.13930773799994,11.6,-6.97905782700002));
#175454=CARTESIAN_POINT('Ctrl Pts',(9.14005731399994,15.2,-6.97920857100002));
#175455=CARTESIAN_POINT('Ctrl Pts',(9.14005731399994,11.6,-6.97920857100002));
#175456=CARTESIAN_POINT('Ctrl Pts',(8.02901631899994,15.2,-6.57080831800001));
#175457=CARTESIAN_POINT('Ctrl Pts',(8.03049110016105,15.2,-6.57181686697944));
#175458=CARTESIAN_POINT('Ctrl Pts',(8.03201610877769,15.2,-6.57285322878717));
#175459=CARTESIAN_POINT('Ctrl Pts',(8.03359089353572,15.2,-6.5739163521752));
#175460=CARTESIAN_POINT('Ctrl Pts',(8.03517327270188,15.2,-6.57498460248157));
#175461=CARTESIAN_POINT('Ctrl Pts',(8.03680591622578,15.2,-6.5760798659982));
#175462=CARTESIAN_POINT('Ctrl Pts',(8.0384883906544,15.2,-6.57720107836683));
#175463=CARTESIAN_POINT('Ctrl Pts',(8.04017086493022,15.2,-6.5783222906336));
#175464=CARTESIAN_POINT('Ctrl Pts',(8.04190317335625,15.2,-6.57946945420923));
#175465=CARTESIAN_POINT('Ctrl Pts',(8.04368489154152,15.2,-6.58064153749996));
#175466=CARTESIAN_POINT('Ctrl Pts',(8.04546660972677,15.2,-6.5818136207907));
#175467=CARTESIAN_POINT('Ctrl Pts',(8.04729774128699,15.1999999999999,-6.58301062499168));
#175468=CARTESIAN_POINT('Ctrl Pts',(8.04917787055977,15.2,-6.58423155042359));
#175469=CARTESIAN_POINT('Ctrl Pts',(8.05105800000331,15.2,-6.5854524759664));
#175470=CARTESIAN_POINT('Ctrl Pts',(8.05298713001268,15.2,-6.58669732252585));
#175471=CARTESIAN_POINT('Ctrl Pts',(8.05496485620711,15.2,-6.58796512017984));
#175472=CARTESIAN_POINT('Ctrl Pts',(8.05694258222188,15.2,-6.58923291771867));
#175473=CARTESIAN_POINT('Ctrl Pts',(8.05896890494999,15.2,-6.59052366460892));
#175474=CARTESIAN_POINT('Ctrl Pts',(8.0610434290508,15.2,-6.59183642123391));
#175475=CARTESIAN_POINT('Ctrl Pts',(8.06311795315161,15.2,-6.59314917785888));
#175476=CARTESIAN_POINT('Ctrl Pts',(8.06524067911272,15.2,-6.59448394143469));
#175477=CARTESIAN_POINT('Ctrl Pts',(8.0674112193651,15.2,-6.59583979613451));
#175478=CARTESIAN_POINT('Ctrl Pts',(8.06958175981464,15.2,-6.59719565095748));
#175479=CARTESIAN_POINT('Ctrl Pts',(8.07180011545347,15.2,-6.59857259622476));
#175480=CARTESIAN_POINT('Ctrl Pts',(8.07406590574684,15.2,-6.5999697421356));
#175481=CARTESIAN_POINT('Ctrl Pts',(8.0763316958344,15.2,-6.60136688791955));
#175482=CARTESIAN_POINT('Ctrl Pts',(8.07864492166241,15.2,-6.60278423372139));
#175483=CARTESIAN_POINT('Ctrl Pts',(8.08100520891203,15.2,-6.6042209115867));
#175484=CARTESIAN_POINT('Ctrl Pts',(8.08336549616167,15.2,-6.605657589452));
#175485=CARTESIAN_POINT('Ctrl Pts',(8.08577284714085,15.2,-6.60711359752408));
#175486=CARTESIAN_POINT('Ctrl Pts',(8.08822689338298,15.2,-6.60858809463637));
#175487=CARTESIAN_POINT('Ctrl Pts',(8.09068093962512,15.2,-6.61006259174866));
#175488=CARTESIAN_POINT('Ctrl Pts',(8.09318168337629,15.2,-6.61155557734142));
#175489=CARTESIAN_POINT('Ctrl Pts',(8.09572876369724,15.2,-6.61306622661866));
#175490=CARTESIAN_POINT('Ctrl Pts',(8.09827584424958,15.2,-6.61457687603312));
#175491=CARTESIAN_POINT('Ctrl Pts',(8.10086926328141,15.2,-6.61610519224932));
#175492=CARTESIAN_POINT('Ctrl Pts',(8.10350866492724,15.2,-6.61765036983427));
#175493=CARTESIAN_POINT('Ctrl Pts',(8.10614806633333,15.2,-6.61919554727886));
#175494=CARTESIAN_POINT('Ctrl Pts',(8.10883345331891,15.2,-6.62075759161615));
#175495=CARTESIAN_POINT('Ctrl Pts',(8.11156447473196,15.2,-6.62233571523261));
#175496=CARTESIAN_POINT('Ctrl Pts',(8.11429549614501,15.2,-6.62391383884906));
#175497=CARTESIAN_POINT('Ctrl Pts',(8.11707215585626,15.2,-6.62550804652576));
#175498=CARTESIAN_POINT('Ctrl Pts',(8.11989411016728,15.2,-6.62711757488289));
#175499=CARTESIAN_POINT('Ctrl Pts',(8.12271606473465,15.2,-6.62872710338622));
#175500=CARTESIAN_POINT('Ctrl Pts',(8.12558331191476,15.2,-6.6303519509994));
#175501=CARTESIAN_POINT('Ctrl Pts',(8.12849551940877,15.2,-6.6319913775894));
#175502=CARTESIAN_POINT('Ctrl Pts',(8.13140772663827,15.2,-6.63363080403048));
#175503=CARTESIAN_POINT('Ctrl Pts',(8.13436489026072,15.2,-6.63528480749396));
#175504=CARTESIAN_POINT('Ctrl Pts',(8.13736668249851,15.2,-6.63695266402424));
#175505=CARTESIAN_POINT('Ctrl Pts',(8.14036847473628,15.2,-6.63862052055451));
#175506=CARTESIAN_POINT('Ctrl Pts',(8.143414891645,15.2,-6.64030222865274));
#175507=CARTESIAN_POINT('Ctrl Pts',(8.14650561086299,15.2,-6.64199708134026));
#175508=CARTESIAN_POINT('Ctrl Pts',(8.14959633036172,15.2,-6.64369193418172));
#175509=CARTESIAN_POINT('Ctrl Pts',(8.15273134873956,15.2,-6.64539993184436));
#175510=CARTESIAN_POINT('Ctrl Pts',(8.15591034657417,15.2,-6.64712038194146));
#175511=CARTESIAN_POINT('Ctrl Pts',(8.15908934412002,15.2,-6.64884083188229));
#175512=CARTESIAN_POINT('Ctrl Pts',(8.16231231913521,15.2,-6.65057373512171));
#175513=CARTESIAN_POINT('Ctrl Pts',(8.1655789546832,15.2,-6.65231841597499));
#175514=CARTESIAN_POINT('Ctrl Pts',(8.16884559023117,15.2,-6.65406309682827));
#175515=CARTESIAN_POINT('Ctrl Pts',(8.17215588798237,15.2,-6.6558195550556));
#175516=CARTESIAN_POINT('Ctrl Pts',(8.17550953269222,15.2,-6.65758713107903));
#175517=CARTESIAN_POINT('Ctrl Pts',(8.1788631777067,15.2,-6.65935470726302));
#175518=CARTESIAN_POINT('Ctrl Pts',(8.18226017085943,15.2,-6.66113339979679));
#175519=CARTESIAN_POINT('Ctrl Pts',(8.18570020263318,15.2,-6.66292256589502));
#175520=CARTESIAN_POINT('Ctrl Pts',(8.18914023409444,15.2,-6.66471173183071));
#175521=CARTESIAN_POINT('Ctrl Pts',(8.19262330411346,15.2,-6.66651136898332));
#175522=CARTESIAN_POINT('Ctrl Pts',(8.19614910850148,15.2,-6.66832084800916));
#175523=CARTESIAN_POINT('Ctrl Pts',(8.1996749128895,15.2,-6.67013032703499));
#175524=CARTESIAN_POINT('Ctrl Pts',(8.20324344950296,15.2,-6.67194964697554));
#175525=CARTESIAN_POINT('Ctrl Pts',(8.20685441903658,15.2,-6.67377819115871));
#175526=CARTESIAN_POINT('Ctrl Pts',(8.20986356042394,15.2,-6.67530197803339));
#175527=CARTESIAN_POINT('Ctrl Pts',(8.21290216949537,15.2,-6.67683217109432));
#175528=CARTESIAN_POINT('Ctrl Pts',(8.21597007254941,15.2,-6.67836841894123));
#175529=CARTESIAN_POINT('Ctrl Pts',(8.21903797560345,15.2,-6.67990466678815));
#175530=CARTESIAN_POINT('Ctrl Pts',(8.22213517386183,15.2,-6.68144697092547));
#175531=CARTESIAN_POINT('Ctrl Pts',(8.22526149526484,15.2,-6.68299498697416));
#175532=CARTESIAN_POINT('Ctrl Pts',(8.22838781666784,15.2,-6.68454300302283));
#175533=CARTESIAN_POINT('Ctrl Pts',(8.23154326107765,15.2,-6.68609673040001));
#175534=CARTESIAN_POINT('Ctrl Pts',(8.2347276622582,15.2,-6.687655832275));
#175535=CARTESIAN_POINT('Ctrl Pts',(8.23791206343875,15.2,-6.68921493415));
#175536=CARTESIAN_POINT('Ctrl Pts',(8.24112541779795,15.2,-6.6907794097326));
#175537=CARTESIAN_POINT('Ctrl Pts',(8.24436756003498,15.2,-6.69234892751752));
#175538=CARTESIAN_POINT('Ctrl Pts',(8.247609702272,15.2,-6.69391844530244));
#175539=CARTESIAN_POINT('Ctrl Pts',(8.25088063221433,15.2,-6.69549300500863));
#175540=CARTESIAN_POINT('Ctrl Pts',(8.25418018346584,15.2,-6.69707228111999));
#175541=CARTESIAN_POINT('Ctrl Pts',(8.25747973471735,15.2,-6.69865155723135));
#175542=CARTESIAN_POINT('Ctrl Pts',(8.2608079052903,15.2,-6.70023554877035));
#175543=CARTESIAN_POINT('Ctrl Pts',(8.26416453494457,15.2,-6.70182393585391));
#175544=CARTESIAN_POINT('Ctrl Pts',(8.26819249038333,15.2,-6.70373000028493));
#175545=CARTESIAN_POINT('Ctrl Pts',(8.27226142321209,15.2,-6.7056423941518));
#175546=CARTESIAN_POINT('Ctrl Pts',(8.27637105274801,15.2,-6.70756057267414));
#175547=CARTESIAN_POINT('Ctrl Pts',(8.27979574415238,15.2,-6.70915905483416));
#175548=CARTESIAN_POINT('Ctrl Pts',(8.28324869616098,15.2,-6.71076155398333));
#175549=CARTESIAN_POINT('Ctrl Pts',(8.28672974921653,15.2,-6.71236776273334));
#175550=CARTESIAN_POINT('Ctrl Pts',(8.29021080227209,15.2,-6.71397397148333));
#175551=CARTESIAN_POINT('Ctrl Pts',(8.29371995550789,15.2,-6.71558388856021));
#175552=CARTESIAN_POINT('Ctrl Pts',(8.29725704871847,15.2,-6.71719721148422));
#175553=CARTESIAN_POINT('Ctrl Pts',(8.30079414192906,15.2,-6.71881053440822));
#175554=CARTESIAN_POINT('Ctrl Pts',(8.3043591753669,15.2,-6.72042726099468));
#175555=CARTESIAN_POINT('Ctrl Pts',(8.30795199078501,15.2,-6.72204709481429));
#175556=CARTESIAN_POINT('Ctrl Pts',(8.31154480620312,15.2,-6.7236669286339));
#175557=CARTESIAN_POINT('Ctrl Pts',(8.31516540310386,15.2,-6.72528986917287));
#175558=CARTESIAN_POINT('Ctrl Pts',(8.3188136237303,15.2,-6.72691562063135));
#175559=CARTESIAN_POINT('Ctrl Pts',(8.32246184435675,15.2,-6.72854137208984));
#175560=CARTESIAN_POINT('Ctrl Pts',(8.32613769026303,15.2,-6.73016993652323));
#175561=CARTESIAN_POINT('Ctrl Pts',(8.32984100345891,15.2,-6.73180102381503));
#175562=CARTESIAN_POINT('Ctrl Pts',(8.33354431665477,15.2,-6.73343211110683));
#175563=CARTESIAN_POINT('Ctrl Pts',(8.33727509776325,15.2,-6.73506572191915));
#175564=CARTESIAN_POINT('Ctrl Pts',(8.34103319274456,15.2,-6.73670157088991));
#175565=CARTESIAN_POINT('Ctrl Pts',(8.34479128772588,15.2,-6.73833741986068));
#175566=CARTESIAN_POINT('Ctrl Pts',(8.34857669571301,15.2,-6.73997550780325));
#175567=CARTESIAN_POINT('Ctrl Pts',(8.3523892630069,15.2,-6.74161555349786));
#175568=CARTESIAN_POINT('Ctrl Pts',(8.35543931659267,15.2,-6.74292758994629));
#175569=CARTESIAN_POINT('Ctrl Pts',(8.35850675181227,15.2,-6.74424087942508));
#175570=CARTESIAN_POINT('Ctrl Pts',(8.36159149144786,15.2,-6.7455552811509));
#175571=CARTESIAN_POINT('Ctrl Pts',(8.36467623150374,15.2,-6.74686968305581));
#175572=CARTESIAN_POINT('Ctrl Pts',(8.36777827623639,15.2,-6.74818519696456));
#175573=CARTESIAN_POINT('Ctrl Pts',(8.37089754645259,15.2,-6.74950168365771));
#175574=CARTESIAN_POINT('Ctrl Pts',(8.3740168162438,15.2,-6.7508181701715));
#175575=CARTESIAN_POINT('Ctrl Pts',(8.37715331159283,15.2,-6.75213562847229));
#175576=CARTESIAN_POINT('Ctrl Pts',(8.38030695650056,15.2,-6.75345392214225));
#175577=CARTESIAN_POINT('Ctrl Pts',(8.38346060183799,15.2,-6.75477221599183));
#175578=CARTESIAN_POINT('Ctrl Pts',(8.3866313966969,15.2,-6.7560913433665));
#175579=CARTESIAN_POINT('Ctrl Pts',(8.38981926276065,15.2,-6.75741116938291));
#175580=CARTESIAN_POINT('Ctrl Pts',(8.39300712839004,15.2,-6.7587309952195));
#175581=CARTESIAN_POINT('Ctrl Pts',(8.3962120660197,15.2,-6.7600515191087));
#175582=CARTESIAN_POINT('Ctrl Pts',(8.39943399924912,15.2,-6.76137260756665));
#175583=CARTESIAN_POINT('Ctrl Pts',(8.40265593291753,15.2,-6.7626936962046));
#175584=CARTESIAN_POINT('Ctrl Pts',(8.40589486317934,15.2,-6.7640153482388));
#175585=CARTESIAN_POINT('Ctrl Pts',(8.40915071252453,15.2,-6.76533743036643));
#175586=CARTESIAN_POINT('Ctrl Pts',(8.41240656142612,15.2,-6.76665951231393));
#175587=CARTESIAN_POINT('Ctrl Pts',(8.415679330241,15.2,-6.76798202511968));
#175588=CARTESIAN_POINT('Ctrl Pts',(8.41896894247038,15.2,-6.76930483823374));
#175589=CARTESIAN_POINT('Ctrl Pts',(8.42225855514796,15.2,-6.77062765152803));
#175590=CARTESIAN_POINT('Ctrl Pts',(8.42556501196421,15.2,-6.77195076309222));
#175591=CARTESIAN_POINT('Ctrl Pts',(8.42888823799381,15.2,-6.77327404522592));
#175592=CARTESIAN_POINT('Ctrl Pts',(8.43221146357063,15.2,-6.77459732717931));
#175593=CARTESIAN_POINT('Ctrl Pts',(8.43555145772161,15.2,-6.77592077960571));
#175594=CARTESIAN_POINT('Ctrl Pts',(8.43890814600107,15.2,-6.77724427277529));
#175595=CARTESIAN_POINT('Ctrl Pts',(8.44226483473787,15.2,-6.7785677661252));
#175596=CARTESIAN_POINT('Ctrl Pts',(8.44563821709011,15.2,-6.77989130153066));
#175597=CARTESIAN_POINT('Ctrl Pts',(8.44902821977487,15.2,-6.78121475099168));
#175598=CARTESIAN_POINT('Ctrl Pts',(8.45241822245964,15.2,-6.7825382004527));
#175599=CARTESIAN_POINT('Ctrl Pts',(8.45582484410188,15.2,-6.78386156511927));
#175600=CARTESIAN_POINT('Ctrl Pts',(8.45924801156791,15.2,-6.78518471869135));
#175601=CARTESIAN_POINT('Ctrl Pts',(8.46267117856753,15.2,-6.78650787208315));
#175602=CARTESIAN_POINT('Ctrl Pts',(8.46611089167832,15.2,-6.78783081717345));
#175603=CARTESIAN_POINT('Ctrl Pts',(8.46956707602253,15.2,-6.78915342651578));
#175604=CARTESIAN_POINT('Ctrl Pts',(8.47302326083764,15.2,-6.79047603603832));
#175605=CARTESIAN_POINT('Ctrl Pts',(8.47649591951185,15.2,-6.79179831183302));
#175606=CARTESIAN_POINT('Ctrl Pts',(8.47998497503701,15.2,-6.7931201306828));
#175607=CARTESIAN_POINT('Ctrl Pts',(8.48434629420578,15.2,-6.79477240415497));
#175608=CARTESIAN_POINT('Ctrl Pts',(8.48873323704162,15.2,-6.79642396448822));
#175609=CARTESIAN_POINT('Ctrl Pts',(8.49314565954369,15.2,-6.79807457622425));
#175610=CARTESIAN_POINT('Ctrl Pts',(8.49667559725679,15.2,-6.79939506550513));
#175611=CARTESIAN_POINT('Ctrl Pts',(8.50022184317258,15.2,-6.8007149468732));
#175612=CARTESIAN_POINT('Ctrl Pts',(8.50378432356412,15.2,-6.80203410221579));
#175613=CARTESIAN_POINT('Ctrl Pts',(8.50734680444106,15.2,-6.80335325773811));
#175614=CARTESIAN_POINT('Ctrl Pts',(8.51092552108452,15.2,-6.80467168701595));
#175615=CARTESIAN_POINT('Ctrl Pts',(8.51452039983765,15.2,-6.80598927119878));
#175616=CARTESIAN_POINT('Ctrl Pts',(8.51901399803416,15.2,-6.80763625133755));
#175617=CARTESIAN_POINT('Ctrl Pts',(8.5235328507533,15.2,-6.80928191254298));
#175618=CARTESIAN_POINT('Ctrl Pts',(8.52807681735257,15.2,-6.81092602768173));
#175619=CARTESIAN_POINT('Ctrl Pts',(8.53171199033481,15.2,-6.81224131968522));
#175620=CARTESIAN_POINT('Ctrl Pts',(8.53536323696391,15.2,-6.81355562115606));
#175621=CARTESIAN_POINT('Ctrl Pts',(8.53903048468072,15.2,-6.81486881849912));
#175622=CARTESIAN_POINT('Ctrl Pts',(8.54361454470147,15.2,-6.81651031531213));
#175623=CARTESIAN_POINT('Ctrl Pts',(8.54822360822211,15.2,-6.81815008554447));
#175624=CARTESIAN_POINT('Ctrl Pts',(8.55285753474988,15.2,-6.81978790901669));
#175625=CARTESIAN_POINT('Ctrl Pts',(8.55656467617414,15.2,-6.82109816786587));
#175626=CARTESIAN_POINT('Ctrl Pts',(8.56028773008913,15.2,-6.82240717878159));
#175627=CARTESIAN_POINT('Ctrl Pts',(8.56402662629453,15.2,-6.82371483296382));
#175628=CARTESIAN_POINT('Ctrl Pts',(8.56776552199051,15.2,-6.8250224869679));
#175629=CARTESIAN_POINT('Ctrl Pts',(8.5715202608996,15.2,-6.82632878219154));
#175630=CARTESIAN_POINT('Ctrl Pts',(8.57529077049732,15.2,-6.82763360825747));
#175631=CARTESIAN_POINT('Ctrl Pts',(8.57906128060877,15.2,-6.82893843450118));
#175632=CARTESIAN_POINT('Ctrl Pts',(8.58284756169325,15.2,-6.8302417913643));
#175633=CARTESIAN_POINT('Ctrl Pts',(8.58664954517985,15.2,-6.83154357021286));
#175634=CARTESIAN_POINT('Ctrl Pts',(8.59045152814842,15.2,-6.83284534888406));
#175635=CARTESIAN_POINT('Ctrl Pts',(8.59426921194549,15.2,-6.83414554742212));
#175636=CARTESIAN_POINT('Ctrl Pts',(8.59810252818666,15.2,-6.83544406009385));
#175637=CARTESIAN_POINT('Ctrl Pts',(8.60193584495011,15.2,-6.83674257294251));
#175638=CARTESIAN_POINT('Ctrl Pts',(8.60578479237932,15.2,-6.83803939856874));
#175639=CARTESIAN_POINT('Ctrl Pts',(8.60964930309095,15.2,-6.8393344296392));
#175640=CARTESIAN_POINT('Ctrl Pts',(8.61351381327604,15.2,-6.84062946053322));
#175641=CARTESIAN_POINT('Ctrl Pts',(8.61739388405433,15.2,-6.84192269777852));
#175642=CARTESIAN_POINT('Ctrl Pts',(8.62128944915137,15.2,-6.84321403457097));
#175643=CARTESIAN_POINT('Ctrl Pts',(8.62518501477918,15.2,-6.84450537153935));
#175644=CARTESIAN_POINT('Ctrl Pts',(8.62909607442824,15.2,-6.84579480803522));
#175645=CARTESIAN_POINT('Ctrl Pts',(8.63302255608769,15.2,-6.84708223910525));
#175646=CARTESIAN_POINT('Ctrl Pts',(8.63694903721214,15.2,-6.84836966999987));
#175647=CARTESIAN_POINT('Ctrl Pts',(8.64089094235293,15.2,-6.84965509620877));
#175648=CARTESIAN_POINT('Ctrl Pts',(8.64484820386122,15.2,-6.85093841304854));
#175649=CARTESIAN_POINT('Ctrl Pts',(8.64880546590867,15.2,-6.85222173006314));
#175650=CARTESIAN_POINT('Ctrl Pts',(8.65277808228654,15.2,-6.85350293838371));
#175651=CARTESIAN_POINT('Ctrl Pts',(8.65676598524427,15.2,-6.85478193529256));
#175652=CARTESIAN_POINT('Ctrl Pts',(8.66075388765865,15.2,-6.85606093202714));
#175653=CARTESIAN_POINT('Ctrl Pts',(8.66475707897294,15.2,-6.85733771569004));
#175654=CARTESIAN_POINT('Ctrl Pts',(8.66877548730955,15.2,-6.85861218780832));
#175655=CARTESIAN_POINT('Ctrl Pts',(8.67279389619365,15.2,-6.85988666010024));
#175656=CARTESIAN_POINT('Ctrl Pts',(8.67682752460145,15.2,-6.86115881834193));
#175657=CARTESIAN_POINT('Ctrl Pts',(8.68087630226655,15.2,-6.86242856330003));
#175658=CARTESIAN_POINT('Ctrl Pts',(8.68492507993166,15.2,-6.86369830825812));
#175659=CARTESIAN_POINT('Ctrl Pts',(8.68898900972352,15.2,-6.8649656394576));
#175660=CARTESIAN_POINT('Ctrl Pts',(8.69306802189181,15.2,-6.86623045724849));
#175661=CARTESIAN_POINT('Ctrl Pts',(8.69714703350433,15.2,-6.86749527486705));
#175662=CARTESIAN_POINT('Ctrl Pts',(8.70124112912272,15.2,-6.86875757934641));
#175663=CARTESIAN_POINT('Ctrl Pts',(8.70535023897209,15.2,-6.87001727224917));
#175664=CARTESIAN_POINT('Ctrl Pts',(8.70945934938132,15.2,-6.87127696532355));
#175665=CARTESIAN_POINT('Ctrl Pts',(8.71358347672731,15.2,-6.8725340465287));
#175666=CARTESIAN_POINT('Ctrl Pts',(8.71772255217663,15.2,-6.87378841943011));
#175667=CARTESIAN_POINT('Ctrl Pts',(8.721861627062,15.2,-6.87504279216062));
#175668=CARTESIAN_POINT('Ctrl Pts',(8.72601564996489,15.2,-6.87629445526927));
#175669=CARTESIAN_POINT('Ctrl Pts',(8.73018455490089,15.2,-6.87754331288957));
#175670=CARTESIAN_POINT('Ctrl Pts',(8.73435346040489,15.2,-6.87879217068005));
#175671=CARTESIAN_POINT('Ctrl Pts',(8.7385372481999,15.2,-6.88003822355357));
#175672=CARTESIAN_POINT('Ctrl Pts',(8.74273585058421,15.2,-6.8812813754054));
#175673=CARTESIAN_POINT('Ctrl Pts',(8.74693445239646,15.2,-6.88252452708784));
#175674=CARTESIAN_POINT('Ctrl Pts',(8.75114786818987,15.2,-6.88376477758314));
#175675=CARTESIAN_POINT('Ctrl Pts',(8.75537603262104,15.2,-6.88500203314885));
#175676=CARTESIAN_POINT('Ctrl Pts',(8.7596041976283,15.2,-6.88623928888314));
#175677=CARTESIAN_POINT('Ctrl Pts',(8.76384711333453,15.2,-6.88747354908375));
#175678=CARTESIAN_POINT('Ctrl Pts',(8.76810470962308,15.2,-6.88870472081731));
#175679=CARTESIAN_POINT('Ctrl Pts',(8.77236230533153,15.2,-6.88993589238313));
#175680=CARTESIAN_POINT('Ctrl Pts',(8.77663458354881,15.2,-6.89116397516093));
#175681=CARTESIAN_POINT('Ctrl Pts',(8.78092147807791,15.2,-6.89238887678894));
#175682=CARTESIAN_POINT('Ctrl Pts',(8.78413664912077,15.2,-6.89330755305166));
#175683=CARTESIAN_POINT('Ctrl Pts',(8.78736004216393,15.2,-6.89422443911686));
#175684=CARTESIAN_POINT('Ctrl Pts',(8.79059162904541,15.2,-6.89513949829221));
#175685=CARTESIAN_POINT('Ctrl Pts',(8.79382321651396,15.2,-6.89605455763379));
#175686=CARTESIAN_POINT('Ctrl Pts',(8.79706299876813,15.2,-6.89696778848317));
#175687=CARTESIAN_POINT('Ctrl Pts',(8.80031094669962,15.2,-6.89787915240704));
#175688=CARTESIAN_POINT('Ctrl Pts',(8.80355889404106,15.2,-6.89879051616534));
#175689=CARTESIAN_POINT('Ctrl Pts',(8.80681500675705,15.2,-6.89970001343207));
#175690=CARTESIAN_POINT('Ctrl Pts',(8.81007925863916,15.2,-6.90060760660726));
#175691=CARTESIAN_POINT('Ctrl Pts',(8.81334351052127,15.2,-6.90151519978245));
#175692=CARTESIAN_POINT('Ctrl Pts',(8.81661590182379,15.2,-6.90242088749626));
#175693=CARTESIAN_POINT('Ctrl Pts',(8.8198964037612,15.2,-6.90332463325918));
#175694=CARTESIAN_POINT('Ctrl Pts',(8.82427040614576,15.2,-6.90452962755502));
#175695=CARTESIAN_POINT('Ctrl Pts',(8.82865882812198,15.2,-6.90573116845173));
#175696=CARTESIAN_POINT('Ctrl Pts',(8.83306160503838,15.2,-6.90692916735415));
#175697=CARTESIAN_POINT('Ctrl Pts',(8.83636368847552,15.2,-6.907827666735));
#175698=CARTESIAN_POINT('Ctrl Pts',(8.83967384675659,15.2,-6.90872417309864));
#175699=CARTESIAN_POINT('Ctrl Pts',(8.84299205173993,15.2,-6.90961865093669));
#175700=CARTESIAN_POINT('Ctrl Pts',(8.84631025612047,15.2,-6.91051312861225));
#175701=CARTESIAN_POINT('Ctrl Pts',(8.84963650746724,15.2,-6.91140557539624));
#175702=CARTESIAN_POINT('Ctrl Pts',(8.85297077888846,15.2,-6.91229595661371));
#175703=CARTESIAN_POINT('Ctrl Pts',(8.85630505030968,15.2,-6.91318633783118));
#175704=CARTESIAN_POINT('Ctrl Pts',(8.85964734197608,15.2,-6.91407465216235));
#175705=CARTESIAN_POINT('Ctrl Pts',(8.86299762545293,15.2,-6.91496086350917));
#175706=CARTESIAN_POINT('Ctrl Pts',(8.8663479089298,15.2,-6.91584707485598));
#175707=CARTESIAN_POINT('Ctrl Pts',(8.86970618587056,15.2,-6.91673118386059));
#175708=CARTESIAN_POINT('Ctrl Pts',(8.87307242772183,15.2,-6.91761315270756));
#175709=CARTESIAN_POINT('Ctrl Pts',(8.87643866957311,15.2,-6.91849512155453));
#175710=CARTESIAN_POINT('Ctrl Pts',(8.8798128768216,15.2,-6.91937495058603));
#175711=CARTESIAN_POINT('Ctrl Pts',(8.88319502219804,15.2,-6.920252604846));
#175712=CARTESIAN_POINT('Ctrl Pts',(8.88657716757447,15.2,-6.92113025910596));
#175713=CARTESIAN_POINT('Ctrl Pts',(8.889967250867,15.2,-6.92200573824108));
#175714=CARTESIAN_POINT('Ctrl Pts',(8.8933652462008,15.2,-6.92287900508466));
#175715=CARTESIAN_POINT('Ctrl Pts',(8.89676324215189,15.2,-6.92375227208687));
#175716=CARTESIAN_POINT('Ctrl Pts',(8.90016914879689,15.2,-6.9246233281468));
#175717=CARTESIAN_POINT('Ctrl Pts',(8.90358293975244,15.2,-6.92549213668943));
#175718=CARTESIAN_POINT('Ctrl Pts',(8.90699673008781,15.2,-6.92636094507422));
#175719=CARTESIAN_POINT('Ctrl Pts',(8.91041840489919,15.2,-6.92722750737238));
#175720=CARTESIAN_POINT('Ctrl Pts',(8.91384793694683,15.2,-6.92809178767556));
#175721=CARTESIAN_POINT('Ctrl Pts',(8.91727746899448,15.2,-6.92895606797873));
#175722=CARTESIAN_POINT('Ctrl Pts',(8.92071485800005,15.2,-6.9298180650918));
#175723=CARTESIAN_POINT('Ctrl Pts',(8.92416007737555,15.2,-6.93067774585203));
#175724=CARTESIAN_POINT('Ctrl Pts',(8.92760529675105,15.2,-6.93153742661226));
#175725=CARTESIAN_POINT('Ctrl Pts',(8.93105834645897,15.2,-6.93239478966444));
#175726=CARTESIAN_POINT('Ctrl Pts',(8.93451920029155,15.2,-6.93324980100837));
#175727=CARTESIAN_POINT('Ctrl Pts',(8.93798005412414,15.2,-6.9341048123523));
#175728=CARTESIAN_POINT('Ctrl Pts',(8.94144871118141,15.2,-6.93495747230466));
#175729=CARTESIAN_POINT('Ctrl Pts',(8.94492514463776,15.2,-6.93580774514898));
#175730=CARTESIAN_POINT('Ctrl Pts',(8.94840157809411,15.2,-6.9366580179933));
#175731=CARTESIAN_POINT('Ctrl Pts',(8.95188578906658,15.2,-6.9375059040961));
#175732=CARTESIAN_POINT('Ctrl Pts',(8.95537774998032,15.2,-6.93835137031572));
#175733=CARTESIAN_POINT('Ctrl Pts',(8.95886971152843,15.2,-6.93919683668892));
#175734=CARTESIAN_POINT('Ctrl Pts',(8.96236942322039,15.2,-6.94003988076145));
#175735=CARTESIAN_POINT('Ctrl Pts',(8.96587685823119,15.2,-6.94088047117494));
#175736=CARTESIAN_POINT('Ctrl Pts',(8.9693842926048,15.2,-6.94172106143573));
#175737=CARTESIAN_POINT('Ctrl Pts',(8.97289945094933,15.2,-6.94255919708392));
#175738=CARTESIAN_POINT('Ctrl Pts',(8.97642230599822,15.2,-6.94339484397002));
#175739=CARTESIAN_POINT('Ctrl Pts',(8.97994516104711,15.2,-6.94423049085612));
#175740=CARTESIAN_POINT('Ctrl Pts',(8.98347571304691,15.2,-6.94506364925427));
#175741=CARTESIAN_POINT('Ctrl Pts',(8.98701393541902,15.2,-6.94589428559886));
#175742=CARTESIAN_POINT('Ctrl Pts',(8.99055215779113,15.2,-6.94672492194347));
#175743=CARTESIAN_POINT('Ctrl Pts',(8.99409804994567,15.2,-6.94755303563003));
#175744=CARTESIAN_POINT('Ctrl Pts',(8.99765158677489,15.2,-6.9483785940167));
#175745=CARTESIAN_POINT('Ctrl Pts',(9.00238963631089,15.2,-6.94947933863225));
#175746=CARTESIAN_POINT('Ctrl Pts',(9.00714127398459,15.2,-6.95057554109726));
#175747=CARTESIAN_POINT('Ctrl Pts',(9.011906439579,15.2,-6.95166712171184));
#175748=CARTESIAN_POINT('Ctrl Pts',(9.01548031345019,15.2,-6.9524858070984));
#175749=CARTESIAN_POINT('Ctrl Pts',(9.01906179657791,15.2,-6.95330189324661));
#175750=CARTESIAN_POINT('Ctrl Pts',(9.02265086121103,15.2,-6.95411534763239));
#175751=CARTESIAN_POINT('Ctrl Pts',(9.02623992584414,15.2,-6.95492880201817));
#175752=CARTESIAN_POINT('Ctrl Pts',(9.02983657273984,15.2,-6.95573962368434));
#175753=CARTESIAN_POINT('Ctrl Pts',(9.03344077565121,15.2,-6.95654778007141));
#175754=CARTESIAN_POINT('Ctrl Pts',(9.03704497856259,15.2,-6.95735593645849));
#175755=CARTESIAN_POINT('Ctrl Pts',(9.04065673728139,15.2,-6.9581614281292));
#175756=CARTESIAN_POINT('Ctrl Pts',(9.04427602623322,15.2,-6.9589642235167));
#175757=CARTESIAN_POINT('Ctrl Pts',(9.04789531518505,15.2,-6.9597670189042));
#175758=CARTESIAN_POINT('Ctrl Pts',(9.05152213511992,15.2,-6.96056711802514));
#175759=CARTESIAN_POINT('Ctrl Pts',(9.05515645857055,15.2,-6.96136448837141));
#175760=CARTESIAN_POINT('Ctrl Pts',(9.05879078202118,15.2,-6.96216185871767));
#175761=CARTESIAN_POINT('Ctrl Pts',(9.06243261019506,15.2,-6.96295649975236));
#175762=CARTESIAN_POINT('Ctrl Pts',(9.06608191474392,15.2,-6.9637483795968));
#175763=CARTESIAN_POINT('Ctrl Pts',(9.07094765458435,15.2,-6.96480421948529));
#175764=CARTESIAN_POINT('Ctrl Pts',(9.07582668513524,15.2,-6.96585514807604));
#175765=CARTESIAN_POINT('Ctrl Pts',(9.08071894812496,15.2,-6.96690109407716));
#175766=CARTESIAN_POINT('Ctrl Pts',(9.08438814503396,15.2,-6.96768555350675));
#175767=CARTESIAN_POINT('Ctrl Pts',(9.08806478513374,15.2,-6.968467210345));
#175768=CARTESIAN_POINT('Ctrl Pts',(9.09174884449989,15.2,-6.96924603623337));
#175769=CARTESIAN_POINT('Ctrl Pts',(9.09666092410094,15.2,-6.97028447084552));
#175770=CARTESIAN_POINT('Ctrl Pts',(9.1015861961174,15.2,-6.97131787373208));
#175771=CARTESIAN_POINT('Ctrl Pts',(9.10652458633233,15.2,-6.97234615817649));
#175772=CARTESIAN_POINT('Ctrl Pts',(9.11022837865709,15.2,-6.97311737143975));
#175773=CARTESIAN_POINT('Ctrl Pts',(9.11393954876789,15.2,-6.97388570387134));
#175774=CARTESIAN_POINT('Ctrl Pts',(9.11765806998607,15.2,-6.97465112288143));
#175775=CARTESIAN_POINT('Ctrl Pts',(9.12137659120426,15.2,-6.97541654189152));
#175776=CARTESIAN_POINT('Ctrl Pts',(9.12510246279873,15.2,-6.97617904627868));
#175777=CARTESIAN_POINT('Ctrl Pts',(9.12883567209274,15.2,-6.9769386231241));
#175778=CARTESIAN_POINT('Ctrl Pts',(9.13256888138674,15.2,-6.97769819996954));
#175779=CARTESIAN_POINT('Ctrl Pts',(9.13630943331908,15.2,-6.9784548508631));
#175780=CARTESIAN_POINT('Ctrl Pts',(9.14005731399994,15.2,-6.97920857100002));
#175781=CARTESIAN_POINT('Ctrl Pts',(8.02901631899994,12.2,-6.57080831800001));
#175782=CARTESIAN_POINT('Ctrl Pts',(8.03049110016105,12.2,-6.57181686697944));
#175783=CARTESIAN_POINT('Ctrl Pts',(8.03201610877769,12.2,-6.57285322878717));
#175784=CARTESIAN_POINT('Ctrl Pts',(8.03359089353572,12.2,-6.5739163521752));
#175785=CARTESIAN_POINT('Ctrl Pts',(8.03517327270188,12.2,-6.57498460248157));
#175786=CARTESIAN_POINT('Ctrl Pts',(8.03680591622578,12.2,-6.5760798659982));
#175787=CARTESIAN_POINT('Ctrl Pts',(8.0384883906544,12.2,-6.57720107836683));
#175788=CARTESIAN_POINT('Ctrl Pts',(8.04017086493022,12.2,-6.5783222906336));
#175789=CARTESIAN_POINT('Ctrl Pts',(8.04190317335625,12.2,-6.57946945420923));
#175790=CARTESIAN_POINT('Ctrl Pts',(8.04368489154152,12.2,-6.58064153749996));
#175791=CARTESIAN_POINT('Ctrl Pts',(8.04546660972677,12.2,-6.5818136207907));
#175792=CARTESIAN_POINT('Ctrl Pts',(8.04729774128699,12.2,-6.58301062499168));
#175793=CARTESIAN_POINT('Ctrl Pts',(8.04917787055977,12.2,-6.58423155042359));
#175794=CARTESIAN_POINT('Ctrl Pts',(8.05105800000331,12.2,-6.5854524759664));
#175795=CARTESIAN_POINT('Ctrl Pts',(8.05298713001268,12.2,-6.58669732252585));
#175796=CARTESIAN_POINT('Ctrl Pts',(8.05496485620711,12.2,-6.58796512017984));
#175797=CARTESIAN_POINT('Ctrl Pts',(8.05694258222188,12.2,-6.58923291771867));
#175798=CARTESIAN_POINT('Ctrl Pts',(8.05896890494999,12.2,-6.59052366460892));
#175799=CARTESIAN_POINT('Ctrl Pts',(8.0610434290508,12.2,-6.59183642123391));
#175800=CARTESIAN_POINT('Ctrl Pts',(8.06311795315161,12.2,-6.59314917785888));
#175801=CARTESIAN_POINT('Ctrl Pts',(8.06524067911272,12.2,-6.59448394143469));
#175802=CARTESIAN_POINT('Ctrl Pts',(8.0674112193651,12.2,-6.59583979613451));
#175803=CARTESIAN_POINT('Ctrl Pts',(8.06958175981464,12.2,-6.59719565095748));
#175804=CARTESIAN_POINT('Ctrl Pts',(8.07180011545347,12.2,-6.59857259622476));
#175805=CARTESIAN_POINT('Ctrl Pts',(8.07406590574684,12.2,-6.5999697421356));
#175806=CARTESIAN_POINT('Ctrl Pts',(8.0763316958344,12.2,-6.60136688791955));
#175807=CARTESIAN_POINT('Ctrl Pts',(8.07864492166241,12.2,-6.60278423372139));
#175808=CARTESIAN_POINT('Ctrl Pts',(8.08100520891203,12.2,-6.6042209115867));
#175809=CARTESIAN_POINT('Ctrl Pts',(8.08336549616167,12.2,-6.605657589452));
#175810=CARTESIAN_POINT('Ctrl Pts',(8.08577284714085,12.2,-6.60711359752408));
#175811=CARTESIAN_POINT('Ctrl Pts',(8.08822689338298,12.2,-6.60858809463637));
#175812=CARTESIAN_POINT('Ctrl Pts',(8.09068093962512,12.2,-6.61006259174866));
#175813=CARTESIAN_POINT('Ctrl Pts',(8.09318168337629,12.2,-6.61155557734142));
#175814=CARTESIAN_POINT('Ctrl Pts',(8.09572876369724,12.2,-6.61306622661866));
#175815=CARTESIAN_POINT('Ctrl Pts',(8.09827584424958,12.2,-6.61457687603312));
#175816=CARTESIAN_POINT('Ctrl Pts',(8.10086926328141,12.2,-6.61610519224932));
#175817=CARTESIAN_POINT('Ctrl Pts',(8.10350866492724,12.2,-6.61765036983427));
#175818=CARTESIAN_POINT('Ctrl Pts',(8.10614806633333,12.2,-6.61919554727886));
#175819=CARTESIAN_POINT('Ctrl Pts',(8.1088334533189,12.2,-6.62075759161615));
#175820=CARTESIAN_POINT('Ctrl Pts',(8.11156447473195,12.2,-6.6223357152326));
#175821=CARTESIAN_POINT('Ctrl Pts',(8.114295496145,12.2,-6.62391383884905));
#175822=CARTESIAN_POINT('Ctrl Pts',(8.11707215585626,12.2,-6.62550804652576));
#175823=CARTESIAN_POINT('Ctrl Pts',(8.11989411016728,12.2,-6.62711757488289));
#175824=CARTESIAN_POINT('Ctrl Pts',(8.12271606473465,12.2,-6.62872710338622));
#175825=CARTESIAN_POINT('Ctrl Pts',(8.12558331191476,12.2,-6.6303519509994));
#175826=CARTESIAN_POINT('Ctrl Pts',(8.12849551940877,12.2,-6.6319913775894));
#175827=CARTESIAN_POINT('Ctrl Pts',(8.13140772663827,12.2,-6.63363080403048));
#175828=CARTESIAN_POINT('Ctrl Pts',(8.13436489026073,12.2,-6.63528480749396));
#175829=CARTESIAN_POINT('Ctrl Pts',(8.13736668249851,12.2,-6.63695266402424));
#175830=CARTESIAN_POINT('Ctrl Pts',(8.14036847473629,12.2,-6.63862052055451));
#175831=CARTESIAN_POINT('Ctrl Pts',(8.143414891645,12.2,-6.64030222865274));
#175832=CARTESIAN_POINT('Ctrl Pts',(8.14650561086298,12.2,-6.64199708134025));
#175833=CARTESIAN_POINT('Ctrl Pts',(8.14959633036172,12.2,-6.64369193418172));
#175834=CARTESIAN_POINT('Ctrl Pts',(8.15273134873956,12.2,-6.64539993184436));
#175835=CARTESIAN_POINT('Ctrl Pts',(8.15591034657417,12.2,-6.64712038194146));
#175836=CARTESIAN_POINT('Ctrl Pts',(8.15908934412002,12.2,-6.64884083188229));
#175837=CARTESIAN_POINT('Ctrl Pts',(8.16231231913522,12.2,-6.65057373512172));
#175838=CARTESIAN_POINT('Ctrl Pts',(8.16557895468321,12.2,-6.652318415975));
#175839=CARTESIAN_POINT('Ctrl Pts',(8.16884559023118,12.2,-6.65406309682828));
#175840=CARTESIAN_POINT('Ctrl Pts',(8.17215588798237,12.2,-6.6558195550556));
#175841=CARTESIAN_POINT('Ctrl Pts',(8.17550953269222,12.2,-6.65758713107903));
#175842=CARTESIAN_POINT('Ctrl Pts',(8.1788631777067,12.2,-6.65935470726302));
#175843=CARTESIAN_POINT('Ctrl Pts',(8.18226017085943,12.2,-6.66113339979679));
#175844=CARTESIAN_POINT('Ctrl Pts',(8.18570020263318,12.2,-6.66292256589502));
#175845=CARTESIAN_POINT('Ctrl Pts',(8.18914023409444,12.2,-6.66471173183071));
#175846=CARTESIAN_POINT('Ctrl Pts',(8.19262330411346,12.2,-6.66651136898332));
#175847=CARTESIAN_POINT('Ctrl Pts',(8.19614910850148,12.2,-6.66832084800916));
#175848=CARTESIAN_POINT('Ctrl Pts',(8.1996749128895,12.2,-6.67013032703499));
#175849=CARTESIAN_POINT('Ctrl Pts',(8.20324344950297,12.2,-6.67194964697555));
#175850=CARTESIAN_POINT('Ctrl Pts',(8.20685441903659,12.2,-6.67377819115872));
#175851=CARTESIAN_POINT('Ctrl Pts',(8.20986356042395,12.2,-6.67530197803339));
#175852=CARTESIAN_POINT('Ctrl Pts',(8.21290216949536,12.2,-6.67683217109432));
#175853=CARTESIAN_POINT('Ctrl Pts',(8.21597007254941,12.2,-6.67836841894123));
#175854=CARTESIAN_POINT('Ctrl Pts',(8.21903797560345,12.2,-6.67990466678815));
#175855=CARTESIAN_POINT('Ctrl Pts',(8.22213517386183,12.2,-6.68144697092547));
#175856=CARTESIAN_POINT('Ctrl Pts',(8.22526149526484,12.2,-6.68299498697416));
#175857=CARTESIAN_POINT('Ctrl Pts',(8.22838781666785,12.2,-6.68454300302284));
#175858=CARTESIAN_POINT('Ctrl Pts',(8.23154326107765,12.2,-6.68609673040001));
#175859=CARTESIAN_POINT('Ctrl Pts',(8.2347276622582,12.2,-6.687655832275));
#175860=CARTESIAN_POINT('Ctrl Pts',(8.23791206343875,12.2,-6.68921493415));
#175861=CARTESIAN_POINT('Ctrl Pts',(8.24112541779795,12.2,-6.6907794097326));
#175862=CARTESIAN_POINT('Ctrl Pts',(8.24436756003497,12.2,-6.69234892751752));
#175863=CARTESIAN_POINT('Ctrl Pts',(8.247609702272,12.2,-6.69391844530244));
#175864=CARTESIAN_POINT('Ctrl Pts',(8.25088063221432,12.2,-6.69549300500862));
#175865=CARTESIAN_POINT('Ctrl Pts',(8.25418018346583,12.2,-6.69707228111998));
#175866=CARTESIAN_POINT('Ctrl Pts',(8.25747973471734,12.2,-6.69865155723135));
#175867=CARTESIAN_POINT('Ctrl Pts',(8.2608079052903,12.2,-6.70023554877035));
#175868=CARTESIAN_POINT('Ctrl Pts',(8.26416453494457,12.2,-6.70182393585391));
#175869=CARTESIAN_POINT('Ctrl Pts',(8.26752116459883,12.2,-6.70341232293748));
#175870=CARTESIAN_POINT('Ctrl Pts',(8.27090625117372,12.2,-6.70500510627755));
#175871=CARTESIAN_POINT('Ctrl Pts',(8.27431963113788,12.2,-6.70660196851039));
#175872=CARTESIAN_POINT('Ctrl Pts',(8.27773301110205,12.2,-6.70819883074322));
#175873=CARTESIAN_POINT('Ctrl Pts',(8.28117468484588,12.2,-6.70979977331515));
#175874=CARTESIAN_POINT('Ctrl Pts',(8.28464449123708,12.2,-6.71140448546824));
#175875=CARTESIAN_POINT('Ctrl Pts',(8.28811429762827,12.2,-6.71300919762133));
#175876=CARTESIAN_POINT('Ctrl Pts',(8.29161223679768,12.2,-6.71461768115501));
#175877=CARTESIAN_POINT('Ctrl Pts',(8.2951381474944,12.2,-6.71622962921085));
#175878=CARTESIAN_POINT('Ctrl Pts',(8.29866405780679,12.2,-6.71784157709098));
#175879=CARTESIAN_POINT('Ctrl Pts',(8.30221794072407,12.2,-6.71945699085943));
#175880=CARTESIAN_POINT('Ctrl Pts',(8.3057996359564,12.2,-6.72107556957163));
#175881=CARTESIAN_POINT('Ctrl Pts',(8.30938133157914,12.2,-6.72269414846026));
#175882=CARTESIAN_POINT('Ctrl Pts',(8.3129908419153,12.2,-6.72431589354331));
#175883=CARTESIAN_POINT('Ctrl Pts',(8.31662800677414,12.2,-6.72594050902918));
#175884=CARTESIAN_POINT('Ctrl Pts',(8.32026517163299,12.2,-6.72756512451505));
#175885=CARTESIAN_POINT('Ctrl Pts',(8.32392999151359,12.2,-6.72919260987033));
#175886=CARTESIAN_POINT('Ctrl Pts',(8.32762231206693,12.2,-6.73082267632846));
#175887=CARTESIAN_POINT('Ctrl Pts',(8.33131463262026,12.2,-6.73245274278659));
#175888=CARTESIAN_POINT('Ctrl Pts',(8.33503444951857,12.2,-6.73408539065649));
#175889=CARTESIAN_POINT('Ctrl Pts',(8.33878161352332,12.2,-6.73572033233523));
#175890=CARTESIAN_POINT('Ctrl Pts',(8.34252877752806,12.2,-6.73735527401396));
#175891=CARTESIAN_POINT('Ctrl Pts',(8.34630328487505,12.2,-6.73899251140958));
#175892=CARTESIAN_POINT('Ctrl Pts',(8.35010498223474,12.2,-6.74063176286782));
#175893=CARTESIAN_POINT('Ctrl Pts',(8.35390667959444,12.2,-6.74227101432605));
#175894=CARTESIAN_POINT('Ctrl Pts',(8.35773556658815,12.2,-6.74391227885931));
#175895=CARTESIAN_POINT('Ctrl Pts',(8.36159149144786,12.2,-6.7455552811509));
#175896=CARTESIAN_POINT('Ctrl Pts',(8.36467623150374,12.2,-6.74686968305581));
#175897=CARTESIAN_POINT('Ctrl Pts',(8.36777827623639,12.2,-6.74818519696456));
#175898=CARTESIAN_POINT('Ctrl Pts',(8.37089754645259,12.2,-6.74950168365771));
#175899=CARTESIAN_POINT('Ctrl Pts',(8.3740168162438,12.2,-6.7508181701715));
#175900=CARTESIAN_POINT('Ctrl Pts',(8.37715331159283,12.2,-6.75213562847229));
#175901=CARTESIAN_POINT('Ctrl Pts',(8.38030695650056,12.2,-6.75345392214225));
#175902=CARTESIAN_POINT('Ctrl Pts',(8.38346060183799,12.2,-6.75477221599183));
#175903=CARTESIAN_POINT('Ctrl Pts',(8.3866313966969,12.2,-6.7560913433665));
#175904=CARTESIAN_POINT('Ctrl Pts',(8.38981926276065,12.2,-6.75741116938291));
#175905=CARTESIAN_POINT('Ctrl Pts',(8.39300712839004,12.2,-6.7587309952195));
#175906=CARTESIAN_POINT('Ctrl Pts',(8.3962120660197,12.2,-6.7600515191087));
#175907=CARTESIAN_POINT('Ctrl Pts',(8.39943399924911,12.2,-6.76137260756665));
#175908=CARTESIAN_POINT('Ctrl Pts',(8.40265593291753,12.2,-6.7626936962046));
#175909=CARTESIAN_POINT('Ctrl Pts',(8.40589486317934,12.2,-6.7640153482388));
#175910=CARTESIAN_POINT('Ctrl Pts',(8.40915071252453,12.2,-6.76533743036643));
#175911=CARTESIAN_POINT('Ctrl Pts',(8.41240656142612,12.2,-6.76665951231393));
#175912=CARTESIAN_POINT('Ctrl Pts',(8.415679330241,12.2,-6.76798202511968));
#175913=CARTESIAN_POINT('Ctrl Pts',(8.41896894247037,12.2,-6.76930483823374));
#175914=CARTESIAN_POINT('Ctrl Pts',(8.42225855514795,12.2,-6.77062765152802));
#175915=CARTESIAN_POINT('Ctrl Pts',(8.42556501196421,12.2,-6.77195076309222));
#175916=CARTESIAN_POINT('Ctrl Pts',(8.42888823799381,12.2,-6.77327404522592));
#175917=CARTESIAN_POINT('Ctrl Pts',(8.43221146357063,12.2,-6.77459732717931));
#175918=CARTESIAN_POINT('Ctrl Pts',(8.43555145772162,12.2,-6.77592077960571));
#175919=CARTESIAN_POINT('Ctrl Pts',(8.43890814600108,12.2,-6.7772442727753));
#175920=CARTESIAN_POINT('Ctrl Pts',(8.44226483473788,12.2,-6.77856776612521));
#175921=CARTESIAN_POINT('Ctrl Pts',(8.44563821709011,12.2,-6.77989130153066));
#175922=CARTESIAN_POINT('Ctrl Pts',(8.44902821977488,12.2,-6.78121475099168));
#175923=CARTESIAN_POINT('Ctrl Pts',(8.45241822245964,12.2,-6.7825382004527));
#175924=CARTESIAN_POINT('Ctrl Pts',(8.45582484410188,12.2,-6.78386156511927));
#175925=CARTESIAN_POINT('Ctrl Pts',(8.45924801156791,12.2,-6.78518471869135));
#175926=CARTESIAN_POINT('Ctrl Pts',(8.46267117856753,12.2,-6.78650787208315));
#175927=CARTESIAN_POINT('Ctrl Pts',(8.46611089167832,12.2,-6.78783081717345));
#175928=CARTESIAN_POINT('Ctrl Pts',(8.46956707602253,12.2,-6.78915342651578));
#175929=CARTESIAN_POINT('Ctrl Pts',(8.47302326083764,12.2,-6.79047603603832));
#175930=CARTESIAN_POINT('Ctrl Pts',(8.47649591951185,12.2,-6.79179831183302));
#175931=CARTESIAN_POINT('Ctrl Pts',(8.47998497503701,12.2,-6.7931201306828));
#175932=CARTESIAN_POINT('Ctrl Pts',(8.4834740300868,12.2,-6.79444194935248));
#175933=CARTESIAN_POINT('Ctrl Pts',(8.48697948355943,12.2,-6.79576331160275));
#175934=CARTESIAN_POINT('Ctrl Pts',(8.49050126377046,12.2,-6.79708409688371));
#175935=CARTESIAN_POINT('Ctrl Pts',(8.49402304446134,12.2,-6.79840488234462));
#175936=CARTESIAN_POINT('Ctrl Pts',(8.49756114899859,12.2,-6.79972509074538));
#175937=CARTESIAN_POINT('Ctrl Pts',(8.5011155084824,12.2,-6.80104460171649));
#175938=CARTESIAN_POINT('Ctrl Pts',(8.50466986748193,12.2,-6.80236411250781));
#175939=CARTESIAN_POINT('Ctrl Pts',(8.50824047931775,12.2,-6.80368292767495));
#175940=CARTESIAN_POINT('Ctrl Pts',(8.51182727169015,12.2,-6.8050009264006));
#175941=CARTESIAN_POINT('Ctrl Pts',(8.51541406455124,12.2,-6.80631892530581));
#175942=CARTESIAN_POINT('Ctrl Pts',(8.51901703779205,12.2,-6.80763610905538));
#175943=CARTESIAN_POINT('Ctrl Pts',(8.52263612054589,12.2,-6.80895236184928));
#175944=CARTESIAN_POINT('Ctrl Pts',(8.52625520280664,12.2,-6.81026861446384));
#175945=CARTESIAN_POINT('Ctrl Pts',(8.52989039319317,12.2,-6.8115839357121));
#175946=CARTESIAN_POINT('Ctrl Pts',(8.53354162218682,12.2,-6.8128982085593));
#175947=CARTESIAN_POINT('Ctrl Pts',(8.53719285167795,12.2,-6.81421248158557));
#175948=CARTESIAN_POINT('Ctrl Pts',(8.54086011784936,12.2,-6.8155257078775));
#175949=CARTESIAN_POINT('Ctrl Pts',(8.54454335005114,12.2,-6.8168377721156));
#175950=CARTESIAN_POINT('Ctrl Pts',(8.54822658175108,12.2,-6.81814983617493));
#175951=CARTESIAN_POINT('Ctrl Pts',(8.55192578000058,12.2,-6.81946073921782));
#175952=CARTESIAN_POINT('Ctrl Pts',(8.55564087241747,12.2,-6.82077036727756));
#175953=CARTESIAN_POINT('Ctrl Pts',(8.55935596534054,12.2,-6.82207999551573));
#175954=CARTESIAN_POINT('Ctrl Pts',(8.56308695390617,12.2,-6.82338834881264));
#175955=CARTESIAN_POINT('Ctrl Pts',(8.5668337672941,12.2,-6.82469531700091));
#175956=CARTESIAN_POINT('Ctrl Pts',(8.57058058017153,12.2,-6.82600228501111));
#175957=CARTESIAN_POINT('Ctrl Pts',(8.57434321779261,12.2,-6.82730786580159));
#175958=CARTESIAN_POINT('Ctrl Pts',(8.57812160814879,12.2,-6.82861195052847));
#175959=CARTESIAN_POINT('Ctrl Pts',(8.58189999901978,12.2,-6.82991603543304));
#175960=CARTESIAN_POINT('Ctrl Pts',(8.58569414515892,12.2,-6.83121862397356));
#175961=CARTESIAN_POINT('Ctrl Pts',(8.58950397469988,12.2,-6.83251960626669));
#175962=CARTESIAN_POINT('Ctrl Pts',(8.59426626136654,12.2,-6.83414583404446));
#175963=CARTESIAN_POINT('Ctrl Pts',(8.59905305545545,12.2,-6.83576955228337));
#175964=CARTESIAN_POINT('Ctrl Pts',(8.60386421802488,12.2,-6.83739055020003));
#175965=CARTESIAN_POINT('Ctrl Pts',(8.60771314829021,12.2,-6.83868734860403));
#175966=CARTESIAN_POINT('Ctrl Pts',(8.61157767655179,12.2,-6.83998240684951));
#175967=CARTESIAN_POINT('Ctrl Pts',(8.61545773137595,12.2,-6.84127561775313));
#175968=CARTESIAN_POINT('Ctrl Pts',(8.61933778567146,12.2,-6.84256882848056));
#175969=CARTESIAN_POINT('Ctrl Pts',(8.62323336771314,12.2,-6.84386019109314));
#175970=CARTESIAN_POINT('Ctrl Pts',(8.62714440868889,12.2,-6.84514960121581));
#175971=CARTESIAN_POINT('Ctrl Pts',(8.63105545019752,12.2,-6.84643901151416));
#175972=CARTESIAN_POINT('Ctrl Pts',(8.63498194935854,12.2,-6.84772646893479));
#175973=CARTESIAN_POINT('Ctrl Pts',(8.63892383818605,12.2,-6.84901186922685));
#175974=CARTESIAN_POINT('Ctrl Pts',(8.64286572647648,12.2,-6.85029726934378));
#175975=CARTESIAN_POINT('Ctrl Pts',(8.64682300519824,12.2,-6.85158061194986));
#175976=CARTESIAN_POINT('Ctrl Pts',(8.65079560415027,12.2,-6.8528617941786));
#175977=CARTESIAN_POINT('Ctrl Pts',(8.65476820364356,12.2,-6.85414297658189));
#175978=CARTESIAN_POINT('Ctrl Pts',(8.65875612331969,12.2,-6.85542199905211));
#175979=CARTESIAN_POINT('Ctrl Pts',(8.66275929757252,12.2,-6.85669875818528));
#175980=CARTESIAN_POINT('Ctrl Pts',(8.66676247127991,12.2,-6.8579755171445));
#175981=CARTESIAN_POINT('Ctrl Pts',(8.67078089611491,12.2,-6.8592500152193));
#175982=CARTESIAN_POINT('Ctrl Pts',(8.67481450639528,12.2,-6.860522148171));
#175983=CARTESIAN_POINT('Ctrl Pts',(8.67884811722522,12.2,-6.86179428129605));
#175984=CARTESIAN_POINT('Ctrl Pts',(8.68289691163479,12.2,-6.86306405099859));
#175985=CARTESIAN_POINT('Ctrl Pts',(8.68696082435725,12.2,-6.86433135734527));
#175986=CARTESIAN_POINT('Ctrl Pts',(8.69102473652601,12.2,-6.86559866351929));
#175987=CARTESIAN_POINT('Ctrl Pts',(8.69510376418181,12.2,-6.86686350616786));
#175988=CARTESIAN_POINT('Ctrl Pts',(8.6991978426059,12.2,-6.86812578635018));
#175989=CARTESIAN_POINT('Ctrl Pts',(8.70329192158781,12.2,-6.86938806670449));
#175990=CARTESIAN_POINT('Ctrl Pts',(8.70740104922534,12.2,-6.87064778431777));
#175991=CARTESIAN_POINT('Ctrl Pts',(8.71152515939551,12.2,-6.8719048413861));
#175992=CARTESIAN_POINT('Ctrl Pts',(8.71564926900379,12.2,-6.87316189828317));
#175993=CARTESIAN_POINT('Ctrl Pts',(8.71978836024517,12.2,-6.87441629478354));
#175994=CARTESIAN_POINT('Ctrl Pts',(8.72394236657071,12.2,-6.87566793373705));
#175995=CARTESIAN_POINT('Ctrl Pts',(8.72809637346226,12.2,-6.8769195728611));
#175996=CARTESIAN_POINT('Ctrl Pts',(8.73226529536955,12.2,-6.87816845470787));
#175997=CARTESIAN_POINT('Ctrl Pts',(8.73644906622774,12.2,-6.87941448372587));
#175998=CARTESIAN_POINT('Ctrl Pts',(8.74063283651589,12.2,-6.88066051257411));
#175999=CARTESIAN_POINT('Ctrl Pts',(8.74483145490418,12.2,-6.88190368835111));
#176000=CARTESIAN_POINT('Ctrl Pts',(8.74904485450267,12.2,-6.88314391530558));
#176001=CARTESIAN_POINT('Ctrl Pts',(8.75325825467524,12.2,-6.88438414242903));
#176002=CARTESIAN_POINT('Ctrl Pts',(8.75748643633254,12.2,-6.88562142168276));
#176003=CARTESIAN_POINT('Ctrl Pts',(8.76172933450822,12.2,-6.88685565875003));
#176004=CARTESIAN_POINT('Ctrl Pts',(8.76703295693875,12.2,-6.88839845500002));
#176005=CARTESIAN_POINT('Ctrl Pts',(8.77235957187289,12.2,-6.8899364977828));
#176006=CARTESIAN_POINT('Ctrl Pts',(8.77770904953614,12.2,-6.89146960577586));
#176007=CARTESIAN_POINT('Ctrl Pts',(8.78091873601747,12.2,-6.89238947053828));
#176008=CARTESIAN_POINT('Ctrl Pts',(8.78413665429956,12.2,-6.89330755887832));
#176009=CARTESIAN_POINT('Ctrl Pts',(8.78736277523863,12.2,-6.8942238317242));
#176010=CARTESIAN_POINT('Ctrl Pts',(8.79058889617769,12.2,-6.89514010457007));
#176011=CARTESIAN_POINT('Ctrl Pts',(8.79382322081512,12.2,-6.89605456383352));
#176012=CARTESIAN_POINT('Ctrl Pts',(8.79706572115493,12.2,-6.89696716767552));
#176013=CARTESIAN_POINT('Ctrl Pts',(8.80030822149474,12.2,-6.89787977151753));
#176014=CARTESIAN_POINT('Ctrl Pts',(8.80355889662566,12.2,-6.89879052146799));
#176015=CARTESIAN_POINT('Ctrl Pts',(8.80681771950614,12.2,-6.89969937976857));
#176016=CARTESIAN_POINT('Ctrl Pts',(8.81007654297864,12.2,-6.90060823823424));
#176017=CARTESIAN_POINT('Ctrl Pts',(8.81334351458678,12.2,-6.90151520521606));
#176018=CARTESIAN_POINT('Ctrl Pts',(8.81661860698053,12.2,-6.90242024168066));
#176019=CARTESIAN_POINT('Ctrl Pts',(8.81989369877931,12.2,-6.90332527798084));
#176020=CARTESIAN_POINT('Ctrl Pts',(8.8231769106243,12.2,-6.90422838507897));
#176021=CARTESIAN_POINT('Ctrl Pts',(8.82646821517008,12.2,-6.90512952396602));
#176022=CARTESIAN_POINT('Ctrl Pts',(8.82975951971587,12.2,-6.90603066285308));
#176023=CARTESIAN_POINT('Ctrl Pts',(8.83305891673001,12.2,-6.90692983469723));
#176024=CARTESIAN_POINT('Ctrl Pts',(8.83636637961053,12.2,-6.90782700108112));
#176025=CARTESIAN_POINT('Ctrl Pts',(8.83967384249106,12.2,-6.90872416746502));
#176026=CARTESIAN_POINT('Ctrl Pts',(8.84298937082064,12.2,-6.90961933044915));
#176027=CARTESIAN_POINT('Ctrl Pts',(8.84631293674155,12.2,-6.9105124502917));
#176028=CARTESIAN_POINT('Ctrl Pts',(8.84963650266246,12.2,-6.91140557013425));
#176029=CARTESIAN_POINT('Ctrl Pts',(8.85296810679138,12.2,-6.91229664810188));
#176030=CARTESIAN_POINT('Ctrl Pts',(8.856307722086,12.2,-6.91318564740309));
#176031=CARTESIAN_POINT('Ctrl Pts',(8.85964733738063,12.2,-6.91407464670431));
#176032=CARTESIAN_POINT('Ctrl Pts',(8.86299496240595,12.2,-6.91496156678319));
#176033=CARTESIAN_POINT('Ctrl Pts',(8.86635057186741,12.2,-6.91584637254549));
#176034=CARTESIAN_POINT('Ctrl Pts',(8.86970618132887,12.2,-6.91673117830779));
#176035=CARTESIAN_POINT('Ctrl Pts',(8.87306977413848,12.2,-6.91761386835644));
#176036=CARTESIAN_POINT('Ctrl Pts',(8.87644132305657,12.2,-6.91849440707474));
#176037=CARTESIAN_POINT('Ctrl Pts',(8.87981287258715,12.2,-6.91937494595301));
#176038=CARTESIAN_POINT('Ctrl Pts',(8.88319237864497,12.2,-6.920253332864));
#176039=CARTESIAN_POINT('Ctrl Pts',(8.88657981368003,12.2,-6.92112953324104));
#176040=CARTESIAN_POINT('Ctrl Pts',(8.8899672480997,12.2,-6.9220057334589));
#176041=CARTESIAN_POINT('Ctrl Pts',(8.89336261259395,12.2,-6.92287974501023));
#176042=CARTESIAN_POINT('Ctrl Pts',(8.89676587892931,12.2,-6.92375153381169));
#176043=CARTESIAN_POINT('Ctrl Pts',(8.90016914526467,12.2,-6.92462332261315));
#176044=CARTESIAN_POINT('Ctrl Pts',(8.90358031307833,12.2,-6.92549288789506));
#176045=CARTESIAN_POINT('Ctrl Pts',(8.90699935651133,12.2,-6.92636019474249));
#176046=CARTESIAN_POINT('Ctrl Pts',(8.91041839994434,12.2,-6.9272275015899));
#176047=CARTESIAN_POINT('Ctrl Pts',(8.91384531928933,12.2,-6.92809255112666));
#176048=CARTESIAN_POINT('Ctrl Pts',(8.91728008622177,12.2,-6.92895530551591));
#176049=CARTESIAN_POINT('Ctrl Pts',(8.92071485315421,12.2,-6.92981805990516));
#176050=CARTESIAN_POINT('Ctrl Pts',(8.9241574686833,12.2,-6.93067852082076));
#176051=CARTESIAN_POINT('Ctrl Pts',(8.92760790514059,12.2,-6.93153665266479));
#176052=CARTESIAN_POINT('Ctrl Pts',(8.93105834159788,12.2,-6.93239478450881));
#176053=CARTESIAN_POINT('Ctrl Pts',(8.93451660055463,12.2,-6.93325058724467));
#176054=CARTESIAN_POINT('Ctrl Pts',(8.9379826534693,12.2,-6.93410402704731));
#176055=CARTESIAN_POINT('Ctrl Pts',(8.94144870701363,12.2,-6.934957467005));
#176056=CARTESIAN_POINT('Ctrl Pts',(8.9449225547185,12.2,-6.93580854341203));
#176057=CARTESIAN_POINT('Ctrl Pts',(8.94840417072556,12.2,-6.93665722145171));
#176058=CARTESIAN_POINT('Ctrl Pts',(8.95188578610012,12.2,-6.93750589933722));
#176059=CARTESIAN_POINT('Ctrl Pts',(8.95537516979094,12.2,-6.93835218048951));
#176060=CARTESIAN_POINT('Ctrl Pts',(8.95887229462287,12.2,-6.9391960283753));
#176061=CARTESIAN_POINT('Ctrl Pts',(8.96236941945481,12.2,-6.9400398762611));
#176062=CARTESIAN_POINT('Ctrl Pts',(8.96587428511472,12.2,-6.94088129189414));
#176063=CARTESIAN_POINT('Ctrl Pts',(8.96938686554475,12.2,-6.94172024178413));
#176064=CARTESIAN_POINT('Ctrl Pts',(8.97289944597478,12.2,-6.94255919167411));
#176065=CARTESIAN_POINT('Ctrl Pts',(8.97641974169222,12.2,-6.94339567577577));
#176066=CARTESIAN_POINT('Ctrl Pts',(8.97994772470502,12.2,-6.94422965970761));
#176067=CARTESIAN_POINT('Ctrl Pts',(8.98347570771783,12.2,-6.94506364363944));
#176068=CARTESIAN_POINT('Ctrl Pts',(8.98701138010987,12.2,-6.94589512877286));
#176069=CARTESIAN_POINT('Ctrl Pts',(8.99055471260546,12.2,-6.94672407965963));
#176070=CARTESIAN_POINT('Ctrl Pts',(8.99409804510107,12.2,-6.9475530305464));
#176071=CARTESIAN_POINT('Ctrl Pts',(8.99764904030446,12.2,-6.94837944795001));
#176072=CARTESIAN_POINT('Ctrl Pts',(9.00120766971578,12.2,-6.94920329929543));
#176073=CARTESIAN_POINT('Ctrl Pts',(9.00476629977359,12.2,-6.95002715079051));
#176074=CARTESIAN_POINT('Ctrl Pts',(9.00833256505857,12.2,-6.95084843617654));
#176075=CARTESIAN_POINT('Ctrl Pts',(9.01190643957901,12.2,-6.95166712171184));
#176076=CARTESIAN_POINT('Ctrl Pts',(9.0154803134502,12.2,-6.9524858070984));
#176077=CARTESIAN_POINT('Ctrl Pts',(9.01906179657792,12.2,-6.95330189324661));
#176078=CARTESIAN_POINT('Ctrl Pts',(9.02265086121103,12.2,-6.95411534763239));
#176079=CARTESIAN_POINT('Ctrl Pts',(9.02623992584414,12.2,-6.95492880201817));
#176080=CARTESIAN_POINT('Ctrl Pts',(9.02983657273984,12.2,-6.95573962368434));
#176081=CARTESIAN_POINT('Ctrl Pts',(9.03344077565121,12.2,-6.95654778007141));
#176082=CARTESIAN_POINT('Ctrl Pts',(9.03704497856259,12.2,-6.95735593645849));
#176083=CARTESIAN_POINT('Ctrl Pts',(9.04065673728139,12.2,-6.9581614281292));
#176084=CARTESIAN_POINT('Ctrl Pts',(9.04427602623322,12.2,-6.9589642235167));
#176085=CARTESIAN_POINT('Ctrl Pts',(9.04789531518505,12.2,-6.9597670189042));
#176086=CARTESIAN_POINT('Ctrl Pts',(9.05152213511992,12.2,-6.96056711802514));
#176087=CARTESIAN_POINT('Ctrl Pts',(9.05515645857055,12.2,-6.96136448837141));
#176088=CARTESIAN_POINT('Ctrl Pts',(9.05879078202118,12.2,-6.96216185871767));
#176089=CARTESIAN_POINT('Ctrl Pts',(9.06243261019506,12.2,-6.96295649975236));
#176090=CARTESIAN_POINT('Ctrl Pts',(9.06608191474392,12.2,-6.9637483795968));
#176091=CARTESIAN_POINT('Ctrl Pts',(9.07094765458435,12.2,-6.96480421948529));
#176092=CARTESIAN_POINT('Ctrl Pts',(9.07582668513524,12.2,-6.96585514807604));
#176093=CARTESIAN_POINT('Ctrl Pts',(9.08071894812496,12.2,-6.96690109407716));
#176094=CARTESIAN_POINT('Ctrl Pts',(9.08438814503396,12.2,-6.96768555350675));
#176095=CARTESIAN_POINT('Ctrl Pts',(9.08806478513374,12.2,-6.968467210345));
#176096=CARTESIAN_POINT('Ctrl Pts',(9.09174884449989,12.2,-6.96924603623337));
#176097=CARTESIAN_POINT('Ctrl Pts',(9.09543290386604,12.2,-6.97002486212174));
#176098=CARTESIAN_POINT('Ctrl Pts',(9.09912438294854,12.2,-6.97080085739356));
#176099=CARTESIAN_POINT('Ctrl Pts',(9.10282325310517,12.2,-6.97157398615738));
#176100=CARTESIAN_POINT('Ctrl Pts',(9.10652212326181,12.2,-6.97234711492121));
#176101=CARTESIAN_POINT('Ctrl Pts',(9.11022838124838,12.2,-6.97311737640742));
#176102=CARTESIAN_POINT('Ctrl Pts',(9.11394199879815,12.2,-6.97388473387654));
#176103=CARTESIAN_POINT('Ctrl Pts',(9.1176556163479,12.2,-6.97465209134567));
#176104=CARTESIAN_POINT('Ctrl Pts',(9.12137659252359,12.2,-6.97541654399462));
#176105=CARTESIAN_POINT('Ctrl Pts',(9.12510490826213,12.2,-6.97617807080069));
#176106=CARTESIAN_POINT('Ctrl Pts',(9.13007599636506,12.2,-6.97719343996767));
#176107=CARTESIAN_POINT('Ctrl Pts',(9.13506013930488,12.2,-6.97820361072618));
#176108=CARTESIAN_POINT('Ctrl Pts',(9.14005731399994,12.2,-6.97920857100002));
#176109=CARTESIAN_POINT('Ctrl Pts',(9.36775917499994,15.2,-6.67046385500001));
#176110=CARTESIAN_POINT('Ctrl Pts',(9.36775917499994,11.6,-6.67046385500001));
#176111=CARTESIAN_POINT('Ctrl Pts',(9.36739372899994,15.2,-6.66979226100001));
#176112=CARTESIAN_POINT('Ctrl Pts',(9.36739372899994,11.6,-6.66979226100001));
#176113=CARTESIAN_POINT('Ctrl Pts',(9.36666279599994,15.2,-6.66844959700001));
#176114=CARTESIAN_POINT('Ctrl Pts',(9.36666279599994,11.6,-6.66844959700001));
#176115=CARTESIAN_POINT('Ctrl Pts',(9.36556626999994,15.2,-6.66643717600002));
#176116=CARTESIAN_POINT('Ctrl Pts',(9.36556626999994,11.6,-6.66643717600002));
#176117=CARTESIAN_POINT('Ctrl Pts',(9.36410398399994,15.2,-6.66375709800001));
#176118=CARTESIAN_POINT('Ctrl Pts',(9.36410398399994,11.6,-6.66375709800001));
#176119=CARTESIAN_POINT('Ctrl Pts',(9.36227570599995,15.2,-6.66041225100001));
#176120=CARTESIAN_POINT('Ctrl Pts',(9.36227570599995,11.6,-6.66041225100001));
#176121=CARTESIAN_POINT('Ctrl Pts',(9.36044700899994,15.2,-6.65707265500001));
#176122=CARTESIAN_POINT('Ctrl Pts',(9.36044700899994,11.6,-6.65707265500001));
#176123=CARTESIAN_POINT('Ctrl Pts',(9.35861789699995,15.2,-6.65373831100001));
#176124=CARTESIAN_POINT('Ctrl Pts',(9.35861789699995,11.6,-6.65373831100001));
#176125=CARTESIAN_POINT('Ctrl Pts',(9.35678837099994,15.2,-6.65040921900002));
#176126=CARTESIAN_POINT('Ctrl Pts',(9.35678837099994,11.6,-6.65040921900002));
#176127=CARTESIAN_POINT('Ctrl Pts',(9.35495843699995,15.2,-6.64708538300002));
#176128=CARTESIAN_POINT('Ctrl Pts',(9.35495843699995,11.6,-6.64708538300002));
#176129=CARTESIAN_POINT('Ctrl Pts',(9.35312810399994,15.2,-6.64376680700002));
#176130=CARTESIAN_POINT('Ctrl Pts',(9.35312810399994,11.6,-6.64376680700002));
#176131=CARTESIAN_POINT('Ctrl Pts',(9.35129737799994,15.2,-6.64045349300002));
#176132=CARTESIAN_POINT('Ctrl Pts',(9.35129737799994,11.6,-6.64045349300002));
#176133=CARTESIAN_POINT('Ctrl Pts',(9.34946627399994,15.2,-6.63714544600002));
#176134=CARTESIAN_POINT('Ctrl Pts',(9.34946627399994,11.6,-6.63714544600002));
#176135=CARTESIAN_POINT('Ctrl Pts',(9.34763479699994,15.2,-6.63384267000002));
#176136=CARTESIAN_POINT('Ctrl Pts',(9.34763479699994,11.6,-6.63384267000002));
#176137=CARTESIAN_POINT('Ctrl Pts',(9.34580295999995,15.2,-6.63054516900001));
#176138=CARTESIAN_POINT('Ctrl Pts',(9.34580295999995,11.6,-6.63054516900001));
#176139=CARTESIAN_POINT('Ctrl Pts',(9.34397077299994,15.2,-6.62725294900002));
#176140=CARTESIAN_POINT('Ctrl Pts',(9.34397077299994,11.6,-6.62725294900002));
#176141=CARTESIAN_POINT('Ctrl Pts',(9.34213824299994,15.2,-6.62396601100002));
#176142=CARTESIAN_POINT('Ctrl Pts',(9.34213824299994,11.6,-6.62396601100002));
#176143=CARTESIAN_POINT('Ctrl Pts',(9.34030537899995,15.2,-6.62068435900002));
#176144=CARTESIAN_POINT('Ctrl Pts',(9.34030537899995,11.6,-6.62068435900002));
#176145=CARTESIAN_POINT('Ctrl Pts',(9.33847218899994,15.2,-6.61740799700001));
#176146=CARTESIAN_POINT('Ctrl Pts',(9.33847218899994,11.6,-6.61740799700001));
#176147=CARTESIAN_POINT('Ctrl Pts',(9.33663867899994,15.2,-6.61413692800001));
#176148=CARTESIAN_POINT('Ctrl Pts',(9.33663867899994,11.6,-6.61413692800001));
#176149=CARTESIAN_POINT('Ctrl Pts',(9.33480485899995,15.2,-6.61087115400001));
#176150=CARTESIAN_POINT('Ctrl Pts',(9.33480485899995,11.6,-6.61087115400001));
#176151=CARTESIAN_POINT('Ctrl Pts',(9.33297073499994,15.2,-6.60761068000002));
#176152=CARTESIAN_POINT('Ctrl Pts',(9.33297073499994,11.6,-6.60761068000002));
#176153=CARTESIAN_POINT('Ctrl Pts',(9.33113631499995,15.2,-6.60435550800001));
#176154=CARTESIAN_POINT('Ctrl Pts',(9.33113631499995,11.6,-6.60435550800001));
#176155=CARTESIAN_POINT('Ctrl Pts',(9.32930160899994,15.2,-6.60110564200002));
#176156=CARTESIAN_POINT('Ctrl Pts',(9.32930160899994,11.6,-6.60110564200002));
#176157=CARTESIAN_POINT('Ctrl Pts',(9.32746662499994,15.2,-6.59786108500001));
#176158=CARTESIAN_POINT('Ctrl Pts',(9.32746662499994,11.6,-6.59786108500001));
#176159=CARTESIAN_POINT('Ctrl Pts',(9.32563137099994,15.2,-6.59462184300001));
#176160=CARTESIAN_POINT('Ctrl Pts',(9.32563137099994,11.6,-6.59462184300001));
#176161=CARTESIAN_POINT('Ctrl Pts',(9.32379585799995,15.2,-6.59138791600002));
#176162=CARTESIAN_POINT('Ctrl Pts',(9.32379585799995,11.6,-6.59138791600002));
#176163=CARTESIAN_POINT('Ctrl Pts',(9.32196009399994,15.2,-6.58815931000002));
#176164=CARTESIAN_POINT('Ctrl Pts',(9.32196009399994,11.6,-6.58815931000002));
#176165=CARTESIAN_POINT('Ctrl Pts',(9.32012408599994,15.2,-6.58493602700001));
#176166=CARTESIAN_POINT('Ctrl Pts',(9.32012408599994,11.6,-6.58493602700001));
#176167=CARTESIAN_POINT('Ctrl Pts',(9.31828784399995,15.2,-6.58171807200001));
#176168=CARTESIAN_POINT('Ctrl Pts',(9.31828784399995,11.6,-6.58171807200001));
#176169=CARTESIAN_POINT('Ctrl Pts',(9.31645137599994,15.2,-6.57850544700001));
#176170=CARTESIAN_POINT('Ctrl Pts',(9.31645137599994,11.6,-6.57850544700001));
#176171=CARTESIAN_POINT('Ctrl Pts',(9.31461468999995,15.2,-6.57529815700002));
#176172=CARTESIAN_POINT('Ctrl Pts',(9.31461468999995,11.6,-6.57529815700002));
#176173=CARTESIAN_POINT('Ctrl Pts',(9.31277779499995,15.2,-6.57209620300002));
#176174=CARTESIAN_POINT('Ctrl Pts',(9.31277779499995,11.6,-6.57209620300002));
#176175=CARTESIAN_POINT('Ctrl Pts',(9.31094069999994,15.2,-6.56889959000001));
#176176=CARTESIAN_POINT('Ctrl Pts',(9.31094069999994,11.6,-6.56889959000001));
#176177=CARTESIAN_POINT('Ctrl Pts',(9.30910341199995,15.2,-6.56570832200002));
#176178=CARTESIAN_POINT('Ctrl Pts',(9.30910341199995,11.6,-6.56570832200002));
#176179=CARTESIAN_POINT('Ctrl Pts',(9.30726594099994,15.2,-6.56252240200002));
#176180=CARTESIAN_POINT('Ctrl Pts',(9.30726594099994,11.6,-6.56252240200002));
#176181=CARTESIAN_POINT('Ctrl Pts',(9.30542829499995,15.2,-6.55934183200002));
#176182=CARTESIAN_POINT('Ctrl Pts',(9.30542829499995,11.6,-6.55934183200002));
#176183=CARTESIAN_POINT('Ctrl Pts',(9.30359048399995,15.2,-6.55616661700002));
#176184=CARTESIAN_POINT('Ctrl Pts',(9.30359048399995,11.6,-6.55616661700002));
#176185=CARTESIAN_POINT('Ctrl Pts',(9.30175251499995,15.2,-6.55299676000002));
#176186=CARTESIAN_POINT('Ctrl Pts',(9.30175251499995,11.6,-6.55299676000002));
#176187=CARTESIAN_POINT('Ctrl Pts',(9.29991439799995,15.2,-6.54983226400002));
#176188=CARTESIAN_POINT('Ctrl Pts',(9.29991439799995,11.6,-6.54983226400002));
#176189=CARTESIAN_POINT('Ctrl Pts',(9.29807614099994,15.2,-6.54667313400001));
#176190=CARTESIAN_POINT('Ctrl Pts',(9.29807614099994,11.6,-6.54667313400001));
#176191=CARTESIAN_POINT('Ctrl Pts',(9.29623775399994,15.2,-6.54351937200002));
#176192=CARTESIAN_POINT('Ctrl Pts',(9.29623775399994,11.6,-6.54351937200002));
#176193=CARTESIAN_POINT('Ctrl Pts',(9.29439924399994,15.2,-6.54037098200002));
#176194=CARTESIAN_POINT('Ctrl Pts',(9.29439924399994,11.6,-6.54037098200002));
#176195=CARTESIAN_POINT('Ctrl Pts',(9.29256062099994,15.2,-6.53722796600002));
#176196=CARTESIAN_POINT('Ctrl Pts',(9.29256062099994,11.6,-6.53722796600002));
#176197=CARTESIAN_POINT('Ctrl Pts',(9.29072189399994,15.2,-6.53409033000001));
#176198=CARTESIAN_POINT('Ctrl Pts',(9.29072189399994,11.6,-6.53409033000001));
#176199=CARTESIAN_POINT('Ctrl Pts',(9.28888307099994,15.2,-6.53095807600002));
#176200=CARTESIAN_POINT('Ctrl Pts',(9.28888307099994,11.6,-6.53095807600002));
#176201=CARTESIAN_POINT('Ctrl Pts',(9.28704415999994,15.2,-6.52783120700001));
#176202=CARTESIAN_POINT('Ctrl Pts',(9.28704415999994,11.6,-6.52783120700001));
#176203=CARTESIAN_POINT('Ctrl Pts',(9.28520517099994,15.2,-6.52470972700002));
#176204=CARTESIAN_POINT('Ctrl Pts',(9.28520517099994,11.6,-6.52470972700002));
#176205=CARTESIAN_POINT('Ctrl Pts',(9.28336611299994,15.2,-6.52159363900001));
#176206=CARTESIAN_POINT('Ctrl Pts',(9.28336611299994,11.6,-6.52159363900001));
#176207=CARTESIAN_POINT('Ctrl Pts',(9.28152699599995,15.2,-6.51848294700001));
#176208=CARTESIAN_POINT('Ctrl Pts',(9.28152699599995,11.6,-6.51848294700001));
#176209=CARTESIAN_POINT('Ctrl Pts',(9.27968782599994,15.2,-6.51537765500001));
#176210=CARTESIAN_POINT('Ctrl Pts',(9.27968782599994,11.6,-6.51537765500001));
#176211=CARTESIAN_POINT('Ctrl Pts',(9.27784861399994,15.2,-6.51227776500001));
#176212=CARTESIAN_POINT('Ctrl Pts',(9.27784861399994,11.6,-6.51227776500001));
#176213=CARTESIAN_POINT('Ctrl Pts',(9.27600936899994,15.2,-6.50918328100002));
#176214=CARTESIAN_POINT('Ctrl Pts',(9.27600936899994,11.6,-6.50918328100002));
#176215=CARTESIAN_POINT('Ctrl Pts',(9.27417009899994,15.2,-6.50609420700002));
#176216=CARTESIAN_POINT('Ctrl Pts',(9.27417009899994,11.6,-6.50609420700002));
#176217=CARTESIAN_POINT('Ctrl Pts',(9.27233081399994,15.2,-6.50301054500002));
#176218=CARTESIAN_POINT('Ctrl Pts',(9.27233081399994,11.6,-6.50301054500002));
#176219=CARTESIAN_POINT('Ctrl Pts',(9.27049152299994,15.2,-6.49993230000002));
#176220=CARTESIAN_POINT('Ctrl Pts',(9.27049152299994,11.6,-6.49993230000002));
#176221=CARTESIAN_POINT('Ctrl Pts',(9.26865223299994,15.2,-6.49685947500001));
#176222=CARTESIAN_POINT('Ctrl Pts',(9.26865223299994,11.6,-6.49685947500001));
#176223=CARTESIAN_POINT('Ctrl Pts',(9.26681295499994,15.2,-6.49379207200001));
#176224=CARTESIAN_POINT('Ctrl Pts',(9.26681295499994,11.6,-6.49379207200001));
#176225=CARTESIAN_POINT('Ctrl Pts',(9.26497369799995,15.2,-6.49073009700002));
#176226=CARTESIAN_POINT('Ctrl Pts',(9.26497369799995,11.6,-6.49073009700002));
#176227=CARTESIAN_POINT('Ctrl Pts',(9.26313447099995,15.2,-6.48767355100001));
#176228=CARTESIAN_POINT('Ctrl Pts',(9.26313447099995,11.6,-6.48767355100001));
#176229=CARTESIAN_POINT('Ctrl Pts',(9.26129528299995,15.2,-6.48462243900001));
#176230=CARTESIAN_POINT('Ctrl Pts',(9.26129528299995,11.6,-6.48462243900001));
#176231=CARTESIAN_POINT('Ctrl Pts',(9.25945614099994,15.2,-6.48157676400002));
#176232=CARTESIAN_POINT('Ctrl Pts',(9.25945614099994,11.6,-6.48157676400002));
#176233=CARTESIAN_POINT('Ctrl Pts',(9.25761705899994,15.2,-6.47853652900002));
#176234=CARTESIAN_POINT('Ctrl Pts',(9.25761705899994,11.6,-6.47853652900002));
#176235=CARTESIAN_POINT('Ctrl Pts',(9.25577804099994,15.2,-6.47550173700001));
#176236=CARTESIAN_POINT('Ctrl Pts',(9.25577804099994,11.6,-6.47550173700001));
#176237=CARTESIAN_POINT('Ctrl Pts',(9.25393909899995,15.2,-6.47247239300001));
#176238=CARTESIAN_POINT('Ctrl Pts',(9.25393909899995,11.6,-6.47247239300001));
#176239=CARTESIAN_POINT('Ctrl Pts',(9.25210024199994,15.2,-6.46944849900001));
#176240=CARTESIAN_POINT('Ctrl Pts',(9.25210024199994,11.6,-6.46944849900001));
#176241=CARTESIAN_POINT('Ctrl Pts',(9.25026147799995,15.2,-6.46643005900001));
#176242=CARTESIAN_POINT('Ctrl Pts',(9.25026147799995,11.6,-6.46643005900001));
#176243=CARTESIAN_POINT('Ctrl Pts',(9.24842281799994,15.2,-6.46341707500002));
#176244=CARTESIAN_POINT('Ctrl Pts',(9.24842281799994,11.6,-6.46341707500002));
#176245=CARTESIAN_POINT('Ctrl Pts',(9.24658427099994,15.2,-6.46040955400002));
#176246=CARTESIAN_POINT('Ctrl Pts',(9.24658427099994,11.6,-6.46040955400002));
#176247=CARTESIAN_POINT('Ctrl Pts',(9.24474584399994,15.2,-6.45740749500002));
#176248=CARTESIAN_POINT('Ctrl Pts',(9.24474584399994,11.6,-6.45740749500002));
#176249=CARTESIAN_POINT('Ctrl Pts',(9.24290754899994,15.2,-6.45441090500002));
#176250=CARTESIAN_POINT('Ctrl Pts',(9.24290754899994,11.6,-6.45441090500002));
#176251=CARTESIAN_POINT('Ctrl Pts',(9.24106939399995,15.2,-6.45141978400002));
#176252=CARTESIAN_POINT('Ctrl Pts',(9.24106939399995,11.6,-6.45141978400002));
#176253=CARTESIAN_POINT('Ctrl Pts',(9.23923138799994,15.2,-6.44843413900002));
#176254=CARTESIAN_POINT('Ctrl Pts',(9.23923138799994,11.6,-6.44843413900002));
#176255=CARTESIAN_POINT('Ctrl Pts',(9.23739354199994,15.2,-6.44545397100002));
#176256=CARTESIAN_POINT('Ctrl Pts',(9.23739354199994,11.6,-6.44545397100002));
#176257=CARTESIAN_POINT('Ctrl Pts',(9.23555586399995,15.2,-6.44247928500001));
#176258=CARTESIAN_POINT('Ctrl Pts',(9.23555586399995,11.6,-6.44247928500001));
#176259=CARTESIAN_POINT('Ctrl Pts',(9.23371836299994,15.2,-6.43951008200002));
#176260=CARTESIAN_POINT('Ctrl Pts',(9.23371836299994,11.6,-6.43951008200002));
#176261=CARTESIAN_POINT('Ctrl Pts',(9.23188104999995,15.2,-6.43654636700001));
#176262=CARTESIAN_POINT('Ctrl Pts',(9.23188104999995,11.6,-6.43654636700001));
#176263=CARTESIAN_POINT('Ctrl Pts',(9.23004393299994,15.2,-6.43358814300001));
#176264=CARTESIAN_POINT('Ctrl Pts',(9.23004393299994,11.6,-6.43358814300001));
#176265=CARTESIAN_POINT('Ctrl Pts',(9.22820702199994,15.2,-6.43063541500001));
#176266=CARTESIAN_POINT('Ctrl Pts',(9.22820702199994,11.6,-6.43063541500001));
#176267=CARTESIAN_POINT('Ctrl Pts',(9.22637032699994,15.2,-6.42768818500001));
#176268=CARTESIAN_POINT('Ctrl Pts',(9.22637032699994,11.6,-6.42768818500001));
#176269=CARTESIAN_POINT('Ctrl Pts',(9.22453385699994,15.2,-6.42474645400001));
#176270=CARTESIAN_POINT('Ctrl Pts',(9.22453385699994,11.6,-6.42474645400001));
#176271=CARTESIAN_POINT('Ctrl Pts',(9.22269762199995,15.2,-6.42181023000001));
#176272=CARTESIAN_POINT('Ctrl Pts',(9.22269762199995,11.6,-6.42181023000001));
#176273=CARTESIAN_POINT('Ctrl Pts',(9.22086162999994,15.2,-6.41887951300002));
#176274=CARTESIAN_POINT('Ctrl Pts',(9.22086162999994,11.6,-6.41887951300002));
#176275=CARTESIAN_POINT('Ctrl Pts',(9.21902589199994,15.2,-6.41595430800002));
#176276=CARTESIAN_POINT('Ctrl Pts',(9.21902589199994,11.6,-6.41595430800002));
#176277=CARTESIAN_POINT('Ctrl Pts',(9.21719041799994,15.2,-6.41303461800002));
#176278=CARTESIAN_POINT('Ctrl Pts',(9.21719041799994,11.6,-6.41303461800002));
#176279=CARTESIAN_POINT('Ctrl Pts',(9.21535521599994,15.2,-6.41012044600001));
#176280=CARTESIAN_POINT('Ctrl Pts',(9.21535521599994,11.6,-6.41012044600001));
#176281=CARTESIAN_POINT('Ctrl Pts',(9.21352029599994,15.2,-6.40721179700002));
#176282=CARTESIAN_POINT('Ctrl Pts',(9.21352029599994,11.6,-6.40721179700002));
#176283=CARTESIAN_POINT('Ctrl Pts',(9.21168566899994,15.2,-6.40430867100001));
#176284=CARTESIAN_POINT('Ctrl Pts',(9.21168566899994,11.6,-6.40430867100001));
#176285=CARTESIAN_POINT('Ctrl Pts',(9.20985134399994,15.2,-6.40141107500002));
#176286=CARTESIAN_POINT('Ctrl Pts',(9.20985134399994,11.6,-6.40141107500002));
#176287=CARTESIAN_POINT('Ctrl Pts',(9.20801732999994,15.2,-6.39851901000001));
#176288=CARTESIAN_POINT('Ctrl Pts',(9.20801732999994,11.6,-6.39851901000001));
#176289=CARTESIAN_POINT('Ctrl Pts',(9.20618363699995,15.2,-6.39563248100002));
#176290=CARTESIAN_POINT('Ctrl Pts',(9.20618363699995,11.6,-6.39563248100002));
#176291=CARTESIAN_POINT('Ctrl Pts',(9.20435027499994,15.2,-6.39275149000002));
#176292=CARTESIAN_POINT('Ctrl Pts',(9.20435027499994,11.6,-6.39275149000002));
#176293=CARTESIAN_POINT('Ctrl Pts',(9.20251725399994,15.2,-6.38987604000001));
#176294=CARTESIAN_POINT('Ctrl Pts',(9.20251725399994,11.6,-6.38987604000001));
#176295=CARTESIAN_POINT('Ctrl Pts',(9.20068458299994,15.2,-6.38700613600002));
#176296=CARTESIAN_POINT('Ctrl Pts',(9.20068458299994,11.6,-6.38700613600002));
#176297=CARTESIAN_POINT('Ctrl Pts',(9.19885227299994,15.2,-6.38414178100002));
#176298=CARTESIAN_POINT('Ctrl Pts',(9.19885227299994,11.6,-6.38414178100002));
#176299=CARTESIAN_POINT('Ctrl Pts',(9.19702033199994,15.2,-6.38128297800002));
#176300=CARTESIAN_POINT('Ctrl Pts',(9.19702033199994,11.6,-6.38128297800002));
#176301=CARTESIAN_POINT('Ctrl Pts',(9.19518877099994,15.2,-6.37842973000001));
#176302=CARTESIAN_POINT('Ctrl Pts',(9.19518877099994,11.6,-6.37842973000001));
#176303=CARTESIAN_POINT('Ctrl Pts',(9.19335759999995,15.2,-6.37558204000002));
#176304=CARTESIAN_POINT('Ctrl Pts',(9.19335759999995,11.6,-6.37558204000002));
#176305=CARTESIAN_POINT('Ctrl Pts',(9.19152682999994,15.2,-6.37273991300002));
#176306=CARTESIAN_POINT('Ctrl Pts',(9.19152682999994,11.6,-6.37273991300002));
#176307=CARTESIAN_POINT('Ctrl Pts',(9.18969646699994,15.2,-6.36990335200001));
#176308=CARTESIAN_POINT('Ctrl Pts',(9.18969646699994,11.6,-6.36990335200001));
#176309=CARTESIAN_POINT('Ctrl Pts',(9.18786652499995,15.2,-6.36707235900002));
#176310=CARTESIAN_POINT('Ctrl Pts',(9.18786652499995,11.6,-6.36707235900002));
#176311=CARTESIAN_POINT('Ctrl Pts',(9.18603701199994,15.2,-6.36424693700001));
#176312=CARTESIAN_POINT('Ctrl Pts',(9.18603701199994,11.6,-6.36424693700001));
#176313=CARTESIAN_POINT('Ctrl Pts',(9.18420793799994,15.2,-6.36142709300002));
#176314=CARTESIAN_POINT('Ctrl Pts',(9.18420793799994,11.6,-6.36142709300002));
#176315=CARTESIAN_POINT('Ctrl Pts',(9.18237931399995,15.2,-6.35861282700001));
#176316=CARTESIAN_POINT('Ctrl Pts',(9.18237931399995,11.6,-6.35861282700001));
#176317=CARTESIAN_POINT('Ctrl Pts',(9.18055114899994,15.2,-6.35580414200002));
#176318=CARTESIAN_POINT('Ctrl Pts',(9.18055114899994,11.6,-6.35580414200002));
#176319=CARTESIAN_POINT('Ctrl Pts',(9.17872345399994,15.2,-6.35300104400002));
#176320=CARTESIAN_POINT('Ctrl Pts',(9.17872345399994,11.6,-6.35300104400002));
#176321=CARTESIAN_POINT('Ctrl Pts',(9.17689623699994,15.2,-6.35020353500002));
#176322=CARTESIAN_POINT('Ctrl Pts',(9.17689623699994,11.6,-6.35020353500002));
#176323=CARTESIAN_POINT('Ctrl Pts',(9.17506951099995,15.2,-6.34741161800001));
#176324=CARTESIAN_POINT('Ctrl Pts',(9.17506951099995,11.6,-6.34741161800001));
#176325=CARTESIAN_POINT('Ctrl Pts',(9.17324328399994,15.2,-6.34462529700001));
#176326=CARTESIAN_POINT('Ctrl Pts',(9.17324328399994,11.6,-6.34462529700001));
#176327=CARTESIAN_POINT('Ctrl Pts',(9.17141756599994,15.2,-6.34184457400002));
#176328=CARTESIAN_POINT('Ctrl Pts',(9.17141756599994,11.6,-6.34184457400002));
#176329=CARTESIAN_POINT('Ctrl Pts',(9.16959236899995,15.2,-6.33906945400001));
#176330=CARTESIAN_POINT('Ctrl Pts',(9.16959236899995,11.6,-6.33906945400001));
#176331=CARTESIAN_POINT('Ctrl Pts',(9.16776770299995,15.2,-6.33629993900002));
#176332=CARTESIAN_POINT('Ctrl Pts',(9.16776770299995,11.6,-6.33629993900002));
#176333=CARTESIAN_POINT('Ctrl Pts',(9.16594357499994,15.2,-6.33353603400002));
#176334=CARTESIAN_POINT('Ctrl Pts',(9.16594357499994,11.6,-6.33353603400002));
#176335=CARTESIAN_POINT('Ctrl Pts',(9.16411999899994,15.2,-6.33077774000002));
#176336=CARTESIAN_POINT('Ctrl Pts',(9.16411999899994,11.6,-6.33077774000002));
#176337=CARTESIAN_POINT('Ctrl Pts',(9.16229698199994,15.2,-6.32802506300001));
#176338=CARTESIAN_POINT('Ctrl Pts',(9.16229698199994,11.6,-6.32802506300001));
#176339=CARTESIAN_POINT('Ctrl Pts',(9.16047453799994,15.2,-6.32527800400001));
#176340=CARTESIAN_POINT('Ctrl Pts',(9.16047453799994,11.6,-6.32527800400001));
#176341=CARTESIAN_POINT('Ctrl Pts',(9.15865267499994,15.2,-6.32253656800002));
#176342=CARTESIAN_POINT('Ctrl Pts',(9.15865267499994,11.6,-6.32253656800002));
#176343=CARTESIAN_POINT('Ctrl Pts',(9.15683140299994,15.2,-6.31980075800002));
#176344=CARTESIAN_POINT('Ctrl Pts',(9.15683140299994,11.6,-6.31980075800002));
#176345=CARTESIAN_POINT('Ctrl Pts',(9.15501073299994,15.2,-6.31707057600002));
#176346=CARTESIAN_POINT('Ctrl Pts',(9.15501073299994,11.6,-6.31707057600002));
#176347=CARTESIAN_POINT('Ctrl Pts',(9.15319067499994,15.2,-6.31434602700002));
#176348=CARTESIAN_POINT('Ctrl Pts',(9.15319067499994,11.6,-6.31434602700002));
#176349=CARTESIAN_POINT('Ctrl Pts',(9.15137123999994,15.2,-6.31162711400002));
#176350=CARTESIAN_POINT('Ctrl Pts',(9.15137123999994,11.6,-6.31162711400002));
#176351=CARTESIAN_POINT('Ctrl Pts',(9.14955243799995,15.2,-6.30891384000002));
#176352=CARTESIAN_POINT('Ctrl Pts',(9.14955243799995,11.6,-6.30891384000002));
#176353=CARTESIAN_POINT('Ctrl Pts',(9.14773427999994,15.2,-6.30620620700002));
#176354=CARTESIAN_POINT('Ctrl Pts',(9.14773427999994,11.6,-6.30620620700002));
#176355=CARTESIAN_POINT('Ctrl Pts',(9.14591677499994,15.2,-6.30350422100002));
#176356=CARTESIAN_POINT('Ctrl Pts',(9.14591677499994,11.6,-6.30350422100002));
#176357=CARTESIAN_POINT('Ctrl Pts',(9.14409993499994,15.2,-6.30080788400001));
#176358=CARTESIAN_POINT('Ctrl Pts',(9.14409993499994,11.6,-6.30080788400001));
#176359=CARTESIAN_POINT('Ctrl Pts',(9.14228376999995,15.2,-6.29811719800002));
#176360=CARTESIAN_POINT('Ctrl Pts',(9.14228376999995,11.6,-6.29811719800002));
#176361=CARTESIAN_POINT('Ctrl Pts',(9.14046828999994,15.2,-6.29543216900001));
#176362=CARTESIAN_POINT('Ctrl Pts',(9.14046828999994,11.6,-6.29543216900001));
#176363=CARTESIAN_POINT('Ctrl Pts',(9.13865350699994,15.2,-6.29275279900002));
#176364=CARTESIAN_POINT('Ctrl Pts',(9.13865350699994,11.6,-6.29275279900002));
#176365=CARTESIAN_POINT('Ctrl Pts',(9.13683942899995,15.2,-6.29007909000002));
#176366=CARTESIAN_POINT('Ctrl Pts',(9.13683942899995,11.6,-6.29007909000002));
#176367=CARTESIAN_POINT('Ctrl Pts',(9.13502606899995,15.2,-6.28741104800002));
#176368=CARTESIAN_POINT('Ctrl Pts',(9.13502606899995,11.6,-6.28741104800002));
#176369=CARTESIAN_POINT('Ctrl Pts',(9.13321343699995,15.2,-6.28474867500002));
#176370=CARTESIAN_POINT('Ctrl Pts',(9.13321343699995,11.6,-6.28474867500002));
#176371=CARTESIAN_POINT('Ctrl Pts',(9.13140154299995,15.2,-6.28209197300002));
#176372=CARTESIAN_POINT('Ctrl Pts',(9.13140154299995,11.6,-6.28209197300002));
#176373=CARTESIAN_POINT('Ctrl Pts',(9.12959039799994,15.2,-6.27944094700001));
#176374=CARTESIAN_POINT('Ctrl Pts',(9.12959039799994,11.6,-6.27944094700001));
#176375=CARTESIAN_POINT('Ctrl Pts',(9.12778001299994,15.2,-6.27679560000002));
#176376=CARTESIAN_POINT('Ctrl Pts',(9.12778001299994,11.6,-6.27679560000002));
#176377=CARTESIAN_POINT('Ctrl Pts',(9.12597039799994,15.2,-6.27415593400002));
#176378=CARTESIAN_POINT('Ctrl Pts',(9.12597039799994,11.6,-6.27415593400002));
#176379=CARTESIAN_POINT('Ctrl Pts',(9.12416156499994,15.2,-6.27152195500001));
#176380=CARTESIAN_POINT('Ctrl Pts',(9.12416156499994,11.6,-6.27152195500001));
#176381=CARTESIAN_POINT('Ctrl Pts',(9.12235352399994,15.2,-6.26889366400002));
#176382=CARTESIAN_POINT('Ctrl Pts',(9.12235352399994,11.6,-6.26889366400002));
#176383=CARTESIAN_POINT('Ctrl Pts',(9.12054628499994,15.2,-6.26627106500001));
#176384=CARTESIAN_POINT('Ctrl Pts',(9.12054628499994,11.6,-6.26627106500001));
#176385=CARTESIAN_POINT('Ctrl Pts',(9.11873985999994,15.2,-6.26365416200001));
#176386=CARTESIAN_POINT('Ctrl Pts',(9.11873985999994,11.6,-6.26365416200001));
#176387=CARTESIAN_POINT('Ctrl Pts',(9.11693425999994,15.2,-6.26104295700002));
#176388=CARTESIAN_POINT('Ctrl Pts',(9.11693425999994,11.6,-6.26104295700002));
#176389=CARTESIAN_POINT('Ctrl Pts',(9.11512949499994,15.2,-6.25843745400001));
#176390=CARTESIAN_POINT('Ctrl Pts',(9.11512949499994,11.6,-6.25843745400001));
#176391=CARTESIAN_POINT('Ctrl Pts',(9.11332557599994,15.2,-6.25583765700001));
#176392=CARTESIAN_POINT('Ctrl Pts',(9.11332557599994,11.6,-6.25583765700001));
#176393=CARTESIAN_POINT('Ctrl Pts',(9.11152251499994,15.2,-6.25324356700002));
#176394=CARTESIAN_POINT('Ctrl Pts',(9.11152251499994,11.6,-6.25324356700002));
#176395=CARTESIAN_POINT('Ctrl Pts',(9.10972032099994,15.2,-6.25065519100002));
#176396=CARTESIAN_POINT('Ctrl Pts',(9.10972032099994,11.6,-6.25065519100002));
#176397=CARTESIAN_POINT('Ctrl Pts',(9.10791900599994,15.2,-6.24807252900001));
#176398=CARTESIAN_POINT('Ctrl Pts',(9.10791900599994,11.6,-6.24807252900001));
#176399=CARTESIAN_POINT('Ctrl Pts',(9.10611858299994,15.2,-6.24549558500001));
#176400=CARTESIAN_POINT('Ctrl Pts',(9.10611858299994,11.6,-6.24549558500001));
#176401=CARTESIAN_POINT('Ctrl Pts',(9.10431905899994,15.2,-6.24292436300002));
#176402=CARTESIAN_POINT('Ctrl Pts',(9.10431905899994,11.6,-6.24292436300002));
#176403=CARTESIAN_POINT('Ctrl Pts',(9.10252044799994,15.2,-6.24035886600002));
#176404=CARTESIAN_POINT('Ctrl Pts',(9.10252044799994,11.6,-6.24035886600002));
#176405=CARTESIAN_POINT('Ctrl Pts',(9.10072275999994,15.2,-6.23779909700002));
#176406=CARTESIAN_POINT('Ctrl Pts',(9.10072275999994,11.6,-6.23779909700002));
#176407=CARTESIAN_POINT('Ctrl Pts',(9.09892600699994,15.2,-6.23524506100001));
#176408=CARTESIAN_POINT('Ctrl Pts',(9.09892600699994,11.6,-6.23524506100001));
#176409=CARTESIAN_POINT('Ctrl Pts',(9.09713019799994,15.2,-6.23269675900002));
#176410=CARTESIAN_POINT('Ctrl Pts',(9.09713019799994,11.6,-6.23269675900002));
#176411=CARTESIAN_POINT('Ctrl Pts',(9.09533534799994,15.2,-6.23015419500001));
#176412=CARTESIAN_POINT('Ctrl Pts',(9.09533534799994,11.6,-6.23015419500001));
#176413=CARTESIAN_POINT('Ctrl Pts',(9.09354146399994,15.2,-6.22761737200002));
#176414=CARTESIAN_POINT('Ctrl Pts',(9.09354146399994,11.6,-6.22761737200002));
#176415=CARTESIAN_POINT('Ctrl Pts',(9.09174855899994,15.2,-6.22508629400001));
#176416=CARTESIAN_POINT('Ctrl Pts',(9.09174855899994,11.6,-6.22508629400001));
#176417=CARTESIAN_POINT('Ctrl Pts',(9.08995664499994,15.2,-6.22256096500001));
#176418=CARTESIAN_POINT('Ctrl Pts',(9.08995664499994,11.6,-6.22256096500001));
#176419=CARTESIAN_POINT('Ctrl Pts',(9.08816573199994,15.2,-6.22004138600002));
#176420=CARTESIAN_POINT('Ctrl Pts',(9.08816573199994,11.6,-6.22004138600002));
#176421=CARTESIAN_POINT('Ctrl Pts',(9.08637583199994,15.2,-6.21752756200002));
#176422=CARTESIAN_POINT('Ctrl Pts',(9.08637583199994,11.6,-6.21752756200002));
#176423=CARTESIAN_POINT('Ctrl Pts',(9.08458695599995,15.2,-6.21501949500002));
#176424=CARTESIAN_POINT('Ctrl Pts',(9.08458695599995,11.6,-6.21501949500002));
#176425=CARTESIAN_POINT('Ctrl Pts',(9.08279911599994,15.2,-6.21251719000002));
#176426=CARTESIAN_POINT('Ctrl Pts',(9.08279911599994,11.6,-6.21251719000002));
#176427=CARTESIAN_POINT('Ctrl Pts',(9.08101232199994,15.2,-6.21002065000001));
#176428=CARTESIAN_POINT('Ctrl Pts',(9.08101232199994,11.6,-6.21002065000001));
#176429=CARTESIAN_POINT('Ctrl Pts',(9.07922658799994,15.2,-6.20752987600002));
#176430=CARTESIAN_POINT('Ctrl Pts',(9.07922658799994,11.6,-6.20752987600002));
#176431=CARTESIAN_POINT('Ctrl Pts',(9.07744192199995,15.2,-6.20504487400002));
#176432=CARTESIAN_POINT('Ctrl Pts',(9.07744192199995,11.6,-6.20504487400002));
#176433=CARTESIAN_POINT('Ctrl Pts',(9.07565833799995,15.2,-6.20256564500002));
#176434=CARTESIAN_POINT('Ctrl Pts',(9.07565833799995,11.6,-6.20256564500002));
#176435=CARTESIAN_POINT('Ctrl Pts',(9.07387584499994,15.2,-6.20009219400002));
#176436=CARTESIAN_POINT('Ctrl Pts',(9.07387584499994,11.6,-6.20009219400002));
#176437=CARTESIAN_POINT('Ctrl Pts',(9.07209445899994,15.2,-6.19762452400002));
#176438=CARTESIAN_POINT('Ctrl Pts',(9.07209445899994,11.6,-6.19762452400002));
#176439=CARTESIAN_POINT('Ctrl Pts',(9.07031418699994,15.2,-6.19516263800002));
#176440=CARTESIAN_POINT('Ctrl Pts',(9.07031418699994,11.6,-6.19516263800002));
#176441=CARTESIAN_POINT('Ctrl Pts',(9.06853504099994,15.2,-6.19270653800001));
#176442=CARTESIAN_POINT('Ctrl Pts',(9.06853504099994,11.6,-6.19270653800001));
#176443=CARTESIAN_POINT('Ctrl Pts',(9.06675703599995,15.2,-6.19025623000002));
#176444=CARTESIAN_POINT('Ctrl Pts',(9.06675703599995,11.6,-6.19025623000002));
#176445=CARTESIAN_POINT('Ctrl Pts',(9.06498018099994,15.2,-6.18781171400002));
#176446=CARTESIAN_POINT('Ctrl Pts',(9.06498018099994,11.6,-6.18781171400002));
#176447=CARTESIAN_POINT('Ctrl Pts',(9.06320448699995,15.2,-6.18537299700002));
#176448=CARTESIAN_POINT('Ctrl Pts',(9.06320448699995,11.6,-6.18537299700002));
#176449=CARTESIAN_POINT('Ctrl Pts',(9.06142996799994,15.2,-6.18294007900002));
#176450=CARTESIAN_POINT('Ctrl Pts',(9.06142996799994,11.6,-6.18294007900002));
#176451=CARTESIAN_POINT('Ctrl Pts',(9.05965663399994,15.2,-6.18051296400001));
#176452=CARTESIAN_POINT('Ctrl Pts',(9.05965663399994,11.6,-6.18051296400001));
#176453=CARTESIAN_POINT('Ctrl Pts',(9.05788449699994,15.2,-6.17809165700002));
#176454=CARTESIAN_POINT('Ctrl Pts',(9.05788449699994,11.6,-6.17809165700002));
#176455=CARTESIAN_POINT('Ctrl Pts',(9.05611356899995,15.2,-6.17567615900001));
#176456=CARTESIAN_POINT('Ctrl Pts',(9.05611356899995,11.6,-6.17567615900001));
#176457=CARTESIAN_POINT('Ctrl Pts',(9.05434386299994,15.2,-6.17326647400001));
#176458=CARTESIAN_POINT('Ctrl Pts',(9.05434386299994,11.6,-6.17326647400001));
#176459=CARTESIAN_POINT('Ctrl Pts',(9.05257538899994,15.2,-6.17086260600002));
#176460=CARTESIAN_POINT('Ctrl Pts',(9.05257538899994,11.6,-6.17086260600002));
#176461=CARTESIAN_POINT('Ctrl Pts',(9.05080815899994,15.2,-6.16846455700002));
#176462=CARTESIAN_POINT('Ctrl Pts',(9.05080815899994,11.6,-6.16846455700002));
#176463=CARTESIAN_POINT('Ctrl Pts',(9.04904218599994,15.2,-6.16607233100002));
#176464=CARTESIAN_POINT('Ctrl Pts',(9.04904218599994,11.6,-6.16607233100002));
#176465=CARTESIAN_POINT('Ctrl Pts',(9.04727748099994,15.2,-6.16368593200002));
#176466=CARTESIAN_POINT('Ctrl Pts',(9.04727748099994,11.6,-6.16368593200002));
#176467=CARTESIAN_POINT('Ctrl Pts',(9.04551405599994,15.2,-6.16130536200002));
#176468=CARTESIAN_POINT('Ctrl Pts',(9.04551405599994,11.6,-6.16130536200002));
#176469=CARTESIAN_POINT('Ctrl Pts',(9.04375192399994,15.2,-6.15893062400002));
#176470=CARTESIAN_POINT('Ctrl Pts',(9.04375192399994,11.6,-6.15893062400002));
#176471=CARTESIAN_POINT('Ctrl Pts',(9.04199109499995,15.2,-6.15656172200002));
#176472=CARTESIAN_POINT('Ctrl Pts',(9.04199109499995,11.6,-6.15656172200002));
#176473=CARTESIAN_POINT('Ctrl Pts',(9.04023158399994,15.2,-6.15419865900002));
#176474=CARTESIAN_POINT('Ctrl Pts',(9.04023158399994,11.6,-6.15419865900002));
#176475=CARTESIAN_POINT('Ctrl Pts',(9.03847339899994,15.2,-6.15184143900001));
#176476=CARTESIAN_POINT('Ctrl Pts',(9.03847339899994,11.6,-6.15184143900001));
#176477=CARTESIAN_POINT('Ctrl Pts',(9.03671655699995,15.2,-6.14949006400002));
#176478=CARTESIAN_POINT('Ctrl Pts',(9.03671655699995,11.6,-6.14949006400002));
#176479=CARTESIAN_POINT('Ctrl Pts',(9.03496106599994,15.2,-6.14714453800002));
#176480=CARTESIAN_POINT('Ctrl Pts',(9.03496106599994,11.6,-6.14714453800002));
#176481=CARTESIAN_POINT('Ctrl Pts',(9.03320693999994,15.2,-6.14480486300002));
#176482=CARTESIAN_POINT('Ctrl Pts',(9.03320693999994,11.6,-6.14480486300002));
#176483=CARTESIAN_POINT('Ctrl Pts',(9.03145419199994,15.2,-6.14247104400001));
#176484=CARTESIAN_POINT('Ctrl Pts',(9.03145419199994,11.6,-6.14247104400001));
#176485=CARTESIAN_POINT('Ctrl Pts',(9.02970283099994,15.2,-6.14014308300002));
#176486=CARTESIAN_POINT('Ctrl Pts',(9.02970283099994,11.6,-6.14014308300002));
#176487=CARTESIAN_POINT('Ctrl Pts',(9.02795287299995,15.2,-6.13782098500002));
#176488=CARTESIAN_POINT('Ctrl Pts',(9.02795287299995,11.6,-6.13782098500002));
#176489=CARTESIAN_POINT('Ctrl Pts',(9.02620432799995,15.2,-6.13550475000002));
#176490=CARTESIAN_POINT('Ctrl Pts',(9.02620432799995,11.6,-6.13550475000002));
#176491=CARTESIAN_POINT('Ctrl Pts',(9.02445720899994,15.2,-6.13319438400002));
#176492=CARTESIAN_POINT('Ctrl Pts',(9.02445720899994,11.6,-6.13319438400002));
#176493=CARTESIAN_POINT('Ctrl Pts',(9.02271152799995,15.2,-6.13088988900002));
#176494=CARTESIAN_POINT('Ctrl Pts',(9.02271152799995,11.6,-6.13088988900002));
#176495=CARTESIAN_POINT('Ctrl Pts',(9.02096729899995,15.2,-6.12859126900001));
#176496=CARTESIAN_POINT('Ctrl Pts',(9.02096729899995,11.6,-6.12859126900001));
#176497=CARTESIAN_POINT('Ctrl Pts',(9.01922453199994,15.2,-6.12629852600002));
#176498=CARTESIAN_POINT('Ctrl Pts',(9.01922453199994,11.6,-6.12629852600002));
#176499=CARTESIAN_POINT('Ctrl Pts',(9.01748323999995,15.2,-6.12401166400002));
#176500=CARTESIAN_POINT('Ctrl Pts',(9.01748323999995,11.6,-6.12401166400002));
#176501=CARTESIAN_POINT('Ctrl Pts',(9.01574343699994,15.2,-6.12173068600002));
#176502=CARTESIAN_POINT('Ctrl Pts',(9.01574343699994,11.6,-6.12173068600002));
#176503=CARTESIAN_POINT('Ctrl Pts',(9.01400513499994,15.2,-6.11945559600001));
#176504=CARTESIAN_POINT('Ctrl Pts',(9.01400513499994,11.6,-6.11945559600001));
#176505=CARTESIAN_POINT('Ctrl Pts',(9.01226834599994,15.2,-6.11718639600002));
#176506=CARTESIAN_POINT('Ctrl Pts',(9.01226834599994,11.6,-6.11718639600002));
#176507=CARTESIAN_POINT('Ctrl Pts',(9.01053308099995,15.2,-6.11492308900001));
#176508=CARTESIAN_POINT('Ctrl Pts',(9.01053308099995,11.6,-6.11492308900001));
#176509=CARTESIAN_POINT('Ctrl Pts',(9.00879935499994,15.2,-6.11266568000002));
#176510=CARTESIAN_POINT('Ctrl Pts',(9.00879935499994,11.6,-6.11266568000002));
#176511=CARTESIAN_POINT('Ctrl Pts',(9.00706718099994,15.2,-6.11041417100001));
#176512=CARTESIAN_POINT('Ctrl Pts',(9.00706718099994,11.6,-6.11041417100001));
#176513=CARTESIAN_POINT('Ctrl Pts',(9.00533656799994,15.2,-6.10816856500002));
#176514=CARTESIAN_POINT('Ctrl Pts',(9.00533656799994,11.6,-6.10816856500002));
#176515=CARTESIAN_POINT('Ctrl Pts',(9.00360753399994,15.2,-6.10592886600001));
#176516=CARTESIAN_POINT('Ctrl Pts',(9.00360753399994,11.6,-6.10592886600001));
#176517=CARTESIAN_POINT('Ctrl Pts',(9.00188008699994,15.2,-6.10369507500002));
#176518=CARTESIAN_POINT('Ctrl Pts',(9.00188008699994,11.6,-6.10369507500002));
#176519=CARTESIAN_POINT('Ctrl Pts',(9.00015424299994,15.2,-6.10146719900002));
#176520=CARTESIAN_POINT('Ctrl Pts',(9.00015424299994,11.6,-6.10146719900002));
#176521=CARTESIAN_POINT('Ctrl Pts',(8.99843001299995,15.2,-6.09924523800002));
#176522=CARTESIAN_POINT('Ctrl Pts',(8.99843001299995,11.6,-6.09924523800002));
#176523=CARTESIAN_POINT('Ctrl Pts',(8.99670740999994,15.2,-6.09702919700001));
#176524=CARTESIAN_POINT('Ctrl Pts',(8.99670740999994,11.6,-6.09702919700001));
#176525=CARTESIAN_POINT('Ctrl Pts',(8.99498644699994,15.2,-6.09481907700002));
#176526=CARTESIAN_POINT('Ctrl Pts',(8.99498644699994,11.6,-6.09481907700002));
#176527=CARTESIAN_POINT('Ctrl Pts',(8.99326713699995,15.2,-6.09261488300002));
#176528=CARTESIAN_POINT('Ctrl Pts',(8.99326713699995,11.6,-6.09261488300002));
#176529=CARTESIAN_POINT('Ctrl Pts',(8.99154949399994,15.2,-6.09041661900001));
#176530=CARTESIAN_POINT('Ctrl Pts',(8.99154949399994,11.6,-6.09041661900001));
#176531=CARTESIAN_POINT('Ctrl Pts',(8.98983352999995,15.2,-6.08822428600002));
#176532=CARTESIAN_POINT('Ctrl Pts',(8.98983352999995,11.6,-6.08822428600002));
#176533=CARTESIAN_POINT('Ctrl Pts',(8.98811925699994,15.2,-6.08603788900002));
#176534=CARTESIAN_POINT('Ctrl Pts',(8.98811925699994,11.6,-6.08603788900002));
#176535=CARTESIAN_POINT('Ctrl Pts',(8.98640668999995,15.2,-6.08385743000002));
#176536=CARTESIAN_POINT('Ctrl Pts',(8.98640668999995,11.6,-6.08385743000002));
#176537=CARTESIAN_POINT('Ctrl Pts',(8.98469584099994,15.2,-6.08168291200001));
#176538=CARTESIAN_POINT('Ctrl Pts',(8.98469584099994,11.6,-6.08168291200001));
#176539=CARTESIAN_POINT('Ctrl Pts',(8.98298672299994,15.2,-6.07951433900002));
#176540=CARTESIAN_POINT('Ctrl Pts',(8.98298672299994,11.6,-6.07951433900002));
#176541=CARTESIAN_POINT('Ctrl Pts',(8.98127934999994,15.2,-6.07735171400002));
#176542=CARTESIAN_POINT('Ctrl Pts',(8.98127934999994,11.6,-6.07735171400002));
#176543=CARTESIAN_POINT('Ctrl Pts',(8.97957373299995,15.2,-6.07519503900001));
#176544=CARTESIAN_POINT('Ctrl Pts',(8.97957373299995,11.6,-6.07519503900001));
#176545=CARTESIAN_POINT('Ctrl Pts',(8.97786988799995,15.2,-6.07304431900002));
#176546=CARTESIAN_POINT('Ctrl Pts',(8.97786988799995,11.6,-6.07304431900002));
#176547=CARTESIAN_POINT('Ctrl Pts',(8.97616782599994,15.2,-6.07089955700002));
#176548=CARTESIAN_POINT('Ctrl Pts',(8.97616782599994,11.6,-6.07089955700002));
#176549=CARTESIAN_POINT('Ctrl Pts',(8.97446756199994,15.2,-6.06876075400002));
#176550=CARTESIAN_POINT('Ctrl Pts',(8.97446756199994,11.6,-6.06876075400002));
#176551=CARTESIAN_POINT('Ctrl Pts',(8.97276910899994,15.2,-6.06662791500002));
#176552=CARTESIAN_POINT('Ctrl Pts',(8.97276910899994,11.6,-6.06662791500002));
#176553=CARTESIAN_POINT('Ctrl Pts',(8.97107247999994,15.2,-6.06450104300002));
#176554=CARTESIAN_POINT('Ctrl Pts',(8.97107247999994,11.6,-6.06450104300002));
#176555=CARTESIAN_POINT('Ctrl Pts',(8.96937768699994,15.2,-6.06238014200001));
#176556=CARTESIAN_POINT('Ctrl Pts',(8.96937768699994,11.6,-6.06238014200001));
#176557=CARTESIAN_POINT('Ctrl Pts',(8.96768474699994,15.2,-6.06026521400001));
#176558=CARTESIAN_POINT('Ctrl Pts',(8.96768474699994,11.6,-6.06026521400001));
#176559=CARTESIAN_POINT('Ctrl Pts',(8.96599366899994,15.2,-6.05815626100001));
#176560=CARTESIAN_POINT('Ctrl Pts',(8.96599366899994,11.6,-6.05815626100001));
#176561=CARTESIAN_POINT('Ctrl Pts',(8.96430446999995,15.2,-6.05605328800002));
#176562=CARTESIAN_POINT('Ctrl Pts',(8.96430446999995,11.6,-6.05605328800002));
#176563=CARTESIAN_POINT('Ctrl Pts',(8.96261716099995,15.2,-6.05395629800002));
#176564=CARTESIAN_POINT('Ctrl Pts',(8.96261716099995,11.6,-6.05395629800002));
#176565=CARTESIAN_POINT('Ctrl Pts',(8.96093175899994,15.2,-6.05186529300001));
#176566=CARTESIAN_POINT('Ctrl Pts',(8.96093175899994,11.6,-6.05186529300001));
#176567=CARTESIAN_POINT('Ctrl Pts',(8.95924827399995,15.2,-6.04978027700002));
#176568=CARTESIAN_POINT('Ctrl Pts',(8.95924827399995,11.6,-6.04978027700002));
#176569=CARTESIAN_POINT('Ctrl Pts',(8.95756672099994,15.2,-6.04770125400002));
#176570=CARTESIAN_POINT('Ctrl Pts',(8.95756672099994,11.6,-6.04770125400002));
#176571=CARTESIAN_POINT('Ctrl Pts',(8.95588711299995,15.2,-6.04562822500001));
#176572=CARTESIAN_POINT('Ctrl Pts',(8.95588711299995,11.6,-6.04562822500001));
#176573=CARTESIAN_POINT('Ctrl Pts',(8.95420946599994,15.2,-6.04356119500002));
#176574=CARTESIAN_POINT('Ctrl Pts',(8.95420946599994,11.6,-6.04356119500002));
#176575=CARTESIAN_POINT('Ctrl Pts',(8.95253379199995,15.2,-6.04150016600002));
#176576=CARTESIAN_POINT('Ctrl Pts',(8.95253379199995,11.6,-6.04150016600002));
#176577=CARTESIAN_POINT('Ctrl Pts',(8.95086010499995,15.2,-6.03944514200002));
#176578=CARTESIAN_POINT('Ctrl Pts',(8.95086010499995,11.6,-6.03944514200002));
#176579=CARTESIAN_POINT('Ctrl Pts',(8.94918841899995,15.2,-6.03739612600001));
#176580=CARTESIAN_POINT('Ctrl Pts',(8.94918841899995,11.6,-6.03739612600001));
#176581=CARTESIAN_POINT('Ctrl Pts',(8.94751874699995,15.2,-6.03535312000002));
#176582=CARTESIAN_POINT('Ctrl Pts',(8.94751874699995,11.6,-6.03535312000002));
#176583=CARTESIAN_POINT('Ctrl Pts',(8.94585110499994,15.2,-6.03331612800002));
#176584=CARTESIAN_POINT('Ctrl Pts',(8.94585110499994,11.6,-6.03331612800002));
#176585=CARTESIAN_POINT('Ctrl Pts',(8.94418550499994,15.2,-6.03128515400002));
#176586=CARTESIAN_POINT('Ctrl Pts',(8.94418550499994,11.6,-6.03128515400002));
#176587=CARTESIAN_POINT('Ctrl Pts',(8.94252196199995,15.2,-6.02926020000002));
#176588=CARTESIAN_POINT('Ctrl Pts',(8.94252196199995,11.6,-6.02926020000002));
#176589=CARTESIAN_POINT('Ctrl Pts',(8.94086048799995,15.2,-6.02724126900001));
#176590=CARTESIAN_POINT('Ctrl Pts',(8.94086048799995,11.6,-6.02724126900001));
#176591=CARTESIAN_POINT('Ctrl Pts',(8.93920109999994,15.2,-6.02522836400002));
#176592=CARTESIAN_POINT('Ctrl Pts',(8.93920109999994,11.6,-6.02522836400002));
#176593=CARTESIAN_POINT('Ctrl Pts',(8.93754381099994,15.2,-6.02322149000001));
#176594=CARTESIAN_POINT('Ctrl Pts',(8.93754381099994,11.6,-6.02322149000001));
#176595=CARTESIAN_POINT('Ctrl Pts',(8.93588863499994,15.2,-6.02122064700002));
#176596=CARTESIAN_POINT('Ctrl Pts',(8.93588863499994,11.6,-6.02122064700002));
#176597=CARTESIAN_POINT('Ctrl Pts',(8.93423558499994,15.2,-6.01922584200001));
#176598=CARTESIAN_POINT('Ctrl Pts',(8.93423558499994,11.6,-6.01922584200001));
#176599=CARTESIAN_POINT('Ctrl Pts',(8.93258467799994,15.2,-6.01723707400001));
#176600=CARTESIAN_POINT('Ctrl Pts',(8.93258467799994,11.6,-6.01723707400001));
#176601=CARTESIAN_POINT('Ctrl Pts',(8.93093592599995,15.2,-6.01525434800001));
#176602=CARTESIAN_POINT('Ctrl Pts',(8.93093592599995,11.6,-6.01525434800001));
#176603=CARTESIAN_POINT('Ctrl Pts',(8.92928934299994,15.2,-6.01327766800001));
#176604=CARTESIAN_POINT('Ctrl Pts',(8.92928934299994,11.6,-6.01327766800001));
#176605=CARTESIAN_POINT('Ctrl Pts',(8.92764494599994,15.2,-6.01130703600001));
#176606=CARTESIAN_POINT('Ctrl Pts',(8.92764494599994,11.6,-6.01130703600001));
#176607=CARTESIAN_POINT('Ctrl Pts',(8.92600274799995,15.2,-6.00934245600002));
#176608=CARTESIAN_POINT('Ctrl Pts',(8.92600274799995,11.6,-6.00934245600002));
#176609=CARTESIAN_POINT('Ctrl Pts',(8.92436276099994,15.2,-6.00738393100002));
#176610=CARTESIAN_POINT('Ctrl Pts',(8.92436276099994,11.6,-6.00738393100002));
#176611=CARTESIAN_POINT('Ctrl Pts',(8.92272500299994,15.2,-6.00543146300001));
#176612=CARTESIAN_POINT('Ctrl Pts',(8.92272500299994,11.6,-6.00543146300001));
#176613=CARTESIAN_POINT('Ctrl Pts',(8.92108948699994,15.2,-6.00348505400002));
#176614=CARTESIAN_POINT('Ctrl Pts',(8.92108948699994,11.6,-6.00348505400002));
#176615=CARTESIAN_POINT('Ctrl Pts',(8.91945622699994,15.2,-6.00154471100002));
#176616=CARTESIAN_POINT('Ctrl Pts',(8.91945622699994,11.6,-6.00154471100002));
#176617=CARTESIAN_POINT('Ctrl Pts',(8.91782523999994,15.2,-5.99961043300001));
#176618=CARTESIAN_POINT('Ctrl Pts',(8.91782523999994,11.6,-5.99961043300001));
#176619=CARTESIAN_POINT('Ctrl Pts',(8.91619653799994,15.2,-5.99768222700002));
#176620=CARTESIAN_POINT('Ctrl Pts',(8.91619653799994,11.6,-5.99768222700002));
#176621=CARTESIAN_POINT('Ctrl Pts',(8.91457013499994,15.2,-5.99576009400002));
#176622=CARTESIAN_POINT('Ctrl Pts',(8.91457013499994,11.6,-5.99576009400002));
#176623=CARTESIAN_POINT('Ctrl Pts',(8.91294604899995,15.2,-5.99384403500002));
#176624=CARTESIAN_POINT('Ctrl Pts',(8.91294604899995,11.6,-5.99384403500002));
#176625=CARTESIAN_POINT('Ctrl Pts',(8.91132429299994,15.2,-5.99193405800002));
#176626=CARTESIAN_POINT('Ctrl Pts',(8.91132429299994,11.6,-5.99193405800002));
#176627=CARTESIAN_POINT('Ctrl Pts',(8.90970488099994,15.2,-5.99003016200002));
#176628=CARTESIAN_POINT('Ctrl Pts',(8.90970488099994,11.6,-5.99003016200002));
#176629=CARTESIAN_POINT('Ctrl Pts',(8.90808782999994,15.2,-5.98813235200002));
#176630=CARTESIAN_POINT('Ctrl Pts',(8.90808782999994,11.6,-5.98813235200002));
#176631=CARTESIAN_POINT('Ctrl Pts',(8.90647315299995,15.2,-5.98624063000001));
#176632=CARTESIAN_POINT('Ctrl Pts',(8.90647315299995,11.6,-5.98624063000001));
#176633=CARTESIAN_POINT('Ctrl Pts',(8.90486086599994,15.2,-5.98435499900001));
#176634=CARTESIAN_POINT('Ctrl Pts',(8.90486086599994,11.6,-5.98435499900001));
#176635=CARTESIAN_POINT('Ctrl Pts',(8.90325098299994,15.2,-5.98247546400002));
#176636=CARTESIAN_POINT('Ctrl Pts',(8.90325098299994,11.6,-5.98247546400002));
#176637=CARTESIAN_POINT('Ctrl Pts',(8.90164351899994,15.2,-5.98060202600001));
#176638=CARTESIAN_POINT('Ctrl Pts',(8.90164351899994,11.6,-5.98060202600001));
#176639=CARTESIAN_POINT('Ctrl Pts',(8.90003849099994,15.2,-5.97873468800002));
#176640=CARTESIAN_POINT('Ctrl Pts',(8.90003849099994,11.6,-5.97873468800002));
#176641=CARTESIAN_POINT('Ctrl Pts',(8.89843591199994,15.2,-5.97687345600002));
#176642=CARTESIAN_POINT('Ctrl Pts',(8.89843591199994,11.6,-5.97687345600002));
#176643=CARTESIAN_POINT('Ctrl Pts',(8.89683579899994,15.2,-5.97501833000001));
#176644=CARTESIAN_POINT('Ctrl Pts',(8.89683579899994,11.6,-5.97501833000001));
#176645=CARTESIAN_POINT('Ctrl Pts',(8.89523816499995,15.2,-5.97316931300002));
#176646=CARTESIAN_POINT('Ctrl Pts',(8.89523816499995,11.6,-5.97316931300002));
#176647=CARTESIAN_POINT('Ctrl Pts',(8.89364302699994,15.2,-5.97132641100002));
#176648=CARTESIAN_POINT('Ctrl Pts',(8.89364302699994,11.6,-5.97132641100002));
#176649=CARTESIAN_POINT('Ctrl Pts',(8.89205039799995,15.2,-5.96948962400001));
#176650=CARTESIAN_POINT('Ctrl Pts',(8.89205039799995,11.6,-5.96948962400001));
#176651=CARTESIAN_POINT('Ctrl Pts',(8.89046029699994,15.2,-5.96765895700001));
#176652=CARTESIAN_POINT('Ctrl Pts',(8.89046029699994,11.6,-5.96765895700001));
#176653=CARTESIAN_POINT('Ctrl Pts',(8.88887273699994,15.2,-5.96583441200002));
#176654=CARTESIAN_POINT('Ctrl Pts',(8.88887273699994,11.6,-5.96583441200002));
#176655=CARTESIAN_POINT('Ctrl Pts',(8.88728773299994,15.2,-5.96401599200002));
#176656=CARTESIAN_POINT('Ctrl Pts',(8.88728773299994,11.6,-5.96401599200002));
#176657=CARTESIAN_POINT('Ctrl Pts',(8.88570530199994,15.2,-5.96220370100002));
#176658=CARTESIAN_POINT('Ctrl Pts',(8.88570530199994,11.6,-5.96220370100002));
#176659=CARTESIAN_POINT('Ctrl Pts',(8.88412545799994,15.2,-5.96039754200002));
#176660=CARTESIAN_POINT('Ctrl Pts',(8.88412545799994,11.6,-5.96039754200002));
#176661=CARTESIAN_POINT('Ctrl Pts',(8.88254821799995,15.2,-5.95859751700001));
#176662=CARTESIAN_POINT('Ctrl Pts',(8.88254821799995,11.6,-5.95859751700001));
#176663=CARTESIAN_POINT('Ctrl Pts',(8.88097359799995,15.2,-5.95680362900002));
#176664=CARTESIAN_POINT('Ctrl Pts',(8.88097359799995,11.6,-5.95680362900002));
#176665=CARTESIAN_POINT('Ctrl Pts',(8.87940161099994,15.2,-5.95501588200002));
#176666=CARTESIAN_POINT('Ctrl Pts',(8.87940161099994,11.6,-5.95501588200002));
#176667=CARTESIAN_POINT('Ctrl Pts',(8.87783227599994,15.2,-5.95323427800002));
#176668=CARTESIAN_POINT('Ctrl Pts',(8.87783227599994,11.6,-5.95323427800002));
#176669=CARTESIAN_POINT('Ctrl Pts',(8.87626560599994,15.2,-5.95145882200002));
#176670=CARTESIAN_POINT('Ctrl Pts',(8.87626560599994,11.6,-5.95145882200002));
#176671=CARTESIAN_POINT('Ctrl Pts',(8.87470161799994,15.2,-5.94968951600002));
#176672=CARTESIAN_POINT('Ctrl Pts',(8.87470161799994,11.6,-5.94968951600002));
#176673=CARTESIAN_POINT('Ctrl Pts',(8.87314032799994,15.2,-5.94792636200002));
#176674=CARTESIAN_POINT('Ctrl Pts',(8.87314032799994,11.6,-5.94792636200002));
#176675=CARTESIAN_POINT('Ctrl Pts',(8.87158175199994,15.2,-5.94616936400002));
#176676=CARTESIAN_POINT('Ctrl Pts',(8.87158175199994,11.6,-5.94616936400002));
#176677=CARTESIAN_POINT('Ctrl Pts',(8.87002590499994,15.2,-5.94441852500001));
#176678=CARTESIAN_POINT('Ctrl Pts',(8.87002590499994,11.6,-5.94441852500001));
#176679=CARTESIAN_POINT('Ctrl Pts',(8.86847280499994,15.2,-5.94267384800002));
#176680=CARTESIAN_POINT('Ctrl Pts',(8.86847280499994,11.6,-5.94267384800002));
#176681=CARTESIAN_POINT('Ctrl Pts',(8.86692246499994,15.2,-5.94093533700002));
#176682=CARTESIAN_POINT('Ctrl Pts',(8.86692246499994,11.6,-5.94093533700002));
#176683=CARTESIAN_POINT('Ctrl Pts',(8.86537490399994,15.2,-5.93920299200001));
#176684=CARTESIAN_POINT('Ctrl Pts',(8.86537490399994,11.6,-5.93920299200001));
#176685=CARTESIAN_POINT('Ctrl Pts',(8.86383013599995,15.2,-5.93747681900001));
#176686=CARTESIAN_POINT('Ctrl Pts',(8.86383013599995,11.6,-5.93747681900001));
#176687=CARTESIAN_POINT('Ctrl Pts',(8.86228817799994,15.2,-5.93575682000001));
#176688=CARTESIAN_POINT('Ctrl Pts',(8.86228817799994,11.6,-5.93575682000001));
#176689=CARTESIAN_POINT('Ctrl Pts',(8.86074904799995,15.2,-5.93404299900002));
#176690=CARTESIAN_POINT('Ctrl Pts',(8.86074904799995,11.6,-5.93404299900002));
#176691=CARTESIAN_POINT('Ctrl Pts',(8.85921275899994,15.2,-5.93233535700002));
#176692=CARTESIAN_POINT('Ctrl Pts',(8.85921275899994,11.6,-5.93233535700002));
#176693=CARTESIAN_POINT('Ctrl Pts',(8.85767932999994,15.2,-5.93063389900002));
#176694=CARTESIAN_POINT('Ctrl Pts',(8.85767932999994,11.6,-5.93063389900002));
#176695=CARTESIAN_POINT('Ctrl Pts',(8.85614877599994,15.2,-5.92893862600001));
#176696=CARTESIAN_POINT('Ctrl Pts',(8.85614877599994,11.6,-5.92893862600001));
#176697=CARTESIAN_POINT('Ctrl Pts',(8.85462111399994,15.2,-5.92724954300002));
#176698=CARTESIAN_POINT('Ctrl Pts',(8.85462111399994,11.6,-5.92724954300002));
#176699=CARTESIAN_POINT('Ctrl Pts',(8.85309636199995,15.2,-5.92556665200001));
#176700=CARTESIAN_POINT('Ctrl Pts',(8.85309636199995,11.6,-5.92556665200001));
#176701=CARTESIAN_POINT('Ctrl Pts',(8.85157453299995,15.2,-5.92388995600002));
#176702=CARTESIAN_POINT('Ctrl Pts',(8.85157453299995,11.6,-5.92388995600002));
#176703=CARTESIAN_POINT('Ctrl Pts',(8.85005564599994,15.2,-5.92221945900001));
#176704=CARTESIAN_POINT('Ctrl Pts',(8.85005564599994,11.6,-5.92221945900001));
#176705=CARTESIAN_POINT('Ctrl Pts',(8.84853971699994,15.2,-5.92055516300002));
#176706=CARTESIAN_POINT('Ctrl Pts',(8.84853971699994,11.6,-5.92055516300002));
#176707=CARTESIAN_POINT('Ctrl Pts',(8.84702676399994,15.2,-5.91889707100002));
#176708=CARTESIAN_POINT('Ctrl Pts',(8.84702676399994,11.6,-5.91889707100002));
#176709=CARTESIAN_POINT('Ctrl Pts',(8.84551680199994,15.2,-5.91724518500002));
#176710=CARTESIAN_POINT('Ctrl Pts',(8.84551680199994,11.6,-5.91724518500002));
#176711=CARTESIAN_POINT('Ctrl Pts',(8.84400984899994,15.2,-5.91559951100002));
#176712=CARTESIAN_POINT('Ctrl Pts',(8.84400984899994,11.6,-5.91559951100002));
#176713=CARTESIAN_POINT('Ctrl Pts',(8.84250591999994,15.2,-5.91396005000002));
#176714=CARTESIAN_POINT('Ctrl Pts',(8.84250591999994,11.6,-5.91396005000002));
#176715=CARTESIAN_POINT('Ctrl Pts',(8.84100503499995,15.2,-5.91232680500001));
#176716=CARTESIAN_POINT('Ctrl Pts',(8.84100503499995,11.6,-5.91232680500001));
#176717=CARTESIAN_POINT('Ctrl Pts',(8.83950720899995,15.2,-5.91069977900001));
#176718=CARTESIAN_POINT('Ctrl Pts',(8.83950720899995,11.6,-5.91069977900001));
#176719=CARTESIAN_POINT('Ctrl Pts',(8.83801245899994,15.2,-5.90907897500001));
#176720=CARTESIAN_POINT('Ctrl Pts',(8.83801245899994,11.6,-5.90907897500001));
#176721=CARTESIAN_POINT('Ctrl Pts',(8.83652080299994,15.2,-5.90746439700002));
#176722=CARTESIAN_POINT('Ctrl Pts',(8.83652080299994,11.6,-5.90746439700002));
#176723=CARTESIAN_POINT('Ctrl Pts',(8.83503225599994,15.2,-5.90585604700002));
#176724=CARTESIAN_POINT('Ctrl Pts',(8.83503225599994,11.6,-5.90585604700002));
#176725=CARTESIAN_POINT('Ctrl Pts',(8.83354683899995,15.2,-5.90425392800002));
#176726=CARTESIAN_POINT('Ctrl Pts',(8.83354683899995,11.6,-5.90425392800002));
#176727=CARTESIAN_POINT('Ctrl Pts',(8.83206456499994,15.2,-5.90265804300002));
#176728=CARTESIAN_POINT('Ctrl Pts',(8.83206456499994,11.6,-5.90265804300002));
#176729=CARTESIAN_POINT('Ctrl Pts',(8.83058545399994,15.2,-5.90106839600002));
#176730=CARTESIAN_POINT('Ctrl Pts',(8.83058545399994,11.6,-5.90106839600002));
#176731=CARTESIAN_POINT('Ctrl Pts',(8.82910952299994,15.2,-5.89948498800001));
#176732=CARTESIAN_POINT('Ctrl Pts',(8.82910952299994,11.6,-5.89948498800001));
#176733=CARTESIAN_POINT('Ctrl Pts',(8.82763678999994,15.2,-5.89790782400001));
#176734=CARTESIAN_POINT('Ctrl Pts',(8.82763678999994,11.6,-5.89790782400001));
#176735=CARTESIAN_POINT('Ctrl Pts',(8.82616726999995,15.2,-5.89633690700002));
#176736=CARTESIAN_POINT('Ctrl Pts',(8.82616726999995,11.6,-5.89633690700002));
#176737=CARTESIAN_POINT('Ctrl Pts',(8.82470098299994,15.2,-5.89477223700002));
#176738=CARTESIAN_POINT('Ctrl Pts',(8.82470098299994,11.6,-5.89477223700002));
#176739=CARTESIAN_POINT('Ctrl Pts',(8.82323794599994,15.2,-5.89321382000002));
#176740=CARTESIAN_POINT('Ctrl Pts',(8.82323794599994,11.6,-5.89321382000002));
#176741=CARTESIAN_POINT('Ctrl Pts',(8.82177817599995,15.2,-5.89166165800002));
#176742=CARTESIAN_POINT('Ctrl Pts',(8.82177817599995,11.6,-5.89166165800002));
#176743=CARTESIAN_POINT('Ctrl Pts',(8.82032169199995,15.2,-5.89011575500002));
#176744=CARTESIAN_POINT('Ctrl Pts',(8.82032169199995,11.6,-5.89011575500002));
#176745=CARTESIAN_POINT('Ctrl Pts',(8.81886850899994,15.2,-5.88857611200002));
#176746=CARTESIAN_POINT('Ctrl Pts',(8.81886850899994,11.6,-5.88857611200002));
#176747=CARTESIAN_POINT('Ctrl Pts',(8.81741864799995,15.2,-5.88704273300002));
#176748=CARTESIAN_POINT('Ctrl Pts',(8.81741864799995,11.6,-5.88704273300002));
#176749=CARTESIAN_POINT('Ctrl Pts',(8.81597212499994,15.2,-5.88551562100001));
#176750=CARTESIAN_POINT('Ctrl Pts',(8.81597212499994,11.6,-5.88551562100001));
#176751=CARTESIAN_POINT('Ctrl Pts',(8.81452895999994,15.2,-5.88399477900002));
#176752=CARTESIAN_POINT('Ctrl Pts',(8.81452895999994,11.6,-5.88399477900002));
#176753=CARTESIAN_POINT('Ctrl Pts',(8.81308916799994,15.2,-5.88248021000001));
#176754=CARTESIAN_POINT('Ctrl Pts',(8.81308916799994,11.6,-5.88248021000001));
#176755=CARTESIAN_POINT('Ctrl Pts',(8.81165276999995,15.2,-5.88097191600002));
#176756=CARTESIAN_POINT('Ctrl Pts',(8.81165276999995,11.6,-5.88097191600002));
#176757=CARTESIAN_POINT('Ctrl Pts',(8.81021978099995,15.2,-5.87946990100002));
#176758=CARTESIAN_POINT('Ctrl Pts',(8.81021978099995,11.6,-5.87946990100002));
#176759=CARTESIAN_POINT('Ctrl Pts',(8.80879022299995,15.2,-5.87797416800001));
#176760=CARTESIAN_POINT('Ctrl Pts',(8.80879022299995,11.6,-5.87797416800001));
#176761=CARTESIAN_POINT('Ctrl Pts',(8.80736410999994,15.2,-5.87648472000001));
#176762=CARTESIAN_POINT('Ctrl Pts',(8.80736410999994,11.6,-5.87648472000001));
#176763=CARTESIAN_POINT('Ctrl Pts',(8.80594146399994,15.2,-5.87500155900001));
#176764=CARTESIAN_POINT('Ctrl Pts',(8.80594146399994,11.6,-5.87500155900001));
#176765=CARTESIAN_POINT('Ctrl Pts',(8.80452230199994,15.2,-5.87352468900002));
#176766=CARTESIAN_POINT('Ctrl Pts',(8.80452230199994,11.6,-5.87352468900002));
#176767=CARTESIAN_POINT('Ctrl Pts',(8.80310664299994,15.2,-5.87205411200002));
#176768=CARTESIAN_POINT('Ctrl Pts',(8.80310664299994,11.6,-5.87205411200002));
#176769=CARTESIAN_POINT('Ctrl Pts',(8.80169450299995,15.2,-5.87058983100002));
#176770=CARTESIAN_POINT('Ctrl Pts',(8.80169450299995,11.6,-5.87058983100002));
#176771=CARTESIAN_POINT('Ctrl Pts',(8.80028590299995,15.2,-5.86913185100002));
#176772=CARTESIAN_POINT('Ctrl Pts',(8.80028590299995,11.6,-5.86913185100002));
#176773=CARTESIAN_POINT('Ctrl Pts',(8.79888086099994,15.2,-5.86768017200002));
#176774=CARTESIAN_POINT('Ctrl Pts',(8.79888086099994,11.6,-5.86768017200002));
#176775=CARTESIAN_POINT('Ctrl Pts',(8.79747939599994,15.2,-5.86623479800001));
#176776=CARTESIAN_POINT('Ctrl Pts',(8.79747939599994,11.6,-5.86623479800001));
#176777=CARTESIAN_POINT('Ctrl Pts',(8.79608152699995,15.2,-5.86479573300001));
#176778=CARTESIAN_POINT('Ctrl Pts',(8.79608152699995,11.6,-5.86479573300001));
#176779=CARTESIAN_POINT('Ctrl Pts',(8.79468727199994,15.2,-5.86336297900001));
#176780=CARTESIAN_POINT('Ctrl Pts',(8.79468727199994,11.6,-5.86336297900001));
#176781=CARTESIAN_POINT('Ctrl Pts',(8.79329664999995,15.2,-5.86193653900001));
#176782=CARTESIAN_POINT('Ctrl Pts',(8.79329664999995,11.6,-5.86193653900001));
#176783=CARTESIAN_POINT('Ctrl Pts',(8.79190967899994,15.2,-5.86051641600001));
#176784=CARTESIAN_POINT('Ctrl Pts',(8.79190967899994,11.6,-5.86051641600001));
#176785=CARTESIAN_POINT('Ctrl Pts',(8.79052638099994,15.2,-5.85910261200001));
#176786=CARTESIAN_POINT('Ctrl Pts',(8.79052638099994,11.6,-5.85910261200001));
#176787=CARTESIAN_POINT('Ctrl Pts',(8.78914677299995,15.2,-5.85769513200002));
#176788=CARTESIAN_POINT('Ctrl Pts',(8.78914677299995,11.6,-5.85769513200002));
#176789=CARTESIAN_POINT('Ctrl Pts',(8.78777087299994,15.2,-5.85629397800002));
#176790=CARTESIAN_POINT('Ctrl Pts',(8.78777087299994,11.6,-5.85629397800002));
#176791=CARTESIAN_POINT('Ctrl Pts',(8.78639870199994,15.2,-5.85489915100001));
#176792=CARTESIAN_POINT('Ctrl Pts',(8.78639870199994,11.6,-5.85489915100001));
#176793=CARTESIAN_POINT('Ctrl Pts',(8.78503027999994,15.2,-5.85351065700002));
#176794=CARTESIAN_POINT('Ctrl Pts',(8.78503027999994,11.6,-5.85351065700002));
#176795=CARTESIAN_POINT('Ctrl Pts',(8.78366562499994,15.2,-5.85212849700002));
#176796=CARTESIAN_POINT('Ctrl Pts',(8.78366562499994,11.6,-5.85212849700002));
#176797=CARTESIAN_POINT('Ctrl Pts',(8.78230475599995,15.2,-5.85075267500001));
#176798=CARTESIAN_POINT('Ctrl Pts',(8.78230475599995,11.6,-5.85075267500001));
#176799=CARTESIAN_POINT('Ctrl Pts',(8.78094769299994,15.2,-5.84938319200001));
#176800=CARTESIAN_POINT('Ctrl Pts',(8.78094769299994,11.6,-5.84938319200001));
#176801=CARTESIAN_POINT('Ctrl Pts',(8.77959445599994,15.2,-5.84802005300002));
#176802=CARTESIAN_POINT('Ctrl Pts',(8.77959445599994,11.6,-5.84802005300002));
#176803=CARTESIAN_POINT('Ctrl Pts',(8.77824506399994,15.2,-5.84666326000002));
#176804=CARTESIAN_POINT('Ctrl Pts',(8.77824506399994,11.6,-5.84666326000002));
#176805=CARTESIAN_POINT('Ctrl Pts',(8.77689953799995,15.2,-5.84531281600002));
#176806=CARTESIAN_POINT('Ctrl Pts',(8.77689953799995,11.6,-5.84531281600002));
#176807=CARTESIAN_POINT('Ctrl Pts',(8.77555789499995,15.2,-5.84396872400001));
#176808=CARTESIAN_POINT('Ctrl Pts',(8.77555789499995,11.6,-5.84396872400001));
#176809=CARTESIAN_POINT('Ctrl Pts',(8.77422015899995,15.2,-5.84263098700001));
#176810=CARTESIAN_POINT('Ctrl Pts',(8.77422015899995,11.6,-5.84263098700001));
#176811=CARTESIAN_POINT('Ctrl Pts',(8.77288634599994,15.2,-5.84129960800002));
#176812=CARTESIAN_POINT('Ctrl Pts',(8.77288634599994,11.6,-5.84129960800002));
#176813=CARTESIAN_POINT('Ctrl Pts',(8.77155647799994,15.2,-5.83997458900001));
#176814=CARTESIAN_POINT('Ctrl Pts',(8.77155647799994,11.6,-5.83997458900001));
#176815=CARTESIAN_POINT('Ctrl Pts',(8.77023057299994,15.2,-5.83865593400001));
#176816=CARTESIAN_POINT('Ctrl Pts',(8.77023057299994,11.6,-5.83865593400001));
#176817=CARTESIAN_POINT('Ctrl Pts',(8.76890865499995,15.2,-5.83734364500001));
#176818=CARTESIAN_POINT('Ctrl Pts',(8.76890865499995,11.6,-5.83734364500001));
#176819=CARTESIAN_POINT('Ctrl Pts',(8.76759074099994,15.2,-5.83603772600001));
#176820=CARTESIAN_POINT('Ctrl Pts',(8.76759074099994,11.6,-5.83603772600001));
#176821=CARTESIAN_POINT('Ctrl Pts',(8.76627685199994,15.2,-5.83473817900002));
#176822=CARTESIAN_POINT('Ctrl Pts',(8.76627685199994,11.6,-5.83473817900002));
#176823=CARTESIAN_POINT('Ctrl Pts',(8.76496700799994,15.2,-5.83344500600001));
#176824=CARTESIAN_POINT('Ctrl Pts',(8.76496700799994,11.6,-5.83344500600001));
#176825=CARTESIAN_POINT('Ctrl Pts',(8.76366123099995,15.2,-5.83215821200002));
#176826=CARTESIAN_POINT('Ctrl Pts',(8.76366123099995,11.6,-5.83215821200002));
#176827=CARTESIAN_POINT('Ctrl Pts',(8.76235953899995,15.2,-5.83087780000002));
#176828=CARTESIAN_POINT('Ctrl Pts',(8.76235953899995,11.6,-5.83087780000002));
#176829=CARTESIAN_POINT('Ctrl Pts',(8.76106195499995,15.2,-5.82960377000001));
#176830=CARTESIAN_POINT('Ctrl Pts',(8.76106195499995,11.6,-5.82960377000001));
#176831=CARTESIAN_POINT('Ctrl Pts',(8.75976849799994,15.2,-5.82833612700002));
#176832=CARTESIAN_POINT('Ctrl Pts',(8.75976849799994,11.6,-5.82833612700002));
#176833=CARTESIAN_POINT('Ctrl Pts',(8.75847918999994,15.2,-5.82707487400001));
#176834=CARTESIAN_POINT('Ctrl Pts',(8.75847918999994,11.6,-5.82707487400001));
#176835=CARTESIAN_POINT('Ctrl Pts',(8.75719405099994,15.2,-5.82582001200001));
#176836=CARTESIAN_POINT('Ctrl Pts',(8.75719405099994,11.6,-5.82582001200001));
#176837=CARTESIAN_POINT('Ctrl Pts',(8.75591310099994,15.2,-5.82457154700001));
#176838=CARTESIAN_POINT('Ctrl Pts',(8.75591310099994,11.6,-5.82457154700001));
#176839=CARTESIAN_POINT('Ctrl Pts',(8.75463636299994,15.2,-5.82332947900002));
#176840=CARTESIAN_POINT('Ctrl Pts',(8.75463636299994,11.6,-5.82332947900002));
#176841=CARTESIAN_POINT('Ctrl Pts',(8.75336385699995,15.2,-5.82209381200002));
#176842=CARTESIAN_POINT('Ctrl Pts',(8.75336385699995,11.6,-5.82209381200002));
#176843=CARTESIAN_POINT('Ctrl Pts',(8.75209560399994,15.2,-5.82086454900002));
#176844=CARTESIAN_POINT('Ctrl Pts',(8.75209560399994,11.6,-5.82086454900002));
#176845=CARTESIAN_POINT('Ctrl Pts',(8.75083162399994,15.2,-5.81964169300001));
#176846=CARTESIAN_POINT('Ctrl Pts',(8.75083162399994,11.6,-5.81964169300001));
#176847=CARTESIAN_POINT('Ctrl Pts',(8.74957194099995,15.2,-5.81842524600001));
#176848=CARTESIAN_POINT('Ctrl Pts',(8.74957194099995,11.6,-5.81842524600001));
#176849=CARTESIAN_POINT('Ctrl Pts',(8.74831657499995,15.2,-5.81721521200001));
#176850=CARTESIAN_POINT('Ctrl Pts',(8.74831657499995,11.6,-5.81721521200001));
#176851=CARTESIAN_POINT('Ctrl Pts',(8.74706554699994,15.2,-5.81601159300002));
#176852=CARTESIAN_POINT('Ctrl Pts',(8.74706554699994,11.6,-5.81601159300002));
#176853=CARTESIAN_POINT('Ctrl Pts',(8.74581887699994,15.2,-5.81481439200001));
#176854=CARTESIAN_POINT('Ctrl Pts',(8.74581887699994,11.6,-5.81481439200001));
#176855=CARTESIAN_POINT('Ctrl Pts',(8.74457659099994,15.2,-5.81362361200001));
#176856=CARTESIAN_POINT('Ctrl Pts',(8.74457659099994,11.6,-5.81362361200001));
#176857=CARTESIAN_POINT('Ctrl Pts',(8.74333870599994,15.2,-5.81243925600001));
#176858=CARTESIAN_POINT('Ctrl Pts',(8.74333870599994,11.6,-5.81243925600001));
#176859=CARTESIAN_POINT('Ctrl Pts',(8.74210524799994,15.2,-5.81126132700001));
#176860=CARTESIAN_POINT('Ctrl Pts',(8.74210524799994,11.6,-5.81126132700001));
#176861=CARTESIAN_POINT('Ctrl Pts',(8.74087623499994,15.2,-5.81008982700002));
#176862=CARTESIAN_POINT('Ctrl Pts',(8.74087623499994,11.6,-5.81008982700002));
#176863=CARTESIAN_POINT('Ctrl Pts',(8.73965169199994,15.2,-5.80892476100002));
#176864=CARTESIAN_POINT('Ctrl Pts',(8.73965169199994,11.6,-5.80892476100002));
#176865=CARTESIAN_POINT('Ctrl Pts',(8.73843163899994,15.2,-5.80776612800002));
#176866=CARTESIAN_POINT('Ctrl Pts',(8.73843163899994,11.6,-5.80776612800002));
#176867=CARTESIAN_POINT('Ctrl Pts',(8.73721609799994,15.2,-5.80661393400002));
#176868=CARTESIAN_POINT('Ctrl Pts',(8.73721609799994,11.6,-5.80661393400002));
#176869=CARTESIAN_POINT('Ctrl Pts',(8.73600509299994,15.2,-5.80546818100002));
#176870=CARTESIAN_POINT('Ctrl Pts',(8.73600509299994,11.6,-5.80546818100002));
#176871=CARTESIAN_POINT('Ctrl Pts',(8.73479864499994,15.2,-5.80432887100002));
#176872=CARTESIAN_POINT('Ctrl Pts',(8.73479864499994,11.6,-5.80432887100002));
#176873=CARTESIAN_POINT('Ctrl Pts',(8.73359677499994,15.2,-5.80319600900002));
#176874=CARTESIAN_POINT('Ctrl Pts',(8.73359677499994,11.6,-5.80319600900002));
#176875=CARTESIAN_POINT('Ctrl Pts',(8.73239950899995,15.2,-5.80206959500002));
#176876=CARTESIAN_POINT('Ctrl Pts',(8.73239950899995,11.6,-5.80206959500002));
#176877=CARTESIAN_POINT('Ctrl Pts',(8.73120686699994,15.2,-5.80094963400001));
#176878=CARTESIAN_POINT('Ctrl Pts',(8.73120686699994,11.6,-5.80094963400001));
#176879=CARTESIAN_POINT('Ctrl Pts',(8.73001887199995,15.2,-5.79983612900002));
#176880=CARTESIAN_POINT('Ctrl Pts',(8.73001887199995,11.6,-5.79983612900002));
#176881=CARTESIAN_POINT('Ctrl Pts',(8.72883554599994,15.2,-5.79872908100001));
#176882=CARTESIAN_POINT('Ctrl Pts',(8.72883554599994,11.6,-5.79872908100001));
#176883=CARTESIAN_POINT('Ctrl Pts',(8.72765691199995,15.2,-5.79762849300002));
#176884=CARTESIAN_POINT('Ctrl Pts',(8.72765691199995,11.6,-5.79762849300002));
#176885=CARTESIAN_POINT('Ctrl Pts',(8.72648299499994,15.2,-5.79653436900001));
#176886=CARTESIAN_POINT('Ctrl Pts',(8.72648299499994,11.6,-5.79653436900001));
#176887=CARTESIAN_POINT('Ctrl Pts',(8.72531381599994,15.2,-5.79544671200001));
#176888=CARTESIAN_POINT('Ctrl Pts',(8.72531381599994,11.6,-5.79544671200001));
#176889=CARTESIAN_POINT('Ctrl Pts',(8.72414939899994,15.2,-5.79436552400002));
#176890=CARTESIAN_POINT('Ctrl Pts',(8.72414939899994,11.6,-5.79436552400002));
#176891=CARTESIAN_POINT('Ctrl Pts',(8.72298976599994,15.2,-5.79329080700001));
#176892=CARTESIAN_POINT('Ctrl Pts',(8.72298976599994,11.6,-5.79329080700001));
#176893=CARTESIAN_POINT('Ctrl Pts',(8.72183494099994,15.2,-5.79222256600002));
#176894=CARTESIAN_POINT('Ctrl Pts',(8.72183494099994,11.6,-5.79222256600002));
#176895=CARTESIAN_POINT('Ctrl Pts',(8.72068494799995,15.2,-5.79116080200002));
#176896=CARTESIAN_POINT('Ctrl Pts',(8.72068494799995,11.6,-5.79116080200002));
#176897=CARTESIAN_POINT('Ctrl Pts',(8.71953980799994,15.2,-5.79010551900002));
#176898=CARTESIAN_POINT('Ctrl Pts',(8.71953980799994,11.6,-5.79010551900002));
#176899=CARTESIAN_POINT('Ctrl Pts',(8.71839954799994,15.2,-5.78905671900002));
#176900=CARTESIAN_POINT('Ctrl Pts',(8.71839954799994,11.6,-5.78905671900002));
#176901=CARTESIAN_POINT('Ctrl Pts',(8.71726418899994,15.2,-5.78801440500002));
#176902=CARTESIAN_POINT('Ctrl Pts',(8.71726418899994,11.6,-5.78801440500002));
#176903=CARTESIAN_POINT('Ctrl Pts',(8.71613375599994,15.2,-5.78697858000002));
#176904=CARTESIAN_POINT('Ctrl Pts',(8.71613375599994,11.6,-5.78697858000002));
#176905=CARTESIAN_POINT('Ctrl Pts',(8.71500827199995,15.2,-5.78594924700001));
#176906=CARTESIAN_POINT('Ctrl Pts',(8.71500827199995,11.6,-5.78594924700001));
#176907=CARTESIAN_POINT('Ctrl Pts',(8.71388776199994,15.2,-5.78492640800001));
#176908=CARTESIAN_POINT('Ctrl Pts',(8.71388776199994,11.6,-5.78492640800001));
#176909=CARTESIAN_POINT('Ctrl Pts',(8.71277224899995,15.2,-5.78391006700001));
#176910=CARTESIAN_POINT('Ctrl Pts',(8.71277224899995,11.6,-5.78391006700001));
#176911=CARTESIAN_POINT('Ctrl Pts',(8.71166175799994,15.2,-5.78290022500001));
#176912=CARTESIAN_POINT('Ctrl Pts',(8.71166175799994,11.6,-5.78290022500001));
#176913=CARTESIAN_POINT('Ctrl Pts',(8.71055631199994,15.2,-5.78189688600002));
#176914=CARTESIAN_POINT('Ctrl Pts',(8.71055631199994,11.6,-5.78189688600002));
#176915=CARTESIAN_POINT('Ctrl Pts',(8.70945593699994,15.2,-5.78090005400002));
#176916=CARTESIAN_POINT('Ctrl Pts',(8.70945593699994,11.6,-5.78090005400002));
#176917=CARTESIAN_POINT('Ctrl Pts',(8.70836065599994,15.2,-5.77990973000002));
#176918=CARTESIAN_POINT('Ctrl Pts',(8.70836065599994,11.6,-5.77990973000002));
#176919=CARTESIAN_POINT('Ctrl Pts',(8.70727049299994,15.2,-5.77892591600002));
#176920=CARTESIAN_POINT('Ctrl Pts',(8.70727049299994,11.6,-5.77892591600002));
#176921=CARTESIAN_POINT('Ctrl Pts',(8.70618547399994,15.2,-5.77794861800002));
#176922=CARTESIAN_POINT('Ctrl Pts',(8.70618547399994,11.6,-5.77794861800002));
#176923=CARTESIAN_POINT('Ctrl Pts',(8.70510562399994,15.2,-5.77697783500002));
#176924=CARTESIAN_POINT('Ctrl Pts',(8.70510562399994,11.6,-5.77697783500002));
#176925=CARTESIAN_POINT('Ctrl Pts',(8.70403096699994,15.2,-5.77601357300002));
#176926=CARTESIAN_POINT('Ctrl Pts',(8.70403096699994,11.6,-5.77601357300002));
#176927=CARTESIAN_POINT('Ctrl Pts',(8.70296152799994,15.2,-5.77505583400002));
#176928=CARTESIAN_POINT('Ctrl Pts',(8.70296152799994,11.6,-5.77505583400002));
#176929=CARTESIAN_POINT('Ctrl Pts',(8.70189733199994,15.2,-5.77410461900002));
#176930=CARTESIAN_POINT('Ctrl Pts',(8.70189733199994,11.6,-5.77410461900002));
#176931=CARTESIAN_POINT('Ctrl Pts',(8.70083840399994,15.2,-5.77315993200001));
#176932=CARTESIAN_POINT('Ctrl Pts',(8.70083840399994,11.6,-5.77315993200001));
#176933=CARTESIAN_POINT('Ctrl Pts',(8.69978476999994,15.2,-5.77222177600002));
#176934=CARTESIAN_POINT('Ctrl Pts',(8.69978476999994,11.6,-5.77222177600002));
#176935=CARTESIAN_POINT('Ctrl Pts',(8.69873645399995,15.2,-5.77129015300001));
#176936=CARTESIAN_POINT('Ctrl Pts',(8.69873645399995,11.6,-5.77129015300001));
#176937=CARTESIAN_POINT('Ctrl Pts',(8.69769348299995,15.2,-5.77036506700002));
#176938=CARTESIAN_POINT('Ctrl Pts',(8.69769348299995,11.6,-5.77036506700002));
#176939=CARTESIAN_POINT('Ctrl Pts',(8.69665588299994,15.2,-5.76944652000002));
#176940=CARTESIAN_POINT('Ctrl Pts',(8.69665588299994,11.6,-5.76944652000002));
#176941=CARTESIAN_POINT('Ctrl Pts',(8.69562367699995,15.2,-5.76853451600002));
#176942=CARTESIAN_POINT('Ctrl Pts',(8.69562367699995,11.6,-5.76853451600002));
#176943=CARTESIAN_POINT('Ctrl Pts',(8.69459689299994,15.2,-5.76762905500001));
#176944=CARTESIAN_POINT('Ctrl Pts',(8.69459689299994,11.6,-5.76762905500001));
#176945=CARTESIAN_POINT('Ctrl Pts',(8.69357555699995,15.2,-5.76673014200002));
#176946=CARTESIAN_POINT('Ctrl Pts',(8.69357555699995,11.6,-5.76673014200002));
#176947=CARTESIAN_POINT('Ctrl Pts',(8.69255969299994,15.2,-5.76583777900002));
#176948=CARTESIAN_POINT('Ctrl Pts',(8.69255969299994,11.6,-5.76583777900002));
#176949=CARTESIAN_POINT('Ctrl Pts',(8.69154932899994,15.2,-5.76495197000002));
#176950=CARTESIAN_POINT('Ctrl Pts',(8.69154932899994,11.6,-5.76495197000002));
#176951=CARTESIAN_POINT('Ctrl Pts',(8.69054449099995,15.2,-5.76407271500001));
#176952=CARTESIAN_POINT('Ctrl Pts',(8.69054449099995,11.6,-5.76407271500001));
#176953=CARTESIAN_POINT('Ctrl Pts',(8.68954520599994,15.2,-5.76320002000001));
#176954=CARTESIAN_POINT('Ctrl Pts',(8.68954520599994,11.6,-5.76320002000001));
#176955=CARTESIAN_POINT('Ctrl Pts',(8.68855149799994,15.2,-5.76233388600001));
#176956=CARTESIAN_POINT('Ctrl Pts',(8.68855149799994,11.6,-5.76233388600001));
#176957=CARTESIAN_POINT('Ctrl Pts',(8.68756339599994,15.2,-5.76147431500001));
#176958=CARTESIAN_POINT('Ctrl Pts',(8.68756339599994,11.6,-5.76147431500001));
#176959=CARTESIAN_POINT('Ctrl Pts',(8.68658092499994,15.2,-5.76062131100001));
#176960=CARTESIAN_POINT('Ctrl Pts',(8.68658092499994,11.6,-5.76062131100001));
#176961=CARTESIAN_POINT('Ctrl Pts',(8.68560411399995,15.2,-5.75977487700002));
#176962=CARTESIAN_POINT('Ctrl Pts',(8.68560411399995,11.6,-5.75977487700002));
#176963=CARTESIAN_POINT('Ctrl Pts',(8.68463298799995,15.2,-5.75893501600002));
#176964=CARTESIAN_POINT('Ctrl Pts',(8.68463298799995,11.6,-5.75893501600002));
#176965=CARTESIAN_POINT('Ctrl Pts',(8.68366757599994,15.2,-5.75810172900002));
#176966=CARTESIAN_POINT('Ctrl Pts',(8.68366757599994,11.6,-5.75810172900002));
#176967=CARTESIAN_POINT('Ctrl Pts',(8.68270790299994,15.2,-5.75727502000002));
#176968=CARTESIAN_POINT('Ctrl Pts',(8.68270790299994,11.6,-5.75727502000002));
#176969=CARTESIAN_POINT('Ctrl Pts',(8.68175399699994,15.2,-5.75645489200002));
#176970=CARTESIAN_POINT('Ctrl Pts',(8.68175399699994,11.6,-5.75645489200002));
#176971=CARTESIAN_POINT('Ctrl Pts',(8.68080588599994,15.2,-5.75564134800001));
#176972=CARTESIAN_POINT('Ctrl Pts',(8.68080588599994,11.6,-5.75564134800001));
#176973=CARTESIAN_POINT('Ctrl Pts',(8.67986359699995,15.2,-5.75483438900001));
#176974=CARTESIAN_POINT('Ctrl Pts',(8.67986359699995,11.6,-5.75483438900001));
#176975=CARTESIAN_POINT('Ctrl Pts',(8.67892715799995,15.2,-5.75403401900001));
#176976=CARTESIAN_POINT('Ctrl Pts',(8.67892715799995,11.6,-5.75403401900001));
#176977=CARTESIAN_POINT('Ctrl Pts',(8.67799659699994,15.2,-5.75324024000002));
#176978=CARTESIAN_POINT('Ctrl Pts',(8.67799659699994,11.6,-5.75324024000002));
#176979=CARTESIAN_POINT('Ctrl Pts',(8.67707194199994,15.2,-5.75245305500002));
#176980=CARTESIAN_POINT('Ctrl Pts',(8.67707194199994,11.6,-5.75245305500002));
#176981=CARTESIAN_POINT('Ctrl Pts',(8.67615321999994,15.2,-5.75167246800002));
#176982=CARTESIAN_POINT('Ctrl Pts',(8.67615321999994,11.6,-5.75167246800002));
#176983=CARTESIAN_POINT('Ctrl Pts',(8.67524046199994,15.2,-5.75089848100002));
#176984=CARTESIAN_POINT('Ctrl Pts',(8.67524046199994,11.6,-5.75089848100002));
#176985=CARTESIAN_POINT('Ctrl Pts',(8.67433369199994,15.2,-5.75013109600001));
#176986=CARTESIAN_POINT('Ctrl Pts',(8.67433369199994,11.6,-5.75013109600001));
#176987=CARTESIAN_POINT('Ctrl Pts',(8.67343294199994,15.2,-5.74937031600002));
#176988=CARTESIAN_POINT('Ctrl Pts',(8.67343294199994,11.6,-5.74937031600002));
#176989=CARTESIAN_POINT('Ctrl Pts',(8.67253823899994,15.2,-5.74861614500002));
#176990=CARTESIAN_POINT('Ctrl Pts',(8.67253823899994,11.6,-5.74861614500002));
#176991=CARTESIAN_POINT('Ctrl Pts',(8.67164961199994,15.2,-5.74786858400002));
#176992=CARTESIAN_POINT('Ctrl Pts',(8.67164961199994,11.6,-5.74786858400002));
#176993=CARTESIAN_POINT('Ctrl Pts',(8.67076709099995,15.2,-5.74712763600001));
#176994=CARTESIAN_POINT('Ctrl Pts',(8.67076709099995,11.6,-5.74712763600001));
#176995=CARTESIAN_POINT('Ctrl Pts',(8.66989070299995,15.2,-5.74639330500001));
#176996=CARTESIAN_POINT('Ctrl Pts',(8.66989070299995,11.6,-5.74639330500001));
#176997=CARTESIAN_POINT('Ctrl Pts',(8.66902047899995,15.2,-5.74566559300001));
#176998=CARTESIAN_POINT('Ctrl Pts',(8.66902047899995,11.6,-5.74566559300001));
#176999=CARTESIAN_POINT('Ctrl Pts',(8.66815644699994,15.2,-5.74494450200002));
#177000=CARTESIAN_POINT('Ctrl Pts',(8.66815644699994,11.6,-5.74494450200002));
#177001=CARTESIAN_POINT('Ctrl Pts',(8.66729863599994,15.2,-5.74423003600002));
#177002=CARTESIAN_POINT('Ctrl Pts',(8.66729863599994,11.6,-5.74423003600002));
#177003=CARTESIAN_POINT('Ctrl Pts',(8.66644707699994,15.2,-5.74352219600001));
#177004=CARTESIAN_POINT('Ctrl Pts',(8.66644707699994,11.6,-5.74352219600001));
#177005=CARTESIAN_POINT('Ctrl Pts',(8.66560179899994,15.2,-5.74282098700002));
#177006=CARTESIAN_POINT('Ctrl Pts',(8.66560179899994,11.6,-5.74282098700002));
#177007=CARTESIAN_POINT('Ctrl Pts',(8.66476283199994,15.2,-5.74212641100001));
#177008=CARTESIAN_POINT('Ctrl Pts',(8.66476283199994,11.6,-5.74212641100001));
#177009=CARTESIAN_POINT('Ctrl Pts',(8.66393020599994,15.2,-5.74143847000002));
#177010=CARTESIAN_POINT('Ctrl Pts',(8.66393020599994,11.6,-5.74143847000002));
#177011=CARTESIAN_POINT('Ctrl Pts',(8.66310394999994,15.2,-5.74075716600002));
#177012=CARTESIAN_POINT('Ctrl Pts',(8.66310394999994,11.6,-5.74075716600002));
#177013=CARTESIAN_POINT('Ctrl Pts',(8.66228409599995,15.2,-5.74008250400002));
#177014=CARTESIAN_POINT('Ctrl Pts',(8.66228409599995,11.6,-5.74008250400002));
#177015=CARTESIAN_POINT('Ctrl Pts',(8.66147067299995,15.2,-5.73941448500002));
#177016=CARTESIAN_POINT('Ctrl Pts',(8.66147067299995,11.6,-5.73941448500002));
#177017=CARTESIAN_POINT('Ctrl Pts',(8.66066371399994,15.2,-5.73875311200001));
#177018=CARTESIAN_POINT('Ctrl Pts',(8.66066371399994,11.6,-5.73875311200001));
#177019=CARTESIAN_POINT('Ctrl Pts',(8.65986324599995,15.2,-5.73809838800001));
#177020=CARTESIAN_POINT('Ctrl Pts',(8.65986324599995,11.6,-5.73809838800001));
#177021=CARTESIAN_POINT('Ctrl Pts',(8.65906930199994,15.2,-5.73745031600001));
#177022=CARTESIAN_POINT('Ctrl Pts',(8.65906930199994,11.6,-5.73745031600001));
#177023=CARTESIAN_POINT('Ctrl Pts',(8.65828191299994,15.2,-5.73680889800002));
#177024=CARTESIAN_POINT('Ctrl Pts',(8.65828191299994,11.6,-5.73680889800002));
#177025=CARTESIAN_POINT('Ctrl Pts',(8.65750110999995,15.2,-5.73617413800001));
#177026=CARTESIAN_POINT('Ctrl Pts',(8.65750110999995,11.6,-5.73617413800001));
#177027=CARTESIAN_POINT('Ctrl Pts',(8.65672692399994,15.2,-5.73554603700002));
#177028=CARTESIAN_POINT('Ctrl Pts',(8.65672692399994,11.6,-5.73554603700002));
#177029=CARTESIAN_POINT('Ctrl Pts',(8.65595938699995,15.2,-5.73492459900002));
#177030=CARTESIAN_POINT('Ctrl Pts',(8.65595938699995,11.6,-5.73492459900002));
#177031=CARTESIAN_POINT('Ctrl Pts',(8.65519852999994,15.2,-5.73430982600001));
#177032=CARTESIAN_POINT('Ctrl Pts',(8.65519852999994,11.6,-5.73430982600001));
#177033=CARTESIAN_POINT('Ctrl Pts',(8.65444438599994,15.2,-5.73370172000002));
#177034=CARTESIAN_POINT('Ctrl Pts',(8.65444438599994,11.6,-5.73370172000002));
#177035=CARTESIAN_POINT('Ctrl Pts',(8.65369698499994,15.2,-5.73310028600002));
#177036=CARTESIAN_POINT('Ctrl Pts',(8.65369698499994,11.6,-5.73310028600002));
#177037=CARTESIAN_POINT('Ctrl Pts',(8.65295636099994,15.2,-5.73250552500002));
#177038=CARTESIAN_POINT('Ctrl Pts',(8.65295636099994,11.6,-5.73250552500002));
#177039=CARTESIAN_POINT('Ctrl Pts',(8.65222254499994,15.2,-5.73191744000002));
#177040=CARTESIAN_POINT('Ctrl Pts',(8.65222254499994,11.6,-5.73191744000002));
#177041=CARTESIAN_POINT('Ctrl Pts',(8.65149556899994,15.2,-5.73133603500001));
#177042=CARTESIAN_POINT('Ctrl Pts',(8.65149556899994,11.6,-5.73133603500001));
#177043=CARTESIAN_POINT('Ctrl Pts',(8.65077961599994,15.2,-5.73076462100002));
#177044=CARTESIAN_POINT('Ctrl Pts',(8.65077961599994,11.6,-5.73076462100002));
#177045=CARTESIAN_POINT('Ctrl Pts',(8.65021312699995,15.2,-5.73031342200002));
#177046=CARTESIAN_POINT('Ctrl Pts',(8.65021312699995,11.6,-5.73031342200002));
#177047=CARTESIAN_POINT('Ctrl Pts',(8.64979234999995,15.2,-5.72997879200001));
#177048=CARTESIAN_POINT('Ctrl Pts',(8.64979234999995,11.6,-5.72997879200001));
#177049=CARTESIAN_POINT('Ctrl Pts',(8.64951454399994,15.2,-5.72975808600001));
#177050=CARTESIAN_POINT('Ctrl Pts',(8.64951454399994,11.6,-5.72975808600001));
#177051=CARTESIAN_POINT('Ctrl Pts',(8.64937799899994,15.2,-5.72964966100002));
#177052=CARTESIAN_POINT('Ctrl Pts',(8.64937799899994,11.6,-5.72964966100002));
#177053=CARTESIAN_POINT('',(8.64937799799994,12.2,-5.72964966100002));
#177054=CARTESIAN_POINT('',(8.64937799799994,15.2,-5.72964966100002));
#177055=CARTESIAN_POINT('',(8.64937799799994,12.2,-5.72964966100002));
#177056=CARTESIAN_POINT('Ctrl Pts',(9.36775917477149,12.2,-6.67046385458018));
#177057=CARTESIAN_POINT('Ctrl Pts',(9.36593194451564,12.2,-6.66710588411075));
#177058=CARTESIAN_POINT('Ctrl Pts',(9.36410408859324,12.2,-6.6637557852869));
#177059=CARTESIAN_POINT('Ctrl Pts',(9.36227560146925,12.2,-6.66041356411704));
#177060=CARTESIAN_POINT('Ctrl Pts',(9.36044711426905,12.2,-6.65707134280789));
#177061=CARTESIAN_POINT('Ctrl Pts',(9.3586179987788,12.2,-6.65373699735653));
#177062=CARTESIAN_POINT('Ctrl Pts',(9.35678826937895,12.2,-6.65041053364363));
#177063=CARTESIAN_POINT('Ctrl Pts',(9.35434862995754,12.2,-6.64597524829023));
#177064=CARTESIAN_POINT('Ctrl Pts',(9.35190790041681,12.2,-6.64155397851797));
#177065=CARTESIAN_POINT('Ctrl Pts',(9.34946618061699,12.2,-6.63714676338981));
#177066=CARTESIAN_POINT('Ctrl Pts',(9.34763489093348,12.2,-6.63384135234392));
#177067=CARTESIAN_POINT('Ctrl Pts',(9.34580304503337,12.2,-6.63054384819711));
#177068=CARTESIAN_POINT('Ctrl Pts',(9.34397068726661,12.2,-6.62725426952495));
#177069=CARTESIAN_POINT('Ctrl Pts',(9.34213832949985,12.2,-6.6239646908528));
#177070=CARTESIAN_POINT('Ctrl Pts',(9.34030545849978,12.2,-6.62068303577201));
#177071=CARTESIAN_POINT('Ctrl Pts',(9.33847210923311,12.2,-6.61740932059859));
#177072=CARTESIAN_POINT('Ctrl Pts',(9.33663875996642,12.2,-6.61413560542518));
#177073=CARTESIAN_POINT('Ctrl Pts',(9.33480493264643,12.2,-6.61086982894232));
#177074=CARTESIAN_POINT('Ctrl Pts',(9.3329706613715,12.2,-6.60761200614702));
#177075=CARTESIAN_POINT('Ctrl Pts',(9.33052496611611,12.2,-6.6032682420254));
#177076=CARTESIAN_POINT('Ctrl Pts',(9.32807848310274,12.2,-6.59893861734822));
#177077=CARTESIAN_POINT('Ctrl Pts',(9.32563130602488,12.2,-6.59462317144731));
#177078=CARTESIAN_POINT('Ctrl Pts',(9.32379592338321,12.2,-6.59138658731561));
#177079=CARTESIAN_POINT('Ctrl Pts',(9.32196015166656,12.2,-6.58815797756626));
#177080=CARTESIAN_POINT('Ctrl Pts',(9.32012402748328,12.2,-6.58493735897495));
#177081=CARTESIAN_POINT('Ctrl Pts',(9.3182879033,12.2,-6.58171674038365));
#177082=CARTESIAN_POINT('Ctrl Pts',(9.3164514276334,12.2,-6.57850411301701));
#177083=CARTESIAN_POINT('Ctrl Pts',(9.31461463795015,12.2,-6.57529949138273));
#177084=CARTESIAN_POINT('Ctrl Pts',(9.3127778482669,12.2,-6.57209486974845));
#177085=CARTESIAN_POINT('Ctrl Pts',(9.31094074536376,12.2,-6.56889825344464));
#177086=CARTESIAN_POINT('Ctrl Pts',(9.30910336658877,12.2,-6.56570965960862));
#177087=CARTESIAN_POINT('Ctrl Pts',(9.30726598781377,12.2,-6.5625210657726));
#177088=CARTESIAN_POINT('Ctrl Pts',(9.30542833415045,12.2,-6.55934049282739));
#177089=CARTESIAN_POINT('Ctrl Pts',(9.30359044492561,12.2,-6.55616795719158));
#177090=CARTESIAN_POINT('Ctrl Pts',(9.30175255536688,12.2,-6.55299542097943));
#177091=CARTESIAN_POINT('Ctrl Pts',(9.29991442963305,12.2,-6.54983092153616));
#177092=CARTESIAN_POINT('Ctrl Pts',(9.29807610807419,12.2,-6.54667447532853));
#177093=CARTESIAN_POINT('Ctrl Pts',(9.29623778684929,12.2,-6.54351802969431));
#177094=CARTESIAN_POINT('Ctrl Pts',(9.29439926901607,12.2,-6.54036963617634));
#177095=CARTESIAN_POINT('Ctrl Pts',(9.29256059479119,12.2,-6.53722931062446));
#177096=CARTESIAN_POINT('Ctrl Pts',(9.29072192056631,12.2,-6.53408898507259));
#177097=CARTESIAN_POINT('Ctrl Pts',(9.28888308963982,12.2,-6.53095672834776));
#177098=CARTESIAN_POINT('Ctrl Pts',(9.28704414048994,12.2,-6.52783255423879));
#177099=CARTESIAN_POINT('Ctrl Pts',(9.28520519134007,12.2,-6.52470838012981));
#177100=CARTESIAN_POINT('Ctrl Pts',(9.28336612552649,12.2,-6.52159228863737));
#177101=CARTESIAN_POINT('Ctrl Pts',(9.28152698279328,12.2,-6.51848429698611));
#177102=CARTESIAN_POINT('Ctrl Pts',(9.27968784006007,12.2,-6.51537630533485));
#177103=CARTESIAN_POINT('Ctrl Pts',(9.27784861965025,12.2,-6.51227641245879));
#177104=CARTESIAN_POINT('Ctrl Pts',(9.27600936296709,12.2,-6.50918463382044));
#177105=CARTESIAN_POINT('Ctrl Pts',(9.27417010628393,12.2,-6.50609285518209));
#177106=CARTESIAN_POINT('Ctrl Pts',(9.27233081336741,12.2,-6.50300919034312));
#177107=CARTESIAN_POINT('Ctrl Pts',(9.27049152368424,12.2,-6.4999336556621));
#177108=CARTESIAN_POINT('Ctrl Pts',(9.26865223366693,12.2,-6.49685812042235));
#177109=CARTESIAN_POINT('Ctrl Pts',(9.26681294661628,12.2,-6.49379071430988));
#177110=CARTESIAN_POINT('Ctrl Pts',(9.26497370509899,12.2,-6.49073145361638));
#177111=CARTESIAN_POINT('Ctrl Pts',(9.26313446391583,12.2,-6.48767219347865));
#177112=CARTESIAN_POINT('Ctrl Pts',(9.26129526689933,12.2,-6.48462107830714));
#177113=CARTESIAN_POINT('Ctrl Pts',(9.25945615571615,12.2,-6.48157812366841));
#177114=CARTESIAN_POINT('Ctrl Pts',(9.25761704453297,12.2,-6.47853516902967));
#177115=CARTESIAN_POINT('Ctrl Pts',(9.25577801897314,12.2,-6.47550037416762));
#177116=CARTESIAN_POINT('Ctrl Pts',(9.25393912023994,12.2,-6.47247375551388));
#177117=CARTESIAN_POINT('Ctrl Pts',(9.25210022150674,12.2,-6.46944713686013));
#177118=CARTESIAN_POINT('Ctrl Pts',(9.25026144900983,12.2,-6.46642869284037));
#177119=CARTESIAN_POINT('Ctrl Pts',(9.24842284623495,12.2,-6.46341844068603));
#177120=CARTESIAN_POINT('Ctrl Pts',(9.24658424346006,12.2,-6.46040818853168));
#177121=CARTESIAN_POINT('Ctrl Pts',(9.24474580843353,12.2,-6.45740612773502));
#177122=CARTESIAN_POINT('Ctrl Pts',(9.24290758420865,12.2,-6.45441227263476));
#177123=CARTESIAN_POINT('Ctrl Pts',(9.24045661835284,12.2,-6.45042046547183));
#177124=CARTESIAN_POINT('Ctrl Pts',(9.23800602642203,12.2,-6.44644324800782));
#177125=CARTESIAN_POINT('Ctrl Pts',(9.23555590806632,12.2,-6.44248065545949));
#177126=CARTESIAN_POINT('Ctrl Pts',(9.23371831946645,12.2,-6.43950871131819));
#177127=CARTESIAN_POINT('Ctrl Pts',(9.23188099760653,12.2,-6.4365449925866));
#177128=CARTESIAN_POINT('Ctrl Pts',(9.23004398449828,12.2,-6.43358951697227));
#177129=CARTESIAN_POINT('Ctrl Pts',(9.22820697139002,12.2,-6.43063404135795));
#177130=CARTESIAN_POINT('Ctrl Pts',(9.22637026742656,12.2,-6.42768680775923));
#177131=CARTESIAN_POINT('Ctrl Pts',(9.22453391573494,12.2,-6.42474783068596));
#177132=CARTESIAN_POINT('Ctrl Pts',(9.22269756404333,12.2,-6.4218088536127));
#177133=CARTESIAN_POINT('Ctrl Pts',(9.2208615633667,12.2,-6.41887813421319));
#177134=CARTESIAN_POINT('Ctrl Pts',(9.21902595818336,12.2,-6.41595568706864));
#177135=CARTESIAN_POINT('Ctrl Pts',(9.21657848438326,12.2,-6.41205909052198));
#177136=CARTESIAN_POINT('Ctrl Pts',(9.21413171143324,12.2,-6.4081772008993));
#177137=CARTESIAN_POINT('Ctrl Pts',(9.21168574429999,12.2,-6.40431005313396));
#177138=CARTESIAN_POINT('Ctrl Pts',(9.20985126911668,12.2,-6.4014096925734));
#177139=CARTESIAN_POINT('Ctrl Pts',(9.20801724635665,12.2,-6.39851762520561));
#177140=CARTESIAN_POINT('Ctrl Pts',(9.20618371974827,12.2,-6.39563386550567));
#177141=CARTESIAN_POINT('Ctrl Pts',(9.20435019313991,12.2,-6.39275010580573));
#177142=CARTESIAN_POINT('Ctrl Pts',(9.20251716287668,12.2,-6.38987465241145));
#177143=CARTESIAN_POINT('Ctrl Pts',(9.2006846732266,12.2,-6.38700752325256));
#177144=CARTESIAN_POINT('Ctrl Pts',(9.19885218357653,12.2,-6.38414039409368));
#177145=CARTESIAN_POINT('Ctrl Pts',(9.19702023376641,12.2,-6.38128158839129));
#177146=CARTESIAN_POINT('Ctrl Pts',(9.1951888687079,12.2,-6.37843111982747));
#177147=CARTESIAN_POINT('Ctrl Pts',(9.1933575036494,12.2,-6.37558065126365));
#177148=CARTESIAN_POINT('Ctrl Pts',(9.19152672411584,12.2,-6.37273852131591));
#177149=CARTESIAN_POINT('Ctrl Pts',(9.18969657259892,12.2,-6.36990474462607));
#177150=CARTESIAN_POINT('Ctrl Pts',(9.18786642074951,12.2,-6.36707096742142));
#177151=CARTESIAN_POINT('Ctrl Pts',(9.18603689851695,12.2,-6.36424554219412));
#177152=CARTESIAN_POINT('Ctrl Pts',(9.18420805008458,12.2,-6.36142848691084));
#177153=CARTESIAN_POINT('Ctrl Pts',(9.18237920198445,12.2,-6.35861143213933));
#177154=CARTESIAN_POINT('Ctrl Pts',(9.18055102833788,12.2,-6.35580274404545));
#177155=CARTESIAN_POINT('Ctrl Pts',(9.17872357318804,12.2,-6.35300244071658));
#177156=CARTESIAN_POINT('Ctrl Pts',(9.17689611803822,12.2,-6.35020213738771));
#177157=CARTESIAN_POINT('Ctrl Pts',(9.17506938258452,12.2,-6.34741021782817));
#177158=CARTESIAN_POINT('Ctrl Pts',(9.17324341106759,12.2,-6.34462669622169));
#177159=CARTESIAN_POINT('Ctrl Pts',(9.17080878248892,12.2,-6.34091533424828));
#177160=CARTESIAN_POINT('Ctrl Pts',(9.16837551464056,12.2,-6.33721890270524));
#177161=CARTESIAN_POINT('Ctrl Pts',(9.16594371333921,12.2,-6.33353743739355));
#177162=CARTESIAN_POINT('Ctrl Pts',(9.16351191170653,12.2,-6.32985597158027));
#177163=CARTESIAN_POINT('Ctrl Pts',(9.1610815784,12.2,-6.32618947176022));
#177164=CARTESIAN_POINT('Ctrl Pts',(9.15865282275661,12.2,-6.32253797448913));
#177165=CARTESIAN_POINT('Ctrl Pts',(9.15622406744414,12.2,-6.31888647771557));
#177166=CARTESIAN_POINT('Ctrl Pts',(9.15379688862335,12.2,-6.3152499817614));
#177167=CARTESIAN_POINT('Ctrl Pts',(9.15137139865484,12.2,-6.31162852433374));
#177168=CARTESIAN_POINT('Ctrl Pts',(9.14894590835584,12.2,-6.30800706641266));
#177169=CARTESIAN_POINT('Ctrl Pts',(9.14652210610415,12.2,-6.30440064520123));
#177170=CARTESIAN_POINT('Ctrl Pts',(9.14410010374994,12.2,-6.30080929678329));
#177171=CARTESIAN_POINT('Ctrl Pts',(9.14167810139572,12.2,-6.29721794836534));
#177172=CARTESIAN_POINT('Ctrl Pts',(9.13925789893337,12.2,-6.29364167321581));
#177173=CARTESIAN_POINT('Ctrl Pts',(9.13683960807955,12.2,-6.29008050613438));
#177174=CARTESIAN_POINT('Ctrl Pts',(9.13442131755522,12.2,-6.28651933953817));
#177175=CARTESIAN_POINT('Ctrl Pts',(9.13200493997352,12.2,-6.28297328152702));
#177176=CARTESIAN_POINT('Ctrl Pts',(9.12959058799325,12.2,-6.27944236674403));
#177177=CARTESIAN_POINT('Ctrl Pts',(9.12717623568403,12.2,-6.27591145147995));
#177178=CARTESIAN_POINT('Ctrl Pts',(9.12476390969812,12.2,-6.27239567950574));
#177179=CARTESIAN_POINT('Ctrl Pts',(9.12235372412254,12.2,-6.26889508642761));
#177180=CARTESIAN_POINT('Ctrl Pts',(9.11994353887535,12.2,-6.26539449382644));
#177181=CARTESIAN_POINT('Ctrl Pts',(9.11753549456399,12.2,-6.26190908019832));
#177182=CARTESIAN_POINT('Ctrl Pts',(9.11512970670496,12.2,-6.25843888075878));
#177183=CARTESIAN_POINT('Ctrl Pts',(9.11212247163533,12.2,-6.25410113110475));
#177184=CARTESIAN_POINT('Ctrl Pts',(9.10911876219854,12.2,-6.24978715336073));
#177185=CARTESIAN_POINT('Ctrl Pts',(9.1061188078099,12.2,-6.24549701549396));
#177186=CARTESIAN_POINT('Ctrl Pts',(9.10371884416819,12.2,-6.24206490501349));
#177187=CARTESIAN_POINT('Ctrl Pts',(9.10132128278861,12.2,-6.23864805254152));
#177188=CARTESIAN_POINT('Ctrl Pts',(9.09892624265835,12.2,-6.2352464939688));
#177189=CARTESIAN_POINT('Ctrl Pts',(9.0965312028544,12.2,-6.23184493585956));
#177190=CARTESIAN_POINT('Ctrl Pts',(9.09413868484457,12.2,-6.22845866894833));
#177191=CARTESIAN_POINT('Ctrl Pts',(9.09174880692867,12.2,-6.22508773150067));
#177192=CARTESIAN_POINT('Ctrl Pts',(9.08876145928956,12.2,-6.22087405934664));
#177193=CARTESIAN_POINT('Ctrl Pts',(9.08577823754842,12.2,-6.21668433514341));
#177194=CARTESIAN_POINT('Ctrl Pts',(9.08279937753489,12.2,-6.21251863123556));
#177195=CARTESIAN_POINT('Ctrl Pts',(9.08041628939419,12.2,-6.20918606792766));
#177196=CARTESIAN_POINT('Ctrl Pts',(9.07803599382661,12.2,-6.20586887534404));
#177197=CARTESIAN_POINT('Ctrl Pts',(9.07565861041957,12.2,-6.20256708894346));
#177198=CARTESIAN_POINT('Ctrl Pts',(9.07328122733644,12.2,-6.19926530299274));
#177199=CARTESIAN_POINT('Ctrl Pts',(9.07090675886684,12.2,-6.19597892428445));
#177200=CARTESIAN_POINT('Ctrl Pts',(9.06853532639383,12.2,-6.1927079862175));
#177201=CARTESIAN_POINT('Ctrl Pts',(9.06616389359771,12.2,-6.18943704770488));
#177202=CARTESIAN_POINT('Ctrl Pts',(9.06379549831308,12.2,-6.18618155116913));
#177203=CARTESIAN_POINT('Ctrl Pts',(9.06143026407328,12.2,-6.18294152949357));
#177204=CARTESIAN_POINT('Ctrl Pts',(9.05906503015573,12.2,-6.17970150825946));
#177205=CARTESIAN_POINT('Ctrl Pts',(9.05670295672863,12.2,-6.17647696359835));
#177206=CARTESIAN_POINT('Ctrl Pts',(9.05434417135889,12.2,-6.17326792869902));
#177207=CARTESIAN_POINT('Ctrl Pts',(9.05198538566777,12.2,-6.17005889336246));
#177208=CARTESIAN_POINT('Ctrl Pts',(9.04962988622175,12.2,-6.16686536822637));
#177209=CARTESIAN_POINT('Ctrl Pts',(9.04727780081601,12.2,-6.16368738899864));
#177210=CARTESIAN_POINT('Ctrl Pts',(9.04492571573076,12.2,-6.1605094102039));
#177211=CARTESIAN_POINT('Ctrl Pts',(9.04257704504476,12.2,-6.15734697499212));
#177212=CARTESIAN_POINT('Ctrl Pts',(9.04023191595836,12.2,-6.15420012024781));
#177213=CARTESIAN_POINT('Ctrl Pts',(9.03788678655243,12.2,-6.15105326507474));
#177214=CARTESIAN_POINT('Ctrl Pts',(9.0355451993808,12.2,-6.14792198943451));
#177215=CARTESIAN_POINT('Ctrl Pts',(9.033207284465,12.2,-6.14480632697283));
#177216=CARTESIAN_POINT('Ctrl Pts',(9.03086936986776,12.2,-6.14169066493567));
#177217=CARTESIAN_POINT('Ctrl Pts',(9.02853512596027,12.2,-6.13859061769259));
#177218=CARTESIAN_POINT('Ctrl Pts',(9.02620468487263,12.2,-6.13550621772093));
#177219=CARTESIAN_POINT('Ctrl Pts',(9.02387424346746,12.2,-6.13242181732903));
#177220=CARTESIAN_POINT('Ctrl Pts',(9.02154760538484,12.2,-6.12935306601911));
#177221=CARTESIAN_POINT('Ctrl Pts',(9.01922490075826,12.2,-6.12629999624162));
#177222=CARTESIAN_POINT('Ctrl Pts',(9.01690219613168,12.2,-6.12324692646413));
#177223=CARTESIAN_POINT('Ctrl Pts',(9.01458342800276,12.2,-6.12020953982454));
#177224=CARTESIAN_POINT('Ctrl Pts',(9.01226872665481,12.2,-6.11718786877259));
#177225=CARTESIAN_POINT('Ctrl Pts',(9.00995402562225,12.2,-6.11416619813234));
#177226=CARTESIAN_POINT('Ctrl Pts',(9.00764339237899,12.2,-6.11116024455174));
#177227=CARTESIAN_POINT('Ctrl Pts',(9.00533696266817,12.2,-6.108170041727));
#177228=CARTESIAN_POINT('Ctrl Pts',(9.00303053264308,12.2,-6.10517983849484));
#177229=CARTESIAN_POINT('Ctrl Pts',(9.00072830672124,12.2,-6.10220538530919));
#177230=CARTESIAN_POINT('Ctrl Pts',(8.99843041937422,12.2,-6.09924671748288));
#177231=CARTESIAN_POINT('Ctrl Pts',(8.9961325323403,12.2,-6.0962880500597));
#177232=CARTESIAN_POINT('Ctrl Pts',(8.99383898375026,12.2,-6.09334516611781));
#177233=CARTESIAN_POINT('Ctrl Pts',(8.9915499139371,12.2,-6.09041810202272));
#177234=CARTESIAN_POINT('Ctrl Pts',(8.98926084381204,12.2,-6.08749103752882));
#177235=CARTESIAN_POINT('Ctrl Pts',(8.9869762501652,12.2,-6.08457979173375));
#177236=CARTESIAN_POINT('Ctrl Pts',(8.98469627342745,12.2,-6.08168439782157));
#177237=CARTESIAN_POINT('Ctrl Pts',(8.98241629700034,12.2,-6.07878900430389));
#177238=CARTESIAN_POINT('Ctrl Pts',(8.98014093700583,12.2,-6.07590946292891));
#177239=CARTESIAN_POINT('Ctrl Pts',(8.97787033396893,12.2,-6.07304580871754));
#177240=CARTESIAN_POINT('Ctrl Pts',(8.97559973062265,12.2,-6.070182154116));
#177241=CARTESIAN_POINT('Ctrl Pts',(8.9733338853686,12.2,-6.06733438398857));
#177242=CARTESIAN_POINT('Ctrl Pts',(8.9710729388568,12.2,-6.06450253550193));
#177243=CARTESIAN_POINT('Ctrl Pts',(8.96881199265306,12.2,-6.06167068740113));
#177244=CARTESIAN_POINT('Ctrl Pts',(8.96655594658323,12.2,-6.05885475911592));
#177245=CARTESIAN_POINT('Ctrl Pts',(8.96430494287659,12.2,-6.05605478414801));
#177246=CARTESIAN_POINT('Ctrl Pts',(8.96205393886325,12.2,-6.0532548087986));
#177247=CARTESIAN_POINT('Ctrl Pts',(8.95980797960246,12.2,-6.05047078679032));
#177248=CARTESIAN_POINT('Ctrl Pts',(8.95756720709179,12.2,-6.04770275230715));
#177249=CARTESIAN_POINT('Ctrl Pts',(8.95532643488641,12.2,-6.04493471820114));
#177250=CARTESIAN_POINT('Ctrl Pts',(8.95309085259114,12.2,-6.04218267060583));
#177251=CARTESIAN_POINT('Ctrl Pts',(8.95086060560624,12.2,-6.03944664443897));
#177252=CARTESIAN_POINT('Ctrl Pts',(8.94863035831747,12.2,-6.03671061789931));
#177253=CARTESIAN_POINT('Ctrl Pts',(8.9464054465211,12.2,-6.03399061088827));
#177254=CARTESIAN_POINT('Ctrl Pts',(8.94418601922341,12.2,-6.03128665900645));
#177255=CARTESIAN_POINT('Ctrl Pts',(8.94196659222811,12.2,-6.02858270749303));
#177256=CARTESIAN_POINT('Ctrl Pts',(8.93975264792269,12.2,-6.02589480897279));
#177257=CARTESIAN_POINT('Ctrl Pts',(8.93754433960266,12.2,-6.02322299824515));
#177258=CARTESIAN_POINT('Ctrl Pts',(8.93533603098175,12.2,-6.02055118715346));
#177259=CARTESIAN_POINT('Ctrl Pts',(8.93313335667242,12.2,-6.01789546329379));
#177260=CARTESIAN_POINT('Ctrl Pts',(8.93093646827492,12.2,-6.01525585948327));
#177261=CARTESIAN_POINT('Ctrl Pts',(8.92873957987742,12.2,-6.01261625567276));
#177262=CARTESIAN_POINT('Ctrl Pts',(8.92654847958058,12.2,-6.00999277340856));
#177263=CARTESIAN_POINT('Ctrl Pts',(8.92436331785097,12.2,-6.00738544482365));
#177264=CARTESIAN_POINT('Ctrl Pts',(8.92217815641909,12.2,-6.00477811659399));
#177265=CARTESIAN_POINT('Ctrl Pts',(8.91999893565585,12.2,-6.00218693964183));
#177266=CARTESIAN_POINT('Ctrl Pts',(8.91782581126807,12.2,-5.99961195095171));
#177267=CARTESIAN_POINT('Ctrl Pts',(8.91565268658419,12.2,-5.99703696191074));
#177268=CARTESIAN_POINT('Ctrl Pts',(8.91348565573319,12.2,-5.99447815979893));
#177269=CARTESIAN_POINT('Ctrl Pts',(8.91132487867164,12.2,-5.99193557788425));
#177270=CARTESIAN_POINT('Ctrl Pts',(8.9086239074919,12.2,-5.98875735066412));
#177271=CARTESIAN_POINT('Ctrl Pts',(8.90593270769286,12.2,-5.9856044650777));
#177272=CARTESIAN_POINT('Ctrl Pts',(8.90325158741589,12.2,-5.98247698785755));
#177273=CARTESIAN_POINT('Ctrl Pts',(8.90057046743118,12.2,-5.97934951097829));
#177274=CARTESIAN_POINT('Ctrl Pts',(8.89789943027546,12.2,-5.97624744051913));
#177275=CARTESIAN_POINT('Ctrl Pts',(8.8952387893146,12.2,-5.97317084210238));
#177276=CARTESIAN_POINT('Ctrl Pts',(8.89257814806374,12.2,-5.97009424335028));
#177277=CARTESIAN_POINT('Ctrl Pts',(8.88992790358494,12.2,-5.96704311665336));
#177278=CARTESIAN_POINT('Ctrl Pts',(8.88728837657017,12.2,-5.96401752463737));
#177279=CARTESIAN_POINT('Ctrl Pts',(8.8846488495554,12.2,-5.96099193262139));
#177280=CARTESIAN_POINT('Ctrl Pts',(8.88202004040435,12.2,-5.95799187684668));
#177281=CARTESIAN_POINT('Ctrl Pts',(8.87940227429232,12.2,-5.95501741816402));
#177282=CARTESIAN_POINT('Ctrl Pts',(8.87678450818029,12.2,-5.95204295948134));
#177283=CARTESIAN_POINT('Ctrl Pts',(8.87417778491502,12.2,-5.94909410132054));
#177284=CARTESIAN_POINT('Ctrl Pts',(8.87158243457623,12.2,-5.94617090408938));
#177285=CARTESIAN_POINT('Ctrl Pts',(8.86898708423745,12.2,-5.94324770685821));
#177286=CARTESIAN_POINT('Ctrl Pts',(8.86640310791324,12.2,-5.94035017228924));
#177287=CARTESIAN_POINT('Ctrl Pts',(8.86383083867653,12.2,-5.93747836270457));
#177288=CARTESIAN_POINT('Ctrl Pts',(8.86125856943983,12.2,-5.93460655311991));
#177289=CARTESIAN_POINT('Ctrl Pts',(8.8586980100784,12.2,-5.93176046984146));
#177290=CARTESIAN_POINT('Ctrl Pts',(8.85614949917499,12.2,-5.92894017365955));
#177291=CARTESIAN_POINT('Ctrl Pts',(8.85360098827159,12.2,-5.92611987747765));
#177292=CARTESIAN_POINT('Ctrl Pts',(8.85106452702945,12.2,-5.9233253703252));
#177293=CARTESIAN_POINT('Ctrl Pts',(8.8485404609763,12.2,-5.92055671399313));
#177294=CARTESIAN_POINT('Ctrl Pts',(8.84601639492315,12.2,-5.91778805766107));
#177295=CARTESIAN_POINT('Ctrl Pts',(8.84350472337769,12.2,-5.91504525183329));
#177296=CARTESIAN_POINT('Ctrl Pts',(8.84100579976657,12.2,-5.91232835974994));
#177297=CARTESIAN_POINT('Ctrl Pts',(8.83850687615545,12.2,-5.9096114676666));
#177298=CARTESIAN_POINT('Ctrl Pts',(8.83602069835975,12.2,-5.90692048936608));
#177299=CARTESIAN_POINT('Ctrl Pts',(8.8335476248069,12.2,-5.90425548650684));
#177300=CARTESIAN_POINT('Ctrl Pts',(8.83107455125404,12.2,-5.90159048364759));
#177301=CARTESIAN_POINT('Ctrl Pts',(8.82861458132818,12.2,-5.89895145737786));
#177302=CARTESIAN_POINT('Ctrl Pts',(8.82616807806498,12.2,-5.89633846862921));
#177303=CARTESIAN_POINT('Ctrl Pts',(8.8237215748018,12.2,-5.89372547988056));
#177304=CARTESIAN_POINT('Ctrl Pts',(8.82128854006328,12.2,-5.89113852900349));
#177305=CARTESIAN_POINT('Ctrl Pts',(8.81886933930011,12.2,-5.8885776778243));
#177306=CARTESIAN_POINT('Ctrl Pts',(8.81645013853696,12.2,-5.88601682664509));
#177307=CARTESIAN_POINT('Ctrl Pts',(8.81404477541309,12.2,-5.88348207592123));
#177308=CARTESIAN_POINT('Ctrl Pts',(8.81165362203072,12.2,-5.8809734854505));
#177309=CARTESIAN_POINT('Ctrl Pts',(8.80926246864835,12.2,-5.87846489497977));
#177310=CARTESIAN_POINT('Ctrl Pts',(8.80688552581751,12.2,-5.87598246742099));
#177311=CARTESIAN_POINT('Ctrl Pts',(8.80452317741592,12.2,-5.87352626193703));
#177312=CARTESIAN_POINT('Ctrl Pts',(8.80216082901434,12.2,-5.87107005645307));
#177313=CARTESIAN_POINT('Ctrl Pts',(8.79981307044913,12.2,-5.86864007366674));
#177314=CARTESIAN_POINT('Ctrl Pts',(8.79748029468645,12.2,-5.86623637491888));
#177315=CARTESIAN_POINT('Ctrl Pts',(8.79468096387296,12.2,-5.86335193652626));
#177316=CARTESIAN_POINT('Ctrl Pts',(8.79190320452374,12.2,-5.86050534698501));
#177317=CARTESIAN_POINT('Ctrl Pts',(8.78914769987482,12.2,-5.8576967133387));
#177318=CARTESIAN_POINT('Ctrl Pts',(8.7863921952259,12.2,-5.85488807969241));
#177319=CARTESIAN_POINT('Ctrl Pts',(8.7836589462919,12.2,-5.85211739944306));
#177320=CARTESIAN_POINT('Ctrl Pts',(8.78094864963938,12.2,-5.84938477812404));
#177321=CARTESIAN_POINT('Ctrl Pts',(8.77823835298686,12.2,-5.846652156805));
#177322=CARTESIAN_POINT('Ctrl Pts',(8.77555101007843,12.2,-5.84395759571227));
#177323=CARTESIAN_POINT('Ctrl Pts',(8.77288733250692,12.2,-5.84130119830617));
#177324=CARTESIAN_POINT('Ctrl Pts',(8.77022365469345,12.2,-5.83864480065879));
#177325=CARTESIAN_POINT('Ctrl Pts',(8.76758364238227,12.2,-5.83602656706512));
#177326=CARTESIAN_POINT('Ctrl Pts',(8.76496802457412,12.2,-5.83344660059284));
#177327=CARTESIAN_POINT('Ctrl Pts',(8.76235240700355,12.2,-5.8308666343549));
#177328=CARTESIAN_POINT('Ctrl Pts',(8.75976118361121,12.2,-5.8283249376216));
#177329=CARTESIAN_POINT('Ctrl Pts',(8.75719509827607,12.2,-5.82582161120109));
#177330=CARTESIAN_POINT('Ctrl Pts',(8.75462901294091,12.2,-5.82331828478057));
#177331=CARTESIAN_POINT('Ctrl Pts',(8.75208806602611,12.2,-5.82085332991225));
#177332=CARTESIAN_POINT('Ctrl Pts',(8.74957302053237,12.2,-5.81842684949777));
#177333=CARTESIAN_POINT('Ctrl Pts',(8.74705797481019,12.2,-5.8160003688629));
#177334=CARTESIAN_POINT('Ctrl Pts',(8.74456882674242,12.2,-5.8136123627076));
#177335=CARTESIAN_POINT('Ctrl Pts',(8.74210635907009,12.2,-5.81126293404777));
#177336=CARTESIAN_POINT('Ctrl Pts',(8.73964389162143,12.2,-5.80891350560134));
#177337=CARTESIAN_POINT('Ctrl Pts',(8.73720810353741,12.2,-5.80660265445907));
#177338=CARTESIAN_POINT('Ctrl Pts',(8.73479978954156,12.2,-5.80433048295828));
#177339=CARTESIAN_POINT('Ctrl Pts',(8.7323914755457,12.2,-5.80205831145748));
#177340=CARTESIAN_POINT('Ctrl Pts',(8.73001063855613,12.2,-5.79982482057042));
#177341=CARTESIAN_POINT('Ctrl Pts',(8.72765809147299,12.2,-5.79763010923084));
#177342=CARTESIAN_POINT('Ctrl Pts',(8.72530554417617,12.2,-5.79543539769191));
#177343=CARTESIAN_POINT('Ctrl Pts',(8.722981290316,12.2,-5.79327946874748));
#177344=CARTESIAN_POINT('Ctrl Pts',(8.72068616107794,12.2,-5.79116242202858));
#177345=CARTESIAN_POINT('Ctrl Pts',(8.71839103204836,12.2,-5.78904537550198));
#177346=CARTESIAN_POINT('Ctrl Pts',(8.71612503018531,12.2,-5.78696721198419));
#177347=CARTESIAN_POINT('Ctrl Pts',(8.71388901126655,12.2,-5.78492803247494));
#177348=CARTESIAN_POINT('Ctrl Pts',(8.71165299234779,12.2,-5.7828888529657));
#177349=CARTESIAN_POINT('Ctrl Pts',(8.70944695698349,12.2,-5.78088865674373));
#177350=CARTESIAN_POINT('Ctrl Pts',(8.70727177920206,12.2,-5.77892754513143));
#177351=CARTESIAN_POINT('Ctrl Pts',(8.70509660122307,12.2,-5.77696643334098));
#177352=CARTESIAN_POINT('Ctrl Pts',(8.70295228519926,12.2,-5.77504440721966));
#177353=CARTESIAN_POINT('Ctrl Pts',(8.70083972725296,12.2,-5.77316156453639));
#177354=CARTESIAN_POINT('Ctrl Pts',(8.69872716949857,12.2,-5.77127872202416));
#177355=CARTESIAN_POINT('Ctrl Pts',(8.69664637075043,12.2,-5.76943506533334));
#177356=CARTESIAN_POINT('Ctrl Pts',(8.6945982549823,12.2,-5.76763069197414));
#177357=CARTESIAN_POINT('Ctrl Pts',(8.69255013921417,12.2,-5.76582631861494));
#177358=CARTESIAN_POINT('Ctrl Pts',(8.69053470500416,12.2,-5.76406123129984));
#177359=CARTESIAN_POINT('Ctrl Pts',(8.6885528995747,12.2,-5.76233552686083));
#177360=CARTESIAN_POINT('Ctrl Pts',(8.68657109396523,12.2,-5.76060982226505));
#177361=CARTESIAN_POINT('Ctrl Pts',(8.68462291897657,12.2,-5.75892350165751));
#177362=CARTESIAN_POINT('Ctrl Pts',(8.68270934454132,12.2,-5.75727666507045));
#177363=CARTESIAN_POINT('Ctrl Pts',(8.68079577027988,12.2,-5.75562982863299));
#177364=CARTESIAN_POINT('Ctrl Pts',(8.67891679728105,12.2,-5.75402247583932));
#177365=CARTESIAN_POINT('Ctrl Pts',(8.6770734251829,12.2,-5.752454704398));
#177366=CARTESIAN_POINT('Ctrl Pts',(8.67523005308474,12.2,-5.75088693295667));
#177367=CARTESIAN_POINT('Ctrl Pts',(8.67342228175881,12.2,-5.7493587457039));
#177368=CARTESIAN_POINT('Ctrl Pts',(8.67165113857156,12.2,-5.74787023733957));
#177369=CARTESIAN_POINT('Ctrl Pts',(8.6698799953843,12.2,-5.74638172897523));
#177370=CARTESIAN_POINT('Ctrl Pts',(8.66814547946741,12.2,-5.74493290224673));
#177371=CARTESIAN_POINT('Ctrl Pts',(8.66644864744318,12.2,-5.74352385387854));
#177372=CARTESIAN_POINT('Ctrl Pts',(8.66475181526481,12.2,-5.74211480538238));
#177373=CARTESIAN_POINT('Ctrl Pts',(8.66309266594835,12.2,-5.74074553799837));
#177374=CARTESIAN_POINT('Ctrl Pts',(8.66147228886173,12.2,-5.73941614642766));
#177375=CARTESIAN_POINT('Ctrl Pts',(8.65985191192229,12.2,-5.7380867549777));
#177376=CARTESIAN_POINT('Ctrl Pts',(8.65827030394331,12.2,-5.7367972411942));
#177377=CARTESIAN_POINT('Ctrl Pts',(8.65672858624224,12.2,-5.73554770273385));
#177378=CARTESIAN_POINT('Ctrl Pts',(8.65416645576684,12.2,-5.73347113543021));
#177379=CARTESIAN_POINT('Ctrl Pts',(8.65171447039556,12.2,-5.73150496079906));
#177380=CARTESIAN_POINT('Ctrl Pts',(8.64937799899994,12.2,-5.72964966100002));
#177381=CARTESIAN_POINT('Ctrl Pts',(8.64937799899994,15.2,-5.72964966100002));
#177382=CARTESIAN_POINT('Ctrl Pts',(8.65077718280868,15.2,-5.73076069768724));
#177383=CARTESIAN_POINT('Ctrl Pts',(8.65221780094386,15.2,-5.73191150037687));
#177384=CARTESIAN_POINT('Ctrl Pts',(8.65369867906269,15.2,-5.73310195413624));
#177385=CARTESIAN_POINT('Ctrl Pts',(8.65518669872435,15.2,-5.73429814886537));
#177386=CARTESIAN_POINT('Ctrl Pts',(8.65671537265224,15.2,-5.73553438487953));
#177387=CARTESIAN_POINT('Ctrl Pts',(8.65828355965168,15.2,-5.7368105625985));
#177388=CARTESIAN_POINT('Ctrl Pts',(8.65985174650868,15.2,-5.73808674020155));
#177389=CARTESIAN_POINT('Ctrl Pts',(8.661459445618,15.2,-5.73940286101586));
#177390=CARTESIAN_POINT('Ctrl Pts',(8.66310555047487,15.2,-5.7407588264666));
#177391=CARTESIAN_POINT('Ctrl Pts',(8.66475165533174,15.2,-5.74211479191736));
#177392=CARTESIAN_POINT('Ctrl Pts',(8.66643616407876,15.2,-5.74351060148557));
#177393=CARTESIAN_POINT('Ctrl Pts',(8.66815800210007,15.2,-5.74494615808617));
#177394=CARTESIAN_POINT('Ctrl Pts',(8.66987984027778,15.2,-5.74638171481717));
#177395=CARTESIAN_POINT('Ctrl Pts',(8.67163900552859,15.2,-5.74785701772148));
#177396=CARTESIAN_POINT('Ctrl Pts',(8.67343445396226,15.2,-5.74937196839009));
#177397=CARTESIAN_POINT('Ctrl Pts',(8.67522990223283,15.2,-5.75088691892109));
#177398=CARTESIAN_POINT('Ctrl Pts',(8.67706163222665,15.2,-5.75244151822626));
#177399=CARTESIAN_POINT('Ctrl Pts',(8.67892862750073,15.2,-5.75403566675901));
#177400=CARTESIAN_POINT('Ctrl Pts',(8.6807956227748,15.2,-5.75562981529175));
#177401=CARTESIAN_POINT('Ctrl Pts',(8.68269788293301,15.2,-5.75726351191311));
#177402=CARTESIAN_POINT('Ctrl Pts',(8.68463441636115,15.2,-5.75893665943392));
#177403=CARTESIAN_POINT('Ctrl Pts',(8.6865709499652,15.2,-5.76060980710673));
#177404=CARTESIAN_POINT('Ctrl Pts',(8.68854176058186,15.2,-5.76232240563443));
#177405=CARTESIAN_POINT('Ctrl Pts',(8.69054587944334,15.2,-5.76407435514925));
#177406=CARTESIAN_POINT('Ctrl Pts',(8.69254999812279,15.2,-5.76582630450495));
#177407=CARTESIAN_POINT('Ctrl Pts',(8.6945874299783,15.2,-5.76761760521468));
#177408=CARTESIAN_POINT('Ctrl Pts',(8.6966572316545,15.2,-5.76944815581655));
#177409=CARTESIAN_POINT('Ctrl Pts',(8.69872703333071,15.2,-5.77127870641841));
#177410=CARTESIAN_POINT('Ctrl Pts',(8.7008292078793,15.2,-5.77314851140881));
#177411=CARTESIAN_POINT('Ctrl Pts',(8.70296283863374,15.2,-5.77505746492108));
#177412=CARTESIAN_POINT('Ctrl Pts',(8.70509646938817,15.2,-5.77696641843334));
#177413=CARTESIAN_POINT('Ctrl Pts',(8.70726155826744,15.2,-5.77891452511656));
#177414=CARTESIAN_POINT('Ctrl Pts',(8.7094572102689,15.2,-5.78090168079169));
#177415=CARTESIAN_POINT('Ctrl Pts',(8.7116528624698,15.2,-5.78288883664731));
#177416=CARTESIAN_POINT('Ctrl Pts',(8.71387908026539,15.2,-5.78491504540674));
#177417=CARTESIAN_POINT('Ctrl Pts',(8.71613499338963,15.2,-5.78698020310433));
#177418=CARTESIAN_POINT('Ctrl Pts',(8.71839090630897,15.2,-5.78904536061433));
#177419=CARTESIAN_POINT('Ctrl Pts',(8.72067651407248,15.2,-5.79114946853386));
#177420=CARTESIAN_POINT('Ctrl Pts',(8.72299096799885,15.2,-5.79329242596564));
#177421=CARTESIAN_POINT('Ctrl Pts',(8.72530542192521,15.2,-5.79543538339742));
#177422=CARTESIAN_POINT('Ctrl Pts',(8.72764872183785,15.2,-5.79761719044126));
#177423=CARTESIAN_POINT('Ctrl Pts',(8.73002003899976,15.2,-5.79983774302458));
#177424=CARTESIAN_POINT('Ctrl Pts',(8.73239135637707,15.2,-5.80205829580961));
#177425=CARTESIAN_POINT('Ctrl Pts',(8.73479068972382,15.2,-5.80431759758176));
#177426=CARTESIAN_POINT('Ctrl Pts',(8.73721723210726,15.2,-5.80661554437535));
#177427=CARTESIAN_POINT('Ctrl Pts',(8.73964377427027,15.2,-5.80891349096022));
#177428=CARTESIAN_POINT('Ctrl Pts',(8.74209752398602,15.2,-5.81125008257448));
#177429=CARTESIAN_POINT('Ctrl Pts',(8.74457769132377,15.2,-5.81362521799887));
#177430=CARTESIAN_POINT('Ctrl Pts',(8.74705785866152,15.2,-5.81600035342327));
#177431=CARTESIAN_POINT('Ctrl Pts',(8.74956444276769,15.2,-5.81841403198276));
#177432=CARTESIAN_POINT('Ctrl Pts',(8.75209667200723,15.2,-5.82086615047434));
#177433=CARTESIAN_POINT('Ctrl Pts',(8.75462890147678,15.2,-5.82331826918867));
#177434=CARTESIAN_POINT('Ctrl Pts',(8.75718677371192,15.2,-5.82580882879497));
#177435=CARTESIAN_POINT('Ctrl Pts',(8.75976953548314,15.2,-5.82833772472801));
#177436=CARTESIAN_POINT('Ctrl Pts',(8.76235229701977,15.2,-5.83086662043136));
#177437=CARTESIAN_POINT('Ctrl Pts',(8.76495994775387,15.2,-5.83343385342796));
#177438=CARTESIAN_POINT('Ctrl Pts',(8.76759174724156,15.2,-5.83603931899994));
#177439=CARTESIAN_POINT('Ctrl Pts',(8.77022354672925,15.2,-5.83864478457192));
#177440=CARTESIAN_POINT('Ctrl Pts',(8.7728794957223,15.2,-5.84128848395629));
#177441=CARTESIAN_POINT('Ctrl Pts',(8.7755588714241,15.2,-5.84397031249061));
#177442=CARTESIAN_POINT('Ctrl Pts',(8.77823824736928,15.2,-5.84665214126852));
#177443=CARTESIAN_POINT('Ctrl Pts',(8.78094105090526,15.2,-5.84937210003936));
#177444=CARTESIAN_POINT('Ctrl Pts',(8.78366657180533,15.2,-5.85213008177558));
#177445=CARTESIAN_POINT('Ctrl Pts',(8.78639209245782,15.2,-5.85488806326128));
#177446=CARTESIAN_POINT('Ctrl Pts',(8.78914033154752,15.2,-5.85768406944958));
#177447=CARTESIAN_POINT('Ctrl Pts',(8.7919105972095,15.2,-5.86051799577624));
#177448=CARTESIAN_POINT('Ctrl Pts',(8.79468086287148,15.2,-5.8633519221029));
#177449=CARTESIAN_POINT('Ctrl Pts',(8.7974731535415,15.2,-5.86622376756559));
#177450=CARTESIAN_POINT('Ctrl Pts',(8.80028679235499,15.2,-5.86913342612486));
#177451=CARTESIAN_POINT('Ctrl Pts',(8.80263149145141,15.2,-5.87155814167902));
#177452=CARTESIAN_POINT('Ctrl Pts',(8.80499101342884,15.2,-5.87400911785615));
#177453=CARTESIAN_POINT('Ctrl Pts',(8.80736497655307,15.2,-5.87648629160477));
#177454=CARTESIAN_POINT('Ctrl Pts',(8.8097389396773,15.2,-5.87896346535338));
#177455=CARTESIAN_POINT('Ctrl Pts',(8.81212734162106,15.2,-5.88146683840938));
#177456=CARTESIAN_POINT('Ctrl Pts',(8.8145298032986,15.2,-5.88399634724024));
#177457=CARTESIAN_POINT('Ctrl Pts',(8.81693226497614,15.2,-5.8865258560711));
#177458=CARTESIAN_POINT('Ctrl Pts',(8.81934878816102,15.2,-5.88908150223884));
#177459=CARTESIAN_POINT('Ctrl Pts',(8.82177899746658,15.2,-5.89166322272495));
#177460=CARTESIAN_POINT('Ctrl Pts',(8.82420920677214,15.2,-5.89424494321107));
#177461=CARTESIAN_POINT('Ctrl Pts',(8.82665310475672,15.2,-5.89685273952825));
#177462=CARTESIAN_POINT('Ctrl Pts',(8.82911032247625,15.2,-5.89948654898472));
#177463=CARTESIAN_POINT('Ctrl Pts',(8.83156754019577,15.2,-5.9021203584412));
#177464=CARTESIAN_POINT('Ctrl Pts',(8.83403808046173,15.2,-5.90478018119662));
#177465=CARTESIAN_POINT('Ctrl Pts',(8.83652158046241,15.2,-5.90746595418409));
#177466=CARTESIAN_POINT('Ctrl Pts',(8.83900508046309,15.2,-5.91015172717154));
#177467=CARTESIAN_POINT('Ctrl Pts',(8.8415015393023,15.2,-5.91286345222221));
#177468=CARTESIAN_POINT('Ctrl Pts',(8.84401060520575,15.2,-5.91560106444582));
#177469=CARTESIAN_POINT('Ctrl Pts',(8.8470214841805,15.2,-5.91888619899478));
#177470=CARTESIAN_POINT('Ctrl Pts',(8.85005051456211,15.2,-5.92220861444699));
#177471=CARTESIAN_POINT('Ctrl Pts',(8.85309709279853,15.2,-5.92556820075676));
#177472=CARTESIAN_POINT('Ctrl Pts',(8.85563590808779,15.2,-5.92836785611662));
#177473=CARTESIAN_POINT('Ctrl Pts',(8.85818691135547,15.2,-5.9311933250333));
#177474=CARTESIAN_POINT('Ctrl Pts',(8.86074975829991,15.2,-5.93404454378328));
#177475=CARTESIAN_POINT('Ctrl Pts',(8.86331260524433,15.2,-5.93689576253325));
#177476=CARTESIAN_POINT('Ctrl Pts',(8.86588729726176,15.2,-5.93977273306605));
#177477=CARTESIAN_POINT('Ctrl Pts',(8.86847349505133,15.2,-5.9426753894682));
#177478=CARTESIAN_POINT('Ctrl Pts',(8.8710596928409,15.2,-5.94557804587036));
#177479=CARTESIAN_POINT('Ctrl Pts',(8.87365739728669,15.2,-5.94850639163639));
#177480=CARTESIAN_POINT('Ctrl Pts',(8.87626627666227,15.2,-5.95146035969329));
#177481=CARTESIAN_POINT('Ctrl Pts',(8.87887515603786,15.2,-5.9544143277502));
#177482=CARTESIAN_POINT('Ctrl Pts',(8.88149520812149,15.2,-5.95739392271755));
#177483=CARTESIAN_POINT('Ctrl Pts',(8.88412610916371,15.2,-5.96039907570498));
#177484=CARTESIAN_POINT('Ctrl Pts',(8.88675701020592,15.2,-5.9634042286924));
#177485=CARTESIAN_POINT('Ctrl Pts',(8.88939875734511,15.2,-5.96643494299308));
#177486=CARTESIAN_POINT('Ctrl Pts',(8.89205103012344,15.2,-5.96949115417498));
#177487=CARTESIAN_POINT('Ctrl Pts',(8.89470330290178,15.2,-5.97254736535688));
#177488=CARTESIAN_POINT('Ctrl Pts',(8.89736609970933,15.2,-5.97562907340372));
#177489=CARTESIAN_POINT('Ctrl Pts',(8.90003910359358,15.2,-5.97873621481074));
#177490=CARTESIAN_POINT('Ctrl Pts',(8.90271210747784,15.2,-5.98184335621774));
#177491=CARTESIAN_POINT('Ctrl Pts',(8.90539531922359,15.2,-5.98497593143315));
#177492=CARTESIAN_POINT('Ctrl Pts',(8.90808842387718,15.2,-5.98813387442135));
#177493=CARTESIAN_POINT('Ctrl Pts',(8.91024290742391,15.2,-5.99066022860537));
#177494=CARTESIAN_POINT('Ctrl Pts',(8.91240372326427,15.2,-5.99320281839282));
#177495=CARTESIAN_POINT('Ctrl Pts',(8.91457071403116,15.2,-5.99576161234926));
#177496=CARTESIAN_POINT('Ctrl Pts',(8.91727945271122,15.2,-5.99896010505626));
#177497=CARTESIAN_POINT('Ctrl Pts',(8.91999783703608,15.2,-6.00218391423351));
#177498=CARTESIAN_POINT('Ctrl Pts',(8.92272556350677,15.2,-6.00543297778985));
#177499=CARTESIAN_POINT('Ctrl Pts',(8.92490774480225,15.2,-6.00803222877659));
#177500=CARTESIAN_POINT('Ctrl Pts',(8.92709590470514,15.2,-6.01064763930181));
#177501=CARTESIAN_POINT('Ctrl Pts',(8.9292898898253,15.2,-6.01327918044687));
#177502=CARTESIAN_POINT('Ctrl Pts',(8.93148387464653,15.2,-6.01591072123339));
#177503=CARTESIAN_POINT('Ctrl Pts',(8.93368368420034,15.2,-6.01855839143449));
#177504=CARTESIAN_POINT('Ctrl Pts',(8.93588916635301,15.2,-6.02122215621567));
#177505=CARTESIAN_POINT('Ctrl Pts',(8.93809464880617,15.2,-6.0238859213598));
#177506=CARTESIAN_POINT('Ctrl Pts',(8.94030580299235,15.2,-6.02656578285822));
#177507=CARTESIAN_POINT('Ctrl Pts',(8.94252247961327,15.2,-6.02926170614124));
#177508=CARTESIAN_POINT('Ctrl Pts',(8.94473915593218,15.2,-6.03195762905694));
#177509=CARTESIAN_POINT('Ctrl Pts',(8.94696135213644,15.2,-6.03466961418449));
#177510=CARTESIAN_POINT('Ctrl Pts',(8.94918892234288,15.2,-6.03739762829376));
#177511=CARTESIAN_POINT('Ctrl Pts',(8.95197338532854,15.2,-6.04080764620911));
#177512=CARTESIAN_POINT('Ctrl Pts',(8.95476624160609,15.2,-6.04424270939178));
#177513=CARTESIAN_POINT('Ctrl Pts',(8.95756720709179,15.2,-6.04770275230715));
#177514=CARTESIAN_POINT('Ctrl Pts',(8.95980797960246,15.2,-6.05047078679032));
#177515=CARTESIAN_POINT('Ctrl Pts',(8.96205393886324,15.2,-6.05325480879859));
#177516=CARTESIAN_POINT('Ctrl Pts',(8.96430494287659,15.2,-6.056054784148));
#177517=CARTESIAN_POINT('Ctrl Pts',(8.96655594658323,15.2,-6.05885475911592));
#177518=CARTESIAN_POINT('Ctrl Pts',(8.96881199265308,15.2,-6.06167068740115));
#177519=CARTESIAN_POINT('Ctrl Pts',(8.97107293885681,15.2,-6.06450253550193));
#177520=CARTESIAN_POINT('Ctrl Pts',(8.9738991218425,15.2,-6.06804234591729));
#177521=CARTESIAN_POINT('Ctrl Pts',(8.97673295931455,15.2,-6.07160703222221));
#177522=CARTESIAN_POINT('Ctrl Pts',(8.97957417577249,15.2,-6.07519652749868));
#177523=CARTESIAN_POINT('Ctrl Pts',(8.98184714906271,15.2,-6.07806812387637));
#177524=CARTESIAN_POINT('Ctrl Pts',(8.98412484365622,15.2,-6.08095559776391));
#177525=CARTESIAN_POINT('Ctrl Pts',(8.98640711983946,15.2,-6.08385891567967));
#177526=CARTESIAN_POINT('Ctrl Pts',(8.98868939571174,15.2,-6.08676223319985));
#177527=CARTESIAN_POINT('Ctrl Pts',(8.99097625317804,15.2,-6.08968139375391));
#177528=CARTESIAN_POINT('Ctrl Pts',(8.99326755354599,15.2,-6.09261636523518));
#177529=CARTESIAN_POINT('Ctrl Pts',(8.99555885422614,15.2,-6.09555133711633));
#177530=CARTESIAN_POINT('Ctrl Pts',(8.99785459857904,15.2,-6.09850212014937));
#177531=CARTESIAN_POINT('Ctrl Pts',(9.00015464670467,15.2,-6.10146867803429));
#177532=CARTESIAN_POINT('Ctrl Pts',(9.00245469451691,15.2,-6.10443523551501));
#177533=CARTESIAN_POINT('Ctrl Pts',(9.00475904789705,15.2,-6.10741757014222));
#177534=CARTESIAN_POINT('Ctrl Pts',(9.00706757098997,15.2,-6.11041564632334));
#177535=CARTESIAN_POINT('Ctrl Pts',(9.00937609439743,15.2,-6.11341372291293));
#177536=CARTESIAN_POINT('Ctrl Pts',(9.01168878724896,15.2,-6.11642754220109));
#177537=CARTESIAN_POINT('Ctrl Pts',(9.01400551343103,15.2,-6.1194570687561));
#177538=CARTESIAN_POINT('Ctrl Pts',(9.01632223929744,15.2,-6.12248659489834));
#177539=CARTESIAN_POINT('Ctrl Pts',(9.01864300161307,15.2,-6.12553182968468));
#177540=CARTESIAN_POINT('Ctrl Pts',(9.02096766414485,15.2,-6.12859273776618));
#177541=CARTESIAN_POINT('Ctrl Pts',(9.02329232699336,15.2,-6.13165364626472));
#177542=CARTESIAN_POINT('Ctrl Pts',(9.02562089208325,15.2,-6.13473022895278));
#177543=CARTESIAN_POINT('Ctrl Pts',(9.02795322627652,15.2,-6.13782245080206));
#177544=CARTESIAN_POINT('Ctrl Pts',(9.03028556015201,15.2,-6.14091467223004));
#177545=CARTESIAN_POINT('Ctrl Pts',(9.03262166388402,15.2,-6.14402253357677));
#177546=CARTESIAN_POINT('Ctrl Pts',(9.03496140685905,15.2,-6.14714600026428));
#177547=CARTESIAN_POINT('Ctrl Pts',(9.03730115015287,15.2,-6.15026946737736));
#177548=CARTESIAN_POINT('Ctrl Pts',(9.03964453225813,15.2,-6.1534085386419));
#177549=CARTESIAN_POINT('Ctrl Pts',(9.0419914244416,15.2,-6.15656318175828));
#177550=CARTESIAN_POINT('Ctrl Pts',(9.04433831662507,15.2,-6.15971782487466));
#177551=CARTESIAN_POINT('Ctrl Pts',(9.04668871920892,15.2,-6.16288803841228));
#177552=CARTESIAN_POINT('Ctrl Pts',(9.04904250339311,15.2,-6.16607378825416));
#177553=CARTESIAN_POINT('Ctrl Pts',(9.05139628725659,15.2,-6.16925953766198));
#177554=CARTESIAN_POINT('Ctrl Pts',(9.05375345326669,15.2,-6.17246082427395));
#177555=CARTESIAN_POINT('Ctrl Pts',(9.05611387447333,15.2,-6.17567761224777));
#177556=CARTESIAN_POINT('Ctrl Pts',(9.05847429600157,15.2,-6.17889440065986));
#177557=CARTESIAN_POINT('Ctrl Pts',(9.06083797364093,15.2,-6.18212669069127));
#177558=CARTESIAN_POINT('Ctrl Pts',(9.06320478110357,15.2,-6.18537444731431));
#177559=CARTESIAN_POINT('Ctrl Pts',(9.06557158824375,15.2,-6.18862220349484));
#177560=CARTESIAN_POINT('Ctrl Pts',(9.06794152469183,15.2,-6.19188542764556));
#177561=CARTESIAN_POINT('Ctrl Pts',(9.07031446833097,15.2,-6.1951640842654));
#177562=CARTESIAN_POINT('Ctrl Pts',(9.07268741229343,15.2,-6.19844274133196));
#177563=CARTESIAN_POINT('Ctrl Pts',(9.07506336046737,15.2,-6.20173683037261));
#177564=CARTESIAN_POINT('Ctrl Pts',(9.07744219265276,15.2,-6.20504631755398));
#177565=CARTESIAN_POINT('Ctrl Pts',(9.07982102451402,15.2,-6.20835580428443));
#177566=CARTESIAN_POINT('Ctrl Pts',(9.0822027386022,15.2,-6.21168068755065));
#177567=CARTESIAN_POINT('Ctrl Pts',(9.08458721463728,15.2,-6.21502093499869));
#177568=CARTESIAN_POINT('Ctrl Pts',(9.08697169099724,15.2,-6.21836118290184));
#177569=CARTESIAN_POINT('Ctrl Pts',(9.08935892868715,15.2,-6.22171679359375));
#177570=CARTESIAN_POINT('Ctrl Pts',(9.09174880692867,15.2,-6.22508773150067));
#177571=CARTESIAN_POINT('Ctrl Pts',(9.09413868484456,15.2,-6.2284586689483));
#177572=CARTESIAN_POINT('Ctrl Pts',(9.09653120285438,15.2,-6.23184493585954));
#177573=CARTESIAN_POINT('Ctrl Pts',(9.09892624265835,15.2,-6.23524649396881));
#177574=CARTESIAN_POINT('Ctrl Pts',(9.10132128278864,15.2,-6.23864805254156));
#177575=CARTESIAN_POINT('Ctrl Pts',(9.10371884416819,15.2,-6.2420649050135));
#177576=CARTESIAN_POINT('Ctrl Pts',(9.1061188078099,15.2,-6.24549701549396));
#177577=CARTESIAN_POINT('Ctrl Pts',(9.10851877112462,15.2,-6.2489291255068));
#177578=CARTESIAN_POINT('Ctrl Pts',(9.11092113811192,15.2,-6.25237649262957));
#177579=CARTESIAN_POINT('Ctrl Pts',(9.11332579008178,15.2,-6.25583908323383));
#177580=CARTESIAN_POINT('Ctrl Pts',(9.11573044237927,15.2,-6.25930167430988));
#177581=CARTESIAN_POINT('Ctrl Pts',(9.11813738030475,15.2,-6.26277948779292));
#177582=CARTESIAN_POINT('Ctrl Pts',(9.1205464884916,15.2,-6.26627248898328));
#177583=CARTESIAN_POINT('Ctrl Pts',(9.12295559667845,15.2,-6.26976549017364));
#177584=CARTESIAN_POINT('Ctrl Pts',(9.12536687366834,15.2,-6.27327367911025));
#177585=CARTESIAN_POINT('Ctrl Pts',(9.12778020591118,15.2,-6.27679702085936));
#177586=CARTESIAN_POINT('Ctrl Pts',(9.1301935378252,15.2,-6.28032036212842));
#177587=CARTESIAN_POINT('Ctrl Pts',(9.13260892429605,15.2,-6.28385885574417));
#177588=CARTESIAN_POINT('Ctrl Pts',(9.13502625099829,15.2,-6.28741246524754));
#177589=CARTESIAN_POINT('Ctrl Pts',(9.13804790962313,15.2,-6.29185447748989));
#177590=CARTESIAN_POINT('Ctrl Pts',(9.14107260097217,15.2,-6.29632011150551));
#177591=CARTESIAN_POINT('Ctrl Pts',(9.14410010374993,15.2,-6.30080929678328));
#177592=CARTESIAN_POINT('Ctrl Pts',(9.14652210610415,15.2,-6.30440064520122));
#177593=CARTESIAN_POINT('Ctrl Pts',(9.14894590835582,15.2,-6.30800706641262));
#177594=CARTESIAN_POINT('Ctrl Pts',(9.15137139865484,15.2,-6.31162852433374));
#177595=CARTESIAN_POINT('Ctrl Pts',(9.15379688862337,15.2,-6.31524998176143));
#177596=CARTESIAN_POINT('Ctrl Pts',(9.15622406744413,15.2,-6.31888647771555));
#177597=CARTESIAN_POINT('Ctrl Pts',(9.15865282275662,15.2,-6.32253797448914));
#177598=CARTESIAN_POINT('Ctrl Pts',(9.16108157840002,15.2,-6.32618947176025));
#177599=CARTESIAN_POINT('Ctrl Pts',(9.16351191170652,15.2,-6.32985597158025));
#177600=CARTESIAN_POINT('Ctrl Pts',(9.1659437133392,15.2,-6.33353743739355));
#177601=CARTESIAN_POINT('Ctrl Pts',(9.16837551464057,15.2,-6.33721890270526));
#177602=CARTESIAN_POINT('Ctrl Pts',(9.17080878248892,15.2,-6.34091533424829));
#177603=CARTESIAN_POINT('Ctrl Pts',(9.17324341106759,15.2,-6.3446266962217));
#177604=CARTESIAN_POINT('Ctrl Pts',(9.17506938258452,15.2,-6.34741021782817));
#177605=CARTESIAN_POINT('Ctrl Pts',(9.17689611803823,15.2,-6.35020213738773));
#177606=CARTESIAN_POINT('Ctrl Pts',(9.17872357318805,15.2,-6.35300244071658));
#177607=CARTESIAN_POINT('Ctrl Pts',(9.1811601802758,15.2,-6.35673617882753));
#177608=CARTESIAN_POINT('Ctrl Pts',(9.18359806499132,15.2,-6.36048482126557));
#177609=CARTESIAN_POINT('Ctrl Pts',(9.18603712195768,15.2,-6.36424833174944));
#177610=CARTESIAN_POINT('Ctrl Pts',(9.18786641451628,15.2,-6.36707096435595));
#177611=CARTESIAN_POINT('Ctrl Pts',(9.18969636621646,15.2,-6.36990196080313));
#177612=CARTESIAN_POINT('Ctrl Pts',(9.1915269318166,15.2,-6.37274130449161));
#177613=CARTESIAN_POINT('Ctrl Pts',(9.19335749741674,15.2,-6.37558064818009));
#177614=CARTESIAN_POINT('Ctrl Pts',(9.19518867673356,15.2,-6.37842834129329));
#177615=CARTESIAN_POINT('Ctrl Pts',(9.19702042679196,15.2,-6.38128436643879));
#177616=CARTESIAN_POINT('Ctrl Pts',(9.19885217685036,15.2,-6.3841403915843));
#177617=CARTESIAN_POINT('Ctrl Pts',(9.20068449597042,15.2,-6.38700474922275));
#177618=CARTESIAN_POINT('Ctrl Pts',(9.20251734116201,15.2,-6.38987742592759));
#177619=CARTESIAN_POINT('Ctrl Pts',(9.20435018635358,15.2,-6.39275010263242));
#177620=CARTESIAN_POINT('Ctrl Pts',(9.20618355725019,15.2,-6.39563109674288));
#177621=CARTESIAN_POINT('Ctrl Pts',(9.20801740985017,15.2,-6.3985203933451));
#177622=CARTESIAN_POINT('Ctrl Pts',(9.20985126278329,15.2,-6.40140969047222));
#177623=CARTESIAN_POINT('Ctrl Pts',(9.21168559669987,15.2,-6.40430729080999));
#177624=CARTESIAN_POINT('Ctrl Pts',(9.21352036963325,15.2,-6.40721317844178));
#177625=CARTESIAN_POINT('Ctrl Pts',(9.21535514223331,15.2,-6.41011906554565));
#177626=CARTESIAN_POINT('Ctrl Pts',(9.21719035300002,15.2,-6.4130332399241));
#177627=CARTESIAN_POINT('Ctrl Pts',(9.21902595818336,15.2,-6.41595568706865));
#177628=CARTESIAN_POINT('Ctrl Pts',(9.22086156336671,15.2,-6.4188781342132));
#177629=CARTESIAN_POINT('Ctrl Pts',(9.22269756404333,15.2,-6.4218088536127));
#177630=CARTESIAN_POINT('Ctrl Pts',(9.22453391573494,15.2,-6.42474783068596));
#177631=CARTESIAN_POINT('Ctrl Pts',(9.22637026742656,15.2,-6.42768680775922));
#177632=CARTESIAN_POINT('Ctrl Pts',(9.22820697139,15.2,-6.43063404135792));
#177633=CARTESIAN_POINT('Ctrl Pts',(9.23004398449827,15.2,-6.43358951697227));
#177634=CARTESIAN_POINT('Ctrl Pts',(9.23188099760654,15.2,-6.43654499258663));
#177635=CARTESIAN_POINT('Ctrl Pts',(9.23371831946644,15.2,-6.43950871131818));
#177636=CARTESIAN_POINT('Ctrl Pts',(9.23555590806632,15.2,-6.44248065545949));
#177637=CARTESIAN_POINT('Ctrl Pts',(9.2373934966662,15.2,-6.4454525996008));
#177638=CARTESIAN_POINT('Ctrl Pts',(9.23923135126605,15.2,-6.44843276974153));
#177639=CARTESIAN_POINT('Ctrl Pts',(9.24106943086591,15.2,-6.45142115229851));
#177640=CARTESIAN_POINT('Ctrl Pts',(9.24290751079969,15.2,-6.45440953539837));
#177641=CARTESIAN_POINT('Ctrl Pts',(9.24474581496685,15.2,-6.45740613003387));
#177642=CARTESIAN_POINT('Ctrl Pts',(9.2465843014424,15.2,-6.46041092022168));
#177643=CARTESIAN_POINT('Ctrl Pts',(9.24842278758395,15.2,-6.46341570986361));
#177644=CARTESIAN_POINT('Ctrl Pts',(9.25026145589731,15.2,-6.46642869627579));
#177645=CARTESIAN_POINT('Ctrl Pts',(9.25210026563071,15.2,-6.46944986306789));
#177646=CARTESIAN_POINT('Ctrl Pts',(9.25393907536411,15.2,-6.47247102985999));
#177647=CARTESIAN_POINT('Ctrl Pts',(9.25577802600054,15.2,-6.47550037704083));
#177648=CARTESIAN_POINT('Ctrl Pts',(9.25761707526707,15.2,-6.47853789009785));
#177649=CARTESIAN_POINT('Ctrl Pts',(9.25945612453359,15.2,-6.48157540315487));
#177650=CARTESIAN_POINT('Ctrl Pts',(9.26129527396678,15.2,-6.48462108092759));
#177651=CARTESIAN_POINT('Ctrl Pts',(9.26313448073328,15.2,-6.48767490948329));
#177652=CARTESIAN_POINT('Ctrl Pts',(9.26497368749979,15.2,-6.49072873803899));
#177653=CARTESIAN_POINT('Ctrl Pts',(9.26681295268296,15.2,-6.49379071664437));
#177654=CARTESIAN_POINT('Ctrl Pts',(9.2686522357828,15.2,-6.49686083019878));
#177655=CARTESIAN_POINT('Ctrl Pts',(9.27049151888264,15.2,-6.4999309437532));
#177656=CARTESIAN_POINT('Ctrl Pts',(9.27233081819915,15.2,-6.50300919175707));
#177657=CARTESIAN_POINT('Ctrl Pts',(9.27417009484065,15.2,-6.50609555935214));
#177658=CARTESIAN_POINT('Ctrl Pts',(9.27600937181628,15.2,-6.50918192750791));
#177659=CARTESIAN_POINT('Ctrl Pts',(9.27784862545027,15.2,-6.51227641499099));
#177660=CARTESIAN_POINT('Ctrl Pts',(9.27968781588422,15.2,-6.51537900619299));
#177661=CARTESIAN_POINT('Ctrl Pts',(9.28152700598405,15.2,-6.51848159683136));
#177662=CARTESIAN_POINT('Ctrl Pts',(9.28336613138071,15.2,-6.52159229186002));
#177663=CARTESIAN_POINT('Ctrl Pts',(9.28520515411408,15.2,-6.52471107561178));
#177664=CARTESIAN_POINT('Ctrl Pts',(9.28704417684745,15.2,-6.52782985936353));
#177665=CARTESIAN_POINT('Ctrl Pts',(9.28888309593385,15.2,-6.53095673117165));
#177666=CARTESIAN_POINT('Ctrl Pts',(9.29072187020037,15.2,-6.53409167585014));
#177667=CARTESIAN_POINT('Ctrl Pts',(9.29317356911104,15.2,-6.53827160189827));
#177668=CARTESIAN_POINT('Ctrl Pts',(9.29562501321898,15.2,-6.54246588134071));
#177669=CARTESIAN_POINT('Ctrl Pts',(9.2980761080742,15.2,-6.54667447532854));
#177670=CARTESIAN_POINT('Ctrl Pts',(9.29991442963306,15.2,-6.54983092153617));
#177671=CARTESIAN_POINT('Ctrl Pts',(9.30175255536687,15.2,-6.55299542097941));
#177672=CARTESIAN_POINT('Ctrl Pts',(9.3035904449256,15.2,-6.55616795719157));
#177673=CARTESIAN_POINT('Ctrl Pts',(9.30542833415045,15.2,-6.55934049282739));
#177674=CARTESIAN_POINT('Ctrl Pts',(9.30726598781376,15.2,-6.56252106577258));
#177675=CARTESIAN_POINT('Ctrl Pts',(9.30910336658876,15.2,-6.56570965960861));
#177676=CARTESIAN_POINT('Ctrl Pts',(9.31094074536376,15.2,-6.56889825344465));
#177677=CARTESIAN_POINT('Ctrl Pts',(9.31277784826691,15.2,-6.57209486974847));
#177678=CARTESIAN_POINT('Ctrl Pts',(9.31461463795015,15.2,-6.57529949138273));
#177679=CARTESIAN_POINT('Ctrl Pts',(9.31645142763339,15.2,-6.578504113017));
#177680=CARTESIAN_POINT('Ctrl Pts',(9.31828790329999,15.2,-6.58171674038364));
#177681=CARTESIAN_POINT('Ctrl Pts',(9.32012402748328,15.2,-6.58493735897495));
#177682=CARTESIAN_POINT('Ctrl Pts',(9.32196015166657,15.2,-6.58815797756627));
#177683=CARTESIAN_POINT('Ctrl Pts',(9.32379592338319,15.2,-6.59138658731558));
#177684=CARTESIAN_POINT('Ctrl Pts',(9.32563130602488,15.2,-6.5946231714473));
#177685=CARTESIAN_POINT('Ctrl Pts',(9.32746668866658,15.2,-6.59785975557902));
#177686=CARTESIAN_POINT('Ctrl Pts',(9.32930168085329,15.2,-6.6011043151107));
#177687=CARTESIAN_POINT('Ctrl Pts',(9.33113624312833,15.2,-6.60435683386242));
#177688=CARTESIAN_POINT('Ctrl Pts',(9.33297080540338,15.2,-6.60760935261415));
#177689=CARTESIAN_POINT('Ctrl Pts',(9.33480493680011,15.2,-6.61086982997397));
#177690=CARTESIAN_POINT('Ctrl Pts',(9.33663860106688,15.2,-6.61413825106245));
#177691=CARTESIAN_POINT('Ctrl Pts',(9.33847226566676,15.2,-6.61740667274471));
#177692=CARTESIAN_POINT('Ctrl Pts',(9.34030546333319,15.2,-6.62068303807088));
#177693=CARTESIAN_POINT('Ctrl Pts',(9.34213815989114,15.2,-6.62396733321595));
#177694=CARTESIAN_POINT('Ctrl Pts',(9.34458175474684,15.2,-6.62834639241495));
#177695=CARTESIAN_POINT('Ctrl Pts',(9.34702446114987,15.2,-6.63273954886213));
#177696=CARTESIAN_POINT('Ctrl Pts',(9.349466180617,15.2,-6.63714676338981));
#177697=CARTESIAN_POINT('Ctrl Pts',(9.35129747030051,15.2,-6.64045217443569));
#177698=CARTESIAN_POINT('Ctrl Pts',(9.35312820397086,15.2,-6.64376549154647));
#177699=CARTESIAN_POINT('Ctrl Pts',(9.35495833687086,15.2,-6.64708669734081));
#177700=CARTESIAN_POINT('Ctrl Pts',(9.35678846977087,15.2,-6.65040790313515));
#177701=CARTESIAN_POINT('Ctrl Pts',(9.35861800060096,15.2,-6.65373699742817));
#177702=CARTESIAN_POINT('Ctrl Pts',(9.36044690482625,15.2,-6.65707396726418));
#177703=CARTESIAN_POINT('Ctrl Pts',(9.36288544393859,15.2,-6.66152326064393));
#177704=CARTESIAN_POINT('Ctrl Pts',(9.36532286751701,15.2,-6.66598656016761));
#177705=CARTESIAN_POINT('Ctrl Pts',(9.36775917477149,15.2,-6.67046385458018));
#177706=CARTESIAN_POINT('Origin',(-5.66257110645729E-14,15.2,-1.77635683940025E-14));
#177707=CARTESIAN_POINT('',(8.88241603246431,15.2,-5.36127880541243));
#177708=CARTESIAN_POINT('',(8.88241603246431,12.2,-5.36127880541243));
#177709=CARTESIAN_POINT('',(8.88241603199995,15.2,-5.36127880500001));
#177710=CARTESIAN_POINT('Origin',(-5.66257110645729E-14,12.2,-1.77635683940025E-14));
#177711=CARTESIAN_POINT('Origin',(-5.66257110645729E-14,15.2,-1.77635683940025E-14));
#177712=CARTESIAN_POINT('Origin',(-5.66257110645729E-14,15.2,-1.77635683940025E-14));
#177713=CARTESIAN_POINT('',(10.0402696489999,15.2,-5.60740451200001));
#177714=CARTESIAN_POINT('',(10.2217148779999,15.2,-5.26939701900002));
#177715=CARTESIAN_POINT('Origin',(-5.66257110645729E-14,15.2,-1.77635683940025E-14));
#177716=CARTESIAN_POINT('',(10.2217148779999,12.2,-5.26939701900002));
#177717=CARTESIAN_POINT('',(10.2217148779999,15.2,-5.26939701900002));
#177718=CARTESIAN_POINT('',(10.0402696489999,12.2,-5.60740451200001));
#177719=CARTESIAN_POINT('Origin',(-5.66257110645729E-14,12.2,-1.77635683940025E-14));
#177720=CARTESIAN_POINT('',(10.0402696489999,15.2,-5.60740451200001));
#177721=CARTESIAN_POINT('Ctrl Pts',(10.2217148779999,15.2,-5.26939701900002));
#177722=CARTESIAN_POINT('Ctrl Pts',(10.2217148779999,11.6,-5.26939701900002));
#177723=CARTESIAN_POINT('Ctrl Pts',(10.2212575739999,15.2,-5.26878426900002));
#177724=CARTESIAN_POINT('Ctrl Pts',(10.2212575739999,11.6,-5.26878426900002));
#177725=CARTESIAN_POINT('Ctrl Pts',(10.2203429999999,15.2,-5.26755929400001));
#177726=CARTESIAN_POINT('Ctrl Pts',(10.2203429999999,11.6,-5.26755929400001));
#177727=CARTESIAN_POINT('Ctrl Pts',(10.2189712369999,15.2,-5.26572340900001));
#177728=CARTESIAN_POINT('Ctrl Pts',(10.2189712369999,11.6,-5.26572340900001));
#177729=CARTESIAN_POINT('Ctrl Pts',(10.2171424209999,15.2,-5.26327871600001));
#177730=CARTESIAN_POINT('Ctrl Pts',(10.2171424209999,11.6,-5.26327871600001));
#177731=CARTESIAN_POINT('Ctrl Pts',(10.2148567309999,15.2,-5.26022810500002));
#177732=CARTESIAN_POINT('Ctrl Pts',(10.2148567309999,11.6,-5.26022810500002));
#177733=CARTESIAN_POINT('Ctrl Pts',(10.2125713739999,15.2,-5.25718275100001));
#177734=CARTESIAN_POINT('Ctrl Pts',(10.2125713739999,11.6,-5.25718275100001));
#177735=CARTESIAN_POINT('Ctrl Pts',(10.2102863519999,15.2,-5.25414265600002));
#177736=CARTESIAN_POINT('Ctrl Pts',(10.2102863519999,11.6,-5.25414265600002));
#177737=CARTESIAN_POINT('Ctrl Pts',(10.2080016679999,15.2,-5.25110781800001));
#177738=CARTESIAN_POINT('Ctrl Pts',(10.2080016679999,11.6,-5.25110781800001));
#177739=CARTESIAN_POINT('Ctrl Pts',(10.2057173299999,15.2,-5.24807824100002));
#177740=CARTESIAN_POINT('Ctrl Pts',(10.2057173299999,11.6,-5.24807824100002));
#177741=CARTESIAN_POINT('Ctrl Pts',(10.2034333439999,15.2,-5.24505392700001));
#177742=CARTESIAN_POINT('Ctrl Pts',(10.2034333439999,11.6,-5.24505392700001));
#177743=CARTESIAN_POINT('Ctrl Pts',(10.2011497209999,15.2,-5.24203487700001));
#177744=CARTESIAN_POINT('Ctrl Pts',(10.2011497209999,11.6,-5.24203487700001));
#177745=CARTESIAN_POINT('Ctrl Pts',(10.1988664679999,15.2,-5.23902109400002));
#177746=CARTESIAN_POINT('Ctrl Pts',(10.1988664679999,11.6,-5.23902109400002));
#177747=CARTESIAN_POINT('Ctrl Pts',(10.1965835999999,15.2,-5.23601258300001));
#177748=CARTESIAN_POINT('Ctrl Pts',(10.1965835999999,11.6,-5.23601258300001));
#177749=CARTESIAN_POINT('Ctrl Pts',(10.1943011249999,15.2,-5.23300934300002));
#177750=CARTESIAN_POINT('Ctrl Pts',(10.1943011249999,11.6,-5.23300934300002));
#177751=CARTESIAN_POINT('Ctrl Pts',(10.1920190549999,15.2,-5.23001138000001));
#177752=CARTESIAN_POINT('Ctrl Pts',(10.1920190549999,11.6,-5.23001138000001));
#177753=CARTESIAN_POINT('Ctrl Pts',(10.1897373969999,15.2,-5.22701869500001));
#177754=CARTESIAN_POINT('Ctrl Pts',(10.1897373969999,11.6,-5.22701869500001));
#177755=CARTESIAN_POINT('Ctrl Pts',(10.1874561619999,15.2,-5.22403129000002));
#177756=CARTESIAN_POINT('Ctrl Pts',(10.1874561619999,11.6,-5.22403129000002));
#177757=CARTESIAN_POINT('Ctrl Pts',(10.1851753559999,15.2,-5.22104916700001));
#177758=CARTESIAN_POINT('Ctrl Pts',(10.1851753559999,11.6,-5.22104916700001));
#177759=CARTESIAN_POINT('Ctrl Pts',(10.1828949879999,15.2,-5.21807232700001));
#177760=CARTESIAN_POINT('Ctrl Pts',(10.1828949879999,11.6,-5.21807232700001));
#177761=CARTESIAN_POINT('Ctrl Pts',(10.1806150639999,15.2,-5.21510077400002));
#177762=CARTESIAN_POINT('Ctrl Pts',(10.1806150639999,11.6,-5.21510077400002));
#177763=CARTESIAN_POINT('Ctrl Pts',(10.1783355949999,15.2,-5.21213451000001));
#177764=CARTESIAN_POINT('Ctrl Pts',(10.1783355949999,11.6,-5.21213451000001));
#177765=CARTESIAN_POINT('Ctrl Pts',(10.1760565879999,15.2,-5.20917353600002));
#177766=CARTESIAN_POINT('Ctrl Pts',(10.1760565879999,11.6,-5.20917353600002));
#177767=CARTESIAN_POINT('Ctrl Pts',(10.1737780519999,15.2,-5.20621785500001));
#177768=CARTESIAN_POINT('Ctrl Pts',(10.1737780519999,11.6,-5.20621785500001));
#177769=CARTESIAN_POINT('Ctrl Pts',(10.1714999969999,15.2,-5.20326746900002));
#177770=CARTESIAN_POINT('Ctrl Pts',(10.1714999969999,11.6,-5.20326746900002));
#177771=CARTESIAN_POINT('Ctrl Pts',(10.1692224309999,15.2,-5.20032238000002));
#177772=CARTESIAN_POINT('Ctrl Pts',(10.1692224309999,11.6,-5.20032238000002));
#177773=CARTESIAN_POINT('Ctrl Pts',(10.1669453649999,15.2,-5.19738259100002));
#177774=CARTESIAN_POINT('Ctrl Pts',(10.1669453649999,11.6,-5.19738259100002));
#177775=CARTESIAN_POINT('Ctrl Pts',(10.1646688079999,15.2,-5.19444810300001));
#177776=CARTESIAN_POINT('Ctrl Pts',(10.1646688079999,11.6,-5.19444810300001));
#177777=CARTESIAN_POINT('Ctrl Pts',(10.1623927679999,15.2,-5.19151892100002));
#177778=CARTESIAN_POINT('Ctrl Pts',(10.1623927679999,11.6,-5.19151892100002));
#177779=CARTESIAN_POINT('Ctrl Pts',(10.1601172529999,15.2,-5.18859504400002));
#177780=CARTESIAN_POINT('Ctrl Pts',(10.1601172529999,11.6,-5.18859504400002));
#177781=CARTESIAN_POINT('Ctrl Pts',(10.1578422729999,15.2,-5.18567647600001));
#177782=CARTESIAN_POINT('Ctrl Pts',(10.1578422729999,11.6,-5.18567647600001));
#177783=CARTESIAN_POINT('Ctrl Pts',(10.1555678379999,15.2,-5.18276321900002));
#177784=CARTESIAN_POINT('Ctrl Pts',(10.1555678379999,11.6,-5.18276321900002));
#177785=CARTESIAN_POINT('Ctrl Pts',(10.1532939539999,15.2,-5.17985527400001));
#177786=CARTESIAN_POINT('Ctrl Pts',(10.1532939539999,11.6,-5.17985527400001));
#177787=CARTESIAN_POINT('Ctrl Pts',(10.1510206309999,15.2,-5.17695264500002));
#177788=CARTESIAN_POINT('Ctrl Pts',(10.1510206309999,11.6,-5.17695264500002));
#177789=CARTESIAN_POINT('Ctrl Pts',(10.1487478799999,15.2,-5.17405533200002));
#177790=CARTESIAN_POINT('Ctrl Pts',(10.1487478799999,11.6,-5.17405533200002));
#177791=CARTESIAN_POINT('Ctrl Pts',(10.1464757069999,15.2,-5.17116333800002));
#177792=CARTESIAN_POINT('Ctrl Pts',(10.1464757069999,11.6,-5.17116333800002));
#177793=CARTESIAN_POINT('Ctrl Pts',(10.1442041239999,15.2,-5.16827666700001));
#177794=CARTESIAN_POINT('Ctrl Pts',(10.1442041239999,11.6,-5.16827666700001));
#177795=CARTESIAN_POINT('Ctrl Pts',(10.1419331389999,15.2,-5.16539531900001));
#177796=CARTESIAN_POINT('Ctrl Pts',(10.1419331389999,11.6,-5.16539531900001));
#177797=CARTESIAN_POINT('Ctrl Pts',(10.1396627609999,15.2,-5.16251929700001));
#177798=CARTESIAN_POINT('Ctrl Pts',(10.1396627609999,11.6,-5.16251929700001));
#177799=CARTESIAN_POINT('Ctrl Pts',(10.1373929979999,15.2,-5.15964860200001));
#177800=CARTESIAN_POINT('Ctrl Pts',(10.1373929979999,11.6,-5.15964860200001));
#177801=CARTESIAN_POINT('Ctrl Pts',(10.1351238609999,15.2,-5.15678323800001));
#177802=CARTESIAN_POINT('Ctrl Pts',(10.1351238609999,11.6,-5.15678323800001));
#177803=CARTESIAN_POINT('Ctrl Pts',(10.1328553589999,15.2,-5.15392320600002));
#177804=CARTESIAN_POINT('Ctrl Pts',(10.1328553589999,11.6,-5.15392320600002));
#177805=CARTESIAN_POINT('Ctrl Pts',(10.1305874999999,15.2,-5.15106851000001));
#177806=CARTESIAN_POINT('Ctrl Pts',(10.1305874999999,11.6,-5.15106851000001));
#177807=CARTESIAN_POINT('Ctrl Pts',(10.1283202939999,15.2,-5.14821914900002));
#177808=CARTESIAN_POINT('Ctrl Pts',(10.1283202939999,11.6,-5.14821914900002));
#177809=CARTESIAN_POINT('Ctrl Pts',(10.1260537499999,15.2,-5.14537512800001));
#177810=CARTESIAN_POINT('Ctrl Pts',(10.1260537499999,11.6,-5.14537512800001));
#177811=CARTESIAN_POINT('Ctrl Pts',(10.1237878759999,15.2,-5.14253644700001));
#177812=CARTESIAN_POINT('Ctrl Pts',(10.1237878759999,11.6,-5.14253644700001));
#177813=CARTESIAN_POINT('Ctrl Pts',(10.1215226839999,15.2,-5.13970310900001));
#177814=CARTESIAN_POINT('Ctrl Pts',(10.1215226839999,11.6,-5.13970310900001));
#177815=CARTESIAN_POINT('Ctrl Pts',(10.1192581799999,15.2,-5.13687511700001));
#177816=CARTESIAN_POINT('Ctrl Pts',(10.1192581799999,11.6,-5.13687511700001));
#177817=CARTESIAN_POINT('Ctrl Pts',(10.1169943759999,15.2,-5.13405247200001));
#177818=CARTESIAN_POINT('Ctrl Pts',(10.1169943759999,11.6,-5.13405247200001));
#177819=CARTESIAN_POINT('Ctrl Pts',(10.1147312799999,15.2,-5.13123517600001));
#177820=CARTESIAN_POINT('Ctrl Pts',(10.1147312799999,11.6,-5.13123517600001));
#177821=CARTESIAN_POINT('Ctrl Pts',(10.1124689019999,15.2,-5.12842323200001));
#177822=CARTESIAN_POINT('Ctrl Pts',(10.1124689019999,11.6,-5.12842323200001));
#177823=CARTESIAN_POINT('Ctrl Pts',(10.1102072499999,15.2,-5.12561664200001));
#177824=CARTESIAN_POINT('Ctrl Pts',(10.1102072499999,11.6,-5.12561664200001));
#177825=CARTESIAN_POINT('Ctrl Pts',(10.1079463349999,15.2,-5.12281540800001));
#177826=CARTESIAN_POINT('Ctrl Pts',(10.1079463349999,11.6,-5.12281540800001));
#177827=CARTESIAN_POINT('Ctrl Pts',(10.1056861639999,15.2,-5.12001953100001));
#177828=CARTESIAN_POINT('Ctrl Pts',(10.1056861639999,11.6,-5.12001953100001));
#177829=CARTESIAN_POINT('Ctrl Pts',(10.1034267499999,15.2,-5.11722901400002));
#177830=CARTESIAN_POINT('Ctrl Pts',(10.1034267499999,11.6,-5.11722901400002));
#177831=CARTESIAN_POINT('Ctrl Pts',(10.1011680999999,15.2,-5.11444386000001));
#177832=CARTESIAN_POINT('Ctrl Pts',(10.1011680999999,11.6,-5.11444386000001));
#177833=CARTESIAN_POINT('Ctrl Pts',(10.0989102229999,15.2,-5.11166406900001));
#177834=CARTESIAN_POINT('Ctrl Pts',(10.0989102229999,11.6,-5.11166406900001));
#177835=CARTESIAN_POINT('Ctrl Pts',(10.0966531299999,15.2,-5.10888964500001));
#177836=CARTESIAN_POINT('Ctrl Pts',(10.0966531299999,11.6,-5.10888964500001));
#177837=CARTESIAN_POINT('Ctrl Pts',(10.0943968289999,15.2,-5.10612059000001));
#177838=CARTESIAN_POINT('Ctrl Pts',(10.0943968289999,11.6,-5.10612059000001));
#177839=CARTESIAN_POINT('Ctrl Pts',(10.0921413299999,15.2,-5.10335690500002));
#177840=CARTESIAN_POINT('Ctrl Pts',(10.0921413299999,11.6,-5.10335690500002));
#177841=CARTESIAN_POINT('Ctrl Pts',(10.0898866439999,15.2,-5.10059859300001));
#177842=CARTESIAN_POINT('Ctrl Pts',(10.0898866439999,11.6,-5.10059859300001));
#177843=CARTESIAN_POINT('Ctrl Pts',(10.0876327779999,15.2,-5.09784565500001));
#177844=CARTESIAN_POINT('Ctrl Pts',(10.0876327779999,11.6,-5.09784565500001));
#177845=CARTESIAN_POINT('Ctrl Pts',(10.0853797429999,15.2,-5.09509809400001));
#177846=CARTESIAN_POINT('Ctrl Pts',(10.0853797429999,11.6,-5.09509809400001));
#177847=CARTESIAN_POINT('Ctrl Pts',(10.0831275479999,15.2,-5.09235591100001));
#177848=CARTESIAN_POINT('Ctrl Pts',(10.0831275479999,11.6,-5.09235591100001));
#177849=CARTESIAN_POINT('Ctrl Pts',(10.0808762039999,15.2,-5.08961911000001));
#177850=CARTESIAN_POINT('Ctrl Pts',(10.0808762039999,11.6,-5.08961911000001));
#177851=CARTESIAN_POINT('Ctrl Pts',(10.0786257189999,15.2,-5.08688769200001));
#177852=CARTESIAN_POINT('Ctrl Pts',(10.0786257189999,11.6,-5.08688769200001));
#177853=CARTESIAN_POINT('Ctrl Pts',(10.0763761029999,15.2,-5.08416165800002));
#177854=CARTESIAN_POINT('Ctrl Pts',(10.0763761029999,11.6,-5.08416165800002));
#177855=CARTESIAN_POINT('Ctrl Pts',(10.0741273649999,15.2,-5.08144101100001));
#177856=CARTESIAN_POINT('Ctrl Pts',(10.0741273649999,11.6,-5.08144101100001));
#177857=CARTESIAN_POINT('Ctrl Pts',(10.0718795159999,15.2,-5.07872575400001));
#177858=CARTESIAN_POINT('Ctrl Pts',(10.0718795159999,11.6,-5.07872575400001));
#177859=CARTESIAN_POINT('Ctrl Pts',(10.0696325649999,15.2,-5.07601588800001));
#177860=CARTESIAN_POINT('Ctrl Pts',(10.0696325649999,11.6,-5.07601588800001));
#177861=CARTESIAN_POINT('Ctrl Pts',(10.0673865209999,15.2,-5.07331141500002));
#177862=CARTESIAN_POINT('Ctrl Pts',(10.0673865209999,11.6,-5.07331141500002));
#177863=CARTESIAN_POINT('Ctrl Pts',(10.0651413949999,15.2,-5.07061233700002));
#177864=CARTESIAN_POINT('Ctrl Pts',(10.0651413949999,11.6,-5.07061233700002));
#177865=CARTESIAN_POINT('Ctrl Pts',(10.0628971959999,15.2,-5.06791865600002));
#177866=CARTESIAN_POINT('Ctrl Pts',(10.0628971959999,11.6,-5.06791865600002));
#177867=CARTESIAN_POINT('Ctrl Pts',(10.0606539349999,15.2,-5.06523037500001));
#177868=CARTESIAN_POINT('Ctrl Pts',(10.0606539349999,11.6,-5.06523037500001));
#177869=CARTESIAN_POINT('Ctrl Pts',(10.0584116189999,15.2,-5.06254749600001));
#177870=CARTESIAN_POINT('Ctrl Pts',(10.0584116189999,11.6,-5.06254749600001));
#177871=CARTESIAN_POINT('Ctrl Pts',(10.0561702599999,15.2,-5.05987001900001));
#177872=CARTESIAN_POINT('Ctrl Pts',(10.0561702599999,11.6,-5.05987001900001));
#177873=CARTESIAN_POINT('Ctrl Pts',(10.0539298679999,15.2,-5.05719794800001));
#177874=CARTESIAN_POINT('Ctrl Pts',(10.0539298679999,11.6,-5.05719794800001));
#177875=CARTESIAN_POINT('Ctrl Pts',(10.0516904509999,15.2,-5.05453128400001));
#177876=CARTESIAN_POINT('Ctrl Pts',(10.0516904509999,11.6,-5.05453128400001));
#177877=CARTESIAN_POINT('Ctrl Pts',(10.0494520199999,15.2,-5.05187002900001));
#177878=CARTESIAN_POINT('Ctrl Pts',(10.0494520199999,11.6,-5.05187002900001));
#177879=CARTESIAN_POINT('Ctrl Pts',(10.0472145849999,15.2,-5.04921418600001));
#177880=CARTESIAN_POINT('Ctrl Pts',(10.0472145849999,11.6,-5.04921418600001));
#177881=CARTESIAN_POINT('Ctrl Pts',(10.0449781559999,15.2,-5.04656375500002));
#177882=CARTESIAN_POINT('Ctrl Pts',(10.0449781559999,11.6,-5.04656375500002));
#177883=CARTESIAN_POINT('Ctrl Pts',(10.0427427419999,15.2,-5.04391874100001));
#177884=CARTESIAN_POINT('Ctrl Pts',(10.0427427419999,11.6,-5.04391874100001));
#177885=CARTESIAN_POINT('Ctrl Pts',(10.0405083539999,15.2,-5.04127914300001));
#177886=CARTESIAN_POINT('Ctrl Pts',(10.0405083539999,11.6,-5.04127914300001));
#177887=CARTESIAN_POINT('Ctrl Pts',(10.0382750009999,15.2,-5.03864496500002));
#177888=CARTESIAN_POINT('Ctrl Pts',(10.0382750009999,11.6,-5.03864496500002));
#177889=CARTESIAN_POINT('Ctrl Pts',(10.0360426939999,15.2,-5.03601620900001));
#177890=CARTESIAN_POINT('Ctrl Pts',(10.0360426939999,11.6,-5.03601620900001));
#177891=CARTESIAN_POINT('Ctrl Pts',(10.0338114419999,15.2,-5.03339287600001));
#177892=CARTESIAN_POINT('Ctrl Pts',(10.0338114419999,11.6,-5.03339287600001));
#177893=CARTESIAN_POINT('Ctrl Pts',(10.0315812549999,15.2,-5.03077496800001));
#177894=CARTESIAN_POINT('Ctrl Pts',(10.0315812549999,11.6,-5.03077496800001));
#177895=CARTESIAN_POINT('Ctrl Pts',(10.0293521449999,15.2,-5.02816248700002));
#177896=CARTESIAN_POINT('Ctrl Pts',(10.0293521449999,11.6,-5.02816248700002));
#177897=CARTESIAN_POINT('Ctrl Pts',(10.0271241189999,15.2,-5.02555543600002));
#177898=CARTESIAN_POINT('Ctrl Pts',(10.0271241189999,11.6,-5.02555543600002));
#177899=CARTESIAN_POINT('Ctrl Pts',(10.0248971889999,15.2,-5.02295381500002));
#177900=CARTESIAN_POINT('Ctrl Pts',(10.0248971889999,11.6,-5.02295381500002));
#177901=CARTESIAN_POINT('Ctrl Pts',(10.0226713639999,15.2,-5.02035762800002));
#177902=CARTESIAN_POINT('Ctrl Pts',(10.0226713639999,11.6,-5.02035762800002));
#177903=CARTESIAN_POINT('Ctrl Pts',(10.0204466549999,15.2,-5.01776687600001));
#177904=CARTESIAN_POINT('Ctrl Pts',(10.0204466549999,11.6,-5.01776687600001));
#177905=CARTESIAN_POINT('Ctrl Pts',(10.0182230729999,15.2,-5.01518156000001));
#177906=CARTESIAN_POINT('Ctrl Pts',(10.0182230729999,11.6,-5.01518156000001));
#177907=CARTESIAN_POINT('Ctrl Pts',(10.0160006259999,15.2,-5.01260168400002));
#177908=CARTESIAN_POINT('Ctrl Pts',(10.0160006259999,11.6,-5.01260168400002));
#177909=CARTESIAN_POINT('Ctrl Pts',(10.0137793259999,15.2,-5.01002724800002));
#177910=CARTESIAN_POINT('Ctrl Pts',(10.0137793259999,11.6,-5.01002724800002));
#177911=CARTESIAN_POINT('Ctrl Pts',(10.0115591819999,15.2,-5.00745825600001));
#177912=CARTESIAN_POINT('Ctrl Pts',(10.0115591819999,11.6,-5.00745825600001));
#177913=CARTESIAN_POINT('Ctrl Pts',(10.0093402039999,15.2,-5.00489470900002));
#177914=CARTESIAN_POINT('Ctrl Pts',(10.0093402039999,11.6,-5.00489470900002));
#177915=CARTESIAN_POINT('Ctrl Pts',(10.0071224029999,15.2,-5.00233660800002));
#177916=CARTESIAN_POINT('Ctrl Pts',(10.0071224029999,11.6,-5.00233660800002));
#177917=CARTESIAN_POINT('Ctrl Pts',(10.0049057889999,15.2,-4.99978395500001));
#177918=CARTESIAN_POINT('Ctrl Pts',(10.0049057889999,11.6,-4.99978395500001));
#177919=CARTESIAN_POINT('Ctrl Pts',(10.0026903729999,15.2,-4.99723675300002));
#177920=CARTESIAN_POINT('Ctrl Pts',(10.0026903729999,11.6,-4.99723675300002));
#177921=CARTESIAN_POINT('Ctrl Pts',(10.0004761639999,15.2,-4.99469500400001));
#177922=CARTESIAN_POINT('Ctrl Pts',(10.0004761639999,11.6,-4.99469500400001));
#177923=CARTESIAN_POINT('Ctrl Pts',(9.99826317399994,15.2,-4.99215870900001));
#177924=CARTESIAN_POINT('Ctrl Pts',(9.99826317399994,11.6,-4.99215870900002));
#177925=CARTESIAN_POINT('Ctrl Pts',(9.99605141199994,15.2,-4.98962787000002));
#177926=CARTESIAN_POINT('Ctrl Pts',(9.99605141199994,11.6,-4.98962787000002));
#177927=CARTESIAN_POINT('Ctrl Pts',(9.99384088799994,15.2,-4.98710249000001));
#177928=CARTESIAN_POINT('Ctrl Pts',(9.99384088799994,11.6,-4.98710249000002));
#177929=CARTESIAN_POINT('Ctrl Pts',(9.99163161399995,15.2,-4.98458256900001));
#177930=CARTESIAN_POINT('Ctrl Pts',(9.99163161399995,11.6,-4.98458256900001));
#177931=CARTESIAN_POINT('Ctrl Pts',(9.98942359899995,15.2,-4.98206811000002));
#177932=CARTESIAN_POINT('Ctrl Pts',(9.98942359899995,11.6,-4.98206811000002));
#177933=CARTESIAN_POINT('Ctrl Pts',(9.98721685399994,15.2,-4.97955911500001));
#177934=CARTESIAN_POINT('Ctrl Pts',(9.98721685399994,11.6,-4.97955911500001));
#177935=CARTESIAN_POINT('Ctrl Pts',(9.98501138999995,15.2,-4.97705558600002));
#177936=CARTESIAN_POINT('Ctrl Pts',(9.98501138999995,11.6,-4.97705558600002));
#177937=CARTESIAN_POINT('Ctrl Pts',(9.98280721699994,15.2,-4.97455752400001));
#177938=CARTESIAN_POINT('Ctrl Pts',(9.98280721699994,11.6,-4.97455752400001));
#177939=CARTESIAN_POINT('Ctrl Pts',(9.98060434499994,15.2,-4.97206493200002));
#177940=CARTESIAN_POINT('Ctrl Pts',(9.98060434499994,11.6,-4.97206493200002));
#177941=CARTESIAN_POINT('Ctrl Pts',(9.97840278499995,15.2,-4.96957781100001));
#177942=CARTESIAN_POINT('Ctrl Pts',(9.97840278499995,11.6,-4.96957781100001));
#177943=CARTESIAN_POINT('Ctrl Pts',(9.97620254699994,15.2,-4.96709616400001));
#177944=CARTESIAN_POINT('Ctrl Pts',(9.97620254699994,11.6,-4.96709616400001));
#177945=CARTESIAN_POINT('Ctrl Pts',(9.97400364199994,15.2,-4.96461999100001));
#177946=CARTESIAN_POINT('Ctrl Pts',(9.97400364199994,11.6,-4.96461999100002));
#177947=CARTESIAN_POINT('Ctrl Pts',(9.97180608099995,15.2,-4.96214929600002));
#177948=CARTESIAN_POINT('Ctrl Pts',(9.97180608099995,11.6,-4.96214929600002));
#177949=CARTESIAN_POINT('Ctrl Pts',(9.96960987299994,15.2,-4.95968407800001));
#177950=CARTESIAN_POINT('Ctrl Pts',(9.96960987299994,11.6,-4.95968407800001));
#177951=CARTESIAN_POINT('Ctrl Pts',(9.96741503199994,15.2,-4.95722434200002));
#177952=CARTESIAN_POINT('Ctrl Pts',(9.96741503199994,11.6,-4.95722434200002));
#177953=CARTESIAN_POINT('Ctrl Pts',(9.96522156599994,15.2,-4.95477008800002));
#177954=CARTESIAN_POINT('Ctrl Pts',(9.96522156599994,11.6,-4.95477008800002));
#177955=CARTESIAN_POINT('Ctrl Pts',(9.96302948499994,15.2,-4.95232131800002));
#177956=CARTESIAN_POINT('Ctrl Pts',(9.96302948499994,11.6,-4.95232131800002));
#177957=CARTESIAN_POINT('Ctrl Pts',(9.96083880199994,15.2,-4.94987803500001));
#177958=CARTESIAN_POINT('Ctrl Pts',(9.96083880199994,11.6,-4.94987803500001));
#177959=CARTESIAN_POINT('Ctrl Pts',(9.95864952599995,15.2,-4.94744023800001));
#177960=CARTESIAN_POINT('Ctrl Pts',(9.95864952599995,11.6,-4.94744023800001));
#177961=CARTESIAN_POINT('Ctrl Pts',(9.95646166799995,15.2,-4.94500793200002));
#177962=CARTESIAN_POINT('Ctrl Pts',(9.95646166799995,11.6,-4.94500793200002));
#177963=CARTESIAN_POINT('Ctrl Pts',(9.95427523999994,15.2,-4.94258111700002));
#177964=CARTESIAN_POINT('Ctrl Pts',(9.95427523999994,11.6,-4.94258111700002));
#177965=CARTESIAN_POINT('Ctrl Pts',(9.95209025099994,15.2,-4.94015979700002));
#177966=CARTESIAN_POINT('Ctrl Pts',(9.95209025099994,11.6,-4.94015979700002));
#177967=CARTESIAN_POINT('Ctrl Pts',(9.94990671399995,15.2,-4.93774397000001));
#177968=CARTESIAN_POINT('Ctrl Pts',(9.94990671399995,11.6,-4.93774397000002));
#177969=CARTESIAN_POINT('Ctrl Pts',(9.94772463699995,15.2,-4.93533364100001));
#177970=CARTESIAN_POINT('Ctrl Pts',(9.94772463699995,11.6,-4.93533364100002));
#177971=CARTESIAN_POINT('Ctrl Pts',(9.94554403299994,15.2,-4.93292881000002));
#177972=CARTESIAN_POINT('Ctrl Pts',(9.94554403299994,11.6,-4.93292881000002));
#177973=CARTESIAN_POINT('Ctrl Pts',(9.94336491299994,15.2,-4.93052948100001));
#177974=CARTESIAN_POINT('Ctrl Pts',(9.94336491299994,11.6,-4.93052948100001));
#177975=CARTESIAN_POINT('Ctrl Pts',(9.94118728699994,15.2,-4.92813565300001));
#177976=CARTESIAN_POINT('Ctrl Pts',(9.94118728699994,11.6,-4.92813565300002));
#177977=CARTESIAN_POINT('Ctrl Pts',(9.93901116599995,15.2,-4.92574732900001));
#177978=CARTESIAN_POINT('Ctrl Pts',(9.93901116599995,11.6,-4.92574732900002));
#177979=CARTESIAN_POINT('Ctrl Pts',(9.93683656099994,15.2,-4.92336451100002));
#177980=CARTESIAN_POINT('Ctrl Pts',(9.93683656099994,11.6,-4.92336451100002));
#177981=CARTESIAN_POINT('Ctrl Pts',(9.93466348399994,15.2,-4.92098720100001));
#177982=CARTESIAN_POINT('Ctrl Pts',(9.93466348399994,11.6,-4.92098720100001));
#177983=CARTESIAN_POINT('Ctrl Pts',(9.93249194399995,15.2,-4.91861540000002));
#177984=CARTESIAN_POINT('Ctrl Pts',(9.93249194399995,11.6,-4.91861540000002));
#177985=CARTESIAN_POINT('Ctrl Pts',(9.93032195399994,15.2,-4.91624911100002));
#177986=CARTESIAN_POINT('Ctrl Pts',(9.93032195399994,11.6,-4.91624911100002));
#177987=CARTESIAN_POINT('Ctrl Pts',(9.92815352399995,15.2,-4.91388833500002));
#177988=CARTESIAN_POINT('Ctrl Pts',(9.92815352399995,11.6,-4.91388833500002));
#177989=CARTESIAN_POINT('Ctrl Pts',(9.92598666499994,15.2,-4.91153307200001));
#177990=CARTESIAN_POINT('Ctrl Pts',(9.92598666499994,11.6,-4.91153307200001));
#177991=CARTESIAN_POINT('Ctrl Pts',(9.92382138899995,15.2,-4.90918332600002));
#177992=CARTESIAN_POINT('Ctrl Pts',(9.92382138899995,11.6,-4.90918332600002));
#177993=CARTESIAN_POINT('Ctrl Pts',(9.92165770599994,15.2,-4.90683909900001));
#177994=CARTESIAN_POINT('Ctrl Pts',(9.92165770599994,11.6,-4.90683909900001));
#177995=CARTESIAN_POINT('Ctrl Pts',(9.91949562799994,15.2,-4.90450039100002));
#177996=CARTESIAN_POINT('Ctrl Pts',(9.91949562799994,11.6,-4.90450039100002));
#177997=CARTESIAN_POINT('Ctrl Pts',(9.91733516599995,15.2,-4.90216720500001));
#177998=CARTESIAN_POINT('Ctrl Pts',(9.91733516599995,11.6,-4.90216720500001));
#177999=CARTESIAN_POINT('Ctrl Pts',(9.91517632999994,15.2,-4.89983954200001));
#178000=CARTESIAN_POINT('Ctrl Pts',(9.91517632999994,11.6,-4.89983954200001));
#178001=CARTESIAN_POINT('Ctrl Pts',(9.91301913399995,15.2,-4.89751740500001));
#178002=CARTESIAN_POINT('Ctrl Pts',(9.91301913399995,11.6,-4.89751740500001));
#178003=CARTESIAN_POINT('Ctrl Pts',(9.91086358699994,15.2,-4.89520079400001));
#178004=CARTESIAN_POINT('Ctrl Pts',(9.91086358699994,11.6,-4.89520079400002));
#178005=CARTESIAN_POINT('Ctrl Pts',(9.90870969999994,15.2,-4.89288971200001));
#178006=CARTESIAN_POINT('Ctrl Pts',(9.90870969999994,11.6,-4.89288971200002));
#178007=CARTESIAN_POINT('Ctrl Pts',(9.90655748599995,15.2,-4.89058415900002));
#178008=CARTESIAN_POINT('Ctrl Pts',(9.90655748599995,11.6,-4.89058415900002));
#178009=CARTESIAN_POINT('Ctrl Pts',(9.90440695499995,15.2,-4.88828413900002));
#178010=CARTESIAN_POINT('Ctrl Pts',(9.90440695499995,11.6,-4.88828413900002));
#178011=CARTESIAN_POINT('Ctrl Pts',(9.90225811999995,15.2,-4.88598965200001));
#178012=CARTESIAN_POINT('Ctrl Pts',(9.90225811999995,11.6,-4.88598965200001));
#178013=CARTESIAN_POINT('Ctrl Pts',(9.90011098899994,15.2,-4.88370070000002));
#178014=CARTESIAN_POINT('Ctrl Pts',(9.90011098899994,11.6,-4.88370070000002));
#178015=CARTESIAN_POINT('Ctrl Pts',(9.89796557699995,15.2,-4.88141728600001));
#178016=CARTESIAN_POINT('Ctrl Pts',(9.89796557699995,11.6,-4.88141728600001));
#178017=CARTESIAN_POINT('Ctrl Pts',(9.89582189499994,15.2,-4.87913940900001));
#178018=CARTESIAN_POINT('Ctrl Pts',(9.89582189499994,11.6,-4.87913940900001));
#178019=CARTESIAN_POINT('Ctrl Pts',(9.89367995199995,15.2,-4.87686707300002));
#178020=CARTESIAN_POINT('Ctrl Pts',(9.89367995199995,11.6,-4.87686707300002));
#178021=CARTESIAN_POINT('Ctrl Pts',(9.89153976099994,15.2,-4.87460027900001));
#178022=CARTESIAN_POINT('Ctrl Pts',(9.89153976099994,11.6,-4.87460027900002));
#178023=CARTESIAN_POINT('Ctrl Pts',(9.88940133499994,15.2,-4.87233902900002));
#178024=CARTESIAN_POINT('Ctrl Pts',(9.88940133499994,11.6,-4.87233902900002));
#178025=CARTESIAN_POINT('Ctrl Pts',(9.88726468299994,15.2,-4.87008332300002));
#178026=CARTESIAN_POINT('Ctrl Pts',(9.88726468299994,11.6,-4.87008332300002));
#178027=CARTESIAN_POINT('Ctrl Pts',(9.88512981699994,15.2,-4.86783316500001));
#178028=CARTESIAN_POINT('Ctrl Pts',(9.88512981699994,11.6,-4.86783316500001));
#178029=CARTESIAN_POINT('Ctrl Pts',(9.88299674999995,15.2,-4.86558855600002));
#178030=CARTESIAN_POINT('Ctrl Pts',(9.88299674999995,11.6,-4.86558855600002));
#178031=CARTESIAN_POINT('Ctrl Pts',(9.88086549299994,15.2,-4.86334949700002));
#178032=CARTESIAN_POINT('Ctrl Pts',(9.88086549299994,11.6,-4.86334949700002));
#178033=CARTESIAN_POINT('Ctrl Pts',(9.87873605699994,15.2,-4.86111598900001));
#178034=CARTESIAN_POINT('Ctrl Pts',(9.87873605699994,11.6,-4.86111598900001));
#178035=CARTESIAN_POINT('Ctrl Pts',(9.87660845399994,15.2,-4.85888803500002));
#178036=CARTESIAN_POINT('Ctrl Pts',(9.87660845399994,11.6,-4.85888803500002));
#178037=CARTESIAN_POINT('Ctrl Pts',(9.87448269599994,15.2,-4.85666563600001));
#178038=CARTESIAN_POINT('Ctrl Pts',(9.87448269599994,11.6,-4.85666563600002));
#178039=CARTESIAN_POINT('Ctrl Pts',(9.87235879499995,15.2,-4.85444879300001));
#178040=CARTESIAN_POINT('Ctrl Pts',(9.87235879499995,11.6,-4.85444879300002));
#178041=CARTESIAN_POINT('Ctrl Pts',(9.87023676299994,15.2,-4.85223750900001));
#178042=CARTESIAN_POINT('Ctrl Pts',(9.87023676299994,11.6,-4.85223750900001));
#178043=CARTESIAN_POINT('Ctrl Pts',(9.86811660899994,15.2,-4.85003178400001));
#178044=CARTESIAN_POINT('Ctrl Pts',(9.86811660899994,11.6,-4.85003178400001));
#178045=CARTESIAN_POINT('Ctrl Pts',(9.86599834899994,15.2,-4.84783162100001));
#178046=CARTESIAN_POINT('Ctrl Pts',(9.86599834899994,11.6,-4.84783162100001));
#178047=CARTESIAN_POINT('Ctrl Pts',(9.86388199199994,15.2,-4.84563702200001));
#178048=CARTESIAN_POINT('Ctrl Pts',(9.86388199199994,11.6,-4.84563702200001));
#178049=CARTESIAN_POINT('Ctrl Pts',(9.86176754899994,15.2,-4.84344798700001));
#178050=CARTESIAN_POINT('Ctrl Pts',(9.86176754899994,11.6,-4.84344798700001));
#178051=CARTESIAN_POINT('Ctrl Pts',(9.85965503599994,15.2,-4.84126451800002));
#178052=CARTESIAN_POINT('Ctrl Pts',(9.85965503599994,11.6,-4.84126451800002));
#178053=CARTESIAN_POINT('Ctrl Pts',(9.85754445999994,15.2,-4.83908661700001));
#178054=CARTESIAN_POINT('Ctrl Pts',(9.85754445999994,11.6,-4.83908661700002));
#178055=CARTESIAN_POINT('Ctrl Pts',(9.85543583699994,15.2,-4.83691428600002));
#178056=CARTESIAN_POINT('Ctrl Pts',(9.85543583699994,11.6,-4.83691428600002));
#178057=CARTESIAN_POINT('Ctrl Pts',(9.85332917699995,15.2,-4.83474752600001));
#178058=CARTESIAN_POINT('Ctrl Pts',(9.85332917699995,11.6,-4.83474752600001));
#178059=CARTESIAN_POINT('Ctrl Pts',(9.85122449199994,15.2,-4.83258633800002));
#178060=CARTESIAN_POINT('Ctrl Pts',(9.85122449199994,11.6,-4.83258633800002));
#178061=CARTESIAN_POINT('Ctrl Pts',(9.84912179299995,15.2,-4.83043072400001));
#178062=CARTESIAN_POINT('Ctrl Pts',(9.84912179299995,11.6,-4.83043072400002));
#178063=CARTESIAN_POINT('Ctrl Pts',(9.84702109499995,15.2,-4.82828068500002));
#178064=CARTESIAN_POINT('Ctrl Pts',(9.84702109499995,11.6,-4.82828068500002));
#178065=CARTESIAN_POINT('Ctrl Pts',(9.84492240799995,15.2,-4.82613622400001));
#178066=CARTESIAN_POINT('Ctrl Pts',(9.84492240799995,11.6,-4.82613622400002));
#178067=CARTESIAN_POINT('Ctrl Pts',(9.84282574499994,15.2,-4.82399734200001));
#178068=CARTESIAN_POINT('Ctrl Pts',(9.84282574499994,11.6,-4.82399734200001));
#178069=CARTESIAN_POINT('Ctrl Pts',(9.84073111699994,15.2,-4.82186404000001));
#178070=CARTESIAN_POINT('Ctrl Pts',(9.84073111699994,11.6,-4.82186404000002));
#178071=CARTESIAN_POINT('Ctrl Pts',(9.83863853799994,15.2,-4.81973632000001));
#178072=CARTESIAN_POINT('Ctrl Pts',(9.83863853799994,11.6,-4.81973632000001));
#178073=CARTESIAN_POINT('Ctrl Pts',(9.83654801799995,15.2,-4.81761418300001));
#178074=CARTESIAN_POINT('Ctrl Pts',(9.83654801799995,11.6,-4.81761418300001));
#178075=CARTESIAN_POINT('Ctrl Pts',(9.83445956999994,15.2,-4.81549763000002));
#178076=CARTESIAN_POINT('Ctrl Pts',(9.83445956999994,11.6,-4.81549763000002));
#178077=CARTESIAN_POINT('Ctrl Pts',(9.83237320799994,15.2,-4.81338666500001));
#178078=CARTESIAN_POINT('Ctrl Pts',(9.83237320799994,11.6,-4.81338666500002));
#178079=CARTESIAN_POINT('Ctrl Pts',(9.83028894099995,15.2,-4.81128128700002));
#178080=CARTESIAN_POINT('Ctrl Pts',(9.83028894099995,11.6,-4.81128128700002));
#178081=CARTESIAN_POINT('Ctrl Pts',(9.82820678499994,15.2,-4.80918149800001));
#178082=CARTESIAN_POINT('Ctrl Pts',(9.82820678499994,11.6,-4.80918149800001));
#178083=CARTESIAN_POINT('Ctrl Pts',(9.82612674899995,15.2,-4.80708730000002));
#178084=CARTESIAN_POINT('Ctrl Pts',(9.82612674899995,11.6,-4.80708730000002));
#178085=CARTESIAN_POINT('Ctrl Pts',(9.82404884799994,15.2,-4.80499869500001));
#178086=CARTESIAN_POINT('Ctrl Pts',(9.82404884799994,11.6,-4.80499869500001));
#178087=CARTESIAN_POINT('Ctrl Pts',(9.82197309199995,15.2,-4.80291568300002));
#178088=CARTESIAN_POINT('Ctrl Pts',(9.82197309199995,11.6,-4.80291568300002));
#178089=CARTESIAN_POINT('Ctrl Pts',(9.81989949599994,15.2,-4.80083826600001));
#178090=CARTESIAN_POINT('Ctrl Pts',(9.81989949599994,11.6,-4.80083826600001));
#178091=CARTESIAN_POINT('Ctrl Pts',(9.81782806999994,15.2,-4.79876644700001));
#178092=CARTESIAN_POINT('Ctrl Pts',(9.81782806999994,11.6,-4.79876644700001));
#178093=CARTESIAN_POINT('Ctrl Pts',(9.81575882799994,15.2,-4.79670022500001));
#178094=CARTESIAN_POINT('Ctrl Pts',(9.81575882799994,11.6,-4.79670022500002));
#178095=CARTESIAN_POINT('Ctrl Pts',(9.81369178299994,15.2,-4.79463960300002));
#178096=CARTESIAN_POINT('Ctrl Pts',(9.81369178299994,11.6,-4.79463960300002));
#178097=CARTESIAN_POINT('Ctrl Pts',(9.81162694599995,15.2,-4.79258458200002));
#178098=CARTESIAN_POINT('Ctrl Pts',(9.81162694599995,11.6,-4.79258458200002));
#178099=CARTESIAN_POINT('Ctrl Pts',(9.80956432999994,15.2,-4.79053516400001));
#178100=CARTESIAN_POINT('Ctrl Pts',(9.80956432999994,11.6,-4.79053516400001));
#178101=CARTESIAN_POINT('Ctrl Pts',(9.80750394899994,15.2,-4.78849134900001));
#178102=CARTESIAN_POINT('Ctrl Pts',(9.80750394899994,11.6,-4.78849134900001));
#178103=CARTESIAN_POINT('Ctrl Pts',(9.80544581399995,15.2,-4.78645314000001));
#178104=CARTESIAN_POINT('Ctrl Pts',(9.80544581399995,11.6,-4.78645314000001));
#178105=CARTESIAN_POINT('Ctrl Pts',(9.80338993799995,15.2,-4.78442053800002));
#178106=CARTESIAN_POINT('Ctrl Pts',(9.80338993799995,11.6,-4.78442053800002));
#178107=CARTESIAN_POINT('Ctrl Pts',(9.80133633399995,15.2,-4.78239354400001));
#178108=CARTESIAN_POINT('Ctrl Pts',(9.80133633399995,11.6,-4.78239354400001));
#178109=CARTESIAN_POINT('Ctrl Pts',(9.79928501499994,15.2,-4.78037216000001));
#178110=CARTESIAN_POINT('Ctrl Pts',(9.79928501499994,11.6,-4.78037216000002));
#178111=CARTESIAN_POINT('Ctrl Pts',(9.79723599299994,15.2,-4.77835638700002));
#178112=CARTESIAN_POINT('Ctrl Pts',(9.79723599299994,11.6,-4.77835638700002));
#178113=CARTESIAN_POINT('Ctrl Pts',(9.79518928099995,15.2,-4.77634622600001));
#178114=CARTESIAN_POINT('Ctrl Pts',(9.79518928099995,11.6,-4.77634622600002));
#178115=CARTESIAN_POINT('Ctrl Pts',(9.79314489299994,15.2,-4.77434167900002));
#178116=CARTESIAN_POINT('Ctrl Pts',(9.79314489299994,11.6,-4.77434167900002));
#178117=CARTESIAN_POINT('Ctrl Pts',(9.79110284099994,15.2,-4.77234274600002));
#178118=CARTESIAN_POINT('Ctrl Pts',(9.79110284099994,11.6,-4.77234274600002));
#178119=CARTESIAN_POINT('Ctrl Pts',(9.78906313699994,15.2,-4.77034943200001));
#178120=CARTESIAN_POINT('Ctrl Pts',(9.78906313699994,11.6,-4.77034943200001));
#178121=CARTESIAN_POINT('Ctrl Pts',(9.78702579499994,15.2,-4.76836173400002));
#178122=CARTESIAN_POINT('Ctrl Pts',(9.78702579499994,11.6,-4.76836173400002));
#178123=CARTESIAN_POINT('Ctrl Pts',(9.78499082799994,15.2,-4.76637965700001));
#178124=CARTESIAN_POINT('Ctrl Pts',(9.78499082799994,11.6,-4.76637965700002));
#178125=CARTESIAN_POINT('Ctrl Pts',(9.78295824899994,15.2,-4.76440319900002));
#178126=CARTESIAN_POINT('Ctrl Pts',(9.78295824899994,11.6,-4.76440319900002));
#178127=CARTESIAN_POINT('Ctrl Pts',(9.78092806999994,15.2,-4.76243236400002));
#178128=CARTESIAN_POINT('Ctrl Pts',(9.78092806999994,11.6,-4.76243236400002));
#178129=CARTESIAN_POINT('Ctrl Pts',(9.77890030599994,15.2,-4.76046715200001));
#178130=CARTESIAN_POINT('Ctrl Pts',(9.77890030599994,11.6,-4.76046715200001));
#178131=CARTESIAN_POINT('Ctrl Pts',(9.77687496799994,15.2,-4.75850756500002));
#178132=CARTESIAN_POINT('Ctrl Pts',(9.77687496799994,11.6,-4.75850756500002));
#178133=CARTESIAN_POINT('Ctrl Pts',(9.77485206899994,15.2,-4.75655360400001));
#178134=CARTESIAN_POINT('Ctrl Pts',(9.77485206899994,11.6,-4.75655360400001));
#178135=CARTESIAN_POINT('Ctrl Pts',(9.77283162499995,15.2,-4.75460527100001));
#178136=CARTESIAN_POINT('Ctrl Pts',(9.77283162499995,11.6,-4.75460527100002));
#178137=CARTESIAN_POINT('Ctrl Pts',(9.77081364699995,15.2,-4.75266256500001));
#178138=CARTESIAN_POINT('Ctrl Pts',(9.77081364699995,11.6,-4.75266256500001));
#178139=CARTESIAN_POINT('Ctrl Pts',(9.76879814799995,15.2,-4.75072549100001));
#178140=CARTESIAN_POINT('Ctrl Pts',(9.76879814799995,11.6,-4.75072549100001));
#178141=CARTESIAN_POINT('Ctrl Pts',(9.76678514199994,15.2,-4.74879404700001));
#178142=CARTESIAN_POINT('Ctrl Pts',(9.76678514199994,11.6,-4.74879404700001));
#178143=CARTESIAN_POINT('Ctrl Pts',(9.76477464199995,15.2,-4.74686823700001));
#178144=CARTESIAN_POINT('Ctrl Pts',(9.76477464199995,11.6,-4.74686823700001));
#178145=CARTESIAN_POINT('Ctrl Pts',(9.76276666199994,15.2,-4.74494806000001));
#178146=CARTESIAN_POINT('Ctrl Pts',(9.76276666199994,11.6,-4.74494806000001));
#178147=CARTESIAN_POINT('Ctrl Pts',(9.76076121399995,15.2,-4.74303351800001));
#178148=CARTESIAN_POINT('Ctrl Pts',(9.76076121399995,11.6,-4.74303351800002));
#178149=CARTESIAN_POINT('Ctrl Pts',(9.75875831199994,15.2,-4.74112461300002));
#178150=CARTESIAN_POINT('Ctrl Pts',(9.75875831199994,11.6,-4.74112461300002));
#178151=CARTESIAN_POINT('Ctrl Pts',(9.75675797099995,15.2,-4.73922134600001));
#178152=CARTESIAN_POINT('Ctrl Pts',(9.75675797099995,11.6,-4.73922134600001));
#178153=CARTESIAN_POINT('Ctrl Pts',(9.75476020099994,15.2,-4.73732371700001));
#178154=CARTESIAN_POINT('Ctrl Pts',(9.75476020099994,11.6,-4.73732371700002));
#178155=CARTESIAN_POINT('Ctrl Pts',(9.75276501899994,15.2,-4.73543173000001));
#178156=CARTESIAN_POINT('Ctrl Pts',(9.75276501899994,11.6,-4.73543173000001));
#178157=CARTESIAN_POINT('Ctrl Pts',(9.75077243699995,15.2,-4.73354538300002));
#178158=CARTESIAN_POINT('Ctrl Pts',(9.75077243699995,11.6,-4.73354538300002));
#178159=CARTESIAN_POINT('Ctrl Pts',(9.74878246899994,15.2,-4.73166467900001));
#178160=CARTESIAN_POINT('Ctrl Pts',(9.74878246899994,11.6,-4.73166467900001));
#178161=CARTESIAN_POINT('Ctrl Pts',(9.74679512899994,15.2,-4.72978962000001));
#178162=CARTESIAN_POINT('Ctrl Pts',(9.74679512899994,11.6,-4.72978962000001));
#178163=CARTESIAN_POINT('Ctrl Pts',(9.74481042799994,15.2,-4.72792020600002));
#178164=CARTESIAN_POINT('Ctrl Pts',(9.74481042799994,11.6,-4.72792020600002));
#178165=CARTESIAN_POINT('Ctrl Pts',(9.74282838199995,15.2,-4.72605643900001));
#178166=CARTESIAN_POINT('Ctrl Pts',(9.74282838199995,11.6,-4.72605643900002));
#178167=CARTESIAN_POINT('Ctrl Pts',(9.74084900499994,15.2,-4.72419831800002));
#178168=CARTESIAN_POINT('Ctrl Pts',(9.74084900499994,11.6,-4.72419831800002));
#178169=CARTESIAN_POINT('Ctrl Pts',(9.73887230999994,15.2,-4.72234584700002));
#178170=CARTESIAN_POINT('Ctrl Pts',(9.73887230999994,11.6,-4.72234584700002));
#178171=CARTESIAN_POINT('Ctrl Pts',(9.73689830999995,15.2,-4.72049902600002));
#178172=CARTESIAN_POINT('Ctrl Pts',(9.73689830999995,11.6,-4.72049902600002));
#178173=CARTESIAN_POINT('Ctrl Pts',(9.73492701999995,15.2,-4.71865785700002));
#178174=CARTESIAN_POINT('Ctrl Pts',(9.73492701999995,11.6,-4.71865785700002));
#178175=CARTESIAN_POINT('Ctrl Pts',(9.73295845299995,15.2,-4.71682234000002));
#178176=CARTESIAN_POINT('Ctrl Pts',(9.73295845299995,11.6,-4.71682234000002));
#178177=CARTESIAN_POINT('Ctrl Pts',(9.73099262399994,15.2,-4.71499247700002));
#178178=CARTESIAN_POINT('Ctrl Pts',(9.73099262399994,11.6,-4.71499247700002));
#178179=CARTESIAN_POINT('Ctrl Pts',(9.72902954599994,15.2,-4.71316826800001));
#178180=CARTESIAN_POINT('Ctrl Pts',(9.72902954599994,11.6,-4.71316826800001));
#178181=CARTESIAN_POINT('Ctrl Pts',(9.72706923299994,15.2,-4.71134971600002));
#178182=CARTESIAN_POINT('Ctrl Pts',(9.72706923299994,11.6,-4.71134971600002));
#178183=CARTESIAN_POINT('Ctrl Pts',(9.72511169899994,15.2,-4.70953682000002));
#178184=CARTESIAN_POINT('Ctrl Pts',(9.72511169899994,11.6,-4.70953682000002));
#178185=CARTESIAN_POINT('Ctrl Pts',(9.72315695899994,15.2,-4.70772958400001));
#178186=CARTESIAN_POINT('Ctrl Pts',(9.72315695899994,11.6,-4.70772958400001));
#178187=CARTESIAN_POINT('Ctrl Pts',(9.72120502599994,15.2,-4.70592800700001));
#178188=CARTESIAN_POINT('Ctrl Pts',(9.72120502599994,11.6,-4.70592800700001));
#178189=CARTESIAN_POINT('Ctrl Pts',(9.71925591399994,15.2,-4.70413209100002));
#178190=CARTESIAN_POINT('Ctrl Pts',(9.71925591399994,11.6,-4.70413209100002));
#178191=CARTESIAN_POINT('Ctrl Pts',(9.71730963799994,15.2,-4.70234183600001));
#178192=CARTESIAN_POINT('Ctrl Pts',(9.71730963799994,11.6,-4.70234183600002));
#178193=CARTESIAN_POINT('Ctrl Pts',(9.71536621099995,15.2,-4.70055724400002));
#178194=CARTESIAN_POINT('Ctrl Pts',(9.71536621099995,11.6,-4.70055724400002));
#178195=CARTESIAN_POINT('Ctrl Pts',(9.71342564799994,15.2,-4.69877831600002));
#178196=CARTESIAN_POINT('Ctrl Pts',(9.71342564799994,11.6,-4.69877831600002));
#178197=CARTESIAN_POINT('Ctrl Pts',(9.71148796399994,15.2,-4.69700505400001));
#178198=CARTESIAN_POINT('Ctrl Pts',(9.71148796399994,11.6,-4.69700505400002));
#178199=CARTESIAN_POINT('Ctrl Pts',(9.70955317199994,15.2,-4.69523745800001));
#178200=CARTESIAN_POINT('Ctrl Pts',(9.70955317199994,11.6,-4.69523745800002));
#178201=CARTESIAN_POINT('Ctrl Pts',(9.70762128699995,15.2,-4.69347552800001));
#178202=CARTESIAN_POINT('Ctrl Pts',(9.70762128699995,11.6,-4.69347552800001));
#178203=CARTESIAN_POINT('Ctrl Pts',(9.70569232299994,15.2,-4.69171926800001));
#178204=CARTESIAN_POINT('Ctrl Pts',(9.70569232299994,11.6,-4.69171926800002));
#178205=CARTESIAN_POINT('Ctrl Pts',(9.70376629399994,15.2,-4.68996867700001));
#178206=CARTESIAN_POINT('Ctrl Pts',(9.70376629399994,11.6,-4.68996867700001));
#178207=CARTESIAN_POINT('Ctrl Pts',(9.70184321499995,15.2,-4.68822375800002));
#178208=CARTESIAN_POINT('Ctrl Pts',(9.70184321499995,11.6,-4.68822375800002));
#178209=CARTESIAN_POINT('Ctrl Pts',(9.69992310199994,15.2,-4.68648450800002));
#178210=CARTESIAN_POINT('Ctrl Pts',(9.69992310199994,11.6,-4.68648450800002));
#178211=CARTESIAN_POINT('Ctrl Pts',(9.69800596699995,15.2,-4.68475093300002));
#178212=CARTESIAN_POINT('Ctrl Pts',(9.69800596699995,11.6,-4.68475093300002));
#178213=CARTESIAN_POINT('Ctrl Pts',(9.69609182599994,15.2,-4.68302303000002));
#178214=CARTESIAN_POINT('Ctrl Pts',(9.69609182599994,11.6,-4.68302303000002));
#178215=CARTESIAN_POINT('Ctrl Pts',(9.69418069299994,15.2,-4.68130080300002));
#178216=CARTESIAN_POINT('Ctrl Pts',(9.69418069299994,11.6,-4.68130080300002));
#178217=CARTESIAN_POINT('Ctrl Pts',(9.69227258299994,15.2,-4.67958425200001));
#178218=CARTESIAN_POINT('Ctrl Pts',(9.69227258299994,11.6,-4.67958425200001));
#178219=CARTESIAN_POINT('Ctrl Pts',(9.69036750899994,15.2,-4.67787337800001));
#178220=CARTESIAN_POINT('Ctrl Pts',(9.69036750899994,11.6,-4.67787337800001));
#178221=CARTESIAN_POINT('Ctrl Pts',(9.68846548899995,15.2,-4.67616818100002));
#178222=CARTESIAN_POINT('Ctrl Pts',(9.68846548899995,11.6,-4.67616818100002));
#178223=CARTESIAN_POINT('Ctrl Pts',(9.68656653499995,15.2,-4.67446866300001));
#178224=CARTESIAN_POINT('Ctrl Pts',(9.68656653499995,11.6,-4.67446866300001));
#178225=CARTESIAN_POINT('Ctrl Pts',(9.68467066399995,15.2,-4.67277482500001));
#178226=CARTESIAN_POINT('Ctrl Pts',(9.68467066399995,11.6,-4.67277482500002));
#178227=CARTESIAN_POINT('Ctrl Pts',(9.68277788899995,15.2,-4.67108666800002));
#178228=CARTESIAN_POINT('Ctrl Pts',(9.68277788899995,11.6,-4.67108666800002));
#178229=CARTESIAN_POINT('Ctrl Pts',(9.68088822599995,15.2,-4.66940419300002));
#178230=CARTESIAN_POINT('Ctrl Pts',(9.68088822599995,11.6,-4.66940419300002));
#178231=CARTESIAN_POINT('Ctrl Pts',(9.67900168899994,15.2,-4.66772740200001));
#178232=CARTESIAN_POINT('Ctrl Pts',(9.67900168899994,11.6,-4.66772740200002));
#178233=CARTESIAN_POINT('Ctrl Pts',(9.67711829399994,15.2,-4.66605629400001));
#178234=CARTESIAN_POINT('Ctrl Pts',(9.67711829399994,11.6,-4.66605629400001));
#178235=CARTESIAN_POINT('Ctrl Pts',(9.67523805399994,15.2,-4.66439087100001));
#178236=CARTESIAN_POINT('Ctrl Pts',(9.67523805399994,11.6,-4.66439087100001));
#178237=CARTESIAN_POINT('Ctrl Pts',(9.67336098799995,15.2,-4.66273113300002));
#178238=CARTESIAN_POINT('Ctrl Pts',(9.67336098799995,11.6,-4.66273113300002));
#178239=CARTESIAN_POINT('Ctrl Pts',(9.67148710599995,15.2,-4.66107708200001));
#178240=CARTESIAN_POINT('Ctrl Pts',(9.67148710599995,11.6,-4.66107708200001));
#178241=CARTESIAN_POINT('Ctrl Pts',(9.66961642799994,15.2,-4.65942871900001));
#178242=CARTESIAN_POINT('Ctrl Pts',(9.66961642799994,11.6,-4.65942871900001));
#178243=CARTESIAN_POINT('Ctrl Pts',(9.66774896599994,15.2,-4.65778604500001));
#178244=CARTESIAN_POINT('Ctrl Pts',(9.66774896599994,11.6,-4.65778604500002));
#178245=CARTESIAN_POINT('Ctrl Pts',(9.66588473599994,15.2,-4.65614906000001));
#178246=CARTESIAN_POINT('Ctrl Pts',(9.66588473599994,11.6,-4.65614906000001));
#178247=CARTESIAN_POINT('Ctrl Pts',(9.66402375299995,15.2,-4.65451776500001));
#178248=CARTESIAN_POINT('Ctrl Pts',(9.66402375299995,11.6,-4.65451776500002));
#178249=CARTESIAN_POINT('Ctrl Pts',(9.66216603399995,15.2,-4.65289216300001));
#178250=CARTESIAN_POINT('Ctrl Pts',(9.66216603399995,11.6,-4.65289216300001));
#178251=CARTESIAN_POINT('Ctrl Pts',(9.66031159299994,15.2,-4.65127225200002));
#178252=CARTESIAN_POINT('Ctrl Pts',(9.66031159299994,11.6,-4.65127225200002));
#178253=CARTESIAN_POINT('Ctrl Pts',(9.65846044499994,15.2,-4.64965803400001));
#178254=CARTESIAN_POINT('Ctrl Pts',(9.65846044499994,11.6,-4.64965803400002));
#178255=CARTESIAN_POINT('Ctrl Pts',(9.65661260499994,15.2,-4.64804951100001));
#178256=CARTESIAN_POINT('Ctrl Pts',(9.65661260499994,11.6,-4.64804951100002));
#178257=CARTESIAN_POINT('Ctrl Pts',(9.65476809099994,15.2,-4.64644668200001));
#178258=CARTESIAN_POINT('Ctrl Pts',(9.65476809099994,11.6,-4.64644668200001));
#178259=CARTESIAN_POINT('Ctrl Pts',(9.65292691699995,15.2,-4.64484954900001));
#178260=CARTESIAN_POINT('Ctrl Pts',(9.65292691699995,11.6,-4.64484954900002));
#178261=CARTESIAN_POINT('Ctrl Pts',(9.65108909699994,15.2,-4.64325811300002));
#178262=CARTESIAN_POINT('Ctrl Pts',(9.65108909699994,11.6,-4.64325811300002));
#178263=CARTESIAN_POINT('Ctrl Pts',(9.64925464999994,15.2,-4.64167237400002));
#178264=CARTESIAN_POINT('Ctrl Pts',(9.64925464999994,11.6,-4.64167237400002));
#178265=CARTESIAN_POINT('Ctrl Pts',(9.64742358899995,15.2,-4.64009233400001));
#178266=CARTESIAN_POINT('Ctrl Pts',(9.64742358899995,11.6,-4.64009233400002));
#178267=CARTESIAN_POINT('Ctrl Pts',(9.64559592999995,15.2,-4.63851799300001));
#178268=CARTESIAN_POINT('Ctrl Pts',(9.64559592999995,11.6,-4.63851799300001));
#178269=CARTESIAN_POINT('Ctrl Pts',(9.64377168999994,15.2,-4.63694935100001));
#178270=CARTESIAN_POINT('Ctrl Pts',(9.64377168999994,11.6,-4.63694935100001));
#178271=CARTESIAN_POINT('Ctrl Pts',(9.64195088399994,15.2,-4.63538641000001));
#178272=CARTESIAN_POINT('Ctrl Pts',(9.64195088399994,11.6,-4.63538641000001));
#178273=CARTESIAN_POINT('Ctrl Pts',(9.64013352699994,15.2,-4.63382917200001));
#178274=CARTESIAN_POINT('Ctrl Pts',(9.64013352699994,11.6,-4.63382917200002));
#178275=CARTESIAN_POINT('Ctrl Pts',(9.63831963699995,15.2,-4.63227763600001));
#178276=CARTESIAN_POINT('Ctrl Pts',(9.63831963699995,11.6,-4.63227763600001));
#178277=CARTESIAN_POINT('Ctrl Pts',(9.63650922799994,15.2,-4.63073180200002));
#178278=CARTESIAN_POINT('Ctrl Pts',(9.63650922799994,11.6,-4.63073180200002));
#178279=CARTESIAN_POINT('Ctrl Pts',(9.63470231799995,15.2,-4.62919167300001));
#178280=CARTESIAN_POINT('Ctrl Pts',(9.63470231799995,11.6,-4.62919167300001));
#178281=CARTESIAN_POINT('Ctrl Pts',(9.63289892099995,15.2,-4.62765724900001));
#178282=CARTESIAN_POINT('Ctrl Pts',(9.63289892099995,11.6,-4.62765724900002));
#178283=CARTESIAN_POINT('Ctrl Pts',(9.63109905299994,15.2,-4.62612853000001));
#178284=CARTESIAN_POINT('Ctrl Pts',(9.63109905299994,11.6,-4.62612853000001));
#178285=CARTESIAN_POINT('Ctrl Pts',(9.62930273199994,15.2,-4.62460551700001));
#178286=CARTESIAN_POINT('Ctrl Pts',(9.62930273199994,11.6,-4.62460551700001));
#178287=CARTESIAN_POINT('Ctrl Pts',(9.62750997299995,15.2,-4.62308821200001));
#178288=CARTESIAN_POINT('Ctrl Pts',(9.62750997299995,11.6,-4.62308821200002));
#178289=CARTESIAN_POINT('Ctrl Pts',(9.62572079199994,15.2,-4.62157661300001));
#178290=CARTESIAN_POINT('Ctrl Pts',(9.62572079199994,11.6,-4.62157661300001));
#178291=CARTESIAN_POINT('Ctrl Pts',(9.62393520599995,15.2,-4.62007072400001));
#178292=CARTESIAN_POINT('Ctrl Pts',(9.62393520599995,11.6,-4.62007072400001));
#178293=CARTESIAN_POINT('Ctrl Pts',(9.62215323099995,15.2,-4.61857054400001));
#178294=CARTESIAN_POINT('Ctrl Pts',(9.62215323099995,11.6,-4.61857054400001));
#178295=CARTESIAN_POINT('Ctrl Pts',(9.62037488299995,15.2,-4.61707607400001));
#178296=CARTESIAN_POINT('Ctrl Pts',(9.62037488299995,11.6,-4.61707607400002));
#178297=CARTESIAN_POINT('Ctrl Pts',(9.61860017899994,15.2,-4.61558731400002));
#178298=CARTESIAN_POINT('Ctrl Pts',(9.61860017899994,11.6,-4.61558731400002));
#178299=CARTESIAN_POINT('Ctrl Pts',(9.61682913599994,15.2,-4.61410426600001));
#178300=CARTESIAN_POINT('Ctrl Pts',(9.61682913599994,11.6,-4.61410426600002));
#178301=CARTESIAN_POINT('Ctrl Pts',(9.61506176799995,15.2,-4.61262692900001));
#178302=CARTESIAN_POINT('Ctrl Pts',(9.61506176799995,11.6,-4.61262692900002));
#178303=CARTESIAN_POINT('Ctrl Pts',(9.61329809399994,15.2,-4.61115530500001));
#178304=CARTESIAN_POINT('Ctrl Pts',(9.61329809399994,11.6,-4.61115530500001));
#178305=CARTESIAN_POINT('Ctrl Pts',(9.61153812999994,15.2,-4.60968939500002));
#178306=CARTESIAN_POINT('Ctrl Pts',(9.61153812999994,11.6,-4.60968939500002));
#178307=CARTESIAN_POINT('Ctrl Pts',(9.60978189399994,15.2,-4.60822919900002));
#178308=CARTESIAN_POINT('Ctrl Pts',(9.60978189399994,11.6,-4.60822919900002));
#178309=CARTESIAN_POINT('Ctrl Pts',(9.60802939899994,15.2,-4.60677471700001));
#178310=CARTESIAN_POINT('Ctrl Pts',(9.60802939899994,11.6,-4.60677471700001));
#178311=CARTESIAN_POINT('Ctrl Pts',(9.60628066499994,15.2,-4.60532595000001));
#178312=CARTESIAN_POINT('Ctrl Pts',(9.60628066499994,11.6,-4.60532595000002));
#178313=CARTESIAN_POINT('Ctrl Pts',(9.60453570799995,15.2,-4.60388290000001));
#178314=CARTESIAN_POINT('Ctrl Pts',(9.60453570799995,11.6,-4.60388290000001));
#178315=CARTESIAN_POINT('Ctrl Pts',(9.60279454499995,15.2,-4.60244556600002));
#178316=CARTESIAN_POINT('Ctrl Pts',(9.60279454499995,11.6,-4.60244556600002));
#178317=CARTESIAN_POINT('Ctrl Pts',(9.60105719199994,15.2,-4.60101394900001));
#178318=CARTESIAN_POINT('Ctrl Pts',(9.60105719199994,11.6,-4.60101394900002));
#178319=CARTESIAN_POINT('Ctrl Pts',(9.59932366799995,15.2,-4.59958805000001));
#178320=CARTESIAN_POINT('Ctrl Pts',(9.59932366799995,11.6,-4.59958805000001));
#178321=CARTESIAN_POINT('Ctrl Pts',(9.59759398799994,15.2,-4.59816786900001));
#178322=CARTESIAN_POINT('Ctrl Pts',(9.59759398799994,11.6,-4.59816786900001));
#178323=CARTESIAN_POINT('Ctrl Pts',(9.59586816799994,15.2,-4.59675340600001));
#178324=CARTESIAN_POINT('Ctrl Pts',(9.59586816799994,11.6,-4.59675340600001));
#178325=CARTESIAN_POINT('Ctrl Pts',(9.59414622799994,15.2,-4.59534466400001));
#178326=CARTESIAN_POINT('Ctrl Pts',(9.59414622799994,11.6,-4.59534466400001));
#178327=CARTESIAN_POINT('Ctrl Pts',(9.59242818399994,15.2,-4.59394164100001));
#178328=CARTESIAN_POINT('Ctrl Pts',(9.59242818399994,11.6,-4.59394164100001));
#178329=CARTESIAN_POINT('Ctrl Pts',(9.59071405399994,15.2,-4.59254433900002));
#178330=CARTESIAN_POINT('Ctrl Pts',(9.59071405399994,11.6,-4.59254433900002));
#178331=CARTESIAN_POINT('Ctrl Pts',(9.58900385399994,15.2,-4.59115275800002));
#178332=CARTESIAN_POINT('Ctrl Pts',(9.58900385399994,11.6,-4.59115275800002));
#178333=CARTESIAN_POINT('Ctrl Pts',(9.58729760199994,15.2,-4.58976689800001));
#178334=CARTESIAN_POINT('Ctrl Pts',(9.58729760199994,11.6,-4.58976689800001));
#178335=CARTESIAN_POINT('Ctrl Pts',(9.58559531499995,15.2,-4.58838676100001));
#178336=CARTESIAN_POINT('Ctrl Pts',(9.58559531499995,11.6,-4.58838676100001));
#178337=CARTESIAN_POINT('Ctrl Pts',(9.58389701199994,15.2,-4.58701234700001));
#178338=CARTESIAN_POINT('Ctrl Pts',(9.58389701199994,11.6,-4.58701234700001));
#178339=CARTESIAN_POINT('Ctrl Pts',(9.58220270699995,15.2,-4.58564365500001));
#178340=CARTESIAN_POINT('Ctrl Pts',(9.58220270699995,11.6,-4.58564365500001));
#178341=CARTESIAN_POINT('Ctrl Pts',(9.58051242199994,15.2,-4.58428068800002));
#178342=CARTESIAN_POINT('Ctrl Pts',(9.58051242199994,11.6,-4.58428068800002));
#178343=CARTESIAN_POINT('Ctrl Pts',(9.57882617099994,15.2,-4.58292344400002));
#178344=CARTESIAN_POINT('Ctrl Pts',(9.57882617099994,11.6,-4.58292344400002));
#178345=CARTESIAN_POINT('Ctrl Pts',(9.57714397399995,15.2,-4.58157192400002));
#178346=CARTESIAN_POINT('Ctrl Pts',(9.57714397399995,11.6,-4.58157192400002));
#178347=CARTESIAN_POINT('Ctrl Pts',(9.57546584599994,15.2,-4.58022613000002));
#178348=CARTESIAN_POINT('Ctrl Pts',(9.57546584599994,11.6,-4.58022613000002));
#178349=CARTESIAN_POINT('Ctrl Pts',(9.57379180899995,15.2,-4.57888606200001));
#178350=CARTESIAN_POINT('Ctrl Pts',(9.57379180899995,11.6,-4.57888606200001));
#178351=CARTESIAN_POINT('Ctrl Pts',(9.57212187699995,15.2,-4.57755172000001));
#178352=CARTESIAN_POINT('Ctrl Pts',(9.57212187699995,11.6,-4.57755172000002));
#178353=CARTESIAN_POINT('Ctrl Pts',(9.57045606999994,15.2,-4.57622310400001));
#178354=CARTESIAN_POINT('Ctrl Pts',(9.57045606999994,11.6,-4.57622310400002));
#178355=CARTESIAN_POINT('Ctrl Pts',(9.56879440599995,15.2,-4.57490021400002));
#178356=CARTESIAN_POINT('Ctrl Pts',(9.56879440599995,11.6,-4.57490021400002));
#178357=CARTESIAN_POINT('Ctrl Pts',(9.56713690099994,15.2,-4.57358305200001));
#178358=CARTESIAN_POINT('Ctrl Pts',(9.56713690099994,11.6,-4.57358305200002));
#178359=CARTESIAN_POINT('Ctrl Pts',(9.56548357399994,15.2,-4.57227161800001));
#178360=CARTESIAN_POINT('Ctrl Pts',(9.56548357399994,11.6,-4.57227161800002));
#178361=CARTESIAN_POINT('Ctrl Pts',(9.56383444399994,15.2,-4.57096591100001));
#178362=CARTESIAN_POINT('Ctrl Pts',(9.56383444399994,11.6,-4.57096591100001));
#178363=CARTESIAN_POINT('Ctrl Pts',(9.56218952899994,15.2,-4.56966593300002));
#178364=CARTESIAN_POINT('Ctrl Pts',(9.56218952899994,11.6,-4.56966593300002));
#178365=CARTESIAN_POINT('Ctrl Pts',(9.56054884799994,15.2,-4.56837168300002));
#178366=CARTESIAN_POINT('Ctrl Pts',(9.56054884799994,11.6,-4.56837168300002));
#178367=CARTESIAN_POINT('Ctrl Pts',(9.55891241699995,15.2,-4.56708316300002));
#178368=CARTESIAN_POINT('Ctrl Pts',(9.55891241699995,11.6,-4.56708316300002));
#178369=CARTESIAN_POINT('Ctrl Pts',(9.55728025499995,15.2,-4.56580037200002));
#178370=CARTESIAN_POINT('Ctrl Pts',(9.55728025499995,11.6,-4.56580037200002));
#178371=CARTESIAN_POINT('Ctrl Pts',(9.55565238299994,15.2,-4.56452331000001));
#178372=CARTESIAN_POINT('Ctrl Pts',(9.55565238299994,11.6,-4.56452331000001));
#178373=CARTESIAN_POINT('Ctrl Pts',(9.55402881599994,15.2,-4.56325197900001));
#178374=CARTESIAN_POINT('Ctrl Pts',(9.55402881599994,11.6,-4.56325197900001));
#178375=CARTESIAN_POINT('Ctrl Pts',(9.55240957399995,15.2,-4.56198637800002));
#178376=CARTESIAN_POINT('Ctrl Pts',(9.55240957399995,11.6,-4.56198637800002));
#178377=CARTESIAN_POINT('Ctrl Pts',(9.55079467599995,15.2,-4.56072650800001));
#178378=CARTESIAN_POINT('Ctrl Pts',(9.55079467599995,11.6,-4.56072650800001));
#178379=CARTESIAN_POINT('Ctrl Pts',(9.54918413999994,15.2,-4.55947236900001));
#178380=CARTESIAN_POINT('Ctrl Pts',(9.54918413999994,11.6,-4.55947236900002));
#178381=CARTESIAN_POINT('Ctrl Pts',(9.54757798599994,15.2,-4.55822396200002));
#178382=CARTESIAN_POINT('Ctrl Pts',(9.54757798599994,11.6,-4.55822396200002));
#178383=CARTESIAN_POINT('Ctrl Pts',(9.54597623199994,15.2,-4.55698128600002));
#178384=CARTESIAN_POINT('Ctrl Pts',(9.54597623199994,11.6,-4.55698128600002));
#178385=CARTESIAN_POINT('Ctrl Pts',(9.54437889599994,15.2,-4.55574434100001));
#178386=CARTESIAN_POINT('Ctrl Pts',(9.54437889599994,11.6,-4.55574434100001));
#178387=CARTESIAN_POINT('Ctrl Pts',(9.54278599799995,15.2,-4.55451312900002));
#178388=CARTESIAN_POINT('Ctrl Pts',(9.54278599799995,11.6,-4.55451312900002));
#178389=CARTESIAN_POINT('Ctrl Pts',(9.54119755599995,15.2,-4.55328764900001));
#178390=CARTESIAN_POINT('Ctrl Pts',(9.54119755599995,11.6,-4.55328764900001));
#178391=CARTESIAN_POINT('Ctrl Pts',(9.53961358999995,15.2,-4.55206790100001));
#178392=CARTESIAN_POINT('Ctrl Pts',(9.53961358999995,11.6,-4.55206790100002));
#178393=CARTESIAN_POINT('Ctrl Pts',(9.53803411899995,15.2,-4.55085388600001));
#178394=CARTESIAN_POINT('Ctrl Pts',(9.53803411899995,11.6,-4.55085388600002));
#178395=CARTESIAN_POINT('Ctrl Pts',(9.53645916199994,15.2,-4.54964560500001));
#178396=CARTESIAN_POINT('Ctrl Pts',(9.53645916199994,11.6,-4.54964560500002));
#178397=CARTESIAN_POINT('Ctrl Pts',(9.53488873799994,15.2,-4.54844305600002));
#178398=CARTESIAN_POINT('Ctrl Pts',(9.53488873799994,11.6,-4.54844305600002));
#178399=CARTESIAN_POINT('Ctrl Pts',(9.53332286699995,15.2,-4.54724624000002));
#178400=CARTESIAN_POINT('Ctrl Pts',(9.53332286699995,11.6,-4.54724624000002));
#178401=CARTESIAN_POINT('Ctrl Pts',(9.53176156699995,15.2,-4.54605515800001));
#178402=CARTESIAN_POINT('Ctrl Pts',(9.53176156699995,11.6,-4.54605515800001));
#178403=CARTESIAN_POINT('Ctrl Pts',(9.53020485899994,15.2,-4.54486981000001));
#178404=CARTESIAN_POINT('Ctrl Pts',(9.53020485899994,11.6,-4.54486981000001));
#178405=CARTESIAN_POINT('Ctrl Pts',(9.52865276099994,15.2,-4.54369019500001));
#178406=CARTESIAN_POINT('Ctrl Pts',(9.52865276099994,11.6,-4.54369019500002));
#178407=CARTESIAN_POINT('Ctrl Pts',(9.52710529499995,15.2,-4.54251631400002));
#178408=CARTESIAN_POINT('Ctrl Pts',(9.52710529499995,11.6,-4.54251631400002));
#178409=CARTESIAN_POINT('Ctrl Pts',(9.52556247699994,15.2,-4.54134816700002));
#178410=CARTESIAN_POINT('Ctrl Pts',(9.52556247699994,11.6,-4.54134816700002));
#178411=CARTESIAN_POINT('Ctrl Pts',(9.52402432899994,15.2,-4.54018575400001));
#178412=CARTESIAN_POINT('Ctrl Pts',(9.52402432899994,11.6,-4.54018575400002));
#178413=CARTESIAN_POINT('Ctrl Pts',(9.52249087199995,15.2,-4.53902907500002));
#178414=CARTESIAN_POINT('Ctrl Pts',(9.52249087199995,11.6,-4.53902907500002));
#178415=CARTESIAN_POINT('Ctrl Pts',(9.52096212299995,15.2,-4.53787813200002));
#178416=CARTESIAN_POINT('Ctrl Pts',(9.52096212299995,11.6,-4.53787813200002));
#178417=CARTESIAN_POINT('Ctrl Pts',(9.51943810399994,15.2,-4.53673292200001));
#178418=CARTESIAN_POINT('Ctrl Pts',(9.51943810399994,11.6,-4.53673292200001));
#178419=CARTESIAN_POINT('Ctrl Pts',(9.51791883399994,15.2,-4.53559344600002));
#178420=CARTESIAN_POINT('Ctrl Pts',(9.51791883399994,11.6,-4.53559344600002));
#178421=CARTESIAN_POINT('Ctrl Pts',(9.51640433299995,15.2,-4.53445970600002));
#178422=CARTESIAN_POINT('Ctrl Pts',(9.51640433299995,11.6,-4.53445970600002));
#178423=CARTESIAN_POINT('Ctrl Pts',(9.51489462199994,15.2,-4.53333169900001));
#178424=CARTESIAN_POINT('Ctrl Pts',(9.51489462199994,11.6,-4.53333169900001));
#178425=CARTESIAN_POINT('Ctrl Pts',(9.51338971899995,15.2,-4.53220942700002));
#178426=CARTESIAN_POINT('Ctrl Pts',(9.51338971899995,11.6,-4.53220942700002));
#178427=CARTESIAN_POINT('Ctrl Pts',(9.51188964699995,15.2,-4.53109288900002));
#178428=CARTESIAN_POINT('Ctrl Pts',(9.51188964699995,11.6,-4.53109288900002));
#178429=CARTESIAN_POINT('Ctrl Pts',(9.51039442599994,15.2,-4.52998208700001));
#178430=CARTESIAN_POINT('Ctrl Pts',(9.51039442599994,11.6,-4.52998208700001));
#178431=CARTESIAN_POINT('Ctrl Pts',(9.50890407399994,15.2,-4.52887701800002));
#178432=CARTESIAN_POINT('Ctrl Pts',(9.50890407399994,11.6,-4.52887701800002));
#178433=CARTESIAN_POINT('Ctrl Pts',(9.50741861299995,15.2,-4.52777768500002));
#178434=CARTESIAN_POINT('Ctrl Pts',(9.50741861299995,11.6,-4.52777768500002));
#178435=CARTESIAN_POINT('Ctrl Pts',(9.50593806399995,15.2,-4.52668408600001));
#178436=CARTESIAN_POINT('Ctrl Pts',(9.50593806399995,11.6,-4.52668408600002));
#178437=CARTESIAN_POINT('Ctrl Pts',(9.50446244799994,15.2,-4.52559622000001));
#178438=CARTESIAN_POINT('Ctrl Pts',(9.50446244799994,11.6,-4.52559622000001));
#178439=CARTESIAN_POINT('Ctrl Pts',(9.50299178499994,15.2,-4.52451409000002));
#178440=CARTESIAN_POINT('Ctrl Pts',(9.50299178499994,11.6,-4.52451409000002));
#178441=CARTESIAN_POINT('Ctrl Pts',(9.50152609399994,15.2,-4.52343769300001));
#178442=CARTESIAN_POINT('Ctrl Pts',(9.50152609399994,11.6,-4.52343769300002));
#178443=CARTESIAN_POINT('Ctrl Pts',(9.50006539899995,15.2,-4.52236703200001));
#178444=CARTESIAN_POINT('Ctrl Pts',(9.50006539899995,11.6,-4.52236703200002));
#178445=CARTESIAN_POINT('Ctrl Pts',(9.49860971899994,15.2,-4.52130210400002));
#178446=CARTESIAN_POINT('Ctrl Pts',(9.49860971899994,11.6,-4.52130210400002));
#178447=CARTESIAN_POINT('Ctrl Pts',(9.49715907499994,15.2,-4.52024291000001));
#178448=CARTESIAN_POINT('Ctrl Pts',(9.49715907499994,11.6,-4.52024291000001));
#178449=CARTESIAN_POINT('Ctrl Pts',(9.49571348799994,15.2,-4.51918944900001));
#178450=CARTESIAN_POINT('Ctrl Pts',(9.49571348799994,11.6,-4.51918944900001));
#178451=CARTESIAN_POINT('Ctrl Pts',(9.49427298099994,15.2,-4.51814172300002));
#178452=CARTESIAN_POINT('Ctrl Pts',(9.49427298099994,11.6,-4.51814172300002));
#178453=CARTESIAN_POINT('Ctrl Pts',(9.49283757399994,15.2,-4.51709973000002));
#178454=CARTESIAN_POINT('Ctrl Pts',(9.49283757399994,11.6,-4.51709973000002));
#178455=CARTESIAN_POINT('Ctrl Pts',(9.49140728699994,15.2,-4.51606347000002));
#178456=CARTESIAN_POINT('Ctrl Pts',(9.49140728699994,11.6,-4.51606347000002));
#178457=CARTESIAN_POINT('Ctrl Pts',(9.48998214199994,15.2,-4.51503294400001));
#178458=CARTESIAN_POINT('Ctrl Pts',(9.48998214199994,11.6,-4.51503294400002));
#178459=CARTESIAN_POINT('Ctrl Pts',(9.48856216199994,15.2,-4.51400815100001));
#178460=CARTESIAN_POINT('Ctrl Pts',(9.48856216199994,11.6,-4.51400815100001));
#178461=CARTESIAN_POINT('Ctrl Pts',(9.48714736699995,15.2,-4.51298909100001));
#178462=CARTESIAN_POINT('Ctrl Pts',(9.48714736699995,11.6,-4.51298909100002));
#178463=CARTESIAN_POINT('Ctrl Pts',(9.48573777999994,15.2,-4.51197576300002));
#178464=CARTESIAN_POINT('Ctrl Pts',(9.48573777999994,11.6,-4.51197576300002));
#178465=CARTESIAN_POINT('Ctrl Pts',(9.48433342199994,15.2,-4.51096816700002));
#178466=CARTESIAN_POINT('Ctrl Pts',(9.48433342199994,11.6,-4.51096816700002));
#178467=CARTESIAN_POINT('Ctrl Pts',(9.48293431399994,15.2,-4.50996630300001));
#178468=CARTESIAN_POINT('Ctrl Pts',(9.48293431399994,11.6,-4.50996630300002));
#178469=CARTESIAN_POINT('Ctrl Pts',(9.48154047899994,15.2,-4.50897017200001));
#178470=CARTESIAN_POINT('Ctrl Pts',(9.48154047899994,11.6,-4.50897017200001));
#178471=CARTESIAN_POINT('Ctrl Pts',(9.48015193699994,15.2,-4.50797977200001));
#178472=CARTESIAN_POINT('Ctrl Pts',(9.48015193699994,11.6,-4.50797977200002));
#178473=CARTESIAN_POINT('Ctrl Pts',(9.47876871299994,15.2,-4.50699510200002));
#178474=CARTESIAN_POINT('Ctrl Pts',(9.47876871299994,11.6,-4.50699510200002));
#178475=CARTESIAN_POINT('Ctrl Pts',(9.47739082699995,15.2,-4.50601616500002));
#178476=CARTESIAN_POINT('Ctrl Pts',(9.47739082699995,11.6,-4.50601616500002));
#178477=CARTESIAN_POINT('Ctrl Pts',(9.47601830199994,15.2,-4.50504295800001));
#178478=CARTESIAN_POINT('Ctrl Pts',(9.47601830199994,11.6,-4.50504295800001));
#178479=CARTESIAN_POINT('Ctrl Pts',(9.47465115999995,15.2,-4.50407548100001));
#178480=CARTESIAN_POINT('Ctrl Pts',(9.47465115999995,11.6,-4.50407548100001));
#178481=CARTESIAN_POINT('Ctrl Pts',(9.47328942199994,15.2,-4.50311373400002));
#178482=CARTESIAN_POINT('Ctrl Pts',(9.47328942199994,11.6,-4.50311373400002));
#178483=CARTESIAN_POINT('Ctrl Pts',(9.47193311299994,15.2,-4.50215771600002));
#178484=CARTESIAN_POINT('Ctrl Pts',(9.47193311299994,11.6,-4.50215771600002));
#178485=CARTESIAN_POINT('Ctrl Pts',(9.47058225499994,15.2,-4.50120742900001));
#178486=CARTESIAN_POINT('Ctrl Pts',(9.47058225499994,11.6,-4.50120742900001));
#178487=CARTESIAN_POINT('Ctrl Pts',(9.46923686899994,15.2,-4.50026286900002));
#178488=CARTESIAN_POINT('Ctrl Pts',(9.46923686899994,11.6,-4.50026286900002));
#178489=CARTESIAN_POINT('Ctrl Pts',(9.46789697899994,15.2,-4.49932403800001));
#178490=CARTESIAN_POINT('Ctrl Pts',(9.46789697899994,11.6,-4.49932403800002));
#178491=CARTESIAN_POINT('Ctrl Pts',(9.46656260799994,15.2,-4.49839093600001));
#178492=CARTESIAN_POINT('Ctrl Pts',(9.46656260799994,11.6,-4.49839093600001));
#178493=CARTESIAN_POINT('Ctrl Pts',(9.46523377699994,15.2,-4.49746356000002));
#178494=CARTESIAN_POINT('Ctrl Pts',(9.46523377699994,11.6,-4.49746356000002));
#178495=CARTESIAN_POINT('Ctrl Pts',(9.46391051099994,15.2,-4.49654191200001));
#178496=CARTESIAN_POINT('Ctrl Pts',(9.46391051099994,11.6,-4.49654191200001));
#178497=CARTESIAN_POINT('Ctrl Pts',(9.46259283199995,15.2,-4.49562599100001));
#178498=CARTESIAN_POINT('Ctrl Pts',(9.46259283199995,11.6,-4.49562599100001));
#178499=CARTESIAN_POINT('Ctrl Pts',(9.46128076299994,15.2,-4.49471579600001));
#178500=CARTESIAN_POINT('Ctrl Pts',(9.46128076299994,11.6,-4.49471579600001));
#178501=CARTESIAN_POINT('Ctrl Pts',(9.45997432899994,15.2,-4.49381132600001));
#178502=CARTESIAN_POINT('Ctrl Pts',(9.45997432899994,11.6,-4.49381132600002));
#178503=CARTESIAN_POINT('Ctrl Pts',(9.45867355199994,15.2,-4.49291258200001));
#178504=CARTESIAN_POINT('Ctrl Pts',(9.45867355199994,11.6,-4.49291258200002));
#178505=CARTESIAN_POINT('Ctrl Pts',(9.45737845499995,15.2,-4.49201956300001));
#178506=CARTESIAN_POINT('Ctrl Pts',(9.45737845499995,11.6,-4.49201956300001));
#178507=CARTESIAN_POINT('Ctrl Pts',(9.45608906199995,15.2,-4.49113226700002));
#178508=CARTESIAN_POINT('Ctrl Pts',(9.45608906199995,11.6,-4.49113226700002));
#178509=CARTESIAN_POINT('Ctrl Pts',(9.45480539699994,15.2,-4.49025069500002));
#178510=CARTESIAN_POINT('Ctrl Pts',(9.45480539699994,11.6,-4.49025069500002));
#178511=CARTESIAN_POINT('Ctrl Pts',(9.45352748199995,15.2,-4.48937484700001));
#178512=CARTESIAN_POINT('Ctrl Pts',(9.45352748199995,11.6,-4.48937484700001));
#178513=CARTESIAN_POINT('Ctrl Pts',(9.45225534299994,15.2,-4.48850472100002));
#178514=CARTESIAN_POINT('Ctrl Pts',(9.45225534299994,11.6,-4.48850472100002));
#178515=CARTESIAN_POINT('Ctrl Pts',(9.45098900299995,15.2,-4.48764031700001));
#178516=CARTESIAN_POINT('Ctrl Pts',(9.45098900299995,11.6,-4.48764031700002));
#178517=CARTESIAN_POINT('Ctrl Pts',(9.44972848499994,15.2,-4.48678163300002));
#178518=CARTESIAN_POINT('Ctrl Pts',(9.44972848499994,11.6,-4.48678163300002));
#178519=CARTESIAN_POINT('Ctrl Pts',(9.44847381499994,15.2,-4.48592867100002));
#178520=CARTESIAN_POINT('Ctrl Pts',(9.44847381499994,11.6,-4.48592867100002));
#178521=CARTESIAN_POINT('Ctrl Pts',(9.44722501599994,15.2,-4.48508142800002));
#178522=CARTESIAN_POINT('Ctrl Pts',(9.44722501599994,11.6,-4.48508142800002));
#178523=CARTESIAN_POINT('Ctrl Pts',(9.44598211199994,15.2,-4.48423990500002));
#178524=CARTESIAN_POINT('Ctrl Pts',(9.44598211199994,11.6,-4.48423990500002));
#178525=CARTESIAN_POINT('Ctrl Pts',(9.44474512899994,15.2,-4.48340410000001));
#178526=CARTESIAN_POINT('Ctrl Pts',(9.44474512899994,11.6,-4.48340410000002));
#178527=CARTESIAN_POINT('Ctrl Pts',(9.44351408899994,15.2,-4.48257401400001));
#178528=CARTESIAN_POINT('Ctrl Pts',(9.44351408899994,11.6,-4.48257401400001));
#178529=CARTESIAN_POINT('Ctrl Pts',(9.44228901899995,15.2,-4.48174964400001));
#178530=CARTESIAN_POINT('Ctrl Pts',(9.44228901899995,11.6,-4.48174964400002));
#178531=CARTESIAN_POINT('Ctrl Pts',(9.44106994199995,15.2,-4.48093099100001));
#178532=CARTESIAN_POINT('Ctrl Pts',(9.44106994199995,11.6,-4.48093099100001));
#178533=CARTESIAN_POINT('Ctrl Pts',(9.43985688299994,15.2,-4.48011805400002));
#178534=CARTESIAN_POINT('Ctrl Pts',(9.43985688299994,11.6,-4.48011805400002));
#178535=CARTESIAN_POINT('Ctrl Pts',(9.43864986699994,15.2,-4.47931083200002));
#178536=CARTESIAN_POINT('Ctrl Pts',(9.43864986699994,11.6,-4.47931083200002));
#178537=CARTESIAN_POINT('Ctrl Pts',(9.43744891899994,15.2,-4.47850932400002));
#178538=CARTESIAN_POINT('Ctrl Pts',(9.43744891899994,11.6,-4.47850932400002));
#178539=CARTESIAN_POINT('Ctrl Pts',(9.43625406499994,15.2,-4.47771352900002));
#178540=CARTESIAN_POINT('Ctrl Pts',(9.43625406499994,11.6,-4.47771352900002));
#178541=CARTESIAN_POINT('Ctrl Pts',(9.43506532899995,15.2,-4.47692344800001));
#178542=CARTESIAN_POINT('Ctrl Pts',(9.43506532899995,11.6,-4.47692344800002));
#178543=CARTESIAN_POINT('Ctrl Pts',(9.43388273599994,15.2,-4.47613907800001));
#178544=CARTESIAN_POINT('Ctrl Pts',(9.43388273599994,11.6,-4.47613907800002));
#178545=CARTESIAN_POINT('Ctrl Pts',(9.43270631299994,15.2,-4.47536041800001));
#178546=CARTESIAN_POINT('Ctrl Pts',(9.43270631299994,11.6,-4.47536041800001));
#178547=CARTESIAN_POINT('Ctrl Pts',(9.43153608499994,15.2,-4.47458746900002));
#178548=CARTESIAN_POINT('Ctrl Pts',(9.43153608499994,11.6,-4.47458746900002));
#178549=CARTESIAN_POINT('Ctrl Pts',(9.43037207599994,15.2,-4.47382023000001));
#178550=CARTESIAN_POINT('Ctrl Pts',(9.43037207599994,11.6,-4.47382023000001));
#178551=CARTESIAN_POINT('Ctrl Pts',(9.42921431399995,15.2,-4.47305869800001));
#178552=CARTESIAN_POINT('Ctrl Pts',(9.42921431399995,11.6,-4.47305869800002));
#178553=CARTESIAN_POINT('Ctrl Pts',(9.42806282299994,15.2,-4.47230287400001));
#178554=CARTESIAN_POINT('Ctrl Pts',(9.42806282299994,11.6,-4.47230287400001));
#178555=CARTESIAN_POINT('Ctrl Pts',(9.42691762999995,15.2,-4.47155275600001));
#178556=CARTESIAN_POINT('Ctrl Pts',(9.42691762999995,11.6,-4.47155275600002));
#178557=CARTESIAN_POINT('Ctrl Pts',(9.42577875999994,15.2,-4.47080834400001));
#178558=CARTESIAN_POINT('Ctrl Pts',(9.42577875999994,11.6,-4.47080834400001));
#178559=CARTESIAN_POINT('Ctrl Pts',(9.42464624099994,15.2,-4.47006963700002));
#178560=CARTESIAN_POINT('Ctrl Pts',(9.42464624099994,11.6,-4.47006963700002));
#178561=CARTESIAN_POINT('Ctrl Pts',(9.42352009699994,15.2,-4.46933663400001));
#178562=CARTESIAN_POINT('Ctrl Pts',(9.42352009699994,11.6,-4.46933663400001));
#178563=CARTESIAN_POINT('Ctrl Pts',(9.42240035499994,15.2,-4.46860933200002));
#178564=CARTESIAN_POINT('Ctrl Pts',(9.42240035499994,11.6,-4.46860933200002));
#178565=CARTESIAN_POINT('Ctrl Pts',(9.42128704299994,15.2,-4.46788773300002));
#178566=CARTESIAN_POINT('Ctrl Pts',(9.42128704299994,11.6,-4.46788773300002));
#178567=CARTESIAN_POINT('Ctrl Pts',(9.42018018699994,15.2,-4.46717183400001));
#178568=CARTESIAN_POINT('Ctrl Pts',(9.42018018699994,11.6,-4.46717183400002));
#178569=CARTESIAN_POINT('Ctrl Pts',(9.41907981199994,15.2,-4.46646163500001));
#178570=CARTESIAN_POINT('Ctrl Pts',(9.41907981199994,11.6,-4.46646163500002));
#178571=CARTESIAN_POINT('Ctrl Pts',(9.41798594799995,15.2,-4.46575713300001));
#178572=CARTESIAN_POINT('Ctrl Pts',(9.41798594799995,11.6,-4.46575713300002));
#178573=CARTESIAN_POINT('Ctrl Pts',(9.41689861899994,15.2,-4.46505832900002));
#178574=CARTESIAN_POINT('Ctrl Pts',(9.41689861899994,11.6,-4.46505832900002));
#178575=CARTESIAN_POINT('Ctrl Pts',(9.41581785299995,15.2,-4.46436522100001));
#178576=CARTESIAN_POINT('Ctrl Pts',(9.41581785299995,11.6,-4.46436522100001));
#178577=CARTESIAN_POINT('Ctrl Pts',(9.41474367699995,15.2,-4.46367780900002));
#178578=CARTESIAN_POINT('Ctrl Pts',(9.41474367699995,11.6,-4.46367780900002));
#178579=CARTESIAN_POINT('Ctrl Pts',(9.41367611899994,15.2,-4.46299609100001));
#178580=CARTESIAN_POINT('Ctrl Pts',(9.41367611899994,11.6,-4.46299609100001));
#178581=CARTESIAN_POINT('Ctrl Pts',(9.41261520599994,15.2,-4.46232006500002));
#178582=CARTESIAN_POINT('Ctrl Pts',(9.41261520599994,11.6,-4.46232006500002));
#178583=CARTESIAN_POINT('Ctrl Pts',(9.41156096599994,15.2,-4.46164973100001));
#178584=CARTESIAN_POINT('Ctrl Pts',(9.41156096599994,11.6,-4.46164973100002));
#178585=CARTESIAN_POINT('Ctrl Pts',(9.41051342599994,15.2,-4.46098508800001));
#178586=CARTESIAN_POINT('Ctrl Pts',(9.41051342599994,11.6,-4.46098508800001));
#178587=CARTESIAN_POINT('Ctrl Pts',(9.40947261499995,15.2,-4.46032613400002));
#178588=CARTESIAN_POINT('Ctrl Pts',(9.40947261499995,11.6,-4.46032613400002));
#178589=CARTESIAN_POINT('Ctrl Pts',(9.40843855899995,15.2,-4.45967286700002));
#178590=CARTESIAN_POINT('Ctrl Pts',(9.40843855899995,11.6,-4.45967286700002));
#178591=CARTESIAN_POINT('Ctrl Pts',(9.40741128799995,15.2,-4.45902528700001));
#178592=CARTESIAN_POINT('Ctrl Pts',(9.40741128799995,11.6,-4.45902528700001));
#178593=CARTESIAN_POINT('Ctrl Pts',(9.40639082799994,15.2,-4.45838339300002));
#178594=CARTESIAN_POINT('Ctrl Pts',(9.40639082799994,11.6,-4.45838339300002));
#178595=CARTESIAN_POINT('Ctrl Pts',(9.40537720899994,15.2,-4.45774718300001));
#178596=CARTESIAN_POINT('Ctrl Pts',(9.40537720899994,11.6,-4.45774718300001));
#178597=CARTESIAN_POINT('Ctrl Pts',(9.40437045999994,15.2,-4.45711665500002));
#178598=CARTESIAN_POINT('Ctrl Pts',(9.40437045999994,11.6,-4.45711665500002));
#178599=CARTESIAN_POINT('Ctrl Pts',(9.40337060799994,15.2,-4.45649181000002));
#178600=CARTESIAN_POINT('Ctrl Pts',(9.40337060799994,11.6,-4.45649181000002));
#178601=CARTESIAN_POINT('Ctrl Pts',(9.40237768099994,15.2,-4.45587264400002));
#178602=CARTESIAN_POINT('Ctrl Pts',(9.40237768099994,11.6,-4.45587264400002));
#178603=CARTESIAN_POINT('Ctrl Pts',(9.40139171099995,15.2,-4.45525915600001));
#178604=CARTESIAN_POINT('Ctrl Pts',(9.40139171099995,11.6,-4.45525915600001));
#178605=CARTESIAN_POINT('Ctrl Pts',(9.40041272399995,15.2,-4.45465134700001));
#178606=CARTESIAN_POINT('Ctrl Pts',(9.40041272399995,11.6,-4.45465134700001));
#178607=CARTESIAN_POINT('Ctrl Pts',(9.39944075099995,15.2,-4.45404921300002));
#178608=CARTESIAN_POINT('Ctrl Pts',(9.39944075099995,11.6,-4.45404921300002));
#178609=CARTESIAN_POINT('Ctrl Pts',(9.39847581899994,15.2,-4.45345275400001));
#178610=CARTESIAN_POINT('Ctrl Pts',(9.39847581899994,11.6,-4.45345275400001));
#178611=CARTESIAN_POINT('Ctrl Pts',(9.39751795899994,15.2,-4.45286196700001));
#178612=CARTESIAN_POINT('Ctrl Pts',(9.39751795899994,11.6,-4.45286196700002));
#178613=CARTESIAN_POINT('Ctrl Pts',(9.39656720199994,15.2,-4.45227685300001));
#178614=CARTESIAN_POINT('Ctrl Pts',(9.39656720199994,11.6,-4.45227685300001));
#178615=CARTESIAN_POINT('Ctrl Pts',(9.39562357399994,15.2,-4.45169740800001));
#178616=CARTESIAN_POINT('Ctrl Pts',(9.39562357399994,11.6,-4.45169740800001));
#178617=CARTESIAN_POINT('Ctrl Pts',(9.39468710699994,15.2,-4.45112363100002));
#178618=CARTESIAN_POINT('Ctrl Pts',(9.39468710699994,11.6,-4.45112363100002));
#178619=CARTESIAN_POINT('Ctrl Pts',(9.39375783099995,15.2,-4.45055552200001));
#178620=CARTESIAN_POINT('Ctrl Pts',(9.39375783099995,11.6,-4.45055552200001));
#178621=CARTESIAN_POINT('Ctrl Pts',(9.39283577499994,15.2,-4.44999307800002));
#178622=CARTESIAN_POINT('Ctrl Pts',(9.39283577499994,11.6,-4.44999307800002));
#178623=CARTESIAN_POINT('Ctrl Pts',(9.39192097099994,15.2,-4.44943629800001));
#178624=CARTESIAN_POINT('Ctrl Pts',(9.39192097099994,11.6,-4.44943629800001));
#178625=CARTESIAN_POINT('Ctrl Pts',(9.39101344699995,15.2,-4.44888518000001));
#178626=CARTESIAN_POINT('Ctrl Pts',(9.39101344699995,11.6,-4.44888518000001));
#178627=CARTESIAN_POINT('Ctrl Pts',(9.39011323499994,15.2,-4.44833972300001));
#178628=CARTESIAN_POINT('Ctrl Pts',(9.39011323499994,11.6,-4.44833972300002));
#178629=CARTESIAN_POINT('Ctrl Pts',(9.38922036599994,15.2,-4.44779992400001));
#178630=CARTESIAN_POINT('Ctrl Pts',(9.38922036599994,11.6,-4.44779992400001));
#178631=CARTESIAN_POINT('Ctrl Pts',(9.38833486899994,15.2,-4.44726578300001));
#178632=CARTESIAN_POINT('Ctrl Pts',(9.38833486899994,11.6,-4.44726578300001));
#178633=CARTESIAN_POINT('Ctrl Pts',(9.38745677599995,15.2,-4.44673729700002));
#178634=CARTESIAN_POINT('Ctrl Pts',(9.38745677599995,11.6,-4.44673729700002));
#178635=CARTESIAN_POINT('Ctrl Pts',(9.38658611799994,15.2,-4.44621446500001));
#178636=CARTESIAN_POINT('Ctrl Pts',(9.38658611799994,11.6,-4.44621446500001));
#178637=CARTESIAN_POINT('Ctrl Pts',(9.38572292599994,15.2,-4.44569728500001));
#178638=CARTESIAN_POINT('Ctrl Pts',(9.38572292599994,11.6,-4.44569728500001));
#178639=CARTESIAN_POINT('Ctrl Pts',(9.38486723299994,15.2,-4.44518575500001));
#178640=CARTESIAN_POINT('Ctrl Pts',(9.38486723299994,11.6,-4.44518575500001));
#178641=CARTESIAN_POINT('Ctrl Pts',(9.38401906799994,15.2,-4.44467987500001));
#178642=CARTESIAN_POINT('Ctrl Pts',(9.38401906799994,11.6,-4.44467987500001));
#178643=CARTESIAN_POINT('Ctrl Pts',(9.38317846499995,15.2,-4.44417964100001));
#178644=CARTESIAN_POINT('Ctrl Pts',(9.38317846499995,11.6,-4.44417964100001));
#178645=CARTESIAN_POINT('Ctrl Pts',(9.38234545299995,15.2,-4.44368505100002));
#178646=CARTESIAN_POINT('Ctrl Pts',(9.38234545299995,11.6,-4.44368505100002));
#178647=CARTESIAN_POINT('Ctrl Pts',(9.38152006799994,15.2,-4.44319610500001));
#178648=CARTESIAN_POINT('Ctrl Pts',(9.38152006799994,11.6,-4.44319610500001));
#178649=CARTESIAN_POINT('Ctrl Pts',(9.38070233899994,15.2,-4.44271280000001));
#178650=CARTESIAN_POINT('Ctrl Pts',(9.38070233899994,11.6,-4.44271280000002));
#178651=CARTESIAN_POINT('Ctrl Pts',(9.37989229799994,15.2,-4.44223513400001));
#178652=CARTESIAN_POINT('Ctrl Pts',(9.37989229799994,11.6,-4.44223513400001));
#178653=CARTESIAN_POINT('Ctrl Pts',(9.37908997999994,15.2,-4.44176310500001));
#178654=CARTESIAN_POINT('Ctrl Pts',(9.37908997999994,11.6,-4.44176310500001));
#178655=CARTESIAN_POINT('Ctrl Pts',(9.37829999299994,15.2,-4.44129939800002));
#178656=CARTESIAN_POINT('Ctrl Pts',(9.37829999299994,11.6,-4.44129939800002));
#178657=CARTESIAN_POINT('Ctrl Pts',(9.37767505799994,15.2,-4.44093341200002));
#178658=CARTESIAN_POINT('Ctrl Pts',(9.37767505799994,11.6,-4.44093341200002));
#178659=CARTESIAN_POINT('Ctrl Pts',(9.37721094099994,15.2,-4.44066207100001));
#178660=CARTESIAN_POINT('Ctrl Pts',(9.37721094099994,11.6,-4.44066207100002));
#178661=CARTESIAN_POINT('Ctrl Pts',(9.37690455299995,15.2,-4.44048314800002));
#178662=CARTESIAN_POINT('Ctrl Pts',(9.37690455299995,11.6,-4.44048314800002));
#178663=CARTESIAN_POINT('Ctrl Pts',(9.37675396699994,15.2,-4.44039525800001));
#178664=CARTESIAN_POINT('Ctrl Pts',(9.37675396699994,11.6,-4.44039525800001));
#178665=CARTESIAN_POINT('',(9.37675396699994,12.2,-4.44039525800001));
#178666=CARTESIAN_POINT('',(9.37675396699994,15.2,-4.44039525800001));
#178667=CARTESIAN_POINT('',(9.37675396699994,12.2,-4.44039525800001));
#178668=CARTESIAN_POINT('Ctrl Pts',(10.2217148779999,12.2,-5.26939701900002));
#178669=CARTESIAN_POINT('Ctrl Pts',(10.2212575739999,12.2,-5.26878426900002));
#178670=CARTESIAN_POINT('Ctrl Pts',(10.2203429999999,12.2,-5.26755929400001));
#178671=CARTESIAN_POINT('Ctrl Pts',(10.2189712369999,12.2,-5.26572340900001));
#178672=CARTESIAN_POINT('Ctrl Pts',(10.2171424209999,12.2,-5.26327871600001));
#178673=CARTESIAN_POINT('Ctrl Pts',(10.2148567309999,12.2,-5.26022810500002));
#178674=CARTESIAN_POINT('Ctrl Pts',(10.2125713739999,12.2,-5.25718275100001));
#178675=CARTESIAN_POINT('Ctrl Pts',(10.2102863519999,12.2,-5.25414265600002));
#178676=CARTESIAN_POINT('Ctrl Pts',(10.2080016679999,12.2,-5.25110781800001));
#178677=CARTESIAN_POINT('Ctrl Pts',(10.2057173299999,12.2,-5.24807824100002));
#178678=CARTESIAN_POINT('Ctrl Pts',(10.2034333439999,12.2,-5.24505392700001));
#178679=CARTESIAN_POINT('Ctrl Pts',(10.2011497209999,12.2,-5.24203487700001));
#178680=CARTESIAN_POINT('Ctrl Pts',(10.1988664679999,12.2,-5.23902109400002));
#178681=CARTESIAN_POINT('Ctrl Pts',(10.1965835999999,12.2,-5.23601258300001));
#178682=CARTESIAN_POINT('Ctrl Pts',(10.1943011249999,12.2,-5.23300934300002));
#178683=CARTESIAN_POINT('Ctrl Pts',(10.1920190549999,12.2,-5.23001138000001));
#178684=CARTESIAN_POINT('Ctrl Pts',(10.1897373969999,12.2,-5.22701869500001));
#178685=CARTESIAN_POINT('Ctrl Pts',(10.1874561619999,12.2,-5.22403129000002));
#178686=CARTESIAN_POINT('Ctrl Pts',(10.1851753559999,12.2,-5.22104916700001));
#178687=CARTESIAN_POINT('Ctrl Pts',(10.1828949879999,12.2,-5.21807232700001));
#178688=CARTESIAN_POINT('Ctrl Pts',(10.1806150639999,12.2,-5.21510077400002));
#178689=CARTESIAN_POINT('Ctrl Pts',(10.1783355949999,12.2,-5.21213451000001));
#178690=CARTESIAN_POINT('Ctrl Pts',(10.1760565879999,12.2,-5.20917353600002));
#178691=CARTESIAN_POINT('Ctrl Pts',(10.1737780519999,12.2,-5.20621785500001));
#178692=CARTESIAN_POINT('Ctrl Pts',(10.1714999969999,12.2,-5.20326746900002));
#178693=CARTESIAN_POINT('Ctrl Pts',(10.1692224309999,12.2,-5.20032238000002));
#178694=CARTESIAN_POINT('Ctrl Pts',(10.1669453649999,12.2,-5.19738259100002));
#178695=CARTESIAN_POINT('Ctrl Pts',(10.1646688079999,12.2,-5.19444810300001));
#178696=CARTESIAN_POINT('Ctrl Pts',(10.1623927679999,12.2,-5.19151892100002));
#178697=CARTESIAN_POINT('Ctrl Pts',(10.1601172529999,12.2,-5.18859504400002));
#178698=CARTESIAN_POINT('Ctrl Pts',(10.1578422729999,12.2,-5.18567647600001));
#178699=CARTESIAN_POINT('Ctrl Pts',(10.1555678379999,12.2,-5.18276321900002));
#178700=CARTESIAN_POINT('Ctrl Pts',(10.1532939539999,12.2,-5.17985527400001));
#178701=CARTESIAN_POINT('Ctrl Pts',(10.1510206309999,12.2,-5.17695264500002));
#178702=CARTESIAN_POINT('Ctrl Pts',(10.1487478799999,12.2,-5.17405533200002));
#178703=CARTESIAN_POINT('Ctrl Pts',(10.1464757069999,12.2,-5.17116333800002));
#178704=CARTESIAN_POINT('Ctrl Pts',(10.1442041239999,12.2,-5.16827666700001));
#178705=CARTESIAN_POINT('Ctrl Pts',(10.1419331389999,12.2,-5.16539531900001));
#178706=CARTESIAN_POINT('Ctrl Pts',(10.1396627609999,12.2,-5.16251929700001));
#178707=CARTESIAN_POINT('Ctrl Pts',(10.1373929979999,12.2,-5.15964860200001));
#178708=CARTESIAN_POINT('Ctrl Pts',(10.1351238609999,12.2,-5.15678323800001));
#178709=CARTESIAN_POINT('Ctrl Pts',(10.1328553589999,12.2,-5.15392320600002));
#178710=CARTESIAN_POINT('Ctrl Pts',(10.1305874999999,12.2,-5.15106851000001));
#178711=CARTESIAN_POINT('Ctrl Pts',(10.1283202939999,12.2,-5.14821914900002));
#178712=CARTESIAN_POINT('Ctrl Pts',(10.1260537499999,12.2,-5.14537512800001));
#178713=CARTESIAN_POINT('Ctrl Pts',(10.1237878759999,12.2,-5.14253644700001));
#178714=CARTESIAN_POINT('Ctrl Pts',(10.1215226839999,12.2,-5.13970310900001));
#178715=CARTESIAN_POINT('Ctrl Pts',(10.1192581799999,12.2,-5.13687511700001));
#178716=CARTESIAN_POINT('Ctrl Pts',(10.1169943759999,12.2,-5.13405247200001));
#178717=CARTESIAN_POINT('Ctrl Pts',(10.1147312799999,12.2,-5.13123517600001));
#178718=CARTESIAN_POINT('Ctrl Pts',(10.1124689019999,12.2,-5.12842323200001));
#178719=CARTESIAN_POINT('Ctrl Pts',(10.1102072499999,12.2,-5.12561664200001));
#178720=CARTESIAN_POINT('Ctrl Pts',(10.1079463349999,12.2,-5.12281540800001));
#178721=CARTESIAN_POINT('Ctrl Pts',(10.1056861639999,12.2,-5.12001953100001));
#178722=CARTESIAN_POINT('Ctrl Pts',(10.1034267499999,12.2,-5.11722901400002));
#178723=CARTESIAN_POINT('Ctrl Pts',(10.1011680999999,12.2,-5.11444386000001));
#178724=CARTESIAN_POINT('Ctrl Pts',(10.0989102229999,12.2,-5.11166406900001));
#178725=CARTESIAN_POINT('Ctrl Pts',(10.0966531299999,12.2,-5.10888964500001));
#178726=CARTESIAN_POINT('Ctrl Pts',(10.0943968289999,12.2,-5.10612059000001));
#178727=CARTESIAN_POINT('Ctrl Pts',(10.0921413299999,12.2,-5.10335690500002));
#178728=CARTESIAN_POINT('Ctrl Pts',(10.0898866439999,12.2,-5.10059859300001));
#178729=CARTESIAN_POINT('Ctrl Pts',(10.0876327779999,12.2,-5.09784565500001));
#178730=CARTESIAN_POINT('Ctrl Pts',(10.0853797429999,12.2,-5.09509809400001));
#178731=CARTESIAN_POINT('Ctrl Pts',(10.0831275479999,12.2,-5.09235591100001));
#178732=CARTESIAN_POINT('Ctrl Pts',(10.0808762039999,12.2,-5.08961911000001));
#178733=CARTESIAN_POINT('Ctrl Pts',(10.0786257189999,12.2,-5.08688769200001));
#178734=CARTESIAN_POINT('Ctrl Pts',(10.0763761029999,12.2,-5.08416165800002));
#178735=CARTESIAN_POINT('Ctrl Pts',(10.0741273649999,12.2,-5.08144101100001));
#178736=CARTESIAN_POINT('Ctrl Pts',(10.0718795159999,12.2,-5.07872575400001));
#178737=CARTESIAN_POINT('Ctrl Pts',(10.0696325649999,12.2,-5.07601588800001));
#178738=CARTESIAN_POINT('Ctrl Pts',(10.0673865209999,12.2,-5.07331141500002));
#178739=CARTESIAN_POINT('Ctrl Pts',(10.0651413949999,12.2,-5.07061233700002));
#178740=CARTESIAN_POINT('Ctrl Pts',(10.0628971959999,12.2,-5.06791865600002));
#178741=CARTESIAN_POINT('Ctrl Pts',(10.0606539349999,12.2,-5.06523037500001));
#178742=CARTESIAN_POINT('Ctrl Pts',(10.0584116189999,12.2,-5.06254749600001));
#178743=CARTESIAN_POINT('Ctrl Pts',(10.0561702599999,12.2,-5.05987001900001));
#178744=CARTESIAN_POINT('Ctrl Pts',(10.0539298679999,12.2,-5.05719794800001));
#178745=CARTESIAN_POINT('Ctrl Pts',(10.0516904509999,12.2,-5.05453128400001));
#178746=CARTESIAN_POINT('Ctrl Pts',(10.0494520199999,12.2,-5.05187002900001));
#178747=CARTESIAN_POINT('Ctrl Pts',(10.0472145849999,12.2,-5.04921418600001));
#178748=CARTESIAN_POINT('Ctrl Pts',(10.0449781559999,12.2,-5.04656375500002));
#178749=CARTESIAN_POINT('Ctrl Pts',(10.0427427419999,12.2,-5.04391874100001));
#178750=CARTESIAN_POINT('Ctrl Pts',(10.0405083539999,12.2,-5.04127914300001));
#178751=CARTESIAN_POINT('Ctrl Pts',(10.0382750009999,12.2,-5.03864496500002));
#178752=CARTESIAN_POINT('Ctrl Pts',(10.0360426939999,12.2,-5.03601620900001));
#178753=CARTESIAN_POINT('Ctrl Pts',(10.0338114419999,12.2,-5.03339287600001));
#178754=CARTESIAN_POINT('Ctrl Pts',(10.0315812549999,12.2,-5.03077496800001));
#178755=CARTESIAN_POINT('Ctrl Pts',(10.0293521449999,12.2,-5.02816248700002));
#178756=CARTESIAN_POINT('Ctrl Pts',(10.0271241189999,12.2,-5.02555543600002));
#178757=CARTESIAN_POINT('Ctrl Pts',(10.0248971889999,12.2,-5.02295381500002));
#178758=CARTESIAN_POINT('Ctrl Pts',(10.0226713639999,12.2,-5.02035762800002));
#178759=CARTESIAN_POINT('Ctrl Pts',(10.0204466549999,12.2,-5.01776687600001));
#178760=CARTESIAN_POINT('Ctrl Pts',(10.0182230729999,12.2,-5.01518156000001));
#178761=CARTESIAN_POINT('Ctrl Pts',(10.0160006259999,12.2,-5.01260168400002));
#178762=CARTESIAN_POINT('Ctrl Pts',(10.0137793259999,12.2,-5.01002724800002));
#178763=CARTESIAN_POINT('Ctrl Pts',(10.0115591819999,12.2,-5.00745825600001));
#178764=CARTESIAN_POINT('Ctrl Pts',(10.0093402039999,12.2,-5.00489470900002));
#178765=CARTESIAN_POINT('Ctrl Pts',(10.0071224029999,12.2,-5.00233660800002));
#178766=CARTESIAN_POINT('Ctrl Pts',(10.0049057889999,12.2,-4.99978395500001));
#178767=CARTESIAN_POINT('Ctrl Pts',(10.0026903729999,12.2,-4.99723675300002));
#178768=CARTESIAN_POINT('Ctrl Pts',(10.0004761639999,12.2,-4.99469500400001));
#178769=CARTESIAN_POINT('Ctrl Pts',(9.99826317399994,12.2,-4.99215870900001));
#178770=CARTESIAN_POINT('Ctrl Pts',(9.99605141199994,12.2,-4.98962787000002));
#178771=CARTESIAN_POINT('Ctrl Pts',(9.99384088799994,12.2,-4.98710249000001));
#178772=CARTESIAN_POINT('Ctrl Pts',(9.99163161399995,12.2,-4.98458256900001));
#178773=CARTESIAN_POINT('Ctrl Pts',(9.98942359899995,12.2,-4.98206811000002));
#178774=CARTESIAN_POINT('Ctrl Pts',(9.98721685399994,12.2,-4.97955911500001));
#178775=CARTESIAN_POINT('Ctrl Pts',(9.98501138999995,12.2,-4.97705558600002));
#178776=CARTESIAN_POINT('Ctrl Pts',(9.98280721699994,12.2,-4.97455752400001));
#178777=CARTESIAN_POINT('Ctrl Pts',(9.98060434499994,12.2,-4.97206493200002));
#178778=CARTESIAN_POINT('Ctrl Pts',(9.97840278499995,12.2,-4.96957781100001));
#178779=CARTESIAN_POINT('Ctrl Pts',(9.97620254699994,12.2,-4.96709616400001));
#178780=CARTESIAN_POINT('Ctrl Pts',(9.97400364199994,12.2,-4.96461999100001));
#178781=CARTESIAN_POINT('Ctrl Pts',(9.97180608099995,12.2,-4.96214929600002));
#178782=CARTESIAN_POINT('Ctrl Pts',(9.96960987299994,12.2,-4.95968407800001));
#178783=CARTESIAN_POINT('Ctrl Pts',(9.96741503199994,12.2,-4.95722434200002));
#178784=CARTESIAN_POINT('Ctrl Pts',(9.96522156599994,12.2,-4.95477008800002));
#178785=CARTESIAN_POINT('Ctrl Pts',(9.96302948499994,12.2,-4.95232131800002));
#178786=CARTESIAN_POINT('Ctrl Pts',(9.96083880199994,12.2,-4.94987803500001));
#178787=CARTESIAN_POINT('Ctrl Pts',(9.95864952599995,12.2,-4.94744023800001));
#178788=CARTESIAN_POINT('Ctrl Pts',(9.95646166799995,12.2,-4.94500793200002));
#178789=CARTESIAN_POINT('Ctrl Pts',(9.95427523999994,12.2,-4.94258111700002));
#178790=CARTESIAN_POINT('Ctrl Pts',(9.95209025099994,12.2,-4.94015979700002));
#178791=CARTESIAN_POINT('Ctrl Pts',(9.94990671399995,12.2,-4.93774397000001));
#178792=CARTESIAN_POINT('Ctrl Pts',(9.94772463699995,12.2,-4.93533364100001));
#178793=CARTESIAN_POINT('Ctrl Pts',(9.94554403299994,12.2,-4.93292881000002));
#178794=CARTESIAN_POINT('Ctrl Pts',(9.94336491299994,12.2,-4.93052948100001));
#178795=CARTESIAN_POINT('Ctrl Pts',(9.94118728699994,12.2,-4.92813565300001));
#178796=CARTESIAN_POINT('Ctrl Pts',(9.93901116599995,12.2,-4.92574732900001));
#178797=CARTESIAN_POINT('Ctrl Pts',(9.93683656099994,12.2,-4.92336451100002));
#178798=CARTESIAN_POINT('Ctrl Pts',(9.93466348399994,12.2,-4.92098720100001));
#178799=CARTESIAN_POINT('Ctrl Pts',(9.93249194399995,12.2,-4.91861540000002));
#178800=CARTESIAN_POINT('Ctrl Pts',(9.93032195399994,12.2,-4.91624911100002));
#178801=CARTESIAN_POINT('Ctrl Pts',(9.92815352399995,12.2,-4.91388833500002));
#178802=CARTESIAN_POINT('Ctrl Pts',(9.92598666499994,12.2,-4.91153307200001));
#178803=CARTESIAN_POINT('Ctrl Pts',(9.92382138899995,12.2,-4.90918332600002));
#178804=CARTESIAN_POINT('Ctrl Pts',(9.92165770599994,12.2,-4.90683909900001));
#178805=CARTESIAN_POINT('Ctrl Pts',(9.91949562799994,12.2,-4.90450039100002));
#178806=CARTESIAN_POINT('Ctrl Pts',(9.91733516599995,12.2,-4.90216720500001));
#178807=CARTESIAN_POINT('Ctrl Pts',(9.91517632999994,12.2,-4.89983954200001));
#178808=CARTESIAN_POINT('Ctrl Pts',(9.91301913399995,12.2,-4.89751740500001));
#178809=CARTESIAN_POINT('Ctrl Pts',(9.91086358699994,12.2,-4.89520079400001));
#178810=CARTESIAN_POINT('Ctrl Pts',(9.90870969999994,12.2,-4.89288971200001));
#178811=CARTESIAN_POINT('Ctrl Pts',(9.90655748599995,12.2,-4.89058415900002));
#178812=CARTESIAN_POINT('Ctrl Pts',(9.90440695499995,12.2,-4.88828413900002));
#178813=CARTESIAN_POINT('Ctrl Pts',(9.90225811999995,12.2,-4.88598965200001));
#178814=CARTESIAN_POINT('Ctrl Pts',(9.90011098899994,12.2,-4.88370070000002));
#178815=CARTESIAN_POINT('Ctrl Pts',(9.89796557699995,12.2,-4.88141728600001));
#178816=CARTESIAN_POINT('Ctrl Pts',(9.89582189499994,12.2,-4.87913940900001));
#178817=CARTESIAN_POINT('Ctrl Pts',(9.89367995199995,12.2,-4.87686707300002));
#178818=CARTESIAN_POINT('Ctrl Pts',(9.89153976099994,12.2,-4.87460027900001));
#178819=CARTESIAN_POINT('Ctrl Pts',(9.88940133499994,12.2,-4.87233902900002));
#178820=CARTESIAN_POINT('Ctrl Pts',(9.88726468299994,12.2,-4.87008332300002));
#178821=CARTESIAN_POINT('Ctrl Pts',(9.88512981699994,12.2,-4.86783316500001));
#178822=CARTESIAN_POINT('Ctrl Pts',(9.88299674999995,12.2,-4.86558855600002));
#178823=CARTESIAN_POINT('Ctrl Pts',(9.88086549299994,12.2,-4.86334949700002));
#178824=CARTESIAN_POINT('Ctrl Pts',(9.87873605699994,12.2,-4.86111598900001));
#178825=CARTESIAN_POINT('Ctrl Pts',(9.87660845399994,12.2,-4.85888803500002));
#178826=CARTESIAN_POINT('Ctrl Pts',(9.87448269599994,12.2,-4.85666563600001));
#178827=CARTESIAN_POINT('Ctrl Pts',(9.87235879499995,12.2,-4.85444879300001));
#178828=CARTESIAN_POINT('Ctrl Pts',(9.87023676299994,12.2,-4.85223750900001));
#178829=CARTESIAN_POINT('Ctrl Pts',(9.86811660899994,12.2,-4.85003178400001));
#178830=CARTESIAN_POINT('Ctrl Pts',(9.86599834899994,12.2,-4.84783162100001));
#178831=CARTESIAN_POINT('Ctrl Pts',(9.86388199199994,12.2,-4.84563702200001));
#178832=CARTESIAN_POINT('Ctrl Pts',(9.86176754899994,12.2,-4.84344798700001));
#178833=CARTESIAN_POINT('Ctrl Pts',(9.85965503599994,12.2,-4.84126451800002));
#178834=CARTESIAN_POINT('Ctrl Pts',(9.85754445999994,12.2,-4.83908661700001));
#178835=CARTESIAN_POINT('Ctrl Pts',(9.85543583699994,12.2,-4.83691428600002));
#178836=CARTESIAN_POINT('Ctrl Pts',(9.85332917699995,12.2,-4.83474752600001));
#178837=CARTESIAN_POINT('Ctrl Pts',(9.85122449199994,12.2,-4.83258633800002));
#178838=CARTESIAN_POINT('Ctrl Pts',(9.84912179299995,12.2,-4.83043072400001));
#178839=CARTESIAN_POINT('Ctrl Pts',(9.84702109499995,12.2,-4.82828068500002));
#178840=CARTESIAN_POINT('Ctrl Pts',(9.84492240799995,12.2,-4.82613622400001));
#178841=CARTESIAN_POINT('Ctrl Pts',(9.84282574499994,12.2,-4.82399734200001));
#178842=CARTESIAN_POINT('Ctrl Pts',(9.84073111699994,12.2,-4.82186404000001));
#178843=CARTESIAN_POINT('Ctrl Pts',(9.83863853799994,12.2,-4.81973632000001));
#178844=CARTESIAN_POINT('Ctrl Pts',(9.83654801799995,12.2,-4.81761418300001));
#178845=CARTESIAN_POINT('Ctrl Pts',(9.83445956999994,12.2,-4.81549763000002));
#178846=CARTESIAN_POINT('Ctrl Pts',(9.83237320799994,12.2,-4.81338666500001));
#178847=CARTESIAN_POINT('Ctrl Pts',(9.83028894099995,12.2,-4.81128128700002));
#178848=CARTESIAN_POINT('Ctrl Pts',(9.82820678499994,12.2,-4.80918149800001));
#178849=CARTESIAN_POINT('Ctrl Pts',(9.82612674899995,12.2,-4.80708730000002));
#178850=CARTESIAN_POINT('Ctrl Pts',(9.82404884799994,12.2,-4.80499869500001));
#178851=CARTESIAN_POINT('Ctrl Pts',(9.82197309199995,12.2,-4.80291568300002));
#178852=CARTESIAN_POINT('Ctrl Pts',(9.81989949599994,12.2,-4.80083826600001));
#178853=CARTESIAN_POINT('Ctrl Pts',(9.81782806999994,12.2,-4.79876644700001));
#178854=CARTESIAN_POINT('Ctrl Pts',(9.81575882799994,12.2,-4.79670022500001));
#178855=CARTESIAN_POINT('Ctrl Pts',(9.81369178299994,12.2,-4.79463960300002));
#178856=CARTESIAN_POINT('Ctrl Pts',(9.81162694599995,12.2,-4.79258458200002));
#178857=CARTESIAN_POINT('Ctrl Pts',(9.80956432999994,12.2,-4.79053516400001));
#178858=CARTESIAN_POINT('Ctrl Pts',(9.80750394899994,12.2,-4.78849134900001));
#178859=CARTESIAN_POINT('Ctrl Pts',(9.80544581399995,12.2,-4.78645314000001));
#178860=CARTESIAN_POINT('Ctrl Pts',(9.80338993799995,12.2,-4.78442053800002));
#178861=CARTESIAN_POINT('Ctrl Pts',(9.80133633399995,12.2,-4.78239354400001));
#178862=CARTESIAN_POINT('Ctrl Pts',(9.79928501499994,12.2,-4.78037216000001));
#178863=CARTESIAN_POINT('Ctrl Pts',(9.79723599299994,12.2,-4.77835638700002));
#178864=CARTESIAN_POINT('Ctrl Pts',(9.79518928099995,12.2,-4.77634622600001));
#178865=CARTESIAN_POINT('Ctrl Pts',(9.79314489299994,12.2,-4.77434167900002));
#178866=CARTESIAN_POINT('Ctrl Pts',(9.79110284099994,12.2,-4.77234274600002));
#178867=CARTESIAN_POINT('Ctrl Pts',(9.78906313699994,12.2,-4.77034943200001));
#178868=CARTESIAN_POINT('Ctrl Pts',(9.78702579499994,12.2,-4.76836173400002));
#178869=CARTESIAN_POINT('Ctrl Pts',(9.78499082799994,12.2,-4.76637965700001));
#178870=CARTESIAN_POINT('Ctrl Pts',(9.78295824899994,12.2,-4.76440319900002));
#178871=CARTESIAN_POINT('Ctrl Pts',(9.78092806999994,12.2,-4.76243236400002));
#178872=CARTESIAN_POINT('Ctrl Pts',(9.77890030599994,12.2,-4.76046715200001));
#178873=CARTESIAN_POINT('Ctrl Pts',(9.77687496799994,12.2,-4.75850756500002));
#178874=CARTESIAN_POINT('Ctrl Pts',(9.77485206899994,12.2,-4.75655360400001));
#178875=CARTESIAN_POINT('Ctrl Pts',(9.77283162499995,12.2,-4.75460527100001));
#178876=CARTESIAN_POINT('Ctrl Pts',(9.77081364699995,12.2,-4.75266256500001));
#178877=CARTESIAN_POINT('Ctrl Pts',(9.76879814799995,12.2,-4.75072549100001));
#178878=CARTESIAN_POINT('Ctrl Pts',(9.76678514199994,12.2,-4.74879404700001));
#178879=CARTESIAN_POINT('Ctrl Pts',(9.76477464199995,12.2,-4.74686823700001));
#178880=CARTESIAN_POINT('Ctrl Pts',(9.76276666199994,12.2,-4.74494806000001));
#178881=CARTESIAN_POINT('Ctrl Pts',(9.76076121399995,12.2,-4.74303351800001));
#178882=CARTESIAN_POINT('Ctrl Pts',(9.75875831199994,12.2,-4.74112461300002));
#178883=CARTESIAN_POINT('Ctrl Pts',(9.75675797099995,12.2,-4.73922134600001));
#178884=CARTESIAN_POINT('Ctrl Pts',(9.75476020099994,12.2,-4.73732371700001));
#178885=CARTESIAN_POINT('Ctrl Pts',(9.75276501899994,12.2,-4.73543173000001));
#178886=CARTESIAN_POINT('Ctrl Pts',(9.75077243699995,12.2,-4.73354538300002));
#178887=CARTESIAN_POINT('Ctrl Pts',(9.74878246899994,12.2,-4.73166467900001));
#178888=CARTESIAN_POINT('Ctrl Pts',(9.74679512899994,12.2,-4.72978962000001));
#178889=CARTESIAN_POINT('Ctrl Pts',(9.74481042799994,12.2,-4.72792020600002));
#178890=CARTESIAN_POINT('Ctrl Pts',(9.74282838199995,12.2,-4.72605643900001));
#178891=CARTESIAN_POINT('Ctrl Pts',(9.74084900499994,12.2,-4.72419831800002));
#178892=CARTESIAN_POINT('Ctrl Pts',(9.73887230999994,12.2,-4.72234584700002));
#178893=CARTESIAN_POINT('Ctrl Pts',(9.73689830999995,12.2,-4.72049902600002));
#178894=CARTESIAN_POINT('Ctrl Pts',(9.73492701999995,12.2,-4.71865785700002));
#178895=CARTESIAN_POINT('Ctrl Pts',(9.73295845299995,12.2,-4.71682234000002));
#178896=CARTESIAN_POINT('Ctrl Pts',(9.73099262399994,12.2,-4.71499247700002));
#178897=CARTESIAN_POINT('Ctrl Pts',(9.72902954599994,12.2,-4.71316826800001));
#178898=CARTESIAN_POINT('Ctrl Pts',(9.72706923299994,12.2,-4.71134971600002));
#178899=CARTESIAN_POINT('Ctrl Pts',(9.72511169899994,12.2,-4.70953682000002));
#178900=CARTESIAN_POINT('Ctrl Pts',(9.72315695899994,12.2,-4.70772958400001));
#178901=CARTESIAN_POINT('Ctrl Pts',(9.72120502599994,12.2,-4.70592800700001));
#178902=CARTESIAN_POINT('Ctrl Pts',(9.71925591399994,12.2,-4.70413209100002));
#178903=CARTESIAN_POINT('Ctrl Pts',(9.71730963799994,12.2,-4.70234183600001));
#178904=CARTESIAN_POINT('Ctrl Pts',(9.71536621099995,12.2,-4.70055724400002));
#178905=CARTESIAN_POINT('Ctrl Pts',(9.71342564799994,12.2,-4.69877831600002));
#178906=CARTESIAN_POINT('Ctrl Pts',(9.71148796399994,12.2,-4.69700505400001));
#178907=CARTESIAN_POINT('Ctrl Pts',(9.70955317199994,12.2,-4.69523745800001));
#178908=CARTESIAN_POINT('Ctrl Pts',(9.70762128699995,12.2,-4.69347552800001));
#178909=CARTESIAN_POINT('Ctrl Pts',(9.70569232299994,12.2,-4.69171926800001));
#178910=CARTESIAN_POINT('Ctrl Pts',(9.70376629399994,12.2,-4.68996867700001));
#178911=CARTESIAN_POINT('Ctrl Pts',(9.70184321499995,12.2,-4.68822375800002));
#178912=CARTESIAN_POINT('Ctrl Pts',(9.69992310199994,12.2,-4.68648450800002));
#178913=CARTESIAN_POINT('Ctrl Pts',(9.69800596699995,12.2,-4.68475093300002));
#178914=CARTESIAN_POINT('Ctrl Pts',(9.69609182599994,12.2,-4.68302303000002));
#178915=CARTESIAN_POINT('Ctrl Pts',(9.69418069299994,12.2,-4.68130080300002));
#178916=CARTESIAN_POINT('Ctrl Pts',(9.69227258299994,12.2,-4.67958425200001));
#178917=CARTESIAN_POINT('Ctrl Pts',(9.69036750899994,12.2,-4.67787337800001));
#178918=CARTESIAN_POINT('Ctrl Pts',(9.68846548899995,12.2,-4.67616818100002));
#178919=CARTESIAN_POINT('Ctrl Pts',(9.68656653499995,12.2,-4.67446866300001));
#178920=CARTESIAN_POINT('Ctrl Pts',(9.68467066399995,12.2,-4.67277482500001));
#178921=CARTESIAN_POINT('Ctrl Pts',(9.68277788899995,12.2,-4.67108666800002));
#178922=CARTESIAN_POINT('Ctrl Pts',(9.68088822599995,12.2,-4.66940419300002));
#178923=CARTESIAN_POINT('Ctrl Pts',(9.67900168899994,12.2,-4.66772740200001));
#178924=CARTESIAN_POINT('Ctrl Pts',(9.67711829399994,12.2,-4.66605629400001));
#178925=CARTESIAN_POINT('Ctrl Pts',(9.67523805399994,12.2,-4.66439087100001));
#178926=CARTESIAN_POINT('Ctrl Pts',(9.67336098799995,12.2,-4.66273113300002));
#178927=CARTESIAN_POINT('Ctrl Pts',(9.67148710599995,12.2,-4.66107708200001));
#178928=CARTESIAN_POINT('Ctrl Pts',(9.66961642799994,12.2,-4.65942871900001));
#178929=CARTESIAN_POINT('Ctrl Pts',(9.66774896599994,12.2,-4.65778604500001));
#178930=CARTESIAN_POINT('Ctrl Pts',(9.66588473599994,12.2,-4.65614906000001));
#178931=CARTESIAN_POINT('Ctrl Pts',(9.66402375299995,12.2,-4.65451776500001));
#178932=CARTESIAN_POINT('Ctrl Pts',(9.66216603399995,12.2,-4.65289216300001));
#178933=CARTESIAN_POINT('Ctrl Pts',(9.66031159299994,12.2,-4.65127225200002));
#178934=CARTESIAN_POINT('Ctrl Pts',(9.65846044499994,12.2,-4.64965803400001));
#178935=CARTESIAN_POINT('Ctrl Pts',(9.65661260499994,12.2,-4.64804951100001));
#178936=CARTESIAN_POINT('Ctrl Pts',(9.65476809099994,12.2,-4.64644668200001));
#178937=CARTESIAN_POINT('Ctrl Pts',(9.65292691699995,12.2,-4.64484954900001));
#178938=CARTESIAN_POINT('Ctrl Pts',(9.65108909699994,12.2,-4.64325811300002));
#178939=CARTESIAN_POINT('Ctrl Pts',(9.64925464999994,12.2,-4.64167237400002));
#178940=CARTESIAN_POINT('Ctrl Pts',(9.64742358899995,12.2,-4.64009233400001));
#178941=CARTESIAN_POINT('Ctrl Pts',(9.64559592999995,12.2,-4.63851799300001));
#178942=CARTESIAN_POINT('Ctrl Pts',(9.64377168999994,12.2,-4.63694935100001));
#178943=CARTESIAN_POINT('Ctrl Pts',(9.64195088399994,12.2,-4.63538641000001));
#178944=CARTESIAN_POINT('Ctrl Pts',(9.64013352699994,12.2,-4.63382917200001));
#178945=CARTESIAN_POINT('Ctrl Pts',(9.63831963699995,12.2,-4.63227763600001));
#178946=CARTESIAN_POINT('Ctrl Pts',(9.63650922799994,12.2,-4.63073180200002));
#178947=CARTESIAN_POINT('Ctrl Pts',(9.63470231799995,12.2,-4.62919167300001));
#178948=CARTESIAN_POINT('Ctrl Pts',(9.63289892099995,12.2,-4.62765724900001));
#178949=CARTESIAN_POINT('Ctrl Pts',(9.63109905299994,12.2,-4.62612853000001));
#178950=CARTESIAN_POINT('Ctrl Pts',(9.62930273199994,12.2,-4.62460551700001));
#178951=CARTESIAN_POINT('Ctrl Pts',(9.62750997299995,12.2,-4.62308821200001));
#178952=CARTESIAN_POINT('Ctrl Pts',(9.62572079199994,12.2,-4.62157661300001));
#178953=CARTESIAN_POINT('Ctrl Pts',(9.62393520599995,12.2,-4.62007072400001));
#178954=CARTESIAN_POINT('Ctrl Pts',(9.62215323099995,12.2,-4.61857054400001));
#178955=CARTESIAN_POINT('Ctrl Pts',(9.62037488299995,12.2,-4.61707607400001));
#178956=CARTESIAN_POINT('Ctrl Pts',(9.61860017899994,12.2,-4.61558731400002));
#178957=CARTESIAN_POINT('Ctrl Pts',(9.61682913599994,12.2,-4.61410426600001));
#178958=CARTESIAN_POINT('Ctrl Pts',(9.61506176799995,12.2,-4.61262692900001));
#178959=CARTESIAN_POINT('Ctrl Pts',(9.61329809399994,12.2,-4.61115530500001));
#178960=CARTESIAN_POINT('Ctrl Pts',(9.61153812999994,12.2,-4.60968939500002));
#178961=CARTESIAN_POINT('Ctrl Pts',(9.60978189399994,12.2,-4.60822919900002));
#178962=CARTESIAN_POINT('Ctrl Pts',(9.60802939899994,12.2,-4.60677471700001));
#178963=CARTESIAN_POINT('Ctrl Pts',(9.60628066499994,12.2,-4.60532595000001));
#178964=CARTESIAN_POINT('Ctrl Pts',(9.60453570799995,12.2,-4.60388290000001));
#178965=CARTESIAN_POINT('Ctrl Pts',(9.60279454499995,12.2,-4.60244556600002));
#178966=CARTESIAN_POINT('Ctrl Pts',(9.60105719199994,12.2,-4.60101394900001));
#178967=CARTESIAN_POINT('Ctrl Pts',(9.59932366799995,12.2,-4.59958805000001));
#178968=CARTESIAN_POINT('Ctrl Pts',(9.59759398799994,12.2,-4.59816786900001));
#178969=CARTESIAN_POINT('Ctrl Pts',(9.59586816799994,12.2,-4.59675340600001));
#178970=CARTESIAN_POINT('Ctrl Pts',(9.59414622799994,12.2,-4.59534466400001));
#178971=CARTESIAN_POINT('Ctrl Pts',(9.59242818399994,12.2,-4.59394164100001));
#178972=CARTESIAN_POINT('Ctrl Pts',(9.59071405399994,12.2,-4.59254433900002));
#178973=CARTESIAN_POINT('Ctrl Pts',(9.58900385399994,12.2,-4.59115275800002));
#178974=CARTESIAN_POINT('Ctrl Pts',(9.58729760199994,12.2,-4.58976689800001));
#178975=CARTESIAN_POINT('Ctrl Pts',(9.58559531499995,12.2,-4.58838676100001));
#178976=CARTESIAN_POINT('Ctrl Pts',(9.58389701199994,12.2,-4.58701234700001));
#178977=CARTESIAN_POINT('Ctrl Pts',(9.58220270699995,12.2,-4.58564365500001));
#178978=CARTESIAN_POINT('Ctrl Pts',(9.58051242199994,12.2,-4.58428068800002));
#178979=CARTESIAN_POINT('Ctrl Pts',(9.57882617099994,12.2,-4.58292344400002));
#178980=CARTESIAN_POINT('Ctrl Pts',(9.57714397399995,12.2,-4.58157192400002));
#178981=CARTESIAN_POINT('Ctrl Pts',(9.57546584599994,12.2,-4.58022613000002));
#178982=CARTESIAN_POINT('Ctrl Pts',(9.57379180899995,12.2,-4.57888606200001));
#178983=CARTESIAN_POINT('Ctrl Pts',(9.57212187699995,12.2,-4.57755172000001));
#178984=CARTESIAN_POINT('Ctrl Pts',(9.57045606999994,12.2,-4.57622310400001));
#178985=CARTESIAN_POINT('Ctrl Pts',(9.56879440599995,12.2,-4.57490021400002));
#178986=CARTESIAN_POINT('Ctrl Pts',(9.56713690099994,12.2,-4.57358305200001));
#178987=CARTESIAN_POINT('Ctrl Pts',(9.56548357399994,12.2,-4.57227161800001));
#178988=CARTESIAN_POINT('Ctrl Pts',(9.56383444399994,12.2,-4.57096591100001));
#178989=CARTESIAN_POINT('Ctrl Pts',(9.56218952899994,12.2,-4.56966593300002));
#178990=CARTESIAN_POINT('Ctrl Pts',(9.56054884799994,12.2,-4.56837168300002));
#178991=CARTESIAN_POINT('Ctrl Pts',(9.55891241699995,12.2,-4.56708316300002));
#178992=CARTESIAN_POINT('Ctrl Pts',(9.55728025499995,12.2,-4.56580037200002));
#178993=CARTESIAN_POINT('Ctrl Pts',(9.55565238299994,12.2,-4.56452331000001));
#178994=CARTESIAN_POINT('Ctrl Pts',(9.55402881599994,12.2,-4.56325197900001));
#178995=CARTESIAN_POINT('Ctrl Pts',(9.55240957399995,12.2,-4.56198637800002));
#178996=CARTESIAN_POINT('Ctrl Pts',(9.55079467599995,12.2,-4.56072650800001));
#178997=CARTESIAN_POINT('Ctrl Pts',(9.54918413999994,12.2,-4.55947236900001));
#178998=CARTESIAN_POINT('Ctrl Pts',(9.54757798599994,12.2,-4.55822396200002));
#178999=CARTESIAN_POINT('Ctrl Pts',(9.54597623199994,12.2,-4.55698128600002));
#179000=CARTESIAN_POINT('Ctrl Pts',(9.54437889599994,12.2,-4.55574434100001));
#179001=CARTESIAN_POINT('Ctrl Pts',(9.54278599799995,12.2,-4.55451312900002));
#179002=CARTESIAN_POINT('Ctrl Pts',(9.54119755599995,12.2,-4.55328764900001));
#179003=CARTESIAN_POINT('Ctrl Pts',(9.53961358999995,12.2,-4.55206790100001));
#179004=CARTESIAN_POINT('Ctrl Pts',(9.53803411899995,12.2,-4.55085388600001));
#179005=CARTESIAN_POINT('Ctrl Pts',(9.53645916199994,12.2,-4.54964560500001));
#179006=CARTESIAN_POINT('Ctrl Pts',(9.53488873799994,12.2,-4.54844305600002));
#179007=CARTESIAN_POINT('Ctrl Pts',(9.53332286699995,12.2,-4.54724624000002));
#179008=CARTESIAN_POINT('Ctrl Pts',(9.53176156699995,12.2,-4.54605515800001));
#179009=CARTESIAN_POINT('Ctrl Pts',(9.53020485899994,12.2,-4.54486981000001));
#179010=CARTESIAN_POINT('Ctrl Pts',(9.52865276099994,12.2,-4.54369019500001));
#179011=CARTESIAN_POINT('Ctrl Pts',(9.52710529499995,12.2,-4.54251631400002));
#179012=CARTESIAN_POINT('Ctrl Pts',(9.52556247699994,12.2,-4.54134816700002));
#179013=CARTESIAN_POINT('Ctrl Pts',(9.52402432899994,12.2,-4.54018575400001));
#179014=CARTESIAN_POINT('Ctrl Pts',(9.52249087199995,12.2,-4.53902907500002));
#179015=CARTESIAN_POINT('Ctrl Pts',(9.52096212299995,12.2,-4.53787813200002));
#179016=CARTESIAN_POINT('Ctrl Pts',(9.51943810399994,12.2,-4.53673292200001));
#179017=CARTESIAN_POINT('Ctrl Pts',(9.51791883399994,12.2,-4.53559344600002));
#179018=CARTESIAN_POINT('Ctrl Pts',(9.51640433299995,12.2,-4.53445970600002));
#179019=CARTESIAN_POINT('Ctrl Pts',(9.51489462199994,12.2,-4.53333169900001));
#179020=CARTESIAN_POINT('Ctrl Pts',(9.51338971899995,12.2,-4.53220942700002));
#179021=CARTESIAN_POINT('Ctrl Pts',(9.51188964699995,12.2,-4.53109288900002));
#179022=CARTESIAN_POINT('Ctrl Pts',(9.51039442599994,12.2,-4.52998208700001));
#179023=CARTESIAN_POINT('Ctrl Pts',(9.50890407399994,12.2,-4.52887701800002));
#179024=CARTESIAN_POINT('Ctrl Pts',(9.50741861299995,12.2,-4.52777768500002));
#179025=CARTESIAN_POINT('Ctrl Pts',(9.50593806399995,12.2,-4.52668408600001));
#179026=CARTESIAN_POINT('Ctrl Pts',(9.50446244799994,12.2,-4.52559622000001));
#179027=CARTESIAN_POINT('Ctrl Pts',(9.50299178499994,12.2,-4.52451409000002));
#179028=CARTESIAN_POINT('Ctrl Pts',(9.50152609399994,12.2,-4.52343769300001));
#179029=CARTESIAN_POINT('Ctrl Pts',(9.50006539899995,12.2,-4.52236703200001));
#179030=CARTESIAN_POINT('Ctrl Pts',(9.49860971899994,12.2,-4.52130210400002));
#179031=CARTESIAN_POINT('Ctrl Pts',(9.49715907499994,12.2,-4.52024291000001));
#179032=CARTESIAN_POINT('Ctrl Pts',(9.49571348799994,12.2,-4.51918944900001));
#179033=CARTESIAN_POINT('Ctrl Pts',(9.49427298099994,12.2,-4.51814172300002));
#179034=CARTESIAN_POINT('Ctrl Pts',(9.49283757399994,12.2,-4.51709973000002));
#179035=CARTESIAN_POINT('Ctrl Pts',(9.49140728699994,12.2,-4.51606347000002));
#179036=CARTESIAN_POINT('Ctrl Pts',(9.48998214199994,12.2,-4.51503294400001));
#179037=CARTESIAN_POINT('Ctrl Pts',(9.48856216199994,12.2,-4.51400815100001));
#179038=CARTESIAN_POINT('Ctrl Pts',(9.48714736699995,12.2,-4.51298909100001));
#179039=CARTESIAN_POINT('Ctrl Pts',(9.48573777999994,12.2,-4.51197576300002));
#179040=CARTESIAN_POINT('Ctrl Pts',(9.48433342199994,12.2,-4.51096816700002));
#179041=CARTESIAN_POINT('Ctrl Pts',(9.48293431399994,12.2,-4.50996630300001));
#179042=CARTESIAN_POINT('Ctrl Pts',(9.48154047899994,12.2,-4.50897017200001));
#179043=CARTESIAN_POINT('Ctrl Pts',(9.48015193699994,12.2,-4.50797977200001));
#179044=CARTESIAN_POINT('Ctrl Pts',(9.47876871299994,12.2,-4.50699510200002));
#179045=CARTESIAN_POINT('Ctrl Pts',(9.47739082699995,12.2,-4.50601616500002));
#179046=CARTESIAN_POINT('Ctrl Pts',(9.47601830199994,12.2,-4.50504295800001));
#179047=CARTESIAN_POINT('Ctrl Pts',(9.47465115999995,12.2,-4.50407548100001));
#179048=CARTESIAN_POINT('Ctrl Pts',(9.47328942199994,12.2,-4.50311373400002));
#179049=CARTESIAN_POINT('Ctrl Pts',(9.47193311299994,12.2,-4.50215771600002));
#179050=CARTESIAN_POINT('Ctrl Pts',(9.47058225499994,12.2,-4.50120742900001));
#179051=CARTESIAN_POINT('Ctrl Pts',(9.46923686899994,12.2,-4.50026286900002));
#179052=CARTESIAN_POINT('Ctrl Pts',(9.46789697899994,12.2,-4.49932403800001));
#179053=CARTESIAN_POINT('Ctrl Pts',(9.46656260799994,12.2,-4.49839093600001));
#179054=CARTESIAN_POINT('Ctrl Pts',(9.46523377699994,12.2,-4.49746356000002));
#179055=CARTESIAN_POINT('Ctrl Pts',(9.46391051099994,12.2,-4.49654191200001));
#179056=CARTESIAN_POINT('Ctrl Pts',(9.46259283199995,12.2,-4.49562599100001));
#179057=CARTESIAN_POINT('Ctrl Pts',(9.46128076299994,12.2,-4.49471579600001));
#179058=CARTESIAN_POINT('Ctrl Pts',(9.45997432899994,12.2,-4.49381132600001));
#179059=CARTESIAN_POINT('Ctrl Pts',(9.45867355199994,12.2,-4.49291258200001));
#179060=CARTESIAN_POINT('Ctrl Pts',(9.45737845499995,12.2,-4.49201956300001));
#179061=CARTESIAN_POINT('Ctrl Pts',(9.45608906199995,12.2,-4.49113226700002));
#179062=CARTESIAN_POINT('Ctrl Pts',(9.45480539699994,12.2,-4.49025069500002));
#179063=CARTESIAN_POINT('Ctrl Pts',(9.45352748199995,12.2,-4.48937484700001));
#179064=CARTESIAN_POINT('Ctrl Pts',(9.45225534299994,12.2,-4.48850472100002));
#179065=CARTESIAN_POINT('Ctrl Pts',(9.45098900299995,12.2,-4.48764031700001));
#179066=CARTESIAN_POINT('Ctrl Pts',(9.44972848499994,12.2,-4.48678163300002));
#179067=CARTESIAN_POINT('Ctrl Pts',(9.44847381499994,12.2,-4.48592867100002));
#179068=CARTESIAN_POINT('Ctrl Pts',(9.44722501599994,12.2,-4.48508142800002));
#179069=CARTESIAN_POINT('Ctrl Pts',(9.44598211199994,12.2,-4.48423990500002));
#179070=CARTESIAN_POINT('Ctrl Pts',(9.44474512899994,12.2,-4.48340410000001));
#179071=CARTESIAN_POINT('Ctrl Pts',(9.44351408899994,12.2,-4.48257401400001));
#179072=CARTESIAN_POINT('Ctrl Pts',(9.44228901899995,12.2,-4.48174964400001));
#179073=CARTESIAN_POINT('Ctrl Pts',(9.44106994199995,12.2,-4.48093099100001));
#179074=CARTESIAN_POINT('Ctrl Pts',(9.43985688299994,12.2,-4.48011805400002));
#179075=CARTESIAN_POINT('Ctrl Pts',(9.43864986699994,12.2,-4.47931083200002));
#179076=CARTESIAN_POINT('Ctrl Pts',(9.43744891899994,12.2,-4.47850932400002));
#179077=CARTESIAN_POINT('Ctrl Pts',(9.43625406499994,12.2,-4.47771352900002));
#179078=CARTESIAN_POINT('Ctrl Pts',(9.43506532899995,12.2,-4.47692344800001));
#179079=CARTESIAN_POINT('Ctrl Pts',(9.43388273599994,12.2,-4.47613907800001));
#179080=CARTESIAN_POINT('Ctrl Pts',(9.43270631299994,12.2,-4.47536041800001));
#179081=CARTESIAN_POINT('Ctrl Pts',(9.43153608499994,12.2,-4.47458746900002));
#179082=CARTESIAN_POINT('Ctrl Pts',(9.43037207599994,12.2,-4.47382023000001));
#179083=CARTESIAN_POINT('Ctrl Pts',(9.42921431399995,12.2,-4.47305869800001));
#179084=CARTESIAN_POINT('Ctrl Pts',(9.42806282299994,12.2,-4.47230287400001));
#179085=CARTESIAN_POINT('Ctrl Pts',(9.42691762999995,12.2,-4.47155275600001));
#179086=CARTESIAN_POINT('Ctrl Pts',(9.42577875999994,12.2,-4.47080834400001));
#179087=CARTESIAN_POINT('Ctrl Pts',(9.42464624099994,12.2,-4.47006963700002));
#179088=CARTESIAN_POINT('Ctrl Pts',(9.42352009699994,12.2,-4.46933663400001));
#179089=CARTESIAN_POINT('Ctrl Pts',(9.42240035499994,12.2,-4.46860933200002));
#179090=CARTESIAN_POINT('Ctrl Pts',(9.42128704299994,12.2,-4.46788773300002));
#179091=CARTESIAN_POINT('Ctrl Pts',(9.42018018699994,12.2,-4.46717183400001));
#179092=CARTESIAN_POINT('Ctrl Pts',(9.41907981199994,12.2,-4.46646163500001));
#179093=CARTESIAN_POINT('Ctrl Pts',(9.41798594799995,12.2,-4.46575713300001));
#179094=CARTESIAN_POINT('Ctrl Pts',(9.41689861899994,12.2,-4.46505832900002));
#179095=CARTESIAN_POINT('Ctrl Pts',(9.41581785299995,12.2,-4.46436522100001));
#179096=CARTESIAN_POINT('Ctrl Pts',(9.41474367699995,12.2,-4.46367780900002));
#179097=CARTESIAN_POINT('Ctrl Pts',(9.41367611899994,12.2,-4.46299609100001));
#179098=CARTESIAN_POINT('Ctrl Pts',(9.41261520599994,12.2,-4.46232006500002));
#179099=CARTESIAN_POINT('Ctrl Pts',(9.41156096599994,12.2,-4.46164973100001));
#179100=CARTESIAN_POINT('Ctrl Pts',(9.41051342599994,12.2,-4.46098508800001));
#179101=CARTESIAN_POINT('Ctrl Pts',(9.40947261499995,12.2,-4.46032613400002));
#179102=CARTESIAN_POINT('Ctrl Pts',(9.40843855899995,12.2,-4.45967286700002));
#179103=CARTESIAN_POINT('Ctrl Pts',(9.40741128799995,12.2,-4.45902528700001));
#179104=CARTESIAN_POINT('Ctrl Pts',(9.40639082799994,12.2,-4.45838339300002));
#179105=CARTESIAN_POINT('Ctrl Pts',(9.40537720899994,12.2,-4.45774718300001));
#179106=CARTESIAN_POINT('Ctrl Pts',(9.40437045999994,12.2,-4.45711665500002));
#179107=CARTESIAN_POINT('Ctrl Pts',(9.40337060799994,12.2,-4.45649181000002));
#179108=CARTESIAN_POINT('Ctrl Pts',(9.40237768099994,12.2,-4.45587264400002));
#179109=CARTESIAN_POINT('Ctrl Pts',(9.40139171099995,12.2,-4.45525915600001));
#179110=CARTESIAN_POINT('Ctrl Pts',(9.40041272399995,12.2,-4.45465134700001));
#179111=CARTESIAN_POINT('Ctrl Pts',(9.39944075099995,12.2,-4.45404921300002));
#179112=CARTESIAN_POINT('Ctrl Pts',(9.39847581899994,12.2,-4.45345275400001));
#179113=CARTESIAN_POINT('Ctrl Pts',(9.39751795899994,12.2,-4.45286196700001));
#179114=CARTESIAN_POINT('Ctrl Pts',(9.39656720199994,12.2,-4.45227685300001));
#179115=CARTESIAN_POINT('Ctrl Pts',(9.39562357399994,12.2,-4.45169740800001));
#179116=CARTESIAN_POINT('Ctrl Pts',(9.39468710699994,12.2,-4.45112363100002));
#179117=CARTESIAN_POINT('Ctrl Pts',(9.39375783099995,12.2,-4.45055552200001));
#179118=CARTESIAN_POINT('Ctrl Pts',(9.39283577499994,12.2,-4.44999307800002));
#179119=CARTESIAN_POINT('Ctrl Pts',(9.39192097099994,12.2,-4.44943629800001));
#179120=CARTESIAN_POINT('Ctrl Pts',(9.39101344699995,12.2,-4.44888518000001));
#179121=CARTESIAN_POINT('Ctrl Pts',(9.39011323499994,12.2,-4.44833972300001));
#179122=CARTESIAN_POINT('Ctrl Pts',(9.38922036599994,12.2,-4.44779992400001));
#179123=CARTESIAN_POINT('Ctrl Pts',(9.38833486899994,12.2,-4.44726578300001));
#179124=CARTESIAN_POINT('Ctrl Pts',(9.38745677599995,12.2,-4.44673729700002));
#179125=CARTESIAN_POINT('Ctrl Pts',(9.38658611799994,12.2,-4.44621446500001));
#179126=CARTESIAN_POINT('Ctrl Pts',(9.38572292599994,12.2,-4.44569728500001));
#179127=CARTESIAN_POINT('Ctrl Pts',(9.38486723299994,12.2,-4.44518575500001));
#179128=CARTESIAN_POINT('Ctrl Pts',(9.38401906799994,12.2,-4.44467987500001));
#179129=CARTESIAN_POINT('Ctrl Pts',(9.38317846499995,12.2,-4.44417964100001));
#179130=CARTESIAN_POINT('Ctrl Pts',(9.38234545299995,12.2,-4.44368505100002));
#179131=CARTESIAN_POINT('Ctrl Pts',(9.38152006799994,12.2,-4.44319610500001));
#179132=CARTESIAN_POINT('Ctrl Pts',(9.38070233899994,12.2,-4.44271280000001));
#179133=CARTESIAN_POINT('Ctrl Pts',(9.37989229799994,12.2,-4.44223513400001));
#179134=CARTESIAN_POINT('Ctrl Pts',(9.37908997999994,12.2,-4.44176310500001));
#179135=CARTESIAN_POINT('Ctrl Pts',(9.37829999299994,12.2,-4.44129939800002));
#179136=CARTESIAN_POINT('Ctrl Pts',(9.37767505699994,12.2,-4.44093341100002));
#179137=CARTESIAN_POINT('Ctrl Pts',(9.37721094099994,12.2,-4.44066207000001));
#179138=CARTESIAN_POINT('Ctrl Pts',(9.37690455199995,12.2,-4.44048314700002));
#179139=CARTESIAN_POINT('Ctrl Pts',(9.37675396699994,12.2,-4.44039525800001));
#179140=CARTESIAN_POINT('Ctrl Pts',(9.37675396699994,15.2,-4.44039525800001));
#179141=CARTESIAN_POINT('Ctrl Pts',(9.37690455199995,15.2,-4.44048314700002));
#179142=CARTESIAN_POINT('Ctrl Pts',(9.37721094099994,15.2,-4.44066207000001));
#179143=CARTESIAN_POINT('Ctrl Pts',(9.37767505699994,15.2,-4.44093341100002));
#179144=CARTESIAN_POINT('Ctrl Pts',(9.37829999299994,15.2,-4.44129939800002));
#179145=CARTESIAN_POINT('Ctrl Pts',(9.37908997999994,15.2,-4.44176310500001));
#179146=CARTESIAN_POINT('Ctrl Pts',(9.37989229799994,15.2,-4.44223513400001));
#179147=CARTESIAN_POINT('Ctrl Pts',(9.38070233899994,15.2,-4.44271280000001));
#179148=CARTESIAN_POINT('Ctrl Pts',(9.38152006799994,15.2,-4.44319610500001));
#179149=CARTESIAN_POINT('Ctrl Pts',(9.38234545299995,15.2,-4.44368505100002));
#179150=CARTESIAN_POINT('Ctrl Pts',(9.38317846499995,15.2,-4.44417964100001));
#179151=CARTESIAN_POINT('Ctrl Pts',(9.38401906799994,15.2,-4.44467987500001));
#179152=CARTESIAN_POINT('Ctrl Pts',(9.38486723299994,15.2,-4.44518575500001));
#179153=CARTESIAN_POINT('Ctrl Pts',(9.38572292599994,15.2,-4.44569728500001));
#179154=CARTESIAN_POINT('Ctrl Pts',(9.38658611799994,15.2,-4.44621446500001));
#179155=CARTESIAN_POINT('Ctrl Pts',(9.38745677599995,15.2,-4.44673729700002));
#179156=CARTESIAN_POINT('Ctrl Pts',(9.38833486899994,15.2,-4.44726578300001));
#179157=CARTESIAN_POINT('Ctrl Pts',(9.38922036599994,15.2,-4.44779992400001));
#179158=CARTESIAN_POINT('Ctrl Pts',(9.39011323499994,15.2,-4.44833972300001));
#179159=CARTESIAN_POINT('Ctrl Pts',(9.39101344699995,15.2,-4.44888518000001));
#179160=CARTESIAN_POINT('Ctrl Pts',(9.39192097099994,15.2,-4.44943629800001));
#179161=CARTESIAN_POINT('Ctrl Pts',(9.39283577499994,15.2,-4.44999307800002));
#179162=CARTESIAN_POINT('Ctrl Pts',(9.39375783099995,15.2,-4.45055552200001));
#179163=CARTESIAN_POINT('Ctrl Pts',(9.39468710699994,15.2,-4.45112363100002));
#179164=CARTESIAN_POINT('Ctrl Pts',(9.39562357399994,15.2,-4.45169740800001));
#179165=CARTESIAN_POINT('Ctrl Pts',(9.39656720199994,15.2,-4.45227685300001));
#179166=CARTESIAN_POINT('Ctrl Pts',(9.39751795899994,15.2,-4.45286196700001));
#179167=CARTESIAN_POINT('Ctrl Pts',(9.39847581899994,15.2,-4.45345275400001));
#179168=CARTESIAN_POINT('Ctrl Pts',(9.39944075099995,15.2,-4.45404921300002));
#179169=CARTESIAN_POINT('Ctrl Pts',(9.40041272399995,15.2,-4.45465134700001));
#179170=CARTESIAN_POINT('Ctrl Pts',(9.40139171099995,15.2,-4.45525915600001));
#179171=CARTESIAN_POINT('Ctrl Pts',(9.40237768099994,15.2,-4.45587264400002));
#179172=CARTESIAN_POINT('Ctrl Pts',(9.40337060799994,15.2,-4.45649181000002));
#179173=CARTESIAN_POINT('Ctrl Pts',(9.40437045999994,15.2,-4.45711665500002));
#179174=CARTESIAN_POINT('Ctrl Pts',(9.40537720899994,15.2,-4.45774718300001));
#179175=CARTESIAN_POINT('Ctrl Pts',(9.40639082799994,15.2,-4.45838339300002));
#179176=CARTESIAN_POINT('Ctrl Pts',(9.40741128799995,15.2,-4.45902528700001));
#179177=CARTESIAN_POINT('Ctrl Pts',(9.40843855899995,15.2,-4.45967286700002));
#179178=CARTESIAN_POINT('Ctrl Pts',(9.40947261499995,15.2,-4.46032613400002));
#179179=CARTESIAN_POINT('Ctrl Pts',(9.41051342599994,15.2,-4.46098508800001));
#179180=CARTESIAN_POINT('Ctrl Pts',(9.41156096599994,15.2,-4.46164973100001));
#179181=CARTESIAN_POINT('Ctrl Pts',(9.41261520599994,15.2,-4.46232006500002));
#179182=CARTESIAN_POINT('Ctrl Pts',(9.41367611899994,15.2,-4.46299609100001));
#179183=CARTESIAN_POINT('Ctrl Pts',(9.41474367699995,15.2,-4.46367780900002));
#179184=CARTESIAN_POINT('Ctrl Pts',(9.41581785299995,15.2,-4.46436522100001));
#179185=CARTESIAN_POINT('Ctrl Pts',(9.41689861899994,15.2,-4.46505832900002));
#179186=CARTESIAN_POINT('Ctrl Pts',(9.41798594799995,15.2,-4.46575713300001));
#179187=CARTESIAN_POINT('Ctrl Pts',(9.41907981199994,15.2,-4.46646163500001));
#179188=CARTESIAN_POINT('Ctrl Pts',(9.42018018699994,15.2,-4.46717183400001));
#179189=CARTESIAN_POINT('Ctrl Pts',(9.42128704299994,15.2,-4.46788773300002));
#179190=CARTESIAN_POINT('Ctrl Pts',(9.42240035499994,15.2,-4.46860933200002));
#179191=CARTESIAN_POINT('Ctrl Pts',(9.42352009699994,15.2,-4.46933663400001));
#179192=CARTESIAN_POINT('Ctrl Pts',(9.42464624099994,15.2,-4.47006963700002));
#179193=CARTESIAN_POINT('Ctrl Pts',(9.42577875999994,15.2,-4.47080834400001));
#179194=CARTESIAN_POINT('Ctrl Pts',(9.42691762999995,15.2,-4.47155275600001));
#179195=CARTESIAN_POINT('Ctrl Pts',(9.42806282299994,15.2,-4.47230287400001));
#179196=CARTESIAN_POINT('Ctrl Pts',(9.42921431399995,15.2,-4.47305869800001));
#179197=CARTESIAN_POINT('Ctrl Pts',(9.43037207599994,15.2,-4.47382023000001));
#179198=CARTESIAN_POINT('Ctrl Pts',(9.43153608499994,15.2,-4.47458746900002));
#179199=CARTESIAN_POINT('Ctrl Pts',(9.43270631299994,15.2,-4.47536041800001));
#179200=CARTESIAN_POINT('Ctrl Pts',(9.43388273599994,15.2,-4.47613907800001));
#179201=CARTESIAN_POINT('Ctrl Pts',(9.43506532899995,15.2,-4.47692344800001));
#179202=CARTESIAN_POINT('Ctrl Pts',(9.43625406499994,15.2,-4.47771352900002));
#179203=CARTESIAN_POINT('Ctrl Pts',(9.43744891899994,15.2,-4.47850932400002));
#179204=CARTESIAN_POINT('Ctrl Pts',(9.43864986699994,15.2,-4.47931083200002));
#179205=CARTESIAN_POINT('Ctrl Pts',(9.43985688299994,15.2,-4.48011805400002));
#179206=CARTESIAN_POINT('Ctrl Pts',(9.44106994199995,15.2,-4.48093099100001));
#179207=CARTESIAN_POINT('Ctrl Pts',(9.44228901899995,15.2,-4.48174964400001));
#179208=CARTESIAN_POINT('Ctrl Pts',(9.44351408899994,15.2,-4.48257401400001));
#179209=CARTESIAN_POINT('Ctrl Pts',(9.44474512899994,15.2,-4.48340410000001));
#179210=CARTESIAN_POINT('Ctrl Pts',(9.44598211199994,15.2,-4.48423990500002));
#179211=CARTESIAN_POINT('Ctrl Pts',(9.44722501599994,15.2,-4.48508142800002));
#179212=CARTESIAN_POINT('Ctrl Pts',(9.44847381499994,15.2,-4.48592867100002));
#179213=CARTESIAN_POINT('Ctrl Pts',(9.44972848499994,15.2,-4.48678163300002));
#179214=CARTESIAN_POINT('Ctrl Pts',(9.45098900299995,15.2,-4.48764031700001));
#179215=CARTESIAN_POINT('Ctrl Pts',(9.45225534299994,15.2,-4.48850472100002));
#179216=CARTESIAN_POINT('Ctrl Pts',(9.45352748199995,15.2,-4.48937484700001));
#179217=CARTESIAN_POINT('Ctrl Pts',(9.45480539699994,15.2,-4.49025069500002));
#179218=CARTESIAN_POINT('Ctrl Pts',(9.45608906199995,15.2,-4.49113226700002));
#179219=CARTESIAN_POINT('Ctrl Pts',(9.45737845499995,15.2,-4.49201956300001));
#179220=CARTESIAN_POINT('Ctrl Pts',(9.45867355199994,15.2,-4.49291258200001));
#179221=CARTESIAN_POINT('Ctrl Pts',(9.45997432899994,15.2,-4.49381132600001));
#179222=CARTESIAN_POINT('Ctrl Pts',(9.46128076299994,15.2,-4.49471579600001));
#179223=CARTESIAN_POINT('Ctrl Pts',(9.46259283199995,15.2,-4.49562599100001));
#179224=CARTESIAN_POINT('Ctrl Pts',(9.46391051099994,15.2,-4.49654191200001));
#179225=CARTESIAN_POINT('Ctrl Pts',(9.46523377699994,15.2,-4.49746356000002));
#179226=CARTESIAN_POINT('Ctrl Pts',(9.46656260799994,15.2,-4.49839093600001));
#179227=CARTESIAN_POINT('Ctrl Pts',(9.46789697899994,15.2,-4.49932403800001));
#179228=CARTESIAN_POINT('Ctrl Pts',(9.46923686899994,15.2,-4.50026286900002));
#179229=CARTESIAN_POINT('Ctrl Pts',(9.47058225499994,15.2,-4.50120742900001));
#179230=CARTESIAN_POINT('Ctrl Pts',(9.47193311299994,15.2,-4.50215771600002));
#179231=CARTESIAN_POINT('Ctrl Pts',(9.47328942199994,15.2,-4.50311373400002));
#179232=CARTESIAN_POINT('Ctrl Pts',(9.47465115999995,15.2,-4.50407548100001));
#179233=CARTESIAN_POINT('Ctrl Pts',(9.47601830199994,15.2,-4.50504295800001));
#179234=CARTESIAN_POINT('Ctrl Pts',(9.47739082699995,15.2,-4.50601616500002));
#179235=CARTESIAN_POINT('Ctrl Pts',(9.47876871299994,15.2,-4.50699510200002));
#179236=CARTESIAN_POINT('Ctrl Pts',(9.48015193699994,15.2,-4.50797977200001));
#179237=CARTESIAN_POINT('Ctrl Pts',(9.48154047899994,15.2,-4.50897017200001));
#179238=CARTESIAN_POINT('Ctrl Pts',(9.48293431399994,15.2,-4.50996630300001));
#179239=CARTESIAN_POINT('Ctrl Pts',(9.48433342199994,15.2,-4.51096816700002));
#179240=CARTESIAN_POINT('Ctrl Pts',(9.48573777999994,15.2,-4.51197576300002));
#179241=CARTESIAN_POINT('Ctrl Pts',(9.48714736699995,15.2,-4.51298909100001));
#179242=CARTESIAN_POINT('Ctrl Pts',(9.48856216199994,15.2,-4.51400815100001));
#179243=CARTESIAN_POINT('Ctrl Pts',(9.48998214199994,15.2,-4.51503294400001));
#179244=CARTESIAN_POINT('Ctrl Pts',(9.49140728699994,15.2,-4.51606347000002));
#179245=CARTESIAN_POINT('Ctrl Pts',(9.49283757399994,15.2,-4.51709973000002));
#179246=CARTESIAN_POINT('Ctrl Pts',(9.49427298099994,15.2,-4.51814172300002));
#179247=CARTESIAN_POINT('Ctrl Pts',(9.49571348799994,15.2,-4.51918944900001));
#179248=CARTESIAN_POINT('Ctrl Pts',(9.49715907499994,15.2,-4.52024291000001));
#179249=CARTESIAN_POINT('Ctrl Pts',(9.49860971899994,15.2,-4.52130210400002));
#179250=CARTESIAN_POINT('Ctrl Pts',(9.50006539899995,15.2,-4.52236703200001));
#179251=CARTESIAN_POINT('Ctrl Pts',(9.50152609399994,15.2,-4.52343769300001));
#179252=CARTESIAN_POINT('Ctrl Pts',(9.50299178499994,15.2,-4.52451409000002));
#179253=CARTESIAN_POINT('Ctrl Pts',(9.50446244799994,15.2,-4.52559622000001));
#179254=CARTESIAN_POINT('Ctrl Pts',(9.50593806399995,15.2,-4.52668408600001));
#179255=CARTESIAN_POINT('Ctrl Pts',(9.50741861299995,15.2,-4.52777768500002));
#179256=CARTESIAN_POINT('Ctrl Pts',(9.50890407399994,15.2,-4.52887701800002));
#179257=CARTESIAN_POINT('Ctrl Pts',(9.51039442599994,15.2,-4.52998208700001));
#179258=CARTESIAN_POINT('Ctrl Pts',(9.51188964699995,15.2,-4.53109288900002));
#179259=CARTESIAN_POINT('Ctrl Pts',(9.51338971899995,15.2,-4.53220942700002));
#179260=CARTESIAN_POINT('Ctrl Pts',(9.51489462199994,15.2,-4.53333169900001));
#179261=CARTESIAN_POINT('Ctrl Pts',(9.51640433299995,15.2,-4.53445970600002));
#179262=CARTESIAN_POINT('Ctrl Pts',(9.51791883399994,15.2,-4.53559344600002));
#179263=CARTESIAN_POINT('Ctrl Pts',(9.51943810399994,15.2,-4.53673292200001));
#179264=CARTESIAN_POINT('Ctrl Pts',(9.52096212299995,15.2,-4.53787813200002));
#179265=CARTESIAN_POINT('Ctrl Pts',(9.52249087199995,15.2,-4.53902907500002));
#179266=CARTESIAN_POINT('Ctrl Pts',(9.52402432899994,15.2,-4.54018575400001));
#179267=CARTESIAN_POINT('Ctrl Pts',(9.52556247699994,15.2,-4.54134816700002));
#179268=CARTESIAN_POINT('Ctrl Pts',(9.52710529499995,15.2,-4.54251631400002));
#179269=CARTESIAN_POINT('Ctrl Pts',(9.52865276099994,15.2,-4.54369019500001));
#179270=CARTESIAN_POINT('Ctrl Pts',(9.53020485899994,15.2,-4.54486981000001));
#179271=CARTESIAN_POINT('Ctrl Pts',(9.53176156699995,15.2,-4.54605515800001));
#179272=CARTESIAN_POINT('Ctrl Pts',(9.53332286699995,15.2,-4.54724624000002));
#179273=CARTESIAN_POINT('Ctrl Pts',(9.53488873799994,15.2,-4.54844305600002));
#179274=CARTESIAN_POINT('Ctrl Pts',(9.53645916199994,15.2,-4.54964560500001));
#179275=CARTESIAN_POINT('Ctrl Pts',(9.53803411899995,15.2,-4.55085388600001));
#179276=CARTESIAN_POINT('Ctrl Pts',(9.53961358999995,15.2,-4.55206790100001));
#179277=CARTESIAN_POINT('Ctrl Pts',(9.54119755599995,15.2,-4.55328764900001));
#179278=CARTESIAN_POINT('Ctrl Pts',(9.54278599799995,15.2,-4.55451312900002));
#179279=CARTESIAN_POINT('Ctrl Pts',(9.54437889599994,15.2,-4.55574434100001));
#179280=CARTESIAN_POINT('Ctrl Pts',(9.54597623199994,15.2,-4.55698128600002));
#179281=CARTESIAN_POINT('Ctrl Pts',(9.54757798599994,15.2,-4.55822396200002));
#179282=CARTESIAN_POINT('Ctrl Pts',(9.54918413999994,15.2,-4.55947236900001));
#179283=CARTESIAN_POINT('Ctrl Pts',(9.55079467599995,15.2,-4.56072650800001));
#179284=CARTESIAN_POINT('Ctrl Pts',(9.55240957399995,15.2,-4.56198637800002));
#179285=CARTESIAN_POINT('Ctrl Pts',(9.55402881599994,15.2,-4.56325197900001));
#179286=CARTESIAN_POINT('Ctrl Pts',(9.55565238299994,15.2,-4.56452331000001));
#179287=CARTESIAN_POINT('Ctrl Pts',(9.55728025499995,15.2,-4.56580037200002));
#179288=CARTESIAN_POINT('Ctrl Pts',(9.55891241699995,15.2,-4.56708316300002));
#179289=CARTESIAN_POINT('Ctrl Pts',(9.56054884799994,15.2,-4.56837168300002));
#179290=CARTESIAN_POINT('Ctrl Pts',(9.56218952899994,15.2,-4.56966593300002));
#179291=CARTESIAN_POINT('Ctrl Pts',(9.56383444399994,15.2,-4.57096591100001));
#179292=CARTESIAN_POINT('Ctrl Pts',(9.56548357399994,15.2,-4.57227161800001));
#179293=CARTESIAN_POINT('Ctrl Pts',(9.56713690099994,15.2,-4.57358305200001));
#179294=CARTESIAN_POINT('Ctrl Pts',(9.56879440599995,15.2,-4.57490021400002));
#179295=CARTESIAN_POINT('Ctrl Pts',(9.57045606999994,15.2,-4.57622310400001));
#179296=CARTESIAN_POINT('Ctrl Pts',(9.57212187699995,15.2,-4.57755172000001));
#179297=CARTESIAN_POINT('Ctrl Pts',(9.57379180899995,15.2,-4.57888606200001));
#179298=CARTESIAN_POINT('Ctrl Pts',(9.57546584599994,15.2,-4.58022613000002));
#179299=CARTESIAN_POINT('Ctrl Pts',(9.57714397399995,15.2,-4.58157192400002));
#179300=CARTESIAN_POINT('Ctrl Pts',(9.57882617099994,15.2,-4.58292344400002));
#179301=CARTESIAN_POINT('Ctrl Pts',(9.58051242199994,15.2,-4.58428068800002));
#179302=CARTESIAN_POINT('Ctrl Pts',(9.58220270699995,15.2,-4.58564365500001));
#179303=CARTESIAN_POINT('Ctrl Pts',(9.58389701199994,15.2,-4.58701234700001));
#179304=CARTESIAN_POINT('Ctrl Pts',(9.58559531499995,15.2,-4.58838676100001));
#179305=CARTESIAN_POINT('Ctrl Pts',(9.58729760199994,15.2,-4.58976689800001));
#179306=CARTESIAN_POINT('Ctrl Pts',(9.58900385399994,15.2,-4.59115275800002));
#179307=CARTESIAN_POINT('Ctrl Pts',(9.59071405399994,15.2,-4.59254433900002));
#179308=CARTESIAN_POINT('Ctrl Pts',(9.59242818399994,15.2,-4.59394164100001));
#179309=CARTESIAN_POINT('Ctrl Pts',(9.59414622799994,15.2,-4.59534466400001));
#179310=CARTESIAN_POINT('Ctrl Pts',(9.59586816799994,15.2,-4.59675340600001));
#179311=CARTESIAN_POINT('Ctrl Pts',(9.59759398799994,15.2,-4.59816786900001));
#179312=CARTESIAN_POINT('Ctrl Pts',(9.59932366799995,15.2,-4.59958805000001));
#179313=CARTESIAN_POINT('Ctrl Pts',(9.60105719199994,15.2,-4.60101394900001));
#179314=CARTESIAN_POINT('Ctrl Pts',(9.60279454499995,15.2,-4.60244556600002));
#179315=CARTESIAN_POINT('Ctrl Pts',(9.60453570799995,15.2,-4.60388290000001));
#179316=CARTESIAN_POINT('Ctrl Pts',(9.60628066499994,15.2,-4.60532595000001));
#179317=CARTESIAN_POINT('Ctrl Pts',(9.60802939899994,15.2,-4.60677471700001));
#179318=CARTESIAN_POINT('Ctrl Pts',(9.60978189399994,15.2,-4.60822919900002));
#179319=CARTESIAN_POINT('Ctrl Pts',(9.61153812999994,15.2,-4.60968939500002));
#179320=CARTESIAN_POINT('Ctrl Pts',(9.61329809399994,15.2,-4.61115530500001));
#179321=CARTESIAN_POINT('Ctrl Pts',(9.61506176799995,15.2,-4.61262692900001));
#179322=CARTESIAN_POINT('Ctrl Pts',(9.61682913599994,15.2,-4.61410426600001));
#179323=CARTESIAN_POINT('Ctrl Pts',(9.61860017899994,15.2,-4.61558731400002));
#179324=CARTESIAN_POINT('Ctrl Pts',(9.62037488299995,15.2,-4.61707607400001));
#179325=CARTESIAN_POINT('Ctrl Pts',(9.62215323099995,15.2,-4.61857054400001));
#179326=CARTESIAN_POINT('Ctrl Pts',(9.62393520599995,15.2,-4.62007072400001));
#179327=CARTESIAN_POINT('Ctrl Pts',(9.62572079199994,15.2,-4.62157661300001));
#179328=CARTESIAN_POINT('Ctrl Pts',(9.62750997299995,15.2,-4.62308821200001));
#179329=CARTESIAN_POINT('Ctrl Pts',(9.62930273199994,15.2,-4.62460551700001));
#179330=CARTESIAN_POINT('Ctrl Pts',(9.63109905299994,15.2,-4.62612853000001));
#179331=CARTESIAN_POINT('Ctrl Pts',(9.63289892099995,15.2,-4.62765724900001));
#179332=CARTESIAN_POINT('Ctrl Pts',(9.63470231799995,15.2,-4.62919167300001));
#179333=CARTESIAN_POINT('Ctrl Pts',(9.63650922799994,15.2,-4.63073180200002));
#179334=CARTESIAN_POINT('Ctrl Pts',(9.63831963699995,15.2,-4.63227763600001));
#179335=CARTESIAN_POINT('Ctrl Pts',(9.64013352699994,15.2,-4.63382917200001));
#179336=CARTESIAN_POINT('Ctrl Pts',(9.64195088399994,15.2,-4.63538641000001));
#179337=CARTESIAN_POINT('Ctrl Pts',(9.64377168999994,15.2,-4.63694935100001));
#179338=CARTESIAN_POINT('Ctrl Pts',(9.64559592999995,15.2,-4.63851799300001));
#179339=CARTESIAN_POINT('Ctrl Pts',(9.64742358899995,15.2,-4.64009233400001));
#179340=CARTESIAN_POINT('Ctrl Pts',(9.64925464999994,15.2,-4.64167237400002));
#179341=CARTESIAN_POINT('Ctrl Pts',(9.65108909699994,15.2,-4.64325811300002));
#179342=CARTESIAN_POINT('Ctrl Pts',(9.65292691699995,15.2,-4.64484954900001));
#179343=CARTESIAN_POINT('Ctrl Pts',(9.65476809099994,15.2,-4.64644668200001));
#179344=CARTESIAN_POINT('Ctrl Pts',(9.65661260499994,15.2,-4.64804951100001));
#179345=CARTESIAN_POINT('Ctrl Pts',(9.65846044499994,15.2,-4.64965803400001));
#179346=CARTESIAN_POINT('Ctrl Pts',(9.66031159299994,15.2,-4.65127225200002));
#179347=CARTESIAN_POINT('Ctrl Pts',(9.66216603399995,15.2,-4.65289216300001));
#179348=CARTESIAN_POINT('Ctrl Pts',(9.66402375299995,15.2,-4.65451776500001));
#179349=CARTESIAN_POINT('Ctrl Pts',(9.66588473599994,15.2,-4.65614906000001));
#179350=CARTESIAN_POINT('Ctrl Pts',(9.66774896599994,15.2,-4.65778604500001));
#179351=CARTESIAN_POINT('Ctrl Pts',(9.66961642799994,15.2,-4.65942871900001));
#179352=CARTESIAN_POINT('Ctrl Pts',(9.67148710599995,15.2,-4.66107708200001));
#179353=CARTESIAN_POINT('Ctrl Pts',(9.67336098799995,15.2,-4.66273113300002));
#179354=CARTESIAN_POINT('Ctrl Pts',(9.67523805399994,15.2,-4.66439087100001));
#179355=CARTESIAN_POINT('Ctrl Pts',(9.67711829399994,15.2,-4.66605629400001));
#179356=CARTESIAN_POINT('Ctrl Pts',(9.67900168899994,15.2,-4.66772740200001));
#179357=CARTESIAN_POINT('Ctrl Pts',(9.68088822599995,15.2,-4.66940419300002));
#179358=CARTESIAN_POINT('Ctrl Pts',(9.68277788899995,15.2,-4.67108666800002));
#179359=CARTESIAN_POINT('Ctrl Pts',(9.68467066399995,15.2,-4.67277482500001));
#179360=CARTESIAN_POINT('Ctrl Pts',(9.68656653499995,15.2,-4.67446866300001));
#179361=CARTESIAN_POINT('Ctrl Pts',(9.68846548899995,15.2,-4.67616818100002));
#179362=CARTESIAN_POINT('Ctrl Pts',(9.69036750899994,15.2,-4.67787337800001));
#179363=CARTESIAN_POINT('Ctrl Pts',(9.69227258299994,15.2,-4.67958425200001));
#179364=CARTESIAN_POINT('Ctrl Pts',(9.69418069299994,15.2,-4.68130080300002));
#179365=CARTESIAN_POINT('Ctrl Pts',(9.69609182599994,15.2,-4.68302303000002));
#179366=CARTESIAN_POINT('Ctrl Pts',(9.69800596699995,15.2,-4.68475093300002));
#179367=CARTESIAN_POINT('Ctrl Pts',(9.69992310199994,15.2,-4.68648450800002));
#179368=CARTESIAN_POINT('Ctrl Pts',(9.70184321499995,15.2,-4.68822375800002));
#179369=CARTESIAN_POINT('Ctrl Pts',(9.70376629399994,15.2,-4.68996867700001));
#179370=CARTESIAN_POINT('Ctrl Pts',(9.70569232299994,15.2,-4.69171926800001));
#179371=CARTESIAN_POINT('Ctrl Pts',(9.70762128699995,15.2,-4.69347552800001));
#179372=CARTESIAN_POINT('Ctrl Pts',(9.70955317199994,15.2,-4.69523745800001));
#179373=CARTESIAN_POINT('Ctrl Pts',(9.71148796399994,15.2,-4.69700505400001));
#179374=CARTESIAN_POINT('Ctrl Pts',(9.71342564799994,15.2,-4.69877831600002));
#179375=CARTESIAN_POINT('Ctrl Pts',(9.71536621099995,15.2,-4.70055724400002));
#179376=CARTESIAN_POINT('Ctrl Pts',(9.71730963799994,15.2,-4.70234183600001));
#179377=CARTESIAN_POINT('Ctrl Pts',(9.71925591399994,15.2,-4.70413209100002));
#179378=CARTESIAN_POINT('Ctrl Pts',(9.72120502599994,15.2,-4.70592800700001));
#179379=CARTESIAN_POINT('Ctrl Pts',(9.72315695899994,15.2,-4.70772958400001));
#179380=CARTESIAN_POINT('Ctrl Pts',(9.72511169899994,15.2,-4.70953682000002));
#179381=CARTESIAN_POINT('Ctrl Pts',(9.72706923299994,15.2,-4.71134971600002));
#179382=CARTESIAN_POINT('Ctrl Pts',(9.72902954599994,15.2,-4.71316826800001));
#179383=CARTESIAN_POINT('Ctrl Pts',(9.73099262399994,15.2,-4.71499247700002));
#179384=CARTESIAN_POINT('Ctrl Pts',(9.73295845299995,15.2,-4.71682234000002));
#179385=CARTESIAN_POINT('Ctrl Pts',(9.73492701999995,15.2,-4.71865785700002));
#179386=CARTESIAN_POINT('Ctrl Pts',(9.73689830999995,15.2,-4.72049902600002));
#179387=CARTESIAN_POINT('Ctrl Pts',(9.73887230999994,15.2,-4.72234584700002));
#179388=CARTESIAN_POINT('Ctrl Pts',(9.74084900499994,15.2,-4.72419831800002));
#179389=CARTESIAN_POINT('Ctrl Pts',(9.74282838199995,15.2,-4.72605643900001));
#179390=CARTESIAN_POINT('Ctrl Pts',(9.74481042799994,15.2,-4.72792020600002));
#179391=CARTESIAN_POINT('Ctrl Pts',(9.74679512899994,15.2,-4.72978962000001));
#179392=CARTESIAN_POINT('Ctrl Pts',(9.74878246899994,15.2,-4.73166467900001));
#179393=CARTESIAN_POINT('Ctrl Pts',(9.75077243699995,15.2,-4.73354538300002));
#179394=CARTESIAN_POINT('Ctrl Pts',(9.75276501899994,15.2,-4.73543173000001));
#179395=CARTESIAN_POINT('Ctrl Pts',(9.75476020099994,15.2,-4.73732371700001));
#179396=CARTESIAN_POINT('Ctrl Pts',(9.75675797099995,15.2,-4.73922134600001));
#179397=CARTESIAN_POINT('Ctrl Pts',(9.75875831199994,15.2,-4.74112461300002));
#179398=CARTESIAN_POINT('Ctrl Pts',(9.76076121399995,15.2,-4.74303351800001));
#179399=CARTESIAN_POINT('Ctrl Pts',(9.76276666199994,15.2,-4.74494806000001));
#179400=CARTESIAN_POINT('Ctrl Pts',(9.76477464199995,15.2,-4.74686823700001));
#179401=CARTESIAN_POINT('Ctrl Pts',(9.76678514199994,15.2,-4.74879404700001));
#179402=CARTESIAN_POINT('Ctrl Pts',(9.76879814799995,15.2,-4.75072549100001));
#179403=CARTESIAN_POINT('Ctrl Pts',(9.77081364699995,15.2,-4.75266256500001));
#179404=CARTESIAN_POINT('Ctrl Pts',(9.77283162499995,15.2,-4.75460527100001));
#179405=CARTESIAN_POINT('Ctrl Pts',(9.77485206899994,15.2,-4.75655360400001));
#179406=CARTESIAN_POINT('Ctrl Pts',(9.77687496799994,15.2,-4.75850756500002));
#179407=CARTESIAN_POINT('Ctrl Pts',(9.77890030599994,15.2,-4.76046715200001));
#179408=CARTESIAN_POINT('Ctrl Pts',(9.78092806999994,15.2,-4.76243236400002));
#179409=CARTESIAN_POINT('Ctrl Pts',(9.78295824899994,15.2,-4.76440319900002));
#179410=CARTESIAN_POINT('Ctrl Pts',(9.78499082799994,15.2,-4.76637965700001));
#179411=CARTESIAN_POINT('Ctrl Pts',(9.78702579499994,15.2,-4.76836173400002));
#179412=CARTESIAN_POINT('Ctrl Pts',(9.78906313699994,15.2,-4.77034943200001));
#179413=CARTESIAN_POINT('Ctrl Pts',(9.79110284099994,15.2,-4.77234274600002));
#179414=CARTESIAN_POINT('Ctrl Pts',(9.79314489299994,15.2,-4.77434167900002));
#179415=CARTESIAN_POINT('Ctrl Pts',(9.79518928099995,15.2,-4.77634622600001));
#179416=CARTESIAN_POINT('Ctrl Pts',(9.79723599299994,15.2,-4.77835638700002));
#179417=CARTESIAN_POINT('Ctrl Pts',(9.79928501499994,15.2,-4.78037216000001));
#179418=CARTESIAN_POINT('Ctrl Pts',(9.80133633399995,15.2,-4.78239354400001));
#179419=CARTESIAN_POINT('Ctrl Pts',(9.80338993799995,15.2,-4.78442053800002));
#179420=CARTESIAN_POINT('Ctrl Pts',(9.80544581399995,15.2,-4.78645314000001));
#179421=CARTESIAN_POINT('Ctrl Pts',(9.80750394899994,15.2,-4.78849134900001));
#179422=CARTESIAN_POINT('Ctrl Pts',(9.80956432999994,15.2,-4.79053516400001));
#179423=CARTESIAN_POINT('Ctrl Pts',(9.81162694599995,15.2,-4.79258458200002));
#179424=CARTESIAN_POINT('Ctrl Pts',(9.81369178299994,15.2,-4.79463960300002));
#179425=CARTESIAN_POINT('Ctrl Pts',(9.81575882799994,15.2,-4.79670022500001));
#179426=CARTESIAN_POINT('Ctrl Pts',(9.81782806999994,15.2,-4.79876644700001));
#179427=CARTESIAN_POINT('Ctrl Pts',(9.81989949599994,15.2,-4.80083826600001));
#179428=CARTESIAN_POINT('Ctrl Pts',(9.82197309199995,15.2,-4.80291568300002));
#179429=CARTESIAN_POINT('Ctrl Pts',(9.82404884799994,15.2,-4.80499869500001));
#179430=CARTESIAN_POINT('Ctrl Pts',(9.82612674899995,15.2,-4.80708730000002));
#179431=CARTESIAN_POINT('Ctrl Pts',(9.82820678499994,15.2,-4.80918149800001));
#179432=CARTESIAN_POINT('Ctrl Pts',(9.83028894099995,15.2,-4.81128128700002));
#179433=CARTESIAN_POINT('Ctrl Pts',(9.83237320799994,15.2,-4.81338666500001));
#179434=CARTESIAN_POINT('Ctrl Pts',(9.83445956999994,15.2,-4.81549763000002));
#179435=CARTESIAN_POINT('Ctrl Pts',(9.83654801799995,15.2,-4.81761418300001));
#179436=CARTESIAN_POINT('Ctrl Pts',(9.83863853799994,15.2,-4.81973632000001));
#179437=CARTESIAN_POINT('Ctrl Pts',(9.84073111699994,15.2,-4.82186404000001));
#179438=CARTESIAN_POINT('Ctrl Pts',(9.84282574499994,15.2,-4.82399734200001));
#179439=CARTESIAN_POINT('Ctrl Pts',(9.84492240799995,15.2,-4.82613622400001));
#179440=CARTESIAN_POINT('Ctrl Pts',(9.84702109499995,15.2,-4.82828068500002));
#179441=CARTESIAN_POINT('Ctrl Pts',(9.84912179299995,15.2,-4.83043072400001));
#179442=CARTESIAN_POINT('Ctrl Pts',(9.85122449199994,15.2,-4.83258633800002));
#179443=CARTESIAN_POINT('Ctrl Pts',(9.85332917699995,15.2,-4.83474752600001));
#179444=CARTESIAN_POINT('Ctrl Pts',(9.85543583699994,15.2,-4.83691428600002));
#179445=CARTESIAN_POINT('Ctrl Pts',(9.85754445999994,15.2,-4.83908661700001));
#179446=CARTESIAN_POINT('Ctrl Pts',(9.85965503599994,15.2,-4.84126451800002));
#179447=CARTESIAN_POINT('Ctrl Pts',(9.86176754899994,15.2,-4.84344798700001));
#179448=CARTESIAN_POINT('Ctrl Pts',(9.86388199199994,15.2,-4.84563702200001));
#179449=CARTESIAN_POINT('Ctrl Pts',(9.86599834899994,15.2,-4.84783162100001));
#179450=CARTESIAN_POINT('Ctrl Pts',(9.86811660899994,15.2,-4.85003178400001));
#179451=CARTESIAN_POINT('Ctrl Pts',(9.87023676299994,15.2,-4.85223750900001));
#179452=CARTESIAN_POINT('Ctrl Pts',(9.87235879499995,15.2,-4.85444879300001));
#179453=CARTESIAN_POINT('Ctrl Pts',(9.87448269599994,15.2,-4.85666563600001));
#179454=CARTESIAN_POINT('Ctrl Pts',(9.87660845399994,15.2,-4.85888803500002));
#179455=CARTESIAN_POINT('Ctrl Pts',(9.87873605699994,15.2,-4.86111598900001));
#179456=CARTESIAN_POINT('Ctrl Pts',(9.88086549299994,15.2,-4.86334949700002));
#179457=CARTESIAN_POINT('Ctrl Pts',(9.88299674999995,15.2,-4.86558855600002));
#179458=CARTESIAN_POINT('Ctrl Pts',(9.88512981699994,15.2,-4.86783316500001));
#179459=CARTESIAN_POINT('Ctrl Pts',(9.88726468299994,15.2,-4.87008332300002));
#179460=CARTESIAN_POINT('Ctrl Pts',(9.88940133499994,15.2,-4.87233902900002));
#179461=CARTESIAN_POINT('Ctrl Pts',(9.89153976099994,15.2,-4.87460027900001));
#179462=CARTESIAN_POINT('Ctrl Pts',(9.89367995199995,15.2,-4.87686707300002));
#179463=CARTESIAN_POINT('Ctrl Pts',(9.89582189499994,15.2,-4.87913940900001));
#179464=CARTESIAN_POINT('Ctrl Pts',(9.89796557699995,15.2,-4.88141728600001));
#179465=CARTESIAN_POINT('Ctrl Pts',(9.90011098899994,15.2,-4.88370070000002));
#179466=CARTESIAN_POINT('Ctrl Pts',(9.90225811999995,15.2,-4.88598965200001));
#179467=CARTESIAN_POINT('Ctrl Pts',(9.90440695499995,15.2,-4.88828413900002));
#179468=CARTESIAN_POINT('Ctrl Pts',(9.90655748599995,15.2,-4.89058415900002));
#179469=CARTESIAN_POINT('Ctrl Pts',(9.90870969999994,15.2,-4.89288971200001));
#179470=CARTESIAN_POINT('Ctrl Pts',(9.91086358699994,15.2,-4.89520079400001));
#179471=CARTESIAN_POINT('Ctrl Pts',(9.91301913399995,15.2,-4.89751740500001));
#179472=CARTESIAN_POINT('Ctrl Pts',(9.91517632999994,15.2,-4.89983954200001));
#179473=CARTESIAN_POINT('Ctrl Pts',(9.91733516599995,15.2,-4.90216720500001));
#179474=CARTESIAN_POINT('Ctrl Pts',(9.91949562799994,15.2,-4.90450039100002));
#179475=CARTESIAN_POINT('Ctrl Pts',(9.92165770599994,15.2,-4.90683909900001));
#179476=CARTESIAN_POINT('Ctrl Pts',(9.92382138899995,15.2,-4.90918332600002));
#179477=CARTESIAN_POINT('Ctrl Pts',(9.92598666499994,15.2,-4.91153307200001));
#179478=CARTESIAN_POINT('Ctrl Pts',(9.92815352399995,15.2,-4.91388833500002));
#179479=CARTESIAN_POINT('Ctrl Pts',(9.93032195399994,15.2,-4.91624911100002));
#179480=CARTESIAN_POINT('Ctrl Pts',(9.93249194399995,15.2,-4.91861540000002));
#179481=CARTESIAN_POINT('Ctrl Pts',(9.93466348399994,15.2,-4.92098720100001));
#179482=CARTESIAN_POINT('Ctrl Pts',(9.93683656099994,15.2,-4.92336451100002));
#179483=CARTESIAN_POINT('Ctrl Pts',(9.93901116599995,15.2,-4.92574732900001));
#179484=CARTESIAN_POINT('Ctrl Pts',(9.94118728699994,15.2,-4.92813565300001));
#179485=CARTESIAN_POINT('Ctrl Pts',(9.94336491299994,15.2,-4.93052948100001));
#179486=CARTESIAN_POINT('Ctrl Pts',(9.94554403299994,15.2,-4.93292881000002));
#179487=CARTESIAN_POINT('Ctrl Pts',(9.94772463699995,15.2,-4.93533364100001));
#179488=CARTESIAN_POINT('Ctrl Pts',(9.94990671399995,15.2,-4.93774397000001));
#179489=CARTESIAN_POINT('Ctrl Pts',(9.95209025099994,15.2,-4.94015979700002));
#179490=CARTESIAN_POINT('Ctrl Pts',(9.95427523999994,15.2,-4.94258111700002));
#179491=CARTESIAN_POINT('Ctrl Pts',(9.95646166799995,15.2,-4.94500793200002));
#179492=CARTESIAN_POINT('Ctrl Pts',(9.95864952599995,15.2,-4.94744023800001));
#179493=CARTESIAN_POINT('Ctrl Pts',(9.96083880199994,15.2,-4.94987803500001));
#179494=CARTESIAN_POINT('Ctrl Pts',(9.96302948499994,15.2,-4.95232131800002));
#179495=CARTESIAN_POINT('Ctrl Pts',(9.96522156599994,15.2,-4.95477008800002));
#179496=CARTESIAN_POINT('Ctrl Pts',(9.96741503199994,15.2,-4.95722434200002));
#179497=CARTESIAN_POINT('Ctrl Pts',(9.96960987299994,15.2,-4.95968407800001));
#179498=CARTESIAN_POINT('Ctrl Pts',(9.97180608099995,15.2,-4.96214929600002));
#179499=CARTESIAN_POINT('Ctrl Pts',(9.97400364199994,15.2,-4.96461999100001));
#179500=CARTESIAN_POINT('Ctrl Pts',(9.97620254699994,15.2,-4.96709616400001));
#179501=CARTESIAN_POINT('Ctrl Pts',(9.97840278499995,15.2,-4.96957781100001));
#179502=CARTESIAN_POINT('Ctrl Pts',(9.98060434499994,15.2,-4.97206493200002));
#179503=CARTESIAN_POINT('Ctrl Pts',(9.98280721699994,15.2,-4.97455752400001));
#179504=CARTESIAN_POINT('Ctrl Pts',(9.98501138999995,15.2,-4.97705558600002));
#179505=CARTESIAN_POINT('Ctrl Pts',(9.98721685399994,15.2,-4.97955911500001));
#179506=CARTESIAN_POINT('Ctrl Pts',(9.98942359899995,15.2,-4.98206811000002));
#179507=CARTESIAN_POINT('Ctrl Pts',(9.99163161399995,15.2,-4.98458256900001));
#179508=CARTESIAN_POINT('Ctrl Pts',(9.99384088799994,15.2,-4.98710249000001));
#179509=CARTESIAN_POINT('Ctrl Pts',(9.99605141199994,15.2,-4.98962787000002));
#179510=CARTESIAN_POINT('Ctrl Pts',(9.99826317399994,15.2,-4.99215870900001));
#179511=CARTESIAN_POINT('Ctrl Pts',(10.0004761639999,15.2,-4.99469500400001));
#179512=CARTESIAN_POINT('Ctrl Pts',(10.0026903729999,15.2,-4.99723675300002));
#179513=CARTESIAN_POINT('Ctrl Pts',(10.0049057889999,15.2,-4.99978395500001));
#179514=CARTESIAN_POINT('Ctrl Pts',(10.0071224029999,15.2,-5.00233660800002));
#179515=CARTESIAN_POINT('Ctrl Pts',(10.0093402039999,15.2,-5.00489470900002));
#179516=CARTESIAN_POINT('Ctrl Pts',(10.0115591819999,15.2,-5.00745825600001));
#179517=CARTESIAN_POINT('Ctrl Pts',(10.0137793259999,15.2,-5.01002724800002));
#179518=CARTESIAN_POINT('Ctrl Pts',(10.0160006259999,15.2,-5.01260168400002));
#179519=CARTESIAN_POINT('Ctrl Pts',(10.0182230729999,15.2,-5.01518156000001));
#179520=CARTESIAN_POINT('Ctrl Pts',(10.0204466549999,15.2,-5.01776687600001));
#179521=CARTESIAN_POINT('Ctrl Pts',(10.0226713639999,15.2,-5.02035762800002));
#179522=CARTESIAN_POINT('Ctrl Pts',(10.0248971889999,15.2,-5.02295381500002));
#179523=CARTESIAN_POINT('Ctrl Pts',(10.0271241189999,15.2,-5.02555543600002));
#179524=CARTESIAN_POINT('Ctrl Pts',(10.0293521449999,15.2,-5.02816248700002));
#179525=CARTESIAN_POINT('Ctrl Pts',(10.0315812549999,15.2,-5.03077496800001));
#179526=CARTESIAN_POINT('Ctrl Pts',(10.0338114419999,15.2,-5.03339287600001));
#179527=CARTESIAN_POINT('Ctrl Pts',(10.0360426939999,15.2,-5.03601620900001));
#179528=CARTESIAN_POINT('Ctrl Pts',(10.0382750009999,15.2,-5.03864496500002));
#179529=CARTESIAN_POINT('Ctrl Pts',(10.0405083539999,15.2,-5.04127914300001));
#179530=CARTESIAN_POINT('Ctrl Pts',(10.0427427419999,15.2,-5.04391874100001));
#179531=CARTESIAN_POINT('Ctrl Pts',(10.0449781559999,15.2,-5.04656375500002));
#179532=CARTESIAN_POINT('Ctrl Pts',(10.0472145849999,15.2,-5.04921418600001));
#179533=CARTESIAN_POINT('Ctrl Pts',(10.0494520199999,15.2,-5.05187002900001));
#179534=CARTESIAN_POINT('Ctrl Pts',(10.0516904509999,15.2,-5.05453128400001));
#179535=CARTESIAN_POINT('Ctrl Pts',(10.0539298679999,15.2,-5.05719794800001));
#179536=CARTESIAN_POINT('Ctrl Pts',(10.0561702599999,15.2,-5.05987001900001));
#179537=CARTESIAN_POINT('Ctrl Pts',(10.0584116189999,15.2,-5.06254749600001));
#179538=CARTESIAN_POINT('Ctrl Pts',(10.0606539349999,15.2,-5.06523037500001));
#179539=CARTESIAN_POINT('Ctrl Pts',(10.0628971959999,15.2,-5.06791865600002));
#179540=CARTESIAN_POINT('Ctrl Pts',(10.0651413949999,15.2,-5.07061233700002));
#179541=CARTESIAN_POINT('Ctrl Pts',(10.0673865209999,15.2,-5.07331141500002));
#179542=CARTESIAN_POINT('Ctrl Pts',(10.0696325649999,15.2,-5.07601588800001));
#179543=CARTESIAN_POINT('Ctrl Pts',(10.0718795159999,15.2,-5.07872575400001));
#179544=CARTESIAN_POINT('Ctrl Pts',(10.0741273649999,15.2,-5.08144101100001));
#179545=CARTESIAN_POINT('Ctrl Pts',(10.0763761029999,15.2,-5.08416165800002));
#179546=CARTESIAN_POINT('Ctrl Pts',(10.0786257189999,15.2,-5.08688769200001));
#179547=CARTESIAN_POINT('Ctrl Pts',(10.0808762039999,15.2,-5.08961911000001));
#179548=CARTESIAN_POINT('Ctrl Pts',(10.0831275479999,15.2,-5.09235591100001));
#179549=CARTESIAN_POINT('Ctrl Pts',(10.0853797429999,15.2,-5.09509809400001));
#179550=CARTESIAN_POINT('Ctrl Pts',(10.0876327779999,15.2,-5.09784565500001));
#179551=CARTESIAN_POINT('Ctrl Pts',(10.0898866439999,15.2,-5.10059859300001));
#179552=CARTESIAN_POINT('Ctrl Pts',(10.0921413299999,15.2,-5.10335690500002));
#179553=CARTESIAN_POINT('Ctrl Pts',(10.0943968289999,15.2,-5.10612059000001));
#179554=CARTESIAN_POINT('Ctrl Pts',(10.0966531299999,15.2,-5.10888964500001));
#179555=CARTESIAN_POINT('Ctrl Pts',(10.0989102229999,15.2,-5.11166406900001));
#179556=CARTESIAN_POINT('Ctrl Pts',(10.1011680999999,15.2,-5.11444386000001));
#179557=CARTESIAN_POINT('Ctrl Pts',(10.1034267499999,15.2,-5.11722901400002));
#179558=CARTESIAN_POINT('Ctrl Pts',(10.1056861639999,15.2,-5.12001953100001));
#179559=CARTESIAN_POINT('Ctrl Pts',(10.1079463349999,15.2,-5.12281540800001));
#179560=CARTESIAN_POINT('Ctrl Pts',(10.1102072499999,15.2,-5.12561664200001));
#179561=CARTESIAN_POINT('Ctrl Pts',(10.1124689019999,15.2,-5.12842323200001));
#179562=CARTESIAN_POINT('Ctrl Pts',(10.1147312799999,15.2,-5.13123517600001));
#179563=CARTESIAN_POINT('Ctrl Pts',(10.1169943759999,15.2,-5.13405247200001));
#179564=CARTESIAN_POINT('Ctrl Pts',(10.1192581799999,15.2,-5.13687511700001));
#179565=CARTESIAN_POINT('Ctrl Pts',(10.1215226839999,15.2,-5.13970310900001));
#179566=CARTESIAN_POINT('Ctrl Pts',(10.1237878759999,15.2,-5.14253644700001));
#179567=CARTESIAN_POINT('Ctrl Pts',(10.1260537499999,15.2,-5.14537512800001));
#179568=CARTESIAN_POINT('Ctrl Pts',(10.1283202939999,15.2,-5.14821914900002));
#179569=CARTESIAN_POINT('Ctrl Pts',(10.1305874999999,15.2,-5.15106851000001));
#179570=CARTESIAN_POINT('Ctrl Pts',(10.1328553589999,15.2,-5.15392320600002));
#179571=CARTESIAN_POINT('Ctrl Pts',(10.1351238609999,15.2,-5.15678323800001));
#179572=CARTESIAN_POINT('Ctrl Pts',(10.1373929979999,15.2,-5.15964860200001));
#179573=CARTESIAN_POINT('Ctrl Pts',(10.1396627609999,15.2,-5.16251929700001));
#179574=CARTESIAN_POINT('Ctrl Pts',(10.1419331389999,15.2,-5.16539531900001));
#179575=CARTESIAN_POINT('Ctrl Pts',(10.1442041239999,15.2,-5.16827666700001));
#179576=CARTESIAN_POINT('Ctrl Pts',(10.1464757069999,15.2,-5.17116333800002));
#179577=CARTESIAN_POINT('Ctrl Pts',(10.1487478799999,15.2,-5.17405533200002));
#179578=CARTESIAN_POINT('Ctrl Pts',(10.1510206309999,15.2,-5.17695264500002));
#179579=CARTESIAN_POINT('Ctrl Pts',(10.1532939539999,15.2,-5.17985527400001));
#179580=CARTESIAN_POINT('Ctrl Pts',(10.1555678379999,15.2,-5.18276321900002));
#179581=CARTESIAN_POINT('Ctrl Pts',(10.1578422729999,15.2,-5.18567647600001));
#179582=CARTESIAN_POINT('Ctrl Pts',(10.1601172529999,15.2,-5.18859504400002));
#179583=CARTESIAN_POINT('Ctrl Pts',(10.1623927679999,15.2,-5.19151892100002));
#179584=CARTESIAN_POINT('Ctrl Pts',(10.1646688079999,15.2,-5.19444810300001));
#179585=CARTESIAN_POINT('Ctrl Pts',(10.1669453649999,15.2,-5.19738259100002));
#179586=CARTESIAN_POINT('Ctrl Pts',(10.1692224309999,15.2,-5.20032238000002));
#179587=CARTESIAN_POINT('Ctrl Pts',(10.1714999969999,15.2,-5.20326746900002));
#179588=CARTESIAN_POINT('Ctrl Pts',(10.1737780519999,15.2,-5.20621785500001));
#179589=CARTESIAN_POINT('Ctrl Pts',(10.1760565879999,15.2,-5.20917353600002));
#179590=CARTESIAN_POINT('Ctrl Pts',(10.1783355949999,15.2,-5.21213451000001));
#179591=CARTESIAN_POINT('Ctrl Pts',(10.1806150639999,15.2,-5.21510077400002));
#179592=CARTESIAN_POINT('Ctrl Pts',(10.1828949879999,15.2,-5.21807232700001));
#179593=CARTESIAN_POINT('Ctrl Pts',(10.1851753559999,15.2,-5.22104916700001));
#179594=CARTESIAN_POINT('Ctrl Pts',(10.1874561619999,15.2,-5.22403129000002));
#179595=CARTESIAN_POINT('Ctrl Pts',(10.1897373969999,15.2,-5.22701869500001));
#179596=CARTESIAN_POINT('Ctrl Pts',(10.1920190549999,15.2,-5.23001138000001));
#179597=CARTESIAN_POINT('Ctrl Pts',(10.1943011249999,15.2,-5.23300934300002));
#179598=CARTESIAN_POINT('Ctrl Pts',(10.1965835999999,15.2,-5.23601258300001));
#179599=CARTESIAN_POINT('Ctrl Pts',(10.1988664679999,15.2,-5.23902109400002));
#179600=CARTESIAN_POINT('Ctrl Pts',(10.2011497209999,15.2,-5.24203487700001));
#179601=CARTESIAN_POINT('Ctrl Pts',(10.2034333439999,15.2,-5.24505392700001));
#179602=CARTESIAN_POINT('Ctrl Pts',(10.2057173299999,15.2,-5.24807824100002));
#179603=CARTESIAN_POINT('Ctrl Pts',(10.2080016679999,15.2,-5.25110781800001));
#179604=CARTESIAN_POINT('Ctrl Pts',(10.2102863519999,15.2,-5.25414265600002));
#179605=CARTESIAN_POINT('Ctrl Pts',(10.2125713739999,15.2,-5.25718275100001));
#179606=CARTESIAN_POINT('Ctrl Pts',(10.2148567309999,15.2,-5.26022810500002));
#179607=CARTESIAN_POINT('Ctrl Pts',(10.2171424209999,15.2,-5.26327871600001));
#179608=CARTESIAN_POINT('Ctrl Pts',(10.2189712369999,15.2,-5.26572340900001));
#179609=CARTESIAN_POINT('Ctrl Pts',(10.2203429999999,15.2,-5.26755929400001));
#179610=CARTESIAN_POINT('Ctrl Pts',(10.2212575739999,15.2,-5.26878426900002));
#179611=CARTESIAN_POINT('Ctrl Pts',(10.2217148779999,15.2,-5.26939701900002));
#179612=CARTESIAN_POINT('Ctrl Pts',(8.88241603299995,15.2,-5.36127880600001));
#179613=CARTESIAN_POINT('Ctrl Pts',(8.88241603299995,11.6,-5.36127880600001));
#179614=CARTESIAN_POINT('Ctrl Pts',(8.88257249699994,15.2,-5.36135574400001));
#179615=CARTESIAN_POINT('Ctrl Pts',(8.88257249699994,11.6,-5.36135574400001));
#179616=CARTESIAN_POINT('Ctrl Pts',(8.88289092999995,15.2,-5.36151222900001));
#179617=CARTESIAN_POINT('Ctrl Pts',(8.88289092999995,11.6,-5.36151222900001));
#179618=CARTESIAN_POINT('Ctrl Pts',(8.88337354799994,15.2,-5.36174910400002));
#179619=CARTESIAN_POINT('Ctrl Pts',(8.88337354799994,11.6,-5.36174910400002));
#179620=CARTESIAN_POINT('Ctrl Pts',(8.88402391699995,15.2,-5.36206771000002));
#179621=CARTESIAN_POINT('Ctrl Pts',(8.88402391699995,11.6,-5.36206771000002));
#179622=CARTESIAN_POINT('Ctrl Pts',(8.88484693799995,15.2,-5.36246988000002));
#179623=CARTESIAN_POINT('Ctrl Pts',(8.88484693799995,11.6,-5.36246988000002));
#179624=CARTESIAN_POINT('Ctrl Pts',(8.88568370899995,15.2,-5.36287772900002));
#179625=CARTESIAN_POINT('Ctrl Pts',(8.88568370899995,11.6,-5.36287772900002));
#179626=CARTESIAN_POINT('Ctrl Pts',(8.88652944499994,15.2,-5.36328889700001));
#179627=CARTESIAN_POINT('Ctrl Pts',(8.88652944499994,11.6,-5.36328889700001));
#179628=CARTESIAN_POINT('Ctrl Pts',(8.88738413099994,15.2,-5.36370335800001));
#179629=CARTESIAN_POINT('Ctrl Pts',(8.88738413099994,11.6,-5.36370335800001));
#179630=CARTESIAN_POINT('Ctrl Pts',(8.88824774899994,15.2,-5.36412108300001));
#179631=CARTESIAN_POINT('Ctrl Pts',(8.88824774899994,11.6,-5.36412108300001));
#179632=CARTESIAN_POINT('Ctrl Pts',(8.88912028499995,15.2,-5.36454204400002));
#179633=CARTESIAN_POINT('Ctrl Pts',(8.88912028499995,11.6,-5.36454204400002));
#179634=CARTESIAN_POINT('Ctrl Pts',(8.89000171999994,15.2,-5.36496621500001));
#179635=CARTESIAN_POINT('Ctrl Pts',(8.89000171999994,11.6,-5.36496621500001));
#179636=CARTESIAN_POINT('Ctrl Pts',(8.89089203999994,15.2,-5.36539356700001));
#179637=CARTESIAN_POINT('Ctrl Pts',(8.89089203999994,11.6,-5.36539356700001));
#179638=CARTESIAN_POINT('Ctrl Pts',(8.89179122799994,15.2,-5.36582407300001));
#179639=CARTESIAN_POINT('Ctrl Pts',(8.89179122799994,11.6,-5.36582407300001));
#179640=CARTESIAN_POINT('Ctrl Pts',(8.89269926799994,15.2,-5.36625770500001));
#179641=CARTESIAN_POINT('Ctrl Pts',(8.89269926799994,11.6,-5.36625770500001));
#179642=CARTESIAN_POINT('Ctrl Pts',(8.89361614499995,15.2,-5.36669443700001));
#179643=CARTESIAN_POINT('Ctrl Pts',(8.89361614499995,11.6,-5.36669443700001));
#179644=CARTESIAN_POINT('Ctrl Pts',(8.89454184299994,15.2,-5.36713424100002));
#179645=CARTESIAN_POINT('Ctrl Pts',(8.89454184299994,11.6,-5.36713424100002));
#179646=CARTESIAN_POINT('Ctrl Pts',(8.89547634599994,15.2,-5.36757709000002));
#179647=CARTESIAN_POINT('Ctrl Pts',(8.89547634599994,11.6,-5.36757709000002));
#179648=CARTESIAN_POINT('Ctrl Pts',(8.89641963799994,15.2,-5.36802295800001));
#179649=CARTESIAN_POINT('Ctrl Pts',(8.89641963799994,11.6,-5.36802295800001));
#179650=CARTESIAN_POINT('Ctrl Pts',(8.89737170299994,15.2,-5.36847181900002));
#179651=CARTESIAN_POINT('Ctrl Pts',(8.89737170299994,11.6,-5.36847181900002));
#179652=CARTESIAN_POINT('Ctrl Pts',(8.89833252799994,15.2,-5.36892364600002));
#179653=CARTESIAN_POINT('Ctrl Pts',(8.89833252799994,11.6,-5.36892364600002));
#179654=CARTESIAN_POINT('Ctrl Pts',(8.89930209399994,15.2,-5.36937841200002));
#179655=CARTESIAN_POINT('Ctrl Pts',(8.89930209399994,11.6,-5.36937841200002));
#179656=CARTESIAN_POINT('Ctrl Pts',(8.90028038899995,15.2,-5.36983609200002));
#179657=CARTESIAN_POINT('Ctrl Pts',(8.90028038899995,11.6,-5.36983609200002));
#179658=CARTESIAN_POINT('Ctrl Pts',(8.90126739499994,15.2,-5.37029665800001));
#179659=CARTESIAN_POINT('Ctrl Pts',(8.90126739499994,11.6,-5.37029665800001));
#179660=CARTESIAN_POINT('Ctrl Pts',(8.90226309699995,15.2,-5.37076008600001));
#179661=CARTESIAN_POINT('Ctrl Pts',(8.90226309699995,11.6,-5.37076008600001));
#179662=CARTESIAN_POINT('Ctrl Pts',(8.90326748199995,15.2,-5.37122635100001));
#179663=CARTESIAN_POINT('Ctrl Pts',(8.90326748199995,11.6,-5.37122635100001));
#179664=CARTESIAN_POINT('Ctrl Pts',(8.90428053099994,15.2,-5.37169542400001));
#179665=CARTESIAN_POINT('Ctrl Pts',(8.90428053099994,11.6,-5.37169542400001));
#179666=CARTESIAN_POINT('Ctrl Pts',(8.90530223199994,15.2,-5.37216728200002));
#179667=CARTESIAN_POINT('Ctrl Pts',(8.90530223199994,11.6,-5.37216728200002));
#179668=CARTESIAN_POINT('Ctrl Pts',(8.90633256899994,15.2,-5.37264190000001));
#179669=CARTESIAN_POINT('Ctrl Pts',(8.90633256899994,11.6,-5.37264190000001));
#179670=CARTESIAN_POINT('Ctrl Pts',(8.90737152799994,15.2,-5.37311925000001));
#179671=CARTESIAN_POINT('Ctrl Pts',(8.90737152799994,11.6,-5.37311925000001));
#179672=CARTESIAN_POINT('Ctrl Pts',(8.90841909199995,15.2,-5.37359931000001));
#179673=CARTESIAN_POINT('Ctrl Pts',(8.90841909199995,11.6,-5.37359931000001));
#179674=CARTESIAN_POINT('Ctrl Pts',(8.90947524599994,15.2,-5.37408205300002));
#179675=CARTESIAN_POINT('Ctrl Pts',(8.90947524599994,11.6,-5.37408205300002));
#179676=CARTESIAN_POINT('Ctrl Pts',(8.91053997899995,15.2,-5.37456745500001));
#179677=CARTESIAN_POINT('Ctrl Pts',(8.91053997899995,11.6,-5.37456745500001));
#179678=CARTESIAN_POINT('Ctrl Pts',(8.91161327099995,15.2,-5.37505549100001));
#179679=CARTESIAN_POINT('Ctrl Pts',(8.91161327099995,11.6,-5.37505549100001));
#179680=CARTESIAN_POINT('Ctrl Pts',(8.91269511199994,15.2,-5.37554613500001));
#179681=CARTESIAN_POINT('Ctrl Pts',(8.91269511199994,11.6,-5.37554613500001));
#179682=CARTESIAN_POINT('Ctrl Pts',(8.91378548299994,15.2,-5.37603936500001));
#179683=CARTESIAN_POINT('Ctrl Pts',(8.91378548299994,11.6,-5.37603936500001));
#179684=CARTESIAN_POINT('Ctrl Pts',(8.91488437199994,15.2,-5.37653515400002));
#179685=CARTESIAN_POINT('Ctrl Pts',(8.91488437199994,11.6,-5.37653515400002));
#179686=CARTESIAN_POINT('Ctrl Pts',(8.91599176499994,15.2,-5.37703348000001));
#179687=CARTESIAN_POINT('Ctrl Pts',(8.91599176499994,11.6,-5.37703348000001));
#179688=CARTESIAN_POINT('Ctrl Pts',(8.91710764499994,15.2,-5.37753431800001));
#179689=CARTESIAN_POINT('Ctrl Pts',(8.91710764499994,11.6,-5.37753431800001));
#179690=CARTESIAN_POINT('Ctrl Pts',(8.91823200099994,15.2,-5.37803764300001));
#179691=CARTESIAN_POINT('Ctrl Pts',(8.91823200099994,11.6,-5.37803764300001));
#179692=CARTESIAN_POINT('Ctrl Pts',(8.91936481499994,15.2,-5.37854343100001));
#179693=CARTESIAN_POINT('Ctrl Pts',(8.91936481499994,11.6,-5.37854343100001));
#179694=CARTESIAN_POINT('Ctrl Pts',(8.92050607399994,15.2,-5.37905166000002));
#179695=CARTESIAN_POINT('Ctrl Pts',(8.92050607399994,11.6,-5.37905166000002));
#179696=CARTESIAN_POINT('Ctrl Pts',(8.92165576499995,15.2,-5.37956230500001));
#179697=CARTESIAN_POINT('Ctrl Pts',(8.92165576499995,11.6,-5.37956230500001));
#179698=CARTESIAN_POINT('Ctrl Pts',(8.92281387199995,15.2,-5.38007534200001));
#179699=CARTESIAN_POINT('Ctrl Pts',(8.92281387199995,11.6,-5.38007534200001));
#179700=CARTESIAN_POINT('Ctrl Pts',(8.92398038299994,15.2,-5.38059074800001));
#179701=CARTESIAN_POINT('Ctrl Pts',(8.92398038299994,11.6,-5.38059074800001));
#179702=CARTESIAN_POINT('Ctrl Pts',(8.92515528099995,15.2,-5.38110850000002));
#179703=CARTESIAN_POINT('Ctrl Pts',(8.92515528099995,11.6,-5.38110850000002));
#179704=CARTESIAN_POINT('Ctrl Pts',(8.92633855299995,15.2,-5.38162857400001));
#179705=CARTESIAN_POINT('Ctrl Pts',(8.92633855299995,11.6,-5.38162857400001));
#179706=CARTESIAN_POINT('Ctrl Pts',(8.92753018699995,15.2,-5.38215094700002));
#179707=CARTESIAN_POINT('Ctrl Pts',(8.92753018699995,11.6,-5.38215094700002));
#179708=CARTESIAN_POINT('Ctrl Pts',(8.92873016599994,15.2,-5.38267559600001));
#179709=CARTESIAN_POINT('Ctrl Pts',(8.92873016599994,11.6,-5.38267559600001));
#179710=CARTESIAN_POINT('Ctrl Pts',(8.92993847699995,15.2,-5.38320249900002));
#179711=CARTESIAN_POINT('Ctrl Pts',(8.92993847699995,11.6,-5.38320249900002));
#179712=CARTESIAN_POINT('Ctrl Pts',(8.93115510699995,15.2,-5.38373163200002));
#179713=CARTESIAN_POINT('Ctrl Pts',(8.93115510699995,11.6,-5.38373163200002));
#179714=CARTESIAN_POINT('Ctrl Pts',(8.93238004199995,15.2,-5.38426297200001));
#179715=CARTESIAN_POINT('Ctrl Pts',(8.93238004199995,11.6,-5.38426297200001));
#179716=CARTESIAN_POINT('Ctrl Pts',(8.93361326699995,15.2,-5.38479649700002));
#179717=CARTESIAN_POINT('Ctrl Pts',(8.93361326699995,11.6,-5.38479649700002));
#179718=CARTESIAN_POINT('Ctrl Pts',(8.93485476899994,15.2,-5.38533218400001));
#179719=CARTESIAN_POINT('Ctrl Pts',(8.93485476899994,11.6,-5.38533218400001));
#179720=CARTESIAN_POINT('Ctrl Pts',(8.93610453499995,15.2,-5.38587001200002));
#179721=CARTESIAN_POINT('Ctrl Pts',(8.93610453499995,11.6,-5.38587001200002));
#179722=CARTESIAN_POINT('Ctrl Pts',(8.93736255099994,15.2,-5.38640995700002));
#179723=CARTESIAN_POINT('Ctrl Pts',(8.93736255099994,11.6,-5.38640995700002));
#179724=CARTESIAN_POINT('Ctrl Pts',(8.93862880299995,15.2,-5.38695199700001));
#179725=CARTESIAN_POINT('Ctrl Pts',(8.93862880299995,11.6,-5.38695199700001));
#179726=CARTESIAN_POINT('Ctrl Pts',(8.93990327699994,15.2,-5.38749611000001));
#179727=CARTESIAN_POINT('Ctrl Pts',(8.93990327699994,11.6,-5.38749611000001));
#179728=CARTESIAN_POINT('Ctrl Pts',(8.94118596099995,15.2,-5.38804227600002));
#179729=CARTESIAN_POINT('Ctrl Pts',(8.94118596099995,11.6,-5.38804227600002));
#179730=CARTESIAN_POINT('Ctrl Pts',(8.94247683899994,15.2,-5.38859046900001));
#179731=CARTESIAN_POINT('Ctrl Pts',(8.94247683899994,11.6,-5.38859046900001));
#179732=CARTESIAN_POINT('Ctrl Pts',(8.94377590099995,15.2,-5.38914067100002));
#179733=CARTESIAN_POINT('Ctrl Pts',(8.94377590099995,11.6,-5.38914067100002));
#179734=CARTESIAN_POINT('Ctrl Pts',(8.94508313099994,15.2,-5.38969285800002));
#179735=CARTESIAN_POINT('Ctrl Pts',(8.94508313099994,11.6,-5.38969285800002));
#179736=CARTESIAN_POINT('Ctrl Pts',(8.94639851599995,15.2,-5.39024700900002));
#179737=CARTESIAN_POINT('Ctrl Pts',(8.94639851599995,11.6,-5.39024700900002));
#179738=CARTESIAN_POINT('Ctrl Pts',(8.94772204399995,15.2,-5.39080310300001));
#179739=CARTESIAN_POINT('Ctrl Pts',(8.94772204399995,11.6,-5.39080310300001));
#179740=CARTESIAN_POINT('Ctrl Pts',(8.94905369999995,15.2,-5.39136111800001));
#179741=CARTESIAN_POINT('Ctrl Pts',(8.94905369999995,11.6,-5.39136111800001));
#179742=CARTESIAN_POINT('Ctrl Pts',(8.95039347299995,15.2,-5.39192103300001));
#179743=CARTESIAN_POINT('Ctrl Pts',(8.95039347299995,11.6,-5.39192103300001));
#179744=CARTESIAN_POINT('Ctrl Pts',(8.95174134799994,15.2,-5.39248282600001));
#179745=CARTESIAN_POINT('Ctrl Pts',(8.95174134799994,11.6,-5.39248282600001));
#179746=CARTESIAN_POINT('Ctrl Pts',(8.95309731299994,15.2,-5.39304647600002));
#179747=CARTESIAN_POINT('Ctrl Pts',(8.95309731299994,11.6,-5.39304647600002));
#179748=CARTESIAN_POINT('Ctrl Pts',(8.95446135299995,15.2,-5.39361196400002));
#179749=CARTESIAN_POINT('Ctrl Pts',(8.95446135299995,11.6,-5.39361196400002));
#179750=CARTESIAN_POINT('Ctrl Pts',(8.95583345699994,15.2,-5.39417926600001));
#179751=CARTESIAN_POINT('Ctrl Pts',(8.95583345699994,11.6,-5.39417926600001));
#179752=CARTESIAN_POINT('Ctrl Pts',(8.95721361099995,15.2,-5.39474836400001));
#179753=CARTESIAN_POINT('Ctrl Pts',(8.95721361099995,11.6,-5.39474836400001));
#179754=CARTESIAN_POINT('Ctrl Pts',(8.95860180399995,15.2,-5.39531923500002));
#179755=CARTESIAN_POINT('Ctrl Pts',(8.95860180399995,11.6,-5.39531923500002));
#179756=CARTESIAN_POINT('Ctrl Pts',(8.95999802099994,15.2,-5.39589185900001));
#179757=CARTESIAN_POINT('Ctrl Pts',(8.95999802099994,11.6,-5.39589185900001));
#179758=CARTESIAN_POINT('Ctrl Pts',(8.96140224899994,15.2,-5.39646621400002));
#179759=CARTESIAN_POINT('Ctrl Pts',(8.96140224899994,11.6,-5.39646621400002));
#179760=CARTESIAN_POINT('Ctrl Pts',(8.96281447699995,15.2,-5.39704228300002));
#179761=CARTESIAN_POINT('Ctrl Pts',(8.96281447699995,11.6,-5.39704228300002));
#179762=CARTESIAN_POINT('Ctrl Pts',(8.96423468899994,15.2,-5.39762004300002));
#179763=CARTESIAN_POINT('Ctrl Pts',(8.96423468899994,11.6,-5.39762004300002));
#179764=CARTESIAN_POINT('Ctrl Pts',(8.96566287699994,15.2,-5.39819947400002));
#179765=CARTESIAN_POINT('Ctrl Pts',(8.96566287699994,11.6,-5.39819947400002));
#179766=CARTESIAN_POINT('Ctrl Pts',(8.96709902399994,15.2,-5.39878055600001));
#179767=CARTESIAN_POINT('Ctrl Pts',(8.96709902399994,11.6,-5.39878055600001));
#179768=CARTESIAN_POINT('Ctrl Pts',(8.96854311899994,15.2,-5.39936326900001));
#179769=CARTESIAN_POINT('Ctrl Pts',(8.96854311899994,11.6,-5.39936326900001));
#179770=CARTESIAN_POINT('Ctrl Pts',(8.96999514999994,15.2,-5.39994759300002));
#179771=CARTESIAN_POINT('Ctrl Pts',(8.96999514999994,11.6,-5.39994759300002));
#179772=CARTESIAN_POINT('Ctrl Pts',(8.97145510299995,15.2,-5.40053350700001));
#179773=CARTESIAN_POINT('Ctrl Pts',(8.97145510299995,11.6,-5.40053350700001));
#179774=CARTESIAN_POINT('Ctrl Pts',(8.97292296699994,15.2,-5.40112099200002));
#179775=CARTESIAN_POINT('Ctrl Pts',(8.97292296699994,11.6,-5.40112099200002));
#179776=CARTESIAN_POINT('Ctrl Pts',(8.97439872899995,15.2,-5.40171002900002));
#179777=CARTESIAN_POINT('Ctrl Pts',(8.97439872899995,11.6,-5.40171002900002));
#179778=CARTESIAN_POINT('Ctrl Pts',(8.97588237599994,15.2,-5.40230059700002));
#179779=CARTESIAN_POINT('Ctrl Pts',(8.97588237599994,11.6,-5.40230059700002));
#179780=CARTESIAN_POINT('Ctrl Pts',(8.97737389499994,15.2,-5.40289267700001));
#179781=CARTESIAN_POINT('Ctrl Pts',(8.97737389499994,11.6,-5.40289267700001));
#179782=CARTESIAN_POINT('Ctrl Pts',(8.97887327499994,15.2,-5.40348624900002));
#179783=CARTESIAN_POINT('Ctrl Pts',(8.97887327499994,11.6,-5.40348624900002));
#179784=CARTESIAN_POINT('Ctrl Pts',(8.98038050299995,15.2,-5.40408129400001));
#179785=CARTESIAN_POINT('Ctrl Pts',(8.98038050299995,11.6,-5.40408129400001));
#179786=CARTESIAN_POINT('Ctrl Pts',(8.98189556799995,15.2,-5.40467779100001));
#179787=CARTESIAN_POINT('Ctrl Pts',(8.98189556799995,11.6,-5.40467779100001));
#179788=CARTESIAN_POINT('Ctrl Pts',(8.98341845499995,15.2,-5.40527572300002));
#179789=CARTESIAN_POINT('Ctrl Pts',(8.98341845499995,11.6,-5.40527572300002));
#179790=CARTESIAN_POINT('Ctrl Pts',(8.98494915299995,15.2,-5.40587507000001));
#179791=CARTESIAN_POINT('Ctrl Pts',(8.98494915299995,11.6,-5.40587507000001));
#179792=CARTESIAN_POINT('Ctrl Pts',(8.98648765099994,15.2,-5.40647581200002));
#179793=CARTESIAN_POINT('Ctrl Pts',(8.98648765099994,11.6,-5.40647581200002));
#179794=CARTESIAN_POINT('Ctrl Pts',(8.98803393599995,15.2,-5.40707793100001));
#179795=CARTESIAN_POINT('Ctrl Pts',(8.98803393599995,11.6,-5.40707793100001));
#179796=CARTESIAN_POINT('Ctrl Pts',(8.98958799499994,15.2,-5.40768140800001));
#179797=CARTESIAN_POINT('Ctrl Pts',(8.98958799499994,11.6,-5.40768140800001));
#179798=CARTESIAN_POINT('Ctrl Pts',(8.99114981699995,15.2,-5.40828622400001));
#179799=CARTESIAN_POINT('Ctrl Pts',(8.99114981699995,11.6,-5.40828622400001));
#179800=CARTESIAN_POINT('Ctrl Pts',(8.99271938899994,15.2,-5.40889235900002));
#179801=CARTESIAN_POINT('Ctrl Pts',(8.99271938899994,11.6,-5.40889235900002));
#179802=CARTESIAN_POINT('Ctrl Pts',(8.99429670099994,15.2,-5.40949979500001));
#179803=CARTESIAN_POINT('Ctrl Pts',(8.99429670099994,11.6,-5.40949979500001));
#179804=CARTESIAN_POINT('Ctrl Pts',(8.99588173899994,15.2,-5.41010851400001));
#179805=CARTESIAN_POINT('Ctrl Pts',(8.99588173899994,11.6,-5.41010851400001));
#179806=CARTESIAN_POINT('Ctrl Pts',(8.99747449099995,15.2,-5.41071849700002));
#179807=CARTESIAN_POINT('Ctrl Pts',(8.99747449099995,11.6,-5.41071849700002));
#179808=CARTESIAN_POINT('Ctrl Pts',(8.99907494499995,15.2,-5.41132972500002));
#179809=CARTESIAN_POINT('Ctrl Pts',(8.99907494499995,11.6,-5.41132972500002));
#179810=CARTESIAN_POINT('Ctrl Pts',(9.00068308999994,15.2,-5.41194218000001));
#179811=CARTESIAN_POINT('Ctrl Pts',(9.00068308999994,11.6,-5.41194218000001));
#179812=CARTESIAN_POINT('Ctrl Pts',(9.00229891499994,15.2,-5.41255584400002));
#179813=CARTESIAN_POINT('Ctrl Pts',(9.00229891499994,11.6,-5.41255584400002));
#179814=CARTESIAN_POINT('Ctrl Pts',(9.00392240699994,15.2,-5.41317069800002));
#179815=CARTESIAN_POINT('Ctrl Pts',(9.00392240699994,11.6,-5.41317069800002));
#179816=CARTESIAN_POINT('Ctrl Pts',(9.00555355399994,15.2,-5.41378672400001));
#179817=CARTESIAN_POINT('Ctrl Pts',(9.00555355399994,11.6,-5.41378672400001));
#179818=CARTESIAN_POINT('Ctrl Pts',(9.00719234299994,15.2,-5.41440390400002));
#179819=CARTESIAN_POINT('Ctrl Pts',(9.00719234299994,11.6,-5.41440390400002));
#179820=CARTESIAN_POINT('Ctrl Pts',(9.00883876599995,15.2,-5.41502222000001));
#179821=CARTESIAN_POINT('Ctrl Pts',(9.00883876599995,11.6,-5.41502222000001));
#179822=CARTESIAN_POINT('Ctrl Pts',(9.01049280799995,15.2,-5.41564165400001));
#179823=CARTESIAN_POINT('Ctrl Pts',(9.01049280799995,11.6,-5.41564165400001));
#179824=CARTESIAN_POINT('Ctrl Pts',(9.01215445899994,15.2,-5.41626218700001));
#179825=CARTESIAN_POINT('Ctrl Pts',(9.01215445899994,11.6,-5.41626218700001));
#179826=CARTESIAN_POINT('Ctrl Pts',(9.01382370599995,15.2,-5.41688380300001));
#179827=CARTESIAN_POINT('Ctrl Pts',(9.01382370599995,11.6,-5.41688380300001));
#179828=CARTESIAN_POINT('Ctrl Pts',(9.01550053899994,15.2,-5.41750648300001));
#179829=CARTESIAN_POINT('Ctrl Pts',(9.01550053899994,11.6,-5.41750648300001));
#179830=CARTESIAN_POINT('Ctrl Pts',(9.01718494499994,15.2,-5.41813021000001));
#179831=CARTESIAN_POINT('Ctrl Pts',(9.01718494499994,11.6,-5.41813021000001));
#179832=CARTESIAN_POINT('Ctrl Pts',(9.01887691299994,15.2,-5.41875496600001));
#179833=CARTESIAN_POINT('Ctrl Pts',(9.01887691299994,11.6,-5.41875496600001));
#179834=CARTESIAN_POINT('Ctrl Pts',(9.02057643199995,15.2,-5.41938073300001));
#179835=CARTESIAN_POINT('Ctrl Pts',(9.02057643199995,11.6,-5.41938073300001));
#179836=CARTESIAN_POINT('Ctrl Pts',(9.02228348999994,15.2,-5.42000749500001));
#179837=CARTESIAN_POINT('Ctrl Pts',(9.02228348999994,11.6,-5.42000749500001));
#179838=CARTESIAN_POINT('Ctrl Pts',(9.02399807499994,15.2,-5.42063523200001));
#179839=CARTESIAN_POINT('Ctrl Pts',(9.02399807499994,11.6,-5.42063523200001));
#179840=CARTESIAN_POINT('Ctrl Pts',(9.02572017699995,15.2,-5.42126392800002));
#179841=CARTESIAN_POINT('Ctrl Pts',(9.02572017699995,11.6,-5.42126392800002));
#179842=CARTESIAN_POINT('Ctrl Pts',(9.02744978399994,15.2,-5.42189356800002));
#179843=CARTESIAN_POINT('Ctrl Pts',(9.02744978399994,11.6,-5.42189356800002));
#179844=CARTESIAN_POINT('Ctrl Pts',(9.02918688399994,15.2,-5.42252413100002));
#179845=CARTESIAN_POINT('Ctrl Pts',(9.02918688399994,11.6,-5.42252413100002));
#179846=CARTESIAN_POINT('Ctrl Pts',(9.03093146599995,15.2,-5.42315560300001));
#179847=CARTESIAN_POINT('Ctrl Pts',(9.03093146599995,11.6,-5.42315560300001));
#179848=CARTESIAN_POINT('Ctrl Pts',(9.03268351899994,15.2,-5.42378796400001));
#179849=CARTESIAN_POINT('Ctrl Pts',(9.03268351899994,11.6,-5.42378796400001));
#179850=CARTESIAN_POINT('Ctrl Pts',(9.03444303299995,15.2,-5.42442119900001));
#179851=CARTESIAN_POINT('Ctrl Pts',(9.03444303299995,11.6,-5.42442119900001));
#179852=CARTESIAN_POINT('Ctrl Pts',(9.03620999399994,15.2,-5.42505529000001));
#179853=CARTESIAN_POINT('Ctrl Pts',(9.03620999399994,11.6,-5.42505529000001));
#179854=CARTESIAN_POINT('Ctrl Pts',(9.03798439199995,15.2,-5.42569022100002));
#179855=CARTESIAN_POINT('Ctrl Pts',(9.03798439199995,11.6,-5.42569022100002));
#179856=CARTESIAN_POINT('Ctrl Pts',(9.03976621699995,15.2,-5.42632597500001));
#179857=CARTESIAN_POINT('Ctrl Pts',(9.03976621699995,11.6,-5.42632597500001));
#179858=CARTESIAN_POINT('Ctrl Pts',(9.04155545599994,15.2,-5.42696253500001));
#179859=CARTESIAN_POINT('Ctrl Pts',(9.04155545599994,11.6,-5.42696253500001));
#179860=CARTESIAN_POINT('Ctrl Pts',(9.04335209899994,15.2,-5.42759988400002));
#179861=CARTESIAN_POINT('Ctrl Pts',(9.04335209899994,11.6,-5.42759988400002));
#179862=CARTESIAN_POINT('Ctrl Pts',(9.04515613499994,15.2,-5.42823800600001));
#179863=CARTESIAN_POINT('Ctrl Pts',(9.04515613499994,11.6,-5.42823800600001));
#179864=CARTESIAN_POINT('Ctrl Pts',(9.04696755199994,15.2,-5.42887688500001));
#179865=CARTESIAN_POINT('Ctrl Pts',(9.04696755199994,11.6,-5.42887688500001));
#179866=CARTESIAN_POINT('Ctrl Pts',(9.04878633899994,15.2,-5.42951650200001));
#179867=CARTESIAN_POINT('Ctrl Pts',(9.04878633899994,11.6,-5.42951650200001));
#179868=CARTESIAN_POINT('Ctrl Pts',(9.05061248799995,15.2,-5.43015684400002));
#179869=CARTESIAN_POINT('Ctrl Pts',(9.05061248799995,11.6,-5.43015684400002));
#179870=CARTESIAN_POINT('Ctrl Pts',(9.05244598299995,15.2,-5.43079789200001));
#179871=CARTESIAN_POINT('Ctrl Pts',(9.05244598299995,11.6,-5.43079789200001));
#179872=CARTESIAN_POINT('Ctrl Pts',(9.05428681799994,15.2,-5.43143963100002));
#179873=CARTESIAN_POINT('Ctrl Pts',(9.05428681799994,11.6,-5.43143963100002));
#179874=CARTESIAN_POINT('Ctrl Pts',(9.05613497799994,15.2,-5.43208204400001));
#179875=CARTESIAN_POINT('Ctrl Pts',(9.05613497799994,11.6,-5.43208204400001));
#179876=CARTESIAN_POINT('Ctrl Pts',(9.05799045399995,15.2,-5.43272511600001));
#179877=CARTESIAN_POINT('Ctrl Pts',(9.05799045399995,11.6,-5.43272511600001));
#179878=CARTESIAN_POINT('Ctrl Pts',(9.05985323499995,15.2,-5.43336883000002));
#179879=CARTESIAN_POINT('Ctrl Pts',(9.05985323499995,11.6,-5.43336883000002));
#179880=CARTESIAN_POINT('Ctrl Pts',(9.06172330999994,15.2,-5.43401316900002));
#179881=CARTESIAN_POINT('Ctrl Pts',(9.06172330999994,11.6,-5.43401316900002));
#179882=CARTESIAN_POINT('Ctrl Pts',(9.06360066799994,15.2,-5.43465811900001));
#179883=CARTESIAN_POINT('Ctrl Pts',(9.06360066799994,11.6,-5.43465811900001));
#179884=CARTESIAN_POINT('Ctrl Pts',(9.06548529999995,15.2,-5.43530366300002));
#179885=CARTESIAN_POINT('Ctrl Pts',(9.06548529999995,11.6,-5.43530366300002));
#179886=CARTESIAN_POINT('Ctrl Pts',(9.06737719299995,15.2,-5.43594978600002));
#179887=CARTESIAN_POINT('Ctrl Pts',(9.06737719299995,11.6,-5.43594978600002));
#179888=CARTESIAN_POINT('Ctrl Pts',(9.06927633599994,15.2,-5.43659647000001));
#179889=CARTESIAN_POINT('Ctrl Pts',(9.06927633599994,11.6,-5.43659647000001));
#179890=CARTESIAN_POINT('Ctrl Pts',(9.07118271999994,15.2,-5.43724370100001));
#179891=CARTESIAN_POINT('Ctrl Pts',(9.07118271999994,11.6,-5.43724370100001));
#179892=CARTESIAN_POINT('Ctrl Pts',(9.07309633399995,15.2,-5.43789146400002));
#179893=CARTESIAN_POINT('Ctrl Pts',(9.07309633399995,11.6,-5.43789146400002));
#179894=CARTESIAN_POINT('Ctrl Pts',(9.07501716599995,15.2,-5.43853974100001));
#179895=CARTESIAN_POINT('Ctrl Pts',(9.07501716599995,11.6,-5.43853974100001));
#179896=CARTESIAN_POINT('Ctrl Pts',(9.07694520799994,15.2,-5.43918851900001));
#179897=CARTESIAN_POINT('Ctrl Pts',(9.07694520799994,11.6,-5.43918851900001));
#179898=CARTESIAN_POINT('Ctrl Pts',(9.07888044599994,15.2,-5.43983778100001));
#179899=CARTESIAN_POINT('Ctrl Pts',(9.07888044599994,11.6,-5.43983778100001));
#179900=CARTESIAN_POINT('Ctrl Pts',(9.08082287199995,15.2,-5.44048751200001));
#179901=CARTESIAN_POINT('Ctrl Pts',(9.08082287199995,11.6,-5.44048751200001));
#179902=CARTESIAN_POINT('Ctrl Pts',(9.08277247299995,15.2,-5.44113769600001));
#179903=CARTESIAN_POINT('Ctrl Pts',(9.08277247299995,11.6,-5.44113769600001));
#179904=CARTESIAN_POINT('Ctrl Pts',(9.08472924199994,15.2,-5.44178831900001));
#179905=CARTESIAN_POINT('Ctrl Pts',(9.08472924199994,11.6,-5.44178831900001));
#179906=CARTESIAN_POINT('Ctrl Pts',(9.08669316599994,15.2,-5.44243936400001));
#179907=CARTESIAN_POINT('Ctrl Pts',(9.08669316599994,11.6,-5.44243936400001));
#179908=CARTESIAN_POINT('Ctrl Pts',(9.08866423499994,15.2,-5.44309081600002));
#179909=CARTESIAN_POINT('Ctrl Pts',(9.08866423499994,11.6,-5.44309081600002));
#179910=CARTESIAN_POINT('Ctrl Pts',(9.09064243799994,15.2,-5.44374266200002));
#179911=CARTESIAN_POINT('Ctrl Pts',(9.09064243799994,11.6,-5.44374266200002));
#179912=CARTESIAN_POINT('Ctrl Pts',(9.09262776499994,15.2,-5.44439488400001));
#179913=CARTESIAN_POINT('Ctrl Pts',(9.09262776499994,11.6,-5.44439488400001));
#179914=CARTESIAN_POINT('Ctrl Pts',(9.09462020699995,15.2,-5.44504747000001));
#179915=CARTESIAN_POINT('Ctrl Pts',(9.09462020699995,11.6,-5.44504747000001));
#179916=CARTESIAN_POINT('Ctrl Pts',(9.09661975099995,15.2,-5.44570040100002));
#179917=CARTESIAN_POINT('Ctrl Pts',(9.09661975099995,11.6,-5.44570040100002));
#179918=CARTESIAN_POINT('Ctrl Pts',(9.09862638799994,15.2,-5.44635366600001));
#179919=CARTESIAN_POINT('Ctrl Pts',(9.09862638799994,11.6,-5.44635366600001));
#179920=CARTESIAN_POINT('Ctrl Pts',(9.10064010799994,15.2,-5.44700724700002));
#179921=CARTESIAN_POINT('Ctrl Pts',(9.10064010799994,11.6,-5.44700724700002));
#179922=CARTESIAN_POINT('Ctrl Pts',(9.10266090099995,15.2,-5.44766113100001));
#179923=CARTESIAN_POINT('Ctrl Pts',(9.10266090099995,11.6,-5.44766113100001));
#179924=CARTESIAN_POINT('Ctrl Pts',(9.10468875499994,15.2,-5.44831530400002));
#179925=CARTESIAN_POINT('Ctrl Pts',(9.10468875499994,11.6,-5.44831530400002));
#179926=CARTESIAN_POINT('Ctrl Pts',(9.10672366199995,15.2,-5.44896974900002));
#179927=CARTESIAN_POINT('Ctrl Pts',(9.10672366199995,11.6,-5.44896974900002));
#179928=CARTESIAN_POINT('Ctrl Pts',(9.10876560899995,15.2,-5.44962445200001));
#179929=CARTESIAN_POINT('Ctrl Pts',(9.10876560899995,11.6,-5.44962445200001));
#179930=CARTESIAN_POINT('Ctrl Pts',(9.11081458899995,15.2,-5.45027940000002));
#179931=CARTESIAN_POINT('Ctrl Pts',(9.11081458899995,11.6,-5.45027940000002));
#179932=CARTESIAN_POINT('Ctrl Pts',(9.11287058799994,15.2,-5.45093457500001));
#179933=CARTESIAN_POINT('Ctrl Pts',(9.11287058799994,11.6,-5.45093457500001));
#179934=CARTESIAN_POINT('Ctrl Pts',(9.11493359899995,15.2,-5.45158996700001));
#179935=CARTESIAN_POINT('Ctrl Pts',(9.11493359899995,11.6,-5.45158996700001));
#179936=CARTESIAN_POINT('Ctrl Pts',(9.11700361099994,15.2,-5.45224555800001));
#179937=CARTESIAN_POINT('Ctrl Pts',(9.11700361099994,11.6,-5.45224555800001));
#179938=CARTESIAN_POINT('Ctrl Pts',(9.11908061299994,15.2,-5.45290133500002));
#179939=CARTESIAN_POINT('Ctrl Pts',(9.11908061299994,11.6,-5.45290133500002));
#179940=CARTESIAN_POINT('Ctrl Pts',(9.12116459599994,15.2,-5.45355728300001));
#179941=CARTESIAN_POINT('Ctrl Pts',(9.12116459599994,11.6,-5.45355728300001));
#179942=CARTESIAN_POINT('Ctrl Pts',(9.12325554899994,15.2,-5.45421338800002));
#179943=CARTESIAN_POINT('Ctrl Pts',(9.12325554899994,11.6,-5.45421338800002));
#179944=CARTESIAN_POINT('Ctrl Pts',(9.12535346199994,15.2,-5.45486963700001));
#179945=CARTESIAN_POINT('Ctrl Pts',(9.12535346199994,11.6,-5.45486963700001));
#179946=CARTESIAN_POINT('Ctrl Pts',(9.12745832599994,15.2,-5.45552601400002));
#179947=CARTESIAN_POINT('Ctrl Pts',(9.12745832599994,11.6,-5.45552601400002));
#179948=CARTESIAN_POINT('Ctrl Pts',(9.12957012999994,15.2,-5.45618250500001));
#179949=CARTESIAN_POINT('Ctrl Pts',(9.12957012999994,11.6,-5.45618250500001));
#179950=CARTESIAN_POINT('Ctrl Pts',(9.13168886399994,15.2,-5.45683909600001));
#179951=CARTESIAN_POINT('Ctrl Pts',(9.13168886399994,11.6,-5.45683909600001));
#179952=CARTESIAN_POINT('Ctrl Pts',(9.13381451899994,15.2,-5.45749577400001));
#179953=CARTESIAN_POINT('Ctrl Pts',(9.13381451899994,11.6,-5.45749577400001));
#179954=CARTESIAN_POINT('Ctrl Pts',(9.13594708299994,15.2,-5.45815252500002));
#179955=CARTESIAN_POINT('Ctrl Pts',(9.13594708299994,11.6,-5.45815252500002));
#179956=CARTESIAN_POINT('Ctrl Pts',(9.13808654799994,15.2,-5.45880933300001));
#179957=CARTESIAN_POINT('Ctrl Pts',(9.13808654799994,11.6,-5.45880933300001));
#179958=CARTESIAN_POINT('Ctrl Pts',(9.14023290399994,15.2,-5.45946618500002));
#179959=CARTESIAN_POINT('Ctrl Pts',(9.14023290399994,11.6,-5.45946618500002));
#179960=CARTESIAN_POINT('Ctrl Pts',(9.14238613999995,15.2,-5.46012306900002));
#179961=CARTESIAN_POINT('Ctrl Pts',(9.14238613999995,11.6,-5.46012306900002));
#179962=CARTESIAN_POINT('Ctrl Pts',(9.14454624699994,15.2,-5.46077996900001));
#179963=CARTESIAN_POINT('Ctrl Pts',(9.14454624699994,11.6,-5.46077996900001));
#179964=CARTESIAN_POINT('Ctrl Pts',(9.14671321399994,15.2,-5.46143687300002));
#179965=CARTESIAN_POINT('Ctrl Pts',(9.14671321399994,11.6,-5.46143687300002));
#179966=CARTESIAN_POINT('Ctrl Pts',(9.14888703299994,15.2,-5.46209376400002));
#179967=CARTESIAN_POINT('Ctrl Pts',(9.14888703299994,11.6,-5.46209376400002));
#179968=CARTESIAN_POINT('Ctrl Pts',(9.15106769299994,15.2,-5.46275063300001));
#179969=CARTESIAN_POINT('Ctrl Pts',(9.15106769299994,11.6,-5.46275063300001));
#179970=CARTESIAN_POINT('Ctrl Pts',(9.15325518399994,15.2,-5.46340746200002));
#179971=CARTESIAN_POINT('Ctrl Pts',(9.15325518399994,11.6,-5.46340746200002));
#179972=CARTESIAN_POINT('Ctrl Pts',(9.15544949599994,15.2,-5.46406424100002));
#179973=CARTESIAN_POINT('Ctrl Pts',(9.15544949599994,11.6,-5.46406424100002));
#179974=CARTESIAN_POINT('Ctrl Pts',(9.15765062099995,15.2,-5.46472095300001));
#179975=CARTESIAN_POINT('Ctrl Pts',(9.15765062099995,11.6,-5.46472095300001));
#179976=CARTESIAN_POINT('Ctrl Pts',(9.15985854799995,15.2,-5.46537758800001));
#179977=CARTESIAN_POINT('Ctrl Pts',(9.15985854799995,11.6,-5.46537758800001));
#179978=CARTESIAN_POINT('Ctrl Pts',(9.16207326699995,15.2,-5.46603413000001));
#179979=CARTESIAN_POINT('Ctrl Pts',(9.16207326699995,11.6,-5.46603413000001));
#179980=CARTESIAN_POINT('Ctrl Pts',(9.16429476899994,15.2,-5.46669056600001));
#179981=CARTESIAN_POINT('Ctrl Pts',(9.16429476899994,11.6,-5.46669056600001));
#179982=CARTESIAN_POINT('Ctrl Pts',(9.16652304299994,15.2,-5.46734688400001));
#179983=CARTESIAN_POINT('Ctrl Pts',(9.16652304299994,11.6,-5.46734688400001));
#179984=CARTESIAN_POINT('Ctrl Pts',(9.16875808299995,15.2,-5.46800307100002));
#179985=CARTESIAN_POINT('Ctrl Pts',(9.16875808299995,11.6,-5.46800307100002));
#179986=CARTESIAN_POINT('Ctrl Pts',(9.17099987399994,15.2,-5.46865911100001));
#179987=CARTESIAN_POINT('Ctrl Pts',(9.17099987399994,11.6,-5.46865911100001));
#179988=CARTESIAN_POINT('Ctrl Pts',(9.17324840999994,15.2,-5.46931499300001));
#179989=CARTESIAN_POINT('Ctrl Pts',(9.17324840999994,11.6,-5.46931499300001));
#179990=CARTESIAN_POINT('Ctrl Pts',(9.17550368099995,15.2,-5.46997070300002));
#179991=CARTESIAN_POINT('Ctrl Pts',(9.17550368099995,11.6,-5.46997070300002));
#179992=CARTESIAN_POINT('Ctrl Pts',(9.17776567599994,15.2,-5.47062622900001));
#179993=CARTESIAN_POINT('Ctrl Pts',(9.17776567599994,11.6,-5.47062622900001));
#179994=CARTESIAN_POINT('Ctrl Pts',(9.18003438699994,15.2,-5.47128155600001));
#179995=CARTESIAN_POINT('Ctrl Pts',(9.18003438699994,11.6,-5.47128155600001));
#179996=CARTESIAN_POINT('Ctrl Pts',(9.18230980399994,15.2,-5.47193667300002));
#179997=CARTESIAN_POINT('Ctrl Pts',(9.18230980399994,11.6,-5.47193667300002));
#179998=CARTESIAN_POINT('Ctrl Pts',(9.18459191699995,15.2,-5.47259156500001));
#179999=CARTESIAN_POINT('Ctrl Pts',(9.18459191699995,11.6,-5.47259156500001));
#180000=CARTESIAN_POINT('Ctrl Pts',(9.18688071799994,15.2,-5.47324622200001));
#180001=CARTESIAN_POINT('Ctrl Pts',(9.18688071799994,11.6,-5.47324622200001));
#180002=CARTESIAN_POINT('Ctrl Pts',(9.18917619399994,15.2,-5.47390062900002));
#180003=CARTESIAN_POINT('Ctrl Pts',(9.18917619399994,11.6,-5.47390062900002));
#180004=CARTESIAN_POINT('Ctrl Pts',(9.19147833999994,15.2,-5.47455477200002));
#180005=CARTESIAN_POINT('Ctrl Pts',(9.19147833999994,11.6,-5.47455477200002));
#180006=CARTESIAN_POINT('Ctrl Pts',(9.19378714199994,15.2,-5.47520864000001));
#180007=CARTESIAN_POINT('Ctrl Pts',(9.19378714199994,11.6,-5.47520864000001));
#180008=CARTESIAN_POINT('Ctrl Pts',(9.19610259599994,15.2,-5.47586222000001));
#180009=CARTESIAN_POINT('Ctrl Pts',(9.19610259599994,11.6,-5.47586222000001));
#180010=CARTESIAN_POINT('Ctrl Pts',(9.19842468799994,15.2,-5.47651550000001));
#180011=CARTESIAN_POINT('Ctrl Pts',(9.19842468799994,11.6,-5.47651550000001));
#180012=CARTESIAN_POINT('Ctrl Pts',(9.20075340999994,15.2,-5.47716846600002));
#180013=CARTESIAN_POINT('Ctrl Pts',(9.20075340999994,11.6,-5.47716846600002));
#180014=CARTESIAN_POINT('Ctrl Pts',(9.20308875299994,15.2,-5.47782110600001));
#180015=CARTESIAN_POINT('Ctrl Pts',(9.20308875299994,11.6,-5.47782110600001));
#180016=CARTESIAN_POINT('Ctrl Pts',(9.20543070799994,15.2,-5.47847340700002));
#180017=CARTESIAN_POINT('Ctrl Pts',(9.20543070799994,11.6,-5.47847340700002));
#180018=CARTESIAN_POINT('Ctrl Pts',(9.20777926399994,15.2,-5.47912535600001));
#180019=CARTESIAN_POINT('Ctrl Pts',(9.20777926399994,11.6,-5.47912535600001));
#180020=CARTESIAN_POINT('Ctrl Pts',(9.21013441399994,15.2,-5.47977694200001));
#180021=CARTESIAN_POINT('Ctrl Pts',(9.21013441399994,11.6,-5.47977694200001));
#180022=CARTESIAN_POINT('Ctrl Pts',(9.21249614799994,15.2,-5.48042815200001));
#180023=CARTESIAN_POINT('Ctrl Pts',(9.21249614799994,11.6,-5.48042815200001));
#180024=CARTESIAN_POINT('Ctrl Pts',(9.21486445499994,15.2,-5.48107897300001));
#180025=CARTESIAN_POINT('Ctrl Pts',(9.21486445499994,11.6,-5.48107897300001));
#180026=CARTESIAN_POINT('Ctrl Pts',(9.21723932699994,15.2,-5.48172939300001));
#180027=CARTESIAN_POINT('Ctrl Pts',(9.21723932699994,11.6,-5.48172939300001));
#180028=CARTESIAN_POINT('Ctrl Pts',(9.21962075499994,15.2,-5.48237939900002));
#180029=CARTESIAN_POINT('Ctrl Pts',(9.21962075499994,11.6,-5.48237939900002));
#180030=CARTESIAN_POINT('Ctrl Pts',(9.22200872899994,15.2,-5.48302898000002));
#180031=CARTESIAN_POINT('Ctrl Pts',(9.22200872899994,11.6,-5.48302898000002));
#180032=CARTESIAN_POINT('Ctrl Pts',(9.22440324099994,15.2,-5.48367812300001));
#180033=CARTESIAN_POINT('Ctrl Pts',(9.22440324099994,11.6,-5.48367812300001));
#180034=CARTESIAN_POINT('Ctrl Pts',(9.22680427999994,15.2,-5.48432681500001));
#180035=CARTESIAN_POINT('Ctrl Pts',(9.22680427999994,11.6,-5.48432681500001));
#180036=CARTESIAN_POINT('Ctrl Pts',(9.22921183799994,15.2,-5.48497504600002));
#180037=CARTESIAN_POINT('Ctrl Pts',(9.22921183799994,11.6,-5.48497504600002));
#180038=CARTESIAN_POINT('Ctrl Pts',(9.23162590699994,15.2,-5.48562280100001));
#180039=CARTESIAN_POINT('Ctrl Pts',(9.23162590699994,11.6,-5.48562280100001));
#180040=CARTESIAN_POINT('Ctrl Pts',(9.23404647499994,15.2,-5.48627007100002));
#180041=CARTESIAN_POINT('Ctrl Pts',(9.23404647499994,11.6,-5.48627007100002));
#180042=CARTESIAN_POINT('Ctrl Pts',(9.23647353599995,15.2,-5.48691684200001));
#180043=CARTESIAN_POINT('Ctrl Pts',(9.23647353599995,11.6,-5.48691684200001));
#180044=CARTESIAN_POINT('Ctrl Pts',(9.23890707799995,15.2,-5.48756310100002));
#180045=CARTESIAN_POINT('Ctrl Pts',(9.23890707799995,11.6,-5.48756310100002));
#180046=CARTESIAN_POINT('Ctrl Pts',(9.24134709299994,15.2,-5.48820883900001));
#180047=CARTESIAN_POINT('Ctrl Pts',(9.24134709299994,11.6,-5.48820883900001));
#180048=CARTESIAN_POINT('Ctrl Pts',(9.24379357299994,15.2,-5.48885404200002));
#180049=CARTESIAN_POINT('Ctrl Pts',(9.24379357299994,11.6,-5.48885404200002));
#180050=CARTESIAN_POINT('Ctrl Pts',(9.24624650799995,15.2,-5.48949869700001));
#180051=CARTESIAN_POINT('Ctrl Pts',(9.24624650799995,11.6,-5.48949869700001));
#180052=CARTESIAN_POINT('Ctrl Pts',(9.24870588899994,15.2,-5.49014279500001));
#180053=CARTESIAN_POINT('Ctrl Pts',(9.24870588899994,11.6,-5.49014279500001));
#180054=CARTESIAN_POINT('Ctrl Pts',(9.25117170699994,15.2,-5.49078632400001));
#180055=CARTESIAN_POINT('Ctrl Pts',(9.25117170699994,11.6,-5.49078632400001));
#180056=CARTESIAN_POINT('Ctrl Pts',(9.25364395199994,15.2,-5.49142926900001));
#180057=CARTESIAN_POINT('Ctrl Pts',(9.25364395199994,11.6,-5.49142926900001));
#180058=CARTESIAN_POINT('Ctrl Pts',(9.25612261599994,15.2,-5.49207162100001));
#180059=CARTESIAN_POINT('Ctrl Pts',(9.25612261599994,11.6,-5.49207162100001));
#180060=CARTESIAN_POINT('Ctrl Pts',(9.25860768999994,15.2,-5.49271336700001));
#180061=CARTESIAN_POINT('Ctrl Pts',(9.25860768999994,11.6,-5.49271336700001));
#180062=CARTESIAN_POINT('Ctrl Pts',(9.26109916599994,15.2,-5.49335449700001));
#180063=CARTESIAN_POINT('Ctrl Pts',(9.26109916599994,11.6,-5.49335449700001));
#180064=CARTESIAN_POINT('Ctrl Pts',(9.26359703299994,15.2,-5.49399499800002));
#180065=CARTESIAN_POINT('Ctrl Pts',(9.26359703299994,11.6,-5.49399499800002));
#180066=CARTESIAN_POINT('Ctrl Pts',(9.26610128399994,15.2,-5.49463485800001));
#180067=CARTESIAN_POINT('Ctrl Pts',(9.26610128399994,11.6,-5.49463485800001));
#180068=CARTESIAN_POINT('Ctrl Pts',(9.26861190799994,15.2,-5.49527406700001));
#180069=CARTESIAN_POINT('Ctrl Pts',(9.26861190799994,11.6,-5.49527406700001));
#180070=CARTESIAN_POINT('Ctrl Pts',(9.27112889699995,15.2,-5.49591261200002));
#180071=CARTESIAN_POINT('Ctrl Pts',(9.27112889699995,11.6,-5.49591261200002));
#180072=CARTESIAN_POINT('Ctrl Pts',(9.27365224399994,15.2,-5.49655048200002));
#180073=CARTESIAN_POINT('Ctrl Pts',(9.27365224399994,11.6,-5.49655048200002));
#180074=CARTESIAN_POINT('Ctrl Pts',(9.27618193699994,15.2,-5.49718766700002));
#180075=CARTESIAN_POINT('Ctrl Pts',(9.27618193699994,11.6,-5.49718766700002));
#180076=CARTESIAN_POINT('Ctrl Pts',(9.27871796999994,15.2,-5.49782415300001));
#180077=CARTESIAN_POINT('Ctrl Pts',(9.27871796999994,11.6,-5.49782415300001));
#180078=CARTESIAN_POINT('Ctrl Pts',(9.28126033199994,15.2,-5.49845993000002));
#180079=CARTESIAN_POINT('Ctrl Pts',(9.28126033199994,11.6,-5.49845993000002));
#180080=CARTESIAN_POINT('Ctrl Pts',(9.28380901399994,15.2,-5.49909498700002));
#180081=CARTESIAN_POINT('Ctrl Pts',(9.28380901399994,11.6,-5.49909498700002));
#180082=CARTESIAN_POINT('Ctrl Pts',(9.28636400899994,15.2,-5.49972931200001));
#180083=CARTESIAN_POINT('Ctrl Pts',(9.28636400899994,11.6,-5.49972931200001));
#180084=CARTESIAN_POINT('Ctrl Pts',(9.28892530699994,15.2,-5.50036289400001));
#180085=CARTESIAN_POINT('Ctrl Pts',(9.28892530699994,11.6,-5.50036289400001));
#180086=CARTESIAN_POINT('Ctrl Pts',(9.29149290099994,15.2,-5.50099572100001));
#180087=CARTESIAN_POINT('Ctrl Pts',(9.29149290099994,11.6,-5.50099572100001));
#180088=CARTESIAN_POINT('Ctrl Pts',(9.29406677899994,15.2,-5.50162778400002));
#180089=CARTESIAN_POINT('Ctrl Pts',(9.29406677899994,11.6,-5.50162778400002));
#180090=CARTESIAN_POINT('Ctrl Pts',(9.29664693399994,15.2,-5.50225906900002));
#180091=CARTESIAN_POINT('Ctrl Pts',(9.29664693399994,11.6,-5.50225906900002));
#180092=CARTESIAN_POINT('Ctrl Pts',(9.29923335799995,15.2,-5.50288956800001));
#180093=CARTESIAN_POINT('Ctrl Pts',(9.29923335799995,11.6,-5.50288956800001));
#180094=CARTESIAN_POINT('Ctrl Pts',(9.30182604099994,15.2,-5.50351926600001));
#180095=CARTESIAN_POINT('Ctrl Pts',(9.30182604099994,11.6,-5.50351926600001));
#180096=CARTESIAN_POINT('Ctrl Pts',(9.30442497499994,15.2,-5.50414815500002));
#180097=CARTESIAN_POINT('Ctrl Pts',(9.30442497499994,11.6,-5.50414815500002));
#180098=CARTESIAN_POINT('Ctrl Pts',(9.30703015099994,15.2,-5.50477622400001));
#180099=CARTESIAN_POINT('Ctrl Pts',(9.30703015099994,11.6,-5.50477622400001));
#180100=CARTESIAN_POINT('Ctrl Pts',(9.30964155999994,15.2,-5.50540346000002));
#180101=CARTESIAN_POINT('Ctrl Pts',(9.30964155999994,11.6,-5.50540346000002));
#180102=CARTESIAN_POINT('Ctrl Pts',(9.31225919399994,15.2,-5.50602985400001));
#180103=CARTESIAN_POINT('Ctrl Pts',(9.31225919399994,11.6,-5.50602985400001));
#180104=CARTESIAN_POINT('Ctrl Pts',(9.31488304399995,15.2,-5.50665539400002));
#180105=CARTESIAN_POINT('Ctrl Pts',(9.31488304399995,11.6,-5.50665539400002));
#180106=CARTESIAN_POINT('Ctrl Pts',(9.31751310199994,15.2,-5.50728006800002));
#180107=CARTESIAN_POINT('Ctrl Pts',(9.31751310199994,11.6,-5.50728006800002));
#180108=CARTESIAN_POINT('Ctrl Pts',(9.32014935799995,15.2,-5.50790386900001));
#180109=CARTESIAN_POINT('Ctrl Pts',(9.32014935799995,11.6,-5.50790386900001));
#180110=CARTESIAN_POINT('Ctrl Pts',(9.32279180499994,15.2,-5.50852678200001));
#180111=CARTESIAN_POINT('Ctrl Pts',(9.32279180499994,11.6,-5.50852678200001));
#180112=CARTESIAN_POINT('Ctrl Pts',(9.32544043299995,15.2,-5.50914879900001));
#180113=CARTESIAN_POINT('Ctrl Pts',(9.32544043299995,11.6,-5.50914879900001));
#180114=CARTESIAN_POINT('Ctrl Pts',(9.32809523399994,15.2,-5.50976990700002));
#180115=CARTESIAN_POINT('Ctrl Pts',(9.32809523399994,11.6,-5.50976990700002));
#180116=CARTESIAN_POINT('Ctrl Pts',(9.33075619899994,15.2,-5.51039009700002));
#180117=CARTESIAN_POINT('Ctrl Pts',(9.33075619899994,11.6,-5.51039009700002));
#180118=CARTESIAN_POINT('Ctrl Pts',(9.33342332099994,15.2,-5.51100935800001));
#180119=CARTESIAN_POINT('Ctrl Pts',(9.33342332099994,11.6,-5.51100935800001));
#180120=CARTESIAN_POINT('Ctrl Pts',(9.33609658899995,15.2,-5.51162767900002));
#180121=CARTESIAN_POINT('Ctrl Pts',(9.33609658899995,11.6,-5.51162767900002));
#180122=CARTESIAN_POINT('Ctrl Pts',(9.33877599599995,15.2,-5.51224504900001));
#180123=CARTESIAN_POINT('Ctrl Pts',(9.33877599599995,11.6,-5.51224504900001));
#180124=CARTESIAN_POINT('Ctrl Pts',(9.34146153499994,15.2,-5.51286145900002));
#180125=CARTESIAN_POINT('Ctrl Pts',(9.34146153499994,11.6,-5.51286145900002));
#180126=CARTESIAN_POINT('Ctrl Pts',(9.34415319399994,15.2,-5.51347689700001));
#180127=CARTESIAN_POINT('Ctrl Pts',(9.34415319399994,11.6,-5.51347689700001));
#180128=CARTESIAN_POINT('Ctrl Pts',(9.34685096599994,15.2,-5.51409135300001));
#180129=CARTESIAN_POINT('Ctrl Pts',(9.34685096599994,11.6,-5.51409135300001));
#180130=CARTESIAN_POINT('Ctrl Pts',(9.34955484399994,15.2,-5.51470481500001));
#180131=CARTESIAN_POINT('Ctrl Pts',(9.34955484399994,11.6,-5.51470481500001));
#180132=CARTESIAN_POINT('Ctrl Pts',(9.35226481699994,15.2,-5.51531727600001));
#180133=CARTESIAN_POINT('Ctrl Pts',(9.35226481699994,11.6,-5.51531727600001));
#180134=CARTESIAN_POINT('Ctrl Pts',(9.35498087799994,15.2,-5.51592872200001));
#180135=CARTESIAN_POINT('Ctrl Pts',(9.35498087799994,11.6,-5.51592872200001));
#180136=CARTESIAN_POINT('Ctrl Pts',(9.35770301899994,15.2,-5.51653914500001));
#180137=CARTESIAN_POINT('Ctrl Pts',(9.35770301899994,11.6,-5.51653914500001));
#180138=CARTESIAN_POINT('Ctrl Pts',(9.36043123099994,15.2,-5.51714853300002));
#180139=CARTESIAN_POINT('Ctrl Pts',(9.36043123099994,11.6,-5.51714853300002));
#180140=CARTESIAN_POINT('Ctrl Pts',(9.36316550599994,15.2,-5.51775687700002));
#180141=CARTESIAN_POINT('Ctrl Pts',(9.36316550599994,11.6,-5.51775687700002));
#180142=CARTESIAN_POINT('Ctrl Pts',(9.36590583399994,15.2,-5.51836416600001));
#180143=CARTESIAN_POINT('Ctrl Pts',(9.36590583399994,11.6,-5.51836416600001));
#180144=CARTESIAN_POINT('Ctrl Pts',(9.36865220799995,15.2,-5.51897039100002));
#180145=CARTESIAN_POINT('Ctrl Pts',(9.36865220799995,11.6,-5.51897039100002));
#180146=CARTESIAN_POINT('Ctrl Pts',(9.37140461999994,15.2,-5.51957553900001));
#180147=CARTESIAN_POINT('Ctrl Pts',(9.37140461999994,11.6,-5.51957553900001));
#180148=CARTESIAN_POINT('Ctrl Pts',(9.37416306099994,15.2,-5.52017960100001));
#180149=CARTESIAN_POINT('Ctrl Pts',(9.37416306099994,11.6,-5.52017960100001));
#180150=CARTESIAN_POINT('Ctrl Pts',(9.37692752299995,15.2,-5.52078256900002));
#180151=CARTESIAN_POINT('Ctrl Pts',(9.37692752299995,11.6,-5.52078256900002));
#180152=CARTESIAN_POINT('Ctrl Pts',(9.37969799599994,15.2,-5.52138443100001));
#180153=CARTESIAN_POINT('Ctrl Pts',(9.37969799599994,11.6,-5.52138443100001));
#180154=CARTESIAN_POINT('Ctrl Pts',(9.38247447299995,15.2,-5.52198517600001));
#180155=CARTESIAN_POINT('Ctrl Pts',(9.38247447299995,11.6,-5.52198517600001));
#180156=CARTESIAN_POINT('Ctrl Pts',(9.38525694699995,15.2,-5.52258479600002));
#180157=CARTESIAN_POINT('Ctrl Pts',(9.38525694699995,11.6,-5.52258479600002));
#180158=CARTESIAN_POINT('Ctrl Pts',(9.38804540799994,15.2,-5.52318328000001));
#180159=CARTESIAN_POINT('Ctrl Pts',(9.38804540799994,11.6,-5.52318328000001));
#180160=CARTESIAN_POINT('Ctrl Pts',(9.39083984799994,15.2,-5.52378061700002));
#180161=CARTESIAN_POINT('Ctrl Pts',(9.39083984799994,11.6,-5.52378061700002));
#180162=CARTESIAN_POINT('Ctrl Pts',(9.39364025899994,15.2,-5.52437679800001));
#180163=CARTESIAN_POINT('Ctrl Pts',(9.39364025899994,11.6,-5.52437679800001));
#180164=CARTESIAN_POINT('Ctrl Pts',(9.39644663199994,15.2,-5.52497181400001));
#180165=CARTESIAN_POINT('Ctrl Pts',(9.39644663199994,11.6,-5.52497181400001));
#180166=CARTESIAN_POINT('Ctrl Pts',(9.39925895999994,15.2,-5.52556565300002));
#180167=CARTESIAN_POINT('Ctrl Pts',(9.39925895999994,11.6,-5.52556565300002));
#180168=CARTESIAN_POINT('Ctrl Pts',(9.40207723299994,15.2,-5.52615830700002));
#180169=CARTESIAN_POINT('Ctrl Pts',(9.40207723299994,11.6,-5.52615830700002));
#180170=CARTESIAN_POINT('Ctrl Pts',(9.40490144599995,15.2,-5.52674976500001));
#180171=CARTESIAN_POINT('Ctrl Pts',(9.40490144599995,11.6,-5.52674976500001));
#180172=CARTESIAN_POINT('Ctrl Pts',(9.40773158599994,15.2,-5.52734001800002));
#180173=CARTESIAN_POINT('Ctrl Pts',(9.40773158599994,11.6,-5.52734001800002));
#180174=CARTESIAN_POINT('Ctrl Pts',(9.41056764899994,15.2,-5.52792905400001));
#180175=CARTESIAN_POINT('Ctrl Pts',(9.41056764899994,11.6,-5.52792905400001));
#180176=CARTESIAN_POINT('Ctrl Pts',(9.41340962499994,15.2,-5.52851686700001));
#180177=CARTESIAN_POINT('Ctrl Pts',(9.41340962499994,11.6,-5.52851686700001));
#180178=CARTESIAN_POINT('Ctrl Pts',(9.41625750599994,15.2,-5.52910344300001));
#180179=CARTESIAN_POINT('Ctrl Pts',(9.41625750599994,11.6,-5.52910344300001));
#180180=CARTESIAN_POINT('Ctrl Pts',(9.41911128299994,15.2,-5.52968877500001));
#180181=CARTESIAN_POINT('Ctrl Pts',(9.41911128299994,11.6,-5.52968877500001));
#180182=CARTESIAN_POINT('Ctrl Pts',(9.42197095099995,15.2,-5.53027285400002));
#180183=CARTESIAN_POINT('Ctrl Pts',(9.42197095099995,11.6,-5.53027285400002));
#180184=CARTESIAN_POINT('Ctrl Pts',(9.42483649799994,15.2,-5.53085566800001));
#180185=CARTESIAN_POINT('Ctrl Pts',(9.42483649799994,11.6,-5.53085566800001));
#180186=CARTESIAN_POINT('Ctrl Pts',(9.42770791699994,15.2,-5.53143720800001));
#180187=CARTESIAN_POINT('Ctrl Pts',(9.42770791699994,11.6,-5.53143720800001));
#180188=CARTESIAN_POINT('Ctrl Pts',(9.43058520099994,15.2,-5.53201746500001));
#180189=CARTESIAN_POINT('Ctrl Pts',(9.43058520099994,11.6,-5.53201746500001));
#180190=CARTESIAN_POINT('Ctrl Pts',(9.43346834199994,15.2,-5.53259643000001));
#180191=CARTESIAN_POINT('Ctrl Pts',(9.43346834199994,11.6,-5.53259643000001));
#180192=CARTESIAN_POINT('Ctrl Pts',(9.43635733099994,15.2,-5.53317409200002));
#180193=CARTESIAN_POINT('Ctrl Pts',(9.43635733099994,11.6,-5.53317409200002));
#180194=CARTESIAN_POINT('Ctrl Pts',(9.43925215899995,15.2,-5.53375044300001));
#180195=CARTESIAN_POINT('Ctrl Pts',(9.43925215899995,11.6,-5.53375044300001));
#180196=CARTESIAN_POINT('Ctrl Pts',(9.44215281999995,15.2,-5.53432547200002));
#180197=CARTESIAN_POINT('Ctrl Pts',(9.44215281999995,11.6,-5.53432547200002));
#180198=CARTESIAN_POINT('Ctrl Pts',(9.44505930299995,15.2,-5.53489917000002));
#180199=CARTESIAN_POINT('Ctrl Pts',(9.44505930299995,11.6,-5.53489917000002));
#180200=CARTESIAN_POINT('Ctrl Pts',(9.44797160499995,15.2,-5.53547152800002));
#180201=CARTESIAN_POINT('Ctrl Pts',(9.44797160499995,11.6,-5.53547152800002));
#180202=CARTESIAN_POINT('Ctrl Pts',(9.45088971199995,15.2,-5.53604253600001));
#180203=CARTESIAN_POINT('Ctrl Pts',(9.45088971199995,11.6,-5.53604253600001));
#180204=CARTESIAN_POINT('Ctrl Pts',(9.45381361999994,15.2,-5.53661218600002));
#180205=CARTESIAN_POINT('Ctrl Pts',(9.45381361999994,11.6,-5.53661218600002));
#180206=CARTESIAN_POINT('Ctrl Pts',(9.45674331999994,15.2,-5.53718046700002));
#180207=CARTESIAN_POINT('Ctrl Pts',(9.45674331999994,11.6,-5.53718046700002));
#180208=CARTESIAN_POINT('Ctrl Pts',(9.45967880299994,15.2,-5.53774737000001));
#180209=CARTESIAN_POINT('Ctrl Pts',(9.45967880299994,11.6,-5.53774737000001));
#180210=CARTESIAN_POINT('Ctrl Pts',(9.46262006299994,15.2,-5.53831288700001));
#180211=CARTESIAN_POINT('Ctrl Pts',(9.46262006299994,11.6,-5.53831288700001));
#180212=CARTESIAN_POINT('Ctrl Pts',(9.46556708999994,15.2,-5.53887700700002));
#180213=CARTESIAN_POINT('Ctrl Pts',(9.46556708999994,11.6,-5.53887700700002));
#180214=CARTESIAN_POINT('Ctrl Pts',(9.46851987599995,15.2,-5.53943972100001));
#180215=CARTESIAN_POINT('Ctrl Pts',(9.46851987599995,11.6,-5.53943972100001));
#180216=CARTESIAN_POINT('Ctrl Pts',(9.47147841599994,15.2,-5.54000102100002));
#180217=CARTESIAN_POINT('Ctrl Pts',(9.47147841599994,11.6,-5.54000102100002));
#180218=CARTESIAN_POINT('Ctrl Pts',(9.47444269799995,15.2,-5.54056089700001));
#180219=CARTESIAN_POINT('Ctrl Pts',(9.47444269799995,11.6,-5.54056089700001));
#180220=CARTESIAN_POINT('Ctrl Pts',(9.47741271699994,15.2,-5.54111934000002));
#180221=CARTESIAN_POINT('Ctrl Pts',(9.47741271699994,11.6,-5.54111934000002));
#180222=CARTESIAN_POINT('Ctrl Pts',(9.48038846399994,15.2,-5.54167634100001));
#180223=CARTESIAN_POINT('Ctrl Pts',(9.48038846399994,11.6,-5.54167634100001));
#180224=CARTESIAN_POINT('Ctrl Pts',(9.48336992999995,15.2,-5.54223189000002));
#180225=CARTESIAN_POINT('Ctrl Pts',(9.48336992999995,11.6,-5.54223189000002));
#180226=CARTESIAN_POINT('Ctrl Pts',(9.48635710799994,15.2,-5.54278597900002));
#180227=CARTESIAN_POINT('Ctrl Pts',(9.48635710799994,11.6,-5.54278597900002));
#180228=CARTESIAN_POINT('Ctrl Pts',(9.48934999199994,15.2,-5.54333859800002));
#180229=CARTESIAN_POINT('Ctrl Pts',(9.48934999199994,11.6,-5.54333859800002));
#180230=CARTESIAN_POINT('Ctrl Pts',(9.49234857199994,15.2,-5.54388973900001));
#180231=CARTESIAN_POINT('Ctrl Pts',(9.49234857199994,11.6,-5.54388973900001));
#180232=CARTESIAN_POINT('Ctrl Pts',(9.49535283999994,15.2,-5.54443939200001));
#180233=CARTESIAN_POINT('Ctrl Pts',(9.49535283999994,11.6,-5.54443939200001));
#180234=CARTESIAN_POINT('Ctrl Pts',(9.49836278899994,15.2,-5.54498754900001));
#180235=CARTESIAN_POINT('Ctrl Pts',(9.49836278899994,11.6,-5.54498754900001));
#180236=CARTESIAN_POINT('Ctrl Pts',(9.50137840999994,15.2,-5.54553420100001));
#180237=CARTESIAN_POINT('Ctrl Pts',(9.50137840999994,11.6,-5.54553420100001));
#180238=CARTESIAN_POINT('Ctrl Pts',(9.50439969699995,15.2,-5.54607933800002));
#180239=CARTESIAN_POINT('Ctrl Pts',(9.50439969699995,11.6,-5.54607933800002));
#180240=CARTESIAN_POINT('Ctrl Pts',(9.50742664099995,15.2,-5.54662295200002));
#180241=CARTESIAN_POINT('Ctrl Pts',(9.50742664099995,11.6,-5.54662295200002));
#180242=CARTESIAN_POINT('Ctrl Pts',(9.51045923299995,15.2,-5.54716503400002));
#180243=CARTESIAN_POINT('Ctrl Pts',(9.51045923299995,11.6,-5.54716503400002));
#180244=CARTESIAN_POINT('Ctrl Pts',(9.51349746799995,15.2,-5.54770557400001));
#180245=CARTESIAN_POINT('Ctrl Pts',(9.51349746799995,11.6,-5.54770557400001));
#180246=CARTESIAN_POINT('Ctrl Pts',(9.51654133599994,15.2,-5.54824456500001));
#180247=CARTESIAN_POINT('Ctrl Pts',(9.51654133599994,11.6,-5.54824456500001));
#180248=CARTESIAN_POINT('Ctrl Pts',(9.51959082999995,15.2,-5.54878199800001));
#180249=CARTESIAN_POINT('Ctrl Pts',(9.51959082999995,11.6,-5.54878199800001));
#180250=CARTESIAN_POINT('Ctrl Pts',(9.52264594199994,15.2,-5.54931786200001));
#180251=CARTESIAN_POINT('Ctrl Pts',(9.52264594199994,11.6,-5.54931786200001));
#180252=CARTESIAN_POINT('Ctrl Pts',(9.52570666499994,15.2,-5.54985215100002));
#180253=CARTESIAN_POINT('Ctrl Pts',(9.52570666499994,11.6,-5.54985215100002));
#180254=CARTESIAN_POINT('Ctrl Pts',(9.52877299099995,15.2,-5.55038485500001));
#180255=CARTESIAN_POINT('Ctrl Pts',(9.52877299099995,11.6,-5.55038485500001));
#180256=CARTESIAN_POINT('Ctrl Pts',(9.53184491099995,15.2,-5.55091596500001));
#180257=CARTESIAN_POINT('Ctrl Pts',(9.53184491099995,11.6,-5.55091596500001));
#180258=CARTESIAN_POINT('Ctrl Pts',(9.53492241699994,15.2,-5.55144547300001));
#180259=CARTESIAN_POINT('Ctrl Pts',(9.53492241699994,11.6,-5.55144547300001));
#180260=CARTESIAN_POINT('Ctrl Pts',(9.53800550299994,15.2,-5.55197337000001));
#180261=CARTESIAN_POINT('Ctrl Pts',(9.53800550299994,11.6,-5.55197337000001));
#180262=CARTESIAN_POINT('Ctrl Pts',(9.54109416199995,15.2,-5.55249964700002));
#180263=CARTESIAN_POINT('Ctrl Pts',(9.54109416199995,11.6,-5.55249964700002));
#180264=CARTESIAN_POINT('Ctrl Pts',(9.54418838399994,15.2,-5.55302429700001));
#180265=CARTESIAN_POINT('Ctrl Pts',(9.54418838399994,11.6,-5.55302429700001));
#180266=CARTESIAN_POINT('Ctrl Pts',(9.54728816099994,15.2,-5.55354730900001));
#180267=CARTESIAN_POINT('Ctrl Pts',(9.54728816099994,11.6,-5.55354730900001));
#180268=CARTESIAN_POINT('Ctrl Pts',(9.55039348899994,15.2,-5.55406867700002));
#180269=CARTESIAN_POINT('Ctrl Pts',(9.55039348899994,11.6,-5.55406867700002));
#180270=CARTESIAN_POINT('Ctrl Pts',(9.55350435499994,15.2,-5.55458839000002));
#180271=CARTESIAN_POINT('Ctrl Pts',(9.55350435499994,11.6,-5.55458839000002));
#180272=CARTESIAN_POINT('Ctrl Pts',(9.55662075599994,15.2,-5.55510644200002));
#180273=CARTESIAN_POINT('Ctrl Pts',(9.55662075599994,11.6,-5.55510644200002));
#180274=CARTESIAN_POINT('Ctrl Pts',(9.55974268199995,15.2,-5.55562282200002));
#180275=CARTESIAN_POINT('Ctrl Pts',(9.55974268199995,11.6,-5.55562282200002));
#180276=CARTESIAN_POINT('Ctrl Pts',(9.56287012499994,15.2,-5.55613752300002));
#180277=CARTESIAN_POINT('Ctrl Pts',(9.56287012499994,11.6,-5.55613752300002));
#180278=CARTESIAN_POINT('Ctrl Pts',(9.56600307899994,15.2,-5.55665053600002));
#180279=CARTESIAN_POINT('Ctrl Pts',(9.56600307899994,11.6,-5.55665053600002));
#180280=CARTESIAN_POINT('Ctrl Pts',(9.56914153599994,15.2,-5.55716185400001));
#180281=CARTESIAN_POINT('Ctrl Pts',(9.56914153599994,11.6,-5.55716185400001));
#180282=CARTESIAN_POINT('Ctrl Pts',(9.57228548599995,15.2,-5.55767146700001));
#180283=CARTESIAN_POINT('Ctrl Pts',(9.57228548599995,11.6,-5.55767146700001));
#180284=CARTESIAN_POINT('Ctrl Pts',(9.57543492599994,15.2,-5.55817936800001));
#180285=CARTESIAN_POINT('Ctrl Pts',(9.57543492599994,11.6,-5.55817936800001));
#180286=CARTESIAN_POINT('Ctrl Pts',(9.57858984399994,15.2,-5.55868554600002));
#180287=CARTESIAN_POINT('Ctrl Pts',(9.57858984399994,11.6,-5.55868554600002));
#180288=CARTESIAN_POINT('Ctrl Pts',(9.58175023399994,15.2,-5.55918999500001));
#180289=CARTESIAN_POINT('Ctrl Pts',(9.58175023399994,11.6,-5.55918999500001));
#180290=CARTESIAN_POINT('Ctrl Pts',(9.58491608899994,15.2,-5.55969270700002));
#180291=CARTESIAN_POINT('Ctrl Pts',(9.58491608899994,11.6,-5.55969270700002));
#180292=CARTESIAN_POINT('Ctrl Pts',(9.58808740099995,15.2,-5.56019367300001));
#180293=CARTESIAN_POINT('Ctrl Pts',(9.58808740099995,11.6,-5.56019367300001));
#180294=CARTESIAN_POINT('Ctrl Pts',(9.59126416099994,15.2,-5.56069288500002));
#180295=CARTESIAN_POINT('Ctrl Pts',(9.59126416099994,11.6,-5.56069288500002));
#180296=CARTESIAN_POINT('Ctrl Pts',(9.59444636399994,15.2,-5.56119033300002));
#180297=CARTESIAN_POINT('Ctrl Pts',(9.59444636399994,11.6,-5.56119033300002));
#180298=CARTESIAN_POINT('Ctrl Pts',(9.59763400099994,15.2,-5.56168601100001));
#180299=CARTESIAN_POINT('Ctrl Pts',(9.59763400099994,11.6,-5.56168601100001));
#180300=CARTESIAN_POINT('Ctrl Pts',(9.60082706499995,15.2,-5.56217991100001));
#180301=CARTESIAN_POINT('Ctrl Pts',(9.60082706499995,11.6,-5.56217991100001));
#180302=CARTESIAN_POINT('Ctrl Pts',(9.60402554699994,15.2,-5.56267202300001));
#180303=CARTESIAN_POINT('Ctrl Pts',(9.60402554699994,11.6,-5.56267202300001));
#180304=CARTESIAN_POINT('Ctrl Pts',(9.60722944199994,15.2,-5.56316234000001));
#180305=CARTESIAN_POINT('Ctrl Pts',(9.60722944199994,11.6,-5.56316234000001));
#180306=CARTESIAN_POINT('Ctrl Pts',(9.61043874099994,15.2,-5.56365085400001));
#180307=CARTESIAN_POINT('Ctrl Pts',(9.61043874099994,11.6,-5.56365085400001));
#180308=CARTESIAN_POINT('Ctrl Pts',(9.61365343599994,15.2,-5.56413755600001));
#180309=CARTESIAN_POINT('Ctrl Pts',(9.61365343599994,11.6,-5.56413755600001));
#180310=CARTESIAN_POINT('Ctrl Pts',(9.61687351899995,15.2,-5.56462243900001));
#180311=CARTESIAN_POINT('Ctrl Pts',(9.61687351899995,11.6,-5.56462243900001));
#180312=CARTESIAN_POINT('Ctrl Pts',(9.62009898499995,15.2,-5.56510549400001));
#180313=CARTESIAN_POINT('Ctrl Pts',(9.62009898499995,11.6,-5.56510549400001));
#180314=CARTESIAN_POINT('Ctrl Pts',(9.62332982499994,15.2,-5.56558671400001));
#180315=CARTESIAN_POINT('Ctrl Pts',(9.62332982499994,11.6,-5.56558671400001));
#180316=CARTESIAN_POINT('Ctrl Pts',(9.62656603099994,15.2,-5.56606609100001));
#180317=CARTESIAN_POINT('Ctrl Pts',(9.62656603099994,11.6,-5.56606609100001));
#180318=CARTESIAN_POINT('Ctrl Pts',(9.62980759699994,15.2,-5.56654361600001));
#180319=CARTESIAN_POINT('Ctrl Pts',(9.62980759699994,11.6,-5.56654361600001));
#180320=CARTESIAN_POINT('Ctrl Pts',(9.63305451399994,15.2,-5.56701928100001));
#180321=CARTESIAN_POINT('Ctrl Pts',(9.63305451399994,11.6,-5.56701928100001));
#180322=CARTESIAN_POINT('Ctrl Pts',(9.63630677599994,15.2,-5.56749307900001));
#180323=CARTESIAN_POINT('Ctrl Pts',(9.63630677599994,11.6,-5.56749307900001));
#180324=CARTESIAN_POINT('Ctrl Pts',(9.63956437399995,15.2,-5.56796500300001));
#180325=CARTESIAN_POINT('Ctrl Pts',(9.63956437399995,11.6,-5.56796500300001));
#180326=CARTESIAN_POINT('Ctrl Pts',(9.64282730199994,15.2,-5.56843504200002));
#180327=CARTESIAN_POINT('Ctrl Pts',(9.64282730199994,11.6,-5.56843504200002));
#180328=CARTESIAN_POINT('Ctrl Pts',(9.64609555199995,15.2,-5.56890319100001));
#180329=CARTESIAN_POINT('Ctrl Pts',(9.64609555199995,11.6,-5.56890319100001));
#180330=CARTESIAN_POINT('Ctrl Pts',(9.64936911699995,15.2,-5.56936944000002));
#180331=CARTESIAN_POINT('Ctrl Pts',(9.64936911699995,11.6,-5.56936944000002));
#180332=CARTESIAN_POINT('Ctrl Pts',(9.65264798699994,15.2,-5.56983378400002));
#180333=CARTESIAN_POINT('Ctrl Pts',(9.65264798699994,11.6,-5.56983378400002));
#180334=CARTESIAN_POINT('Ctrl Pts',(9.65593215899995,15.2,-5.57029621200002));
#180335=CARTESIAN_POINT('Ctrl Pts',(9.65593215899995,11.6,-5.57029621200002));
#180336=CARTESIAN_POINT('Ctrl Pts',(9.65922162299995,15.2,-5.57075671900002));
#180337=CARTESIAN_POINT('Ctrl Pts',(9.65922162299995,11.6,-5.57075671900002));
#180338=CARTESIAN_POINT('Ctrl Pts',(9.66251637199995,15.2,-5.57121529500002));
#180339=CARTESIAN_POINT('Ctrl Pts',(9.66251637199995,11.6,-5.57121529500002));
#180340=CARTESIAN_POINT('Ctrl Pts',(9.66581639799994,15.2,-5.57167193400002));
#180341=CARTESIAN_POINT('Ctrl Pts',(9.66581639799994,11.6,-5.57167193400002));
#180342=CARTESIAN_POINT('Ctrl Pts',(9.66912169399994,15.2,-5.57212662600001));
#180343=CARTESIAN_POINT('Ctrl Pts',(9.66912169399994,11.6,-5.57212662600001));
#180344=CARTESIAN_POINT('Ctrl Pts',(9.67243225399995,15.2,-5.57257936700001));
#180345=CARTESIAN_POINT('Ctrl Pts',(9.67243225399995,11.6,-5.57257936700001));
#180346=CARTESIAN_POINT('Ctrl Pts',(9.67574806899995,15.2,-5.57303014600001));
#180347=CARTESIAN_POINT('Ctrl Pts',(9.67574806899995,11.6,-5.57303014600001));
#180348=CARTESIAN_POINT('Ctrl Pts',(9.67906913299995,15.2,-5.57347895600001));
#180349=CARTESIAN_POINT('Ctrl Pts',(9.67906913299995,11.6,-5.57347895600001));
#180350=CARTESIAN_POINT('Ctrl Pts',(9.68239543699994,15.2,-5.57392579100001));
#180351=CARTESIAN_POINT('Ctrl Pts',(9.68239543699994,11.6,-5.57392579100001));
#180352=CARTESIAN_POINT('Ctrl Pts',(9.68572697499994,15.2,-5.57437064100001));
#180353=CARTESIAN_POINT('Ctrl Pts',(9.68572697499994,11.6,-5.57437064100001));
#180354=CARTESIAN_POINT('Ctrl Pts',(9.68906373899994,15.2,-5.57481350100002));
#180355=CARTESIAN_POINT('Ctrl Pts',(9.68906373899994,11.6,-5.57481350100002));
#180356=CARTESIAN_POINT('Ctrl Pts',(9.69240572199995,15.2,-5.57525436100001));
#180357=CARTESIAN_POINT('Ctrl Pts',(9.69240572199995,11.6,-5.57525436100001));
#180358=CARTESIAN_POINT('Ctrl Pts',(9.69575291699995,15.2,-5.57569321400001));
#180359=CARTESIAN_POINT('Ctrl Pts',(9.69575291699995,11.6,-5.57569321400001));
#180360=CARTESIAN_POINT('Ctrl Pts',(9.69910531599995,15.2,-5.57613005500002));
#180361=CARTESIAN_POINT('Ctrl Pts',(9.69910531599995,11.6,-5.57613005500002));
#180362=CARTESIAN_POINT('Ctrl Pts',(9.70246291199994,15.2,-5.57656487300001));
#180363=CARTESIAN_POINT('Ctrl Pts',(9.70246291199994,11.6,-5.57656487300001));
#180364=CARTESIAN_POINT('Ctrl Pts',(9.70582569899994,15.2,-5.57699766300002));
#180365=CARTESIAN_POINT('Ctrl Pts',(9.70582569899994,11.6,-5.57699766300002));
#180366=CARTESIAN_POINT('Ctrl Pts',(9.70919366699994,15.2,-5.57742841500001));
#180367=CARTESIAN_POINT('Ctrl Pts',(9.70919366699994,11.6,-5.57742841500001));
#180368=CARTESIAN_POINT('Ctrl Pts',(9.71256681199995,15.2,-5.57785712500001));
#180369=CARTESIAN_POINT('Ctrl Pts',(9.71256681199995,11.6,-5.57785712500001));
#180370=CARTESIAN_POINT('Ctrl Pts',(9.71594512499994,15.2,-5.57828378300002));
#180371=CARTESIAN_POINT('Ctrl Pts',(9.71594512499994,11.6,-5.57828378300002));
#180372=CARTESIAN_POINT('Ctrl Pts',(9.71932859799994,15.2,-5.57870838100001));
#180373=CARTESIAN_POINT('Ctrl Pts',(9.71932859799994,11.6,-5.57870838100001));
#180374=CARTESIAN_POINT('Ctrl Pts',(9.72271722499995,15.2,-5.57913091500001));
#180375=CARTESIAN_POINT('Ctrl Pts',(9.72271722499995,11.6,-5.57913091500001));
#180376=CARTESIAN_POINT('Ctrl Pts',(9.72611099799994,15.2,-5.57955137400001));
#180377=CARTESIAN_POINT('Ctrl Pts',(9.72611099799994,11.6,-5.57955137400001));
#180378=CARTESIAN_POINT('Ctrl Pts',(9.72950990999994,15.2,-5.57996975200002));
#180379=CARTESIAN_POINT('Ctrl Pts',(9.72950990999994,11.6,-5.57996975200002));
#180380=CARTESIAN_POINT('Ctrl Pts',(9.73291395499994,15.2,-5.58038604300001));
#180381=CARTESIAN_POINT('Ctrl Pts',(9.73291395499994,11.6,-5.58038604300001));
#180382=CARTESIAN_POINT('Ctrl Pts',(9.73632312399995,15.2,-5.58080023800001));
#180383=CARTESIAN_POINT('Ctrl Pts',(9.73632312399995,11.6,-5.58080023800001));
#180384=CARTESIAN_POINT('Ctrl Pts',(9.73973740999994,15.2,-5.58121233000001));
#180385=CARTESIAN_POINT('Ctrl Pts',(9.73973740999994,11.6,-5.58121233000001));
#180386=CARTESIAN_POINT('Ctrl Pts',(9.74315680699995,15.2,-5.58162231200001));
#180387=CARTESIAN_POINT('Ctrl Pts',(9.74315680699995,11.6,-5.58162231200001));
#180388=CARTESIAN_POINT('Ctrl Pts',(9.74658130799994,15.2,-5.58203017700002));
#180389=CARTESIAN_POINT('Ctrl Pts',(9.74658130799994,11.6,-5.58203017700002));
#180390=CARTESIAN_POINT('Ctrl Pts',(9.75001090399994,15.2,-5.58243591700001));
#180391=CARTESIAN_POINT('Ctrl Pts',(9.75001090399994,11.6,-5.58243591700001));
#180392=CARTESIAN_POINT('Ctrl Pts',(9.75344559099995,15.2,-5.58283952600001));
#180393=CARTESIAN_POINT('Ctrl Pts',(9.75344559099995,11.6,-5.58283952600001));
#180394=CARTESIAN_POINT('Ctrl Pts',(9.75688535799994,15.2,-5.58324099500001));
#180395=CARTESIAN_POINT('Ctrl Pts',(9.75688535799994,11.6,-5.58324099500001));
#180396=CARTESIAN_POINT('Ctrl Pts',(9.76033019899995,15.2,-5.58364031900001));
#180397=CARTESIAN_POINT('Ctrl Pts',(9.76033019899995,11.6,-5.58364031900001));
#180398=CARTESIAN_POINT('Ctrl Pts',(9.76378010899994,15.2,-5.58403749000002));
#180399=CARTESIAN_POINT('Ctrl Pts',(9.76378010899994,11.6,-5.58403749000002));
#180400=CARTESIAN_POINT('Ctrl Pts',(9.76723507899995,15.2,-5.58443250000002));
#180401=CARTESIAN_POINT('Ctrl Pts',(9.76723507899995,11.6,-5.58443250000002));
#180402=CARTESIAN_POINT('Ctrl Pts',(9.77069510099994,15.2,-5.58482534100001));
#180403=CARTESIAN_POINT('Ctrl Pts',(9.77069510099994,11.6,-5.58482534100001));
#180404=CARTESIAN_POINT('Ctrl Pts',(9.77416016999994,15.2,-5.58521600900002));
#180405=CARTESIAN_POINT('Ctrl Pts',(9.77416016999994,11.6,-5.58521600900002));
#180406=CARTESIAN_POINT('Ctrl Pts',(9.77763027799995,15.2,-5.58560449600002));
#180407=CARTESIAN_POINT('Ctrl Pts',(9.77763027799995,11.6,-5.58560449600002));
#180408=CARTESIAN_POINT('Ctrl Pts',(9.78110541799994,15.2,-5.58599079400001));
#180409=CARTESIAN_POINT('Ctrl Pts',(9.78110541799994,11.6,-5.58599079400001));
#180410=CARTESIAN_POINT('Ctrl Pts',(9.78458558299995,15.2,-5.58637489500001));
#180411=CARTESIAN_POINT('Ctrl Pts',(9.78458558299995,11.6,-5.58637489500001));
#180412=CARTESIAN_POINT('Ctrl Pts',(9.78807076599994,15.2,-5.58675679400002));
#180413=CARTESIAN_POINT('Ctrl Pts',(9.78807076599994,11.6,-5.58675679400002));
#180414=CARTESIAN_POINT('Ctrl Pts',(9.79156095799994,15.2,-5.58713648300001));
#180415=CARTESIAN_POINT('Ctrl Pts',(9.79156095799994,11.6,-5.58713648300001));
#180416=CARTESIAN_POINT('Ctrl Pts',(9.79505615499994,15.2,-5.58751395600002));
#180417=CARTESIAN_POINT('Ctrl Pts',(9.79505615499994,11.6,-5.58751395600002));
#180418=CARTESIAN_POINT('Ctrl Pts',(9.79855634899994,15.2,-5.58788920400001));
#180419=CARTESIAN_POINT('Ctrl Pts',(9.79855634899994,11.6,-5.58788920400001));
#180420=CARTESIAN_POINT('Ctrl Pts',(9.80206153099994,15.2,-5.58826222200001));
#180421=CARTESIAN_POINT('Ctrl Pts',(9.80206153099994,11.6,-5.58826222200001));
#180422=CARTESIAN_POINT('Ctrl Pts',(9.80557169599994,15.2,-5.58863300200001));
#180423=CARTESIAN_POINT('Ctrl Pts',(9.80557169599994,11.6,-5.58863300200001));
#180424=CARTESIAN_POINT('Ctrl Pts',(9.80908683699995,15.2,-5.58900153800002));
#180425=CARTESIAN_POINT('Ctrl Pts',(9.80908683699995,11.6,-5.58900153800002));
#180426=CARTESIAN_POINT('Ctrl Pts',(9.81260694599994,15.2,-5.58936782200002));
#180427=CARTESIAN_POINT('Ctrl Pts',(9.81260694599994,11.6,-5.58936782200002));
#180428=CARTESIAN_POINT('Ctrl Pts',(9.81613201599994,15.2,-5.58973184900001));
#180429=CARTESIAN_POINT('Ctrl Pts',(9.81613201599994,11.6,-5.58973184900001));
#180430=CARTESIAN_POINT('Ctrl Pts',(9.81966204099994,15.2,-5.59009360900002));
#180431=CARTESIAN_POINT('Ctrl Pts',(9.81966204099994,11.6,-5.59009360900002));
#180432=CARTESIAN_POINT('Ctrl Pts',(9.82319701199994,15.2,-5.59045309800001));
#180433=CARTESIAN_POINT('Ctrl Pts',(9.82319701199994,11.6,-5.59045309800001));
#180434=CARTESIAN_POINT('Ctrl Pts',(9.82673692399995,15.2,-5.59081030900002));
#180435=CARTESIAN_POINT('Ctrl Pts',(9.82673692399995,11.6,-5.59081030900002));
#180436=CARTESIAN_POINT('Ctrl Pts',(9.83028176999994,15.2,-5.59116523300002));
#180437=CARTESIAN_POINT('Ctrl Pts',(9.83028176999994,11.6,-5.59116523300002));
#180438=CARTESIAN_POINT('Ctrl Pts',(9.83383154199995,15.2,-5.59151786600002));
#180439=CARTESIAN_POINT('Ctrl Pts',(9.83383154199995,11.6,-5.59151786600002));
#180440=CARTESIAN_POINT('Ctrl Pts',(9.83738623299995,15.2,-5.59186819800002));
#180441=CARTESIAN_POINT('Ctrl Pts',(9.83738623299995,11.6,-5.59186819800002));
#180442=CARTESIAN_POINT('Ctrl Pts',(9.84094583499994,15.2,-5.59221622600001));
#180443=CARTESIAN_POINT('Ctrl Pts',(9.84094583499994,11.6,-5.59221622600001));
#180444=CARTESIAN_POINT('Ctrl Pts',(9.84451034499994,15.2,-5.59256194000001));
#180445=CARTESIAN_POINT('Ctrl Pts',(9.84451034499994,11.6,-5.59256194000001));
#180446=CARTESIAN_POINT('Ctrl Pts',(9.84807975099995,15.2,-5.59290533500001));
#180447=CARTESIAN_POINT('Ctrl Pts',(9.84807975099995,11.6,-5.59290533500001));
#180448=CARTESIAN_POINT('Ctrl Pts',(9.85165404999995,15.2,-5.59324640400002));
#180449=CARTESIAN_POINT('Ctrl Pts',(9.85165404999995,11.6,-5.59324640400002));
#180450=CARTESIAN_POINT('Ctrl Pts',(9.85523323299994,15.2,-5.59358514100001));
#180451=CARTESIAN_POINT('Ctrl Pts',(9.85523323299994,11.6,-5.59358514100001));
#180452=CARTESIAN_POINT('Ctrl Pts',(9.85881729299994,15.2,-5.59392153800002));
#180453=CARTESIAN_POINT('Ctrl Pts',(9.85881729299994,11.6,-5.59392153800002));
#180454=CARTESIAN_POINT('Ctrl Pts',(9.86240622499994,15.2,-5.59425558900001));
#180455=CARTESIAN_POINT('Ctrl Pts',(9.86240622499994,11.6,-5.59425558900001));
#180456=CARTESIAN_POINT('Ctrl Pts',(9.86600001899994,15.2,-5.59458728700001));
#180457=CARTESIAN_POINT('Ctrl Pts',(9.86600001899994,11.6,-5.59458728700001));
#180458=CARTESIAN_POINT('Ctrl Pts',(9.86959867099995,15.2,-5.59491662600001));
#180459=CARTESIAN_POINT('Ctrl Pts',(9.86959867099995,11.6,-5.59491662600001));
#180460=CARTESIAN_POINT('Ctrl Pts',(9.87320217199994,15.2,-5.59524360000001));
#180461=CARTESIAN_POINT('Ctrl Pts',(9.87320217199994,11.6,-5.59524360000001));
#180462=CARTESIAN_POINT('Ctrl Pts',(9.87681051699994,15.2,-5.59556820100001));
#180463=CARTESIAN_POINT('Ctrl Pts',(9.87681051699994,11.6,-5.59556820100001));
#180464=CARTESIAN_POINT('Ctrl Pts',(9.88042369799994,15.2,-5.59589042300002));
#180465=CARTESIAN_POINT('Ctrl Pts',(9.88042369799994,11.6,-5.59589042300002));
#180466=CARTESIAN_POINT('Ctrl Pts',(9.88404170699994,15.2,-5.59621025900002));
#180467=CARTESIAN_POINT('Ctrl Pts',(9.88404170699994,11.6,-5.59621025900002));
#180468=CARTESIAN_POINT('Ctrl Pts',(9.88766453899995,15.2,-5.59652770400001));
#180469=CARTESIAN_POINT('Ctrl Pts',(9.88766453899995,11.6,-5.59652770400001));
#180470=CARTESIAN_POINT('Ctrl Pts',(9.89129218699994,15.2,-5.59684275000001));
#180471=CARTESIAN_POINT('Ctrl Pts',(9.89129218699994,11.6,-5.59684275000001));
#180472=CARTESIAN_POINT('Ctrl Pts',(9.89492464299994,15.2,-5.59715539100001));
#180473=CARTESIAN_POINT('Ctrl Pts',(9.89492464299994,11.6,-5.59715539100001));
#180474=CARTESIAN_POINT('Ctrl Pts',(9.89856189999994,15.2,-5.59746562100001));
#180475=CARTESIAN_POINT('Ctrl Pts',(9.89856189999994,11.6,-5.59746562100001));
#180476=CARTESIAN_POINT('Ctrl Pts',(9.90220395199995,15.2,-5.59777343200001));
#180477=CARTESIAN_POINT('Ctrl Pts',(9.90220395199995,11.6,-5.59777343200001));
#180478=CARTESIAN_POINT('Ctrl Pts',(9.90585079199995,15.2,-5.59807881900001));
#180479=CARTESIAN_POINT('Ctrl Pts',(9.90585079199995,11.6,-5.59807881900001));
#180480=CARTESIAN_POINT('Ctrl Pts',(9.90950241399995,15.2,-5.59838177500001));
#180481=CARTESIAN_POINT('Ctrl Pts',(9.90950241399995,11.6,-5.59838177500001));
#180482=CARTESIAN_POINT('Ctrl Pts',(9.91315880899995,15.2,-5.59868229500001));
#180483=CARTESIAN_POINT('Ctrl Pts',(9.91315880899995,11.6,-5.59868229500001));
#180484=CARTESIAN_POINT('Ctrl Pts',(9.91681997199995,15.2,-5.59898037100002));
#180485=CARTESIAN_POINT('Ctrl Pts',(9.91681997199995,11.6,-5.59898037100002));
#180486=CARTESIAN_POINT('Ctrl Pts',(9.92048589699994,15.2,-5.59927599600002));
#180487=CARTESIAN_POINT('Ctrl Pts',(9.92048589699994,11.6,-5.59927599600002));
#180488=CARTESIAN_POINT('Ctrl Pts',(9.92415657399994,15.2,-5.59956916600001));
#180489=CARTESIAN_POINT('Ctrl Pts',(9.92415657399994,11.6,-5.59956916600001));
#180490=CARTESIAN_POINT('Ctrl Pts',(9.92783199799995,15.2,-5.59985987200001));
#180491=CARTESIAN_POINT('Ctrl Pts',(9.92783199799995,11.6,-5.59985987200001));
#180492=CARTESIAN_POINT('Ctrl Pts',(9.93151216199994,15.2,-5.60014811000002));
#180493=CARTESIAN_POINT('Ctrl Pts',(9.93151216199994,11.6,-5.60014811000002));
#180494=CARTESIAN_POINT('Ctrl Pts',(9.93519705899994,15.2,-5.60043387200002));
#180495=CARTESIAN_POINT('Ctrl Pts',(9.93519705899994,11.6,-5.60043387200002));
#180496=CARTESIAN_POINT('Ctrl Pts',(9.93888668299994,15.2,-5.60071715300001));
#180497=CARTESIAN_POINT('Ctrl Pts',(9.93888668299994,11.6,-5.60071715300001));
#180498=CARTESIAN_POINT('Ctrl Pts',(9.94258102699994,15.2,-5.60099794600001));
#180499=CARTESIAN_POINT('Ctrl Pts',(9.94258102699994,11.6,-5.60099794600001));
#180500=CARTESIAN_POINT('Ctrl Pts',(9.94628008499994,15.2,-5.60127624400002));
#180501=CARTESIAN_POINT('Ctrl Pts',(9.94628008499994,11.6,-5.60127624400002));
#180502=CARTESIAN_POINT('Ctrl Pts',(9.94998384799995,15.2,-5.60155204300001));
#180503=CARTESIAN_POINT('Ctrl Pts',(9.94998384799995,11.6,-5.60155204300001));
#180504=CARTESIAN_POINT('Ctrl Pts',(9.95369231099994,15.2,-5.60182533700001));
#180505=CARTESIAN_POINT('Ctrl Pts',(9.95369231099994,11.6,-5.60182533700001));
#180506=CARTESIAN_POINT('Ctrl Pts',(9.95740546699994,15.2,-5.60209611600001));
#180507=CARTESIAN_POINT('Ctrl Pts',(9.95740546699994,11.6,-5.60209611600001));
#180508=CARTESIAN_POINT('Ctrl Pts',(9.96112330899994,15.2,-5.60236437800001));
#180509=CARTESIAN_POINT('Ctrl Pts',(9.96112330899994,11.6,-5.60236437800001));
#180510=CARTESIAN_POINT('Ctrl Pts',(9.96484582999994,15.2,-5.60263011400002));
#180511=CARTESIAN_POINT('Ctrl Pts',(9.96484582999994,11.6,-5.60263011400002));
#180512=CARTESIAN_POINT('Ctrl Pts',(9.96857302299994,15.2,-5.60289331700002));
#180513=CARTESIAN_POINT('Ctrl Pts',(9.96857302299994,11.6,-5.60289331700002));
#180514=CARTESIAN_POINT('Ctrl Pts',(9.97230487899994,15.2,-5.60315398300002));
#180515=CARTESIAN_POINT('Ctrl Pts',(9.97230487899994,11.6,-5.60315398300002));
#180516=CARTESIAN_POINT('Ctrl Pts',(9.97604139599994,15.2,-5.60341210500001));
#180517=CARTESIAN_POINT('Ctrl Pts',(9.97604139599994,11.6,-5.60341210500001));
#180518=CARTESIAN_POINT('Ctrl Pts',(9.97978256299995,15.2,-5.60366767600001));
#180519=CARTESIAN_POINT('Ctrl Pts',(9.97978256299995,11.6,-5.60366767600001));
#180520=CARTESIAN_POINT('Ctrl Pts',(9.98352837599995,15.2,-5.60392069300002));
#180521=CARTESIAN_POINT('Ctrl Pts',(9.98352837599995,11.6,-5.60392069300002));
#180522=CARTESIAN_POINT('Ctrl Pts',(9.98727882999994,15.2,-5.60417114700002));
#180523=CARTESIAN_POINT('Ctrl Pts',(9.98727882999994,11.6,-5.60417114700002));
#180524=CARTESIAN_POINT('Ctrl Pts',(9.99103391599995,15.2,-5.60441903700001));
#180525=CARTESIAN_POINT('Ctrl Pts',(9.99103391599995,11.6,-5.60441903700001));
#180526=CARTESIAN_POINT('Ctrl Pts',(9.99479362999995,15.2,-5.60466435300001));
#180527=CARTESIAN_POINT('Ctrl Pts',(9.99479362999995,11.6,-5.60466435300001));
#180528=CARTESIAN_POINT('Ctrl Pts',(9.99855796499994,15.2,-5.60490709200002));
#180529=CARTESIAN_POINT('Ctrl Pts',(9.99855796499994,11.6,-5.60490709200002));
#180530=CARTESIAN_POINT('Ctrl Pts',(10.0023269109999,15.2,-5.60514724400001));
#180531=CARTESIAN_POINT('Ctrl Pts',(10.0023269109999,11.6,-5.60514724400001));
#180532=CARTESIAN_POINT('Ctrl Pts',(10.0061004619999,15.2,-5.60538480400002));
#180533=CARTESIAN_POINT('Ctrl Pts',(10.0061004619999,11.6,-5.60538480400002));
#180534=CARTESIAN_POINT('Ctrl Pts',(10.0098786099999,15.2,-5.60561976300002));
#180535=CARTESIAN_POINT('Ctrl Pts',(10.0098786099999,11.6,-5.60561976300002));
#180536=CARTESIAN_POINT('Ctrl Pts',(10.0136613449999,15.2,-5.60585211500001));
#180537=CARTESIAN_POINT('Ctrl Pts',(10.0136613449999,11.6,-5.60585211500001));
#180538=CARTESIAN_POINT('Ctrl Pts',(10.0174486609999,15.2,-5.60608185200001));
#180539=CARTESIAN_POINT('Ctrl Pts',(10.0174486609999,11.6,-5.60608185200001));
#180540=CARTESIAN_POINT('Ctrl Pts',(10.0212405509999,15.2,-5.60630897000001));
#180541=CARTESIAN_POINT('Ctrl Pts',(10.0212405509999,11.6,-5.60630897000001));
#180542=CARTESIAN_POINT('Ctrl Pts',(10.0250370109999,15.2,-5.60653346400001));
#180543=CARTESIAN_POINT('Ctrl Pts',(10.0250370109999,11.6,-5.60653346400001));
#180544=CARTESIAN_POINT('Ctrl Pts',(10.0288380379999,15.2,-5.60675533200001));
#180545=CARTESIAN_POINT('Ctrl Pts',(10.0288380379999,11.6,-5.60675533200001));
#180546=CARTESIAN_POINT('Ctrl Pts',(10.0326436309999,15.2,-5.60697457300002));
#180547=CARTESIAN_POINT('Ctrl Pts',(10.0326436309999,11.6,-5.60697457300002));
#180548=CARTESIAN_POINT('Ctrl Pts',(10.0356917559999,15.2,-5.60714786300001));
#180549=CARTESIAN_POINT('Ctrl Pts',(10.0356917559999,11.6,-5.60714786300001));
#180550=CARTESIAN_POINT('Ctrl Pts',(10.0379799039999,15.2,-5.60727664700002));
#180551=CARTESIAN_POINT('Ctrl Pts',(10.0379799039999,11.6,-5.60727664700002));
#180552=CARTESIAN_POINT('Ctrl Pts',(10.0395062489999,15.2,-5.60736197900002));
#180553=CARTESIAN_POINT('Ctrl Pts',(10.0395062489999,11.6,-5.60736197900002));
#180554=CARTESIAN_POINT('Ctrl Pts',(10.0402696489999,15.2,-5.60740451200001));
#180555=CARTESIAN_POINT('Ctrl Pts',(10.0402696489999,11.6,-5.60740451200001));
#180556=CARTESIAN_POINT('Ctrl Pts',(8.88241603299995,15.2,-5.36127880600001));
#180557=CARTESIAN_POINT('Ctrl Pts',(8.88401933304833,15.2,-5.36206719629503));
#180558=CARTESIAN_POINT('Ctrl Pts',(8.88567630917062,15.2,-5.36287598656166));
#180559=CARTESIAN_POINT('Ctrl Pts',(8.8873863638459,15.2,-5.36370417391761));
#180560=CARTESIAN_POINT('Ctrl Pts',(8.88910466526922,15.2,-5.36453635521162));
#180561=CARTESIAN_POINT('Ctrl Pts',(8.89087656280783,15.2,-5.36538812047558));
#180562=CARTESIAN_POINT('Ctrl Pts',(8.89270147741819,15.2,-5.36625848006756));
#180563=CARTESIAN_POINT('Ctrl Pts',(8.89452639186279,15.2,-5.3671288395805));
#180564=CARTESIAN_POINT('Ctrl Pts',(8.89640432496164,15.2,-5.36801779213292));
#180565=CARTESIAN_POINT('Ctrl Pts',(8.89833471330818,15.2,-5.36892438076665));
#180566=CARTESIAN_POINT('Ctrl Pts',(8.90026510165471,15.2,-5.36983096940038));
#180567=CARTESIAN_POINT('Ctrl Pts',(8.90224794607846,15.1999999999999,-5.37075519313048));
#180568=CARTESIAN_POINT('Ctrl Pts',(8.90428269376981,15.2,-5.37169612014234));
#180569=CARTESIAN_POINT('Ctrl Pts',(8.90631744164601,15.2,-5.37263704723965));
#180570=CARTESIAN_POINT('Ctrl Pts',(8.90840409644624,15.2,-5.37359467979364));
#180571=CARTESIAN_POINT('Ctrl Pts',(8.91054211906624,15.2,-5.37456811359776));
#180572=CARTESIAN_POINT('Ctrl Pts',(8.91268014149207,15.2,-5.37554154731347));
#180573=CARTESIAN_POINT('Ctrl Pts',(8.91486953043031,15.2,-5.37653078087401));
#180574=CARTESIAN_POINT('Ctrl Pts',(8.91710976394254,15.2,-5.37753493975878));
#180575=CARTESIAN_POINT('Ctrl Pts',(8.91934999745478,15.2,-5.37853909864355));
#180576=CARTESIAN_POINT('Ctrl Pts',(8.92164107324306,15.2,-5.37955818039023));
#180577=CARTESIAN_POINT('Ctrl Pts',(8.92398247965579,15.2,-5.38059133443541));
#180578=CARTESIAN_POINT('Ctrl Pts',(8.9263238862812,15.2,-5.38162448857445));
#180579=CARTESIAN_POINT('Ctrl Pts',(8.92871562078788,15.2,-5.38267171456523));
#180580=CARTESIAN_POINT('Ctrl Pts',(8.93115718350766,15.2,-5.38373218387392));
#180581=CARTESIAN_POINT('Ctrl Pts',(8.93359874600567,15.2,-5.38479265308629));
#180582=CARTESIAN_POINT('Ctrl Pts',(8.93609013491204,15.2,-5.38586636586483));
#180583=CARTESIAN_POINT('Ctrl Pts',(8.9386308586552,15.2,-5.3869525153259));
#180584=CARTESIAN_POINT('Ctrl Pts',(8.94117158239835,15.2,-5.38803866478697));
#180585=CARTESIAN_POINT('Ctrl Pts',(8.94376164092926,15.2,-5.38913725330539));
#180586=CARTESIAN_POINT('Ctrl Pts',(8.94640055158124,15.2,-5.3902474946812));
#180587=CARTESIAN_POINT('Ctrl Pts',(8.94903946223323,15.2,-5.39135773605702));
#180588=CARTESIAN_POINT('Ctrl Pts',(8.95172722686268,15.2,-5.39247963096843));
#180589=CARTESIAN_POINT('Ctrl Pts',(8.95446336867663,15.2,-5.39361241742653));
#180590=CARTESIAN_POINT('Ctrl Pts',(8.95719951073912,15.2,-5.39474520398751));
#180591=CARTESIAN_POINT('Ctrl Pts',(8.95998403506464,15.2,-5.39588888035792));
#180592=CARTESIAN_POINT('Ctrl Pts',(8.9628164732211,15.2,-5.39704270583792));
#180593=CARTESIAN_POINT('Ctrl Pts',(8.96564891112028,15.2,-5.39819653121312));
#180594=CARTESIAN_POINT('Ctrl Pts',(8.96852926582505,15.2,-5.39936050395345));
#180595=CARTESIAN_POINT('Ctrl Pts',(8.97145708073187,15.2,-5.40053389974947));
#180596=CARTESIAN_POINT('Ctrl Pts',(8.97438489563868,15.2,-5.40170729554548));
#180597=CARTESIAN_POINT('Ctrl Pts',(8.97736017116679,15.2,-5.402890118114));
#180598=CARTESIAN_POINT('Ctrl Pts',(8.98038246188711,15.2,-5.40408165690346));
#180599=CARTESIAN_POINT('Ctrl Pts',(8.98340475288196,15.2,-5.40527319580113));
#180600=CARTESIAN_POINT('Ctrl Pts',(8.98647405673137,15.2,-5.40647345299135));
#180601=CARTESIAN_POINT('Ctrl Pts',(8.98958993590321,15.2,-5.40768174280755));
#180602=CARTESIAN_POINT('Ctrl Pts',(8.99270581479201,15.2,-5.408890032514));
#180603=CARTESIAN_POINT('Ctrl Pts',(8.99586827068388,15.2,-5.41010635178838));
#180604=CARTESIAN_POINT('Ctrl Pts',(8.99907686774841,15.2,-5.41133003174945));
#180605=CARTESIAN_POINT('Ctrl Pts',(9.00228546481295,15.2,-5.41255371171051));
#180606=CARTESIAN_POINT('Ctrl Pts',(9.00554020763815,15.2,-5.41378475248552));
#180607=CARTESIAN_POINT('Ctrl Pts',(9.00884067043179,15.2,-5.41502249935676));
#180608=CARTESIAN_POINT('Ctrl Pts',(9.01214113352523,15.2,-5.41626024634042));
#180609=CARTESIAN_POINT('Ctrl Pts',(9.0154873156295,15.2,-5.41750469859));
#180610=CARTESIAN_POINT('Ctrl Pts',(9.01887880106973,15.2,-5.41875521888766));
#180611=CARTESIAN_POINT('Ctrl Pts',(9.0222702862019,15.2,-5.42000573907171));
#180612=CARTESIAN_POINT('Ctrl Pts',(9.02570707445971,15.2,-5.4212623260792));
#180613=CARTESIAN_POINT('Ctrl Pts',(9.02918875449986,15.2,-5.4225243582));
#180614=CARTESIAN_POINT('Ctrl Pts',(9.03325071475754,15.2,-5.42399672908404));
#180615=CARTESIAN_POINT('Ctrl Pts',(9.03737378010303,15.2,-5.42547650832552));
#180616=CARTESIAN_POINT('Ctrl Pts',(9.04155730733853,15.2,-5.42696273238159));
#180617=CARTESIAN_POINT('Ctrl Pts',(9.04514318763997,15.2,-5.42823663864923));
#180618=CARTESIAN_POINT('Ctrl Pts',(9.04877348980836,15.2,-5.42951528044662));
#180619=CARTESIAN_POINT('Ctrl Pts',(9.05244781792486,15.2,-5.43079806473334));
#180620=CARTESIAN_POINT('Ctrl Pts',(9.05612214604136,15.2,-5.43208084902007));
#180621=CARTESIAN_POINT('Ctrl Pts',(9.05984049788733,15.2,-5.43336777604114));
#180622=CARTESIAN_POINT('Ctrl Pts',(9.06360248610272,15.2,-5.43465826739185));
#180623=CARTESIAN_POINT('Ctrl Pts',(9.06736447465983,15.2,-5.43594875885977));
#180624=CARTESIAN_POINT('Ctrl Pts',(9.07117009649003,15.2,-5.43724281378716));
#180625=CARTESIAN_POINT('Ctrl Pts',(9.07501896886941,15.2,-5.43853986635806));
#180626=CARTESIAN_POINT('Ctrl Pts',(9.07822636234408,15.2,-5.43962074344155));
#180627=CARTESIAN_POINT('Ctrl Pts',(9.08146378863036,15.2,-5.4407037035473));
#180628=CARTESIAN_POINT('Ctrl Pts',(9.08473103120224,15.2,-5.44178842465856));
#180629=CARTESIAN_POINT('Ctrl Pts',(9.08799827341799,15.2,-5.44287314565157));
#180630=CARTESIAN_POINT('Ctrl Pts',(9.0912953289909,15.2,-5.44395962754308));
#180631=CARTESIAN_POINT('Ctrl Pts',(9.09462198209809,15.2,-5.44504755617438));
#180632=CARTESIAN_POINT('Ctrl Pts',(9.09794863556789,15.2,-5.44613548492426));
#180633=CARTESIAN_POINT('Ctrl Pts',(9.10130488505945,15.2,-5.44722485903524));
#180634=CARTESIAN_POINT('Ctrl Pts',(9.10469051776537,15.2,-5.44831537188237));
#180635=CARTESIAN_POINT('Ctrl Pts',(9.10807615047132,15.2,-5.44940588472951));
#180636=CARTESIAN_POINT('Ctrl Pts',(9.11149116437456,15.2,-5.45049753292978));
#180637=CARTESIAN_POINT('Ctrl Pts',(9.11493534885015,15.2,-5.45159001666486));
#180638=CARTESIAN_POINT('Ctrl Pts',(9.11837953332575,15.2,-5.45268250039993));
#180639=CARTESIAN_POINT('Ctrl Pts',(9.12185288672808,15.2,-5.45377581602851));
#180640=CARTESIAN_POINT('Ctrl Pts',(9.12535519950433,15.2,-5.45486966894515));
#180641=CARTESIAN_POINT('Ctrl Pts',(9.12955797506489,15.2,-5.45618229251665));
#180642=CARTESIAN_POINT('Ctrl Pts',(9.13380245172231,15.2,-5.45749568616325));
#180643=CARTESIAN_POINT('Ctrl Pts',(9.1380882712087,15.2,-5.45880934415154));
#180644=CARTESIAN_POINT('Ctrl Pts',(9.14165978686342,15.2,-5.45990405896278));
#180645=CARTESIAN_POINT('Ctrl Pts',(9.14526001213977,15.2,-5.46099896027614));
#180646=CARTESIAN_POINT('Ctrl Pts',(9.14888874278358,15.2,-5.46209375828182));
#180647=CARTESIAN_POINT('Ctrl Pts',(9.15251747382291,15.2,-5.46318855640682));
#180648=CARTESIAN_POINT('Ctrl Pts',(9.15617470851458,15.2,-5.46428325247907));
#180649=CARTESIAN_POINT('Ctrl Pts',(9.15986024552615,15.2,-5.46537756463188));
#180650=CARTESIAN_POINT('Ctrl Pts',(9.16428289018106,15.2,-5.46669073928682));
#180651=CARTESIAN_POINT('Ctrl Pts',(9.16874628845453,15.2,-5.46800336017328));
#180652=CARTESIAN_POINT('Ctrl Pts',(9.17325009417733,15.2,-5.46931495014356));
#180653=CARTESIAN_POINT('Ctrl Pts',(9.17700326540845,15.2,-5.47040794172589));
#180654=CARTESIAN_POINT('Ctrl Pts',(9.1807844959125,15.2,-5.47150021725395));
#180655=CARTESIAN_POINT('Ctrl Pts',(9.18459358945645,15.2,-5.47259150635109));
#180656=CARTESIAN_POINT('Ctrl Pts',(9.18840268300039,15.2,-5.47368279544823));
#180657=CARTESIAN_POINT('Ctrl Pts',(9.19223963591422,15.2,-5.47477309693146));
#180658=CARTESIAN_POINT('Ctrl Pts',(9.19610425605537,15.2,-5.4758621451258));
#180659=CARTESIAN_POINT('Ctrl Pts',(9.19996887619653,15.2,-5.47695119332015));
#180660=CARTESIAN_POINT('Ctrl Pts',(9.2038611591659,15.2,-5.47803898787556));
#180661=CARTESIAN_POINT('Ctrl Pts',(9.20778091298759,15.2,-5.47912526537544));
#180662=CARTESIAN_POINT('Ctrl Pts',(9.21170066638203,15.2,-5.48021154275691));
#180663=CARTESIAN_POINT('Ctrl Pts',(9.21564789101545,15.2,-5.48129630520959));
#180664=CARTESIAN_POINT('Ctrl Pts',(9.21962239099669,15.2,-5.4823792925917));
#180665=CARTESIAN_POINT('Ctrl Pts',(9.22359689141114,15.2,-5.48346228009185));
#180666=CARTESIAN_POINT('Ctrl Pts',(9.22759866835845,15.2,-5.48454349366425));
#180667=CARTESIAN_POINT('Ctrl Pts',(9.23162753127291,15.2,-5.4856226795672));
#180668=CARTESIAN_POINT('Ctrl Pts',(9.23485062178014,15.2,-5.48648602833661));
#180669=CARTESIAN_POINT('Ctrl Pts',(9.23809104670969,15.2,-5.4873480793748));
#180670=CARTESIAN_POINT('Ctrl Pts',(9.24134870923543,15.2,-5.48820870525894));
#180671=CARTESIAN_POINT('Ctrl Pts',(9.24460637131731,15.2,-5.48906933102582));
#180672=CARTESIAN_POINT('Ctrl Pts',(9.24788127249917,15.2,-5.48992852997974));
#180673=CARTESIAN_POINT('Ctrl Pts',(9.25117331322831,15.2,-5.4907861779098));
#180674=CARTESIAN_POINT('Ctrl Pts',(9.25446535440599,15.2,-5.4916438259567));
#180675=CARTESIAN_POINT('Ctrl Pts',(9.25777453593526,15.2,-5.49249992043401));
#180676=CARTESIAN_POINT('Ctrl Pts',(9.2611007637832,15.2,-5.49335433975835));
#180677=CARTESIAN_POINT('Ctrl Pts',(9.26442699163114,15.2,-5.4942087590827));
#180678=CARTESIAN_POINT('Ctrl Pts',(9.26777026387831,15.2,-5.49506150118462));
#180679=CARTESIAN_POINT('Ctrl Pts',(9.27113048700762,15.2,-5.49591244339748));
#180680=CARTESIAN_POINT('Ctrl Pts',(9.2744907096791,15.2,-5.49676338549441));
#180681=CARTESIAN_POINT('Ctrl Pts',(9.2778678838319,15.2,-5.49761252866762));
#180682=CARTESIAN_POINT('Ctrl Pts',(9.28126191201423,15.2,-5.49845974999111));
#180683=CARTESIAN_POINT('Ctrl Pts',(9.28465594065901,15.2,-5.49930697143003));
#180684=CARTESIAN_POINT('Ctrl Pts',(9.28806682546901,15.2,-5.50015227132826));
#180685=CARTESIAN_POINT('Ctrl Pts',(9.29149447260197,15.2,-5.50099553009623));
#180686=CARTESIAN_POINT('Ctrl Pts',(9.29577903128468,15.2,-5.50204960349875));
#180687=CARTESIAN_POINT('Ctrl Pts',(9.30008977898167,15.2,-5.50310048678731));
#180688=CARTESIAN_POINT('Ctrl Pts',(9.30442653606713,15.2,-5.50414795012036));
#180689=CARTESIAN_POINT('Ctrl Pts',(9.30789594145187,15.2,-5.5049859207183));
#180690=CARTESIAN_POINT('Ctrl Pts',(9.31138199191798,15.2,-5.50582170266102));
#180691=CARTESIAN_POINT('Ctrl Pts',(9.31488459598083,15.2,-5.50665517754112));
#180692=CARTESIAN_POINT('Ctrl Pts',(9.31838720052091,15.2,-5.50748865253479));
#180693=CARTESIAN_POINT('Ctrl Pts',(9.32190635823638,15.2,-5.50831982309616));
#180694=CARTESIAN_POINT('Ctrl Pts',(9.32544197681963,15.2,-5.50914857191886));
#180695=CARTESIAN_POINT('Ctrl Pts',(9.32986149980783,15.2,-5.51018450789076));
#180696=CARTESIAN_POINT('Ctrl Pts',(9.33430674252704,15.2,-5.51121666056817));
#180697=CARTESIAN_POINT('Ctrl Pts',(9.338777529543,15.2,-5.5122448091095));
#180698=CARTESIAN_POINT('Ctrl Pts',(9.34235415886339,15.2,-5.51306732787533));
#180699=CARTESIAN_POINT('Ctrl Pts',(9.34594713505947,15.2,-5.5138872839209));
#180700=CARTESIAN_POINT('Ctrl Pts',(9.34955636778076,15.2,-5.51470456469113));
#180701=CARTESIAN_POINT('Ctrl Pts',(9.35316560099381,15.2,-5.51552184557273));
#180702=CARTESIAN_POINT('Ctrl Pts',(9.35679109012851,15.2,-5.51633645184991));
#180703=CARTESIAN_POINT('Ctrl Pts',(9.36043274732863,15.2,-5.51714827211609));
#180704=CARTESIAN_POINT('Ctrl Pts',(9.36498481858069,15.2,-5.51816304739351));
#180705=CARTESIAN_POINT('Ctrl Pts',(9.3695621489165,15.2,-5.51917347065419));
#180706=CARTESIAN_POINT('Ctrl Pts',(9.37416456683522,15.2,-5.52017932759826));
#180707=CARTESIAN_POINT('Ctrl Pts',(9.37784650086919,15.2,-5.52098401308774));
#180708=CARTESIAN_POINT('Ctrl Pts',(9.38154448838416,15.2,-5.52178577728337));
#180709=CARTESIAN_POINT('Ctrl Pts',(9.38525844376402,15.2,-5.52258451199948));
#180710=CARTESIAN_POINT('Ctrl Pts',(9.38897239964991,15.2,-5.52338324682443));
#180711=CARTESIAN_POINT('Ctrl Pts',(9.39270232140934,15.2,-5.52417895098118));
#180712=CARTESIAN_POINT('Ctrl Pts',(9.39644812133733,15.2,-5.52497151991294));
#180713=CARTESIAN_POINT('Ctrl Pts',(9.40113037099213,15.2,-5.52596223102365));
#180714=CARTESIAN_POINT('Ctrl Pts',(9.40583742996678,15.2,-5.52694804220095));
#180715=CARTESIAN_POINT('Ctrl Pts',(9.41056912788546,15.2,-5.52792874831163));
#180716=CARTESIAN_POINT('Ctrl Pts',(9.41435448591096,15.2,-5.52871331313605));
#180717=CARTESIAN_POINT('Ctrl Pts',(9.41815561213925,15.2,-5.52949461033455));
#180718=CARTESIAN_POINT('Ctrl Pts',(9.42197242078895,15.2,-5.5302725377745));
#180719=CARTESIAN_POINT('Ctrl Pts',(9.4267434319911,15.2,-5.53124494715393));
#180720=CARTESIAN_POINT('Ctrl Pts',(9.43153894431655,15.2,-5.53221208804447));
#180721=CARTESIAN_POINT('Ctrl Pts',(9.43635879077488,15.2,-5.53317376422503));
#180722=CARTESIAN_POINT('Ctrl Pts',(9.44021466815169,15.2,-5.53394310521141));
#180723=CARTESIAN_POINT('Ctrl Pts',(9.44408611842199,15.2,-5.53470894760014));
#180724=CARTESIAN_POINT('Ctrl Pts',(9.44797305696874,15.2,-5.53547119064132));
#180725=CARTESIAN_POINT('Ctrl Pts',(9.4518599949859,15.2,-5.53623343357864));
#180726=CARTESIAN_POINT('Ctrl Pts',(9.45576241973865,15.2,-5.53699207792168));
#180727=CARTESIAN_POINT('Ctrl Pts',(9.45968024721388,15.2,-5.53774702347451));
#180728=CARTESIAN_POINT('Ctrl Pts',(9.46359807522292,15.2,-5.53850196913021));
#180729=CARTESIAN_POINT('Ctrl Pts',(9.46753130493149,15.2,-5.53925321547911));
#180730=CARTESIAN_POINT('Ctrl Pts',(9.47147985220381,15.2,-5.54000066513057));
#180731=CARTESIAN_POINT('Ctrl Pts',(9.4774026725743,15.2,-5.54112183950591));
#180732=CARTESIAN_POINT('Ctrl Pts',(9.48335995373423,15.2,-5.54223447002347));
#180733=CARTESIAN_POINT('Ctrl Pts',(9.48935141601654,15.2,-5.54333822848336));
#180734=CARTESIAN_POINT('Ctrl Pts',(9.49334572456758,15.2,-5.54407406752347));
#180735=CARTESIAN_POINT('Ctrl Pts',(9.49735522241203,15.2,-5.54480596401311));
#180736=CARTESIAN_POINT('Ctrl Pts',(9.50137982713292,15.2,-5.5455338223857));
#180737=CARTESIAN_POINT('Ctrl Pts',(9.50540443130545,15.2,-5.54626168065912));
#180738=CARTESIAN_POINT('Ctrl Pts',(9.50944414219635,15.2,-5.54698550034398));
#180739=CARTESIAN_POINT('Ctrl Pts',(9.51349887627213,15.2,-5.54770518673287));
#180740=CARTESIAN_POINT('Ctrl Pts',(9.51755361090036,15.2,-5.54842487321982));
#180741=CARTESIAN_POINT('Ctrl Pts',(9.52162336779638,15.2,-5.54914042722522));
#180742=CARTESIAN_POINT('Ctrl Pts',(9.52570806640941,15.2,-5.54985175487466));
#180743=CARTESIAN_POINT('Ctrl Pts',(9.5297927644659,15.2,-5.55056308242719));
#180744=CARTESIAN_POINT('Ctrl Pts',(9.53389240050378,15.2,-5.55127018323859));
#180745=CARTESIAN_POINT('Ctrl Pts',(9.53800689588867,15.2,-5.5519729649592));
#180746=CARTESIAN_POINT('Ctrl Pts',(9.54212139183417,15.2,-5.55267574677557));
#180747=CARTESIAN_POINT('Ctrl Pts',(9.54625074530604,15.2,-5.55337421026472));
#180748=CARTESIAN_POINT('Ctrl Pts',(9.55039487418464,15.2,-5.55406826339239));
#180749=CARTESIAN_POINT('Ctrl Pts',(9.55453900249861,15.2,-5.5547623164255));
#180750=CARTESIAN_POINT('Ctrl Pts',(9.5586979055121,15.2,-5.55545195923859));
#180751=CARTESIAN_POINT('Ctrl Pts',(9.56287150239217,15.2,-5.55613710096065));
#180752=CARTESIAN_POINT('Ctrl Pts',(9.56704509984088,15.2,-5.55682224277606));
#180753=CARTESIAN_POINT('Ctrl Pts',(9.57123339133027,15.2,-5.55750288558815));
#180754=CARTESIAN_POINT('Ctrl Pts',(9.57543629589361,15.2,-5.55817893734692));
#180755=CARTESIAN_POINT('Ctrl Pts',(9.57963919988431,15.2,-5.55885498901358));
#180756=CARTESIAN_POINT('Ctrl Pts',(9.58385671533278,15.2,-5.55952645007404));
#180757=CARTESIAN_POINT('Ctrl Pts',(9.58808876241921,15.2,-5.56019323438658));
#180758=CARTESIAN_POINT('Ctrl Pts',(9.59232081008225,15.2,-5.56086001878998));
#180759=CARTESIAN_POINT('Ctrl Pts',(9.59656738975964,15.2,-5.56152212365432));
#180760=CARTESIAN_POINT('Ctrl Pts',(9.6008284198817,15.2,-5.56217946407872));
#180761=CARTESIAN_POINT('Ctrl Pts',(9.6050894494232,15.2,-5.56283680441356));
#180762=CARTESIAN_POINT('Ctrl Pts',(9.6093649313979,15.2,-5.56348937873547));
#180763=CARTESIAN_POINT('Ctrl Pts',(9.6136547823235,15.2,-5.56413710112746));
#180764=CARTESIAN_POINT('Ctrl Pts',(9.61794463383362,15.2,-5.56478482360771));
#180765=CARTESIAN_POINT('Ctrl Pts',(9.62224885688947,15.2,-5.56542769424893));
#180766=CARTESIAN_POINT('Ctrl Pts',(9.62656737097783,15.2,-5.5660656280088));
#180767=CARTESIAN_POINT('Ctrl Pts',(9.6308858844778,15.2,-5.56670356168176));
#180768=CARTESIAN_POINT('Ctrl Pts',(9.63521868957375,15.2,-5.56733655730374));
#180769=CARTESIAN_POINT('Ctrl Pts',(9.63956570577249,15.2,-5.56796453169736));
#180770=CARTESIAN_POINT('Ctrl Pts',(9.6439127225635,15.2,-5.56859250617654));
#180771=CARTESIAN_POINT('Ctrl Pts',(9.64827395159198,15.2,-5.56921545790525));
#180772=CARTESIAN_POINT('Ctrl Pts',(9.65264931244155,15.2,-5.56983330505004));
#180773=CARTESIAN_POINT('Ctrl Pts',(9.65702467329112,15.2,-5.57045115219482));
#180774=CARTESIAN_POINT('Ctrl Pts',(9.661414168709,15.2,-5.57106389414457));
#180775=CARTESIAN_POINT('Ctrl Pts',(9.66581771622821,15.2,-5.57167144739937));
#180776=CARTESIAN_POINT('Ctrl Pts',(9.66912037656762,15.2,-5.57212711229908));
#180777=CARTESIAN_POINT('Ctrl Pts',(9.67243094294588,15.2,-5.57257985988124));
#180778=CARTESIAN_POINT('Ctrl Pts',(9.675749381867,15.2,-5.57302965384536));
#180779=CARTESIAN_POINT('Ctrl Pts',(9.67906782078813,15.2,-5.57347944780948));
#180780=CARTESIAN_POINT('Ctrl Pts',(9.68239413161724,15.2,-5.57392628914808));
#180781=CARTESIAN_POINT('Ctrl Pts',(9.68572828187178,15.2,-5.5743701435067));
#180782=CARTESIAN_POINT('Ctrl Pts',(9.68906243212632,15.2,-5.57481399786531));
#180783=CARTESIAN_POINT('Ctrl Pts',(9.69240442175493,15.2,-5.57525486463261));
#180784=CARTESIAN_POINT('Ctrl Pts',(9.69575421800822,15.2,-5.57569271095004));
#180785=CARTESIAN_POINT('Ctrl Pts',(9.7002206134183,15.2,-5.57627650609296));
#180786=CARTESIAN_POINT('Ctrl Pts',(9.70470088708556,15.2,-5.57685493062416));
#180787=CARTESIAN_POINT('Ctrl Pts',(9.70919496194301,15.2,-5.57742790454371));
#180788=CARTESIAN_POINT('Ctrl Pts',(9.71256551777994,15.2,-5.57785763494435));
#180789=CARTESIAN_POINT('Ctrl Pts',(9.71594383767472,15.2,-5.57828429964321));
#180790=CARTESIAN_POINT('Ctrl Pts',(9.71932988713841,15.2,-5.57870786502362));
#180791=CARTESIAN_POINT('Ctrl Pts',(9.72271593660211,15.2,-5.57913143040403));
#180792=CARTESIAN_POINT('Ctrl Pts',(9.7261097158437,15.2,-5.57955189641091));
#180793=CARTESIAN_POINT('Ctrl Pts',(9.72951119359578,15.2,-5.57996923027047));
#180794=CARTESIAN_POINT('Ctrl Pts',(9.73291267134787,15.2,-5.58038656413004));
#180795=CARTESIAN_POINT('Ctrl Pts',(9.73632184690737,15.2,-5.58080076609831));
#180796=CARTESIAN_POINT('Ctrl Pts',(9.73973868774155,15.2,-5.58121180250004));
#180797=CARTESIAN_POINT('Ctrl Pts',(9.74315552857575,15.2,-5.58162283890177));
#180798=CARTESIAN_POINT('Ctrl Pts',(9.74658003556795,15.2,-5.5820307103203));
#180799=CARTESIAN_POINT('Ctrl Pts',(9.75001217631758,15.2,-5.58243538418087));
#180800=CARTESIAN_POINT('Ctrl Pts',(9.75344431706722,15.2,-5.58284005804145));
#180801=CARTESIAN_POINT('Ctrl Pts',(9.75688409058689,15.2,-5.58324153383382));
#180802=CARTESIAN_POINT('Ctrl Pts',(9.76033146554965,15.2,-5.58363978067296));
#180803=CARTESIAN_POINT('Ctrl Pts',(9.76377884051241,15.2,-5.58403802751209));
#180804=CARTESIAN_POINT('Ctrl Pts',(9.76723381713857,15.2,-5.58443304364509));
#180805=CARTESIAN_POINT('Ctrl Pts',(9.77069636197007,15.2,-5.5848247976313));
#180806=CARTESIAN_POINT('Ctrl Pts',(9.77415890743059,15.2,-5.58521655168868));
#180807=CARTESIAN_POINT('Ctrl Pts',(9.77762902258492,15.2,-5.58560504584514));
#180808=CARTESIAN_POINT('Ctrl Pts',(9.78110667500803,15.2,-5.58599024485901));
#180809=CARTESIAN_POINT('Ctrl Pts',(9.78458432679936,15.2,-5.58637544380289));
#180810=CARTESIAN_POINT('Ctrl Pts',(9.78806951572364,15.2,-5.58675734865529));
#180811=CARTESIAN_POINT('Ctrl Pts',(9.79156220959739,15.2,-5.58713592901625));
#180812=CARTESIAN_POINT('Ctrl Pts',(9.79505490347114,15.2,-5.5875145093772));
#180813=CARTESIAN_POINT('Ctrl Pts',(9.79855510384789,15.2,-5.58788976411221));
#180814=CARTESIAN_POINT('Ctrl Pts',(9.80206277673642,15.2,-5.58826166251704));
#180815=CARTESIAN_POINT('Ctrl Pts',(9.80557044962494,15.2,-5.58863356092187));
#180816=CARTESIAN_POINT('Ctrl Pts',(9.80908559740872,15.2,-5.58900210284463));
#180817=CARTESIAN_POINT('Ctrl Pts',(9.81260818625503,15.2,-5.58936725770804));
#180818=CARTESIAN_POINT('Ctrl Pts',(9.81613077510134,15.2,-5.58973241257145));
#180819=CARTESIAN_POINT('Ctrl Pts',(9.81966080597694,15.2,-5.59009417912365));
#180820=CARTESIAN_POINT('Ctrl Pts',(9.82319824684777,15.2,-5.59045252844425));
#180821=CARTESIAN_POINT('Ctrl Pts',(9.8267356877186,15.2,-5.59081087776486));
#180822=CARTESIAN_POINT('Ctrl Pts',(9.83028054022225,15.2,-5.59116580878571));
#180823=CARTESIAN_POINT('Ctrl Pts',(9.83383277096718,15.2,-5.59151729073175));
#180824=CARTESIAN_POINT('Ctrl Pts',(9.83738500235744,15.2,-5.59186877274163));
#180825=CARTESIAN_POINT('Ctrl Pts',(9.8409446119581,15.2,-5.59221680625888));
#180826=CARTESIAN_POINT('Ctrl Pts',(9.8445115698525,15.2,-5.59256136030848));
#180827=CARTESIAN_POINT('Ctrl Pts',(9.8480785270989,15.2,-5.59290591429549));
#180828=CARTESIAN_POINT('Ctrl Pts',(9.85165283178658,15.2,-5.59324698964935));
#180829=CARTESIAN_POINT('Ctrl Pts',(9.85523445265708,15.2,-5.59358455605344));
#180830=CARTESIAN_POINT('Ctrl Pts',(9.85881607352759,15.2,-5.59392212245753));
#180831=CARTESIAN_POINT('Ctrl Pts',(9.86240501111746,15.2,-5.59425617926086));
#180832=CARTESIAN_POINT('Ctrl Pts',(9.8660012334615,15.2,-5.59458669725034));
#180833=CARTESIAN_POINT('Ctrl Pts',(9.86959745580553,15.2,-5.59491721523981));
#180834=CARTESIAN_POINT('Ctrl Pts',(9.87320096377811,15.2,-5.59524419529334));
#180835=CARTESIAN_POINT('Ctrl Pts',(9.87681172599662,15.2,-5.59556760624141));
#180836=CARTESIAN_POINT('Ctrl Pts',(9.88282966324612,15.2,-5.59610662450777));
#180837=CARTESIAN_POINT('Ctrl Pts',(9.88886774999433,15.2,-5.59663573003893));
#180838=CARTESIAN_POINT('Ctrl Pts',(9.89492584325822,15.2,-5.59715478823337));
#180839=CARTESIAN_POINT('Ctrl Pts',(9.89977231813347,15.2,-5.59757003481156));
#180840=CARTESIAN_POINT('Ctrl Pts',(9.90463159725743,15.2,-5.59797884940844));
#180841=CARTESIAN_POINT('Ctrl Pts',(9.90950360807981,15.2,-5.59838116604082));
#180842=CARTESIAN_POINT('Ctrl Pts',(9.91315761586468,15.2,-5.59868290348769));
#180843=CARTESIAN_POINT('Ctrl Pts',(9.91681878532555,15.2,-5.59898098530338));
#180844=CARTESIAN_POINT('Ctrl Pts',(9.92048708575136,15.2,-5.5992753822653));
#180845=CARTESIAN_POINT('Ctrl Pts',(9.92415538617716,15.2,-5.59956977922721));
#180846=CARTESIAN_POINT('Ctrl Pts',(9.92783081583459,15.2,-5.59986049160868));
#180847=CARTESIAN_POINT('Ctrl Pts',(9.93151334565974,15.2,-5.60014749105626));
#180848=CARTESIAN_POINT('Ctrl Pts',(9.93519587548489,15.2,-5.60043449050385));
#180849=CARTESIAN_POINT('Ctrl Pts',(9.93888550523421,15.2,-5.60071777724353));
#180850=CARTESIAN_POINT('Ctrl Pts',(9.94258220547489,15.2,-5.60099732227504));
#180851=CARTESIAN_POINT('Ctrl Pts',(9.94627890571557,15.2,-5.60127686730655));
#180852=CARTESIAN_POINT('Ctrl Pts',(9.94998267506431,15.2,-5.60155267229654));
#180853=CARTESIAN_POINT('Ctrl Pts',(9.95369348384554,15.2,-5.60182470828699));
#180854=CARTESIAN_POINT('Ctrl Pts',(9.95740429262676,15.2,-5.60209674427743));
#180855=CARTESIAN_POINT('Ctrl Pts',(9.96112214087936,15.2,-5.60236501167812));
#180856=CARTESIAN_POINT('Ctrl Pts',(9.96484699726263,15.2,-5.60262948072384));
#180857=CARTESIAN_POINT('Ctrl Pts',(9.96981347289146,15.2,-5.60298210615015));
#180858=CARTESIAN_POINT('Ctrl Pts',(9.97479240512689,15.2,-5.60332797945966));
#180859=CARTESIAN_POINT('Ctrl Pts',(9.97978372489972,15.2,-5.6036670374777));
#180860=CARTESIAN_POINT('Ctrl Pts',(9.98352721438932,15.2,-5.60392133096812));
#180861=CARTESIAN_POINT('Ctrl Pts',(9.98727767356974,15.2,-5.604171791109));
#180862=CARTESIAN_POINT('Ctrl Pts',(9.99103507297489,15.2,-5.60441839355838));
#180863=CARTESIAN_POINT('Ctrl Pts',(9.99604493930348,15.2,-5.60474719685407));
#180864=CARTESIAN_POINT('Ctrl Pts',(10.0010671467807,15.2,-5.60506914197675));
#180865=CARTESIAN_POINT('Ctrl Pts',(10.0061016120564,15.2,-5.60538415382655));
#180866=CARTESIAN_POINT('Ctrl Pts',(10.0098774606701,15.2,-5.60562041269244));
#180867=CARTESIAN_POINT('Ctrl Pts',(10.0136602026641,15.2,-5.60585277015821));
#180868=CARTESIAN_POINT('Ctrl Pts',(10.0174498052582,15.2,-5.60608119728586));
#180869=CARTESIAN_POINT('Ctrl Pts',(10.0212394078522,15.2,-5.60630962441352));
#180870=CARTESIAN_POINT('Ctrl Pts',(10.0250358702008,15.2,-5.60653412088277));
#180871=CARTESIAN_POINT('Ctrl Pts',(10.0288391798983,15.2,-5.60675467526975));
#180872=CARTESIAN_POINT('Ctrl Pts',(10.0326424895958,15.2,-5.60697522965674));
#180873=CARTESIAN_POINT('Ctrl Pts',(10.0364526483065,15.2,-5.60719184696139));
#180874=CARTESIAN_POINT('Ctrl Pts',(10.0402696489999,15.2,-5.60740451200001));
#180875=CARTESIAN_POINT('Ctrl Pts',(8.88241603299995,12.2,-5.36127880600001));
#180876=CARTESIAN_POINT('Ctrl Pts',(8.88401933304833,12.2,-5.36206719629503));
#180877=CARTESIAN_POINT('Ctrl Pts',(8.88567630917062,12.2,-5.36287598656166));
#180878=CARTESIAN_POINT('Ctrl Pts',(8.8873863638459,12.2,-5.36370417391761));
#180879=CARTESIAN_POINT('Ctrl Pts',(8.88910466526922,12.2,-5.36453635521162));
#180880=CARTESIAN_POINT('Ctrl Pts',(8.89087656280783,12.2,-5.36538812047557));
#180881=CARTESIAN_POINT('Ctrl Pts',(8.89270147741819,12.2,-5.36625848006756));
#180882=CARTESIAN_POINT('Ctrl Pts',(8.89452639186279,12.2,-5.3671288395805));
#180883=CARTESIAN_POINT('Ctrl Pts',(8.89640432496164,12.2,-5.36801779213292));
#180884=CARTESIAN_POINT('Ctrl Pts',(8.89833471330818,12.2,-5.36892438076665));
#180885=CARTESIAN_POINT('Ctrl Pts',(8.90026510165471,12.2,-5.36983096940038));
#180886=CARTESIAN_POINT('Ctrl Pts',(8.90224794607846,12.2,-5.37075519313048));
#180887=CARTESIAN_POINT('Ctrl Pts',(8.90428269376981,12.2,-5.37169612014234));
#180888=CARTESIAN_POINT('Ctrl Pts',(8.90631744164601,12.2,-5.37263704723965));
#180889=CARTESIAN_POINT('Ctrl Pts',(8.90840409644624,12.2,-5.37359467979364));
#180890=CARTESIAN_POINT('Ctrl Pts',(8.91054211906624,12.2,-5.37456811359776));
#180891=CARTESIAN_POINT('Ctrl Pts',(8.91268014149207,12.2,-5.37554154731347));
#180892=CARTESIAN_POINT('Ctrl Pts',(8.91486953043031,12.2,-5.37653078087401));
#180893=CARTESIAN_POINT('Ctrl Pts',(8.91710976394254,12.2,-5.37753493975878));
#180894=CARTESIAN_POINT('Ctrl Pts',(8.91934999745478,12.2,-5.37853909864355));
#180895=CARTESIAN_POINT('Ctrl Pts',(8.92164107324306,12.2,-5.37955818039023));
#180896=CARTESIAN_POINT('Ctrl Pts',(8.92398247965579,12.2,-5.38059133443541));
#180897=CARTESIAN_POINT('Ctrl Pts',(8.9263238862812,12.2,-5.38162448857445));
#180898=CARTESIAN_POINT('Ctrl Pts',(8.92871562078788,12.2,-5.38267171456523));
#180899=CARTESIAN_POINT('Ctrl Pts',(8.93115718350766,12.2,-5.38373218387392));
#180900=CARTESIAN_POINT('Ctrl Pts',(8.93359874600567,12.2,-5.38479265308629));
#180901=CARTESIAN_POINT('Ctrl Pts',(8.93609013491204,12.2,-5.38586636586483));
#180902=CARTESIAN_POINT('Ctrl Pts',(8.9386308586552,12.2,-5.3869525153259));
#180903=CARTESIAN_POINT('Ctrl Pts',(8.94117158239835,12.2,-5.38803866478697));
#180904=CARTESIAN_POINT('Ctrl Pts',(8.94376164092926,12.2,-5.38913725330539));
#180905=CARTESIAN_POINT('Ctrl Pts',(8.94640055158124,12.2,-5.3902474946812));
#180906=CARTESIAN_POINT('Ctrl Pts',(8.94903946223323,12.2,-5.39135773605702));
#180907=CARTESIAN_POINT('Ctrl Pts',(8.95172722686268,12.2,-5.39247963096843));
#180908=CARTESIAN_POINT('Ctrl Pts',(8.95446336867663,12.2,-5.39361241742653));
#180909=CARTESIAN_POINT('Ctrl Pts',(8.95719951073912,12.2,-5.39474520398751));
#180910=CARTESIAN_POINT('Ctrl Pts',(8.95998403506464,12.2,-5.39588888035792));
#180911=CARTESIAN_POINT('Ctrl Pts',(8.9628164732211,12.2,-5.39704270583792));
#180912=CARTESIAN_POINT('Ctrl Pts',(8.96564891112028,12.2,-5.39819653121312));
#180913=CARTESIAN_POINT('Ctrl Pts',(8.96852926582505,12.2,-5.39936050395345));
#180914=CARTESIAN_POINT('Ctrl Pts',(8.97145708073186,12.2,-5.40053389974946));
#180915=CARTESIAN_POINT('Ctrl Pts',(8.97438489563868,12.2,-5.40170729554548));
#180916=CARTESIAN_POINT('Ctrl Pts',(8.97736017116679,12.2,-5.402890118114));
#180917=CARTESIAN_POINT('Ctrl Pts',(8.98038246188711,12.2,-5.40408165690346));
#180918=CARTESIAN_POINT('Ctrl Pts',(8.98340475288196,12.2,-5.40527319580113));
#180919=CARTESIAN_POINT('Ctrl Pts',(8.98647405673137,12.2,-5.40647345299135));
#180920=CARTESIAN_POINT('Ctrl Pts',(8.98958993590321,12.2,-5.40768174280755));
#180921=CARTESIAN_POINT('Ctrl Pts',(8.99270581479201,12.2,-5.408890032514));
#180922=CARTESIAN_POINT('Ctrl Pts',(8.99586827068388,12.2,-5.41010635178838));
#180923=CARTESIAN_POINT('Ctrl Pts',(8.99907686774841,12.2,-5.41133003174945));
#180924=CARTESIAN_POINT('Ctrl Pts',(9.00228546481295,12.2,-5.41255371171051));
#180925=CARTESIAN_POINT('Ctrl Pts',(9.00554020763815,12.2,-5.41378475248552));
#180926=CARTESIAN_POINT('Ctrl Pts',(9.00884067043179,12.2,-5.41502249935676));
#180927=CARTESIAN_POINT('Ctrl Pts',(9.01214113352523,12.2,-5.41626024634042));
#180928=CARTESIAN_POINT('Ctrl Pts',(9.01548731562951,12.2,-5.41750469859001));
#180929=CARTESIAN_POINT('Ctrl Pts',(9.01887880106974,12.2,-5.41875521888766));
#180930=CARTESIAN_POINT('Ctrl Pts',(9.02227028620191,12.2,-5.42000573907171));
#180931=CARTESIAN_POINT('Ctrl Pts',(9.02570707445971,12.2,-5.4212623260792));
#180932=CARTESIAN_POINT('Ctrl Pts',(9.02918875449986,12.2,-5.4225243582));
#180933=CARTESIAN_POINT('Ctrl Pts',(9.03267043454002,12.2,-5.42378639032082));
#180934=CARTESIAN_POINT('Ctrl Pts',(9.03619700805011,12.2,-5.42505386519323));
#180935=CARTESIAN_POINT('Ctrl Pts',(9.03976807017952,12.2,-5.42632617637694));
#180936=CARTESIAN_POINT('Ctrl Pts',(9.04333913263329,12.2,-5.42759848767622));
#180937=CARTESIAN_POINT('Ctrl Pts',(9.046954682613,12.2,-5.42887563343622));
#180938=CARTESIAN_POINT('Ctrl Pts',(9.05061432498211,12.2,-5.43015702067301));
#180939=CARTESIAN_POINT('Ctrl Pts',(9.05427396701881,12.2,-5.43143840779341));
#180940=CARTESIAN_POINT('Ctrl Pts',(9.05797769955396,12.2,-5.43272403534991));
#180941=CARTESIAN_POINT('Ctrl Pts',(9.06172513076824,12.2,-5.43401332172559));
#180942=CARTESIAN_POINT('Ctrl Pts',(9.06547256198253,12.2,-5.43530260810128));
#180943=CARTESIAN_POINT('Ctrl Pts',(9.06926369413228,12.2,-5.43659555510162));
#180944=CARTESIAN_POINT('Ctrl Pts',(9.07309813832441,12.2,-5.43789159247105));
#180945=CARTESIAN_POINT('Ctrl Pts',(9.0762935086006,12.2,-5.4389716236515));
#180946=CARTESIAN_POINT('Ctrl Pts',(9.07951895779428,12.2,-5.44005380197366));
#180947=CARTESIAN_POINT('Ctrl Pts',(9.08277426473715,12.2,-5.44113780565413));
#180948=CARTESIAN_POINT('Ctrl Pts',(9.08602957168004,12.2,-5.44222180933458));
#180949=CARTESIAN_POINT('Ctrl Pts',(9.08931473772756,12.2,-5.44330763708894));
#180950=CARTESIAN_POINT('Ctrl Pts',(9.09262954371475,12.2,-5.44439497494109));
#180951=CARTESIAN_POINT('Ctrl Pts',(9.09594434970194,12.2,-5.44548231279324));
#180952=CARTESIAN_POINT('Ctrl Pts',(9.09928879517208,12.2,-5.44657115787779));
#180953=CARTESIAN_POINT('Ctrl Pts',(9.1026626662832,12.2,-5.44766120322501));
#180954=CARTESIAN_POINT('Ctrl Pts',(9.10603653739431,12.2,-5.44875124857224));
#180955=CARTESIAN_POINT('Ctrl Pts',(9.1094398338694,12.2,-5.44984249195675));
#180956=CARTESIAN_POINT('Ctrl Pts',(9.11287234096841,12.2,-5.45093462918394));
#180957=CARTESIAN_POINT('Ctrl Pts',(9.11630484806743,12.2,-5.45202676641113));
#180958=CARTESIAN_POINT('Ctrl Pts',(9.11976656888795,12.2,-5.45311979772707));
#180959=CARTESIAN_POINT('Ctrl Pts',(9.12325728923667,12.2,-5.45421342404654));
#180960=CARTESIAN_POINT('Ctrl Pts',(9.12674800958541,12.2,-5.45530705036601));
#180961=CARTESIAN_POINT('Ctrl Pts',(9.13026773206949,12.2,-5.45640127022158));
#180962=CARTESIAN_POINT('Ctrl Pts',(9.13381624651545,12.2,-5.45749579230493));
#180963=CARTESIAN_POINT('Ctrl Pts',(9.1373647609614,12.2,-5.45859031438828));
#180964=CARTESIAN_POINT('Ctrl Pts',(9.14094206858089,12.2,-5.45968513537797));
#180965=CARTESIAN_POINT('Ctrl Pts',(9.14454796244356,12.2,-5.46077997008544));
#180966=CARTESIAN_POINT('Ctrl Pts',(9.14815385630625,12.2,-5.46187480479292));
#180967=CARTESIAN_POINT('Ctrl Pts',(9.15178833685444,12.2,-5.4629696504932));
#180968=CARTESIAN_POINT('Ctrl Pts',(9.15545119970399,12.2,-5.46406422445152));
#180969=CARTESIAN_POINT('Ctrl Pts',(9.15911406255353,12.2,-5.46515879840983));
#180970=CARTESIAN_POINT('Ctrl Pts',(9.16280530803408,12.2,-5.46625309921534));
#180971=CARTESIAN_POINT('Ctrl Pts',(9.16652473491139,12.2,-5.46734685136808));
#180972=CARTESIAN_POINT('Ctrl Pts',(9.17024416138328,12.2,-5.46844060340159));
#180973=CARTESIAN_POINT('Ctrl Pts',(9.17399176781987,12.2,-5.46953380356503));
#180974=CARTESIAN_POINT('Ctrl Pts',(9.17776735448937,12.2,-5.47062617914047));
#180975=CARTESIAN_POINT('Ctrl Pts',(9.18154294157041,12.2,-5.47171855483498));
#180976=CARTESIAN_POINT('Ctrl Pts',(9.18534651057879,12.2,-5.47281010628507));
#180977=CARTESIAN_POINT('Ctrl Pts',(9.18917786092375,12.2,-5.47390056288239));
#180978=CARTESIAN_POINT('Ctrl Pts',(9.1930092112687,12.2,-5.47499101947969));
#180979=CARTESIAN_POINT('Ctrl Pts',(9.19686834516041,12.2,-5.47608038108537));
#180980=CARTESIAN_POINT('Ctrl Pts',(9.20075506474151,12.2,-5.47716838434937));
#180981=CARTESIAN_POINT('Ctrl Pts',(9.2046417843226,12.2,-5.47825638761337));
#180982=CARTESIAN_POINT('Ctrl Pts',(9.2085560911085,12.2,-5.47934303048085));
#180983=CARTESIAN_POINT('Ctrl Pts',(9.21249779081741,12.2,-5.48042805463239));
#180984=CARTESIAN_POINT('Ctrl Pts',(9.21643949052631,12.2,-5.48151307878393));
#180985=CARTESIAN_POINT('Ctrl Pts',(9.22040858133456,12.2,-5.48259648263473));
#180986=CARTESIAN_POINT('Ctrl Pts',(9.22440487251368,12.2,-5.48367801020428));
#180987=CARTESIAN_POINT('Ctrl Pts',(9.22840116369281,12.2,-5.48475953777381));
#180988=CARTESIAN_POINT('Ctrl Pts',(9.23242465490877,12.2,-5.48583919049053));
#180989=CARTESIAN_POINT('Ctrl Pts',(9.23647515601847,12.2,-5.48691671396287));
#180990=CARTESIAN_POINT('Ctrl Pts',(9.23971555708284,12.2,-5.48777873278772));
#180991=CARTESIAN_POINT('Ctrl Pts',(9.24297324329827,12.2,-5.48863939026006));
#180992=CARTESIAN_POINT('Ctrl Pts',(9.24624811997518,12.2,-5.48949855784968));
#180993=CARTESIAN_POINT('Ctrl Pts',(9.24952299620589,12.2,-5.49035772532223));
#180994=CARTESIAN_POINT('Ctrl Pts',(9.25281506078727,12.2,-5.49121540546935));
#180995=CARTESIAN_POINT('Ctrl Pts',(9.25612421823785,12.2,-5.49207146945502));
#180996=CARTESIAN_POINT('Ctrl Pts',(9.25943337613931,12.2,-5.49292753355734));
#180997=CARTESIAN_POINT('Ctrl Pts',(9.26275962842059,12.2,-5.49378198385947));
#180998=CARTESIAN_POINT('Ctrl Pts',(9.26610287754835,12.2,-5.49463469529471));
#180999=CARTESIAN_POINT('Ctrl Pts',(9.2694461262206,12.2,-5.49548740661378));
#181000=CARTESIAN_POINT('Ctrl Pts',(9.27280637185487,12.2,-5.4963383795203));
#181001=CARTESIAN_POINT('Ctrl Pts',(9.27618352146826,12.2,-5.49718749216014));
#181002=CARTESIAN_POINT('Ctrl Pts',(9.27956067154179,12.2,-5.49803660491565));
#181003=CARTESIAN_POINT('Ctrl Pts',(9.28295472381133,12.2,-5.49888385620928));
#181004=CARTESIAN_POINT('Ctrl Pts',(9.28636558505388,12.2,-5.49972912631077));
#181005=CARTESIAN_POINT('Ctrl Pts',(9.29062916137468,12.2,-5.50078571388004));
#181006=CARTESIAN_POINT('Ctrl Pts',(9.29491900179762,12.2,-5.50183920530774));
#181007=CARTESIAN_POINT('Ctrl Pts',(9.29923492304898,12.2,-5.50288936787702));
#181008=CARTESIAN_POINT('Ctrl Pts',(9.30355084430034,12.2,-5.50393953044628));
#181009=CARTESIAN_POINT('Ctrl Pts',(9.30789284614257,12.2,-5.50498636390258));
#181010=CARTESIAN_POINT('Ctrl Pts',(9.31226074851535,12.2,-5.50602964062112));
#181011=CARTESIAN_POINT('Ctrl Pts',(9.31575507012792,12.2,-5.50686426192772));
#181012=CARTESIAN_POINT('Ctrl Pts',(9.31926596793444,12.2,-5.50769660579151));
#181013=CARTESIAN_POINT('Ctrl Pts',(9.32279334997834,12.2,-5.50852655789049));
#181014=CARTESIAN_POINT('Ctrl Pts',(9.32632073250284,12.2,-5.50935651010254));
#181015=CARTESIAN_POINT('Ctrl Pts',(9.32986459862931,12.2,-5.51018406957821));
#181016=CARTESIAN_POINT('Ctrl Pts',(9.33342485782442,12.2,-5.51100912306745));
#181017=CARTESIAN_POINT('Ctrl Pts',(9.33698511653444,12.2,-5.51183417644428));
#181018=CARTESIAN_POINT('Ctrl Pts',(9.34056176862204,12.2,-5.5126567232791));
#181019=CARTESIAN_POINT('Ctrl Pts',(9.34415472172861,12.2,-5.51347665136437));
#181020=CARTESIAN_POINT('Ctrl Pts',(9.34774767532473,12.2,-5.51429657956135));
#181021=CARTESIAN_POINT('Ctrl Pts',(9.35135693103388,12.2,-5.51511388801682));
#181022=CARTESIAN_POINT('Ctrl Pts',(9.35498239828808,12.2,-5.51592846628326));
#181023=CARTESIAN_POINT('Ctrl Pts',(9.35860786504831,12.2,-5.51674304443871));
#181024=CARTESIAN_POINT('Ctrl Pts',(9.36224954469418,12.2,-5.51755489178915));
#181025=CARTESIAN_POINT('Ctrl Pts',(9.36590734489351,12.2,-5.51836389983442));
#181026=CARTESIAN_POINT('Ctrl Pts',(9.36956514559122,12.2,-5.51917290798992));
#181027=CARTESIAN_POINT('Ctrl Pts',(9.37323906983727,12.2,-5.51997907373927));
#181028=CARTESIAN_POINT('Ctrl Pts',(9.3769290257774,12.2,-5.52078229250891));
#181029=CARTESIAN_POINT('Ctrl Pts',(9.38061898121478,12.2,-5.52158551116911));
#181030=CARTESIAN_POINT('Ctrl Pts',(9.38432496933614,12.2,-5.52238578031232));
#181031=CARTESIAN_POINT('Ctrl Pts',(9.38804690214135,12.2,-5.52318299313635));
#181032=CARTESIAN_POINT('Ctrl Pts',(9.39176883545368,12.2,-5.52398020606899));
#181033=CARTESIAN_POINT('Ctrl Pts',(9.3955067129203,12.2,-5.52477436240414));
#181034=CARTESIAN_POINT('Ctrl Pts',(9.39926044629154,12.2,-5.52556535672503));
#181035=CARTESIAN_POINT('Ctrl Pts',(9.40301417966279,12.2,-5.52635635104592));
#181036=CARTESIAN_POINT('Ctrl Pts',(9.40678376934421,12.2,-5.52714418338032));
#181037=CARTESIAN_POINT('Ctrl Pts',(9.41056912788546,12.2,-5.52792874831163));
#181038=CARTESIAN_POINT('Ctrl Pts',(9.41530082528839,12.2,-5.52890945431543));
#181039=CARTESIAN_POINT('Ctrl Pts',(9.42005716186988,12.2,-5.52988505572844));
#181040=CARTESIAN_POINT('Ctrl Pts',(9.42483796537456,12.2,-5.53085534937311));
#181041=CARTESIAN_POINT('Ctrl Pts',(9.42866260880363,12.2,-5.53163158441576));
#181042=CARTESIAN_POINT('Ctrl Pts',(9.43250291339807,12.2,-5.53240442323866));
#181043=CARTESIAN_POINT('Ctrl Pts',(9.43635879077488,12.2,-5.53317376422503));
#181044=CARTESIAN_POINT('Ctrl Pts',(9.44021466815169,12.2,-5.53394310521141));
#181045=CARTESIAN_POINT('Ctrl Pts',(9.44408611842199,12.2,-5.53470894760014));
#181046=CARTESIAN_POINT('Ctrl Pts',(9.44797305696874,12.2,-5.53547119064132));
#181047=CARTESIAN_POINT('Ctrl Pts',(9.4518599949859,12.2,-5.53623343357864));
#181048=CARTESIAN_POINT('Ctrl Pts',(9.45576241973865,12.2,-5.53699207792168));
#181049=CARTESIAN_POINT('Ctrl Pts',(9.45968024721388,12.2,-5.53774702347451));
#181050=CARTESIAN_POINT('Ctrl Pts',(9.46359807522292,12.2,-5.53850196913021));
#181051=CARTESIAN_POINT('Ctrl Pts',(9.46753130493149,12.2,-5.53925321547911));
#181052=CARTESIAN_POINT('Ctrl Pts',(9.47147985220381,12.2,-5.54000066513057));
#181053=CARTESIAN_POINT('Ctrl Pts',(9.47542839893814,12.2,-5.54074811468018));
#181054=CARTESIAN_POINT('Ctrl Pts',(9.47939226273157,12.2,-5.54149176731641));
#181055=CARTESIAN_POINT('Ctrl Pts',(9.48337135768307,12.2,-5.54223152492285));
#181056=CARTESIAN_POINT('Ctrl Pts',(9.48735045317672,12.2,-5.5429712826301));
#181057=CARTESIAN_POINT('Ctrl Pts',(9.49134478323052,12.2,-5.54370714562297));
#181058=CARTESIAN_POINT('Ctrl Pts',(9.49535426056114,12.2,-5.54443901805149));
#181059=CARTESIAN_POINT('Ctrl Pts',(9.49936373734546,12.2,-5.54517089038029));
#181060=CARTESIAN_POINT('Ctrl Pts',(9.50338836268796,12.2,-5.54589877263153));
#181061=CARTESIAN_POINT('Ctrl Pts',(9.50742805244712,12.2,-5.54662256888665));
#181062=CARTESIAN_POINT('Ctrl Pts',(9.51146774275668,12.2,-5.54734636524039));
#181063=CARTESIAN_POINT('Ctrl Pts',(9.51552249811828,12.2,-5.54806607542254));
#181064=CARTESIAN_POINT('Ctrl Pts',(9.51959223484106,12.2,-5.54878160585015));
#181065=CARTESIAN_POINT('Ctrl Pts',(9.52366197100934,12.2,-5.54949713618028));
#181066=CARTESIAN_POINT('Ctrl Pts',(9.52774669062739,12.2,-5.55020848671123));
#181067=CARTESIAN_POINT('Ctrl Pts',(9.53184630684628,12.2,-5.55091556437609));
#181068=CARTESIAN_POINT('Ctrl Pts',(9.53594592362374,12.2,-5.55162264213728));
#181069=CARTESIAN_POINT('Ctrl Pts',(9.54006044054218,12.2,-5.55232544711206));
#181070=CARTESIAN_POINT('Ctrl Pts',(9.54418977278604,12.2,-5.55302388754217));
#181071=CARTESIAN_POINT('Ctrl Pts',(9.54831910446727,12.2,-5.55372232787712));
#181072=CARTESIAN_POINT('Ctrl Pts',(9.55246325326141,12.2,-5.55441640364321));
#181073=CARTESIAN_POINT('Ctrl Pts',(9.55662213658658,12.2,-5.55510602392061));
#181074=CARTESIAN_POINT('Ctrl Pts',(9.5607810204784,12.2,-5.55579564429198));
#181075=CARTESIAN_POINT('Ctrl Pts',(9.56495463846884,12.2,-5.55648080801572));
#181076=CARTESIAN_POINT('Ctrl Pts',(9.56914290930821,12.2,-5.55716142777503));
#181077=CARTESIAN_POINT('Ctrl Pts',(9.57333118014759,12.2,-5.55784204753435));
#181078=CARTESIAN_POINT('Ctrl Pts',(9.57753410486645,12.2,-5.55851812109313));
#181079=CARTESIAN_POINT('Ctrl Pts',(9.58175160093112,12.2,-5.55918956085148));
#181080=CARTESIAN_POINT('Ctrl Pts',(9.58596909642116,12.2,-5.55986100051834));
#181081=CARTESIAN_POINT('Ctrl Pts',(9.59020116373047,12.2,-5.5605278073118));
#181082=CARTESIAN_POINT('Ctrl Pts',(9.59444772251367,12.2,-5.56118989048292));
#181083=CARTESIAN_POINT('Ctrl Pts',(9.59975592142659,12.2,-5.56201749451447));
#181084=CARTESIAN_POINT('Ctrl Pts',(9.60508676277765,12.2,-5.56283772212781));
#181085=CARTESIAN_POINT('Ctrl Pts',(9.61044008999988,12.2,-5.5636504010167));
#181086=CARTESIAN_POINT('Ctrl Pts',(9.61472275201107,12.2,-5.56430054416324));
#181087=CARTESIAN_POINT('Ctrl Pts',(9.61901980376281,12.2,-5.56494585625644));
#181088=CARTESIAN_POINT('Ctrl Pts',(9.62333116722147,12.2,-5.5655862533464));
#181089=CARTESIAN_POINT('Ctrl Pts',(9.6276425300927,12.2,-5.5662266503491));
#181090=CARTESIAN_POINT('Ctrl Pts',(9.63196820452373,12.2,-5.5668621301816));
#181091=CARTESIAN_POINT('Ctrl Pts',(9.63630811002193,12.2,-5.56749261046627));
#181092=CARTESIAN_POINT('Ctrl Pts',(9.64064801611146,12.2,-5.56812309083684));
#181093=CARTESIAN_POINT('Ctrl Pts',(9.64500215450515,12.2,-5.56874856932373));
#181094=CARTESIAN_POINT('Ctrl Pts',(9.64937044402245,12.2,-5.56936896380147));
#181095=CARTESIAN_POINT('Ctrl Pts',(9.65373873294456,12.2,-5.56998935819468));
#181096=CARTESIAN_POINT('Ctrl Pts',(9.65812117542594,12.2,-5.57060466827187));
#181097=CARTESIAN_POINT('Ctrl Pts',(9.66251769089894,12.2,-5.57121481066678));
#181098=CARTESIAN_POINT('Ctrl Pts',(9.66581507765345,12.2,-5.57167241748373));
#181099=CARTESIAN_POINT('Ctrl Pts',(9.66912038021472,12.2,-5.57212711718944));
#181100=CARTESIAN_POINT('Ctrl Pts',(9.67243356713395,12.2,-5.57257887644593));
#181101=CARTESIAN_POINT('Ctrl Pts',(9.67574675405318,12.2,-5.57303063570243));
#181102=CARTESIAN_POINT('Ctrl Pts',(9.67906782446287,12.2,-5.57347945283529));
#181103=CARTESIAN_POINT('Ctrl Pts',(9.68239674475753,12.2,-5.57392529469451));
#181104=CARTESIAN_POINT('Ctrl Pts',(9.68572566565693,12.2,-5.57437113663471));
#181105=CARTESIAN_POINT('Ctrl Pts',(9.68906243685854,12.2,-5.57481400329908));
#181106=CARTESIAN_POINT('Ctrl Pts',(9.69240702572069,12.2,-5.57525385936259));
#181107=CARTESIAN_POINT('Ctrl Pts',(9.69575161397524,12.2,-5.5756937153462));
#181108=CARTESIAN_POINT('Ctrl Pts',(9.69910401937102,12.2,-5.57613056264663));
#181109=CARTESIAN_POINT('Ctrl Pts',(9.70246421008295,12.2,-5.5765643660056));
#181110=CARTESIAN_POINT('Ctrl Pts',(9.70582440079487,12.2,-5.57699816936458));
#181111=CARTESIAN_POINT('Ctrl Pts',(9.70919237582691,12.2,-5.5774289287807));
#181112=CARTESIAN_POINT('Ctrl Pts',(9.71256810401129,12.2,-5.57785661201709));
#181113=CARTESIAN_POINT('Ctrl Pts',(9.71706907471938,12.2,-5.57842685630638));
#181114=CARTESIAN_POINT('Ctrl Pts',(9.72158382644498,12.2,-5.57899162970374));
#181115=CARTESIAN_POINT('Ctrl Pts',(9.72611228201783,12.2,-5.5795508536586));
#181116=CARTESIAN_POINT('Ctrl Pts',(9.72950862446872,12.2,-5.57997027171998));
#181117=CARTESIAN_POINT('Ctrl Pts',(9.73291267654677,12.2,-5.58038656936382));
#181118=CARTESIAN_POINT('Ctrl Pts',(9.73632440400199,12.2,-5.5807997123401));
#181119=CARTESIAN_POINT('Ctrl Pts',(9.74087337290928,12.2,-5.58135056951672));
#181120=CARTESIAN_POINT('Ctrl Pts',(9.74543598885924,12.2,-5.58189581905794));
#181121=CARTESIAN_POINT('Ctrl Pts',(9.75001217631758,12.2,-5.58243538418087));
#181122=CARTESIAN_POINT('Ctrl Pts',(9.75344431706722,12.2,-5.58284005804145));
#181123=CARTESIAN_POINT('Ctrl Pts',(9.75688409058689,12.2,-5.58324153383382));
#181124=CARTESIAN_POINT('Ctrl Pts',(9.76033146554965,12.2,-5.58363978067296));
#181125=CARTESIAN_POINT('Ctrl Pts',(9.76377884051241,12.2,-5.58403802751209));
#181126=CARTESIAN_POINT('Ctrl Pts',(9.76723381713857,12.2,-5.58443304364509));
#181127=CARTESIAN_POINT('Ctrl Pts',(9.77069636197007,12.2,-5.5848247976313));
#181128=CARTESIAN_POINT('Ctrl Pts',(9.77415890743059,12.2,-5.58521655168868));
#181129=CARTESIAN_POINT('Ctrl Pts',(9.77762902258492,12.2,-5.58560504584514));
#181130=CARTESIAN_POINT('Ctrl Pts',(9.78110667500803,12.2,-5.58599024485901));
#181131=CARTESIAN_POINT('Ctrl Pts',(9.78458432679936,12.2,-5.58637544380289));
#181132=CARTESIAN_POINT('Ctrl Pts',(9.78806951572364,12.2,-5.58675734865529));
#181133=CARTESIAN_POINT('Ctrl Pts',(9.79156220959739,12.2,-5.58713592901625));
#181134=CARTESIAN_POINT('Ctrl Pts',(9.79505490347114,12.2,-5.5875145093772));
#181135=CARTESIAN_POINT('Ctrl Pts',(9.79855510384789,12.2,-5.58788976411221));
#181136=CARTESIAN_POINT('Ctrl Pts',(9.80206277673642,12.2,-5.58826166251704));
#181137=CARTESIAN_POINT('Ctrl Pts',(9.8067396737087,12.2,-5.5887575270343));
#181138=CARTESIAN_POINT('Ctrl Pts',(9.81142985850841,12.2,-5.58924742503764));
#181139=CARTESIAN_POINT('Ctrl Pts',(9.8161332539559,12.2,-5.58973128222093));
#181140=CARTESIAN_POINT('Ctrl Pts',(9.81966080134256,12.2,-5.59009417519079));
#181141=CARTESIAN_POINT('Ctrl Pts',(9.82319577937296,12.2,-5.59045367035971));
#181142=CARTESIAN_POINT('Ctrl Pts',(9.8267381582638,12.2,-5.59080973736932));
#181143=CARTESIAN_POINT('Ctrl Pts',(9.8302805365111,12.2,-5.59116580431426));
#181144=CARTESIAN_POINT('Ctrl Pts',(9.83383031526635,12.2,-5.59151844253437));
#181145=CARTESIAN_POINT('Ctrl Pts',(9.83738746117941,12.2,-5.59186762197971));
#181146=CARTESIAN_POINT('Ctrl Pts',(9.84094460709248,12.2,-5.59221680142505));
#181147=CARTESIAN_POINT('Ctrl Pts',(9.84450912232966,12.2,-5.59256252206248));
#181148=CARTESIAN_POINT('Ctrl Pts',(9.84808097419989,12.2,-5.59290475350837));
#181149=CARTESIAN_POINT('Ctrl Pts',(9.85165282607011,12.2,-5.59324698495427));
#181150=CARTESIAN_POINT('Ctrl Pts',(9.85523201532336,12.2,-5.59358572800864));
#181151=CARTESIAN_POINT('Ctrl Pts',(9.85881851056742,12.2,-5.59392095145511));
#181152=CARTESIAN_POINT('Ctrl Pts',(9.86240500581147,12.2,-5.59425617490156));
#181153=CARTESIAN_POINT('Ctrl Pts',(9.86599880662169,12.2,-5.5945878787483));
#181154=CARTESIAN_POINT('Ctrl Pts',(9.86959988258658,12.2,-5.59491603466985));
#181155=CARTESIAN_POINT('Ctrl Pts',(9.87320095855147,12.2,-5.5952441905914));
#181156=CARTESIAN_POINT('Ctrl Pts',(9.87680930991072,12.2,-5.5955687979579));
#181157=CARTESIAN_POINT('Ctrl Pts',(9.8804249042367,12.2,-5.59588982644672));
#181158=CARTESIAN_POINT('Ctrl Pts',(9.88524569710923,12.2,-5.5963178644707));
#181159=CARTESIAN_POINT('Ctrl Pts',(9.89007936838298,12.2,-5.59673954165519));
#181160=CARTESIAN_POINT('Ctrl Pts',(9.89492584325822,12.2,-5.59715478823337));
#181161=CARTESIAN_POINT('Ctrl Pts',(9.89856069908449,12.2,-5.59746622313872));
#181162=CARTESIAN_POINT('Ctrl Pts',(9.90220275683546,12.2,-5.59777404024422));
#181163=CARTESIAN_POINT('Ctrl Pts',(9.90585198707725,12.2,-5.59807821123349));
#181164=CARTESIAN_POINT('Ctrl Pts',(9.90950121731904,12.2,-5.59838238222276));
#181165=CARTESIAN_POINT('Ctrl Pts',(9.91315761837541,12.2,-5.59868290817144));
#181166=CARTESIAN_POINT('Ctrl Pts',(9.91682116175783,12.2,-5.59897975821757));
#181167=CARTESIAN_POINT('Ctrl Pts',(9.92170588671141,12.2,-5.59937555831504));
#181168=CARTESIAN_POINT('Ctrl Pts',(9.92660330544688,12.2,-5.59976482509139));
#181169=CARTESIAN_POINT('Ctrl Pts',(9.93151334565974,12.2,-5.60014749105626));
#181170=CARTESIAN_POINT('Ctrl Pts',(9.93519587548489,12.2,-5.60043449050385));
#181171=CARTESIAN_POINT('Ctrl Pts',(9.93888550523421,12.2,-5.60071777724353));
#181172=CARTESIAN_POINT('Ctrl Pts',(9.94258220547489,12.2,-5.60099732227504));
#181173=CARTESIAN_POINT('Ctrl Pts',(9.94627890571557,12.2,-5.60127686730655));
#181174=CARTESIAN_POINT('Ctrl Pts',(9.94998267506431,12.2,-5.60155267229654));
#181175=CARTESIAN_POINT('Ctrl Pts',(9.95369348384554,12.2,-5.60182470828699));
#181176=CARTESIAN_POINT('Ctrl Pts',(9.95740429262676,12.2,-5.60209674427743));
#181177=CARTESIAN_POINT('Ctrl Pts',(9.96112214087936,12.2,-5.60236501167812));
#181178=CARTESIAN_POINT('Ctrl Pts',(9.96484699726263,12.2,-5.60262948072384));
#181179=CARTESIAN_POINT('Ctrl Pts',(9.96857185364591,12.2,-5.60289394976955));
#181180=CARTESIAN_POINT('Ctrl Pts',(9.97230371650496,12.2,-5.60315462115286));
#181181=CARTESIAN_POINT('Ctrl Pts',(9.97604255774317,12.2,-5.60341146722738));
#181182=CARTESIAN_POINT('Ctrl Pts',(9.9797813996606,12.2,-5.60366831334856));
#181183=CARTESIAN_POINT('Ctrl Pts',(9.98352721885499,12.2,-5.60392133440201));
#181184=CARTESIAN_POINT('Ctrl Pts',(9.98727998885967,12.2,-5.60417050597936));
#181185=CARTESIAN_POINT('Ctrl Pts',(9.99103275818261,12.2,-5.60441967751145));
#181186=CARTESIAN_POINT('Ctrl Pts',(9.99479247849683,12.2,-5.60466500045207));
#181187=CARTESIAN_POINT('Ctrl Pts',(9.99855911819391,12.2,-5.60490644531796));
#181188=CARTESIAN_POINT('Ctrl Pts',(10.002325757891,12.2,-5.60514789018385));
#181189=CARTESIAN_POINT('Ctrl Pts',(10.0060993160735,12.2,-5.60538545632437));
#181190=CARTESIAN_POINT('Ctrl Pts',(10.0098797567867,12.2,-5.60561911123359));
#181191=CARTESIAN_POINT('Ctrl Pts',(10.0136601974998,12.2,-5.60585276614281));
#181192=CARTESIAN_POINT('Ctrl Pts',(10.0174475189171,12.2,-5.60608250832366));
#181193=CARTESIAN_POINT('Ctrl Pts',(10.0212416935048,12.2,-5.60630831402483));
#181194=CARTESIAN_POINT('Ctrl Pts',(10.0275653180473,12.2,-5.60668465687379));
#181195=CARTESIAN_POINT('Ctrl Pts',(10.0339079809464,12.2,-5.6070500702561));
#181196=CARTESIAN_POINT('Ctrl Pts',(10.0402696489999,12.2,-5.60740451200001));
#181197=CARTESIAN_POINT('Origin',(-5.66257110645729E-14,15.2,-1.77635683940025E-14));
#181198=CARTESIAN_POINT('',(9.55499537054798,15.2,-4.04260911609085));
#181199=CARTESIAN_POINT('',(9.55499537054798,12.2,-4.04260911609085));
#181200=CARTESIAN_POINT('',(9.55499536999995,15.2,-4.04260911600002));
#181201=CARTESIAN_POINT('Origin',(-5.66257110645729E-14,12.2,-1.77635683940025E-14));
#181202=CARTESIAN_POINT('Origin',(-5.66257110645729E-14,15.2,-1.77635683940025E-14));
#181203=CARTESIAN_POINT('Origin',(-5.66257110645729E-14,15.2,-1.77635683940025E-14));
#181204=CARTESIAN_POINT('',(10.736091047551,15.2,-4.12144986808358));
#181205=CARTESIAN_POINT('',(10.8675859439999,15.2,-3.76106045600002));
#181206=CARTESIAN_POINT('Origin',(-5.66257110645729E-14,15.2,-1.77635683940025E-14));
#181207=CARTESIAN_POINT('',(10.8675859439999,12.2,-3.76106045600002));
#181208=CARTESIAN_POINT('',(10.8675859439999,15.2,-3.76106045600002));
#181209=CARTESIAN_POINT('',(10.7360910469999,12.2,-4.12144986800001));
#181210=CARTESIAN_POINT('Origin',(-5.66257110645729E-14,12.2,-1.77635683940025E-14));
#181211=CARTESIAN_POINT('',(10.7360910469999,15.2,-4.12144986800001));
#181212=CARTESIAN_POINT('Ctrl Pts',(9.55499537099995,15.2,-4.04260911600002));
#181213=CARTESIAN_POINT('Ctrl Pts',(9.55499537099995,11.6,-4.04260911600002));
#181214=CARTESIAN_POINT('Ctrl Pts',(9.55516119299994,15.2,-4.04266300400002));
#181215=CARTESIAN_POINT('Ctrl Pts',(9.55516119299994,11.6,-4.04266300400002));
#181216=CARTESIAN_POINT('Ctrl Pts',(9.55549865399995,15.2,-4.04277257900001));
#181217=CARTESIAN_POINT('Ctrl Pts',(9.55549865399995,11.6,-4.04277257900001));
#181218=CARTESIAN_POINT('Ctrl Pts',(9.55601007099995,15.2,-4.04293835900001));
#181219=CARTESIAN_POINT('Ctrl Pts',(9.55601007099995,11.6,-4.04293835900001));
#181220=CARTESIAN_POINT('Ctrl Pts',(9.55669916199994,15.2,-4.04316116600001));
#181221=CARTESIAN_POINT('Ctrl Pts',(9.55669916199994,11.6,-4.04316116600001));
#181222=CARTESIAN_POINT('Ctrl Pts',(9.55757104099994,15.2,-4.04344211400002));
#181223=CARTESIAN_POINT('Ctrl Pts',(9.55757104099994,11.6,-4.04344211400002));
#181224=CARTESIAN_POINT('Ctrl Pts',(9.55845733799995,15.2,-4.04372672600001));
#181225=CARTESIAN_POINT('Ctrl Pts',(9.55845733799995,11.6,-4.04372672600002));
#181226=CARTESIAN_POINT('Ctrl Pts',(9.55935298099994,15.2,-4.04401334800002));
#181227=CARTESIAN_POINT('Ctrl Pts',(9.55935298099994,11.6,-4.04401334800002));
#181228=CARTESIAN_POINT('Ctrl Pts',(9.56025795099994,15.2,-4.04430195600002));
#181229=CARTESIAN_POINT('Ctrl Pts',(9.56025795099994,11.6,-4.04430195600002));
#181230=CARTESIAN_POINT('Ctrl Pts',(9.56117222799995,15.2,-4.04459252400001));
#181231=CARTESIAN_POINT('Ctrl Pts',(9.56117222799995,11.6,-4.04459252400002));
#181232=CARTESIAN_POINT('Ctrl Pts',(9.56209578999994,15.2,-4.04488502600001));
#181233=CARTESIAN_POINT('Ctrl Pts',(9.56209578999994,11.6,-4.04488502600001));
#181234=CARTESIAN_POINT('Ctrl Pts',(9.56302861899994,15.2,-4.04517943800002));
#181235=CARTESIAN_POINT('Ctrl Pts',(9.56302861899994,11.6,-4.04517943800002));
#181236=CARTESIAN_POINT('Ctrl Pts',(9.56397069599995,15.2,-4.04547573400002));
#181237=CARTESIAN_POINT('Ctrl Pts',(9.56397069599995,11.6,-4.04547573400002));
#181238=CARTESIAN_POINT('Ctrl Pts',(9.56492199899994,15.2,-4.04577389000002));
#181239=CARTESIAN_POINT('Ctrl Pts',(9.56492199899994,11.6,-4.04577389000002));
#181240=CARTESIAN_POINT('Ctrl Pts',(9.56588250899994,15.2,-4.04607388100001));
#181241=CARTESIAN_POINT('Ctrl Pts',(9.56588250899994,11.6,-4.04607388100001));
#181242=CARTESIAN_POINT('Ctrl Pts',(9.56685220699995,15.2,-4.04637568200001));
#181243=CARTESIAN_POINT('Ctrl Pts',(9.56685220699995,11.6,-4.04637568200001));
#181244=CARTESIAN_POINT('Ctrl Pts',(9.56783107299995,15.2,-4.04667926900002));
#181245=CARTESIAN_POINT('Ctrl Pts',(9.56783107299995,11.6,-4.04667926900002));
#181246=CARTESIAN_POINT('Ctrl Pts',(9.56881908799994,15.2,-4.04698461800002));
#181247=CARTESIAN_POINT('Ctrl Pts',(9.56881908799994,11.6,-4.04698461800002));
#181248=CARTESIAN_POINT('Ctrl Pts',(9.56981623299994,15.2,-4.04729170300001));
#181249=CARTESIAN_POINT('Ctrl Pts',(9.56981623299994,11.6,-4.04729170300001));
#181250=CARTESIAN_POINT('Ctrl Pts',(9.57082248799994,15.2,-4.04760050200001));
#181251=CARTESIAN_POINT('Ctrl Pts',(9.57082248799994,11.6,-4.04760050200002));
#181252=CARTESIAN_POINT('Ctrl Pts',(9.57183783399995,15.2,-4.04791099000001));
#181253=CARTESIAN_POINT('Ctrl Pts',(9.57183783399995,11.6,-4.04791099000002));
#181254=CARTESIAN_POINT('Ctrl Pts',(9.57286225199995,15.2,-4.04822314300001));
#181255=CARTESIAN_POINT('Ctrl Pts',(9.57286225199995,11.6,-4.04822314300001));
#181256=CARTESIAN_POINT('Ctrl Pts',(9.57389572299994,15.2,-4.04853693900002));
#181257=CARTESIAN_POINT('Ctrl Pts',(9.57389572299994,11.6,-4.04853693900002));
#181258=CARTESIAN_POINT('Ctrl Pts',(9.57493822699995,15.2,-4.04885235200001));
#181259=CARTESIAN_POINT('Ctrl Pts',(9.57493822699995,11.6,-4.04885235200002));
#181260=CARTESIAN_POINT('Ctrl Pts',(9.57598974799994,15.2,-4.04916936000001));
#181261=CARTESIAN_POINT('Ctrl Pts',(9.57598974799994,11.6,-4.04916936000001));
#181262=CARTESIAN_POINT('Ctrl Pts',(9.57705026499994,15.2,-4.04948793900001));
#181263=CARTESIAN_POINT('Ctrl Pts',(9.57705026499994,11.6,-4.04948793900001));
#181264=CARTESIAN_POINT('Ctrl Pts',(9.57811975999994,15.2,-4.04980806600001));
#181265=CARTESIAN_POINT('Ctrl Pts',(9.57811975999994,11.6,-4.04980806600001));
#181266=CARTESIAN_POINT('Ctrl Pts',(9.57919821399994,15.2,-4.05012971800002));
#181267=CARTESIAN_POINT('Ctrl Pts',(9.57919821399994,11.6,-4.05012971800002));
#181268=CARTESIAN_POINT('Ctrl Pts',(9.58028560899994,15.2,-4.05045287300001));
#181269=CARTESIAN_POINT('Ctrl Pts',(9.58028560899994,11.6,-4.05045287300002));
#181270=CARTESIAN_POINT('Ctrl Pts',(9.58138192599994,15.2,-4.05077750600002));
#181271=CARTESIAN_POINT('Ctrl Pts',(9.58138192599994,11.6,-4.05077750600002));
#181272=CARTESIAN_POINT('Ctrl Pts',(9.58248714699995,15.2,-4.05110359500001));
#181273=CARTESIAN_POINT('Ctrl Pts',(9.58248714699995,11.6,-4.05110359500001));
#181274=CARTESIAN_POINT('Ctrl Pts',(9.58360125399994,15.2,-4.05143111800002));
#181275=CARTESIAN_POINT('Ctrl Pts',(9.58360125399994,11.6,-4.05143111800002));
#181276=CARTESIAN_POINT('Ctrl Pts',(9.58472422699994,15.2,-4.05176005200001));
#181277=CARTESIAN_POINT('Ctrl Pts',(9.58472422699994,11.6,-4.05176005200001));
#181278=CARTESIAN_POINT('Ctrl Pts',(9.58585604999995,15.2,-4.05209037400001));
#181279=CARTESIAN_POINT('Ctrl Pts',(9.58585604999995,11.6,-4.05209037400002));
#181280=CARTESIAN_POINT('Ctrl Pts',(9.58699670499995,15.2,-4.05242206400001));
#181281=CARTESIAN_POINT('Ctrl Pts',(9.58699670499995,11.6,-4.05242206400002));
#181282=CARTESIAN_POINT('Ctrl Pts',(9.58814617199995,15.2,-4.05275509600001));
#181283=CARTESIAN_POINT('Ctrl Pts',(9.58814617199995,11.6,-4.05275509600001));
#181284=CARTESIAN_POINT('Ctrl Pts',(9.58930443499994,15.2,-4.05308945100002));
#181285=CARTESIAN_POINT('Ctrl Pts',(9.58930443499994,11.6,-4.05308945100002));
#181286=CARTESIAN_POINT('Ctrl Pts',(9.59047147499994,15.2,-4.05342510600001));
#181287=CARTESIAN_POINT('Ctrl Pts',(9.59047147499994,11.6,-4.05342510600002));
#181288=CARTESIAN_POINT('Ctrl Pts',(9.59164727399994,15.2,-4.05376204000001));
#181289=CARTESIAN_POINT('Ctrl Pts',(9.59164727399994,11.6,-4.05376204000001));
#181290=CARTESIAN_POINT('Ctrl Pts',(9.59283181499995,15.2,-4.05410022900002));
#181291=CARTESIAN_POINT('Ctrl Pts',(9.59283181499995,11.6,-4.05410022900002));
#181292=CARTESIAN_POINT('Ctrl Pts',(9.59402507999994,15.2,-4.05443965300002));
#181293=CARTESIAN_POINT('Ctrl Pts',(9.59402507999994,11.6,-4.05443965300002));
#181294=CARTESIAN_POINT('Ctrl Pts',(9.59522705299995,15.2,-4.05478029000002));
#181295=CARTESIAN_POINT('Ctrl Pts',(9.59522705299995,11.6,-4.05478029000002));
#181296=CARTESIAN_POINT('Ctrl Pts',(9.59643771299995,15.2,-4.05512212000001));
#181297=CARTESIAN_POINT('Ctrl Pts',(9.59643771299995,11.6,-4.05512212000002));
#181298=CARTESIAN_POINT('Ctrl Pts',(9.59765704499994,15.2,-4.05546511900001));
#181299=CARTESIAN_POINT('Ctrl Pts',(9.59765704499994,11.6,-4.05546511900001));
#181300=CARTESIAN_POINT('Ctrl Pts',(9.59888503199995,15.2,-4.05580926800001));
#181301=CARTESIAN_POINT('Ctrl Pts',(9.59888503199995,11.6,-4.05580926800001));
#181302=CARTESIAN_POINT('Ctrl Pts',(9.60012165499995,15.2,-4.05615454300001));
#181303=CARTESIAN_POINT('Ctrl Pts',(9.60012165499995,11.6,-4.05615454300001));
#181304=CARTESIAN_POINT('Ctrl Pts',(9.60136689799995,15.2,-4.05650092700002));
#181305=CARTESIAN_POINT('Ctrl Pts',(9.60136689799995,11.6,-4.05650092700002));
#181306=CARTESIAN_POINT('Ctrl Pts',(9.60262074299994,15.2,-4.05684839600001));
#181307=CARTESIAN_POINT('Ctrl Pts',(9.60262074299994,11.6,-4.05684839600002));
#181308=CARTESIAN_POINT('Ctrl Pts',(9.60388317399994,15.2,-4.05719693100002));
#181309=CARTESIAN_POINT('Ctrl Pts',(9.60388317399994,11.6,-4.05719693100002));
#181310=CARTESIAN_POINT('Ctrl Pts',(9.60515417299994,15.2,-4.05754650900001));
#181311=CARTESIAN_POINT('Ctrl Pts',(9.60515417299994,11.6,-4.05754650900001));
#181312=CARTESIAN_POINT('Ctrl Pts',(9.60643372199995,15.2,-4.05789711200002));
#181313=CARTESIAN_POINT('Ctrl Pts',(9.60643372199995,11.6,-4.05789711200002));
#181314=CARTESIAN_POINT('Ctrl Pts',(9.60772180599994,15.2,-4.05824871800001));
#181315=CARTESIAN_POINT('Ctrl Pts',(9.60772180599994,11.6,-4.05824871800002));
#181316=CARTESIAN_POINT('Ctrl Pts',(9.60901840799995,15.2,-4.05860130500002));
#181317=CARTESIAN_POINT('Ctrl Pts',(9.60901840799995,11.6,-4.05860130500002));
#181318=CARTESIAN_POINT('Ctrl Pts',(9.61032350999995,15.2,-4.05895485600002));
#181319=CARTESIAN_POINT('Ctrl Pts',(9.61032350999995,11.6,-4.05895485600002));
#181320=CARTESIAN_POINT('Ctrl Pts',(9.61163709499995,15.2,-4.05930934900002));
#181321=CARTESIAN_POINT('Ctrl Pts',(9.61163709499995,11.6,-4.05930934900002));
#181322=CARTESIAN_POINT('Ctrl Pts',(9.61295914899994,15.2,-4.05966476400001));
#181323=CARTESIAN_POINT('Ctrl Pts',(9.61295914899994,11.6,-4.05966476400002));
#181324=CARTESIAN_POINT('Ctrl Pts',(9.61428965299995,15.2,-4.06002108000001));
#181325=CARTESIAN_POINT('Ctrl Pts',(9.61428965299995,11.6,-4.06002108000001));
#181326=CARTESIAN_POINT('Ctrl Pts',(9.61562858999994,15.2,-4.06037827900001));
#181327=CARTESIAN_POINT('Ctrl Pts',(9.61562858999994,11.6,-4.06037827900002));
#181328=CARTESIAN_POINT('Ctrl Pts',(9.61697594499995,15.2,-4.06073634000002));
#181329=CARTESIAN_POINT('Ctrl Pts',(9.61697594499995,11.6,-4.06073634000002));
#181330=CARTESIAN_POINT('Ctrl Pts',(9.61833169999995,15.2,-4.06109524300001));
#181331=CARTESIAN_POINT('Ctrl Pts',(9.61833169999995,11.6,-4.06109524300002));
#181332=CARTESIAN_POINT('Ctrl Pts',(9.61969584099995,15.2,-4.06145496800002));
#181333=CARTESIAN_POINT('Ctrl Pts',(9.61969584099995,11.6,-4.06145496800002));
#181334=CARTESIAN_POINT('Ctrl Pts',(9.62106834999994,15.2,-4.06181549700001));
#181335=CARTESIAN_POINT('Ctrl Pts',(9.62106834999994,11.6,-4.06181549700001));
#181336=CARTESIAN_POINT('Ctrl Pts',(9.62244921099994,15.2,-4.06217680900001));
#181337=CARTESIAN_POINT('Ctrl Pts',(9.62244921099994,11.6,-4.06217680900001));
#181338=CARTESIAN_POINT('Ctrl Pts',(9.62383840699994,15.2,-4.06253888400002));
#181339=CARTESIAN_POINT('Ctrl Pts',(9.62383840699994,11.6,-4.06253888400002));
#181340=CARTESIAN_POINT('Ctrl Pts',(9.62523592199994,15.2,-4.06290170600001));
#181341=CARTESIAN_POINT('Ctrl Pts',(9.62523592199994,11.6,-4.06290170600002));
#181342=CARTESIAN_POINT('Ctrl Pts',(9.62664174299995,15.2,-4.06326525100001));
#181343=CARTESIAN_POINT('Ctrl Pts',(9.62664174299995,11.6,-4.06326525100001));
#181344=CARTESIAN_POINT('Ctrl Pts',(9.62805584999994,15.2,-4.06362950400001));
#181345=CARTESIAN_POINT('Ctrl Pts',(9.62805584999994,11.6,-4.06362950400002));
#181346=CARTESIAN_POINT('Ctrl Pts',(9.62947822799994,15.2,-4.06399444400002));
#181347=CARTESIAN_POINT('Ctrl Pts',(9.62947822799994,11.6,-4.06399444400002));
#181348=CARTESIAN_POINT('Ctrl Pts',(9.63090886199995,15.2,-4.06436005200002));
#181349=CARTESIAN_POINT('Ctrl Pts',(9.63090886199995,11.6,-4.06436005200002));
#181350=CARTESIAN_POINT('Ctrl Pts',(9.63234773499994,15.2,-4.06472630900002));
#181351=CARTESIAN_POINT('Ctrl Pts',(9.63234773499994,11.6,-4.06472630900002));
#181352=CARTESIAN_POINT('Ctrl Pts',(9.63379483299994,15.2,-4.06509319800001));
#181353=CARTESIAN_POINT('Ctrl Pts',(9.63379483299994,11.6,-4.06509319800001));
#181354=CARTESIAN_POINT('Ctrl Pts',(9.63525013899994,15.2,-4.06546069700001));
#181355=CARTESIAN_POINT('Ctrl Pts',(9.63525013899994,11.6,-4.06546069700001));
#181356=CARTESIAN_POINT('Ctrl Pts',(9.63671363699994,15.2,-4.06582879000001));
#181357=CARTESIAN_POINT('Ctrl Pts',(9.63671363699994,11.6,-4.06582879000002));
#181358=CARTESIAN_POINT('Ctrl Pts',(9.63818531199994,15.2,-4.06619745800001));
#181359=CARTESIAN_POINT('Ctrl Pts',(9.63818531199994,11.6,-4.06619745800001));
#181360=CARTESIAN_POINT('Ctrl Pts',(9.63966514799995,15.2,-4.06656668200001));
#181361=CARTESIAN_POINT('Ctrl Pts',(9.63966514799995,11.6,-4.06656668200002));
#181362=CARTESIAN_POINT('Ctrl Pts',(9.64115312899994,15.2,-4.06693644400002));
#181363=CARTESIAN_POINT('Ctrl Pts',(9.64115312899994,11.6,-4.06693644400002));
#181364=CARTESIAN_POINT('Ctrl Pts',(9.64264924099995,15.2,-4.06730672400001));
#181365=CARTESIAN_POINT('Ctrl Pts',(9.64264924099995,11.6,-4.06730672400002));
#181366=CARTESIAN_POINT('Ctrl Pts',(9.64415346699995,15.2,-4.06767750600002));
#181367=CARTESIAN_POINT('Ctrl Pts',(9.64415346699995,11.6,-4.06767750600002));
#181368=CARTESIAN_POINT('Ctrl Pts',(9.64566579199994,15.2,-4.06804877300001));
#181369=CARTESIAN_POINT('Ctrl Pts',(9.64566579199994,11.6,-4.06804877300001));
#181370=CARTESIAN_POINT('Ctrl Pts',(9.64718620099994,15.2,-4.06842050300002));
#181371=CARTESIAN_POINT('Ctrl Pts',(9.64718620099994,11.6,-4.06842050300002));
#181372=CARTESIAN_POINT('Ctrl Pts',(9.64871467899994,15.2,-4.06879268000001));
#181373=CARTESIAN_POINT('Ctrl Pts',(9.64871467899994,11.6,-4.06879268000001));
#181374=CARTESIAN_POINT('Ctrl Pts',(9.65025120999995,15.2,-4.06916528800001));
#181375=CARTESIAN_POINT('Ctrl Pts',(9.65025120999995,11.6,-4.06916528800001));
#181376=CARTESIAN_POINT('Ctrl Pts',(9.65179577899995,15.2,-4.06953830600001));
#181377=CARTESIAN_POINT('Ctrl Pts',(9.65179577899995,11.6,-4.06953830600001));
#181378=CARTESIAN_POINT('Ctrl Pts',(9.65334837099994,15.2,-4.06991171800001));
#181379=CARTESIAN_POINT('Ctrl Pts',(9.65334837099994,11.6,-4.06991171800002));
#181380=CARTESIAN_POINT('Ctrl Pts',(9.65490896999994,15.2,-4.07028550500002));
#181381=CARTESIAN_POINT('Ctrl Pts',(9.65490896999994,11.6,-4.07028550500002));
#181382=CARTESIAN_POINT('Ctrl Pts',(9.65647756399994,15.2,-4.07065965100001));
#181383=CARTESIAN_POINT('Ctrl Pts',(9.65647756399994,11.6,-4.07065965100002));
#181384=CARTESIAN_POINT('Ctrl Pts',(9.65805413299995,15.2,-4.07103413800002));
#181385=CARTESIAN_POINT('Ctrl Pts',(9.65805413299995,11.6,-4.07103413800002));
#181386=CARTESIAN_POINT('Ctrl Pts',(9.65963866699994,15.2,-4.07140894900001));
#181387=CARTESIAN_POINT('Ctrl Pts',(9.65963866699994,11.6,-4.07140894900001));
#181388=CARTESIAN_POINT('Ctrl Pts',(9.66123114799995,15.2,-4.07178406500002));
#181389=CARTESIAN_POINT('Ctrl Pts',(9.66123114799995,11.6,-4.07178406500002));
#181390=CARTESIAN_POINT('Ctrl Pts',(9.66283156199994,15.2,-4.07215947000001));
#181391=CARTESIAN_POINT('Ctrl Pts',(9.66283156199994,11.6,-4.07215947000001));
#181392=CARTESIAN_POINT('Ctrl Pts',(9.66443989499994,15.2,-4.07253514700002));
#181393=CARTESIAN_POINT('Ctrl Pts',(9.66443989499994,11.6,-4.07253514700002));
#181394=CARTESIAN_POINT('Ctrl Pts',(9.66605613099994,15.2,-4.07291107800001));
#181395=CARTESIAN_POINT('Ctrl Pts',(9.66605613099994,11.6,-4.07291107800001));
#181396=CARTESIAN_POINT('Ctrl Pts',(9.66768025599994,15.2,-4.07328724600001));
#181397=CARTESIAN_POINT('Ctrl Pts',(9.66768025599994,11.6,-4.07328724600002));
#181398=CARTESIAN_POINT('Ctrl Pts',(9.66931225499994,15.2,-4.07366363600001));
#181399=CARTESIAN_POINT('Ctrl Pts',(9.66931225499994,11.6,-4.07366363600001));
#181400=CARTESIAN_POINT('Ctrl Pts',(9.67095211399995,15.2,-4.07404022700002));
#181401=CARTESIAN_POINT('Ctrl Pts',(9.67095211399995,11.6,-4.07404022700002));
#181402=CARTESIAN_POINT('Ctrl Pts',(9.67259981799995,15.2,-4.07441700600002));
#181403=CARTESIAN_POINT('Ctrl Pts',(9.67259981799995,11.6,-4.07441700600002));
#181404=CARTESIAN_POINT('Ctrl Pts',(9.67425535199995,15.2,-4.07479395500001));
#181405=CARTESIAN_POINT('Ctrl Pts',(9.67425535199995,11.6,-4.07479395500001));
#181406=CARTESIAN_POINT('Ctrl Pts',(9.67591870099995,15.2,-4.07517105700002));
#181407=CARTESIAN_POINT('Ctrl Pts',(9.67591870099995,11.6,-4.07517105700002));
#181408=CARTESIAN_POINT('Ctrl Pts',(9.67758985199995,15.2,-4.07554829600001));
#181409=CARTESIAN_POINT('Ctrl Pts',(9.67758985199995,11.6,-4.07554829600001));
#181410=CARTESIAN_POINT('Ctrl Pts',(9.67926879099995,15.2,-4.07592565400002));
#181411=CARTESIAN_POINT('Ctrl Pts',(9.67926879099995,11.6,-4.07592565400002));
#181412=CARTESIAN_POINT('Ctrl Pts',(9.68095550199994,15.2,-4.07630311500002));
#181413=CARTESIAN_POINT('Ctrl Pts',(9.68095550199994,11.6,-4.07630311500002));
#181414=CARTESIAN_POINT('Ctrl Pts',(9.68264997199995,15.2,-4.07668066400001));
#181415=CARTESIAN_POINT('Ctrl Pts',(9.68264997199995,11.6,-4.07668066400001));
#181416=CARTESIAN_POINT('Ctrl Pts',(9.68435218499994,15.2,-4.07705828300001));
#181417=CARTESIAN_POINT('Ctrl Pts',(9.68435218499994,11.6,-4.07705828300002));
#181418=CARTESIAN_POINT('Ctrl Pts',(9.68606212899994,15.2,-4.07743595700001));
#181419=CARTESIAN_POINT('Ctrl Pts',(9.68606212899994,11.6,-4.07743595700001));
#181420=CARTESIAN_POINT('Ctrl Pts',(9.68777978799995,15.2,-4.07781366900001));
#181421=CARTESIAN_POINT('Ctrl Pts',(9.68777978799995,11.6,-4.07781366900002));
#181422=CARTESIAN_POINT('Ctrl Pts',(9.68950514999994,15.2,-4.07819140300001));
#181423=CARTESIAN_POINT('Ctrl Pts',(9.68950514999994,11.6,-4.07819140300001));
#181424=CARTESIAN_POINT('Ctrl Pts',(9.69123819799995,15.2,-4.07856914300002));
#181425=CARTESIAN_POINT('Ctrl Pts',(9.69123819799995,11.6,-4.07856914300002));
#181426=CARTESIAN_POINT('Ctrl Pts',(9.69297891999994,15.2,-4.07894687300002));
#181427=CARTESIAN_POINT('Ctrl Pts',(9.69297891999994,11.6,-4.07894687300002));
#181428=CARTESIAN_POINT('Ctrl Pts',(9.69472730099995,15.2,-4.07932457800001));
#181429=CARTESIAN_POINT('Ctrl Pts',(9.69472730099995,11.6,-4.07932457800001));
#181430=CARTESIAN_POINT('Ctrl Pts',(9.69648332799995,15.2,-4.07970224000001));
#181431=CARTESIAN_POINT('Ctrl Pts',(9.69648332799995,11.6,-4.07970224000001));
#181432=CARTESIAN_POINT('Ctrl Pts',(9.69824698699994,15.2,-4.08007984400002));
#181433=CARTESIAN_POINT('Ctrl Pts',(9.69824698699994,11.6,-4.08007984400002));
#181434=CARTESIAN_POINT('Ctrl Pts',(9.70001826299994,15.2,-4.08045737500002));
#181435=CARTESIAN_POINT('Ctrl Pts',(9.70001826299994,11.6,-4.08045737500002));
#181436=CARTESIAN_POINT('Ctrl Pts',(9.70179714199995,15.2,-4.08083481700002));
#181437=CARTESIAN_POINT('Ctrl Pts',(9.70179714199995,11.6,-4.08083481700002));
#181438=CARTESIAN_POINT('Ctrl Pts',(9.70358361299994,15.2,-4.08121215500001));
#181439=CARTESIAN_POINT('Ctrl Pts',(9.70358361299994,11.6,-4.08121215500001));
#181440=CARTESIAN_POINT('Ctrl Pts',(9.70537765899994,15.2,-4.08158937200001));
#181441=CARTESIAN_POINT('Ctrl Pts',(9.70537765899994,11.6,-4.08158937200001));
#181442=CARTESIAN_POINT('Ctrl Pts',(9.70717926699994,15.2,-4.08196645300002));
#181443=CARTESIAN_POINT('Ctrl Pts',(9.70717926699994,11.6,-4.08196645300002));
#181444=CARTESIAN_POINT('Ctrl Pts',(9.70898842499994,15.2,-4.08234338300002));
#181445=CARTESIAN_POINT('Ctrl Pts',(9.70898842499994,11.6,-4.08234338300002));
#181446=CARTESIAN_POINT('Ctrl Pts',(9.71080511699994,15.2,-4.08272014700001));
#181447=CARTESIAN_POINT('Ctrl Pts',(9.71080511699994,11.6,-4.08272014700001));
#181448=CARTESIAN_POINT('Ctrl Pts',(9.71262933199995,15.2,-4.08309672800002));
#181449=CARTESIAN_POINT('Ctrl Pts',(9.71262933199995,11.6,-4.08309672800002));
#181450=CARTESIAN_POINT('Ctrl Pts',(9.71446105399994,15.2,-4.08347311300002));
#181451=CARTESIAN_POINT('Ctrl Pts',(9.71446105399994,11.6,-4.08347311300002));
#181452=CARTESIAN_POINT('Ctrl Pts',(9.71630027099994,15.2,-4.08384928600002));
#181453=CARTESIAN_POINT('Ctrl Pts',(9.71630027099994,11.6,-4.08384928600002));
#181454=CARTESIAN_POINT('Ctrl Pts',(9.71814696899994,15.2,-4.08422523100001));
#181455=CARTESIAN_POINT('Ctrl Pts',(9.71814696899994,11.6,-4.08422523100001));
#181456=CARTESIAN_POINT('Ctrl Pts',(9.72000113399995,15.2,-4.08460093400001));
#181457=CARTESIAN_POINT('Ctrl Pts',(9.72000113399995,11.6,-4.08460093400001));
#181458=CARTESIAN_POINT('Ctrl Pts',(9.72186275299994,15.2,-4.08497637900001));
#181459=CARTESIAN_POINT('Ctrl Pts',(9.72186275299994,11.6,-4.08497637900001));
#181460=CARTESIAN_POINT('Ctrl Pts',(9.72373181399995,15.2,-4.08535155200001));
#181461=CARTESIAN_POINT('Ctrl Pts',(9.72373181399995,11.6,-4.08535155200001));
#181462=CARTESIAN_POINT('Ctrl Pts',(9.72560830199994,15.2,-4.08572643800001));
#181463=CARTESIAN_POINT('Ctrl Pts',(9.72560830199994,11.6,-4.08572643800001));
#181464=CARTESIAN_POINT('Ctrl Pts',(9.72749220299994,15.2,-4.08610102200001));
#181465=CARTESIAN_POINT('Ctrl Pts',(9.72749220299994,11.6,-4.08610102200001));
#181466=CARTESIAN_POINT('Ctrl Pts',(9.72938350499994,15.2,-4.08647528800001));
#181467=CARTESIAN_POINT('Ctrl Pts',(9.72938350499994,11.6,-4.08647528800001));
#181468=CARTESIAN_POINT('Ctrl Pts',(9.73128219499995,15.2,-4.08684922400001));
#181469=CARTESIAN_POINT('Ctrl Pts',(9.73128219499995,11.6,-4.08684922400001));
#181470=CARTESIAN_POINT('Ctrl Pts',(9.73318825999995,15.2,-4.08722281400001));
#181471=CARTESIAN_POINT('Ctrl Pts',(9.73318825999995,11.6,-4.08722281400001));
#181472=CARTESIAN_POINT('Ctrl Pts',(9.73510168599995,15.2,-4.08759604300001));
#181473=CARTESIAN_POINT('Ctrl Pts',(9.73510168599995,11.6,-4.08759604300002));
#181474=CARTESIAN_POINT('Ctrl Pts',(9.73702245899995,15.2,-4.08796889700001));
#181475=CARTESIAN_POINT('Ctrl Pts',(9.73702245899995,11.6,-4.08796889700001));
#181476=CARTESIAN_POINT('Ctrl Pts',(9.73895056799994,15.2,-4.08834136100001));
#181477=CARTESIAN_POINT('Ctrl Pts',(9.73895056799994,11.6,-4.08834136100001));
#181478=CARTESIAN_POINT('Ctrl Pts',(9.74088599799994,15.2,-4.08871342100001));
#181479=CARTESIAN_POINT('Ctrl Pts',(9.74088599799994,11.6,-4.08871342100001));
#181480=CARTESIAN_POINT('Ctrl Pts',(9.74282873799994,15.2,-4.08908506300001));
#181481=CARTESIAN_POINT('Ctrl Pts',(9.74282873799994,11.6,-4.08908506300001));
#181482=CARTESIAN_POINT('Ctrl Pts',(9.74477877399995,15.2,-4.08945627200001));
#181483=CARTESIAN_POINT('Ctrl Pts',(9.74477877399995,11.6,-4.08945627200001));
#181484=CARTESIAN_POINT('Ctrl Pts',(9.74673609199994,15.2,-4.08982703400001));
#181485=CARTESIAN_POINT('Ctrl Pts',(9.74673609199994,11.6,-4.08982703400001));
#181486=CARTESIAN_POINT('Ctrl Pts',(9.74870068199994,15.2,-4.09019733600001));
#181487=CARTESIAN_POINT('Ctrl Pts',(9.74870068199994,11.6,-4.09019733600002));
#181488=CARTESIAN_POINT('Ctrl Pts',(9.75067252699995,15.2,-4.09056716100002));
#181489=CARTESIAN_POINT('Ctrl Pts',(9.75067252699995,11.6,-4.09056716100002));
#181490=CARTESIAN_POINT('Ctrl Pts',(9.75265161799994,15.2,-4.09093649800001));
#181491=CARTESIAN_POINT('Ctrl Pts',(9.75265161799994,11.6,-4.09093649800001));
#181492=CARTESIAN_POINT('Ctrl Pts',(9.75463793899995,15.2,-4.09130533200001));
#181493=CARTESIAN_POINT('Ctrl Pts',(9.75463793899995,11.6,-4.09130533200001));
#181494=CARTESIAN_POINT('Ctrl Pts',(9.75663147999994,15.2,-4.09167364900001));
#181495=CARTESIAN_POINT('Ctrl Pts',(9.75663147999994,11.6,-4.09167364900001));
#181496=CARTESIAN_POINT('Ctrl Pts',(9.75863222799994,15.2,-4.09204143300002));
#181497=CARTESIAN_POINT('Ctrl Pts',(9.75863222799994,11.6,-4.09204143300002));
#181498=CARTESIAN_POINT('Ctrl Pts',(9.76064016799995,15.2,-4.09240867300001));
#181499=CARTESIAN_POINT('Ctrl Pts',(9.76064016799995,11.6,-4.09240867300001));
#181500=CARTESIAN_POINT('Ctrl Pts',(9.76265528799994,15.2,-4.09277535500001));
#181501=CARTESIAN_POINT('Ctrl Pts',(9.76265528799994,11.6,-4.09277535500001));
#181502=CARTESIAN_POINT('Ctrl Pts',(9.76467757799995,15.2,-4.09314146400002));
#181503=CARTESIAN_POINT('Ctrl Pts',(9.76467757799995,11.6,-4.09314146400002));
#181504=CARTESIAN_POINT('Ctrl Pts',(9.76670702199995,15.2,-4.09350698700001));
#181505=CARTESIAN_POINT('Ctrl Pts',(9.76670702199995,11.6,-4.09350698700001));
#181506=CARTESIAN_POINT('Ctrl Pts',(9.76874360999994,15.2,-4.09387191000001));
#181507=CARTESIAN_POINT('Ctrl Pts',(9.76874360999994,11.6,-4.09387191000001));
#181508=CARTESIAN_POINT('Ctrl Pts',(9.77078732699994,15.2,-4.09423622000002));
#181509=CARTESIAN_POINT('Ctrl Pts',(9.77078732699994,11.6,-4.09423622000002));
#181510=CARTESIAN_POINT('Ctrl Pts',(9.77283816299994,15.2,-4.09459990300002));
#181511=CARTESIAN_POINT('Ctrl Pts',(9.77283816299994,11.6,-4.09459990300002));
#181512=CARTESIAN_POINT('Ctrl Pts',(9.77489610299994,15.2,-4.09496294400002));
#181513=CARTESIAN_POINT('Ctrl Pts',(9.77489610299994,11.6,-4.09496294400002));
#181514=CARTESIAN_POINT('Ctrl Pts',(9.77696113599994,15.2,-4.09532533300002));
#181515=CARTESIAN_POINT('Ctrl Pts',(9.77696113599994,11.6,-4.09532533300002));
#181516=CARTESIAN_POINT('Ctrl Pts',(9.77903324999994,15.2,-4.09568705400002));
#181517=CARTESIAN_POINT('Ctrl Pts',(9.77903324999994,11.6,-4.09568705400002));
#181518=CARTESIAN_POINT('Ctrl Pts',(9.78111243199994,15.2,-4.09604809500001));
#181519=CARTESIAN_POINT('Ctrl Pts',(9.78111243199994,11.6,-4.09604809500001));
#181520=CARTESIAN_POINT('Ctrl Pts',(9.78319866899995,15.2,-4.09640844200001));
#181521=CARTESIAN_POINT('Ctrl Pts',(9.78319866899995,11.6,-4.09640844200002));
#181522=CARTESIAN_POINT('Ctrl Pts',(9.78529195099994,15.2,-4.09676808200001));
#181523=CARTESIAN_POINT('Ctrl Pts',(9.78529195099994,11.6,-4.09676808200001));
#181524=CARTESIAN_POINT('Ctrl Pts',(9.78739226299994,15.2,-4.09712700200001));
#181525=CARTESIAN_POINT('Ctrl Pts',(9.78739226299994,11.6,-4.09712700200001));
#181526=CARTESIAN_POINT('Ctrl Pts',(9.78949959499994,15.2,-4.09748518800002));
#181527=CARTESIAN_POINT('Ctrl Pts',(9.78949959499994,11.6,-4.09748518800002));
#181528=CARTESIAN_POINT('Ctrl Pts',(9.79161393199995,15.2,-4.09784262900001));
#181529=CARTESIAN_POINT('Ctrl Pts',(9.79161393199995,11.6,-4.09784262900002));
#181530=CARTESIAN_POINT('Ctrl Pts',(9.79373526299995,15.2,-4.09819930900001));
#181531=CARTESIAN_POINT('Ctrl Pts',(9.79373526299995,11.6,-4.09819930900001));
#181532=CARTESIAN_POINT('Ctrl Pts',(9.79586357799995,15.2,-4.09855521700001));
#181533=CARTESIAN_POINT('Ctrl Pts',(9.79586357799995,11.6,-4.09855521700001));
#181534=CARTESIAN_POINT('Ctrl Pts',(9.79799886199994,15.2,-4.09891034100001));
#181535=CARTESIAN_POINT('Ctrl Pts',(9.79799886199994,11.6,-4.09891034100002));
#181536=CARTESIAN_POINT('Ctrl Pts',(9.80014110399994,15.2,-4.09926466500002));
#181537=CARTESIAN_POINT('Ctrl Pts',(9.80014110399994,11.6,-4.09926466500002));
#181538=CARTESIAN_POINT('Ctrl Pts',(9.80229029299995,15.2,-4.09961817900002));
#181539=CARTESIAN_POINT('Ctrl Pts',(9.80229029299995,11.6,-4.09961817900002));
#181540=CARTESIAN_POINT('Ctrl Pts',(9.80444641399994,15.2,-4.09997086900002));
#181541=CARTESIAN_POINT('Ctrl Pts',(9.80444641399994,11.6,-4.09997086900002));
#181542=CARTESIAN_POINT('Ctrl Pts',(9.80660945899994,15.2,-4.10032272200001));
#181543=CARTESIAN_POINT('Ctrl Pts',(9.80660945899994,11.6,-4.10032272200001));
#181544=CARTESIAN_POINT('Ctrl Pts',(9.80877941099994,15.2,-4.10067372700002));
#181545=CARTESIAN_POINT('Ctrl Pts',(9.80877941099994,11.6,-4.10067372700002));
#181546=CARTESIAN_POINT('Ctrl Pts',(9.81095626399994,15.2,-4.10102387000002));
#181547=CARTESIAN_POINT('Ctrl Pts',(9.81095626399994,11.6,-4.10102387000002));
#181548=CARTESIAN_POINT('Ctrl Pts',(9.81313999999994,15.2,-4.10137313700002));
#181549=CARTESIAN_POINT('Ctrl Pts',(9.81313999999994,11.6,-4.10137313700002));
#181550=CARTESIAN_POINT('Ctrl Pts',(9.81533061199995,15.2,-4.10172151900001));
#181551=CARTESIAN_POINT('Ctrl Pts',(9.81533061199995,11.6,-4.10172151900001));
#181552=CARTESIAN_POINT('Ctrl Pts',(9.81752808499994,15.2,-4.10206900100002));
#181553=CARTESIAN_POINT('Ctrl Pts',(9.81752808499994,11.6,-4.10206900100002));
#181554=CARTESIAN_POINT('Ctrl Pts',(9.81973240799995,15.2,-4.10241557000001));
#181555=CARTESIAN_POINT('Ctrl Pts',(9.81973240799995,11.6,-4.10241557000001));
#181556=CARTESIAN_POINT('Ctrl Pts',(9.82194356999995,15.2,-4.10276121500001));
#181557=CARTESIAN_POINT('Ctrl Pts',(9.82194356999995,11.6,-4.10276121500001));
#181558=CARTESIAN_POINT('Ctrl Pts',(9.82416155899994,15.2,-4.10310592400001));
#181559=CARTESIAN_POINT('Ctrl Pts',(9.82416155899994,11.6,-4.10310592400002));
#181560=CARTESIAN_POINT('Ctrl Pts',(9.82638636299994,15.2,-4.10344968500001));
#181561=CARTESIAN_POINT('Ctrl Pts',(9.82638636299994,11.6,-4.10344968500001));
#181562=CARTESIAN_POINT('Ctrl Pts',(9.82861796899994,15.2,-4.10379248300002));
#181563=CARTESIAN_POINT('Ctrl Pts',(9.82861796899994,11.6,-4.10379248300002));
#181564=CARTESIAN_POINT('Ctrl Pts',(9.83085636699995,15.2,-4.10413430800002));
#181565=CARTESIAN_POINT('Ctrl Pts',(9.83085636699995,11.6,-4.10413430800002));
#181566=CARTESIAN_POINT('Ctrl Pts',(9.83310154499994,15.2,-4.10447514700001));
#181567=CARTESIAN_POINT('Ctrl Pts',(9.83310154499994,11.6,-4.10447514700001));
#181568=CARTESIAN_POINT('Ctrl Pts',(9.83535349099995,15.2,-4.10481498900001));
#181569=CARTESIAN_POINT('Ctrl Pts',(9.83535349099995,11.6,-4.10481498900001));
#181570=CARTESIAN_POINT('Ctrl Pts',(9.83761219299994,15.2,-4.10515382000002));
#181571=CARTESIAN_POINT('Ctrl Pts',(9.83761219299994,11.6,-4.10515382000002));
#181572=CARTESIAN_POINT('Ctrl Pts',(9.83987763999994,15.2,-4.10549163000002));
#181573=CARTESIAN_POINT('Ctrl Pts',(9.83987763999994,11.6,-4.10549163000002));
#181574=CARTESIAN_POINT('Ctrl Pts',(9.84214981999994,15.2,-4.10582840600001));
#181575=CARTESIAN_POINT('Ctrl Pts',(9.84214981999994,11.6,-4.10582840600001));
#181576=CARTESIAN_POINT('Ctrl Pts',(9.84442872299994,15.2,-4.10616413700001));
#181577=CARTESIAN_POINT('Ctrl Pts',(9.84442872299994,11.6,-4.10616413700002));
#181578=CARTESIAN_POINT('Ctrl Pts',(9.84671433499994,15.2,-4.10649880800001));
#181579=CARTESIAN_POINT('Ctrl Pts',(9.84671433499994,11.6,-4.10649880800001));
#181580=CARTESIAN_POINT('Ctrl Pts',(9.84900664499994,15.2,-4.10683241100001));
#181581=CARTESIAN_POINT('Ctrl Pts',(9.84900664499994,11.6,-4.10683241100002));
#181582=CARTESIAN_POINT('Ctrl Pts',(9.85130564399994,15.2,-4.10716493200002));
#181583=CARTESIAN_POINT('Ctrl Pts',(9.85130564399994,11.6,-4.10716493200002));
#181584=CARTESIAN_POINT('Ctrl Pts',(9.85361131799995,15.2,-4.10749636000002));
#181585=CARTESIAN_POINT('Ctrl Pts',(9.85361131799995,11.6,-4.10749636000002));
#181586=CARTESIAN_POINT('Ctrl Pts',(9.85592365599994,15.2,-4.10782668300001));
#181587=CARTESIAN_POINT('Ctrl Pts',(9.85592365599994,11.6,-4.10782668300001));
#181588=CARTESIAN_POINT('Ctrl Pts',(9.85824264599995,15.2,-4.10815588900002));
#181589=CARTESIAN_POINT('Ctrl Pts',(9.85824264599995,11.6,-4.10815588900002));
#181590=CARTESIAN_POINT('Ctrl Pts',(9.86056827899995,15.2,-4.10848396600001));
#181591=CARTESIAN_POINT('Ctrl Pts',(9.86056827899995,11.6,-4.10848396600001));
#181592=CARTESIAN_POINT('Ctrl Pts',(9.86290054199995,15.2,-4.10881090400002));
#181593=CARTESIAN_POINT('Ctrl Pts',(9.86290054199995,11.6,-4.10881090400002));
#181594=CARTESIAN_POINT('Ctrl Pts',(9.86523942299995,15.2,-4.10913669000001));
#181595=CARTESIAN_POINT('Ctrl Pts',(9.86523942299995,11.6,-4.10913669000002));
#181596=CARTESIAN_POINT('Ctrl Pts',(9.86758491299994,15.2,-4.10946131300001));
#181597=CARTESIAN_POINT('Ctrl Pts',(9.86758491299994,11.6,-4.10946131300001));
#181598=CARTESIAN_POINT('Ctrl Pts',(9.86993699799994,15.2,-4.10978476100002));
#181599=CARTESIAN_POINT('Ctrl Pts',(9.86993699799994,11.6,-4.10978476100002));
#181600=CARTESIAN_POINT('Ctrl Pts',(9.87229566899994,15.2,-4.11010702400001));
#181601=CARTESIAN_POINT('Ctrl Pts',(9.87229566899994,11.6,-4.11010702400001));
#181602=CARTESIAN_POINT('Ctrl Pts',(9.87466091299994,15.2,-4.11042808800001));
#181603=CARTESIAN_POINT('Ctrl Pts',(9.87466091299994,11.6,-4.11042808800001));
#181604=CARTESIAN_POINT('Ctrl Pts',(9.87703271999995,15.2,-4.11074794500002));
#181605=CARTESIAN_POINT('Ctrl Pts',(9.87703271999995,11.6,-4.11074794500002));
#181606=CARTESIAN_POINT('Ctrl Pts',(9.87941107799994,15.2,-4.11106658100001));
#181607=CARTESIAN_POINT('Ctrl Pts',(9.87941107799994,11.6,-4.11106658100001));
#181608=CARTESIAN_POINT('Ctrl Pts',(9.88179597699995,15.2,-4.11138398500002));
#181609=CARTESIAN_POINT('Ctrl Pts',(9.88179597699995,11.6,-4.11138398500002));
#181610=CARTESIAN_POINT('Ctrl Pts',(9.88418740499995,15.2,-4.11170014600001));
#181611=CARTESIAN_POINT('Ctrl Pts',(9.88418740499995,11.6,-4.11170014600002));
#181612=CARTESIAN_POINT('Ctrl Pts',(9.88658535099994,15.2,-4.11201505500001));
#181613=CARTESIAN_POINT('Ctrl Pts',(9.88658535099994,11.6,-4.11201505500001));
#181614=CARTESIAN_POINT('Ctrl Pts',(9.88898980499994,15.2,-4.11232869700001));
#181615=CARTESIAN_POINT('Ctrl Pts',(9.88898980499994,11.6,-4.11232869700001));
#181616=CARTESIAN_POINT('Ctrl Pts',(9.89140075299994,15.2,-4.11264106400001));
#181617=CARTESIAN_POINT('Ctrl Pts',(9.89140075299994,11.6,-4.11264106400001));
#181618=CARTESIAN_POINT('Ctrl Pts',(9.89381818699995,15.2,-4.11295214400001));
#181619=CARTESIAN_POINT('Ctrl Pts',(9.89381818699995,11.6,-4.11295214400001));
#181620=CARTESIAN_POINT('Ctrl Pts',(9.89624209499994,15.2,-4.11326192500002));
#181621=CARTESIAN_POINT('Ctrl Pts',(9.89624209499994,11.6,-4.11326192500002));
#181622=CARTESIAN_POINT('Ctrl Pts',(9.89867246499994,15.2,-4.11357039600002));
#181623=CARTESIAN_POINT('Ctrl Pts',(9.89867246499994,11.6,-4.11357039600002));
#181624=CARTESIAN_POINT('Ctrl Pts',(9.90110928899995,15.2,-4.11387754800002));
#181625=CARTESIAN_POINT('Ctrl Pts',(9.90110928899995,11.6,-4.11387754800002));
#181626=CARTESIAN_POINT('Ctrl Pts',(9.90355255199994,15.2,-4.11418336800002));
#181627=CARTESIAN_POINT('Ctrl Pts',(9.90355255199994,11.6,-4.11418336800002));
#181628=CARTESIAN_POINT('Ctrl Pts',(9.90600224599994,15.2,-4.11448784500001));
#181629=CARTESIAN_POINT('Ctrl Pts',(9.90600224599994,11.6,-4.11448784500002));
#181630=CARTESIAN_POINT('Ctrl Pts',(9.90845835999994,15.2,-4.11479097000001));
#181631=CARTESIAN_POINT('Ctrl Pts',(9.90845835999994,11.6,-4.11479097000001));
#181632=CARTESIAN_POINT('Ctrl Pts',(9.91092088199995,15.2,-4.11509273100001));
#181633=CARTESIAN_POINT('Ctrl Pts',(9.91092088199995,11.6,-4.11509273100001));
#181634=CARTESIAN_POINT('Ctrl Pts',(9.91338980099994,15.2,-4.11539311700002));
#181635=CARTESIAN_POINT('Ctrl Pts',(9.91338980099994,11.6,-4.11539311700002));
#181636=CARTESIAN_POINT('Ctrl Pts',(9.91586510599994,15.2,-4.11569211800002));
#181637=CARTESIAN_POINT('Ctrl Pts',(9.91586510599994,11.6,-4.11569211800002));
#181638=CARTESIAN_POINT('Ctrl Pts',(9.91834678799994,15.2,-4.11598972400002));
#181639=CARTESIAN_POINT('Ctrl Pts',(9.91834678799994,11.6,-4.11598972400002));
#181640=CARTESIAN_POINT('Ctrl Pts',(9.92083483399995,15.2,-4.11628592200001));
#181641=CARTESIAN_POINT('Ctrl Pts',(9.92083483399995,11.6,-4.11628592200001));
#181642=CARTESIAN_POINT('Ctrl Pts',(9.92332923599994,15.2,-4.11658070200001));
#181643=CARTESIAN_POINT('Ctrl Pts',(9.92332923599994,11.6,-4.11658070200002));
#181644=CARTESIAN_POINT('Ctrl Pts',(9.92582998099994,15.2,-4.11687405500002));
#181645=CARTESIAN_POINT('Ctrl Pts',(9.92582998099994,11.6,-4.11687405500002));
#181646=CARTESIAN_POINT('Ctrl Pts',(9.92833705899995,15.2,-4.11716596900002));
#181647=CARTESIAN_POINT('Ctrl Pts',(9.92833705899995,11.6,-4.11716596900002));
#181648=CARTESIAN_POINT('Ctrl Pts',(9.93085045799995,15.2,-4.11745643400002));
#181649=CARTESIAN_POINT('Ctrl Pts',(9.93085045799995,11.6,-4.11745643400002));
#181650=CARTESIAN_POINT('Ctrl Pts',(9.93337016999994,15.2,-4.11774544000002));
#181651=CARTESIAN_POINT('Ctrl Pts',(9.93337016999994,11.6,-4.11774544000002));
#181652=CARTESIAN_POINT('Ctrl Pts',(9.93589618199995,15.2,-4.11803297500001));
#181653=CARTESIAN_POINT('Ctrl Pts',(9.93589618199995,11.6,-4.11803297500002));
#181654=CARTESIAN_POINT('Ctrl Pts',(9.93842848399994,15.2,-4.11831903000001));
#181655=CARTESIAN_POINT('Ctrl Pts',(9.93842848399994,11.6,-4.11831903000001));
#181656=CARTESIAN_POINT('Ctrl Pts',(9.94096706699995,15.2,-4.11860359400002));
#181657=CARTESIAN_POINT('Ctrl Pts',(9.94096706699995,11.6,-4.11860359400002));
#181658=CARTESIAN_POINT('Ctrl Pts',(9.94351191899994,15.2,-4.11888665700001));
#181659=CARTESIAN_POINT('Ctrl Pts',(9.94351191899994,11.6,-4.11888665700001));
#181660=CARTESIAN_POINT('Ctrl Pts',(9.94606302899994,15.2,-4.11916820900001));
#181661=CARTESIAN_POINT('Ctrl Pts',(9.94606302899994,11.6,-4.11916820900002));
#181662=CARTESIAN_POINT('Ctrl Pts',(9.94862038599994,15.2,-4.11944823900001));
#181663=CARTESIAN_POINT('Ctrl Pts',(9.94862038599994,11.6,-4.11944823900001));
#181664=CARTESIAN_POINT('Ctrl Pts',(9.95118398199994,15.2,-4.11972673700001));
#181665=CARTESIAN_POINT('Ctrl Pts',(9.95118398199994,11.6,-4.11972673700001));
#181666=CARTESIAN_POINT('Ctrl Pts',(9.95375380499994,15.2,-4.12000369300001));
#181667=CARTESIAN_POINT('Ctrl Pts',(9.95375380499994,11.6,-4.12000369300001));
#181668=CARTESIAN_POINT('Ctrl Pts',(9.95632984299995,15.2,-4.12027909500001));
#181669=CARTESIAN_POINT('Ctrl Pts',(9.95632984299995,11.6,-4.12027909500001));
#181670=CARTESIAN_POINT('Ctrl Pts',(9.95891208799994,15.2,-4.12055293600002));
#181671=CARTESIAN_POINT('Ctrl Pts',(9.95891208799994,11.6,-4.12055293600002));
#181672=CARTESIAN_POINT('Ctrl Pts',(9.96150052899995,15.2,-4.12082520400002));
#181673=CARTESIAN_POINT('Ctrl Pts',(9.96150052899995,11.6,-4.12082520400002));
#181674=CARTESIAN_POINT('Ctrl Pts',(9.96409515399994,15.2,-4.12109589000002));
#181675=CARTESIAN_POINT('Ctrl Pts',(9.96409515399994,11.6,-4.12109589000002));
#181676=CARTESIAN_POINT('Ctrl Pts',(9.96669595399995,15.2,-4.12136498300002));
#181677=CARTESIAN_POINT('Ctrl Pts',(9.96669595399995,11.6,-4.12136498300002));
#181678=CARTESIAN_POINT('Ctrl Pts',(9.96930291999995,15.2,-4.12163247300001));
#181679=CARTESIAN_POINT('Ctrl Pts',(9.96930291999995,11.6,-4.12163247300002));
#181680=CARTESIAN_POINT('Ctrl Pts',(9.97191603899994,15.2,-4.12189835100001));
#181681=CARTESIAN_POINT('Ctrl Pts',(9.97191603899994,11.6,-4.12189835100001));
#181682=CARTESIAN_POINT('Ctrl Pts',(9.97453530099994,15.2,-4.12216260600001));
#181683=CARTESIAN_POINT('Ctrl Pts',(9.97453530099994,11.6,-4.12216260600002));
#181684=CARTESIAN_POINT('Ctrl Pts',(9.97716069799995,15.2,-4.12242522700002));
#181685=CARTESIAN_POINT('Ctrl Pts',(9.97716069799995,11.6,-4.12242522700002));
#181686=CARTESIAN_POINT('Ctrl Pts',(9.97979221599994,15.2,-4.12268620700001));
#181687=CARTESIAN_POINT('Ctrl Pts',(9.97979221599994,11.6,-4.12268620700001));
#181688=CARTESIAN_POINT('Ctrl Pts',(9.98242984799995,15.2,-4.12294553500002));
#181689=CARTESIAN_POINT('Ctrl Pts',(9.98242984799995,11.6,-4.12294553500002));
#181690=CARTESIAN_POINT('Ctrl Pts',(9.98507358299995,15.2,-4.12320320100001));
#181691=CARTESIAN_POINT('Ctrl Pts',(9.98507358299995,11.6,-4.12320320100002));
#181692=CARTESIAN_POINT('Ctrl Pts',(9.98772340999994,15.2,-4.12345919500002));
#181693=CARTESIAN_POINT('Ctrl Pts',(9.98772340999994,11.6,-4.12345919500002));
#181694=CARTESIAN_POINT('Ctrl Pts',(9.99037931799995,15.2,-4.12371350600001));
#181695=CARTESIAN_POINT('Ctrl Pts',(9.99037931799995,11.6,-4.12371350600001));
#181696=CARTESIAN_POINT('Ctrl Pts',(9.99304129899994,15.2,-4.12396612800002));
#181697=CARTESIAN_POINT('Ctrl Pts',(9.99304129899994,11.6,-4.12396612800002));
#181698=CARTESIAN_POINT('Ctrl Pts',(9.99570934199994,15.2,-4.12421704800002));
#181699=CARTESIAN_POINT('Ctrl Pts',(9.99570934199994,11.6,-4.12421704800002));
#181700=CARTESIAN_POINT('Ctrl Pts',(9.99838343599994,15.2,-4.12446625800001));
#181701=CARTESIAN_POINT('Ctrl Pts',(9.99838343599994,11.6,-4.12446625800001));
#181702=CARTESIAN_POINT('Ctrl Pts',(10.0010635709999,15.2,-4.12471374800001));
#181703=CARTESIAN_POINT('Ctrl Pts',(10.0010635709999,11.6,-4.12471374800001));
#181704=CARTESIAN_POINT('Ctrl Pts',(10.0037497379999,15.2,-4.12495950800002));
#181705=CARTESIAN_POINT('Ctrl Pts',(10.0037497379999,11.6,-4.12495950800002));
#181706=CARTESIAN_POINT('Ctrl Pts',(10.0064419259999,15.2,-4.12520352800001));
#181707=CARTESIAN_POINT('Ctrl Pts',(10.0064419259999,11.6,-4.12520352800002));
#181708=CARTESIAN_POINT('Ctrl Pts',(10.0091401249999,15.2,-4.12544580100001));
#181709=CARTESIAN_POINT('Ctrl Pts',(10.0091401249999,11.6,-4.12544580100001));
#181710=CARTESIAN_POINT('Ctrl Pts',(10.0118443249999,15.2,-4.12568631400001));
#181711=CARTESIAN_POINT('Ctrl Pts',(10.0118443249999,11.6,-4.12568631400002));
#181712=CARTESIAN_POINT('Ctrl Pts',(10.0145545159999,15.2,-4.12592506000002));
#181713=CARTESIAN_POINT('Ctrl Pts',(10.0145545159999,11.6,-4.12592506000002));
#181714=CARTESIAN_POINT('Ctrl Pts',(10.0172706879999,15.2,-4.12616202900002));
#181715=CARTESIAN_POINT('Ctrl Pts',(10.0172706879999,11.6,-4.12616202900002));
#181716=CARTESIAN_POINT('Ctrl Pts',(10.0199928309999,15.2,-4.12639721200001));
#181717=CARTESIAN_POINT('Ctrl Pts',(10.0199928309999,11.6,-4.12639721200002));
#181718=CARTESIAN_POINT('Ctrl Pts',(10.0227209349999,15.2,-4.12663059800002));
#181719=CARTESIAN_POINT('Ctrl Pts',(10.0227209349999,11.6,-4.12663059800002));
#181720=CARTESIAN_POINT('Ctrl Pts',(10.0254549889999,15.2,-4.12686218000001));
#181721=CARTESIAN_POINT('Ctrl Pts',(10.0254549889999,11.6,-4.12686218000002));
#181722=CARTESIAN_POINT('Ctrl Pts',(10.0281949849999,15.2,-4.12709194800001));
#181723=CARTESIAN_POINT('Ctrl Pts',(10.0281949849999,11.6,-4.12709194800002));
#181724=CARTESIAN_POINT('Ctrl Pts',(10.0309409119999,15.2,-4.12731989100001));
#181725=CARTESIAN_POINT('Ctrl Pts',(10.0309409119999,11.6,-4.12731989100002));
#181726=CARTESIAN_POINT('Ctrl Pts',(10.0336927599999,15.2,-4.12754600100001));
#181727=CARTESIAN_POINT('Ctrl Pts',(10.0336927599999,11.6,-4.12754600100001));
#181728=CARTESIAN_POINT('Ctrl Pts',(10.0364505199999,15.2,-4.12777026900002));
#181729=CARTESIAN_POINT('Ctrl Pts',(10.0364505199999,11.6,-4.12777026900002));
#181730=CARTESIAN_POINT('Ctrl Pts',(10.0392141799999,15.2,-4.12799268600001));
#181731=CARTESIAN_POINT('Ctrl Pts',(10.0392141799999,11.6,-4.12799268600002));
#181732=CARTESIAN_POINT('Ctrl Pts',(10.0419837319999,15.2,-4.12821324300001));
#181733=CARTESIAN_POINT('Ctrl Pts',(10.0419837319999,11.6,-4.12821324300001));
#181734=CARTESIAN_POINT('Ctrl Pts',(10.0447591649999,15.2,-4.12843193000001));
#181735=CARTESIAN_POINT('Ctrl Pts',(10.0447591649999,11.6,-4.12843193000001));
#181736=CARTESIAN_POINT('Ctrl Pts',(10.0475404719999,15.2,-4.12864873800002));
#181737=CARTESIAN_POINT('Ctrl Pts',(10.0475404719999,11.6,-4.12864873800002));
#181738=CARTESIAN_POINT('Ctrl Pts',(10.0503276389999,15.2,-4.12886366000001));
#181739=CARTESIAN_POINT('Ctrl Pts',(10.0503276389999,11.6,-4.12886366000001));
#181740=CARTESIAN_POINT('Ctrl Pts',(10.0531206589999,15.2,-4.12907668300001));
#181741=CARTESIAN_POINT('Ctrl Pts',(10.0531206589999,11.6,-4.12907668300001));
#181742=CARTESIAN_POINT('Ctrl Pts',(10.0559195209999,15.2,-4.12928780200001));
#181743=CARTESIAN_POINT('Ctrl Pts',(10.0559195209999,11.6,-4.12928780200002));
#181744=CARTESIAN_POINT('Ctrl Pts',(10.0587242159999,15.2,-4.12949700500001));
#181745=CARTESIAN_POINT('Ctrl Pts',(10.0587242159999,11.6,-4.12949700500001));
#181746=CARTESIAN_POINT('Ctrl Pts',(10.0615347329999,15.2,-4.12970428500001));
#181747=CARTESIAN_POINT('Ctrl Pts',(10.0615347329999,11.6,-4.12970428500001));
#181748=CARTESIAN_POINT('Ctrl Pts',(10.0643510649999,15.2,-4.12990963300001));
#181749=CARTESIAN_POINT('Ctrl Pts',(10.0643510649999,11.6,-4.12990963300001));
#181750=CARTESIAN_POINT('Ctrl Pts',(10.0671731989999,15.2,-4.13011303900001));
#181751=CARTESIAN_POINT('Ctrl Pts',(10.0671731989999,11.6,-4.13011303900001));
#181752=CARTESIAN_POINT('Ctrl Pts',(10.0700011269999,15.2,-4.13031449500001));
#181753=CARTESIAN_POINT('Ctrl Pts',(10.0700011269999,11.6,-4.13031449500001));
#181754=CARTESIAN_POINT('Ctrl Pts',(10.0728348389999,15.2,-4.13051399200001));
#181755=CARTESIAN_POINT('Ctrl Pts',(10.0728348389999,11.6,-4.13051399200001));
#181756=CARTESIAN_POINT('Ctrl Pts',(10.0756743259999,15.2,-4.13071152200001));
#181757=CARTESIAN_POINT('Ctrl Pts',(10.0756743259999,11.6,-4.13071152200002));
#181758=CARTESIAN_POINT('Ctrl Pts',(10.0785195769999,15.2,-4.13090707400002));
#181759=CARTESIAN_POINT('Ctrl Pts',(10.0785195769999,11.6,-4.13090707400002));
#181760=CARTESIAN_POINT('Ctrl Pts',(10.0813705839999,15.2,-4.13110064100001));
#181761=CARTESIAN_POINT('Ctrl Pts',(10.0813705839999,11.6,-4.13110064100001));
#181762=CARTESIAN_POINT('Ctrl Pts',(10.0842273359999,15.2,-4.13129221400002));
#181763=CARTESIAN_POINT('Ctrl Pts',(10.0842273359999,11.6,-4.13129221400002));
#181764=CARTESIAN_POINT('Ctrl Pts',(10.0870898239999,15.2,-4.13148178500002));
#181765=CARTESIAN_POINT('Ctrl Pts',(10.0870898239999,11.6,-4.13148178500002));
#181766=CARTESIAN_POINT('Ctrl Pts',(10.0899580389999,15.2,-4.13166934400001));
#181767=CARTESIAN_POINT('Ctrl Pts',(10.0899580389999,11.6,-4.13166934400001));
#181768=CARTESIAN_POINT('Ctrl Pts',(10.0928319699999,15.2,-4.13185488300002));
#181769=CARTESIAN_POINT('Ctrl Pts',(10.0928319699999,11.6,-4.13185488300002));
#181770=CARTESIAN_POINT('Ctrl Pts',(10.0957116079999,15.2,-4.13203839300001));
#181771=CARTESIAN_POINT('Ctrl Pts',(10.0957116079999,11.6,-4.13203839300001));
#181772=CARTESIAN_POINT('Ctrl Pts',(10.0985969439999,15.2,-4.13221986700002));
#181773=CARTESIAN_POINT('Ctrl Pts',(10.0985969439999,11.6,-4.13221986700002));
#181774=CARTESIAN_POINT('Ctrl Pts',(10.1014879679999,15.2,-4.13239929400001));
#181775=CARTESIAN_POINT('Ctrl Pts',(10.1014879679999,11.6,-4.13239929400001));
#181776=CARTESIAN_POINT('Ctrl Pts',(10.1043846719999,15.2,-4.13257666700002));
#181777=CARTESIAN_POINT('Ctrl Pts',(10.1043846719999,11.6,-4.13257666700002));
#181778=CARTESIAN_POINT('Ctrl Pts',(10.1072870439999,15.2,-4.13275197800001));
#181779=CARTESIAN_POINT('Ctrl Pts',(10.1072870439999,11.6,-4.13275197800001));
#181780=CARTESIAN_POINT('Ctrl Pts',(10.1101950759999,15.2,-4.13292521800001));
#181781=CARTESIAN_POINT('Ctrl Pts',(10.1101950759999,11.6,-4.13292521800001));
#181782=CARTESIAN_POINT('Ctrl Pts',(10.1131087579999,15.2,-4.13309637800001));
#181783=CARTESIAN_POINT('Ctrl Pts',(10.1131087579999,11.6,-4.13309637800001));
#181784=CARTESIAN_POINT('Ctrl Pts',(10.1160280819999,15.2,-4.13326545000002));
#181785=CARTESIAN_POINT('Ctrl Pts',(10.1160280819999,11.6,-4.13326545000002));
#181786=CARTESIAN_POINT('Ctrl Pts',(10.1189530369999,15.2,-4.13343242500002));
#181787=CARTESIAN_POINT('Ctrl Pts',(10.1189530369999,11.6,-4.13343242500002));
#181788=CARTESIAN_POINT('Ctrl Pts',(10.1218836129999,15.2,-4.13359729600002));
#181789=CARTESIAN_POINT('Ctrl Pts',(10.1218836129999,11.6,-4.13359729600002));
#181790=CARTESIAN_POINT('Ctrl Pts',(10.1248198019999,15.2,-4.13376005400002));
#181791=CARTESIAN_POINT('Ctrl Pts',(10.1248198019999,11.6,-4.13376005400002));
#181792=CARTESIAN_POINT('Ctrl Pts',(10.1277615949999,15.2,-4.13392069100002));
#181793=CARTESIAN_POINT('Ctrl Pts',(10.1277615949999,11.6,-4.13392069100002));
#181794=CARTESIAN_POINT('Ctrl Pts',(10.1307089819999,15.2,-4.13407919700001));
#181795=CARTESIAN_POINT('Ctrl Pts',(10.1307089819999,11.6,-4.13407919700001));
#181796=CARTESIAN_POINT('Ctrl Pts',(10.1336619529999,15.2,-4.13423556700002));
#181797=CARTESIAN_POINT('Ctrl Pts',(10.1336619529999,11.6,-4.13423556700002));
#181798=CARTESIAN_POINT('Ctrl Pts',(10.1366204989999,15.2,-4.13438979000002));
#181799=CARTESIAN_POINT('Ctrl Pts',(10.1366204989999,11.6,-4.13438979000002));
#181800=CARTESIAN_POINT('Ctrl Pts',(10.1395846109999,15.2,-4.13454185800001));
#181801=CARTESIAN_POINT('Ctrl Pts',(10.1395846109999,11.6,-4.13454185800001));
#181802=CARTESIAN_POINT('Ctrl Pts',(10.1425542799999,15.2,-4.13469176500001));
#181803=CARTESIAN_POINT('Ctrl Pts',(10.1425542799999,11.6,-4.13469176500001));
#181804=CARTESIAN_POINT('Ctrl Pts',(10.1455294969999,15.2,-4.13483950100002));
#181805=CARTESIAN_POINT('Ctrl Pts',(10.1455294969999,11.6,-4.13483950100002));
#181806=CARTESIAN_POINT('Ctrl Pts',(10.1485102509999,15.2,-4.13498505800002));
#181807=CARTESIAN_POINT('Ctrl Pts',(10.1485102509999,11.6,-4.13498505800002));
#181808=CARTESIAN_POINT('Ctrl Pts',(10.1514965349999,15.2,-4.13512842800001));
#181809=CARTESIAN_POINT('Ctrl Pts',(10.1514965349999,11.6,-4.13512842800001));
#181810=CARTESIAN_POINT('Ctrl Pts',(10.1544883369999,15.2,-4.13526960300001));
#181811=CARTESIAN_POINT('Ctrl Pts',(10.1544883369999,11.6,-4.13526960300001));
#181812=CARTESIAN_POINT('Ctrl Pts',(10.1574856509999,15.2,-4.13540857600001));
#181813=CARTESIAN_POINT('Ctrl Pts',(10.1574856509999,11.6,-4.13540857600002));
#181814=CARTESIAN_POINT('Ctrl Pts',(10.1604884649999,15.2,-4.13554533700002));
#181815=CARTESIAN_POINT('Ctrl Pts',(10.1604884649999,11.6,-4.13554533700002));
#181816=CARTESIAN_POINT('Ctrl Pts',(10.1634967709999,15.2,-4.13567988000001));
#181817=CARTESIAN_POINT('Ctrl Pts',(10.1634967709999,11.6,-4.13567988000001));
#181818=CARTESIAN_POINT('Ctrl Pts',(10.1665105609999,15.2,-4.13581219600001));
#181819=CARTESIAN_POINT('Ctrl Pts',(10.1665105609999,11.6,-4.13581219600002));
#181820=CARTESIAN_POINT('Ctrl Pts',(10.1695298229999,15.2,-4.13594227700001));
#181821=CARTESIAN_POINT('Ctrl Pts',(10.1695298229999,11.6,-4.13594227700001));
#181822=CARTESIAN_POINT('Ctrl Pts',(10.1725545499999,15.2,-4.13607011500002));
#181823=CARTESIAN_POINT('Ctrl Pts',(10.1725545499999,11.6,-4.13607011500002));
#181824=CARTESIAN_POINT('Ctrl Pts',(10.1755847329999,15.2,-4.13619570200002));
#181825=CARTESIAN_POINT('Ctrl Pts',(10.1755847329999,11.6,-4.13619570200002));
#181826=CARTESIAN_POINT('Ctrl Pts',(10.1786203619999,15.2,-4.13631903200002));
#181827=CARTESIAN_POINT('Ctrl Pts',(10.1786203619999,11.6,-4.13631903200002));
#181828=CARTESIAN_POINT('Ctrl Pts',(10.1816614279999,15.2,-4.13644009500001));
#181829=CARTESIAN_POINT('Ctrl Pts',(10.1816614279999,11.6,-4.13644009500001));
#181830=CARTESIAN_POINT('Ctrl Pts',(10.1847079219999,15.2,-4.13655888400001));
#181831=CARTESIAN_POINT('Ctrl Pts',(10.1847079219999,11.6,-4.13655888400002));
#181832=CARTESIAN_POINT('Ctrl Pts',(10.1877598339999,15.2,-4.13667539000001));
#181833=CARTESIAN_POINT('Ctrl Pts',(10.1877598339999,11.6,-4.13667539000001));
#181834=CARTESIAN_POINT('Ctrl Pts',(10.1908171569999,15.2,-4.13678960700001));
#181835=CARTESIAN_POINT('Ctrl Pts',(10.1908171569999,11.6,-4.13678960700001));
#181836=CARTESIAN_POINT('Ctrl Pts',(10.1938798809999,15.2,-4.13690152700001));
#181837=CARTESIAN_POINT('Ctrl Pts',(10.1938798809999,11.6,-4.13690152700002));
#181838=CARTESIAN_POINT('Ctrl Pts',(10.1969479959999,15.2,-4.13701114100002));
#181839=CARTESIAN_POINT('Ctrl Pts',(10.1969479959999,11.6,-4.13701114100002));
#181840=CARTESIAN_POINT('Ctrl Pts',(10.2000214939999,15.2,-4.13711844300002));
#181841=CARTESIAN_POINT('Ctrl Pts',(10.2000214939999,11.6,-4.13711844300002));
#181842=CARTESIAN_POINT('Ctrl Pts',(10.2031003659999,15.2,-4.13722342400002));
#181843=CARTESIAN_POINT('Ctrl Pts',(10.2031003659999,11.6,-4.13722342400002));
#181844=CARTESIAN_POINT('Ctrl Pts',(10.2061846029999,15.2,-4.13732607700001));
#181845=CARTESIAN_POINT('Ctrl Pts',(10.2061846029999,11.6,-4.13732607700002));
#181846=CARTESIAN_POINT('Ctrl Pts',(10.2092741959999,15.2,-4.13742639400001));
#181847=CARTESIAN_POINT('Ctrl Pts',(10.2092741959999,11.6,-4.13742639400002));
#181848=CARTESIAN_POINT('Ctrl Pts',(10.2123691339999,15.2,-4.13752436800001));
#181849=CARTESIAN_POINT('Ctrl Pts',(10.2123691339999,11.6,-4.13752436800001));
#181850=CARTESIAN_POINT('Ctrl Pts',(10.2154694119999,15.2,-4.13761999000001));
#181851=CARTESIAN_POINT('Ctrl Pts',(10.2154694119999,11.6,-4.13761999000002));
#181852=CARTESIAN_POINT('Ctrl Pts',(10.2185750179999,15.2,-4.13771325500001));
#181853=CARTESIAN_POINT('Ctrl Pts',(10.2185750179999,11.6,-4.13771325500001));
#181854=CARTESIAN_POINT('Ctrl Pts',(10.2216859439999,15.2,-4.13780415200002));
#181855=CARTESIAN_POINT('Ctrl Pts',(10.2216859439999,11.6,-4.13780415200002));
#181856=CARTESIAN_POINT('Ctrl Pts',(10.2248021809999,15.2,-4.13789267700002));
#181857=CARTESIAN_POINT('Ctrl Pts',(10.2248021809999,11.6,-4.13789267700002));
#181858=CARTESIAN_POINT('Ctrl Pts',(10.2279237199999,15.2,-4.13797882100001));
#181859=CARTESIAN_POINT('Ctrl Pts',(10.2279237199999,11.6,-4.13797882100001));
#181860=CARTESIAN_POINT('Ctrl Pts',(10.2310505519999,15.2,-4.13806257500001));
#181861=CARTESIAN_POINT('Ctrl Pts',(10.2310505519999,11.6,-4.13806257500002));
#181862=CARTESIAN_POINT('Ctrl Pts',(10.2341826699999,15.2,-4.13814393500001));
#181863=CARTESIAN_POINT('Ctrl Pts',(10.2341826699999,11.6,-4.13814393500001));
#181864=CARTESIAN_POINT('Ctrl Pts',(10.2373200619999,15.2,-4.13822289000001));
#181865=CARTESIAN_POINT('Ctrl Pts',(10.2373200619999,11.6,-4.13822289000001));
#181866=CARTESIAN_POINT('Ctrl Pts',(10.2404627209999,15.2,-4.13829943400001));
#181867=CARTESIAN_POINT('Ctrl Pts',(10.2404627209999,11.6,-4.13829943400002));
#181868=CARTESIAN_POINT('Ctrl Pts',(10.2436106389999,15.2,-4.13837356000001));
#181869=CARTESIAN_POINT('Ctrl Pts',(10.2436106389999,11.6,-4.13837356000002));
#181870=CARTESIAN_POINT('Ctrl Pts',(10.2467638039999,15.2,-4.13844526200001));
#181871=CARTESIAN_POINT('Ctrl Pts',(10.2467638039999,11.6,-4.13844526200002));
#181872=CARTESIAN_POINT('Ctrl Pts',(10.2499222099999,15.2,-4.13851453000001));
#181873=CARTESIAN_POINT('Ctrl Pts',(10.2499222099999,11.6,-4.13851453000001));
#181874=CARTESIAN_POINT('Ctrl Pts',(10.2530858489999,15.2,-4.13858135800002));
#181875=CARTESIAN_POINT('Ctrl Pts',(10.2530858489999,11.6,-4.13858135800002));
#181876=CARTESIAN_POINT('Ctrl Pts',(10.2562547089999,15.2,-4.13864573900002));
#181877=CARTESIAN_POINT('Ctrl Pts',(10.2562547089999,11.6,-4.13864573900002));
#181878=CARTESIAN_POINT('Ctrl Pts',(10.2594287839999,15.2,-4.13870766500001));
#181879=CARTESIAN_POINT('Ctrl Pts',(10.2594287839999,11.6,-4.13870766500002));
#181880=CARTESIAN_POINT('Ctrl Pts',(10.2626080629999,15.2,-4.13876712900001));
#181881=CARTESIAN_POINT('Ctrl Pts',(10.2626080629999,11.6,-4.13876712900001));
#181882=CARTESIAN_POINT('Ctrl Pts',(10.2657925389999,15.2,-4.13882412400001));
#181883=CARTESIAN_POINT('Ctrl Pts',(10.2657925389999,11.6,-4.13882412400001));
#181884=CARTESIAN_POINT('Ctrl Pts',(10.2689822019999,15.2,-4.13887864300001));
#181885=CARTESIAN_POINT('Ctrl Pts',(10.2689822019999,11.6,-4.13887864300001));
#181886=CARTESIAN_POINT('Ctrl Pts',(10.2721770449999,15.2,-4.13893067800001));
#181887=CARTESIAN_POINT('Ctrl Pts',(10.2721770449999,11.6,-4.13893067800002));
#181888=CARTESIAN_POINT('Ctrl Pts',(10.2753770579999,15.2,-4.13898022200001));
#181889=CARTESIAN_POINT('Ctrl Pts',(10.2753770579999,11.6,-4.13898022200002));
#181890=CARTESIAN_POINT('Ctrl Pts',(10.2785822319999,15.2,-4.13902726900002));
#181891=CARTESIAN_POINT('Ctrl Pts',(10.2785822319999,11.6,-4.13902726900002));
#181892=CARTESIAN_POINT('Ctrl Pts',(10.2817925589999,15.2,-4.13907181100001));
#181893=CARTESIAN_POINT('Ctrl Pts',(10.2817925589999,11.6,-4.13907181100001));
#181894=CARTESIAN_POINT('Ctrl Pts',(10.2850080309999,15.2,-4.13911384100001));
#181895=CARTESIAN_POINT('Ctrl Pts',(10.2850080309999,11.6,-4.13911384100001));
#181896=CARTESIAN_POINT('Ctrl Pts',(10.2882286369999,15.2,-4.13915335100001));
#181897=CARTESIAN_POINT('Ctrl Pts',(10.2882286369999,11.6,-4.13915335100001));
#181898=CARTESIAN_POINT('Ctrl Pts',(10.2914543719999,15.2,-4.13919033700001));
#181899=CARTESIAN_POINT('Ctrl Pts',(10.2914543719999,11.6,-4.13919033700001));
#181900=CARTESIAN_POINT('Ctrl Pts',(10.2946852229999,15.2,-4.13922478800002));
#181901=CARTESIAN_POINT('Ctrl Pts',(10.2946852229999,11.6,-4.13922478800002));
#181902=CARTESIAN_POINT('Ctrl Pts',(10.2979211849999,15.2,-4.13925669900001));
#181903=CARTESIAN_POINT('Ctrl Pts',(10.2979211849999,11.6,-4.13925669900001));
#181904=CARTESIAN_POINT('Ctrl Pts',(10.3011622479999,15.2,-4.13928606400002));
#181905=CARTESIAN_POINT('Ctrl Pts',(10.3011622479999,11.6,-4.13928606400002));
#181906=CARTESIAN_POINT('Ctrl Pts',(10.3044084029999,15.2,-4.13931287500001));
#181907=CARTESIAN_POINT('Ctrl Pts',(10.3044084029999,11.6,-4.13931287500001));
#181908=CARTESIAN_POINT('Ctrl Pts',(10.3076596409999,15.2,-4.13933712400001));
#181909=CARTESIAN_POINT('Ctrl Pts',(10.3076596409999,11.6,-4.13933712400001));
#181910=CARTESIAN_POINT('Ctrl Pts',(10.3109159559999,15.2,-4.13935880700001));
#181911=CARTESIAN_POINT('Ctrl Pts',(10.3109159559999,11.6,-4.13935880700001));
#181912=CARTESIAN_POINT('Ctrl Pts',(10.3141773369999,15.2,-4.13937791300001));
#181913=CARTESIAN_POINT('Ctrl Pts',(10.3141773369999,11.6,-4.13937791300001));
#181914=CARTESIAN_POINT('Ctrl Pts',(10.3174437759999,15.2,-4.13939443800002));
#181915=CARTESIAN_POINT('Ctrl Pts',(10.3174437759999,11.6,-4.13939443800002));
#181916=CARTESIAN_POINT('Ctrl Pts',(10.3207152649999,15.2,-4.13940837600002));
#181917=CARTESIAN_POINT('Ctrl Pts',(10.3207152649999,11.6,-4.13940837600002));
#181918=CARTESIAN_POINT('Ctrl Pts',(10.3239917949999,15.2,-4.13941971700002));
#181919=CARTESIAN_POINT('Ctrl Pts',(10.3239917949999,11.6,-4.13941971700002));
#181920=CARTESIAN_POINT('Ctrl Pts',(10.3272733569999,15.2,-4.13942845600001));
#181921=CARTESIAN_POINT('Ctrl Pts',(10.3272733569999,11.6,-4.13942845600001));
#181922=CARTESIAN_POINT('Ctrl Pts',(10.3305599449999,15.2,-4.13943458700002));
#181923=CARTESIAN_POINT('Ctrl Pts',(10.3305599449999,11.6,-4.13943458700002));
#181924=CARTESIAN_POINT('Ctrl Pts',(10.3338515469999,15.2,-4.13943810200001));
#181925=CARTESIAN_POINT('Ctrl Pts',(10.3338515469999,11.6,-4.13943810200002));
#181926=CARTESIAN_POINT('Ctrl Pts',(10.3371481569999,15.2,-4.13943899400001));
#181927=CARTESIAN_POINT('Ctrl Pts',(10.3371481569999,11.6,-4.13943899400001));
#181928=CARTESIAN_POINT('Ctrl Pts',(10.3404497649999,15.2,-4.13943725700001));
#181929=CARTESIAN_POINT('Ctrl Pts',(10.3404497649999,11.6,-4.13943725700001));
#181930=CARTESIAN_POINT('Ctrl Pts',(10.3437563629999,15.2,-4.13943288400001));
#181931=CARTESIAN_POINT('Ctrl Pts',(10.3437563629999,11.6,-4.13943288400001));
#181932=CARTESIAN_POINT('Ctrl Pts',(10.3470679429999,15.2,-4.13942586900002));
#181933=CARTESIAN_POINT('Ctrl Pts',(10.3470679429999,11.6,-4.13942586900002));
#181934=CARTESIAN_POINT('Ctrl Pts',(10.3503844979999,15.2,-4.13941620500001));
#181935=CARTESIAN_POINT('Ctrl Pts',(10.3503844979999,11.6,-4.13941620500002));
#181936=CARTESIAN_POINT('Ctrl Pts',(10.3537060159999,15.2,-4.13940388400002));
#181937=CARTESIAN_POINT('Ctrl Pts',(10.3537060159999,11.6,-4.13940388400002));
#181938=CARTESIAN_POINT('Ctrl Pts',(10.3570324909999,15.2,-4.13938890200001));
#181939=CARTESIAN_POINT('Ctrl Pts',(10.3570324909999,11.6,-4.13938890200001));
#181940=CARTESIAN_POINT('Ctrl Pts',(10.3603639139999,15.2,-4.13937124900002));
#181941=CARTESIAN_POINT('Ctrl Pts',(10.3603639139999,11.6,-4.13937124900002));
#181942=CARTESIAN_POINT('Ctrl Pts',(10.3637002769999,15.2,-4.13935092100001));
#181943=CARTESIAN_POINT('Ctrl Pts',(10.3637002769999,11.6,-4.13935092100001));
#181944=CARTESIAN_POINT('Ctrl Pts',(10.3670415719999,15.2,-4.13932791100001));
#181945=CARTESIAN_POINT('Ctrl Pts',(10.3670415719999,11.6,-4.13932791100002));
#181946=CARTESIAN_POINT('Ctrl Pts',(10.3703877889999,15.2,-4.13930221300001));
#181947=CARTESIAN_POINT('Ctrl Pts',(10.3703877889999,11.6,-4.13930221300001));
#181948=CARTESIAN_POINT('Ctrl Pts',(10.3737389219999,15.2,-4.13927381900002));
#181949=CARTESIAN_POINT('Ctrl Pts',(10.3737389219999,11.6,-4.13927381900002));
#181950=CARTESIAN_POINT('Ctrl Pts',(10.3770949599999,15.2,-4.13924272200001));
#181951=CARTESIAN_POINT('Ctrl Pts',(10.3770949599999,11.6,-4.13924272200001));
#181952=CARTESIAN_POINT('Ctrl Pts',(10.3804558959999,15.2,-4.13920891800001));
#181953=CARTESIAN_POINT('Ctrl Pts',(10.3804558959999,11.6,-4.13920891800002));
#181954=CARTESIAN_POINT('Ctrl Pts',(10.3838217219999,15.2,-4.13917239800002));
#181955=CARTESIAN_POINT('Ctrl Pts',(10.3838217219999,11.6,-4.13917239800002));
#181956=CARTESIAN_POINT('Ctrl Pts',(10.3871924299999,15.2,-4.13913315800002));
#181957=CARTESIAN_POINT('Ctrl Pts',(10.3871924299999,11.6,-4.13913315800002));
#181958=CARTESIAN_POINT('Ctrl Pts',(10.3905680109999,15.2,-4.13909118900001));
#181959=CARTESIAN_POINT('Ctrl Pts',(10.3905680109999,11.6,-4.13909118900001));
#181960=CARTESIAN_POINT('Ctrl Pts',(10.3939484559999,15.2,-4.13904648600001));
#181961=CARTESIAN_POINT('Ctrl Pts',(10.3939484559999,11.6,-4.13904648600001));
#181962=CARTESIAN_POINT('Ctrl Pts',(10.3973337579999,15.2,-4.13899904300001));
#181963=CARTESIAN_POINT('Ctrl Pts',(10.3973337579999,11.6,-4.13899904300001));
#181964=CARTESIAN_POINT('Ctrl Pts',(10.4007239089999,15.2,-4.13894885300001));
#181965=CARTESIAN_POINT('Ctrl Pts',(10.4007239089999,11.6,-4.13894885300001));
#181966=CARTESIAN_POINT('Ctrl Pts',(10.4041188989999,15.2,-4.13889591000002));
#181967=CARTESIAN_POINT('Ctrl Pts',(10.4041188989999,11.6,-4.13889591000002));
#181968=CARTESIAN_POINT('Ctrl Pts',(10.4075187209999,15.2,-4.13884020700001));
#181969=CARTESIAN_POINT('Ctrl Pts',(10.4075187209999,11.6,-4.13884020700001));
#181970=CARTESIAN_POINT('Ctrl Pts',(10.4109233669999,15.2,-4.13878173800001));
#181971=CARTESIAN_POINT('Ctrl Pts',(10.4109233669999,11.6,-4.13878173800002));
#181972=CARTESIAN_POINT('Ctrl Pts',(10.4143328269999,15.2,-4.13872049700001));
#181973=CARTESIAN_POINT('Ctrl Pts',(10.4143328269999,11.6,-4.13872049700002));
#181974=CARTESIAN_POINT('Ctrl Pts',(10.4177470959999,15.2,-4.13865647700002));
#181975=CARTESIAN_POINT('Ctrl Pts',(10.4177470959999,11.6,-4.13865647700002));
#181976=CARTESIAN_POINT('Ctrl Pts',(10.4211661629999,15.2,-4.13858967300001));
#181977=CARTESIAN_POINT('Ctrl Pts',(10.4211661629999,11.6,-4.13858967300001));
#181978=CARTESIAN_POINT('Ctrl Pts',(10.4245900209999,15.2,-4.13852007700001));
#181979=CARTESIAN_POINT('Ctrl Pts',(10.4245900209999,11.6,-4.13852007700002));
#181980=CARTESIAN_POINT('Ctrl Pts',(10.4280186619999,15.2,-4.13844768400002));
#181981=CARTESIAN_POINT('Ctrl Pts',(10.4280186619999,11.6,-4.13844768400002));
#181982=CARTESIAN_POINT('Ctrl Pts',(10.4314520759999,15.2,-4.13837248700001));
#181983=CARTESIAN_POINT('Ctrl Pts',(10.4314520759999,11.6,-4.13837248700002));
#181984=CARTESIAN_POINT('Ctrl Pts',(10.4348902579999,15.2,-4.13829448200001));
#181985=CARTESIAN_POINT('Ctrl Pts',(10.4348902579999,11.6,-4.13829448200001));
#181986=CARTESIAN_POINT('Ctrl Pts',(10.4383331969999,15.2,-4.13821366000001));
#181987=CARTESIAN_POINT('Ctrl Pts',(10.4383331969999,11.6,-4.13821366000002));
#181988=CARTESIAN_POINT('Ctrl Pts',(10.4417808859999,15.2,-4.13813001600001));
#181989=CARTESIAN_POINT('Ctrl Pts',(10.4417808859999,11.6,-4.13813001600001));
#181990=CARTESIAN_POINT('Ctrl Pts',(10.4452333159999,15.2,-4.13804354400002));
#181991=CARTESIAN_POINT('Ctrl Pts',(10.4452333159999,11.6,-4.13804354400002));
#181992=CARTESIAN_POINT('Ctrl Pts',(10.4486904819999,15.2,-4.13795423800002));
#181993=CARTESIAN_POINT('Ctrl Pts',(10.4486904819999,11.6,-4.13795423800002));
#181994=CARTESIAN_POINT('Ctrl Pts',(10.4521523719999,15.2,-4.13786209000001));
#181995=CARTESIAN_POINT('Ctrl Pts',(10.4521523719999,11.6,-4.13786209000001));
#181996=CARTESIAN_POINT('Ctrl Pts',(10.4556189809999,15.2,-4.13776709800001));
#181997=CARTESIAN_POINT('Ctrl Pts',(10.4556189809999,11.6,-4.13776709800001));
#181998=CARTESIAN_POINT('Ctrl Pts',(10.4590902979999,15.2,-4.13766925300001));
#181999=CARTESIAN_POINT('Ctrl Pts',(10.4590902979999,11.6,-4.13766925300001));
#182000=CARTESIAN_POINT('Ctrl Pts',(10.4625663159999,15.2,-4.13756854800001));
#182001=CARTESIAN_POINT('Ctrl Pts',(10.4625663159999,11.6,-4.13756854800001));
#182002=CARTESIAN_POINT('Ctrl Pts',(10.4660470279999,15.2,-4.13746497900001));
#182003=CARTESIAN_POINT('Ctrl Pts',(10.4660470279999,11.6,-4.13746497900001));
#182004=CARTESIAN_POINT('Ctrl Pts',(10.4695324259999,15.2,-4.13735854000001));
#182005=CARTESIAN_POINT('Ctrl Pts',(10.4695324259999,11.6,-4.13735854000001));
#182006=CARTESIAN_POINT('Ctrl Pts',(10.4730225009999,15.2,-4.13724922400001));
#182007=CARTESIAN_POINT('Ctrl Pts',(10.4730225009999,11.6,-4.13724922400002));
#182008=CARTESIAN_POINT('Ctrl Pts',(10.4765172449999,15.2,-4.13713702500001));
#182009=CARTESIAN_POINT('Ctrl Pts',(10.4765172449999,11.6,-4.13713702500001));
#182010=CARTESIAN_POINT('Ctrl Pts',(10.4800166499999,15.2,-4.13702193900002));
#182011=CARTESIAN_POINT('Ctrl Pts',(10.4800166499999,11.6,-4.13702193900002));
#182012=CARTESIAN_POINT('Ctrl Pts',(10.4835207079999,15.2,-4.13690395700002));
#182013=CARTESIAN_POINT('Ctrl Pts',(10.4835207079999,11.6,-4.13690395700002));
#182014=CARTESIAN_POINT('Ctrl Pts',(10.4870294109999,15.2,-4.13678307500001));
#182015=CARTESIAN_POINT('Ctrl Pts',(10.4870294109999,11.6,-4.13678307500002));
#182016=CARTESIAN_POINT('Ctrl Pts',(10.4905427519999,15.2,-4.13665928700001));
#182017=CARTESIAN_POINT('Ctrl Pts',(10.4905427519999,11.6,-4.13665928700001));
#182018=CARTESIAN_POINT('Ctrl Pts',(10.4940607219999,15.2,-4.13653258700001));
#182019=CARTESIAN_POINT('Ctrl Pts',(10.4940607219999,11.6,-4.13653258700002));
#182020=CARTESIAN_POINT('Ctrl Pts',(10.4975833129999,15.2,-4.13640296900001));
#182021=CARTESIAN_POINT('Ctrl Pts',(10.4975833129999,11.6,-4.13640296900002));
#182022=CARTESIAN_POINT('Ctrl Pts',(10.5011105169999,15.2,-4.13627042700002));
#182023=CARTESIAN_POINT('Ctrl Pts',(10.5011105169999,11.6,-4.13627042700002));
#182024=CARTESIAN_POINT('Ctrl Pts',(10.5046423259999,15.2,-4.13613495500002));
#182025=CARTESIAN_POINT('Ctrl Pts',(10.5046423259999,11.6,-4.13613495500002));
#182026=CARTESIAN_POINT('Ctrl Pts',(10.5081787329999,15.2,-4.13599654600001));
#182027=CARTESIAN_POINT('Ctrl Pts',(10.5081787329999,11.6,-4.13599654600001));
#182028=CARTESIAN_POINT('Ctrl Pts',(10.5117197289999,15.2,-4.13585519800002));
#182029=CARTESIAN_POINT('Ctrl Pts',(10.5117197289999,11.6,-4.13585519800002));
#182030=CARTESIAN_POINT('Ctrl Pts',(10.5152653079999,15.2,-4.13571090200001));
#182031=CARTESIAN_POINT('Ctrl Pts',(10.5152653079999,11.6,-4.13571090200001));
#182032=CARTESIAN_POINT('Ctrl Pts',(10.5188154589999,15.2,-4.13556365200002));
#182033=CARTESIAN_POINT('Ctrl Pts',(10.5188154589999,11.6,-4.13556365200002));
#182034=CARTESIAN_POINT('Ctrl Pts',(10.5223701759999,15.2,-4.13541344400001));
#182035=CARTESIAN_POINT('Ctrl Pts',(10.5223701759999,11.6,-4.13541344400001));
#182036=CARTESIAN_POINT('Ctrl Pts',(10.5259294509999,15.2,-4.13526027200001));
#182037=CARTESIAN_POINT('Ctrl Pts',(10.5259294509999,11.6,-4.13526027200002));
#182038=CARTESIAN_POINT('Ctrl Pts',(10.5294932759999,15.2,-4.13510413000001));
#182039=CARTESIAN_POINT('Ctrl Pts',(10.5294932759999,11.6,-4.13510413000001));
#182040=CARTESIAN_POINT('Ctrl Pts',(10.5330616439999,15.2,-4.13494501200002));
#182041=CARTESIAN_POINT('Ctrl Pts',(10.5330616439999,11.6,-4.13494501200002));
#182042=CARTESIAN_POINT('Ctrl Pts',(10.5366345439999,15.2,-4.13478291300001));
#182043=CARTESIAN_POINT('Ctrl Pts',(10.5366345439999,11.6,-4.13478291300002));
#182044=CARTESIAN_POINT('Ctrl Pts',(10.5402119719999,15.2,-4.13461782500002));
#182045=CARTESIAN_POINT('Ctrl Pts',(10.5402119719999,11.6,-4.13461782500002));
#182046=CARTESIAN_POINT('Ctrl Pts',(10.5437939179999,15.2,-4.13444974600001));
#182047=CARTESIAN_POINT('Ctrl Pts',(10.5437939179999,11.6,-4.13444974600001));
#182048=CARTESIAN_POINT('Ctrl Pts',(10.5473803739999,15.2,-4.13427866800001));
#182049=CARTESIAN_POINT('Ctrl Pts',(10.5473803739999,11.6,-4.13427866800001));
#182050=CARTESIAN_POINT('Ctrl Pts',(10.5509713329999,15.2,-4.13410458600001));
#182051=CARTESIAN_POINT('Ctrl Pts',(10.5509713329999,11.6,-4.13410458600001));
#182052=CARTESIAN_POINT('Ctrl Pts',(10.5545667879999,15.2,-4.13392749400002));
#182053=CARTESIAN_POINT('Ctrl Pts',(10.5545667879999,11.6,-4.13392749400002));
#182054=CARTESIAN_POINT('Ctrl Pts',(10.5581667289999,15.2,-4.13374738700002));
#182055=CARTESIAN_POINT('Ctrl Pts',(10.5581667289999,11.6,-4.13374738700002));
#182056=CARTESIAN_POINT('Ctrl Pts',(10.5617711499999,15.2,-4.13356425800002));
#182057=CARTESIAN_POINT('Ctrl Pts',(10.5617711499999,11.6,-4.13356425800002));
#182058=CARTESIAN_POINT('Ctrl Pts',(10.5653800419999,15.2,-4.13337810400002));
#182059=CARTESIAN_POINT('Ctrl Pts',(10.5653800419999,11.6,-4.13337810400002));
#182060=CARTESIAN_POINT('Ctrl Pts',(10.5689933989999,15.2,-4.13318891700001));
#182061=CARTESIAN_POINT('Ctrl Pts',(10.5689933989999,11.6,-4.13318891700001));
#182062=CARTESIAN_POINT('Ctrl Pts',(10.5726112109999,15.2,-4.13299669400002));
#182063=CARTESIAN_POINT('Ctrl Pts',(10.5726112109999,11.6,-4.13299669400002));
#182064=CARTESIAN_POINT('Ctrl Pts',(10.5762334719999,15.2,-4.13280142700001));
#182065=CARTESIAN_POINT('Ctrl Pts',(10.5762334719999,11.6,-4.13280142700002));
#182066=CARTESIAN_POINT('Ctrl Pts',(10.5798601729999,15.2,-4.13260311100001));
#182067=CARTESIAN_POINT('Ctrl Pts',(10.5798601729999,11.6,-4.13260311100002));
#182068=CARTESIAN_POINT('Ctrl Pts',(10.5834913069999,15.2,-4.13240174200002));
#182069=CARTESIAN_POINT('Ctrl Pts',(10.5834913069999,11.6,-4.13240174200002));
#182070=CARTESIAN_POINT('Ctrl Pts',(10.5871268649999,15.2,-4.13219731300002));
#182071=CARTESIAN_POINT('Ctrl Pts',(10.5871268649999,11.6,-4.13219731300002));
#182072=CARTESIAN_POINT('Ctrl Pts',(10.5907668409999,15.2,-4.13198982000001));
#182073=CARTESIAN_POINT('Ctrl Pts',(10.5907668409999,11.6,-4.13198982000001));
#182074=CARTESIAN_POINT('Ctrl Pts',(10.5944112269999,15.2,-4.13177925500001));
#182075=CARTESIAN_POINT('Ctrl Pts',(10.5944112269999,11.6,-4.13177925500001));
#182076=CARTESIAN_POINT('Ctrl Pts',(10.5980600139999,15.2,-4.13156561600001));
#182077=CARTESIAN_POINT('Ctrl Pts',(10.5980600139999,11.6,-4.13156561600002));
#182078=CARTESIAN_POINT('Ctrl Pts',(10.6017131959999,15.2,-4.13134889500002));
#182079=CARTESIAN_POINT('Ctrl Pts',(10.6017131959999,11.6,-4.13134889500002));
#182080=CARTESIAN_POINT('Ctrl Pts',(10.6053707649999,15.2,-4.13112908800001));
#182081=CARTESIAN_POINT('Ctrl Pts',(10.6053707649999,11.6,-4.13112908800001));
#182082=CARTESIAN_POINT('Ctrl Pts',(10.6090327119999,15.2,-4.13090618900001));
#182083=CARTESIAN_POINT('Ctrl Pts',(10.6090327119999,11.6,-4.13090618900002));
#182084=CARTESIAN_POINT('Ctrl Pts',(10.6126990299999,15.2,-4.13068019300002));
#182085=CARTESIAN_POINT('Ctrl Pts',(10.6126990299999,11.6,-4.13068019300002));
#182086=CARTESIAN_POINT('Ctrl Pts',(10.6163697119999,15.2,-4.13045109400001));
#182087=CARTESIAN_POINT('Ctrl Pts',(10.6163697119999,11.6,-4.13045109400001));
#182088=CARTESIAN_POINT('Ctrl Pts',(10.6200447499999,15.2,-4.13021888800001));
#182089=CARTESIAN_POINT('Ctrl Pts',(10.6200447499999,11.6,-4.13021888800001));
#182090=CARTESIAN_POINT('Ctrl Pts',(10.6237241349999,15.2,-4.12998356800002));
#182091=CARTESIAN_POINT('Ctrl Pts',(10.6237241349999,11.6,-4.12998356800002));
#182092=CARTESIAN_POINT('Ctrl Pts',(10.6274078609999,15.2,-4.12974512900002));
#182093=CARTESIAN_POINT('Ctrl Pts',(10.6274078609999,11.6,-4.12974512900002));
#182094=CARTESIAN_POINT('Ctrl Pts',(10.6310959199999,15.2,-4.12950356700001));
#182095=CARTESIAN_POINT('Ctrl Pts',(10.6310959199999,11.6,-4.12950356700002));
#182096=CARTESIAN_POINT('Ctrl Pts',(10.6347883039999,15.2,-4.12925887700001));
#182097=CARTESIAN_POINT('Ctrl Pts',(10.6347883039999,11.6,-4.12925887700002));
#182098=CARTESIAN_POINT('Ctrl Pts',(10.6384850049999,15.2,-4.12901105200001));
#182099=CARTESIAN_POINT('Ctrl Pts',(10.6384850049999,11.6,-4.12901105200001));
#182100=CARTESIAN_POINT('Ctrl Pts',(10.6421860169999,15.2,-4.12876008700001));
#182101=CARTESIAN_POINT('Ctrl Pts',(10.6421860169999,11.6,-4.12876008700001));
#182102=CARTESIAN_POINT('Ctrl Pts',(10.6458913319999,15.2,-4.12850597800002));
#182103=CARTESIAN_POINT('Ctrl Pts',(10.6458913319999,11.6,-4.12850597800002));
#182104=CARTESIAN_POINT('Ctrl Pts',(10.6496009419999,15.2,-4.12824872000002));
#182105=CARTESIAN_POINT('Ctrl Pts',(10.6496009419999,11.6,-4.12824872000002));
#182106=CARTESIAN_POINT('Ctrl Pts',(10.6533148399999,15.2,-4.12798830700002));
#182107=CARTESIAN_POINT('Ctrl Pts',(10.6533148399999,11.6,-4.12798830700002));
#182108=CARTESIAN_POINT('Ctrl Pts',(10.6570330169999,15.2,-4.12772473300001));
#182109=CARTESIAN_POINT('Ctrl Pts',(10.6570330169999,11.6,-4.12772473300001));
#182110=CARTESIAN_POINT('Ctrl Pts',(10.6607554659999,15.2,-4.12745799400001));
#182111=CARTESIAN_POINT('Ctrl Pts',(10.6607554659999,11.6,-4.12745799400002));
#182112=CARTESIAN_POINT('Ctrl Pts',(10.6644821789999,15.2,-4.12718808500002));
#182113=CARTESIAN_POINT('Ctrl Pts',(10.6644821789999,11.6,-4.12718808500002));
#182114=CARTESIAN_POINT('Ctrl Pts',(10.6682131479999,15.2,-4.12691499800002));
#182115=CARTESIAN_POINT('Ctrl Pts',(10.6682131479999,11.6,-4.12691499800002));
#182116=CARTESIAN_POINT('Ctrl Pts',(10.6719483659999,15.2,-4.12663873100001));
#182117=CARTESIAN_POINT('Ctrl Pts',(10.6719483659999,11.6,-4.12663873100001));
#182118=CARTESIAN_POINT('Ctrl Pts',(10.6756878259999,15.2,-4.12635927800002));
#182119=CARTESIAN_POINT('Ctrl Pts',(10.6756878259999,11.6,-4.12635927800002));
#182120=CARTESIAN_POINT('Ctrl Pts',(10.6794315189999,15.2,-4.12607663400001));
#182121=CARTESIAN_POINT('Ctrl Pts',(10.6794315189999,11.6,-4.12607663400001));
#182122=CARTESIAN_POINT('Ctrl Pts',(10.6831794419999,15.2,-4.12579079500001));
#182123=CARTESIAN_POINT('Ctrl Pts',(10.6831794419999,11.6,-4.12579079500001));
#182124=CARTESIAN_POINT('Ctrl Pts',(10.6869315859999,15.2,-4.12550175600002));
#182125=CARTESIAN_POINT('Ctrl Pts',(10.6869315859999,11.6,-4.12550175600002));
#182126=CARTESIAN_POINT('Ctrl Pts',(10.6906879429999,15.2,-4.12520951200001));
#182127=CARTESIAN_POINT('Ctrl Pts',(10.6906879429999,11.6,-4.12520951200001));
#182128=CARTESIAN_POINT('Ctrl Pts',(10.6944485069999,15.2,-4.12491405900001));
#182129=CARTESIAN_POINT('Ctrl Pts',(10.6944485069999,11.6,-4.12491405900001));
#182130=CARTESIAN_POINT('Ctrl Pts',(10.6982132689999,15.2,-4.12461539000001));
#182131=CARTESIAN_POINT('Ctrl Pts',(10.6982132689999,11.6,-4.12461539000002));
#182132=CARTESIAN_POINT('Ctrl Pts',(10.7019822189999,15.2,-4.12431349900002));
#182133=CARTESIAN_POINT('Ctrl Pts',(10.7019822189999,11.6,-4.12431349900002));
#182134=CARTESIAN_POINT('Ctrl Pts',(10.7057553479999,15.2,-4.12400838100002));
#182135=CARTESIAN_POINT('Ctrl Pts',(10.7057553479999,11.6,-4.12400838100002));
#182136=CARTESIAN_POINT('Ctrl Pts',(10.7095326469999,15.2,-4.12370002800001));
#182137=CARTESIAN_POINT('Ctrl Pts',(10.7095326469999,11.6,-4.12370002800001));
#182138=CARTESIAN_POINT('Ctrl Pts',(10.7133141079999,15.2,-4.12338843600002));
#182139=CARTESIAN_POINT('Ctrl Pts',(10.7133141079999,11.6,-4.12338843600002));
#182140=CARTESIAN_POINT('Ctrl Pts',(10.7170997259999,15.2,-4.12307359900002));
#182141=CARTESIAN_POINT('Ctrl Pts',(10.7170997259999,11.6,-4.12307359900002));
#182142=CARTESIAN_POINT('Ctrl Pts',(10.7208894919999,15.2,-4.12275551600001));
#182143=CARTESIAN_POINT('Ctrl Pts',(10.7208894919999,11.6,-4.12275551600001));
#182144=CARTESIAN_POINT('Ctrl Pts',(10.7246834049999,15.2,-4.12243418400001));
#182145=CARTESIAN_POINT('Ctrl Pts',(10.7246834049999,11.6,-4.12243418400002));
#182146=CARTESIAN_POINT('Ctrl Pts',(10.7284814639999,15.2,-4.12210960000001));
#182147=CARTESIAN_POINT('Ctrl Pts',(10.7284814639999,11.6,-4.12210960000001));
#182148=CARTESIAN_POINT('Ctrl Pts',(10.7315232249999,15.2,-4.12184733300001));
#182149=CARTESIAN_POINT('Ctrl Pts',(10.7315232249999,11.6,-4.12184733300002));
#182150=CARTESIAN_POINT('Ctrl Pts',(10.7338064109999,15.2,-4.12164917000001));
#182151=CARTESIAN_POINT('Ctrl Pts',(10.7338064109999,11.6,-4.12164917000002));
#182152=CARTESIAN_POINT('Ctrl Pts',(10.7353293639999,15.2,-4.12151641100001));
#182153=CARTESIAN_POINT('Ctrl Pts',(10.7353293639999,11.6,-4.12151641100001));
#182154=CARTESIAN_POINT('Ctrl Pts',(10.7360910479999,15.2,-4.12144986800001));
#182155=CARTESIAN_POINT('Ctrl Pts',(10.7360910479999,11.6,-4.12144986800001));
#182156=CARTESIAN_POINT('Ctrl Pts',(9.55499537099995,15.2,-4.04260911600002));
#182157=CARTESIAN_POINT('Ctrl Pts',(9.55669454752162,15.2,-4.04316130584455));
#182158=CARTESIAN_POINT('Ctrl Pts',(9.55844976514545,15.2,-4.04372605389322));
#182159=CARTESIAN_POINT('Ctrl Pts',(9.5602602775349,15.2,-4.04430244593687));
#182160=CARTESIAN_POINT('Ctrl Pts',(9.56207952113026,15.2,-4.04488161763431));
#182161=CARTESIAN_POINT('Ctrl Pts',(9.56395460122355,15.2,-4.04547254558642));
#182162=CARTESIAN_POINT('Ctrl Pts',(9.56588480617837,15.2,-4.04607433356657));
#182163=CARTESIAN_POINT('Ctrl Pts',(9.56781501095787,15.2,-4.04667612149206));
#182164=CARTESIAN_POINT('Ctrl Pts',(9.56980034124062,15.2,-4.04728876912261));
#182165=CARTESIAN_POINT('Ctrl Pts',(9.57184010199984,15.2,-4.04791140626666));
#182166=CARTESIAN_POINT('Ctrl Pts',(9.57387986275907,15.2,-4.04853404341071));
#182167=CARTESIAN_POINT('Ctrl Pts',(9.57597405360772,15.1999999999999,-4.04916667193805));
#182168=CARTESIAN_POINT('Ctrl Pts',(9.57812199955053,15.2,-4.04980844719627));
#182169=CARTESIAN_POINT('Ctrl Pts',(9.58026994568846,15.2,-4.05045022251278));
#182170=CARTESIAN_POINT('Ctrl Pts',(9.5824716464358,15.2,-4.0511011466437));
#182171=CARTESIAN_POINT('Ctrl Pts',(9.58472643972897,15.2,-4.05176039909686));
#182172=CARTESIAN_POINT('Ctrl Pts',(9.58698123281733,15.2,-4.05241965149014));
#182173=CARTESIAN_POINT('Ctrl Pts',(9.58928912248419,15.2,-4.05308723447175));
#182174=CARTESIAN_POINT('Ctrl Pts',(9.5916494594926,15.2,-4.05376235378364));
#182175=CARTESIAN_POINT('Ctrl Pts',(9.59400979650101,15.2,-4.05443747309553));
#182176=CARTESIAN_POINT('Ctrl Pts',(9.59642258389921,15.2,-4.05512012896279));
#182177=CARTESIAN_POINT('Ctrl Pts',(9.59888719089075,15.2,-4.05580954952079));
#182178=CARTESIAN_POINT('Ctrl Pts',(9.60135179810616,15.2,-4.0564989701414));
#182179=CARTESIAN_POINT('Ctrl Pts',(9.60386822553632,15.2,-4.05719515745453));
#182180=CARTESIAN_POINT('Ctrl Pts',(9.60643585601307,15.2,-4.05789736282655));
#182181=CARTESIAN_POINT('Ctrl Pts',(9.6090034862566,15.2,-4.05859956813477));
#182182=CARTESIAN_POINT('Ctrl Pts',(9.61162232317368,15.2,-4.05930778903961));
#182183=CARTESIAN_POINT('Ctrl Pts',(9.61429176141222,15.2,-4.06002130076391));
#182184=CARTESIAN_POINT('Ctrl Pts',(9.61696119965077,15.2,-4.06073481248822));
#182185=CARTESIAN_POINT('Ctrl Pts',(9.61968124046026,15.2,-4.06145361577042));
#182186=CARTESIAN_POINT('Ctrl Pts',(9.62245129460743,15.2,-4.06217699974393));
#182187=CARTESIAN_POINT('Ctrl Pts',(9.6252213487546,15.2,-4.06290038371745));
#182188=CARTESIAN_POINT('Ctrl Pts',(9.62804141715304,15.2,-4.06362835221376));
#182189=CARTESIAN_POINT('Ctrl Pts',(9.63091092146209,15.2,-4.0643602141869));
#182190=CARTESIAN_POINT('Ctrl Pts',(9.63378042603179,15.2,-4.06509207622652));
#182191=CARTESIAN_POINT('Ctrl Pts',(9.63669936976461,15.2,-4.06582783364988));
#182192=CARTESIAN_POINT('Ctrl Pts',(9.63966718442848,15.2,-4.06656681652363));
#182193=CARTESIAN_POINT('Ctrl Pts',(9.64263499882278,15.2,-4.06730579933026));
#182194=CARTESIAN_POINT('Ctrl Pts',(9.64565168593768,15.2,-4.06804800581502));
#182195=CARTESIAN_POINT('Ctrl Pts',(9.64871669225681,15.2,-4.06879278770801));
#182196=CARTESIAN_POINT('Ctrl Pts',(9.65178169857594,15.2,-4.06953756960099));
#182197=CARTESIAN_POINT('Ctrl Pts',(9.65489502329009,15.2,-4.07028492392903));
#182198=CARTESIAN_POINT('Ctrl Pts',(9.65805612383864,15.2,-4.07103421890167));
#182199=CARTESIAN_POINT('Ctrl Pts',(9.66121722467433,15.2,-4.07178351394237));
#182200=CARTESIAN_POINT('Ctrl Pts',(9.66442610292301,15.2,-4.07253474644996));
#182201=CARTESIAN_POINT('Ctrl Pts',(9.66768222468585,15.2,-4.07328730149103));
#182202=CARTESIAN_POINT('Ctrl Pts',(9.67093834615294,15.2,-4.07403985646375));
#182203=CARTESIAN_POINT('Ctrl Pts',(9.67424171158829,15.2,-4.07479373162366));
#182204=CARTESIAN_POINT('Ctrl Pts',(9.67759179898168,15.2,-4.07554832576634));
#182205=CARTESIAN_POINT('Ctrl Pts',(9.68094188637507,15.2,-4.07630291990901));
#182206=CARTESIAN_POINT('Ctrl Pts',(9.68433869487785,15.2,-4.07705823111179));
#182207=CARTESIAN_POINT('Ctrl Pts',(9.68778171333292,15.2,-4.07781367441767));
#182208=CARTESIAN_POINT('Ctrl Pts',(9.69122473210076,15.2,-4.07856911779216));
#182209=CARTESIAN_POINT('Ctrl Pts',(9.69471395864503,15.2,-4.07932469331921));
#182210=CARTESIAN_POINT('Ctrl Pts',(9.69824889160027,15.2,-4.08007982581473));
#182211=CARTESIAN_POINT('Ctrl Pts',(9.70178382423443,15.2,-4.08083495824166));
#182212=CARTESIAN_POINT('Ctrl Pts',(9.70536446092327,15.2,-4.0815896501774));
#182213=CARTESIAN_POINT('Ctrl Pts',(9.70899030854152,15.2,-4.08234334148335));
#182214=CARTESIAN_POINT('Ctrl Pts',(9.7126161561598,15.2,-4.0830970327893));
#182215=CARTESIAN_POINT('Ctrl Pts',(9.71628721518416,15.2,-4.08384972393369));
#182216=CARTESIAN_POINT('Ctrl Pts',(9.72000299714885,15.2,-4.08460086944402));
#182217=CARTESIAN_POINT('Ctrl Pts',(9.72371877945107,15.2,-4.08535201502257));
#182218=CARTESIAN_POINT('Ctrl Pts',(9.72747928619589,15.2,-4.08610161413256));
#182219=CARTESIAN_POINT('Ctrl Pts',(9.73128403915626,15.2,-4.08684913758983));
#182220=CARTESIAN_POINT('Ctrl Pts',(9.73508879177105,15.2,-4.0875966609792));
#182221=CARTESIAN_POINT('Ctrl Pts',(9.73893778845863,15.2,-4.08834210619898));
#182222=CARTESIAN_POINT('Ctrl Pts',(9.74283056200164,15.2,-4.08908495475869));
#182223=CARTESIAN_POINT('Ctrl Pts',(9.74737213137088,15.2,-4.08995161145667));
#182224=CARTESIAN_POINT('Ctrl Pts',(9.75197328098147,15.2,-4.09081473398381));
#182225=CARTESIAN_POINT('Ctrl Pts',(9.75663328216859,15.2,-4.09167351587192));
#182226=CARTESIAN_POINT('Ctrl Pts',(9.75996185439326,15.2,-4.09228693149674));
#182227=CARTESIAN_POINT('Ctrl Pts',(9.76332045013508,15.2,-4.09289813396317));
#182228=CARTESIAN_POINT('Ctrl Pts',(9.76670880840141,15.2,-4.09350683708797));
#182229=CARTESIAN_POINT('Ctrl Pts',(9.77009716629839,15.2,-4.09411554014641));
#182230=CARTESIAN_POINT('Ctrl Pts',(9.7735152854049,15.2,-4.09472174296442));
#182231=CARTESIAN_POINT('Ctrl Pts',(9.7769629057906,15.2,-4.09532516595443));
#182232=CARTESIAN_POINT('Ctrl Pts',(9.78041052655207,15.2,-4.09592858901021));
#182233=CARTESIAN_POINT('Ctrl Pts',(9.78388764923809,15.2,-4.09652923184938));
#182234=CARTESIAN_POINT('Ctrl Pts',(9.78739401749958,15.2,-4.09712681844686));
#182235=CARTESIAN_POINT('Ctrl Pts',(9.79090038576108,15.2,-4.09772440504433));
#182236=CARTESIAN_POINT('Ctrl Pts',(9.79443599743787,15.2,-4.0983189360905));
#182237=CARTESIAN_POINT('Ctrl Pts',(9.79800060108618,15.2,-4.09891014098138));
#182238=CARTESIAN_POINT('Ctrl Pts',(9.80156520473446,15.2,-4.09950134587226));
#182239=CARTESIAN_POINT('Ctrl Pts',(9.80515880008132,15.2,-4.10008922340605));
#182240=CARTESIAN_POINT('Ctrl Pts',(9.80878113591315,15.2,-4.10067351146179));
#182241=CARTESIAN_POINT('Ctrl Pts',(9.81240347174498,15.2,-4.10125779951754));
#182242=CARTESIAN_POINT('Ctrl Pts',(9.81605454826645,15.2,-4.10183849555097));
#182243=CARTESIAN_POINT('Ctrl Pts',(9.81973411750107,15.2,-4.10241533895394));
#182244=CARTESIAN_POINT('Ctrl Pts',(9.82341368673569,15.2,-4.10299218235692));
#182245=CARTESIAN_POINT('Ctrl Pts',(9.82712175031428,15.2,-4.10356517651379));
#182246=CARTESIAN_POINT('Ctrl Pts',(9.83085806199784,15.2,-4.10413406151638));
#182247=CARTESIAN_POINT('Ctrl Pts',(9.83459437368139,15.2,-4.10470294651897));
#182248=CARTESIAN_POINT('Ctrl Pts',(9.83835893321653,15.2,-4.10526772402225));
#182249=CARTESIAN_POINT('Ctrl Pts',(9.84215150071653,15.2,-4.10582814471669));
#182250=CARTESIAN_POINT('Ctrl Pts',(9.84594406821654,15.2,-4.10638856541114));
#182251=CARTESIAN_POINT('Ctrl Pts',(9.84976464223998,15.2,-4.10694462624784));
#182252=CARTESIAN_POINT('Ctrl Pts',(9.85361298399364,15.2,-4.10749608375033));
#182253=CARTESIAN_POINT('Ctrl Pts',(9.8574613257473,15.2,-4.10804754125282));
#182254=CARTESIAN_POINT('Ctrl Pts',(9.86133743455946,15.2,-4.10859439337459));
#182255=CARTESIAN_POINT('Ctrl Pts',(9.86524107546368,15.2,-4.10913639927711));
#182256=CARTESIAN_POINT('Ctrl Pts',(9.86914471636789,15.2,-4.10967840517963));
#182257=CARTESIAN_POINT('Ctrl Pts',(9.87307588871861,15.2,-4.11021556404617));
#182258=CARTESIAN_POINT('Ctrl Pts',(9.87703435802559,15.2,-4.11074763980979));
#182259=CARTESIAN_POINT('Ctrl Pts',(9.88099282733258,15.2,-4.11127971557342));
#182260=CARTESIAN_POINT('Ctrl Pts',(9.88497859533885,15.2,-4.11180670547328));
#182261=CARTESIAN_POINT('Ctrl Pts',(9.88899142881248,15.2,-4.11232837825078));
#182262=CARTESIAN_POINT('Ctrl Pts',(9.89300426228612,15.2,-4.11285005102828));
#182263=CARTESIAN_POINT('Ctrl Pts',(9.89704416150592,15.2,-4.11336640671751));
#182264=CARTESIAN_POINT('Ctrl Pts',(9.90111089928039,15.2,-4.11387721507597));
#182265=CARTESIAN_POINT('Ctrl Pts',(9.90517763705487,15.2,-4.11438802343444));
#182266=CARTESIAN_POINT('Ctrl Pts',(9.90927121277551,15.2,-4.11489328303806));
#182267=CARTESIAN_POINT('Ctrl Pts',(9.91339139805547,15.2,-4.11539277081536));
#182268=CARTESIAN_POINT('Ctrl Pts',(9.91668754600997,15.2,-4.11579236100454));
#182269=CARTESIAN_POINT('Ctrl Pts',(9.92000072505391,15.2,-4.11618825772474));
#182270=CARTESIAN_POINT('Ctrl Pts',(9.9233308215028,15.2,-4.11658034519294));
#182271=CARTESIAN_POINT('Ctrl Pts',(9.92666091840542,15.2,-4.11697243271456));
#182272=CARTESIAN_POINT('Ctrl Pts',(9.93000793043803,15.2,-4.11736071279098));
#182273=CARTESIAN_POINT('Ctrl Pts',(9.93337174551308,15.2,-4.11774507233078));
#182274=CARTESIAN_POINT('Ctrl Pts',(9.93757651412774,15.2,-4.11822552172936));
#182275=CARTESIAN_POINT('Ctrl Pts',(9.9418075368157,15.2,-4.11869984502843));
#182276=CARTESIAN_POINT('Ctrl Pts',(9.94606459133171,15.2,-4.11916782856957));
#182277=CARTESIAN_POINT('Ctrl Pts',(9.95032164584772,15.2,-4.11963581211072));
#182278=CARTESIAN_POINT('Ctrl Pts',(9.95460473415027,15.2,-4.12009745346009));
#182279=CARTESIAN_POINT('Ctrl Pts',(9.95891363755516,15.2,-4.12055254283456));
#182280=CARTESIAN_POINT('Ctrl Pts',(9.96236075999727,15.2,-4.12091661430437));
#182281=CARTESIAN_POINT('Ctrl Pts',(9.96582440315237,15.2,-4.12127649245501));
#182282=CARTESIAN_POINT('Ctrl Pts',(9.96930445827251,15.2,-4.12163206998312));
#182283=CARTESIAN_POINT('Ctrl Pts',(9.97278451386681,15.2,-4.12198764755968));
#182284=CARTESIAN_POINT('Ctrl Pts',(9.97628097918112,15.2,-4.12233892321329));
#182285=CARTESIAN_POINT('Ctrl Pts',(9.97979374504089,15.2,-4.12268579406508));
#182286=CARTESIAN_POINT('Ctrl Pts',(9.9841847021263,15.2,-4.12311938260618));
#182287=CARTESIAN_POINT('Ctrl Pts',(9.98860112993991,15.2,-4.12354608572216));
#182288=CARTESIAN_POINT('Ctrl Pts',(9.99304281508086,15.2,-4.12396570259658));
#182289=CARTESIAN_POINT('Ctrl Pts',(9.99659616290314,15.2,-4.12430139606867));
#182290=CARTESIAN_POINT('Ctrl Pts',(10.0001656746993,15.2,-4.12463255399445));
#182291=CARTESIAN_POINT('Ctrl Pts',(10.0037512432558,15.2,-4.12495907302481));
#182292=CARTESIAN_POINT('Ctrl Pts',(10.0073368123007,15.2,-4.12528559209966));
#182293=CARTESIAN_POINT('Ctrl Pts',(10.0109384374204,15.2,-4.12560747351564));
#182294=CARTESIAN_POINT('Ctrl Pts',(10.0145560118414,15.2,-4.12592461581022));
#182295=CARTESIAN_POINT('Ctrl Pts',(10.0181735857695,15.2,-4.12624175806159));
#182296=CARTESIAN_POINT('Ctrl Pts',(10.021807108865,15.2,-4.12655416099134));
#182297=CARTESIAN_POINT('Ctrl Pts',(10.0254564741767,15.2,-4.12686172646651));
#182298=CARTESIAN_POINT('Ctrl Pts',(10.0291058399857,15.2,-4.12716929198359));
#182299=CARTESIAN_POINT('Ctrl Pts',(10.032771049626,15.2,-4.12747201726254));
#182300=CARTESIAN_POINT('Ctrl Pts',(10.0364519955674,15.2,-4.12776980629322));
#182301=CARTESIAN_POINT('Ctrl Pts',(10.0401329410073,15.2,-4.12806759528332));
#182302=CARTESIAN_POINT('Ctrl Pts',(10.0438296222261,15.2,-4.12836044756077));
#182303=CARTESIAN_POINT('Ctrl Pts',(10.0475419367549,15.2,-4.12864826642646));
#182304=CARTESIAN_POINT('Ctrl Pts',(10.0512542517895,15.2,-4.12893608533136));
#182305=CARTESIAN_POINT('Ctrl Pts',(10.0549821979677,15.2,-4.12921886979678));
#182306=CARTESIAN_POINT('Ctrl Pts',(10.0587256718394,15.2,-4.12949652425602));
#182307=CARTESIAN_POINT('Ctrl Pts',(10.0624691452011,15.2,-4.12977417867743));
#182308=CARTESIAN_POINT('Ctrl Pts',(10.0662281469708,15.2,-4.13004670417204));
#182309=CARTESIAN_POINT('Ctrl Pts',(10.0700025724606,15.2,-4.13031400521955));
#182310=CARTESIAN_POINT('Ctrl Pts',(10.0756642114667,15.2,-4.13071495684545));
#182311=CARTESIAN_POINT('Ctrl Pts',(10.0813605547099,15.2,-4.13110415353808));
#182312=CARTESIAN_POINT('Ctrl Pts',(10.0870912563579,15.2,-4.13148128205781));
#182313=CARTESIAN_POINT('Ctrl Pts',(10.0909117236027,15.2,-4.1317327010367));
#182314=CARTESIAN_POINT('Ctrl Pts',(10.094747460351,15.2,-4.1319787556163));
#182315=CARTESIAN_POINT('Ctrl Pts',(10.0985983657019,15.2,-4.13221935526365));
#182316=CARTESIAN_POINT('Ctrl Pts',(10.1024492715774,15.2,-4.13245995494378));
#182317=CARTESIAN_POINT('Ctrl Pts',(10.1063153470064,15.2,-4.13269509896259));
#182318=CARTESIAN_POINT('Ctrl Pts',(10.1101964890798,15.2,-4.13292469804165));
#182319=CARTESIAN_POINT('Ctrl Pts',(10.1160182016611,15.2,-4.13326909662895));
#182320=CARTESIAN_POINT('Ctrl Pts',(10.1218738153805,15.2,-4.13360101655331));
#182321=CARTESIAN_POINT('Ctrl Pts',(10.1277629934999,15.2,-4.13392015829171));
#182322=CARTESIAN_POINT('Ctrl Pts',(10.1316891126027,15.2,-4.13413291946997));
#182323=CARTESIAN_POINT('Ctrl Pts',(10.1356301476796,15.2,-4.13434000196146));
#182324=CARTESIAN_POINT('Ctrl Pts',(10.1395860008967,15.2,-4.13454131774962));
#182325=CARTESIAN_POINT('Ctrl Pts',(10.1435418535748,15.2,-4.13474263351034));
#182326=CARTESIAN_POINT('Ctrl Pts',(10.1475125251883,15.2,-4.13493818343953));
#182327=CARTESIAN_POINT('Ctrl Pts',(10.1514979145472,15.2,-4.13512787925824));
#182328=CARTESIAN_POINT('Ctrl Pts',(10.1554833044491,15.2,-4.13531757510279));
#182329=CARTESIAN_POINT('Ctrl Pts',(10.1594834128471,15.2,-4.13550141822281));
#182330=CARTESIAN_POINT('Ctrl Pts',(10.163498142623,15.2,-4.13567932328746));
#182331=CARTESIAN_POINT('Ctrl Pts',(10.1695202367397,15.2,-4.13594618086018));
#182332=CARTESIAN_POINT('Ctrl Pts',(10.1755752267961,15.2,-4.13619967582542));
#182333=CARTESIAN_POINT('Ctrl Pts',(10.1816627849915,15.2,-4.13643952648337));
#182334=CARTESIAN_POINT('Ctrl Pts',(10.1857211574905,15.2,-4.13659942693653));
#182335=CARTESIAN_POINT('Ctrl Pts',(10.1897940042106,15.2,-4.13675326204176));
#182336=CARTESIAN_POINT('Ctrl Pts',(10.1938812294348,15.2,-4.13690095054918));
#182337=CARTESIAN_POINT('Ctrl Pts',(10.1979684541022,15.2,-4.13704863903648));
#182338=CARTESIAN_POINT('Ctrl Pts',(10.2020700567427,15.2,-4.13719018051871));
#182339=CARTESIAN_POINT('Ctrl Pts',(10.2061859419804,15.2,-4.13732549300828));
#182340=CARTESIAN_POINT('Ctrl Pts',(10.2103018277789,15.2,-4.13746080551629));
#182341=CARTESIAN_POINT('Ctrl Pts',(10.2144319947196,15.2,-4.13758988923906));
#182342=CARTESIAN_POINT('Ctrl Pts',(10.2185763486692,15.2,-4.13771266307844));
#182343=CARTESIAN_POINT('Ctrl Pts',(10.2237567908237,15.2,-4.13786613036931));
#182344=CARTESIAN_POINT('Ctrl Pts',(10.2289593988759,15.2,-4.13800973915722));
#182345=CARTESIAN_POINT('Ctrl Pts',(10.2341839892249,15.2,-4.13814333380918));
#182346=CARTESIAN_POINT('Ctrl Pts',(10.2383636611625,15.2,-4.138250209522));
#182347=CARTESIAN_POINT('Ctrl Pts',(10.2425574013331,15.2,-4.13835067442943));
#182348=CARTESIAN_POINT('Ctrl Pts',(10.2467651142304,15.2,-4.13844465353331));
#182349=CARTESIAN_POINT('Ctrl Pts',(10.250972827701,15.2,-4.13853863264999));
#182350=CARTESIAN_POINT('Ctrl Pts',(10.2551945171602,15.2,-4.13862612362064));
#182351=CARTESIAN_POINT('Ctrl Pts',(10.2594300857257,15.2,-4.13870704951327));
#182352=CARTESIAN_POINT('Ctrl Pts',(10.2647245461442,15.2,-4.13880820687354));
#182353=CARTESIAN_POINT('Ctrl Pts',(10.2700406943019,15.2,-4.13889910621697));
#182354=CARTESIAN_POINT('Ctrl Pts',(10.2753783489564,15.2,-4.1389795977439));
#182355=CARTESIAN_POINT('Ctrl Pts',(10.2796484723309,15.2,-4.13904399096018));
#182356=CARTESIAN_POINT('Ctrl Pts',(10.2839323598455,15.2,-4.13910172344558));
#182357=CARTESIAN_POINT('Ctrl Pts',(10.2882299191803,15.2,-4.13915271994167));
#182358=CARTESIAN_POINT('Ctrl Pts',(10.2925274791007,15.2,-4.13920371644471));
#182359=CARTESIAN_POINT('Ctrl Pts',(10.2968387104699,15.2,-4.13924797572704));
#182360=CARTESIAN_POINT('Ctrl Pts',(10.301163521707,15.2,-4.13928542550616));
#182361=CARTESIAN_POINT('Ctrl Pts',(10.3065695354587,15.2,-4.13933223772751));
#182362=CARTESIAN_POINT('Ctrl Pts',(10.3119967670497,15.2,-4.13936840649868));
#182363=CARTESIAN_POINT('Ctrl Pts',(10.3174450392042,15.2,-4.13939379122003));
#182364=CARTESIAN_POINT('Ctrl Pts',(10.3218036565715,15.2,-4.13941409899544));
#182365=CARTESIAN_POINT('Ctrl Pts',(10.3261757398855,15.2,-4.13942750317551));
#182366=CARTESIAN_POINT('Ctrl Pts',(10.3305611985469,15.2,-4.13943393300837));
#182367=CARTESIAN_POINT('Ctrl Pts',(10.3349466578058,15.2,-4.13944036284211));
#182368=CARTESIAN_POINT('Ctrl Pts',(10.3393454911545,15.2,-4.13943981621382));
#182369=CARTESIAN_POINT('Ctrl Pts',(10.3437576092296,15.2,-4.13943222349046));
#182370=CARTESIAN_POINT('Ctrl Pts',(10.349272756523,15.2,-4.13942273258679));
#182371=CARTESIAN_POINT('Ctrl Pts',(10.3548086625028,15.2,-4.13940223181903));
#182372=CARTESIAN_POINT('Ctrl Pts',(10.3603651497267,15.2,-4.1393705802209));
#182373=CARTESIAN_POINT('Ctrl Pts',(10.3636990419399,15.2,-4.13935158926271));
#182374=CARTESIAN_POINT('Ctrl Pts',(10.367040344268,15.2,-4.13932858562894));
#182375=CARTESIAN_POINT('Ctrl Pts',(10.3703890186062,15.2,-4.1393015390031));
#182376=CARTESIAN_POINT('Ctrl Pts',(10.3737376929443,15.2,-4.13927449237727));
#182377=CARTESIAN_POINT('Ctrl Pts',(10.3770937386549,15.2,-4.13924340157855));
#182378=CARTESIAN_POINT('Ctrl Pts',(10.3804571188666,15.2,-4.13920823903781));
#182379=CARTESIAN_POINT('Ctrl Pts',(10.3838204990784,15.2,-4.13917307649707));
#182380=CARTESIAN_POINT('Ctrl Pts',(10.387191214806,15.2,-4.13913384194847));
#182381=CARTESIAN_POINT('Ctrl Pts',(10.3905692270166,15.2,-4.13909050549171));
#182382=CARTESIAN_POINT('Ctrl Pts',(10.3939472392272,15.2,-4.13904716903495));
#182383=CARTESIAN_POINT('Ctrl Pts',(10.3973325487375,15.2,-4.13899973178669));
#182384=CARTESIAN_POINT('Ctrl Pts',(10.4007251184052,15.2,-4.13894816474726));
#182385=CARTESIAN_POINT('Ctrl Pts',(10.404117688073,15.2,-4.13889659770783));
#182386=CARTESIAN_POINT('Ctrl Pts',(10.4075175174619,15.2,-4.13884090054525));
#182387=CARTESIAN_POINT('Ctrl Pts',(10.4109245698825,15.2,-4.13878104500325));
#182388=CARTESIAN_POINT('Ctrl Pts',(10.414331622303,15.2,-4.13872118946125));
#182389=CARTESIAN_POINT('Ctrl Pts',(10.417745898246,15.2,-4.13865717557852));
#182390=CARTESIAN_POINT('Ctrl Pts',(10.4211673599957,15.2,-4.13858897503991));
#182391=CARTESIAN_POINT('Ctrl Pts',(10.424588822367,15.2,-4.1385207744889));
#182392=CARTESIAN_POINT('Ctrl Pts',(10.4280174708653,15.2,-4.13844838649505));
#182393=CARTESIAN_POINT('Ctrl Pts',(10.4314532686989,15.2,-4.13837178494167));
#182394=CARTESIAN_POINT('Ctrl Pts',(10.4348890659084,15.2,-4.13829518340222));
#182395=CARTESIAN_POINT('Ctrl Pts',(10.4383320128675,15.2,-4.13821436748798));
#182396=CARTESIAN_POINT('Ctrl Pts',(10.4417820716594,15.2,-4.1381293089907));
#182397=CARTESIAN_POINT('Ctrl Pts',(10.4452321304513,15.2,-4.13804425049342));
#182398=CARTESIAN_POINT('Ctrl Pts',(10.4486893029798,15.2,-4.137954949397));
#182399=CARTESIAN_POINT('Ctrl Pts',(10.452153551703,15.2,-4.13786137894162));
#182400=CARTESIAN_POINT('Ctrl Pts',(10.4556178004263,15.2,-4.13776780848625));
#182401=CARTESIAN_POINT('Ctrl Pts',(10.459089125224,15.2,-4.13766996939687));
#182402=CARTESIAN_POINT('Ctrl Pts',(10.4625674894884,15.2,-4.13756783198347));
#182403=CARTESIAN_POINT('Ctrl Pts',(10.4660458537528,15.2,-4.13746569457007));
#182404=CARTESIAN_POINT('Ctrl Pts',(10.4695312591635,15.2,-4.13735926119098));
#182405=CARTESIAN_POINT('Ctrl Pts',(10.4730236678693,15.2,-4.13724850327871));
#182406=CARTESIAN_POINT('Ctrl Pts',(10.4765160765752,15.2,-4.13713774536645));
#182407=CARTESIAN_POINT('Ctrl Pts',(10.4800154887472,15.2,-4.13702266442115));
#182408=CARTESIAN_POINT('Ctrl Pts',(10.4835218684938,15.2,-4.13690323200941));
#182409=CARTESIAN_POINT('Ctrl Pts',(10.4870282488775,15.2,-4.13678379957598));
#182410=CARTESIAN_POINT('Ctrl Pts',(10.4905415976714,15.2,-4.13666001699133));
#182411=CARTESIAN_POINT('Ctrl Pts',(10.4940618780173,15.2,-4.1365318574721));
#182412=CARTESIAN_POINT('Ctrl Pts',(10.4975821577237,15.2,-4.13640369797616));
#182413=CARTESIAN_POINT('Ctrl Pts',(10.5011093687848,15.2,-4.13627116164255));
#182414=CARTESIAN_POINT('Ctrl Pts',(10.5046434761671,15.2,-4.13613422076518));
#182415=CARTESIAN_POINT('Ctrl Pts',(10.5081775835493,15.2,-4.1359972798878));
#182416=CARTESIAN_POINT('Ctrl Pts',(10.511718587265,15.2,-4.13585593691251));
#182417=CARTESIAN_POINT('Ctrl Pts',(10.5152664514284,15.2,-4.13571016350075));
#182418=CARTESIAN_POINT('Ctrl Pts',(10.5188143155918,15.2,-4.13556439008899));
#182419=CARTESIAN_POINT('Ctrl Pts',(10.5223690392626,15.2,-4.13541418699443));
#182420=CARTESIAN_POINT('Ctrl Pts',(10.5259305885082,15.2,-4.13525952950005));
#182421=CARTESIAN_POINT('Ctrl Pts',(10.5294921377538,15.2,-4.13510487200567));
#182422=CARTESIAN_POINT('Ctrl Pts',(10.5330605122741,15.2,-4.13494575972813));
#182423=CARTESIAN_POINT('Ctrl Pts',(10.5366356755603,15.2,-4.1347821658178));
#182424=CARTESIAN_POINT('Ctrl Pts',(10.5402108388465,15.2,-4.13461857190747));
#182425=CARTESIAN_POINT('Ctrl Pts',(10.5437927921822,15.2,-4.13445049748077));
#182426=CARTESIAN_POINT('Ctrl Pts',(10.5473814989676,15.2,-4.13427791702933));
#182427=CARTESIAN_POINT('Ctrl Pts',(10.5509702064049,15.2,-4.13410533654653));
#182428=CARTESIAN_POINT('Ctrl Pts',(10.5545656688607,15.2,-4.13392824993746));
#182429=CARTESIAN_POINT('Ctrl Pts',(10.5581678497602,15.2,-4.13374663149378));
#182430=CARTESIAN_POINT('Ctrl Pts',(10.5617700300052,15.2,-4.1335650130831));
#182431=CARTESIAN_POINT('Ctrl Pts',(10.5653789295994,15.2,-4.1333788633829));
#182432=CARTESIAN_POINT('Ctrl Pts',(10.5689945134828,15.2,-4.13318815792144));
#182433=CARTESIAN_POINT('Ctrl Pts',(10.5726100973662,15.2,-4.13299745245998));
#182434=CARTESIAN_POINT('Ctrl Pts',(10.5762323649268,15.2,-4.13280219065466));
#182435=CARTESIAN_POINT('Ctrl Pts',(10.5798612816289,15.2,-4.13260234770319));
#182436=CARTESIAN_POINT('Ctrl Pts',(10.5834901983309,15.2,-4.13240250475172));
#182437=CARTESIAN_POINT('Ctrl Pts',(10.5871257633322,15.2,-4.13219808145912));
#182438=CARTESIAN_POINT('Ctrl Pts',(10.5907679434916,15.2,-4.13198905205005));
#182439=CARTESIAN_POINT('Ctrl Pts',(10.5956241841451,15.2,-4.13171034614597));
#182440=CARTESIAN_POINT('Ctrl Pts',(10.6004921836028,15.2,-4.13142345292149));
#182441=CARTESIAN_POINT('Ctrl Pts',(10.6053718603144,15.2,-4.13112831496012));
#182442=CARTESIAN_POINT('Ctrl Pts',(10.6090316175157,15.2,-4.1309069615092));
#182443=CARTESIAN_POINT('Ctrl Pts',(10.6126979423598,15.2,-4.13068097014239));
#182444=CARTESIAN_POINT('Ctrl Pts',(10.6163708017022,15.2,-4.13045031718038));
#182445=CARTESIAN_POINT('Ctrl Pts',(10.6200436610447,15.2,-4.13021966421836));
#182446=CARTESIAN_POINT('Ctrl Pts',(10.6237230529518,15.2,-4.12998434908217));
#182447=CARTESIAN_POINT('Ctrl Pts',(10.6274089446518,15.2,-4.12974434821548));
#182448=CARTESIAN_POINT('Ctrl Pts',(10.6310948363517,15.2,-4.12950434734879));
#182449=CARTESIAN_POINT('Ctrl Pts',(10.634787226951,15.2,-4.12925966237432));
#182450=CARTESIAN_POINT('Ctrl Pts',(10.6384860827332,15.2,-4.12901026700838));
#182451=CARTESIAN_POINT('Ctrl Pts',(10.6446508425944,15.2,-4.12859460805005));
#182452=CARTESIAN_POINT('Ctrl Pts',(10.6508335643418,15.2,-4.12816586986851));
#182453=CARTESIAN_POINT('Ctrl Pts',(10.6570340849949,15.2,-4.12772394174147));
#182454=CARTESIAN_POINT('Ctrl Pts',(10.6607543972517,15.2,-4.12745878487488));
#182455=CARTESIAN_POINT('Ctrl Pts',(10.6644811174486,15.2,-4.12718888029154));
#182456=CARTESIAN_POINT('Ctrl Pts',(10.6682142102465,15.2,-4.12691420296696));
#182457=CARTESIAN_POINT('Ctrl Pts',(10.6731916677626,15.2,-4.12654796650093));
#182458=CARTESIAN_POINT('Ctrl Pts',(10.6781804540799,15.2,-4.12617324751469));
#182459=CARTESIAN_POINT('Ctrl Pts',(10.6831804980757,15.2,-4.12578999493738));
#182460=CARTESIAN_POINT('Ctrl Pts',(10.686930530732,15.2,-4.12550255553051));
#182461=CARTESIAN_POINT('Ctrl Pts',(10.6906868948296,15.2,-4.12521031650721));
#182462=CARTESIAN_POINT('Ctrl Pts',(10.6944495569018,15.2,-4.12491325497592));
#182463=CARTESIAN_POINT('Ctrl Pts',(10.698212218974,15.2,-4.12461619344463));
#182464=CARTESIAN_POINT('Ctrl Pts',(10.70198117734,15.2,-4.12431430827337));
#182465=CARTESIAN_POINT('Ctrl Pts',(10.7057563905117,15.2,-4.1240075722831));
#182466=CARTESIAN_POINT('Ctrl Pts',(10.7095316036833,15.2,-4.12370083629283));
#182467=CARTESIAN_POINT('Ctrl Pts',(10.7133130716002,15.2,-4.12338924764025));
#182468=CARTESIAN_POINT('Ctrl Pts',(10.7171007630631,15.2,-4.12307278748367));
#182469=CARTESIAN_POINT('Ctrl Pts',(10.7234135823973,15.2,-4.1225453538702));
#182470=CARTESIAN_POINT('Ctrl Pts',(10.7297436872271,15.2,-4.12200439248384));
#182471=CARTESIAN_POINT('Ctrl Pts',(10.7360910470075,15.2,-4.12144986808671));
#182472=CARTESIAN_POINT('Ctrl Pts',(9.55499537099995,12.2,-4.04260911600002));
#182473=CARTESIAN_POINT('Ctrl Pts',(9.55669454752162,12.2,-4.04316130584455));
#182474=CARTESIAN_POINT('Ctrl Pts',(9.55844976514545,12.2,-4.04372605389323));
#182475=CARTESIAN_POINT('Ctrl Pts',(9.5602602775349,12.2,-4.04430244593687));
#182476=CARTESIAN_POINT('Ctrl Pts',(9.56207952113026,12.2,-4.0448816176343));
#182477=CARTESIAN_POINT('Ctrl Pts',(9.56395460122355,12.2,-4.04547254558642));
#182478=CARTESIAN_POINT('Ctrl Pts',(9.56588480617837,12.2,-4.04607433356657));
#182479=CARTESIAN_POINT('Ctrl Pts',(9.56781501095787,12.2,-4.04667612149206));
#182480=CARTESIAN_POINT('Ctrl Pts',(9.56980034124062,12.2,-4.04728876912262));
#182481=CARTESIAN_POINT('Ctrl Pts',(9.57184010199984,12.2,-4.04791140626666));
#182482=CARTESIAN_POINT('Ctrl Pts',(9.57387986275907,12.2,-4.04853404341071));
#182483=CARTESIAN_POINT('Ctrl Pts',(9.57597405360772,12.2,-4.04916667193806));
#182484=CARTESIAN_POINT('Ctrl Pts',(9.57812199955053,12.2,-4.04980844719627));
#182485=CARTESIAN_POINT('Ctrl Pts',(9.58026994568846,12.2,-4.05045022251278));
#182486=CARTESIAN_POINT('Ctrl Pts',(9.5824716464358,12.2,-4.0511011466437));
#182487=CARTESIAN_POINT('Ctrl Pts',(9.58472643972897,12.2,-4.05176039909686));
#182488=CARTESIAN_POINT('Ctrl Pts',(9.58698123281733,12.2,-4.05241965149014));
#182489=CARTESIAN_POINT('Ctrl Pts',(9.58928912248419,12.2,-4.05308723447175));
#182490=CARTESIAN_POINT('Ctrl Pts',(9.5916494594926,12.2,-4.05376235378364));
#182491=CARTESIAN_POINT('Ctrl Pts',(9.59400979650101,12.2,-4.05443747309554));
#182492=CARTESIAN_POINT('Ctrl Pts',(9.59642258389921,12.2,-4.0551201289628));
#182493=CARTESIAN_POINT('Ctrl Pts',(9.59888719089075,12.2,-4.05580954952079));
#182494=CARTESIAN_POINT('Ctrl Pts',(9.60135179810616,12.2,-4.0564989701414));
#182495=CARTESIAN_POINT('Ctrl Pts',(9.60386822553632,12.2,-4.05719515745453));
#182496=CARTESIAN_POINT('Ctrl Pts',(9.60643585601307,12.2,-4.05789736282655));
#182497=CARTESIAN_POINT('Ctrl Pts',(9.6090034862566,12.2,-4.05859956813477));
#182498=CARTESIAN_POINT('Ctrl Pts',(9.61162232317368,12.2,-4.05930778903961));
#182499=CARTESIAN_POINT('Ctrl Pts',(9.61429176141222,12.2,-4.06002130076391));
#182500=CARTESIAN_POINT('Ctrl Pts',(9.61696119965077,12.2,-4.06073481248822));
#182501=CARTESIAN_POINT('Ctrl Pts',(9.61968124046026,12.2,-4.06145361577042));
#182502=CARTESIAN_POINT('Ctrl Pts',(9.62245129460743,12.2,-4.06217699974393));
#182503=CARTESIAN_POINT('Ctrl Pts',(9.6252213487546,12.2,-4.06290038371745));
#182504=CARTESIAN_POINT('Ctrl Pts',(9.62804141715304,12.2,-4.06362835221376));
#182505=CARTESIAN_POINT('Ctrl Pts',(9.63091092146209,12.2,-4.0643602141869));
#182506=CARTESIAN_POINT('Ctrl Pts',(9.63378042603179,12.2,-4.06509207622652));
#182507=CARTESIAN_POINT('Ctrl Pts',(9.63669936976461,12.2,-4.06582783364988));
#182508=CARTESIAN_POINT('Ctrl Pts',(9.63966718442848,12.2,-4.06656681652363));
#182509=CARTESIAN_POINT('Ctrl Pts',(9.64263499882278,12.2,-4.06730579933026));
#182510=CARTESIAN_POINT('Ctrl Pts',(9.64565168593768,12.2,-4.06804800581502));
#182511=CARTESIAN_POINT('Ctrl Pts',(9.6487166922568,12.2,-4.068792787708));
#182512=CARTESIAN_POINT('Ctrl Pts',(9.65178169857594,12.2,-4.06953756960099));
#182513=CARTESIAN_POINT('Ctrl Pts',(9.65489502329009,12.2,-4.07028492392903));
#182514=CARTESIAN_POINT('Ctrl Pts',(9.65805612383864,12.2,-4.07103421890167));
#182515=CARTESIAN_POINT('Ctrl Pts',(9.66121722467433,12.2,-4.07178351394237));
#182516=CARTESIAN_POINT('Ctrl Pts',(9.66442610292301,12.2,-4.07253474644996));
#182517=CARTESIAN_POINT('Ctrl Pts',(9.66768222468585,12.2,-4.07328730149103));
#182518=CARTESIAN_POINT('Ctrl Pts',(9.67093834615294,12.2,-4.07403985646375));
#182519=CARTESIAN_POINT('Ctrl Pts',(9.67424171158829,12.2,-4.07479373162366));
#182520=CARTESIAN_POINT('Ctrl Pts',(9.67759179898168,12.2,-4.07554832576634));
#182521=CARTESIAN_POINT('Ctrl Pts',(9.68094188637507,12.2,-4.07630291990902));
#182522=CARTESIAN_POINT('Ctrl Pts',(9.68433869487785,12.2,-4.07705823111179));
#182523=CARTESIAN_POINT('Ctrl Pts',(9.68778171333292,12.2,-4.07781367441767));
#182524=CARTESIAN_POINT('Ctrl Pts',(9.69122473210076,12.2,-4.07856911779217));
#182525=CARTESIAN_POINT('Ctrl Pts',(9.69471395864503,12.2,-4.07932469331921));
#182526=CARTESIAN_POINT('Ctrl Pts',(9.69824889160027,12.2,-4.08007982581473));
#182527=CARTESIAN_POINT('Ctrl Pts',(9.70178382423443,12.2,-4.08083495824166));
#182528=CARTESIAN_POINT('Ctrl Pts',(9.70536446092327,12.2,-4.08158965017741));
#182529=CARTESIAN_POINT('Ctrl Pts',(9.70899030854153,12.2,-4.08234334148335));
#182530=CARTESIAN_POINT('Ctrl Pts',(9.7126161561598,12.2,-4.0830970327893));
#182531=CARTESIAN_POINT('Ctrl Pts',(9.71628721518416,12.2,-4.08384972393369));
#182532=CARTESIAN_POINT('Ctrl Pts',(9.72000299714885,12.2,-4.08460086944402));
#182533=CARTESIAN_POINT('Ctrl Pts',(9.72371877945107,12.2,-4.08535201502257));
#182534=CARTESIAN_POINT('Ctrl Pts',(9.72747928619589,12.2,-4.08610161413256));
#182535=CARTESIAN_POINT('Ctrl Pts',(9.73128403915626,12.2,-4.08684913758983));
#182536=CARTESIAN_POINT('Ctrl Pts',(9.73508879177105,12.2,-4.0875966609792));
#182537=CARTESIAN_POINT('Ctrl Pts',(9.73893778845863,12.2,-4.08834210619898));
#182538=CARTESIAN_POINT('Ctrl Pts',(9.74283056200164,12.2,-4.08908495475869));
#182539=CARTESIAN_POINT('Ctrl Pts',(9.74672333554465,12.2,-4.0898278033184));
#182540=CARTESIAN_POINT('Ctrl Pts',(9.75065988382131,12.2,-4.09056805421981));
#182541=CARTESIAN_POINT('Ctrl Pts',(9.75463974375815,12.2,-4.09130520269317));
#182542=CARTESIAN_POINT('Ctrl Pts',(9.75795629382602,12.2,-4.09191949310994));
#182543=CARTESIAN_POINT('Ctrl Pts',(9.76130292313634,12.2,-4.09253162599334));
#182544=CARTESIAN_POINT('Ctrl Pts',(9.76467936632923,12.2,-4.0931413174518));
#182545=CARTESIAN_POINT('Ctrl Pts',(9.76805580952212,12.2,-4.09375100891026));
#182546=CARTESIAN_POINT('Ctrl Pts',(9.77146206698804,12.2,-4.0943582577525));
#182547=CARTESIAN_POINT('Ctrl Pts',(9.77489787623967,12.2,-4.09496278094969));
#182548=CARTESIAN_POINT('Ctrl Pts',(9.77833368549131,12.2,-4.09556730414689));
#182549=CARTESIAN_POINT('Ctrl Pts',(9.78179904861098,12.2,-4.09616910386669));
#182550=CARTESIAN_POINT('Ctrl Pts',(9.78529370854153,12.2,-4.09676790199169));
#182551=CARTESIAN_POINT('Ctrl Pts',(9.78878836847207,12.2,-4.09736670011669));
#182552=CARTESIAN_POINT('Ctrl Pts',(9.79231232290782,12.2,-4.0979624962421));
#182553=CARTESIAN_POINT('Ctrl Pts',(9.79586532028515,12.2,-4.09855502096701));
#182554=CARTESIAN_POINT('Ctrl Pts',(9.79941831766247,12.2,-4.09914754569192));
#182555=CARTESIAN_POINT('Ctrl Pts',(9.80300035684025,12.2,-4.0997367967496));
#182556=CARTESIAN_POINT('Ctrl Pts',(9.80661118607787,12.2,-4.10032251001331));
#182557=CARTESIAN_POINT('Ctrl Pts',(9.8102220153155,12.2,-4.10090822327702));
#182558=CARTESIAN_POINT('Ctrl Pts',(9.8138616359329,12.2,-4.10149039863802));
#182559=CARTESIAN_POINT('Ctrl Pts',(9.81752979773994,12.2,-4.10206877280449));
#182560=CARTESIAN_POINT('Ctrl Pts',(9.82119795954699,12.2,-4.10264714697096));
#182561=CARTESIAN_POINT('Ctrl Pts',(9.82489466542211,12.2,-4.10322172219358));
#182562=CARTESIAN_POINT('Ctrl Pts',(9.82861966741573,12.2,-4.10379223979124));
#182563=CARTESIAN_POINT('Ctrl Pts',(9.83234466940933,12.2,-4.1043627573889));
#182564=CARTESIAN_POINT('Ctrl Pts',(9.83609796945329,12.2,-4.10492921825724));
#182565=CARTESIAN_POINT('Ctrl Pts',(9.83987932376116,12.2,-4.10549137159022));
#182566=CARTESIAN_POINT('Ctrl Pts',(9.84366067806901,12.2,-4.1060535249232));
#182567=CARTESIAN_POINT('Ctrl Pts',(9.84747008751064,12.2,-4.10661136957832));
#182568=CARTESIAN_POINT('Ctrl Pts',(9.85130731327679,12.2,-4.10716465881406));
#182569=CARTESIAN_POINT('Ctrl Pts',(9.8551445386247,12.2,-4.1077179479895));
#182570=CARTESIAN_POINT('Ctrl Pts',(9.85900957790061,12.2,-4.10826668100445));
#182571=CARTESIAN_POINT('Ctrl Pts',(9.86290219601573,12.2,-4.10881061594555));
#182572=CARTESIAN_POINT('Ctrl Pts',(9.86679481455514,12.2,-4.10935455094594));
#182573=CARTESIAN_POINT('Ctrl Pts',(9.87071501224689,12.2,-4.1098936868242));
#182574=CARTESIAN_POINT('Ctrl Pts',(9.87466255321688,12.2,-4.11042778613017));
#182575=CARTESIAN_POINT('Ctrl Pts',(9.87861009418686,12.2,-4.11096188543613));
#182576=CARTESIAN_POINT('Ctrl Pts',(9.88258497911197,12.2,-4.11149094733663));
#182577=CARTESIAN_POINT('Ctrl Pts',(9.88658697744309,12.2,-4.11201473823985));
#182578=CARTESIAN_POINT('Ctrl Pts',(9.8905889757742,12.2,-4.11253852914305));
#182579=CARTESIAN_POINT('Ctrl Pts',(9.89461808436726,12.2,-4.11305704849222));
#182580=CARTESIAN_POINT('Ctrl Pts',(9.8986740779708,12.2,-4.11357006615712));
#182581=CARTESIAN_POINT('Ctrl Pts',(9.90273007157434,12.2,-4.11408308382203));
#182582=CARTESIAN_POINT('Ctrl Pts',(9.90681294834378,12.2,-4.11459059951687));
#182583=CARTESIAN_POINT('Ctrl Pts',(9.91092248098127,12.2,-4.11509238722551));
#182584=CARTESIAN_POINT('Ctrl Pts',(9.91503201361877,12.2,-4.11559417493415));
#182585=CARTESIAN_POINT('Ctrl Pts',(9.9191682006014,12.2,-4.11609023581762));
#182586=CARTESIAN_POINT('Ctrl Pts',(9.9233308215028,12.2,-4.11658034519294));
#182587=CARTESIAN_POINT('Ctrl Pts',(9.92749344240421,12.2,-4.11707045456826));
#182588=CARTESIAN_POINT('Ctrl Pts',(9.93168249413961,12.2,-4.11755461470314));
#182589=CARTESIAN_POINT('Ctrl Pts',(9.93589775450592,12.2,-4.1180326049831));
#182590=CARTESIAN_POINT('Ctrl Pts',(9.93926996298274,12.2,-4.11841499722791));
#182591=CARTESIAN_POINT('Ctrl Pts',(9.9426589475333,12.2,-4.11879344171625));
#182592=CARTESIAN_POINT('Ctrl Pts',(9.94606459133171,12.2,-4.11916782856957));
#182593=CARTESIAN_POINT('Ctrl Pts',(9.94947023466611,12.2,-4.11954221537189));
#182594=CARTESIAN_POINT('Ctrl Pts',(9.95289254044834,12.2,-4.1199125437636));
#182595=CARTESIAN_POINT('Ctrl Pts',(9.95633139444391,12.2,-4.12027870467839));
#182596=CARTESIAN_POINT('Ctrl Pts',(9.95977024890802,12.2,-4.12064486564307));
#182597=CARTESIAN_POINT('Ctrl Pts',(9.96322565282856,12.2,-4.12100686132881));
#182598=CARTESIAN_POINT('Ctrl Pts',(9.96669749597043,12.2,-4.12136458231025));
#182599=CARTESIAN_POINT('Ctrl Pts',(9.97016933863925,12.2,-4.12172230324295));
#182600=CARTESIAN_POINT('Ctrl Pts',(9.9736576194761,12.2,-4.12207575038304));
#182601=CARTESIAN_POINT('Ctrl Pts',(9.97716222802187,12.2,-4.12242481668812));
#182602=CARTESIAN_POINT('Ctrl Pts',(9.98066683704513,12.2,-4.12277388304076));
#182603=CARTESIAN_POINT('Ctrl Pts',(9.98418777475925,12.2,-4.12311857191233));
#182604=CARTESIAN_POINT('Ctrl Pts',(9.98772493056419,12.2,-4.12345877431947));
#182605=CARTESIAN_POINT('Ctrl Pts',(9.9912620858872,12.2,-4.12379897668025));
#182606=CARTESIAN_POINT('Ctrl Pts',(9.99481546091078,12.2,-4.12413469573986));
#182607=CARTESIAN_POINT('Ctrl Pts',(9.99838494574035,12.2,-4.12446582795196));
#182608=CARTESIAN_POINT('Ctrl Pts',(10.0019544310563,12.2,-4.12479696020917));
#182609=CARTESIAN_POINT('Ctrl Pts',(10.0055400271249,12.2,-4.12512350483684));
#182610=CARTESIAN_POINT('Ctrl Pts',(10.0091416255445,12.2,-4.1254453610763));
#182611=CARTESIAN_POINT('Ctrl Pts',(10.0127432234733,12.2,-4.12576721727191));
#182612=CARTESIAN_POINT('Ctrl Pts',(10.0163608241128,12.2,-4.12608438442401));
#182613=CARTESIAN_POINT('Ctrl Pts',(10.0199943206475,12.2,-4.12639676273229));
#182614=CARTESIAN_POINT('Ctrl Pts',(10.0236278176772,12.2,-4.12670914108314));
#182615=CARTESIAN_POINT('Ctrl Pts',(10.0272772097665,12.2,-4.12701673166849));
#182616=CARTESIAN_POINT('Ctrl Pts',(10.0309423922607,12.2,-4.12731943274191));
#182617=CARTESIAN_POINT('Ctrl Pts',(10.0346075742556,12.2,-4.12762213377407));
#182618=CARTESIAN_POINT('Ctrl Pts',(10.038288546316,12.2,-4.12791994720614));
#182619=CARTESIAN_POINT('Ctrl Pts',(10.0419852016788,12.2,-4.12821277546049));
#182620=CARTESIAN_POINT('Ctrl Pts',(10.0456818575453,12.2,-4.12850560375473));
#182621=CARTESIAN_POINT('Ctrl Pts',(10.0493941990912,12.2,-4.1287934465374));
#182622=CARTESIAN_POINT('Ctrl Pts',(10.0531221195165,12.2,-4.1290762069417));
#182623=CARTESIAN_POINT('Ctrl Pts',(10.0568500399419,12.2,-4.129358967346));
#182624=CARTESIAN_POINT('Ctrl Pts',(10.060593539783,12.2,-4.12963664588026));
#182625=CARTESIAN_POINT('Ctrl Pts',(10.0643525161561,12.2,-4.12990914756125));
#182626=CARTESIAN_POINT('Ctrl Pts',(10.0681114920171,12.2,-4.13018164920511));
#182627=CARTESIAN_POINT('Ctrl Pts',(10.0718859430372,12.2,-4.13044897388674));
#182628=CARTESIAN_POINT('Ctrl Pts',(10.0756757670223,12.2,-4.13071102753319));
#182629=CARTESIAN_POINT('Ctrl Pts',(10.0794655915238,12.2,-4.13097308121535));
#182630=CARTESIAN_POINT('Ctrl Pts',(10.0832707885925,12.2,-4.13122986304465));
#182631=CARTESIAN_POINT('Ctrl Pts',(10.0870912563579,12.2,-4.13148128205781));
#182632=CARTESIAN_POINT('Ctrl Pts',(10.0909117236027,12.2,-4.13173270103671));
#182633=CARTESIAN_POINT('Ctrl Pts',(10.094747460351,12.2,-4.13197875561629));
#182634=CARTESIAN_POINT('Ctrl Pts',(10.0985983657019,12.2,-4.13221935526365));
#182635=CARTESIAN_POINT('Ctrl Pts',(10.103411997784,12.2,-4.13252010484743));
#182636=CARTESIAN_POINT('Ctrl Pts',(10.1082493314363,12.2,-4.13281233050412));
#182637=CARTESIAN_POINT('Ctrl Pts',(10.1131101684722,12.2,-4.13309585599155));
#182638=CARTESIAN_POINT('Ctrl Pts',(10.1169988383129,12.2,-4.13332267639385));
#182639=CARTESIAN_POINT('Ctrl Pts',(10.1209025498061,12.2,-4.13354392809078));
#182640=CARTESIAN_POINT('Ctrl Pts',(10.1248212036323,12.2,-4.13375952376862));
#182641=CARTESIAN_POINT('Ctrl Pts',(10.1287398569245,12.2,-4.13397511941709));
#182642=CARTESIAN_POINT('Ctrl Pts',(10.1326734528343,12.2,-4.13418505804406));
#182643=CARTESIAN_POINT('Ctrl Pts',(10.1366218901772,12.2,-4.13438925124996));
#182644=CARTESIAN_POINT('Ctrl Pts',(10.1405703280581,12.2,-4.13459344448368));
#182645=CARTESIAN_POINT('Ctrl Pts',(10.1445336093409,12.2,-4.13479189414723));
#182646=CARTESIAN_POINT('Ctrl Pts',(10.1485116340355,12.2,-4.13498451127796));
#182647=CARTESIAN_POINT('Ctrl Pts',(10.1524896581881,12.2,-4.13517712838243));
#182648=CARTESIAN_POINT('Ctrl Pts',(10.1564824255565,12.2,-4.13536391397459));
#182649=CARTESIAN_POINT('Ctrl Pts',(10.1604898376724,12.2,-4.1355447824602));
#182650=CARTESIAN_POINT('Ctrl Pts',(10.1654991032268,12.2,-4.13577086808568));
#182651=CARTESIAN_POINT('Ctrl Pts',(10.1705312521651,12.2,-4.13598770798037));
#182652=CARTESIAN_POINT('Ctrl Pts',(10.1755860941778,12.2,-4.13619513770308));
#182653=CARTESIAN_POINT('Ctrl Pts',(10.1806409361905,12.2,-4.1364025674258));
#182654=CARTESIAN_POINT('Ctrl Pts',(10.1857184691399,12.2,-4.13660058640938));
#182655=CARTESIAN_POINT('Ctrl Pts',(10.1908185069165,12.2,-4.13678903272932));
#182656=CARTESIAN_POINT('Ctrl Pts',(10.1948985373601,12.2,-4.1369397897935));
#182657=CARTESIAN_POINT('Ctrl Pts',(10.1989929690824,12.2,-4.13708442016451));
#182658=CARTESIAN_POINT('Ctrl Pts',(10.2031017078462,12.2,-4.13722284201176));
#182659=CARTESIAN_POINT('Ctrl Pts',(10.2072104460501,12.2,-4.13736126384015));
#182660=CARTESIAN_POINT('Ctrl Pts',(10.2113334891454,12.2,-4.13749347692179));
#182661=CARTESIAN_POINT('Ctrl Pts',(10.2154707436951,12.2,-4.13761940068969));
#182662=CARTESIAN_POINT('Ctrl Pts',(10.2196079988086,12.2,-4.13774532447474));
#182663=CARTESIAN_POINT('Ctrl Pts',(10.2237594636015,12.2,-4.13786495893404));
#182664=CARTESIAN_POINT('Ctrl Pts',(10.2279250436072,12.2,-4.13797822355091));
#182665=CARTESIAN_POINT('Ctrl Pts',(10.2341734130482,12.2,-4.13814812046077));
#182666=CARTESIAN_POINT('Ctrl Pts',(10.2404535445977,12.2,-4.13830368487109));
#182667=CARTESIAN_POINT('Ctrl Pts',(10.2467651142304,12.2,-4.13844465353331));
#182668=CARTESIAN_POINT('Ctrl Pts',(10.250972827701,12.2,-4.13853863264999));
#182669=CARTESIAN_POINT('Ctrl Pts',(10.2551945171602,12.2,-4.13862612362064));
#182670=CARTESIAN_POINT('Ctrl Pts',(10.2594300857257,12.2,-4.13870704951327));
#182671=CARTESIAN_POINT('Ctrl Pts',(10.2636656537142,12.2,-4.13878797539487));
#182672=CARTESIAN_POINT('Ctrl Pts',(10.2679151012315,12.2,-4.13886233664676));
#182673=CARTESIAN_POINT('Ctrl Pts',(10.2721783371598,12.2,-4.13893005525278));
#182674=CARTESIAN_POINT('Ctrl Pts',(10.2775073825059,12.2,-4.13901470351721));
#182675=CARTESIAN_POINT('Ctrl Pts',(10.2828579695726,12.2,-4.13908897431635));
#182676=CARTESIAN_POINT('Ctrl Pts',(10.2882299191803,12.2,-4.13915271994167));
#182677=CARTESIAN_POINT('Ctrl Pts',(10.2925274791007,12.2,-4.13920371644471));
#182678=CARTESIAN_POINT('Ctrl Pts',(10.2968387104699,12.2,-4.13924797572704));
#182679=CARTESIAN_POINT('Ctrl Pts',(10.301163521707,12.2,-4.13928542550616));
#182680=CARTESIAN_POINT('Ctrl Pts',(10.3054883323548,12.2,-4.13932287528018));
#182681=CARTESIAN_POINT('Ctrl Pts',(10.3098267223898,12.2,-4.13935351428841));
#182682=CARTESIAN_POINT('Ctrl Pts',(10.3141786011443,12.2,-4.13937726773137));
#182683=CARTESIAN_POINT('Ctrl Pts',(10.3185304804917,12.2,-4.13940102117756));
#182684=CARTESIAN_POINT('Ctrl Pts',(10.3228958479601,12.2,-4.13941789142879));
#182685=CARTESIAN_POINT('Ctrl Pts',(10.3272746140854,12.2,-4.13942780398478));
#182686=CARTESIAN_POINT('Ctrl Pts',(10.331653379614,12.2,-4.13943771653941));
#182687=CARTESIAN_POINT('Ctrl Pts',(10.3360455427231,12.2,-4.1394406720634));
#182688=CARTESIAN_POINT('Ctrl Pts',(10.3404510121399,12.2,-4.13943659800864));
#182689=CARTESIAN_POINT('Ctrl Pts',(10.345957849361,12.2,-4.13943150543977));
#182690=CARTESIAN_POINT('Ctrl Pts',(10.3514854804938,12.2,-4.13941543110673));
#182691=CARTESIAN_POINT('Ctrl Pts',(10.3570337276455,12.2,-4.13938823430175));
#182692=CARTESIAN_POINT('Ctrl Pts',(10.3603626758156,12.2,-4.13937191621936));
#182693=CARTESIAN_POINT('Ctrl Pts',(10.3636990465083,12.2,-4.13935159357125));
#182694=CARTESIAN_POINT('Ctrl Pts',(10.3670428018864,12.2,-4.13932723898805));
#182695=CARTESIAN_POINT('Ctrl Pts',(10.3715011427954,12.2,-4.1392947662075));
#182696=CARTESIAN_POINT('Ctrl Pts',(10.3759726115103,12.2,-4.13925512242972));
#182697=CARTESIAN_POINT('Ctrl Pts',(10.3804571188666,12.2,-4.13920823903781));
#182698=CARTESIAN_POINT('Ctrl Pts',(10.3838204990784,12.2,-4.13917307649707));
#182699=CARTESIAN_POINT('Ctrl Pts',(10.387191214806,12.2,-4.13913384194847));
#182700=CARTESIAN_POINT('Ctrl Pts',(10.3905692270166,12.2,-4.13909050549171));
#182701=CARTESIAN_POINT('Ctrl Pts',(10.3939472392272,12.2,-4.13904716903495));
#182702=CARTESIAN_POINT('Ctrl Pts',(10.3973325487375,12.2,-4.13899973178669));
#182703=CARTESIAN_POINT('Ctrl Pts',(10.4007251184052,12.2,-4.13894816474726));
#182704=CARTESIAN_POINT('Ctrl Pts',(10.404117688073,12.2,-4.13889659770783));
#182705=CARTESIAN_POINT('Ctrl Pts',(10.4075175174619,12.2,-4.13884090054525));
#182706=CARTESIAN_POINT('Ctrl Pts',(10.4109245698825,12.2,-4.13878104500325));
#182707=CARTESIAN_POINT('Ctrl Pts',(10.4154673068559,12.2,-4.13870123760667));
#182708=CARTESIAN_POINT('Ctrl Pts',(10.4200228851903,12.2,-4.13861403773121));
#182709=CARTESIAN_POINT('Ctrl Pts',(10.4245912171068,12.2,-4.13851937772557));
#182710=CARTESIAN_POINT('Ctrl Pts',(10.4280174657329,12.2,-4.13844838272778));
#182711=CARTESIAN_POINT('Ctrl Pts',(10.4314508876582,12.2,-4.13837319186383));
#182712=CARTESIAN_POINT('Ctrl Pts',(10.4348914472832,12.2,-4.13829377778338));
#182713=CARTESIAN_POINT('Ctrl Pts',(10.4383320069082,12.2,-4.13821436370293));
#182714=CARTESIAN_POINT('Ctrl Pts',(10.4417797023996,12.2,-4.13813072507266));
#182715=CARTESIAN_POINT('Ctrl Pts',(10.4452344995651,12.2,-4.13804283549289));
#182716=CARTESIAN_POINT('Ctrl Pts',(10.4486892967306,12.2,-4.13795494591312));
#182717=CARTESIAN_POINT('Ctrl Pts',(10.4521511950657,12.2,-4.13786280395281));
#182718=CARTESIAN_POINT('Ctrl Pts',(10.4556201573621,12.2,-4.13776638478532));
#182719=CARTESIAN_POINT('Ctrl Pts',(10.4590891196586,12.2,-4.13766996561784));
#182720=CARTESIAN_POINT('Ctrl Pts',(10.4625651445681,12.2,-4.13756926605186));
#182721=CARTESIAN_POINT('Ctrl Pts',(10.4660481987323,12.2,-4.1374642615146));
#182722=CARTESIAN_POINT('Ctrl Pts',(10.4695312535292,12.2,-4.13735925695826));
#182723=CARTESIAN_POINT('Ctrl Pts',(10.4730213366697,12.2,-4.13724994624237));
#182724=CARTESIAN_POINT('Ctrl Pts',(10.4765184110123,12.2,-4.1371363031836));
#182725=CARTESIAN_POINT('Ctrl Pts',(10.4800154847195,12.2,-4.13702266014548));
#182726=CARTESIAN_POINT('Ctrl Pts',(10.4835195496597,12.2,-4.13690468398257));
#182727=CARTESIAN_POINT('Ctrl Pts',(10.487030570866,12.2,-4.13678234848664));
#182728=CARTESIAN_POINT('Ctrl Pts',(10.4905415920724,12.2,-4.1366600129907));
#182729=CARTESIAN_POINT('Ctrl Pts',(10.4940595695318,12.2,-4.13653331849578));
#182730=CARTESIAN_POINT('Ctrl Pts',(10.4975844662531,12.2,-4.13640223799993));
#182731=CARTESIAN_POINT('Ctrl Pts',(10.5022843283347,12.2,-4.1362274640134));
#182732=CARTESIAN_POINT('Ctrl Pts',(10.5069964919344,12.2,-4.13604489120647));
#182733=CARTESIAN_POINT('Ctrl Pts',(10.5117208739358,12.2,-4.13585446105618));
#182734=CARTESIAN_POINT('Ctrl Pts',(10.5152641612415,12.2,-4.13571163841102));
#182735=CARTESIAN_POINT('Ctrl Pts',(10.5188143204241,12.2,-4.13556439348963));
#182736=CARTESIAN_POINT('Ctrl Pts',(10.5223713162753,12.2,-4.13541270296697));
#182737=CARTESIAN_POINT('Ctrl Pts',(10.5259283114804,12.2,-4.13526101247188));
#182738=CARTESIAN_POINT('Ctrl Pts',(10.5294921442017,12.2,-4.13510487574368));
#182739=CARTESIAN_POINT('Ctrl Pts',(10.5330627774475,12.2,-4.13494426670747));
#182740=CARTESIAN_POINT('Ctrl Pts',(10.5366334106934,12.2,-4.13478365767124));
#182741=CARTESIAN_POINT('Ctrl Pts',(10.5402108452635,12.2,-4.13461857531055));
#182742=CARTESIAN_POINT('Ctrl Pts',(10.5437950455082,12.2,-4.13444899627505));
#182743=CARTESIAN_POINT('Ctrl Pts',(10.547379245753,12.2,-4.13427941723954));
#182744=CARTESIAN_POINT('Ctrl Pts',(10.5509702119392,12.2,-4.13410534024589));
#182745=CARTESIAN_POINT('Ctrl Pts',(10.5545679091412,12.2,-4.13392674025277));
#182746=CARTESIAN_POINT('Ctrl Pts',(10.5581656063432,12.2,-4.13374814025966));
#182747=CARTESIAN_POINT('Ctrl Pts',(10.5617700336362,12.2,-4.13356501678834));
#182748=CARTESIAN_POINT('Ctrl Pts',(10.565381157518,12.2,-4.13337734582798));
#182749=CARTESIAN_POINT('Ctrl Pts',(10.5689922813997,12.2,-4.13318967486761));
#182750=CARTESIAN_POINT('Ctrl Pts',(10.5726101010257,12.2,-4.1329974566685));
#182751=CARTESIAN_POINT('Ctrl Pts',(10.5762345812264,12.2,-4.13280066480128));
#182752=CARTESIAN_POINT('Ctrl Pts',(10.5822753817805,12.2,-4.13247267834398));
#182753=CARTESIAN_POINT('Ctrl Pts',(10.5883346833564,12.2,-4.13213199052301));
#182754=CARTESIAN_POINT('Ctrl Pts',(10.59441232648,12.2,-4.13177848649628));
#182755=CARTESIAN_POINT('Ctrl Pts',(10.598058912884,12.2,-4.13156638404942));
#182756=CARTESIAN_POINT('Ctrl Pts',(10.6017121024483,12.2,-4.13134966845126));
#182757=CARTESIAN_POINT('Ctrl Pts',(10.6053718603144,12.2,-4.13112831496012));
#182758=CARTESIAN_POINT('Ctrl Pts',(10.6090316175157,12.2,-4.13090696150919));
#182759=CARTESIAN_POINT('Ctrl Pts',(10.6126979423598,12.2,-4.13068097014239));
#182760=CARTESIAN_POINT('Ctrl Pts',(10.6163708017022,12.2,-4.13045031718038));
#182761=CARTESIAN_POINT('Ctrl Pts',(10.6200436610447,12.2,-4.13021966421836));
#182762=CARTESIAN_POINT('Ctrl Pts',(10.6237230529518,12.2,-4.12998434908217));
#182763=CARTESIAN_POINT('Ctrl Pts',(10.6274089446518,12.2,-4.12974434821548));
#182764=CARTESIAN_POINT('Ctrl Pts',(10.6310948363517,12.2,-4.12950434734879));
#182765=CARTESIAN_POINT('Ctrl Pts',(10.634787226951,12.2,-4.12925966237432));
#182766=CARTESIAN_POINT('Ctrl Pts',(10.6384860827332,12.2,-4.12901026700838));
#182767=CARTESIAN_POINT('Ctrl Pts',(10.6434178908909,12.2,-4.12867773982359));
#182768=CARTESIAN_POINT('Ctrl Pts',(10.6483611945277,12.2,-4.12833684195172));
#182769=CARTESIAN_POINT('Ctrl Pts',(10.6533159105767,12.2,-4.1279875167096));
#182770=CARTESIAN_POINT('Ctrl Pts',(10.6595093046253,12.2,-4.12755086022833));
#182771=CARTESIAN_POINT('Ctrl Pts',(10.6657205291267,12.2,-4.12710103528128));
#182772=CARTESIAN_POINT('Ctrl Pts',(10.6719494256685,12.2,-4.12663793456895));
#182773=CARTESIAN_POINT('Ctrl Pts',(10.6756867645441,12.2,-4.12636007407089));
#182774=CARTESIAN_POINT('Ctrl Pts',(10.6794304647382,12.2,-4.12607743439647));
#182775=CARTESIAN_POINT('Ctrl Pts',(10.6831804980757,12.2,-4.12578999493738));
#182776=CARTESIAN_POINT('Ctrl Pts',(10.686930530732,12.2,-4.1255025555305));
#182777=CARTESIAN_POINT('Ctrl Pts',(10.6906868948296,12.2,-4.12521031650721));
#182778=CARTESIAN_POINT('Ctrl Pts',(10.6944495569018,12.2,-4.12491325497592));
#182779=CARTESIAN_POINT('Ctrl Pts',(10.698212218974,12.2,-4.12461619344463));
#182780=CARTESIAN_POINT('Ctrl Pts',(10.70198117734,12.2,-4.12431430827338));
#182781=CARTESIAN_POINT('Ctrl Pts',(10.7057563905117,12.2,-4.1240075722831));
#182782=CARTESIAN_POINT('Ctrl Pts',(10.7095316036833,12.2,-4.12370083629283));
#182783=CARTESIAN_POINT('Ctrl Pts',(10.7133130716002,12.2,-4.12338924764025));
#182784=CARTESIAN_POINT('Ctrl Pts',(10.7171007630631,12.2,-4.12307278748367));
#182785=CARTESIAN_POINT('Ctrl Pts',(10.7234135823973,12.2,-4.1225453538702));
#182786=CARTESIAN_POINT('Ctrl Pts',(10.7297436872271,12.2,-4.12200439248384));
#182787=CARTESIAN_POINT('Ctrl Pts',(10.7360910470075,12.2,-4.12144986808672));
#182788=CARTESIAN_POINT('Ctrl Pts',(10.8675859439999,15.2,-3.76106045600002));
#182789=CARTESIAN_POINT('Ctrl Pts',(10.8675859439999,11.6,-3.76106045600002));
#182790=CARTESIAN_POINT('Ctrl Pts',(10.8670460909999,15.2,-3.76051902400001));
#182791=CARTESIAN_POINT('Ctrl Pts',(10.8670460909999,11.6,-3.76051902400001));
#182792=CARTESIAN_POINT('Ctrl Pts',(10.8659664939999,15.2,-3.75943667400001));
#182793=CARTESIAN_POINT('Ctrl Pts',(10.8659664939999,11.6,-3.75943667400001));
#182794=CARTESIAN_POINT('Ctrl Pts',(10.8643474199999,15.2,-3.75781469800001));
#182795=CARTESIAN_POINT('Ctrl Pts',(10.8643474199999,11.6,-3.75781469800002));
#182796=CARTESIAN_POINT('Ctrl Pts',(10.8621893019999,15.2,-3.75565515600002));
#182797=CARTESIAN_POINT('Ctrl Pts',(10.8621893019999,11.6,-3.75565515600002));
#182798=CARTESIAN_POINT('Ctrl Pts',(10.8594927299999,15.2,-3.75296088400002));
#182799=CARTESIAN_POINT('Ctrl Pts',(10.8594927299999,11.6,-3.75296088400002));
#182800=CARTESIAN_POINT('Ctrl Pts',(10.8567972349999,15.2,-3.75027176800002));
#182801=CARTESIAN_POINT('Ctrl Pts',(10.8567972349999,11.6,-3.75027176800002));
#182802=CARTESIAN_POINT('Ctrl Pts',(10.8541028209999,15.2,-3.74758780800001));
#182803=CARTESIAN_POINT('Ctrl Pts',(10.8541028209999,11.6,-3.74758780800002));
#182804=CARTESIAN_POINT('Ctrl Pts',(10.8514094899999,15.2,-3.74490900600001));
#182805=CARTESIAN_POINT('Ctrl Pts',(10.8514094899999,11.6,-3.74490900600001));
#182806=CARTESIAN_POINT('Ctrl Pts',(10.8487172499999,15.2,-3.74223536100001));
#182807=CARTESIAN_POINT('Ctrl Pts',(10.8487172499999,11.6,-3.74223536100002));
#182808=CARTESIAN_POINT('Ctrl Pts',(10.8460261069999,15.2,-3.73956687500002));
#182809=CARTESIAN_POINT('Ctrl Pts',(10.8460261069999,11.6,-3.73956687500002));
#182810=CARTESIAN_POINT('Ctrl Pts',(10.8433360699999,15.2,-3.73690354800001));
#182811=CARTESIAN_POINT('Ctrl Pts',(10.8433360699999,11.6,-3.73690354800001));
#182812=CARTESIAN_POINT('Ctrl Pts',(10.8406471529999,15.2,-3.73424538200001));
#182813=CARTESIAN_POINT('Ctrl Pts',(10.8406471529999,11.6,-3.73424538200001));
#182814=CARTESIAN_POINT('Ctrl Pts',(10.8379593649999,15.2,-3.73159237800001));
#182815=CARTESIAN_POINT('Ctrl Pts',(10.8379593649999,11.6,-3.73159237800001));
#182816=CARTESIAN_POINT('Ctrl Pts',(10.8352727169999,15.2,-3.72894453800001));
#182817=CARTESIAN_POINT('Ctrl Pts',(10.8352727169999,11.6,-3.72894453800001));
#182818=CARTESIAN_POINT('Ctrl Pts',(10.8325872199999,15.2,-3.72630186200002));
#182819=CARTESIAN_POINT('Ctrl Pts',(10.8325872199999,11.6,-3.72630186200002));
#182820=CARTESIAN_POINT('Ctrl Pts',(10.8299028829999,15.2,-3.72366435100002));
#182821=CARTESIAN_POINT('Ctrl Pts',(10.8299028829999,11.6,-3.72366435100002));
#182822=CARTESIAN_POINT('Ctrl Pts',(10.8272197149999,15.2,-3.72103200700002));
#182823=CARTESIAN_POINT('Ctrl Pts',(10.8272197149999,11.6,-3.72103200700002));
#182824=CARTESIAN_POINT('Ctrl Pts',(10.8245377239999,15.2,-3.71840483100002));
#182825=CARTESIAN_POINT('Ctrl Pts',(10.8245377239999,11.6,-3.71840483100002));
#182826=CARTESIAN_POINT('Ctrl Pts',(10.8218569179999,15.2,-3.71578282200002));
#182827=CARTESIAN_POINT('Ctrl Pts',(10.8218569179999,11.6,-3.71578282200002));
#182828=CARTESIAN_POINT('Ctrl Pts',(10.8191773059999,15.2,-3.71316598200002));
#182829=CARTESIAN_POINT('Ctrl Pts',(10.8191773059999,11.6,-3.71316598200002));
#182830=CARTESIAN_POINT('Ctrl Pts',(10.8164988939999,15.2,-3.71055431200002));
#182831=CARTESIAN_POINT('Ctrl Pts',(10.8164988939999,11.6,-3.71055431200002));
#182832=CARTESIAN_POINT('Ctrl Pts',(10.8138216939999,15.2,-3.70794781300001));
#182833=CARTESIAN_POINT('Ctrl Pts',(10.8138216939999,11.6,-3.70794781300001));
#182834=CARTESIAN_POINT('Ctrl Pts',(10.8111457129999,15.2,-3.70534648600001));
#182835=CARTESIAN_POINT('Ctrl Pts',(10.8111457129999,11.6,-3.70534648600001));
#182836=CARTESIAN_POINT('Ctrl Pts',(10.8084709609999,15.2,-3.70275033200001));
#182837=CARTESIAN_POINT('Ctrl Pts',(10.8084709609999,11.6,-3.70275033200001));
#182838=CARTESIAN_POINT('Ctrl Pts',(10.8057974489999,15.2,-3.70015935000001));
#182839=CARTESIAN_POINT('Ctrl Pts',(10.8057974489999,11.6,-3.70015935000001));
#182840=CARTESIAN_POINT('Ctrl Pts',(10.8031251839999,15.2,-3.69757354500001));
#182841=CARTESIAN_POINT('Ctrl Pts',(10.8031251839999,11.6,-3.69757354500001));
#182842=CARTESIAN_POINT('Ctrl Pts',(10.8004541779999,15.2,-3.69499291500002));
#182843=CARTESIAN_POINT('Ctrl Pts',(10.8004541779999,11.6,-3.69499291500002));
#182844=CARTESIAN_POINT('Ctrl Pts',(10.7977844379999,15.2,-3.69241746100001));
#182845=CARTESIAN_POINT('Ctrl Pts',(10.7977844379999,11.6,-3.69241746100002));
#182846=CARTESIAN_POINT('Ctrl Pts',(10.7951159729999,15.2,-3.68984718400001));
#182847=CARTESIAN_POINT('Ctrl Pts',(10.7951159729999,11.6,-3.68984718400002));
#182848=CARTESIAN_POINT('Ctrl Pts',(10.7924487949999,15.2,-3.68728208700002));
#182849=CARTESIAN_POINT('Ctrl Pts',(10.7924487949999,11.6,-3.68728208700002));
#182850=CARTESIAN_POINT('Ctrl Pts',(10.7897829079999,15.2,-3.68472216800001));
#182851=CARTESIAN_POINT('Ctrl Pts',(10.7897829079999,11.6,-3.68472216800001));
#182852=CARTESIAN_POINT('Ctrl Pts',(10.7871183259999,15.2,-3.68216742900001));
#182853=CARTESIAN_POINT('Ctrl Pts',(10.7871183259999,11.6,-3.68216742900001));
#182854=CARTESIAN_POINT('Ctrl Pts',(10.7844550569999,15.2,-3.67961787200001));
#182855=CARTESIAN_POINT('Ctrl Pts',(10.7844550569999,11.6,-3.67961787200001));
#182856=CARTESIAN_POINT('Ctrl Pts',(10.7817931069999,15.2,-3.67707349500002));
#182857=CARTESIAN_POINT('Ctrl Pts',(10.7817931069999,11.6,-3.67707349500002));
#182858=CARTESIAN_POINT('Ctrl Pts',(10.7791324889999,15.2,-3.67453430200001));
#182859=CARTESIAN_POINT('Ctrl Pts',(10.7791324889999,11.6,-3.67453430200001));
#182860=CARTESIAN_POINT('Ctrl Pts',(10.7764732109999,15.2,-3.67200029300002));
#182861=CARTESIAN_POINT('Ctrl Pts',(10.7764732109999,11.6,-3.67200029300002));
#182862=CARTESIAN_POINT('Ctrl Pts',(10.7738152829999,15.2,-3.66947146800001));
#182863=CARTESIAN_POINT('Ctrl Pts',(10.7738152829999,11.6,-3.66947146800001));
#182864=CARTESIAN_POINT('Ctrl Pts',(10.7711587129999,15.2,-3.66694782800002));
#182865=CARTESIAN_POINT('Ctrl Pts',(10.7711587129999,11.6,-3.66694782800002));
#182866=CARTESIAN_POINT('Ctrl Pts',(10.7685035109999,15.2,-3.66442937400001));
#182867=CARTESIAN_POINT('Ctrl Pts',(10.7685035109999,11.6,-3.66442937400001));
#182868=CARTESIAN_POINT('Ctrl Pts',(10.7658496859999,15.2,-3.66191610700001));
#182869=CARTESIAN_POINT('Ctrl Pts',(10.7658496859999,11.6,-3.66191610700001));
#182870=CARTESIAN_POINT('Ctrl Pts',(10.7631972489999,15.2,-3.65940802800001));
#182871=CARTESIAN_POINT('Ctrl Pts',(10.7631972489999,11.6,-3.65940802800001));
#182872=CARTESIAN_POINT('Ctrl Pts',(10.7605462079999,15.2,-3.65690513800002));
#182873=CARTESIAN_POINT('Ctrl Pts',(10.7605462079999,11.6,-3.65690513800002));
#182874=CARTESIAN_POINT('Ctrl Pts',(10.7578965719999,15.2,-3.65440743700002));
#182875=CARTESIAN_POINT('Ctrl Pts',(10.7578965719999,11.6,-3.65440743700002));
#182876=CARTESIAN_POINT('Ctrl Pts',(10.7552483519999,15.2,-3.65191492600001));
#182877=CARTESIAN_POINT('Ctrl Pts',(10.7552483519999,11.6,-3.65191492600002));
#182878=CARTESIAN_POINT('Ctrl Pts',(10.7526015559999,15.2,-3.64942760700002));
#182879=CARTESIAN_POINT('Ctrl Pts',(10.7526015559999,11.6,-3.64942760700002));
#182880=CARTESIAN_POINT('Ctrl Pts',(10.7499561929999,15.2,-3.64694547900001));
#182881=CARTESIAN_POINT('Ctrl Pts',(10.7499561929999,11.6,-3.64694547900001));
#182882=CARTESIAN_POINT('Ctrl Pts',(10.7473122739999,15.2,-3.64446854400001));
#182883=CARTESIAN_POINT('Ctrl Pts',(10.7473122739999,11.6,-3.64446854400002));
#182884=CARTESIAN_POINT('Ctrl Pts',(10.7446698079999,15.2,-3.64199680200001));
#182885=CARTESIAN_POINT('Ctrl Pts',(10.7446698079999,11.6,-3.64199680200001));
#182886=CARTESIAN_POINT('Ctrl Pts',(10.7420288039999,15.2,-3.63953025500001));
#182887=CARTESIAN_POINT('Ctrl Pts',(10.7420288039999,11.6,-3.63953025500001));
#182888=CARTESIAN_POINT('Ctrl Pts',(10.7393892719999,15.2,-3.63706890200001));
#182889=CARTESIAN_POINT('Ctrl Pts',(10.7393892719999,11.6,-3.63706890200001));
#182890=CARTESIAN_POINT('Ctrl Pts',(10.7367512209999,15.2,-3.63461274500001));
#182891=CARTESIAN_POINT('Ctrl Pts',(10.7367512209999,11.6,-3.63461274500001));
#182892=CARTESIAN_POINT('Ctrl Pts',(10.7341146619999,15.2,-3.63216178500001));
#182893=CARTESIAN_POINT('Ctrl Pts',(10.7341146619999,11.6,-3.63216178500001));
#182894=CARTESIAN_POINT('Ctrl Pts',(10.7314796019999,15.2,-3.62971602300002));
#182895=CARTESIAN_POINT('Ctrl Pts',(10.7314796019999,11.6,-3.62971602300002));
#182896=CARTESIAN_POINT('Ctrl Pts',(10.7288460529999,15.2,-3.62727545700002));
#182897=CARTESIAN_POINT('Ctrl Pts',(10.7288460529999,11.6,-3.62727545700002));
#182898=CARTESIAN_POINT('Ctrl Pts',(10.7262140239999,15.2,-3.62484009100001));
#182899=CARTESIAN_POINT('Ctrl Pts',(10.7262140239999,11.6,-3.62484009100001));
#182900=CARTESIAN_POINT('Ctrl Pts',(10.7235835239999,15.2,-3.62240992500002));
#182901=CARTESIAN_POINT('Ctrl Pts',(10.7235835239999,11.6,-3.62240992500002));
#182902=CARTESIAN_POINT('Ctrl Pts',(10.7209545619999,15.2,-3.61998495800002));
#182903=CARTESIAN_POINT('Ctrl Pts',(10.7209545619999,11.6,-3.61998495800002));
#182904=CARTESIAN_POINT('Ctrl Pts',(10.7183271499999,15.2,-3.61756519200001));
#182905=CARTESIAN_POINT('Ctrl Pts',(10.7183271499999,11.6,-3.61756519200001));
#182906=CARTESIAN_POINT('Ctrl Pts',(10.7157012959999,15.2,-3.61515062900001));
#182907=CARTESIAN_POINT('Ctrl Pts',(10.7157012959999,11.6,-3.61515062900002));
#182908=CARTESIAN_POINT('Ctrl Pts',(10.7130770099999,15.2,-3.61274126800001));
#182909=CARTESIAN_POINT('Ctrl Pts',(10.7130770099999,11.6,-3.61274126800002));
#182910=CARTESIAN_POINT('Ctrl Pts',(10.7104543019999,15.2,-3.61033710900001));
#182911=CARTESIAN_POINT('Ctrl Pts',(10.7104543019999,11.6,-3.61033710900002));
#182912=CARTESIAN_POINT('Ctrl Pts',(10.7078331809999,15.2,-3.60793815500001));
#182913=CARTESIAN_POINT('Ctrl Pts',(10.7078331809999,11.6,-3.60793815500001));
#182914=CARTESIAN_POINT('Ctrl Pts',(10.7052136559999,15.2,-3.60554440400001));
#182915=CARTESIAN_POINT('Ctrl Pts',(10.7052136559999,11.6,-3.60554440400001));
#182916=CARTESIAN_POINT('Ctrl Pts',(10.7025957399999,15.2,-3.60315585900001));
#182917=CARTESIAN_POINT('Ctrl Pts',(10.7025957399999,11.6,-3.60315585900001));
#182918=CARTESIAN_POINT('Ctrl Pts',(10.6999794399999,15.2,-3.60077252100002));
#182919=CARTESIAN_POINT('Ctrl Pts',(10.6999794399999,11.6,-3.60077252100002));
#182920=CARTESIAN_POINT('Ctrl Pts',(10.6973647669999,15.2,-3.59839438800002));
#182921=CARTESIAN_POINT('Ctrl Pts',(10.6973647669999,11.6,-3.59839438800002));
#182922=CARTESIAN_POINT('Ctrl Pts',(10.6947517299999,15.2,-3.59602146200002));
#182923=CARTESIAN_POINT('Ctrl Pts',(10.6947517299999,11.6,-3.59602146200002));
#182924=CARTESIAN_POINT('Ctrl Pts',(10.6921403399999,15.2,-3.59365374400001));
#182925=CARTESIAN_POINT('Ctrl Pts',(10.6921403399999,11.6,-3.59365374400001));
#182926=CARTESIAN_POINT('Ctrl Pts',(10.6895306049999,15.2,-3.59129123500002));
#182927=CARTESIAN_POINT('Ctrl Pts',(10.6895306049999,11.6,-3.59129123500002));
#182928=CARTESIAN_POINT('Ctrl Pts',(10.6869225359999,15.2,-3.58893393500002));
#182929=CARTESIAN_POINT('Ctrl Pts',(10.6869225359999,11.6,-3.58893393500002));
#182930=CARTESIAN_POINT('Ctrl Pts',(10.6843161429999,15.2,-3.58658184500001));
#182931=CARTESIAN_POINT('Ctrl Pts',(10.6843161429999,11.6,-3.58658184500001));
#182932=CARTESIAN_POINT('Ctrl Pts',(10.6817114369999,15.2,-3.58423496500002));
#182933=CARTESIAN_POINT('Ctrl Pts',(10.6817114369999,11.6,-3.58423496500002));
#182934=CARTESIAN_POINT('Ctrl Pts',(10.6791084249999,15.2,-3.58189329600001));
#182935=CARTESIAN_POINT('Ctrl Pts',(10.6791084249999,11.6,-3.58189329600001));
#182936=CARTESIAN_POINT('Ctrl Pts',(10.6765071199999,15.2,-3.57955683900002));
#182937=CARTESIAN_POINT('Ctrl Pts',(10.6765071199999,11.6,-3.57955683900002));
#182938=CARTESIAN_POINT('Ctrl Pts',(10.6739075299999,15.2,-3.57722559400001));
#182939=CARTESIAN_POINT('Ctrl Pts',(10.6739075299999,11.6,-3.57722559400001));
#182940=CARTESIAN_POINT('Ctrl Pts',(10.6713096659999,15.2,-3.57489956100002));
#182941=CARTESIAN_POINT('Ctrl Pts',(10.6713096659999,11.6,-3.57489956100002));
#182942=CARTESIAN_POINT('Ctrl Pts',(10.6687135369999,15.2,-3.57257874200001));
#182943=CARTESIAN_POINT('Ctrl Pts',(10.6687135369999,11.6,-3.57257874200001));
#182944=CARTESIAN_POINT('Ctrl Pts',(10.6661191539999,15.2,-3.57026313700001));
#182945=CARTESIAN_POINT('Ctrl Pts',(10.6661191539999,11.6,-3.57026313700001));
#182946=CARTESIAN_POINT('Ctrl Pts',(10.6635265279999,15.2,-3.56795274600001));
#182947=CARTESIAN_POINT('Ctrl Pts',(10.6635265279999,11.6,-3.56795274600001));
#182948=CARTESIAN_POINT('Ctrl Pts',(10.6609356659999,15.2,-3.56564757100001));
#182949=CARTESIAN_POINT('Ctrl Pts',(10.6609356659999,11.6,-3.56564757100002));
#182950=CARTESIAN_POINT('Ctrl Pts',(10.6583465819999,15.2,-3.56334761200001));
#182951=CARTESIAN_POINT('Ctrl Pts',(10.6583465819999,11.6,-3.56334761200001));
#182952=CARTESIAN_POINT('Ctrl Pts',(10.6557592819999,15.2,-3.56105286800001));
#182953=CARTESIAN_POINT('Ctrl Pts',(10.6557592819999,11.6,-3.56105286800001));
#182954=CARTESIAN_POINT('Ctrl Pts',(10.6531737789999,15.2,-3.55876334200001));
#182955=CARTESIAN_POINT('Ctrl Pts',(10.6531737789999,11.6,-3.55876334200001));
#182956=CARTESIAN_POINT('Ctrl Pts',(10.6505900819999,15.2,-3.55647903300001));
#182957=CARTESIAN_POINT('Ctrl Pts',(10.6505900819999,11.6,-3.55647903300001));
#182958=CARTESIAN_POINT('Ctrl Pts',(10.6480082019999,15.2,-3.55419994100002));
#182959=CARTESIAN_POINT('Ctrl Pts',(10.6480082019999,11.6,-3.55419994100002));
#182960=CARTESIAN_POINT('Ctrl Pts',(10.6454281479999,15.2,-3.55192606900002));
#182961=CARTESIAN_POINT('Ctrl Pts',(10.6454281479999,11.6,-3.55192606900002));
#182962=CARTESIAN_POINT('Ctrl Pts',(10.6428499309999,15.2,-3.54965741400001));
#182963=CARTESIAN_POINT('Ctrl Pts',(10.6428499309999,11.6,-3.54965741400001));
#182964=CARTESIAN_POINT('Ctrl Pts',(10.6402735619999,15.2,-3.54739398000001));
#182965=CARTESIAN_POINT('Ctrl Pts',(10.6402735619999,11.6,-3.54739398000001));
#182966=CARTESIAN_POINT('Ctrl Pts',(10.6376990499999,15.2,-3.54513576600001));
#182967=CARTESIAN_POINT('Ctrl Pts',(10.6376990499999,11.6,-3.54513576600001));
#182968=CARTESIAN_POINT('Ctrl Pts',(10.6351264049999,15.2,-3.54288277200002));
#182969=CARTESIAN_POINT('Ctrl Pts',(10.6351264049999,11.6,-3.54288277200002));
#182970=CARTESIAN_POINT('Ctrl Pts',(10.6325556389999,15.2,-3.54063499900001));
#182971=CARTESIAN_POINT('Ctrl Pts',(10.6325556389999,11.6,-3.54063499900001));
#182972=CARTESIAN_POINT('Ctrl Pts',(10.6299867589999,15.2,-3.53839244700001));
#182973=CARTESIAN_POINT('Ctrl Pts',(10.6299867589999,11.6,-3.53839244700001));
#182974=CARTESIAN_POINT('Ctrl Pts',(10.6274197799999,15.2,-3.53615511700001));
#182975=CARTESIAN_POINT('Ctrl Pts',(10.6274197799999,11.6,-3.53615511700002));
#182976=CARTESIAN_POINT('Ctrl Pts',(10.6248547079999,15.2,-3.53392301000001));
#182977=CARTESIAN_POINT('Ctrl Pts',(10.6248547079999,11.6,-3.53392301000001));
#182978=CARTESIAN_POINT('Ctrl Pts',(10.6222915559999,15.2,-3.53169612600002));
#182979=CARTESIAN_POINT('Ctrl Pts',(10.6222915559999,11.6,-3.53169612600002));
#182980=CARTESIAN_POINT('Ctrl Pts',(10.6197303339999,15.2,-3.52947446500002));
#182981=CARTESIAN_POINT('Ctrl Pts',(10.6197303339999,11.6,-3.52947446500002));
#182982=CARTESIAN_POINT('Ctrl Pts',(10.6171710509999,15.2,-3.52725802700002));
#182983=CARTESIAN_POINT('Ctrl Pts',(10.6171710509999,11.6,-3.52725802700002));
#182984=CARTESIAN_POINT('Ctrl Pts',(10.6146137189999,15.2,-3.52504681400001));
#182985=CARTESIAN_POINT('Ctrl Pts',(10.6146137189999,11.6,-3.52504681400002));
#182986=CARTESIAN_POINT('Ctrl Pts',(10.6120583479999,15.2,-3.52284082600002));
#182987=CARTESIAN_POINT('Ctrl Pts',(10.6120583479999,11.6,-3.52284082600002));
#182988=CARTESIAN_POINT('Ctrl Pts',(10.6095049489999,15.2,-3.52064006300001));
#182989=CARTESIAN_POINT('Ctrl Pts',(10.6095049489999,11.6,-3.52064006300001));
#182990=CARTESIAN_POINT('Ctrl Pts',(10.6069535309999,15.2,-3.51844452500002));
#182991=CARTESIAN_POINT('Ctrl Pts',(10.6069535309999,11.6,-3.51844452500002));
#182992=CARTESIAN_POINT('Ctrl Pts',(10.6044041049999,15.2,-3.51625421300001));
#182993=CARTESIAN_POINT('Ctrl Pts',(10.6044041049999,11.6,-3.51625421300001));
#182994=CARTESIAN_POINT('Ctrl Pts',(10.6018566829999,15.2,-3.51406912700002));
#182995=CARTESIAN_POINT('Ctrl Pts',(10.6018566829999,11.6,-3.51406912700002));
#182996=CARTESIAN_POINT('Ctrl Pts',(10.5993112729999,15.2,-3.51188926900001));
#182997=CARTESIAN_POINT('Ctrl Pts',(10.5993112729999,11.6,-3.51188926900001));
#182998=CARTESIAN_POINT('Ctrl Pts',(10.5967678879999,15.2,-3.50971463600001));
#182999=CARTESIAN_POINT('Ctrl Pts',(10.5967678879999,11.6,-3.50971463600001));
#183000=CARTESIAN_POINT('Ctrl Pts',(10.5942265379999,15.2,-3.50754523200001));
#183001=CARTESIAN_POINT('Ctrl Pts',(10.5942265379999,11.6,-3.50754523200001));
#183002=CARTESIAN_POINT('Ctrl Pts',(10.5916872319999,15.2,-3.50538105500001));
#183003=CARTESIAN_POINT('Ctrl Pts',(10.5916872319999,11.6,-3.50538105500001));
#183004=CARTESIAN_POINT('Ctrl Pts',(10.5891499829999,15.2,-3.50322210700002));
#183005=CARTESIAN_POINT('Ctrl Pts',(10.5891499829999,11.6,-3.50322210700002));
#183006=CARTESIAN_POINT('Ctrl Pts',(10.5866147999999,15.2,-3.50106838700002));
#183007=CARTESIAN_POINT('Ctrl Pts',(10.5866147999999,11.6,-3.50106838700002));
#183008=CARTESIAN_POINT('Ctrl Pts',(10.5840816949999,15.2,-3.49891989600001));
#183009=CARTESIAN_POINT('Ctrl Pts',(10.5840816949999,11.6,-3.49891989600001));
#183010=CARTESIAN_POINT('Ctrl Pts',(10.5815506769999,15.2,-3.49677663500001));
#183011=CARTESIAN_POINT('Ctrl Pts',(10.5815506769999,11.6,-3.49677663500001));
#183012=CARTESIAN_POINT('Ctrl Pts',(10.5790217569999,15.2,-3.49463860200002));
#183013=CARTESIAN_POINT('Ctrl Pts',(10.5790217569999,11.6,-3.49463860200002));
#183014=CARTESIAN_POINT('Ctrl Pts',(10.5764949479999,15.2,-3.49250580000001));
#183015=CARTESIAN_POINT('Ctrl Pts',(10.5764949479999,11.6,-3.49250580000001));
#183016=CARTESIAN_POINT('Ctrl Pts',(10.5739702579999,15.2,-3.49037822900002));
#183017=CARTESIAN_POINT('Ctrl Pts',(10.5739702579999,11.6,-3.49037822900002));
#183018=CARTESIAN_POINT('Ctrl Pts',(10.5714476989999,15.2,-3.48825588800001));
#183019=CARTESIAN_POINT('Ctrl Pts',(10.5714476989999,11.6,-3.48825588800001));
#183020=CARTESIAN_POINT('Ctrl Pts',(10.5689272829999,15.2,-3.48613877700001));
#183021=CARTESIAN_POINT('Ctrl Pts',(10.5689272829999,11.6,-3.48613877700001));
#183022=CARTESIAN_POINT('Ctrl Pts',(10.5664090179999,15.2,-3.48402689800002));
#183023=CARTESIAN_POINT('Ctrl Pts',(10.5664090179999,11.6,-3.48402689800002));
#183024=CARTESIAN_POINT('Ctrl Pts',(10.5638929169999,15.2,-3.48192025000001));
#183025=CARTESIAN_POINT('Ctrl Pts',(10.5638929169999,11.6,-3.48192025000001));
#183026=CARTESIAN_POINT('Ctrl Pts',(10.5613789899999,15.2,-3.47981883400001));
#183027=CARTESIAN_POINT('Ctrl Pts',(10.5613789899999,11.6,-3.47981883400002));
#183028=CARTESIAN_POINT('Ctrl Pts',(10.5588672479999,15.2,-3.47772265000001));
#183029=CARTESIAN_POINT('Ctrl Pts',(10.5588672479999,11.6,-3.47772265000002));
#183030=CARTESIAN_POINT('Ctrl Pts',(10.5563577029999,15.2,-3.47563169800001));
#183031=CARTESIAN_POINT('Ctrl Pts',(10.5563577029999,11.6,-3.47563169800001));
#183032=CARTESIAN_POINT('Ctrl Pts',(10.5538503639999,15.2,-3.47354597800001));
#183033=CARTESIAN_POINT('Ctrl Pts',(10.5538503639999,11.6,-3.47354597800001));
#183034=CARTESIAN_POINT('Ctrl Pts',(10.5513452449999,15.2,-3.47146549100001));
#183035=CARTESIAN_POINT('Ctrl Pts',(10.5513452449999,11.6,-3.47146549100001));
#183036=CARTESIAN_POINT('Ctrl Pts',(10.5488423529999,15.2,-3.46939023800001));
#183037=CARTESIAN_POINT('Ctrl Pts',(10.5488423529999,11.6,-3.46939023800001));
#183038=CARTESIAN_POINT('Ctrl Pts',(10.5463417019999,15.2,-3.46732021700001));
#183039=CARTESIAN_POINT('Ctrl Pts',(10.5463417019999,11.6,-3.46732021700001));
#183040=CARTESIAN_POINT('Ctrl Pts',(10.5438433009999,15.2,-3.46525543000002));
#183041=CARTESIAN_POINT('Ctrl Pts',(10.5438433009999,11.6,-3.46525543000002));
#183042=CARTESIAN_POINT('Ctrl Pts',(10.5413471629999,15.2,-3.46319587600001));
#183043=CARTESIAN_POINT('Ctrl Pts',(10.5413471629999,11.6,-3.46319587600001));
#183044=CARTESIAN_POINT('Ctrl Pts',(10.5388532969999,15.2,-3.46114155700001));
#183045=CARTESIAN_POINT('Ctrl Pts',(10.5388532969999,11.6,-3.46114155700001));
#183046=CARTESIAN_POINT('Ctrl Pts',(10.5363617169999,15.2,-3.45909247100002));
#183047=CARTESIAN_POINT('Ctrl Pts',(10.5363617169999,11.6,-3.45909247100002));
#183048=CARTESIAN_POINT('Ctrl Pts',(10.5338724319999,15.2,-3.45704862000002));
#183049=CARTESIAN_POINT('Ctrl Pts',(10.5338724319999,11.6,-3.45704862000002));
#183050=CARTESIAN_POINT('Ctrl Pts',(10.5313854529999,15.2,-3.45501000300001));
#183051=CARTESIAN_POINT('Ctrl Pts',(10.5313854529999,11.6,-3.45501000300001));
#183052=CARTESIAN_POINT('Ctrl Pts',(10.5289007929999,15.2,-3.45297662100001));
#183053=CARTESIAN_POINT('Ctrl Pts',(10.5289007929999,11.6,-3.45297662100002));
#183054=CARTESIAN_POINT('Ctrl Pts',(10.5264184599999,15.2,-3.45094847300001));
#183055=CARTESIAN_POINT('Ctrl Pts',(10.5264184599999,11.6,-3.45094847300001));
#183056=CARTESIAN_POINT('Ctrl Pts',(10.5239384669999,15.2,-3.44892556000001));
#183057=CARTESIAN_POINT('Ctrl Pts',(10.5239384669999,11.6,-3.44892556000001));
#183058=CARTESIAN_POINT('Ctrl Pts',(10.5214608269999,15.2,-3.44690788300001));
#183059=CARTESIAN_POINT('Ctrl Pts',(10.5214608269999,11.6,-3.44690788300001));
#183060=CARTESIAN_POINT('Ctrl Pts',(10.5189855499999,15.2,-3.44489544000002));
#183061=CARTESIAN_POINT('Ctrl Pts',(10.5189855499999,11.6,-3.44489544000002));
#183062=CARTESIAN_POINT('Ctrl Pts',(10.5165126449999,15.2,-3.44288823300001));
#183063=CARTESIAN_POINT('Ctrl Pts',(10.5165126449999,11.6,-3.44288823300001));
#183064=CARTESIAN_POINT('Ctrl Pts',(10.5140421269999,15.2,-3.44088626100001));
#183065=CARTESIAN_POINT('Ctrl Pts',(10.5140421269999,11.6,-3.44088626100001));
#183066=CARTESIAN_POINT('Ctrl Pts',(10.5115740039999,15.2,-3.43888952500001));
#183067=CARTESIAN_POINT('Ctrl Pts',(10.5115740039999,11.6,-3.43888952500001));
#183068=CARTESIAN_POINT('Ctrl Pts',(10.5091082899999,15.2,-3.43689802500001));
#183069=CARTESIAN_POINT('Ctrl Pts',(10.5091082899999,11.6,-3.43689802500002));
#183070=CARTESIAN_POINT('Ctrl Pts',(10.5066449939999,15.2,-3.43491176000001));
#183071=CARTESIAN_POINT('Ctrl Pts',(10.5066449939999,11.6,-3.43491176000001));
#183072=CARTESIAN_POINT('Ctrl Pts',(10.5041841299999,15.2,-3.43293073100002));
#183073=CARTESIAN_POINT('Ctrl Pts',(10.5041841299999,11.6,-3.43293073100002));
#183074=CARTESIAN_POINT('Ctrl Pts',(10.5017257079999,15.2,-3.43095493800002));
#183075=CARTESIAN_POINT('Ctrl Pts',(10.5017257079999,11.6,-3.43095493800002));
#183076=CARTESIAN_POINT('Ctrl Pts',(10.4992697399999,15.2,-3.42898438100002));
#183077=CARTESIAN_POINT('Ctrl Pts',(10.4992697399999,11.6,-3.42898438100002));
#183078=CARTESIAN_POINT('Ctrl Pts',(10.4968162359999,15.2,-3.42701906000002));
#183079=CARTESIAN_POINT('Ctrl Pts',(10.4968162359999,11.6,-3.42701906000002));
#183080=CARTESIAN_POINT('Ctrl Pts',(10.4943652099999,15.2,-3.42505897500001));
#183081=CARTESIAN_POINT('Ctrl Pts',(10.4943652099999,11.6,-3.42505897500002));
#183082=CARTESIAN_POINT('Ctrl Pts',(10.4919166709999,15.2,-3.42310412600002));
#183083=CARTESIAN_POINT('Ctrl Pts',(10.4919166709999,11.6,-3.42310412600002));
#183084=CARTESIAN_POINT('Ctrl Pts',(10.4894706319999,15.2,-3.42115451300002));
#183085=CARTESIAN_POINT('Ctrl Pts',(10.4894706319999,11.6,-3.42115451300002));
#183086=CARTESIAN_POINT('Ctrl Pts',(10.4870271039999,15.2,-3.41921013700001));
#183087=CARTESIAN_POINT('Ctrl Pts',(10.4870271039999,11.6,-3.41921013700001));
#183088=CARTESIAN_POINT('Ctrl Pts',(10.4845860999999,15.2,-3.41727099600002));
#183089=CARTESIAN_POINT('Ctrl Pts',(10.4845860999999,11.6,-3.41727099600002));
#183090=CARTESIAN_POINT('Ctrl Pts',(10.4821476289999,15.2,-3.41533709100001));
#183091=CARTESIAN_POINT('Ctrl Pts',(10.4821476289999,11.6,-3.41533709100002));
#183092=CARTESIAN_POINT('Ctrl Pts',(10.4797117049999,15.2,-3.41340842300002));
#183093=CARTESIAN_POINT('Ctrl Pts',(10.4797117049999,11.6,-3.41340842300002));
#183094=CARTESIAN_POINT('Ctrl Pts',(10.4772783389999,15.2,-3.41148499200001));
#183095=CARTESIAN_POINT('Ctrl Pts',(10.4772783389999,11.6,-3.41148499200001));
#183096=CARTESIAN_POINT('Ctrl Pts',(10.4748475419999,15.2,-3.40956679600001));
#183097=CARTESIAN_POINT('Ctrl Pts',(10.4748475419999,11.6,-3.40956679600001));
#183098=CARTESIAN_POINT('Ctrl Pts',(10.4724193259999,15.2,-3.40765383700001));
#183099=CARTESIAN_POINT('Ctrl Pts',(10.4724193259999,11.6,-3.40765383700001));
#183100=CARTESIAN_POINT('Ctrl Pts',(10.4699937039999,15.2,-3.40574611300001));
#183101=CARTESIAN_POINT('Ctrl Pts',(10.4699937039999,11.6,-3.40574611300001));
#183102=CARTESIAN_POINT('Ctrl Pts',(10.4675706859999,15.2,-3.40384362500001));
#183103=CARTESIAN_POINT('Ctrl Pts',(10.4675706859999,11.6,-3.40384362500001));
#183104=CARTESIAN_POINT('Ctrl Pts',(10.4651502849999,15.2,-3.40194637400002));
#183105=CARTESIAN_POINT('Ctrl Pts',(10.4651502849999,11.6,-3.40194637400002));
#183106=CARTESIAN_POINT('Ctrl Pts',(10.4627325119999,15.2,-3.40005435900002));
#183107=CARTESIAN_POINT('Ctrl Pts',(10.4627325119999,11.6,-3.40005435900002));
#183108=CARTESIAN_POINT('Ctrl Pts',(10.4603173799999,15.2,-3.39816757900001));
#183109=CARTESIAN_POINT('Ctrl Pts',(10.4603173799999,11.6,-3.39816757900001));
#183110=CARTESIAN_POINT('Ctrl Pts',(10.4579048999999,15.2,-3.39628603500001));
#183111=CARTESIAN_POINT('Ctrl Pts',(10.4579048999999,11.6,-3.39628603500001));
#183112=CARTESIAN_POINT('Ctrl Pts',(10.4554950839999,15.2,-3.39440972700002));
#183113=CARTESIAN_POINT('Ctrl Pts',(10.4554950839999,11.6,-3.39440972700002));
#183114=CARTESIAN_POINT('Ctrl Pts',(10.4530879439999,15.2,-3.39253865400002));
#183115=CARTESIAN_POINT('Ctrl Pts',(10.4530879439999,11.6,-3.39253865400002));
#183116=CARTESIAN_POINT('Ctrl Pts',(10.4506834919999,15.2,-3.39067281600002));
#183117=CARTESIAN_POINT('Ctrl Pts',(10.4506834919999,11.6,-3.39067281600002));
#183118=CARTESIAN_POINT('Ctrl Pts',(10.4482817399999,15.2,-3.38881221500001));
#183119=CARTESIAN_POINT('Ctrl Pts',(10.4482817399999,11.6,-3.38881221500001));
#183120=CARTESIAN_POINT('Ctrl Pts',(10.4458826999999,15.2,-3.38695684700001));
#183121=CARTESIAN_POINT('Ctrl Pts',(10.4458826999999,11.6,-3.38695684700001));
#183122=CARTESIAN_POINT('Ctrl Pts',(10.4434863849999,15.2,-3.38510671600002));
#183123=CARTESIAN_POINT('Ctrl Pts',(10.4434863849999,11.6,-3.38510671600002));
#183124=CARTESIAN_POINT('Ctrl Pts',(10.4410928049999,15.2,-3.38326181800001));
#183125=CARTESIAN_POINT('Ctrl Pts',(10.4410928049999,11.6,-3.38326181800001));
#183126=CARTESIAN_POINT('Ctrl Pts',(10.4387019739999,15.2,-3.38142215600001));
#183127=CARTESIAN_POINT('Ctrl Pts',(10.4387019739999,11.6,-3.38142215600001));
#183128=CARTESIAN_POINT('Ctrl Pts',(10.4363139019999,15.2,-3.37958772900001));
#183129=CARTESIAN_POINT('Ctrl Pts',(10.4363139019999,11.6,-3.37958772900001));
#183130=CARTESIAN_POINT('Ctrl Pts',(10.4339286029999,15.2,-3.37775853500001));
#183131=CARTESIAN_POINT('Ctrl Pts',(10.4339286029999,11.6,-3.37775853500002));
#183132=CARTESIAN_POINT('Ctrl Pts',(10.4315460899999,15.2,-3.37593457500001));
#183133=CARTESIAN_POINT('Ctrl Pts',(10.4315460899999,11.6,-3.37593457500002));
#183134=CARTESIAN_POINT('Ctrl Pts',(10.4291663729999,15.2,-3.37411585000002));
#183135=CARTESIAN_POINT('Ctrl Pts',(10.4291663729999,11.6,-3.37411585000002));
#183136=CARTESIAN_POINT('Ctrl Pts',(10.4267894639999,15.2,-3.37230235900002));
#183137=CARTESIAN_POINT('Ctrl Pts',(10.4267894639999,11.6,-3.37230235900002));
#183138=CARTESIAN_POINT('Ctrl Pts',(10.4244153789999,15.2,-3.37049410100001));
#183139=CARTESIAN_POINT('Ctrl Pts',(10.4244153789999,11.6,-3.37049410100001));
#183140=CARTESIAN_POINT('Ctrl Pts',(10.4220441259999,15.2,-3.36869107600001));
#183141=CARTESIAN_POINT('Ctrl Pts',(10.4220441259999,11.6,-3.36869107600001));
#183142=CARTESIAN_POINT('Ctrl Pts',(10.4196757189999,15.2,-3.36689328500002));
#183143=CARTESIAN_POINT('Ctrl Pts',(10.4196757189999,11.6,-3.36689328500002));
#183144=CARTESIAN_POINT('Ctrl Pts',(10.4173101699999,15.2,-3.36510072600001));
#183145=CARTESIAN_POINT('Ctrl Pts',(10.4173101699999,11.6,-3.36510072600001));
#183146=CARTESIAN_POINT('Ctrl Pts',(10.4149474929999,15.2,-3.36331340000001));
#183147=CARTESIAN_POINT('Ctrl Pts',(10.4149474929999,11.6,-3.36331340000001));
#183148=CARTESIAN_POINT('Ctrl Pts',(10.4125876979999,15.2,-3.36153130600001));
#183149=CARTESIAN_POINT('Ctrl Pts',(10.4125876979999,11.6,-3.36153130600001));
#183150=CARTESIAN_POINT('Ctrl Pts',(10.4102307989999,15.2,-3.35975444400002));
#183151=CARTESIAN_POINT('Ctrl Pts',(10.4102307989999,11.6,-3.35975444400002));
#183152=CARTESIAN_POINT('Ctrl Pts',(10.4078768069999,15.2,-3.35798281300002));
#183153=CARTESIAN_POINT('Ctrl Pts',(10.4078768069999,11.6,-3.35798281300002));
#183154=CARTESIAN_POINT('Ctrl Pts',(10.4055257379999,15.2,-3.35621641400001));
#183155=CARTESIAN_POINT('Ctrl Pts',(10.4055257379999,11.6,-3.35621641400001));
#183156=CARTESIAN_POINT('Ctrl Pts',(10.4031775999999,15.2,-3.35445524600001));
#183157=CARTESIAN_POINT('Ctrl Pts',(10.4031775999999,11.6,-3.35445524600001));
#183158=CARTESIAN_POINT('Ctrl Pts',(10.4008324069999,15.2,-3.35269930900001));
#183159=CARTESIAN_POINT('Ctrl Pts',(10.4008324069999,11.6,-3.35269930900001));
#183160=CARTESIAN_POINT('Ctrl Pts',(10.3984901739999,15.2,-3.35094860300002));
#183161=CARTESIAN_POINT('Ctrl Pts',(10.3984901739999,11.6,-3.35094860300002));
#183162=CARTESIAN_POINT('Ctrl Pts',(10.3961509099999,15.2,-3.34920312600001));
#183163=CARTESIAN_POINT('Ctrl Pts',(10.3961509099999,11.6,-3.34920312600001));
#183164=CARTESIAN_POINT('Ctrl Pts',(10.3938146309999,15.2,-3.34746287900002));
#183165=CARTESIAN_POINT('Ctrl Pts',(10.3938146309999,11.6,-3.34746287900002));
#183166=CARTESIAN_POINT('Ctrl Pts',(10.3914813469999,15.2,-3.34572786200001));
#183167=CARTESIAN_POINT('Ctrl Pts',(10.3914813469999,11.6,-3.34572786200001));
#183168=CARTESIAN_POINT('Ctrl Pts',(10.3891510709999,15.2,-3.34399807300001));
#183169=CARTESIAN_POINT('Ctrl Pts',(10.3891510709999,11.6,-3.34399807300001));
#183170=CARTESIAN_POINT('Ctrl Pts',(10.3868238179999,15.2,-3.34227351400001));
#183171=CARTESIAN_POINT('Ctrl Pts',(10.3868238179999,11.6,-3.34227351400001));
#183172=CARTESIAN_POINT('Ctrl Pts',(10.3844995979999,15.2,-3.34055418200002));
#183173=CARTESIAN_POINT('Ctrl Pts',(10.3844995979999,11.6,-3.34055418200002));
#183174=CARTESIAN_POINT('Ctrl Pts',(10.3821784259999,15.2,-3.33884007800001));
#183175=CARTESIAN_POINT('Ctrl Pts',(10.3821784259999,11.6,-3.33884007800001));
#183176=CARTESIAN_POINT('Ctrl Pts',(10.3798603139999,15.2,-3.33713120100001));
#183177=CARTESIAN_POINT('Ctrl Pts',(10.3798603139999,11.6,-3.33713120100001));
#183178=CARTESIAN_POINT('Ctrl Pts',(10.3775452729999,15.2,-3.33542755200002));
#183179=CARTESIAN_POINT('Ctrl Pts',(10.3775452729999,11.6,-3.33542755200002));
#183180=CARTESIAN_POINT('Ctrl Pts',(10.3752333189999,15.2,-3.33372913000002));
#183181=CARTESIAN_POINT('Ctrl Pts',(10.3752333189999,11.6,-3.33372913000002));
#183182=CARTESIAN_POINT('Ctrl Pts',(10.3729244619999,15.2,-3.33203593300002));
#183183=CARTESIAN_POINT('Ctrl Pts',(10.3729244619999,11.6,-3.33203593300002));
#183184=CARTESIAN_POINT('Ctrl Pts',(10.3706187169999,15.2,-3.33034796100002));
#183185=CARTESIAN_POINT('Ctrl Pts',(10.3706187169999,11.6,-3.33034796100002));
#183186=CARTESIAN_POINT('Ctrl Pts',(10.3683160969999,15.2,-3.32866521600002));
#183187=CARTESIAN_POINT('Ctrl Pts',(10.3683160969999,11.6,-3.32866521600002));
#183188=CARTESIAN_POINT('Ctrl Pts',(10.3660166129999,15.2,-3.32698769300002));
#183189=CARTESIAN_POINT('Ctrl Pts',(10.3660166129999,11.6,-3.32698769300002));
#183190=CARTESIAN_POINT('Ctrl Pts',(10.3637202799999,15.2,-3.32531539600001));
#183191=CARTESIAN_POINT('Ctrl Pts',(10.3637202799999,11.6,-3.32531539600002));
#183192=CARTESIAN_POINT('Ctrl Pts',(10.3614271109999,15.2,-3.32364832300001));
#183193=CARTESIAN_POINT('Ctrl Pts',(10.3614271109999,11.6,-3.32364832300002));
#183194=CARTESIAN_POINT('Ctrl Pts',(10.3591371169999,15.2,-3.32198647300002));
#183195=CARTESIAN_POINT('Ctrl Pts',(10.3591371169999,11.6,-3.32198647300002));
#183196=CARTESIAN_POINT('Ctrl Pts',(10.3568503129999,15.2,-3.32032984500001));
#183197=CARTESIAN_POINT('Ctrl Pts',(10.3568503129999,11.6,-3.32032984500001));
#183198=CARTESIAN_POINT('Ctrl Pts',(10.3545667119999,15.2,-3.31867843900001));
#183199=CARTESIAN_POINT('Ctrl Pts',(10.3545667119999,11.6,-3.31867843900001));
#183200=CARTESIAN_POINT('Ctrl Pts',(10.3522863269999,15.2,-3.31703225500001));
#183201=CARTESIAN_POINT('Ctrl Pts',(10.3522863269999,11.6,-3.31703225500001));
#183202=CARTESIAN_POINT('Ctrl Pts',(10.3500091699999,15.2,-3.31539129200001));
#183203=CARTESIAN_POINT('Ctrl Pts',(10.3500091699999,11.6,-3.31539129200001));
#183204=CARTESIAN_POINT('Ctrl Pts',(10.3477352559999,15.2,-3.31375555000001));
#183205=CARTESIAN_POINT('Ctrl Pts',(10.3477352559999,11.6,-3.31375555000002));
#183206=CARTESIAN_POINT('Ctrl Pts',(10.3454645979999,15.2,-3.31212502700001));
#183207=CARTESIAN_POINT('Ctrl Pts',(10.3454645979999,11.6,-3.31212502700002));
#183208=CARTESIAN_POINT('Ctrl Pts',(10.3431972079999,15.2,-3.31049972300002));
#183209=CARTESIAN_POINT('Ctrl Pts',(10.3431972079999,11.6,-3.31049972300002));
#183210=CARTESIAN_POINT('Ctrl Pts',(10.3409331009999,15.2,-3.30887963800001));
#183211=CARTESIAN_POINT('Ctrl Pts',(10.3409331009999,11.6,-3.30887963800001));
#183212=CARTESIAN_POINT('Ctrl Pts',(10.3386722889999,15.2,-3.30726477100002));
#183213=CARTESIAN_POINT('Ctrl Pts',(10.3386722889999,11.6,-3.30726477100002));
#183214=CARTESIAN_POINT('Ctrl Pts',(10.3364147869999,15.2,-3.30565512200002));
#183215=CARTESIAN_POINT('Ctrl Pts',(10.3364147869999,11.6,-3.30565512200002));
#183216=CARTESIAN_POINT('Ctrl Pts',(10.3341606059999,15.2,-3.30405069000001));
#183217=CARTESIAN_POINT('Ctrl Pts',(10.3341606059999,11.6,-3.30405069000001));
#183218=CARTESIAN_POINT('Ctrl Pts',(10.3319097619999,15.2,-3.30245147300001));
#183219=CARTESIAN_POINT('Ctrl Pts',(10.3319097619999,11.6,-3.30245147300001));
#183220=CARTESIAN_POINT('Ctrl Pts',(10.3296622669999,15.2,-3.30085747200001));
#183221=CARTESIAN_POINT('Ctrl Pts',(10.3296622669999,11.6,-3.30085747200001));
#183222=CARTESIAN_POINT('Ctrl Pts',(10.3274181339999,15.2,-3.29926868600001));
#183223=CARTESIAN_POINT('Ctrl Pts',(10.3274181339999,11.6,-3.29926868600001));
#183224=CARTESIAN_POINT('Ctrl Pts',(10.3251773799999,15.2,-3.29768511400002));
#183225=CARTESIAN_POINT('Ctrl Pts',(10.3251773799999,11.6,-3.29768511400002));
#183226=CARTESIAN_POINT('Ctrl Pts',(10.3229400139999,15.2,-3.29610675500001));
#183227=CARTESIAN_POINT('Ctrl Pts',(10.3229400139999,11.6,-3.29610675500001));
#183228=CARTESIAN_POINT('Ctrl Pts',(10.3207060529999,15.2,-3.29453360900001));
#183229=CARTESIAN_POINT('Ctrl Pts',(10.3207060529999,11.6,-3.29453360900001));
#183230=CARTESIAN_POINT('Ctrl Pts',(10.3184755079999,15.2,-3.29296567500001));
#183231=CARTESIAN_POINT('Ctrl Pts',(10.3184755079999,11.6,-3.29296567500002));
#183232=CARTESIAN_POINT('Ctrl Pts',(10.3162483959999,15.2,-3.29140295300002));
#183233=CARTESIAN_POINT('Ctrl Pts',(10.3162483959999,11.6,-3.29140295300002));
#183234=CARTESIAN_POINT('Ctrl Pts',(10.3140247269999,15.2,-3.28984544000001));
#183235=CARTESIAN_POINT('Ctrl Pts',(10.3140247269999,11.6,-3.28984544000001));
#183236=CARTESIAN_POINT('Ctrl Pts',(10.3118045179999,15.2,-3.28829313800002));
#183237=CARTESIAN_POINT('Ctrl Pts',(10.3118045179999,11.6,-3.28829313800002));
#183238=CARTESIAN_POINT('Ctrl Pts',(10.3095877799999,15.2,-3.28674604500002));
#183239=CARTESIAN_POINT('Ctrl Pts',(10.3095877799999,11.6,-3.28674604500002));
#183240=CARTESIAN_POINT('Ctrl Pts',(10.3073745299999,15.2,-3.28520415900002));
#183241=CARTESIAN_POINT('Ctrl Pts',(10.3073745299999,11.6,-3.28520415900002));
#183242=CARTESIAN_POINT('Ctrl Pts',(10.3051647789999,15.2,-3.28366748100001));
#183243=CARTESIAN_POINT('Ctrl Pts',(10.3051647789999,11.6,-3.28366748100001));
#183244=CARTESIAN_POINT('Ctrl Pts',(10.3029585419999,15.2,-3.28213601000002));
#183245=CARTESIAN_POINT('Ctrl Pts',(10.3029585419999,11.6,-3.28213601000002));
#183246=CARTESIAN_POINT('Ctrl Pts',(10.3007558329999,15.2,-3.28060974400001));
#183247=CARTESIAN_POINT('Ctrl Pts',(10.3007558329999,11.6,-3.28060974400001));
#183248=CARTESIAN_POINT('Ctrl Pts',(10.2985566669999,15.2,-3.27908868400002));
#183249=CARTESIAN_POINT('Ctrl Pts',(10.2985566669999,11.6,-3.27908868400002));
#183250=CARTESIAN_POINT('Ctrl Pts',(10.2963610559999,15.2,-3.27757282800002));
#183251=CARTESIAN_POINT('Ctrl Pts',(10.2963610559999,11.6,-3.27757282800002));
#183252=CARTESIAN_POINT('Ctrl Pts',(10.2941690149999,15.2,-3.27606217500001));
#183253=CARTESIAN_POINT('Ctrl Pts',(10.2941690149999,11.6,-3.27606217500001));
#183254=CARTESIAN_POINT('Ctrl Pts',(10.2919805579999,15.2,-3.27455672400002));
#183255=CARTESIAN_POINT('Ctrl Pts',(10.2919805579999,11.6,-3.27455672400002));
#183256=CARTESIAN_POINT('Ctrl Pts',(10.2897957009999,15.2,-3.27305647500001));
#183257=CARTESIAN_POINT('Ctrl Pts',(10.2897957009999,11.6,-3.27305647500001));
#183258=CARTESIAN_POINT('Ctrl Pts',(10.2876144549999,15.2,-3.27156142700002));
#183259=CARTESIAN_POINT('Ctrl Pts',(10.2876144549999,11.6,-3.27156142700002));
#183260=CARTESIAN_POINT('Ctrl Pts',(10.2854368349999,15.2,-3.27007157800002));
#183261=CARTESIAN_POINT('Ctrl Pts',(10.2854368349999,11.6,-3.27007157800002));
#183262=CARTESIAN_POINT('Ctrl Pts',(10.2832628569999,15.2,-3.26858692800001));
#183263=CARTESIAN_POINT('Ctrl Pts',(10.2832628569999,11.6,-3.26858692800002));
#183264=CARTESIAN_POINT('Ctrl Pts',(10.2810925339999,15.2,-3.26710747600002));
#183265=CARTESIAN_POINT('Ctrl Pts',(10.2810925339999,11.6,-3.26710747600002));
#183266=CARTESIAN_POINT('Ctrl Pts',(10.2789258799999,15.2,-3.26563322100001));
#183267=CARTESIAN_POINT('Ctrl Pts',(10.2789258799999,11.6,-3.26563322100002));
#183268=CARTESIAN_POINT('Ctrl Pts',(10.2767629099999,15.2,-3.26416416200002));
#183269=CARTESIAN_POINT('Ctrl Pts',(10.2767629099999,11.6,-3.26416416200002));
#183270=CARTESIAN_POINT('Ctrl Pts',(10.2746036379999,15.2,-3.26270029800002));
#183271=CARTESIAN_POINT('Ctrl Pts',(10.2746036379999,11.6,-3.26270029800002));
#183272=CARTESIAN_POINT('Ctrl Pts',(10.2724480789999,15.2,-3.26124162800001));
#183273=CARTESIAN_POINT('Ctrl Pts',(10.2724480789999,11.6,-3.26124162800001));
#183274=CARTESIAN_POINT('Ctrl Pts',(10.2702962469999,15.2,-3.25978815000001));
#183275=CARTESIAN_POINT('Ctrl Pts',(10.2702962469999,11.6,-3.25978815000001));
#183276=CARTESIAN_POINT('Ctrl Pts',(10.2681481549999,15.2,-3.25833986600002));
#183277=CARTESIAN_POINT('Ctrl Pts',(10.2681481549999,11.6,-3.25833986600002));
#183278=CARTESIAN_POINT('Ctrl Pts',(10.2660038209999,15.2,-3.25689677200002));
#183279=CARTESIAN_POINT('Ctrl Pts',(10.2660038209999,11.6,-3.25689677200002));
#183280=CARTESIAN_POINT('Ctrl Pts',(10.2638632559999,15.2,-3.25545886800001));
#183281=CARTESIAN_POINT('Ctrl Pts',(10.2638632559999,11.6,-3.25545886800001));
#183282=CARTESIAN_POINT('Ctrl Pts',(10.2617264769999,15.2,-3.25402615300002));
#183283=CARTESIAN_POINT('Ctrl Pts',(10.2617264769999,11.6,-3.25402615300002));
#183284=CARTESIAN_POINT('Ctrl Pts',(10.2595934979999,15.2,-3.25259862700001));
#183285=CARTESIAN_POINT('Ctrl Pts',(10.2595934979999,11.6,-3.25259862700001));
#183286=CARTESIAN_POINT('Ctrl Pts',(10.2574643339999,15.2,-3.25117628600001));
#183287=CARTESIAN_POINT('Ctrl Pts',(10.2574643339999,11.6,-3.25117628600002));
#183288=CARTESIAN_POINT('Ctrl Pts',(10.2553389979999,15.2,-3.24975913200001));
#183289=CARTESIAN_POINT('Ctrl Pts',(10.2553389979999,11.6,-3.24975913200001));
#183290=CARTESIAN_POINT('Ctrl Pts',(10.2532175069999,15.2,-3.24834716200002));
#183291=CARTESIAN_POINT('Ctrl Pts',(10.2532175069999,11.6,-3.24834716200002));
#183292=CARTESIAN_POINT('Ctrl Pts',(10.2510998739999,15.2,-3.24694037600001));
#183293=CARTESIAN_POINT('Ctrl Pts',(10.2510998739999,11.6,-3.24694037600001));
#183294=CARTESIAN_POINT('Ctrl Pts',(10.2489861149999,15.2,-3.24553877200001));
#183295=CARTESIAN_POINT('Ctrl Pts',(10.2489861149999,11.6,-3.24553877200001));
#183296=CARTESIAN_POINT('Ctrl Pts',(10.2468762449999,15.2,-3.24414235000001));
#183297=CARTESIAN_POINT('Ctrl Pts',(10.2468762449999,11.6,-3.24414235000001));
#183298=CARTESIAN_POINT('Ctrl Pts',(10.2447702779999,15.2,-3.24275110800002));
#183299=CARTESIAN_POINT('Ctrl Pts',(10.2447702779999,11.6,-3.24275110800002));
#183300=CARTESIAN_POINT('Ctrl Pts',(10.2426682289999,15.2,-3.24136504400002));
#183301=CARTESIAN_POINT('Ctrl Pts',(10.2426682289999,11.6,-3.24136504400002));
#183302=CARTESIAN_POINT('Ctrl Pts',(10.2405701139999,15.2,-3.23998415800002));
#183303=CARTESIAN_POINT('Ctrl Pts',(10.2405701139999,11.6,-3.23998415800002));
#183304=CARTESIAN_POINT('Ctrl Pts',(10.2384759469999,15.2,-3.23860844800001));
#183305=CARTESIAN_POINT('Ctrl Pts',(10.2384759469999,11.6,-3.23860844800001));
#183306=CARTESIAN_POINT('Ctrl Pts',(10.2363857439999,15.2,-3.23723791500001));
#183307=CARTESIAN_POINT('Ctrl Pts',(10.2363857439999,11.6,-3.23723791500001));
#183308=CARTESIAN_POINT('Ctrl Pts',(10.2342995189999,15.2,-3.23587255500001));
#183309=CARTESIAN_POINT('Ctrl Pts',(10.2342995189999,11.6,-3.23587255500001));
#183310=CARTESIAN_POINT('Ctrl Pts',(10.2322172889999,15.2,-3.23451236800001));
#183311=CARTESIAN_POINT('Ctrl Pts',(10.2322172889999,11.6,-3.23451236800001));
#183312=CARTESIAN_POINT('Ctrl Pts',(10.2301390659999,15.2,-3.23315735300001));
#183313=CARTESIAN_POINT('Ctrl Pts',(10.2301390659999,11.6,-3.23315735300001));
#183314=CARTESIAN_POINT('Ctrl Pts',(10.2280648689999,15.2,-3.23180750800002));
#183315=CARTESIAN_POINT('Ctrl Pts',(10.2280648689999,11.6,-3.23180750800002));
#183316=CARTESIAN_POINT('Ctrl Pts',(10.2259947109999,15.2,-3.23046283300001));
#183317=CARTESIAN_POINT('Ctrl Pts',(10.2259947109999,11.6,-3.23046283300001));
#183318=CARTESIAN_POINT('Ctrl Pts',(10.2239286079999,15.2,-3.22912332500001));
#183319=CARTESIAN_POINT('Ctrl Pts',(10.2239286079999,11.6,-3.22912332500001));
#183320=CARTESIAN_POINT('Ctrl Pts',(10.2218665749999,15.2,-3.22778898400002));
#183321=CARTESIAN_POINT('Ctrl Pts',(10.2218665749999,11.6,-3.22778898400002));
#183322=CARTESIAN_POINT('Ctrl Pts',(10.2198086269999,15.2,-3.22645980700001));
#183323=CARTESIAN_POINT('Ctrl Pts',(10.2198086269999,11.6,-3.22645980700001));
#183324=CARTESIAN_POINT('Ctrl Pts',(10.2177547809999,15.2,-3.22513579400002));
#183325=CARTESIAN_POINT('Ctrl Pts',(10.2177547809999,11.6,-3.22513579400002));
#183326=CARTESIAN_POINT('Ctrl Pts',(10.2157050509999,15.2,-3.22381694500002));
#183327=CARTESIAN_POINT('Ctrl Pts',(10.2157050509999,11.6,-3.22381694500002));
#183328=CARTESIAN_POINT('Ctrl Pts',(10.2136594529999,15.2,-3.22250325600002));
#183329=CARTESIAN_POINT('Ctrl Pts',(10.2136594529999,11.6,-3.22250325600002));
#183330=CARTESIAN_POINT('Ctrl Pts',(10.2116180039999,15.2,-3.22119472700001));
#183331=CARTESIAN_POINT('Ctrl Pts',(10.2116180039999,11.6,-3.22119472700001));
#183332=CARTESIAN_POINT('Ctrl Pts',(10.2095807169999,15.2,-3.21989135600001));
#183333=CARTESIAN_POINT('Ctrl Pts',(10.2095807169999,11.6,-3.21989135600001));
#183334=CARTESIAN_POINT('Ctrl Pts',(10.2075476089999,15.2,-3.21859314200001));
#183335=CARTESIAN_POINT('Ctrl Pts',(10.2075476089999,11.6,-3.21859314200002));
#183336=CARTESIAN_POINT('Ctrl Pts',(10.2055186959999,15.2,-3.21730008500001));
#183337=CARTESIAN_POINT('Ctrl Pts',(10.2055186959999,11.6,-3.21730008500001));
#183338=CARTESIAN_POINT('Ctrl Pts',(10.2034939929999,15.2,-3.21601218000001));
#183339=CARTESIAN_POINT('Ctrl Pts',(10.2034939929999,11.6,-3.21601218000001));
#183340=CARTESIAN_POINT('Ctrl Pts',(10.2014735169999,15.2,-3.21472942900002));
#183341=CARTESIAN_POINT('Ctrl Pts',(10.2014735169999,11.6,-3.21472942900002));
#183342=CARTESIAN_POINT('Ctrl Pts',(10.1994572829999,15.2,-3.21345182800002));
#183343=CARTESIAN_POINT('Ctrl Pts',(10.1994572829999,11.6,-3.21345182800002));
#183344=CARTESIAN_POINT('Ctrl Pts',(10.1974453069999,15.2,-3.21217937700002));
#183345=CARTESIAN_POINT('Ctrl Pts',(10.1974453069999,11.6,-3.21217937700002));
#183346=CARTESIAN_POINT('Ctrl Pts',(10.1954376039999,15.2,-3.21091207400002));
#183347=CARTESIAN_POINT('Ctrl Pts',(10.1954376039999,11.6,-3.21091207400002));
#183348=CARTESIAN_POINT('Ctrl Pts',(10.1934341909999,15.2,-3.20964991800002));
#183349=CARTESIAN_POINT('Ctrl Pts',(10.1934341909999,11.6,-3.20964991800002));
#183350=CARTESIAN_POINT('Ctrl Pts',(10.1914350849999,15.2,-3.20839290800001));
#183351=CARTESIAN_POINT('Ctrl Pts',(10.1914350849999,11.6,-3.20839290800001));
#183352=CARTESIAN_POINT('Ctrl Pts',(10.1894402999999,15.2,-3.20714104000002));
#183353=CARTESIAN_POINT('Ctrl Pts',(10.1894402999999,11.6,-3.20714104000002));
#183354=CARTESIAN_POINT('Ctrl Pts',(10.1874498539999,15.2,-3.20589431400002));
#183355=CARTESIAN_POINT('Ctrl Pts',(10.1874498539999,11.6,-3.20589431400002));
#183356=CARTESIAN_POINT('Ctrl Pts',(10.1854637609999,15.2,-3.20465272900002));
#183357=CARTESIAN_POINT('Ctrl Pts',(10.1854637609999,11.6,-3.20465272900002));
#183358=CARTESIAN_POINT('Ctrl Pts',(10.1834820399999,15.2,-3.20341628300001));
#183359=CARTESIAN_POINT('Ctrl Pts',(10.1834820399999,11.6,-3.20341628300001));
#183360=CARTESIAN_POINT('Ctrl Pts',(10.1815047049999,15.2,-3.20218497500001));
#183361=CARTESIAN_POINT('Ctrl Pts',(10.1815047049999,11.6,-3.20218497500001));
#183362=CARTESIAN_POINT('Ctrl Pts',(10.1795317729999,15.2,-3.20095880100002));
#183363=CARTESIAN_POINT('Ctrl Pts',(10.1795317729999,11.6,-3.20095880100002));
#183364=CARTESIAN_POINT('Ctrl Pts',(10.1775632609999,15.2,-3.19973776100001));
#183365=CARTESIAN_POINT('Ctrl Pts',(10.1775632609999,11.6,-3.19973776100001));
#183366=CARTESIAN_POINT('Ctrl Pts',(10.1755991829999,15.2,-3.19852185400002));
#183367=CARTESIAN_POINT('Ctrl Pts',(10.1755991829999,11.6,-3.19852185400002));
#183368=CARTESIAN_POINT('Ctrl Pts',(10.1736395589999,15.2,-3.19731107700001));
#183369=CARTESIAN_POINT('Ctrl Pts',(10.1736395589999,11.6,-3.19731107700001));
#183370=CARTESIAN_POINT('Ctrl Pts',(10.1716844029999,15.2,-3.19610542900001));
#183371=CARTESIAN_POINT('Ctrl Pts',(10.1716844029999,11.6,-3.19610542900001));
#183372=CARTESIAN_POINT('Ctrl Pts',(10.1697337309999,15.2,-3.19490490900002));
#183373=CARTESIAN_POINT('Ctrl Pts',(10.1697337309999,11.6,-3.19490490900002));
#183374=CARTESIAN_POINT('Ctrl Pts',(10.1677875629999,15.2,-3.19370951400002));
#183375=CARTESIAN_POINT('Ctrl Pts',(10.1677875629999,11.6,-3.19370951400002));
#183376=CARTESIAN_POINT('Ctrl Pts',(10.1658459129999,15.2,-3.19251924300001));
#183377=CARTESIAN_POINT('Ctrl Pts',(10.1658459129999,11.6,-3.19251924300001));
#183378=CARTESIAN_POINT('Ctrl Pts',(10.1639087969999,15.2,-3.19133409300001));
#183379=CARTESIAN_POINT('Ctrl Pts',(10.1639087969999,11.6,-3.19133409300001));
#183380=CARTESIAN_POINT('Ctrl Pts',(10.1619762339999,15.2,-3.19015406500001));
#183381=CARTESIAN_POINT('Ctrl Pts',(10.1619762339999,11.6,-3.19015406500002));
#183382=CARTESIAN_POINT('Ctrl Pts',(10.1600482389999,15.2,-3.18897915400001));
#183383=CARTESIAN_POINT('Ctrl Pts',(10.1600482389999,11.6,-3.18897915400001));
#183384=CARTESIAN_POINT('Ctrl Pts',(10.1581248299999,15.2,-3.18780935900001));
#183385=CARTESIAN_POINT('Ctrl Pts',(10.1581248299999,11.6,-3.18780935900001));
#183386=CARTESIAN_POINT('Ctrl Pts',(10.1562060229999,15.2,-3.18664468000001));
#183387=CARTESIAN_POINT('Ctrl Pts',(10.1562060229999,11.6,-3.18664468000002));
#183388=CARTESIAN_POINT('Ctrl Pts',(10.1542918349999,15.2,-3.18548511300001));
#183389=CARTESIAN_POINT('Ctrl Pts',(10.1542918349999,11.6,-3.18548511300001));
#183390=CARTESIAN_POINT('Ctrl Pts',(10.1523822839999,15.2,-3.18433065800001));
#183391=CARTESIAN_POINT('Ctrl Pts',(10.1523822839999,11.6,-3.18433065800001));
#183392=CARTESIAN_POINT('Ctrl Pts',(10.1504773859999,15.2,-3.18318131200002));
#183393=CARTESIAN_POINT('Ctrl Pts',(10.1504773859999,11.6,-3.18318131200002));
#183394=CARTESIAN_POINT('Ctrl Pts',(10.1485771589999,15.2,-3.18203707400002));
#183395=CARTESIAN_POINT('Ctrl Pts',(10.1485771589999,11.6,-3.18203707400002));
#183396=CARTESIAN_POINT('Ctrl Pts',(10.1466816179999,15.2,-3.18089793900001));
#183397=CARTESIAN_POINT('Ctrl Pts',(10.1466816179999,11.6,-3.18089793900001));
#183398=CARTESIAN_POINT('Ctrl Pts',(10.1447907829999,15.2,-3.17976391000002));
#183399=CARTESIAN_POINT('Ctrl Pts',(10.1447907829999,11.6,-3.17976391000002));
#183400=CARTESIAN_POINT('Ctrl Pts',(10.1429046699999,15.2,-3.17863498200001));
#183401=CARTESIAN_POINT('Ctrl Pts',(10.1429046699999,11.6,-3.17863498200001));
#183402=CARTESIAN_POINT('Ctrl Pts',(10.1410232959999,15.2,-3.17751115200001));
#183403=CARTESIAN_POINT('Ctrl Pts',(10.1410232959999,11.6,-3.17751115200001));
#183404=CARTESIAN_POINT('Ctrl Pts',(10.1391466789999,15.2,-3.17639242200002));
#183405=CARTESIAN_POINT('Ctrl Pts',(10.1391466789999,11.6,-3.17639242200002));
#183406=CARTESIAN_POINT('Ctrl Pts',(10.1372748349999,15.2,-3.17527878600002));
#183407=CARTESIAN_POINT('Ctrl Pts',(10.1372748349999,11.6,-3.17527878600002));
#183408=CARTESIAN_POINT('Ctrl Pts',(10.1354077839999,15.2,-3.17417024400001));
#183409=CARTESIAN_POINT('Ctrl Pts',(10.1354077839999,11.6,-3.17417024400001));
#183410=CARTESIAN_POINT('Ctrl Pts',(10.1335455409999,15.2,-3.17306679400001));
#183411=CARTESIAN_POINT('Ctrl Pts',(10.1335455409999,11.6,-3.17306679400002));
#183412=CARTESIAN_POINT('Ctrl Pts',(10.1316881249999,15.2,-3.17196843300001));
#183413=CARTESIAN_POINT('Ctrl Pts',(10.1316881249999,11.6,-3.17196843300001));
#183414=CARTESIAN_POINT('Ctrl Pts',(10.1298355529999,15.2,-3.17087516000001));
#183415=CARTESIAN_POINT('Ctrl Pts',(10.1298355529999,11.6,-3.17087516000001));
#183416=CARTESIAN_POINT('Ctrl Pts',(10.1279878419999,15.2,-3.16978697100001));
#183417=CARTESIAN_POINT('Ctrl Pts',(10.1279878419999,11.6,-3.16978697100002));
#183418=CARTESIAN_POINT('Ctrl Pts',(10.1261450119999,15.2,-3.16870386600002));
#183419=CARTESIAN_POINT('Ctrl Pts',(10.1261450119999,11.6,-3.16870386600002));
#183420=CARTESIAN_POINT('Ctrl Pts',(10.1243070779999,15.2,-3.16762584300001));
#183421=CARTESIAN_POINT('Ctrl Pts',(10.1243070779999,11.6,-3.16762584300002));
#183422=CARTESIAN_POINT('Ctrl Pts',(10.1224740599999,15.2,-3.16655289800002));
#183423=CARTESIAN_POINT('Ctrl Pts',(10.1224740599999,11.6,-3.16655289800002));
#183424=CARTESIAN_POINT('Ctrl Pts',(10.1206459739999,15.2,-3.16548503000002));
#183425=CARTESIAN_POINT('Ctrl Pts',(10.1206459739999,11.6,-3.16548503000002));
#183426=CARTESIAN_POINT('Ctrl Pts',(10.1188228389999,15.2,-3.16442223800002));
#183427=CARTESIAN_POINT('Ctrl Pts',(10.1188228389999,11.6,-3.16442223800002));
#183428=CARTESIAN_POINT('Ctrl Pts',(10.1170046749999,15.2,-3.16336451600002));
#183429=CARTESIAN_POINT('Ctrl Pts',(10.1170046749999,11.6,-3.16336451600002));
#183430=CARTESIAN_POINT('Ctrl Pts',(10.1151914959999,15.2,-3.16231186600001));
#183431=CARTESIAN_POINT('Ctrl Pts',(10.1151914959999,11.6,-3.16231186600001));
#183432=CARTESIAN_POINT('Ctrl Pts',(10.1133833219999,15.2,-3.16126428300001));
#183433=CARTESIAN_POINT('Ctrl Pts',(10.1133833219999,11.6,-3.16126428300001));
#183434=CARTESIAN_POINT('Ctrl Pts',(10.1115801729999,15.2,-3.16022176700002));
#183435=CARTESIAN_POINT('Ctrl Pts',(10.1115801729999,11.6,-3.16022176700002));
#183436=CARTESIAN_POINT('Ctrl Pts',(10.1097820639999,15.2,-3.15918431300001));
#183437=CARTESIAN_POINT('Ctrl Pts',(10.1097820639999,11.6,-3.15918431300001));
#183438=CARTESIAN_POINT('Ctrl Pts',(10.1079890159999,15.2,-3.15815192100001));
#183439=CARTESIAN_POINT('Ctrl Pts',(10.1079890159999,11.6,-3.15815192100001));
#183440=CARTESIAN_POINT('Ctrl Pts',(10.1062010459999,15.2,-3.15712458800002));
#183441=CARTESIAN_POINT('Ctrl Pts',(10.1062010459999,11.6,-3.15712458800002));
#183442=CARTESIAN_POINT('Ctrl Pts',(10.1044181719999,15.2,-3.15610231100001));
#183443=CARTESIAN_POINT('Ctrl Pts',(10.1044181719999,11.6,-3.15610231100001));
#183444=CARTESIAN_POINT('Ctrl Pts',(10.1026404129999,15.2,-3.15508509000002));
#183445=CARTESIAN_POINT('Ctrl Pts',(10.1026404129999,11.6,-3.15508509000002));
#183446=CARTESIAN_POINT('Ctrl Pts',(10.1008677879999,15.2,-3.15407291900001));
#183447=CARTESIAN_POINT('Ctrl Pts',(10.1008677879999,11.6,-3.15407291900002));
#183448=CARTESIAN_POINT('Ctrl Pts',(10.0991003149999,15.2,-3.15306579700001));
#183449=CARTESIAN_POINT('Ctrl Pts',(10.0991003149999,11.6,-3.15306579700001));
#183450=CARTESIAN_POINT('Ctrl Pts',(10.0973380129999,15.2,-3.15206372300001));
#183451=CARTESIAN_POINT('Ctrl Pts',(10.0973380129999,11.6,-3.15206372300001));
#183452=CARTESIAN_POINT('Ctrl Pts',(10.0955808999999,15.2,-3.15106669300001));
#183453=CARTESIAN_POINT('Ctrl Pts',(10.0955808999999,11.6,-3.15106669300001));
#183454=CARTESIAN_POINT('Ctrl Pts',(10.0938289959999,15.2,-3.15007470700001));
#183455=CARTESIAN_POINT('Ctrl Pts',(10.0938289959999,11.6,-3.15007470700001));
#183456=CARTESIAN_POINT('Ctrl Pts',(10.0920823179999,15.2,-3.14908775800002));
#183457=CARTESIAN_POINT('Ctrl Pts',(10.0920823179999,11.6,-3.14908775800002));
#183458=CARTESIAN_POINT('Ctrl Pts',(10.0903408869999,15.2,-3.14810584800002));
#183459=CARTESIAN_POINT('Ctrl Pts',(10.0903408869999,11.6,-3.14810584800002));
#183460=CARTESIAN_POINT('Ctrl Pts',(10.0886047199999,15.2,-3.14712897300002));
#183461=CARTESIAN_POINT('Ctrl Pts',(10.0886047199999,11.6,-3.14712897300002));
#183462=CARTESIAN_POINT('Ctrl Pts',(10.0868738369999,15.2,-3.14615712900002));
#183463=CARTESIAN_POINT('Ctrl Pts',(10.0868738369999,11.6,-3.14615712900002));
#183464=CARTESIAN_POINT('Ctrl Pts',(10.0851482559999,15.2,-3.14519031400001));
#183465=CARTESIAN_POINT('Ctrl Pts',(10.0851482559999,11.6,-3.14519031400002));
#183466=CARTESIAN_POINT('Ctrl Pts',(10.0834279989999,15.2,-3.14422852800002));
#183467=CARTESIAN_POINT('Ctrl Pts',(10.0834279989999,11.6,-3.14422852800002));
#183468=CARTESIAN_POINT('Ctrl Pts',(10.0817130829999,15.2,-3.14327176500001));
#183469=CARTESIAN_POINT('Ctrl Pts',(10.0817130829999,11.6,-3.14327176500001));
#183470=CARTESIAN_POINT('Ctrl Pts',(10.0800035259999,15.2,-3.14232002500002));
#183471=CARTESIAN_POINT('Ctrl Pts',(10.0800035259999,11.6,-3.14232002500002));
#183472=CARTESIAN_POINT('Ctrl Pts',(10.0782993499999,15.2,-3.14137330300001));
#183473=CARTESIAN_POINT('Ctrl Pts',(10.0782993499999,11.6,-3.14137330300001));
#183474=CARTESIAN_POINT('Ctrl Pts',(10.0766005729999,15.2,-3.14043159900002));
#183475=CARTESIAN_POINT('Ctrl Pts',(10.0766005729999,11.6,-3.14043159900002));
#183476=CARTESIAN_POINT('Ctrl Pts',(10.0749072159999,15.2,-3.13949490700002));
#183477=CARTESIAN_POINT('Ctrl Pts',(10.0749072159999,11.6,-3.13949490700002));
#183478=CARTESIAN_POINT('Ctrl Pts',(10.0732192959999,15.2,-3.13856322800001));
#183479=CARTESIAN_POINT('Ctrl Pts',(10.0732192959999,11.6,-3.13856322800001));
#183480=CARTESIAN_POINT('Ctrl Pts',(10.0715368339999,15.2,-3.13763655600001));
#183481=CARTESIAN_POINT('Ctrl Pts',(10.0715368339999,11.6,-3.13763655600001));
#183482=CARTESIAN_POINT('Ctrl Pts',(10.0698598489999,15.2,-3.13671489000001));
#183483=CARTESIAN_POINT('Ctrl Pts',(10.0698598489999,11.6,-3.13671489000001));
#183484=CARTESIAN_POINT('Ctrl Pts',(10.0681883619999,15.2,-3.13579822800001));
#183485=CARTESIAN_POINT('Ctrl Pts',(10.0681883619999,11.6,-3.13579822800001));
#183486=CARTESIAN_POINT('Ctrl Pts',(10.0665223919999,15.2,-3.13488656500001));
#183487=CARTESIAN_POINT('Ctrl Pts',(10.0665223919999,11.6,-3.13488656500002));
#183488=CARTESIAN_POINT('Ctrl Pts',(10.0648619579999,15.2,-3.13397990000002));
#183489=CARTESIAN_POINT('Ctrl Pts',(10.0648619579999,11.6,-3.13397990000002));
#183490=CARTESIAN_POINT('Ctrl Pts',(10.0632070809999,15.2,-3.13307822900001));
#183491=CARTESIAN_POINT('Ctrl Pts',(10.0632070809999,11.6,-3.13307822900002));
#183492=CARTESIAN_POINT('Ctrl Pts',(10.0615577799999,15.2,-3.13218155100001));
#183493=CARTESIAN_POINT('Ctrl Pts',(10.0615577799999,11.6,-3.13218155100001));
#183494=CARTESIAN_POINT('Ctrl Pts',(10.0599140779999,15.2,-3.13128986000001));
#183495=CARTESIAN_POINT('Ctrl Pts',(10.0599140779999,11.6,-3.13128986000002));
#183496=CARTESIAN_POINT('Ctrl Pts',(10.0582759909999,15.2,-3.13040315700002));
#183497=CARTESIAN_POINT('Ctrl Pts',(10.0582759909999,11.6,-3.13040315700002));
#183498=CARTESIAN_POINT('Ctrl Pts',(10.0566435409999,15.2,-3.12952143500001));
#183499=CARTESIAN_POINT('Ctrl Pts',(10.0566435409999,11.6,-3.12952143500001));
#183500=CARTESIAN_POINT('Ctrl Pts',(10.0550167499999,15.2,-3.12864469400001));
#183501=CARTESIAN_POINT('Ctrl Pts',(10.0550167499999,11.6,-3.12864469400001));
#183502=CARTESIAN_POINT('Ctrl Pts',(10.0533956349999,15.2,-3.12777293000002));
#183503=CARTESIAN_POINT('Ctrl Pts',(10.0533956349999,11.6,-3.12777293000002));
#183504=CARTESIAN_POINT('Ctrl Pts',(10.0517802179999,15.2,-3.12690614000001));
#183505=CARTESIAN_POINT('Ctrl Pts',(10.0517802179999,11.6,-3.12690614000001));
#183506=CARTESIAN_POINT('Ctrl Pts',(10.0501705219999,15.2,-3.12604432200001));
#183507=CARTESIAN_POINT('Ctrl Pts',(10.0501705219999,11.6,-3.12604432200001));
#183508=CARTESIAN_POINT('Ctrl Pts',(10.0485665629999,15.2,-3.12518747000002));
#183509=CARTESIAN_POINT('Ctrl Pts',(10.0485665629999,11.6,-3.12518747000002));
#183510=CARTESIAN_POINT('Ctrl Pts',(10.0469683629999,15.2,-3.12433558500001));
#183511=CARTESIAN_POINT('Ctrl Pts',(10.0469683629999,11.6,-3.12433558500001));
#183512=CARTESIAN_POINT('Ctrl Pts',(10.0453759449999,15.2,-3.12348866100002));
#183513=CARTESIAN_POINT('Ctrl Pts',(10.0453759449999,11.6,-3.12348866100002));
#183514=CARTESIAN_POINT('Ctrl Pts',(10.0437893269999,15.2,-3.12264669700001));
#183515=CARTESIAN_POINT('Ctrl Pts',(10.0437893269999,11.6,-3.12264669700001));
#183516=CARTESIAN_POINT('Ctrl Pts',(10.0422085329999,15.2,-3.12180968700002));
#183517=CARTESIAN_POINT('Ctrl Pts',(10.0422085329999,11.6,-3.12180968700002));
#183518=CARTESIAN_POINT('Ctrl Pts',(10.0406335799999,15.2,-3.12097763100001));
#183519=CARTESIAN_POINT('Ctrl Pts',(10.0406335799999,11.6,-3.12097763100002));
#183520=CARTESIAN_POINT('Ctrl Pts',(10.0390644919999,15.2,-3.12015052400001));
#183521=CARTESIAN_POINT('Ctrl Pts',(10.0390644919999,11.6,-3.12015052400001));
#183522=CARTESIAN_POINT('Ctrl Pts',(10.0375012879999,15.2,-3.11932836300001));
#183523=CARTESIAN_POINT('Ctrl Pts',(10.0375012879999,11.6,-3.11932836300001));
#183524=CARTESIAN_POINT('Ctrl Pts',(10.0359439909999,15.2,-3.11851114600001));
#183525=CARTESIAN_POINT('Ctrl Pts',(10.0359439909999,11.6,-3.11851114600001));
#183526=CARTESIAN_POINT('Ctrl Pts',(10.0343926209999,15.2,-3.11769886700001));
#183527=CARTESIAN_POINT('Ctrl Pts',(10.0343926209999,11.6,-3.11769886700001));
#183528=CARTESIAN_POINT('Ctrl Pts',(10.0328471999999,15.2,-3.11689152500001));
#183529=CARTESIAN_POINT('Ctrl Pts',(10.0328471999999,11.6,-3.11689152500001));
#183530=CARTESIAN_POINT('Ctrl Pts',(10.0313077479999,15.2,-3.11608911700001));
#183531=CARTESIAN_POINT('Ctrl Pts',(10.0313077479999,11.6,-3.11608911700001));
#183532=CARTESIAN_POINT('Ctrl Pts',(10.0297742879999,15.2,-3.11529163800001));
#183533=CARTESIAN_POINT('Ctrl Pts',(10.0297742879999,11.6,-3.11529163800001));
#183534=CARTESIAN_POINT('Ctrl Pts',(10.0282468409999,15.2,-3.11449908600002));
#183535=CARTESIAN_POINT('Ctrl Pts',(10.0282468409999,11.6,-3.11449908600002));
#183536=CARTESIAN_POINT('Ctrl Pts',(10.0267254279999,15.2,-3.11371145700001));
#183537=CARTESIAN_POINT('Ctrl Pts',(10.0267254279999,11.6,-3.11371145700001));
#183538=CARTESIAN_POINT('Ctrl Pts',(10.0252100719999,15.2,-3.11292874700001));
#183539=CARTESIAN_POINT('Ctrl Pts',(10.0252100719999,11.6,-3.11292874700001));
#183540=CARTESIAN_POINT('Ctrl Pts',(10.0237007949999,15.2,-3.11215095500001));
#183541=CARTESIAN_POINT('Ctrl Pts',(10.0237007949999,11.6,-3.11215095500002));
#183542=CARTESIAN_POINT('Ctrl Pts',(10.0221976149999,15.2,-3.11137807500002));
#183543=CARTESIAN_POINT('Ctrl Pts',(10.0221976149999,11.6,-3.11137807500002));
#183544=CARTESIAN_POINT('Ctrl Pts',(10.0207005589999,15.2,-3.11061010400001));
#183545=CARTESIAN_POINT('Ctrl Pts',(10.0207005589999,11.6,-3.11061010400001));
#183546=CARTESIAN_POINT('Ctrl Pts',(10.0192096459999,15.2,-3.10984703900001));
#183547=CARTESIAN_POINT('Ctrl Pts',(10.0192096459999,11.6,-3.10984703900001));
#183548=CARTESIAN_POINT('Ctrl Pts',(10.0177248989999,15.2,-3.10908887700001));
#183549=CARTESIAN_POINT('Ctrl Pts',(10.0177248989999,11.6,-3.10908887700002));
#183550=CARTESIAN_POINT('Ctrl Pts',(10.0162463389999,15.2,-3.10833561400001));
#183551=CARTESIAN_POINT('Ctrl Pts',(10.0162463389999,11.6,-3.10833561400001));
#183552=CARTESIAN_POINT('Ctrl Pts',(10.0147739889999,15.2,-3.10758724500001));
#183553=CARTESIAN_POINT('Ctrl Pts',(10.0147739889999,11.6,-3.10758724500001));
#183554=CARTESIAN_POINT('Ctrl Pts',(10.0133078739999,15.2,-3.10684376900001));
#183555=CARTESIAN_POINT('Ctrl Pts',(10.0133078739999,11.6,-3.10684376900001));
#183556=CARTESIAN_POINT('Ctrl Pts',(10.0118480119999,15.2,-3.10610517900002));
#183557=CARTESIAN_POINT('Ctrl Pts',(10.0118480119999,11.6,-3.10610517900002));
#183558=CARTESIAN_POINT('Ctrl Pts',(10.0103944279999,15.2,-3.10537147600002));
#183559=CARTESIAN_POINT('Ctrl Pts',(10.0103944279999,11.6,-3.10537147600002));
#183560=CARTESIAN_POINT('Ctrl Pts',(10.0089471439999,15.2,-3.10464265200002));
#183561=CARTESIAN_POINT('Ctrl Pts',(10.0089471439999,11.6,-3.10464265200002));
#183562=CARTESIAN_POINT('Ctrl Pts',(10.0075061829999,15.2,-3.10391870500001));
#183563=CARTESIAN_POINT('Ctrl Pts',(10.0075061829999,11.6,-3.10391870500002));
#183564=CARTESIAN_POINT('Ctrl Pts',(10.0060715669999,15.2,-3.10319963200001));
#183565=CARTESIAN_POINT('Ctrl Pts',(10.0060715669999,11.6,-3.10319963200001));
#183566=CARTESIAN_POINT('Ctrl Pts',(10.0046433189999,15.2,-3.10248542800001));
#183567=CARTESIAN_POINT('Ctrl Pts',(10.0046433189999,11.6,-3.10248542800002));
#183568=CARTESIAN_POINT('Ctrl Pts',(10.0032214629999,15.2,-3.10177609000001));
#183569=CARTESIAN_POINT('Ctrl Pts',(10.0032214629999,11.6,-3.10177609000002));
#183570=CARTESIAN_POINT('Ctrl Pts',(10.0018060209999,15.2,-3.10107161300001));
#183571=CARTESIAN_POINT('Ctrl Pts',(10.0018060209999,11.6,-3.10107161300001));
#183572=CARTESIAN_POINT('Ctrl Pts',(10.0003970159999,15.2,-3.10037199500002));
#183573=CARTESIAN_POINT('Ctrl Pts',(10.0003970159999,11.6,-3.10037199500002));
#183574=CARTESIAN_POINT('Ctrl Pts',(9.99899447199994,15.2,-3.09967723100002));
#183575=CARTESIAN_POINT('Ctrl Pts',(9.99899447199994,11.6,-3.09967723100002));
#183576=CARTESIAN_POINT('Ctrl Pts',(9.99759841199995,15.2,-3.09898731700001));
#183577=CARTESIAN_POINT('Ctrl Pts',(9.99759841199995,11.6,-3.09898731700002));
#183578=CARTESIAN_POINT('Ctrl Pts',(9.99620885899994,15.2,-3.09830225000002));
#183579=CARTESIAN_POINT('Ctrl Pts',(9.99620885899994,11.6,-3.09830225000002));
#183580=CARTESIAN_POINT('Ctrl Pts',(9.99482583599995,15.2,-3.09762202400002));
#183581=CARTESIAN_POINT('Ctrl Pts',(9.99482583599995,11.6,-3.09762202400002));
#183582=CARTESIAN_POINT('Ctrl Pts',(9.99344936799995,15.2,-3.09694663700002));
#183583=CARTESIAN_POINT('Ctrl Pts',(9.99344936799995,11.6,-3.09694663700002));
#183584=CARTESIAN_POINT('Ctrl Pts',(9.99207947699994,15.2,-3.09627608500001));
#183585=CARTESIAN_POINT('Ctrl Pts',(9.99207947699994,11.6,-3.09627608500001));
#183586=CARTESIAN_POINT('Ctrl Pts',(9.99071618799995,15.2,-3.09561036200002));
#183587=CARTESIAN_POINT('Ctrl Pts',(9.99071618799995,11.6,-3.09561036200002));
#183588=CARTESIAN_POINT('Ctrl Pts',(9.98935952599994,15.2,-3.09494946600001));
#183589=CARTESIAN_POINT('Ctrl Pts',(9.98935952599994,11.6,-3.09494946600001));
#183590=CARTESIAN_POINT('Ctrl Pts',(9.98800951199994,15.2,-3.09429339200001));
#183591=CARTESIAN_POINT('Ctrl Pts',(9.98800951199994,11.6,-3.09429339200001));
#183592=CARTESIAN_POINT('Ctrl Pts',(9.98666617099994,15.2,-3.09364213600002));
#183593=CARTESIAN_POINT('Ctrl Pts',(9.98666617099994,11.6,-3.09364213600002));
#183594=CARTESIAN_POINT('Ctrl Pts',(9.98532952799994,15.2,-3.09299569400002));
#183595=CARTESIAN_POINT('Ctrl Pts',(9.98532952799994,11.6,-3.09299569400002));
#183596=CARTESIAN_POINT('Ctrl Pts',(9.98399960699994,15.2,-3.09235406000001));
#183597=CARTESIAN_POINT('Ctrl Pts',(9.98399960699994,11.6,-3.09235406000001));
#183598=CARTESIAN_POINT('Ctrl Pts',(9.98267643199994,15.2,-3.09171723300001));
#183599=CARTESIAN_POINT('Ctrl Pts',(9.98267643199994,11.6,-3.09171723300001));
#183600=CARTESIAN_POINT('Ctrl Pts',(9.98136002599994,15.2,-3.09108520600001));
#183601=CARTESIAN_POINT('Ctrl Pts',(9.98136002599994,11.6,-3.09108520600002));
#183602=CARTESIAN_POINT('Ctrl Pts',(9.98005041699994,15.2,-3.09045797700001));
#183603=CARTESIAN_POINT('Ctrl Pts',(9.98005041699994,11.6,-3.09045797700001));
#183604=CARTESIAN_POINT('Ctrl Pts',(9.97874762699994,15.2,-3.08983553900001));
#183605=CARTESIAN_POINT('Ctrl Pts',(9.97874762699994,11.6,-3.08983553900001));
#183606=CARTESIAN_POINT('Ctrl Pts',(9.97745168099994,15.2,-3.08921789100001));
#183607=CARTESIAN_POINT('Ctrl Pts',(9.97745168099994,11.6,-3.08921789100001));
#183608=CARTESIAN_POINT('Ctrl Pts',(9.97616260499995,15.2,-3.08860502500002));
#183609=CARTESIAN_POINT('Ctrl Pts',(9.97616260499995,11.6,-3.08860502500002));
#183610=CARTESIAN_POINT('Ctrl Pts',(9.97488042199994,15.2,-3.08799693900002));
#183611=CARTESIAN_POINT('Ctrl Pts',(9.97488042199994,11.6,-3.08799693900002));
#183612=CARTESIAN_POINT('Ctrl Pts',(9.97360515799994,15.2,-3.08739362900001));
#183613=CARTESIAN_POINT('Ctrl Pts',(9.97360515799994,11.6,-3.08739362900001));
#183614=CARTESIAN_POINT('Ctrl Pts',(9.97233683899994,15.2,-3.08679508900001));
#183615=CARTESIAN_POINT('Ctrl Pts',(9.97233683899994,11.6,-3.08679508900001));
#183616=CARTESIAN_POINT('Ctrl Pts',(9.97107548799995,15.2,-3.08620131400001));
#183617=CARTESIAN_POINT('Ctrl Pts',(9.97107548799995,11.6,-3.08620131400001));
#183618=CARTESIAN_POINT('Ctrl Pts',(9.96982113299994,15.2,-3.08561230000001));
#183619=CARTESIAN_POINT('Ctrl Pts',(9.96982113299994,11.6,-3.08561230000001));
#183620=CARTESIAN_POINT('Ctrl Pts',(9.96857379799994,15.2,-3.08502804400002));
#183621=CARTESIAN_POINT('Ctrl Pts',(9.96857379799994,11.6,-3.08502804400002));
#183622=CARTESIAN_POINT('Ctrl Pts',(9.96733350799994,15.2,-3.08444853900002));
#183623=CARTESIAN_POINT('Ctrl Pts',(9.96733350799994,11.6,-3.08444853900002));
#183624=CARTESIAN_POINT('Ctrl Pts',(9.96610028899994,15.2,-3.08387378200001));
#183625=CARTESIAN_POINT('Ctrl Pts',(9.96610028899994,11.6,-3.08387378200001));
#183626=CARTESIAN_POINT('Ctrl Pts',(9.96487416899994,15.2,-3.08330376800001));
#183627=CARTESIAN_POINT('Ctrl Pts',(9.96487416899994,11.6,-3.08330376800001));
#183628=CARTESIAN_POINT('Ctrl Pts',(9.96365516999995,15.2,-3.08273849300001));
#183629=CARTESIAN_POINT('Ctrl Pts',(9.96365516999995,11.6,-3.08273849300001));
#183630=CARTESIAN_POINT('Ctrl Pts',(9.96244331999995,15.2,-3.08217795000001));
#183631=CARTESIAN_POINT('Ctrl Pts',(9.96244331999995,11.6,-3.08217795000001));
#183632=CARTESIAN_POINT('Ctrl Pts',(9.96123864599994,15.2,-3.08162213600002));
#183633=CARTESIAN_POINT('Ctrl Pts',(9.96123864599994,11.6,-3.08162213600002));
#183634=CARTESIAN_POINT('Ctrl Pts',(9.96004117299995,15.2,-3.08107104600001));
#183635=CARTESIAN_POINT('Ctrl Pts',(9.96004117299995,11.6,-3.08107104600001));
#183636=CARTESIAN_POINT('Ctrl Pts',(9.95885092599995,15.2,-3.08052467500001));
#183637=CARTESIAN_POINT('Ctrl Pts',(9.95885092599995,11.6,-3.08052467500001));
#183638=CARTESIAN_POINT('Ctrl Pts',(9.95766793399994,15.2,-3.07998301700001));
#183639=CARTESIAN_POINT('Ctrl Pts',(9.95766793399994,11.6,-3.07998301700001));
#183640=CARTESIAN_POINT('Ctrl Pts',(9.95649222199994,15.2,-3.07944607000001));
#183641=CARTESIAN_POINT('Ctrl Pts',(9.95649222199994,11.6,-3.07944607000001));
#183642=CARTESIAN_POINT('Ctrl Pts',(9.95532381799995,15.2,-3.07891382600001));
#183643=CARTESIAN_POINT('Ctrl Pts',(9.95532381799995,11.6,-3.07891382600001));
#183644=CARTESIAN_POINT('Ctrl Pts',(9.95416274699994,15.2,-3.07838628200001));
#183645=CARTESIAN_POINT('Ctrl Pts',(9.95416274699994,11.6,-3.07838628200001));
#183646=CARTESIAN_POINT('Ctrl Pts',(9.95300903599994,15.2,-3.07786343200001));
#183647=CARTESIAN_POINT('Ctrl Pts',(9.95300903599994,11.6,-3.07786343200001));
#183648=CARTESIAN_POINT('Ctrl Pts',(9.95186271399995,15.2,-3.07734527000001));
#183649=CARTESIAN_POINT('Ctrl Pts',(9.95186271399995,11.6,-3.07734527000001));
#183650=CARTESIAN_POINT('Ctrl Pts',(9.95072380599994,15.2,-3.07683179400001));
#183651=CARTESIAN_POINT('Ctrl Pts',(9.95072380599994,11.6,-3.07683179400001));
#183652=CARTESIAN_POINT('Ctrl Pts',(9.94959233999994,15.2,-3.07632299600002));
#183653=CARTESIAN_POINT('Ctrl Pts',(9.94959233999994,11.6,-3.07632299600002));
#183654=CARTESIAN_POINT('Ctrl Pts',(9.94846834299994,15.2,-3.07581887100001));
#183655=CARTESIAN_POINT('Ctrl Pts',(9.94846834299994,11.6,-3.07581887100001));
#183656=CARTESIAN_POINT('Ctrl Pts',(9.94735184299994,15.2,-3.07531941600002));
#183657=CARTESIAN_POINT('Ctrl Pts',(9.94735184299994,11.6,-3.07531941600002));
#183658=CARTESIAN_POINT('Ctrl Pts',(9.94624286799995,15.2,-3.07482462300001));
#183659=CARTESIAN_POINT('Ctrl Pts',(9.94624286799995,11.6,-3.07482462300001));
#183660=CARTESIAN_POINT('Ctrl Pts',(9.94514144399995,15.2,-3.07433448900001));
#183661=CARTESIAN_POINT('Ctrl Pts',(9.94514144399995,11.6,-3.07433448900001));
#183662=CARTESIAN_POINT('Ctrl Pts',(9.94404760099994,15.2,-3.07384900800002));
#183663=CARTESIAN_POINT('Ctrl Pts',(9.94404760099994,11.6,-3.07384900800002));
#183664=CARTESIAN_POINT('Ctrl Pts',(9.94296136499995,15.2,-3.07336817300001));
#183665=CARTESIAN_POINT('Ctrl Pts',(9.94296136499995,11.6,-3.07336817300001));
#183666=CARTESIAN_POINT('Ctrl Pts',(9.94188276499995,15.2,-3.07289198100001));
#183667=CARTESIAN_POINT('Ctrl Pts',(9.94188276499995,11.6,-3.07289198100001));
#183668=CARTESIAN_POINT('Ctrl Pts',(9.94081182899994,15.2,-3.07242042600001));
#183669=CARTESIAN_POINT('Ctrl Pts',(9.94081182899994,11.6,-3.07242042600001));
#183670=CARTESIAN_POINT('Ctrl Pts',(9.93974858499995,15.2,-3.07195350200002));
#183671=CARTESIAN_POINT('Ctrl Pts',(9.93974858499995,11.6,-3.07195350200002));
#183672=CARTESIAN_POINT('Ctrl Pts',(9.93869306299995,15.2,-3.07149120200001));
#183673=CARTESIAN_POINT('Ctrl Pts',(9.93869306299995,11.6,-3.07149120200001));
#183674=CARTESIAN_POINT('Ctrl Pts',(9.93764528999994,15.2,-3.07103352400001));
#183675=CARTESIAN_POINT('Ctrl Pts',(9.93764528999994,11.6,-3.07103352400001));
#183676=CARTESIAN_POINT('Ctrl Pts',(9.93660529499994,15.2,-3.07058045900002));
#183677=CARTESIAN_POINT('Ctrl Pts',(9.93660529499994,11.6,-3.07058045900002));
#183678=CARTESIAN_POINT('Ctrl Pts',(9.93557310799994,15.2,-3.07013200400001));
#183679=CARTESIAN_POINT('Ctrl Pts',(9.93557310799994,11.6,-3.07013200400002));
#183680=CARTESIAN_POINT('Ctrl Pts',(9.93454875699994,15.2,-3.06968815200001));
#183681=CARTESIAN_POINT('Ctrl Pts',(9.93454875699994,11.6,-3.06968815200001));
#183682=CARTESIAN_POINT('Ctrl Pts',(9.93353226999995,15.2,-3.06924889800001));
#183683=CARTESIAN_POINT('Ctrl Pts',(9.93353226999995,11.6,-3.06924889800001));
#183684=CARTESIAN_POINT('Ctrl Pts',(9.93252367799995,15.2,-3.06881423400001));
#183685=CARTESIAN_POINT('Ctrl Pts',(9.93252367799995,11.6,-3.06881423400002));
#183686=CARTESIAN_POINT('Ctrl Pts',(9.93152301099995,15.2,-3.06838415800001));
#183687=CARTESIAN_POINT('Ctrl Pts',(9.93152301099995,11.6,-3.06838415800002));
#183688=CARTESIAN_POINT('Ctrl Pts',(9.93053029599994,15.2,-3.06795866100002));
#183689=CARTESIAN_POINT('Ctrl Pts',(9.93053029599994,11.6,-3.06795866100002));
#183690=CARTESIAN_POINT('Ctrl Pts',(9.92954556499994,15.2,-3.06753773800001));
#183691=CARTESIAN_POINT('Ctrl Pts',(9.92954556499994,11.6,-3.06753773800002));
#183692=CARTESIAN_POINT('Ctrl Pts',(9.92856884499994,15.2,-3.06712138300002));
#183693=CARTESIAN_POINT('Ctrl Pts',(9.92856884499994,11.6,-3.06712138300002));
#183694=CARTESIAN_POINT('Ctrl Pts',(9.92760016999994,15.2,-3.06670959200002));
#183695=CARTESIAN_POINT('Ctrl Pts',(9.92760016999994,11.6,-3.06670959200002));
#183696=CARTESIAN_POINT('Ctrl Pts',(9.92663956699994,15.2,-3.06630235600001));
#183697=CARTESIAN_POINT('Ctrl Pts',(9.92663956699994,11.6,-3.06630235600002));
#183698=CARTESIAN_POINT('Ctrl Pts',(9.92568706699995,15.2,-3.06589967100001));
#183699=CARTESIAN_POINT('Ctrl Pts',(9.92568706699995,11.6,-3.06589967100001));
#183700=CARTESIAN_POINT('Ctrl Pts',(9.92474269999994,15.2,-3.06550153000002));
#183701=CARTESIAN_POINT('Ctrl Pts',(9.92474269999994,11.6,-3.06550153000002));
#183702=CARTESIAN_POINT('Ctrl Pts',(9.92380649799994,15.2,-3.06510792800001));
#183703=CARTESIAN_POINT('Ctrl Pts',(9.92380649799994,11.6,-3.06510792800002));
#183704=CARTESIAN_POINT('Ctrl Pts',(9.92287849099995,15.2,-3.06471885700002));
#183705=CARTESIAN_POINT('Ctrl Pts',(9.92287849099995,11.6,-3.06471885700002));
#183706=CARTESIAN_POINT('Ctrl Pts',(9.92195870799994,15.2,-3.06433431200002));
#183707=CARTESIAN_POINT('Ctrl Pts',(9.92195870799994,11.6,-3.06433431200002));
#183708=CARTESIAN_POINT('Ctrl Pts',(9.92104718299995,15.2,-3.06395428600001));
#183709=CARTESIAN_POINT('Ctrl Pts',(9.92104718299995,11.6,-3.06395428600002));
#183710=CARTESIAN_POINT('Ctrl Pts',(9.92014394399994,15.2,-3.06357877400002));
#183711=CARTESIAN_POINT('Ctrl Pts',(9.92014394399994,11.6,-3.06357877400002));
#183712=CARTESIAN_POINT('Ctrl Pts',(9.91924902499994,15.2,-3.06320776900002));
#183713=CARTESIAN_POINT('Ctrl Pts',(9.91924902499994,11.6,-3.06320776900002));
#183714=CARTESIAN_POINT('Ctrl Pts',(9.91836245599995,15.2,-3.06284126300001));
#183715=CARTESIAN_POINT('Ctrl Pts',(9.91836245599995,11.6,-3.06284126300001));
#183716=CARTESIAN_POINT('Ctrl Pts',(9.91748426799995,15.2,-3.06247925400001));
#183717=CARTESIAN_POINT('Ctrl Pts',(9.91748426799995,11.6,-3.06247925400001));
#183718=CARTESIAN_POINT('Ctrl Pts',(9.91661449399994,15.2,-3.06212173000001));
#183719=CARTESIAN_POINT('Ctrl Pts',(9.91661449399994,11.6,-3.06212173000001));
#183720=CARTESIAN_POINT('Ctrl Pts',(9.91575316499994,15.2,-3.06176868700001));
#183721=CARTESIAN_POINT('Ctrl Pts',(9.91575316499994,11.6,-3.06176868700002));
#183722=CARTESIAN_POINT('Ctrl Pts',(9.91490522599995,15.2,-3.06142212700002));
#183723=CARTESIAN_POINT('Ctrl Pts',(9.91490522599995,11.6,-3.06142212700002));
#183724=CARTESIAN_POINT('Ctrl Pts',(9.91423456699994,15.2,-3.06114880400001));
#183725=CARTESIAN_POINT('Ctrl Pts',(9.91423456699994,11.6,-3.06114880400001));
#183726=CARTESIAN_POINT('Ctrl Pts',(9.91373655899995,15.2,-3.06094627500002));
#183727=CARTESIAN_POINT('Ctrl Pts',(9.91373655899995,11.6,-3.06094627500002));
#183728=CARTESIAN_POINT('Ctrl Pts',(9.91340782499995,15.2,-3.06081277600001));
#183729=CARTESIAN_POINT('Ctrl Pts',(9.91340782499995,11.6,-3.06081277600002));
#183730=CARTESIAN_POINT('Ctrl Pts',(9.91324626499994,15.2,-3.06074721200002));
#183731=CARTESIAN_POINT('Ctrl Pts',(9.91324626499994,11.6,-3.06074721200002));
#183732=CARTESIAN_POINT('',(9.91324626454087,12.2,-3.06074721206411));
#183733=CARTESIAN_POINT('',(9.91324626454087,15.2,-3.06074721206411));
#183734=CARTESIAN_POINT('',(9.91324626399994,12.2,-3.06074721200002));
#183735=CARTESIAN_POINT('Ctrl Pts',(10.8675859439999,12.2,-3.76106045600002));
#183736=CARTESIAN_POINT('Ctrl Pts',(10.8670460909999,12.2,-3.76051902400001));
#183737=CARTESIAN_POINT('Ctrl Pts',(10.8659664939999,12.2,-3.75943667400001));
#183738=CARTESIAN_POINT('Ctrl Pts',(10.8643474199999,12.2,-3.75781469800001));
#183739=CARTESIAN_POINT('Ctrl Pts',(10.8621893019999,12.2,-3.75565515600002));
#183740=CARTESIAN_POINT('Ctrl Pts',(10.8594927299999,12.2,-3.75296088400002));
#183741=CARTESIAN_POINT('Ctrl Pts',(10.8567972349999,12.2,-3.75027176800002));
#183742=CARTESIAN_POINT('Ctrl Pts',(10.8541028209999,12.2,-3.74758780800001));
#183743=CARTESIAN_POINT('Ctrl Pts',(10.8514094899999,12.2,-3.74490900600001));
#183744=CARTESIAN_POINT('Ctrl Pts',(10.8487172499999,12.2,-3.74223536100001));
#183745=CARTESIAN_POINT('Ctrl Pts',(10.8460261069999,12.2,-3.73956687500002));
#183746=CARTESIAN_POINT('Ctrl Pts',(10.8433360699999,12.2,-3.73690354800001));
#183747=CARTESIAN_POINT('Ctrl Pts',(10.8406471529999,12.2,-3.73424538200001));
#183748=CARTESIAN_POINT('Ctrl Pts',(10.8379593649999,12.2,-3.73159237800001));
#183749=CARTESIAN_POINT('Ctrl Pts',(10.8352727169999,12.2,-3.72894453800001));
#183750=CARTESIAN_POINT('Ctrl Pts',(10.8325872199999,12.2,-3.72630186200002));
#183751=CARTESIAN_POINT('Ctrl Pts',(10.8299028829999,12.2,-3.72366435100002));
#183752=CARTESIAN_POINT('Ctrl Pts',(10.8272197149999,12.2,-3.72103200700002));
#183753=CARTESIAN_POINT('Ctrl Pts',(10.8245377239999,12.2,-3.71840483100002));
#183754=CARTESIAN_POINT('Ctrl Pts',(10.8218569179999,12.2,-3.71578282200002));
#183755=CARTESIAN_POINT('Ctrl Pts',(10.8191773059999,12.2,-3.71316598200002));
#183756=CARTESIAN_POINT('Ctrl Pts',(10.8164988939999,12.2,-3.71055431200002));
#183757=CARTESIAN_POINT('Ctrl Pts',(10.8138216939999,12.2,-3.70794781300001));
#183758=CARTESIAN_POINT('Ctrl Pts',(10.8111457129999,12.2,-3.70534648600001));
#183759=CARTESIAN_POINT('Ctrl Pts',(10.8084709609999,12.2,-3.70275033200001));
#183760=CARTESIAN_POINT('Ctrl Pts',(10.8057974489999,12.2,-3.70015935000001));
#183761=CARTESIAN_POINT('Ctrl Pts',(10.8031251839999,12.2,-3.69757354500001));
#183762=CARTESIAN_POINT('Ctrl Pts',(10.8004541779999,12.2,-3.69499291500002));
#183763=CARTESIAN_POINT('Ctrl Pts',(10.7977844379999,12.2,-3.69241746100001));
#183764=CARTESIAN_POINT('Ctrl Pts',(10.7951159729999,12.2,-3.68984718400001));
#183765=CARTESIAN_POINT('Ctrl Pts',(10.7924487949999,12.2,-3.68728208700002));
#183766=CARTESIAN_POINT('Ctrl Pts',(10.7897829079999,12.2,-3.68472216800001));
#183767=CARTESIAN_POINT('Ctrl Pts',(10.7871183259999,12.2,-3.68216742900001));
#183768=CARTESIAN_POINT('Ctrl Pts',(10.7844550569999,12.2,-3.67961787200001));
#183769=CARTESIAN_POINT('Ctrl Pts',(10.7817931069999,12.2,-3.67707349500002));
#183770=CARTESIAN_POINT('Ctrl Pts',(10.7791324889999,12.2,-3.67453430200001));
#183771=CARTESIAN_POINT('Ctrl Pts',(10.7764732109999,12.2,-3.67200029300002));
#183772=CARTESIAN_POINT('Ctrl Pts',(10.7738152829999,12.2,-3.66947146800001));
#183773=CARTESIAN_POINT('Ctrl Pts',(10.7711587129999,12.2,-3.66694782800002));
#183774=CARTESIAN_POINT('Ctrl Pts',(10.7685035109999,12.2,-3.66442937400001));
#183775=CARTESIAN_POINT('Ctrl Pts',(10.7658496859999,12.2,-3.66191610700001));
#183776=CARTESIAN_POINT('Ctrl Pts',(10.7631972489999,12.2,-3.65940802800001));
#183777=CARTESIAN_POINT('Ctrl Pts',(10.7605462079999,12.2,-3.65690513800002));
#183778=CARTESIAN_POINT('Ctrl Pts',(10.7578965719999,12.2,-3.65440743700002));
#183779=CARTESIAN_POINT('Ctrl Pts',(10.7552483519999,12.2,-3.65191492600001));
#183780=CARTESIAN_POINT('Ctrl Pts',(10.7526015559999,12.2,-3.64942760700002));
#183781=CARTESIAN_POINT('Ctrl Pts',(10.7499561929999,12.2,-3.64694547900001));
#183782=CARTESIAN_POINT('Ctrl Pts',(10.7473122739999,12.2,-3.64446854400001));
#183783=CARTESIAN_POINT('Ctrl Pts',(10.7446698079999,12.2,-3.64199680200001));
#183784=CARTESIAN_POINT('Ctrl Pts',(10.7420288039999,12.2,-3.63953025500001));
#183785=CARTESIAN_POINT('Ctrl Pts',(10.7393892719999,12.2,-3.63706890200001));
#183786=CARTESIAN_POINT('Ctrl Pts',(10.7367512209999,12.2,-3.63461274500001));
#183787=CARTESIAN_POINT('Ctrl Pts',(10.7341146619999,12.2,-3.63216178500001));
#183788=CARTESIAN_POINT('Ctrl Pts',(10.7314796019999,12.2,-3.62971602300002));
#183789=CARTESIAN_POINT('Ctrl Pts',(10.7288460529999,12.2,-3.62727545700002));
#183790=CARTESIAN_POINT('Ctrl Pts',(10.7262140239999,12.2,-3.62484009100001));
#183791=CARTESIAN_POINT('Ctrl Pts',(10.7235835239999,12.2,-3.62240992500002));
#183792=CARTESIAN_POINT('Ctrl Pts',(10.7209545619999,12.2,-3.61998495800002));
#183793=CARTESIAN_POINT('Ctrl Pts',(10.7183271499999,12.2,-3.61756519200001));
#183794=CARTESIAN_POINT('Ctrl Pts',(10.7157012959999,12.2,-3.61515062900001));
#183795=CARTESIAN_POINT('Ctrl Pts',(10.7130770099999,12.2,-3.61274126800001));
#183796=CARTESIAN_POINT('Ctrl Pts',(10.7104543019999,12.2,-3.61033710900001));
#183797=CARTESIAN_POINT('Ctrl Pts',(10.7078331809999,12.2,-3.60793815500001));
#183798=CARTESIAN_POINT('Ctrl Pts',(10.7052136559999,12.2,-3.60554440400001));
#183799=CARTESIAN_POINT('Ctrl Pts',(10.7025957399999,12.2,-3.60315585900001));
#183800=CARTESIAN_POINT('Ctrl Pts',(10.6999794399999,12.2,-3.60077252100002));
#183801=CARTESIAN_POINT('Ctrl Pts',(10.6973647669999,12.2,-3.59839438800002));
#183802=CARTESIAN_POINT('Ctrl Pts',(10.6947517299999,12.2,-3.59602146200002));
#183803=CARTESIAN_POINT('Ctrl Pts',(10.6921403399999,12.2,-3.59365374400001));
#183804=CARTESIAN_POINT('Ctrl Pts',(10.6895306049999,12.2,-3.59129123500002));
#183805=CARTESIAN_POINT('Ctrl Pts',(10.6869225359999,12.2,-3.58893393500002));
#183806=CARTESIAN_POINT('Ctrl Pts',(10.6843161429999,12.2,-3.58658184500001));
#183807=CARTESIAN_POINT('Ctrl Pts',(10.6817114369999,12.2,-3.58423496500002));
#183808=CARTESIAN_POINT('Ctrl Pts',(10.6791084249999,12.2,-3.58189329600001));
#183809=CARTESIAN_POINT('Ctrl Pts',(10.6765071199999,12.2,-3.57955683900002));
#183810=CARTESIAN_POINT('Ctrl Pts',(10.6739075299999,12.2,-3.57722559400001));
#183811=CARTESIAN_POINT('Ctrl Pts',(10.6713096659999,12.2,-3.57489956100002));
#183812=CARTESIAN_POINT('Ctrl Pts',(10.6687135369999,12.2,-3.57257874200001));
#183813=CARTESIAN_POINT('Ctrl Pts',(10.6661191539999,12.2,-3.57026313700001));
#183814=CARTESIAN_POINT('Ctrl Pts',(10.6635265279999,12.2,-3.56795274600001));
#183815=CARTESIAN_POINT('Ctrl Pts',(10.6609356659999,12.2,-3.56564757100001));
#183816=CARTESIAN_POINT('Ctrl Pts',(10.6583465819999,12.2,-3.56334761200001));
#183817=CARTESIAN_POINT('Ctrl Pts',(10.6557592819999,12.2,-3.56105286800001));
#183818=CARTESIAN_POINT('Ctrl Pts',(10.6531737789999,12.2,-3.55876334200001));
#183819=CARTESIAN_POINT('Ctrl Pts',(10.6505900819999,12.2,-3.55647903300001));
#183820=CARTESIAN_POINT('Ctrl Pts',(10.6480082019999,12.2,-3.55419994100002));
#183821=CARTESIAN_POINT('Ctrl Pts',(10.6454281479999,12.2,-3.55192606900002));
#183822=CARTESIAN_POINT('Ctrl Pts',(10.6428499309999,12.2,-3.54965741400001));
#183823=CARTESIAN_POINT('Ctrl Pts',(10.6402735619999,12.2,-3.54739398000001));
#183824=CARTESIAN_POINT('Ctrl Pts',(10.6376990499999,12.2,-3.54513576600001));
#183825=CARTESIAN_POINT('Ctrl Pts',(10.6351264049999,12.2,-3.54288277200002));
#183826=CARTESIAN_POINT('Ctrl Pts',(10.6325556389999,12.2,-3.54063499900001));
#183827=CARTESIAN_POINT('Ctrl Pts',(10.6299867589999,12.2,-3.53839244700001));
#183828=CARTESIAN_POINT('Ctrl Pts',(10.6274197799999,12.2,-3.53615511700001));
#183829=CARTESIAN_POINT('Ctrl Pts',(10.6248547079999,12.2,-3.53392301000001));
#183830=CARTESIAN_POINT('Ctrl Pts',(10.6222915559999,12.2,-3.53169612600002));
#183831=CARTESIAN_POINT('Ctrl Pts',(10.6197303339999,12.2,-3.52947446500002));
#183832=CARTESIAN_POINT('Ctrl Pts',(10.6171710509999,12.2,-3.52725802700002));
#183833=CARTESIAN_POINT('Ctrl Pts',(10.6146137189999,12.2,-3.52504681400001));
#183834=CARTESIAN_POINT('Ctrl Pts',(10.6120583479999,12.2,-3.52284082600002));
#183835=CARTESIAN_POINT('Ctrl Pts',(10.6095049489999,12.2,-3.52064006300001));
#183836=CARTESIAN_POINT('Ctrl Pts',(10.6069535309999,12.2,-3.51844452500002));
#183837=CARTESIAN_POINT('Ctrl Pts',(10.6044041049999,12.2,-3.51625421300001));
#183838=CARTESIAN_POINT('Ctrl Pts',(10.6018566829999,12.2,-3.51406912700002));
#183839=CARTESIAN_POINT('Ctrl Pts',(10.5993112729999,12.2,-3.51188926900001));
#183840=CARTESIAN_POINT('Ctrl Pts',(10.5967678879999,12.2,-3.50971463600001));
#183841=CARTESIAN_POINT('Ctrl Pts',(10.5942265379999,12.2,-3.50754523200001));
#183842=CARTESIAN_POINT('Ctrl Pts',(10.5916872319999,12.2,-3.50538105500001));
#183843=CARTESIAN_POINT('Ctrl Pts',(10.5891499829999,12.2,-3.50322210700002));
#183844=CARTESIAN_POINT('Ctrl Pts',(10.5866147999999,12.2,-3.50106838700002));
#183845=CARTESIAN_POINT('Ctrl Pts',(10.5840816949999,12.2,-3.49891989600001));
#183846=CARTESIAN_POINT('Ctrl Pts',(10.5815506769999,12.2,-3.49677663500001));
#183847=CARTESIAN_POINT('Ctrl Pts',(10.5790217569999,12.2,-3.49463860200002));
#183848=CARTESIAN_POINT('Ctrl Pts',(10.5764949479999,12.2,-3.49250580000001));
#183849=CARTESIAN_POINT('Ctrl Pts',(10.5739702579999,12.2,-3.49037822900002));
#183850=CARTESIAN_POINT('Ctrl Pts',(10.5714476989999,12.2,-3.48825588800001));
#183851=CARTESIAN_POINT('Ctrl Pts',(10.5689272829999,12.2,-3.48613877700001));
#183852=CARTESIAN_POINT('Ctrl Pts',(10.5664090179999,12.2,-3.48402689800002));
#183853=CARTESIAN_POINT('Ctrl Pts',(10.5638929169999,12.2,-3.48192025000001));
#183854=CARTESIAN_POINT('Ctrl Pts',(10.5613789899999,12.2,-3.47981883400001));
#183855=CARTESIAN_POINT('Ctrl Pts',(10.5588672479999,12.2,-3.47772265000001));
#183856=CARTESIAN_POINT('Ctrl Pts',(10.5563577029999,12.2,-3.47563169800001));
#183857=CARTESIAN_POINT('Ctrl Pts',(10.5538503639999,12.2,-3.47354597800001));
#183858=CARTESIAN_POINT('Ctrl Pts',(10.5513452449999,12.2,-3.47146549100001));
#183859=CARTESIAN_POINT('Ctrl Pts',(10.5488423529999,12.2,-3.46939023800001));
#183860=CARTESIAN_POINT('Ctrl Pts',(10.5463417019999,12.2,-3.46732021700001));
#183861=CARTESIAN_POINT('Ctrl Pts',(10.5438433009999,12.2,-3.46525543000002));
#183862=CARTESIAN_POINT('Ctrl Pts',(10.5413471629999,12.2,-3.46319587600001));
#183863=CARTESIAN_POINT('Ctrl Pts',(10.5388532969999,12.2,-3.46114155700001));
#183864=CARTESIAN_POINT('Ctrl Pts',(10.5363617169999,12.2,-3.45909247100002));
#183865=CARTESIAN_POINT('Ctrl Pts',(10.5338724319999,12.2,-3.45704862000002));
#183866=CARTESIAN_POINT('Ctrl Pts',(10.5313854529999,12.2,-3.45501000300001));
#183867=CARTESIAN_POINT('Ctrl Pts',(10.5289007929999,12.2,-3.45297662100001));
#183868=CARTESIAN_POINT('Ctrl Pts',(10.5264184599999,12.2,-3.45094847300001));
#183869=CARTESIAN_POINT('Ctrl Pts',(10.5239384669999,12.2,-3.44892556000001));
#183870=CARTESIAN_POINT('Ctrl Pts',(10.5214608269999,12.2,-3.44690788300001));
#183871=CARTESIAN_POINT('Ctrl Pts',(10.5189855499999,12.2,-3.44489544000002));
#183872=CARTESIAN_POINT('Ctrl Pts',(10.5165126449999,12.2,-3.44288823300001));
#183873=CARTESIAN_POINT('Ctrl Pts',(10.5140421269999,12.2,-3.44088626100001));
#183874=CARTESIAN_POINT('Ctrl Pts',(10.5115740039999,12.2,-3.43888952500001));
#183875=CARTESIAN_POINT('Ctrl Pts',(10.5091082899999,12.2,-3.43689802500001));
#183876=CARTESIAN_POINT('Ctrl Pts',(10.5066449939999,12.2,-3.43491176000001));
#183877=CARTESIAN_POINT('Ctrl Pts',(10.5041841299999,12.2,-3.43293073100002));
#183878=CARTESIAN_POINT('Ctrl Pts',(10.5017257079999,12.2,-3.43095493800002));
#183879=CARTESIAN_POINT('Ctrl Pts',(10.4992697399999,12.2,-3.42898438100002));
#183880=CARTESIAN_POINT('Ctrl Pts',(10.4968162359999,12.2,-3.42701906000002));
#183881=CARTESIAN_POINT('Ctrl Pts',(10.4943652099999,12.2,-3.42505897500001));
#183882=CARTESIAN_POINT('Ctrl Pts',(10.4919166709999,12.2,-3.42310412600002));
#183883=CARTESIAN_POINT('Ctrl Pts',(10.4894706319999,12.2,-3.42115451300002));
#183884=CARTESIAN_POINT('Ctrl Pts',(10.4870271039999,12.2,-3.41921013700001));
#183885=CARTESIAN_POINT('Ctrl Pts',(10.4845860999999,12.2,-3.41727099600002));
#183886=CARTESIAN_POINT('Ctrl Pts',(10.4821476289999,12.2,-3.41533709100001));
#183887=CARTESIAN_POINT('Ctrl Pts',(10.4797117049999,12.2,-3.41340842300002));
#183888=CARTESIAN_POINT('Ctrl Pts',(10.4772783389999,12.2,-3.41148499200001));
#183889=CARTESIAN_POINT('Ctrl Pts',(10.4748475419999,12.2,-3.40956679600001));
#183890=CARTESIAN_POINT('Ctrl Pts',(10.4724193259999,12.2,-3.40765383700001));
#183891=CARTESIAN_POINT('Ctrl Pts',(10.4699937039999,12.2,-3.40574611300001));
#183892=CARTESIAN_POINT('Ctrl Pts',(10.4675706859999,12.2,-3.40384362500001));
#183893=CARTESIAN_POINT('Ctrl Pts',(10.4651502849999,12.2,-3.40194637400002));
#183894=CARTESIAN_POINT('Ctrl Pts',(10.4627325119999,12.2,-3.40005435900002));
#183895=CARTESIAN_POINT('Ctrl Pts',(10.4603173799999,12.2,-3.39816757900001));
#183896=CARTESIAN_POINT('Ctrl Pts',(10.4579048999999,12.2,-3.39628603500001));
#183897=CARTESIAN_POINT('Ctrl Pts',(10.4554950839999,12.2,-3.39440972700002));
#183898=CARTESIAN_POINT('Ctrl Pts',(10.4530879439999,12.2,-3.39253865400002));
#183899=CARTESIAN_POINT('Ctrl Pts',(10.4506834919999,12.2,-3.39067281600002));
#183900=CARTESIAN_POINT('Ctrl Pts',(10.4482817399999,12.2,-3.38881221500001));
#183901=CARTESIAN_POINT('Ctrl Pts',(10.4458826999999,12.2,-3.38695684700001));
#183902=CARTESIAN_POINT('Ctrl Pts',(10.4434863849999,12.2,-3.38510671600002));
#183903=CARTESIAN_POINT('Ctrl Pts',(10.4410928049999,12.2,-3.38326181800001));
#183904=CARTESIAN_POINT('Ctrl Pts',(10.4387019739999,12.2,-3.38142215600001));
#183905=CARTESIAN_POINT('Ctrl Pts',(10.4363139019999,12.2,-3.37958772900001));
#183906=CARTESIAN_POINT('Ctrl Pts',(10.4339286029999,12.2,-3.37775853500001));
#183907=CARTESIAN_POINT('Ctrl Pts',(10.4315460899999,12.2,-3.37593457500001));
#183908=CARTESIAN_POINT('Ctrl Pts',(10.4291663729999,12.2,-3.37411585000002));
#183909=CARTESIAN_POINT('Ctrl Pts',(10.4267894639999,12.2,-3.37230235900002));
#183910=CARTESIAN_POINT('Ctrl Pts',(10.4244153789999,12.2,-3.37049410100001));
#183911=CARTESIAN_POINT('Ctrl Pts',(10.4220441259999,12.2,-3.36869107600001));
#183912=CARTESIAN_POINT('Ctrl Pts',(10.4196757189999,12.2,-3.36689328500002));
#183913=CARTESIAN_POINT('Ctrl Pts',(10.4173101699999,12.2,-3.36510072600001));
#183914=CARTESIAN_POINT('Ctrl Pts',(10.4149474929999,12.2,-3.36331340000001));
#183915=CARTESIAN_POINT('Ctrl Pts',(10.4125876979999,12.2,-3.36153130600001));
#183916=CARTESIAN_POINT('Ctrl Pts',(10.4102307989999,12.2,-3.35975444400002));
#183917=CARTESIAN_POINT('Ctrl Pts',(10.4078768069999,12.2,-3.35798281300002));
#183918=CARTESIAN_POINT('Ctrl Pts',(10.4055257379999,12.2,-3.35621641400001));
#183919=CARTESIAN_POINT('Ctrl Pts',(10.4031775999999,12.2,-3.35445524600001));
#183920=CARTESIAN_POINT('Ctrl Pts',(10.4008324069999,12.2,-3.35269930900001));
#183921=CARTESIAN_POINT('Ctrl Pts',(10.3984901739999,12.2,-3.35094860300002));
#183922=CARTESIAN_POINT('Ctrl Pts',(10.3961509099999,12.2,-3.34920312600001));
#183923=CARTESIAN_POINT('Ctrl Pts',(10.3938146309999,12.2,-3.34746287900002));
#183924=CARTESIAN_POINT('Ctrl Pts',(10.3914813469999,12.2,-3.34572786200001));
#183925=CARTESIAN_POINT('Ctrl Pts',(10.3891510709999,12.2,-3.34399807300001));
#183926=CARTESIAN_POINT('Ctrl Pts',(10.3868238179999,12.2,-3.34227351400001));
#183927=CARTESIAN_POINT('Ctrl Pts',(10.3844995979999,12.2,-3.34055418200002));
#183928=CARTESIAN_POINT('Ctrl Pts',(10.3821784259999,12.2,-3.33884007800001));
#183929=CARTESIAN_POINT('Ctrl Pts',(10.3798603139999,12.2,-3.33713120100001));
#183930=CARTESIAN_POINT('Ctrl Pts',(10.3775452729999,12.2,-3.33542755200002));
#183931=CARTESIAN_POINT('Ctrl Pts',(10.3752333189999,12.2,-3.33372913000002));
#183932=CARTESIAN_POINT('Ctrl Pts',(10.3729244619999,12.2,-3.33203593300002));
#183933=CARTESIAN_POINT('Ctrl Pts',(10.3706187169999,12.2,-3.33034796100002));
#183934=CARTESIAN_POINT('Ctrl Pts',(10.3683160969999,12.2,-3.32866521600002));
#183935=CARTESIAN_POINT('Ctrl Pts',(10.3660166129999,12.2,-3.32698769300002));
#183936=CARTESIAN_POINT('Ctrl Pts',(10.3637202799999,12.2,-3.32531539600001));
#183937=CARTESIAN_POINT('Ctrl Pts',(10.3614271109999,12.2,-3.32364832300001));
#183938=CARTESIAN_POINT('Ctrl Pts',(10.3591371169999,12.2,-3.32198647300002));
#183939=CARTESIAN_POINT('Ctrl Pts',(10.3568503129999,12.2,-3.32032984500001));
#183940=CARTESIAN_POINT('Ctrl Pts',(10.3545667119999,12.2,-3.31867843900001));
#183941=CARTESIAN_POINT('Ctrl Pts',(10.3522863269999,12.2,-3.31703225500001));
#183942=CARTESIAN_POINT('Ctrl Pts',(10.3500091699999,12.2,-3.31539129200001));
#183943=CARTESIAN_POINT('Ctrl Pts',(10.3477352559999,12.2,-3.31375555000001));
#183944=CARTESIAN_POINT('Ctrl Pts',(10.3454645979999,12.2,-3.31212502700001));
#183945=CARTESIAN_POINT('Ctrl Pts',(10.3431972079999,12.2,-3.31049972300002));
#183946=CARTESIAN_POINT('Ctrl Pts',(10.3409331009999,12.2,-3.30887963800001));
#183947=CARTESIAN_POINT('Ctrl Pts',(10.3386722889999,12.2,-3.30726477100002));
#183948=CARTESIAN_POINT('Ctrl Pts',(10.3364147869999,12.2,-3.30565512200002));
#183949=CARTESIAN_POINT('Ctrl Pts',(10.3341606059999,12.2,-3.30405069000001));
#183950=CARTESIAN_POINT('Ctrl Pts',(10.3319097619999,12.2,-3.30245147300001));
#183951=CARTESIAN_POINT('Ctrl Pts',(10.3296622669999,12.2,-3.30085747200001));
#183952=CARTESIAN_POINT('Ctrl Pts',(10.3274181339999,12.2,-3.29926868600001));
#183953=CARTESIAN_POINT('Ctrl Pts',(10.3251773799999,12.2,-3.29768511400002));
#183954=CARTESIAN_POINT('Ctrl Pts',(10.3229400139999,12.2,-3.29610675500001));
#183955=CARTESIAN_POINT('Ctrl Pts',(10.3207060529999,12.2,-3.29453360900001));
#183956=CARTESIAN_POINT('Ctrl Pts',(10.3184755079999,12.2,-3.29296567500001));
#183957=CARTESIAN_POINT('Ctrl Pts',(10.3162483959999,12.2,-3.29140295300002));
#183958=CARTESIAN_POINT('Ctrl Pts',(10.3140247269999,12.2,-3.28984544000001));
#183959=CARTESIAN_POINT('Ctrl Pts',(10.3118045179999,12.2,-3.28829313800002));
#183960=CARTESIAN_POINT('Ctrl Pts',(10.3095877799999,12.2,-3.28674604500002));
#183961=CARTESIAN_POINT('Ctrl Pts',(10.3073745299999,12.2,-3.28520415900002));
#183962=CARTESIAN_POINT('Ctrl Pts',(10.3051647789999,12.2,-3.28366748100001));
#183963=CARTESIAN_POINT('Ctrl Pts',(10.3029585419999,12.2,-3.28213601000002));
#183964=CARTESIAN_POINT('Ctrl Pts',(10.3007558329999,12.2,-3.28060974400001));
#183965=CARTESIAN_POINT('Ctrl Pts',(10.2985566669999,12.2,-3.27908868400002));
#183966=CARTESIAN_POINT('Ctrl Pts',(10.2963610559999,12.2,-3.27757282800002));
#183967=CARTESIAN_POINT('Ctrl Pts',(10.2941690149999,12.2,-3.27606217500001));
#183968=CARTESIAN_POINT('Ctrl Pts',(10.2919805579999,12.2,-3.27455672400002));
#183969=CARTESIAN_POINT('Ctrl Pts',(10.2897957009999,12.2,-3.27305647500001));
#183970=CARTESIAN_POINT('Ctrl Pts',(10.2876144549999,12.2,-3.27156142700002));
#183971=CARTESIAN_POINT('Ctrl Pts',(10.2854368349999,12.2,-3.27007157800002));
#183972=CARTESIAN_POINT('Ctrl Pts',(10.2832628569999,12.2,-3.26858692800001));
#183973=CARTESIAN_POINT('Ctrl Pts',(10.2810925339999,12.2,-3.26710747600002));
#183974=CARTESIAN_POINT('Ctrl Pts',(10.2789258799999,12.2,-3.26563322100001));
#183975=CARTESIAN_POINT('Ctrl Pts',(10.2767629099999,12.2,-3.26416416200002));
#183976=CARTESIAN_POINT('Ctrl Pts',(10.2746036379999,12.2,-3.26270029800002));
#183977=CARTESIAN_POINT('Ctrl Pts',(10.2724480789999,12.2,-3.26124162800001));
#183978=CARTESIAN_POINT('Ctrl Pts',(10.2702962469999,12.2,-3.25978815000001));
#183979=CARTESIAN_POINT('Ctrl Pts',(10.2681481549999,12.2,-3.25833986600002));
#183980=CARTESIAN_POINT('Ctrl Pts',(10.2660038209999,12.2,-3.25689677200002));
#183981=CARTESIAN_POINT('Ctrl Pts',(10.2638632559999,12.2,-3.25545886800001));
#183982=CARTESIAN_POINT('Ctrl Pts',(10.2617264769999,12.2,-3.25402615300002));
#183983=CARTESIAN_POINT('Ctrl Pts',(10.2595934979999,12.2,-3.25259862700001));
#183984=CARTESIAN_POINT('Ctrl Pts',(10.2574643339999,12.2,-3.25117628600001));
#183985=CARTESIAN_POINT('Ctrl Pts',(10.2553389979999,12.2,-3.24975913200001));
#183986=CARTESIAN_POINT('Ctrl Pts',(10.2532175069999,12.2,-3.24834716200002));
#183987=CARTESIAN_POINT('Ctrl Pts',(10.2510998739999,12.2,-3.24694037600001));
#183988=CARTESIAN_POINT('Ctrl Pts',(10.2489861149999,12.2,-3.24553877200001));
#183989=CARTESIAN_POINT('Ctrl Pts',(10.2468762449999,12.2,-3.24414235000001));
#183990=CARTESIAN_POINT('Ctrl Pts',(10.2447702779999,12.2,-3.24275110800002));
#183991=CARTESIAN_POINT('Ctrl Pts',(10.2426682289999,12.2,-3.24136504400002));
#183992=CARTESIAN_POINT('Ctrl Pts',(10.2405701139999,12.2,-3.23998415800002));
#183993=CARTESIAN_POINT('Ctrl Pts',(10.2384759469999,12.2,-3.23860844800001));
#183994=CARTESIAN_POINT('Ctrl Pts',(10.2363857439999,12.2,-3.23723791500001));
#183995=CARTESIAN_POINT('Ctrl Pts',(10.2342995189999,12.2,-3.23587255500001));
#183996=CARTESIAN_POINT('Ctrl Pts',(10.2322172889999,12.2,-3.23451236800001));
#183997=CARTESIAN_POINT('Ctrl Pts',(10.2301390659999,12.2,-3.23315735300001));
#183998=CARTESIAN_POINT('Ctrl Pts',(10.2280648689999,12.2,-3.23180750800002));
#183999=CARTESIAN_POINT('Ctrl Pts',(10.2259947109999,12.2,-3.23046283300001));
#184000=CARTESIAN_POINT('Ctrl Pts',(10.2239286079999,12.2,-3.22912332500001));
#184001=CARTESIAN_POINT('Ctrl Pts',(10.2218665749999,12.2,-3.22778898400002));
#184002=CARTESIAN_POINT('Ctrl Pts',(10.2198086269999,12.2,-3.22645980700001));
#184003=CARTESIAN_POINT('Ctrl Pts',(10.2177547809999,12.2,-3.22513579400002));
#184004=CARTESIAN_POINT('Ctrl Pts',(10.2157050509999,12.2,-3.22381694500002));
#184005=CARTESIAN_POINT('Ctrl Pts',(10.2136594529999,12.2,-3.22250325600002));
#184006=CARTESIAN_POINT('Ctrl Pts',(10.2116180039999,12.2,-3.22119472700001));
#184007=CARTESIAN_POINT('Ctrl Pts',(10.2095807169999,12.2,-3.21989135600001));
#184008=CARTESIAN_POINT('Ctrl Pts',(10.2075476089999,12.2,-3.21859314200001));
#184009=CARTESIAN_POINT('Ctrl Pts',(10.2055186959999,12.2,-3.21730008500001));
#184010=CARTESIAN_POINT('Ctrl Pts',(10.2034939929999,12.2,-3.21601218000001));
#184011=CARTESIAN_POINT('Ctrl Pts',(10.2014735169999,12.2,-3.21472942900002));
#184012=CARTESIAN_POINT('Ctrl Pts',(10.1994572829999,12.2,-3.21345182800002));
#184013=CARTESIAN_POINT('Ctrl Pts',(10.1974453069999,12.2,-3.21217937700002));
#184014=CARTESIAN_POINT('Ctrl Pts',(10.1954376039999,12.2,-3.21091207400002));
#184015=CARTESIAN_POINT('Ctrl Pts',(10.1934341909999,12.2,-3.20964991800002));
#184016=CARTESIAN_POINT('Ctrl Pts',(10.1914350849999,12.2,-3.20839290800001));
#184017=CARTESIAN_POINT('Ctrl Pts',(10.1894402999999,12.2,-3.20714104000002));
#184018=CARTESIAN_POINT('Ctrl Pts',(10.1874498539999,12.2,-3.20589431400002));
#184019=CARTESIAN_POINT('Ctrl Pts',(10.1854637609999,12.2,-3.20465272900002));
#184020=CARTESIAN_POINT('Ctrl Pts',(10.1834820399999,12.2,-3.20341628300001));
#184021=CARTESIAN_POINT('Ctrl Pts',(10.1815047049999,12.2,-3.20218497500001));
#184022=CARTESIAN_POINT('Ctrl Pts',(10.1795317729999,12.2,-3.20095880100002));
#184023=CARTESIAN_POINT('Ctrl Pts',(10.1775632609999,12.2,-3.19973776100001));
#184024=CARTESIAN_POINT('Ctrl Pts',(10.1755991829999,12.2,-3.19852185400002));
#184025=CARTESIAN_POINT('Ctrl Pts',(10.1736395589999,12.2,-3.19731107700001));
#184026=CARTESIAN_POINT('Ctrl Pts',(10.1716844029999,12.2,-3.19610542900001));
#184027=CARTESIAN_POINT('Ctrl Pts',(10.1697337309999,12.2,-3.19490490900002));
#184028=CARTESIAN_POINT('Ctrl Pts',(10.1677875629999,12.2,-3.19370951400002));
#184029=CARTESIAN_POINT('Ctrl Pts',(10.1658459129999,12.2,-3.19251924300001));
#184030=CARTESIAN_POINT('Ctrl Pts',(10.1639087969999,12.2,-3.19133409300001));
#184031=CARTESIAN_POINT('Ctrl Pts',(10.1619762339999,12.2,-3.19015406500001));
#184032=CARTESIAN_POINT('Ctrl Pts',(10.1600482389999,12.2,-3.18897915400001));
#184033=CARTESIAN_POINT('Ctrl Pts',(10.1581248299999,12.2,-3.18780935900001));
#184034=CARTESIAN_POINT('Ctrl Pts',(10.1562060229999,12.2,-3.18664468000001));
#184035=CARTESIAN_POINT('Ctrl Pts',(10.1542918349999,12.2,-3.18548511300001));
#184036=CARTESIAN_POINT('Ctrl Pts',(10.1523822839999,12.2,-3.18433065800001));
#184037=CARTESIAN_POINT('Ctrl Pts',(10.1504773859999,12.2,-3.18318131200002));
#184038=CARTESIAN_POINT('Ctrl Pts',(10.1485771589999,12.2,-3.18203707400002));
#184039=CARTESIAN_POINT('Ctrl Pts',(10.1466816179999,12.2,-3.18089793900001));
#184040=CARTESIAN_POINT('Ctrl Pts',(10.1447907829999,12.2,-3.17976391000002));
#184041=CARTESIAN_POINT('Ctrl Pts',(10.1429046699999,12.2,-3.17863498200001));
#184042=CARTESIAN_POINT('Ctrl Pts',(10.1410232959999,12.2,-3.17751115200001));
#184043=CARTESIAN_POINT('Ctrl Pts',(10.1391466789999,12.2,-3.17639242200002));
#184044=CARTESIAN_POINT('Ctrl Pts',(10.1372748349999,12.2,-3.17527878600002));
#184045=CARTESIAN_POINT('Ctrl Pts',(10.1354077839999,12.2,-3.17417024400001));
#184046=CARTESIAN_POINT('Ctrl Pts',(10.1335455409999,12.2,-3.17306679400001));
#184047=CARTESIAN_POINT('Ctrl Pts',(10.1316881249999,12.2,-3.17196843300001));
#184048=CARTESIAN_POINT('Ctrl Pts',(10.1298355529999,12.2,-3.17087516000001));
#184049=CARTESIAN_POINT('Ctrl Pts',(10.1279878419999,12.2,-3.16978697100001));
#184050=CARTESIAN_POINT('Ctrl Pts',(10.1261450119999,12.2,-3.16870386600002));
#184051=CARTESIAN_POINT('Ctrl Pts',(10.1243070779999,12.2,-3.16762584300001));
#184052=CARTESIAN_POINT('Ctrl Pts',(10.1224740599999,12.2,-3.16655289800002));
#184053=CARTESIAN_POINT('Ctrl Pts',(10.1206459739999,12.2,-3.16548503000002));
#184054=CARTESIAN_POINT('Ctrl Pts',(10.1188228389999,12.2,-3.16442223800002));
#184055=CARTESIAN_POINT('Ctrl Pts',(10.1170046749999,12.2,-3.16336451600002));
#184056=CARTESIAN_POINT('Ctrl Pts',(10.1151914959999,12.2,-3.16231186600001));
#184057=CARTESIAN_POINT('Ctrl Pts',(10.1133833219999,12.2,-3.16126428300001));
#184058=CARTESIAN_POINT('Ctrl Pts',(10.1115801729999,12.2,-3.16022176700002));
#184059=CARTESIAN_POINT('Ctrl Pts',(10.1097820639999,12.2,-3.15918431300001));
#184060=CARTESIAN_POINT('Ctrl Pts',(10.1079890159999,12.2,-3.15815192100001));
#184061=CARTESIAN_POINT('Ctrl Pts',(10.1062010459999,12.2,-3.15712458800002));
#184062=CARTESIAN_POINT('Ctrl Pts',(10.1044181719999,12.2,-3.15610231100001));
#184063=CARTESIAN_POINT('Ctrl Pts',(10.1026404129999,12.2,-3.15508509000002));
#184064=CARTESIAN_POINT('Ctrl Pts',(10.1008677879999,12.2,-3.15407291900001));
#184065=CARTESIAN_POINT('Ctrl Pts',(10.0991003149999,12.2,-3.15306579700001));
#184066=CARTESIAN_POINT('Ctrl Pts',(10.0973380129999,12.2,-3.15206372300001));
#184067=CARTESIAN_POINT('Ctrl Pts',(10.0955808999999,12.2,-3.15106669300001));
#184068=CARTESIAN_POINT('Ctrl Pts',(10.0938289959999,12.2,-3.15007470700001));
#184069=CARTESIAN_POINT('Ctrl Pts',(10.0920823179999,12.2,-3.14908775800002));
#184070=CARTESIAN_POINT('Ctrl Pts',(10.0903408869999,12.2,-3.14810584800002));
#184071=CARTESIAN_POINT('Ctrl Pts',(10.0886047199999,12.2,-3.14712897300002));
#184072=CARTESIAN_POINT('Ctrl Pts',(10.0868738369999,12.2,-3.14615712900002));
#184073=CARTESIAN_POINT('Ctrl Pts',(10.0851482559999,12.2,-3.14519031400001));
#184074=CARTESIAN_POINT('Ctrl Pts',(10.0834279989999,12.2,-3.14422852800002));
#184075=CARTESIAN_POINT('Ctrl Pts',(10.0817130829999,12.2,-3.14327176500001));
#184076=CARTESIAN_POINT('Ctrl Pts',(10.0800035259999,12.2,-3.14232002500002));
#184077=CARTESIAN_POINT('Ctrl Pts',(10.0782993499999,12.2,-3.14137330300001));
#184078=CARTESIAN_POINT('Ctrl Pts',(10.0766005729999,12.2,-3.14043159900002));
#184079=CARTESIAN_POINT('Ctrl Pts',(10.0749072159999,12.2,-3.13949490700002));
#184080=CARTESIAN_POINT('Ctrl Pts',(10.0732192959999,12.2,-3.13856322800001));
#184081=CARTESIAN_POINT('Ctrl Pts',(10.0715368339999,12.2,-3.13763655600001));
#184082=CARTESIAN_POINT('Ctrl Pts',(10.0698598489999,12.2,-3.13671489000001));
#184083=CARTESIAN_POINT('Ctrl Pts',(10.0681883619999,12.2,-3.13579822800001));
#184084=CARTESIAN_POINT('Ctrl Pts',(10.0665223919999,12.2,-3.13488656500001));
#184085=CARTESIAN_POINT('Ctrl Pts',(10.0648619579999,12.2,-3.13397990000002));
#184086=CARTESIAN_POINT('Ctrl Pts',(10.0632070809999,12.2,-3.13307822900001));
#184087=CARTESIAN_POINT('Ctrl Pts',(10.0615577799999,12.2,-3.13218155100001));
#184088=CARTESIAN_POINT('Ctrl Pts',(10.0599140779999,12.2,-3.13128986000001));
#184089=CARTESIAN_POINT('Ctrl Pts',(10.0582759909999,12.2,-3.13040315700002));
#184090=CARTESIAN_POINT('Ctrl Pts',(10.0566435409999,12.2,-3.12952143500001));
#184091=CARTESIAN_POINT('Ctrl Pts',(10.0550167499999,12.2,-3.12864469400001));
#184092=CARTESIAN_POINT('Ctrl Pts',(10.0533956349999,12.2,-3.12777293000002));
#184093=CARTESIAN_POINT('Ctrl Pts',(10.0517802179999,12.2,-3.12690614000001));
#184094=CARTESIAN_POINT('Ctrl Pts',(10.0501705219999,12.2,-3.12604432200001));
#184095=CARTESIAN_POINT('Ctrl Pts',(10.0485665629999,12.2,-3.12518747000002));
#184096=CARTESIAN_POINT('Ctrl Pts',(10.0469683629999,12.2,-3.12433558500001));
#184097=CARTESIAN_POINT('Ctrl Pts',(10.0453759449999,12.2,-3.12348866100002));
#184098=CARTESIAN_POINT('Ctrl Pts',(10.0437893269999,12.2,-3.12264669700001));
#184099=CARTESIAN_POINT('Ctrl Pts',(10.0422085329999,12.2,-3.12180968700002));
#184100=CARTESIAN_POINT('Ctrl Pts',(10.0406335799999,12.2,-3.12097763100001));
#184101=CARTESIAN_POINT('Ctrl Pts',(10.0390644919999,12.2,-3.12015052400001));
#184102=CARTESIAN_POINT('Ctrl Pts',(10.0375012879999,12.2,-3.11932836300001));
#184103=CARTESIAN_POINT('Ctrl Pts',(10.0359439909999,12.2,-3.11851114600001));
#184104=CARTESIAN_POINT('Ctrl Pts',(10.0343926209999,12.2,-3.11769886700001));
#184105=CARTESIAN_POINT('Ctrl Pts',(10.0328471999999,12.2,-3.11689152500001));
#184106=CARTESIAN_POINT('Ctrl Pts',(10.0313077479999,12.2,-3.11608911700001));
#184107=CARTESIAN_POINT('Ctrl Pts',(10.0297742879999,12.2,-3.11529163800001));
#184108=CARTESIAN_POINT('Ctrl Pts',(10.0282468409999,12.2,-3.11449908600002));
#184109=CARTESIAN_POINT('Ctrl Pts',(10.0267254279999,12.2,-3.11371145700001));
#184110=CARTESIAN_POINT('Ctrl Pts',(10.0252100719999,12.2,-3.11292874700001));
#184111=CARTESIAN_POINT('Ctrl Pts',(10.0237007949999,12.2,-3.11215095500001));
#184112=CARTESIAN_POINT('Ctrl Pts',(10.0221976149999,12.2,-3.11137807500002));
#184113=CARTESIAN_POINT('Ctrl Pts',(10.0207005589999,12.2,-3.11061010400001));
#184114=CARTESIAN_POINT('Ctrl Pts',(10.0192096459999,12.2,-3.10984703900001));
#184115=CARTESIAN_POINT('Ctrl Pts',(10.0177248989999,12.2,-3.10908887700001));
#184116=CARTESIAN_POINT('Ctrl Pts',(10.0162463389999,12.2,-3.10833561400001));
#184117=CARTESIAN_POINT('Ctrl Pts',(10.0147739889999,12.2,-3.10758724500001));
#184118=CARTESIAN_POINT('Ctrl Pts',(10.0133078739999,12.2,-3.10684376900001));
#184119=CARTESIAN_POINT('Ctrl Pts',(10.0118480119999,12.2,-3.10610517900002));
#184120=CARTESIAN_POINT('Ctrl Pts',(10.0103944279999,12.2,-3.10537147600002));
#184121=CARTESIAN_POINT('Ctrl Pts',(10.0089471439999,12.2,-3.10464265200002));
#184122=CARTESIAN_POINT('Ctrl Pts',(10.0075061829999,12.2,-3.10391870500001));
#184123=CARTESIAN_POINT('Ctrl Pts',(10.0060715669999,12.2,-3.10319963200001));
#184124=CARTESIAN_POINT('Ctrl Pts',(10.0046433189999,12.2,-3.10248542800001));
#184125=CARTESIAN_POINT('Ctrl Pts',(10.0032214629999,12.2,-3.10177609000001));
#184126=CARTESIAN_POINT('Ctrl Pts',(10.0018060209999,12.2,-3.10107161300001));
#184127=CARTESIAN_POINT('Ctrl Pts',(10.0003970159999,12.2,-3.10037199500002));
#184128=CARTESIAN_POINT('Ctrl Pts',(9.99899447199994,12.2,-3.09967723100002));
#184129=CARTESIAN_POINT('Ctrl Pts',(9.99759841199995,12.2,-3.09898731700001));
#184130=CARTESIAN_POINT('Ctrl Pts',(9.99620885899994,12.2,-3.09830225000002));
#184131=CARTESIAN_POINT('Ctrl Pts',(9.99482583599995,12.2,-3.09762202400002));
#184132=CARTESIAN_POINT('Ctrl Pts',(9.99344936799995,12.2,-3.09694663700002));
#184133=CARTESIAN_POINT('Ctrl Pts',(9.99207947699994,12.2,-3.09627608500001));
#184134=CARTESIAN_POINT('Ctrl Pts',(9.99071618799995,12.2,-3.09561036200002));
#184135=CARTESIAN_POINT('Ctrl Pts',(9.98935952599994,12.2,-3.09494946600001));
#184136=CARTESIAN_POINT('Ctrl Pts',(9.98800951199994,12.2,-3.09429339200001));
#184137=CARTESIAN_POINT('Ctrl Pts',(9.98666617099994,12.2,-3.09364213600002));
#184138=CARTESIAN_POINT('Ctrl Pts',(9.98532952799994,12.2,-3.09299569400002));
#184139=CARTESIAN_POINT('Ctrl Pts',(9.98399960699994,12.2,-3.09235406000001));
#184140=CARTESIAN_POINT('Ctrl Pts',(9.98267643199994,12.2,-3.09171723300001));
#184141=CARTESIAN_POINT('Ctrl Pts',(9.98136002599994,12.2,-3.09108520600001));
#184142=CARTESIAN_POINT('Ctrl Pts',(9.98005041699994,12.2,-3.09045797700001));
#184143=CARTESIAN_POINT('Ctrl Pts',(9.97874762699994,12.2,-3.08983553900001));
#184144=CARTESIAN_POINT('Ctrl Pts',(9.97745168099994,12.2,-3.08921789100001));
#184145=CARTESIAN_POINT('Ctrl Pts',(9.97616260499995,12.2,-3.08860502500002));
#184146=CARTESIAN_POINT('Ctrl Pts',(9.97488042199994,12.2,-3.08799693900002));
#184147=CARTESIAN_POINT('Ctrl Pts',(9.97360515799994,12.2,-3.08739362900001));
#184148=CARTESIAN_POINT('Ctrl Pts',(9.97233683899994,12.2,-3.08679508900001));
#184149=CARTESIAN_POINT('Ctrl Pts',(9.97107548799995,12.2,-3.08620131400001));
#184150=CARTESIAN_POINT('Ctrl Pts',(9.96982113299994,12.2,-3.08561230000001));
#184151=CARTESIAN_POINT('Ctrl Pts',(9.96857379799994,12.2,-3.08502804400002));
#184152=CARTESIAN_POINT('Ctrl Pts',(9.96733350799994,12.2,-3.08444853900002));
#184153=CARTESIAN_POINT('Ctrl Pts',(9.96610028899994,12.2,-3.08387378200001));
#184154=CARTESIAN_POINT('Ctrl Pts',(9.96487416899994,12.2,-3.08330376800001));
#184155=CARTESIAN_POINT('Ctrl Pts',(9.96365516999995,12.2,-3.08273849300001));
#184156=CARTESIAN_POINT('Ctrl Pts',(9.96244331999995,12.2,-3.08217795000001));
#184157=CARTESIAN_POINT('Ctrl Pts',(9.96123864599994,12.2,-3.08162213600002));
#184158=CARTESIAN_POINT('Ctrl Pts',(9.96004117299995,12.2,-3.08107104600001));
#184159=CARTESIAN_POINT('Ctrl Pts',(9.95885092599995,12.2,-3.08052467500001));
#184160=CARTESIAN_POINT('Ctrl Pts',(9.95766793399994,12.2,-3.07998301700001));
#184161=CARTESIAN_POINT('Ctrl Pts',(9.95649222199994,12.2,-3.07944607000001));
#184162=CARTESIAN_POINT('Ctrl Pts',(9.95532381799995,12.2,-3.07891382600001));
#184163=CARTESIAN_POINT('Ctrl Pts',(9.95416274699994,12.2,-3.07838628200001));
#184164=CARTESIAN_POINT('Ctrl Pts',(9.95300903599994,12.2,-3.07786343200001));
#184165=CARTESIAN_POINT('Ctrl Pts',(9.95186271399995,12.2,-3.07734527000001));
#184166=CARTESIAN_POINT('Ctrl Pts',(9.95072380599994,12.2,-3.07683179400001));
#184167=CARTESIAN_POINT('Ctrl Pts',(9.94959233999994,12.2,-3.07632299600002));
#184168=CARTESIAN_POINT('Ctrl Pts',(9.94846834299994,12.2,-3.07581887100001));
#184169=CARTESIAN_POINT('Ctrl Pts',(9.94735184299994,12.2,-3.07531941600002));
#184170=CARTESIAN_POINT('Ctrl Pts',(9.94624286799995,12.2,-3.07482462300001));
#184171=CARTESIAN_POINT('Ctrl Pts',(9.94514144399995,12.2,-3.07433448900001));
#184172=CARTESIAN_POINT('Ctrl Pts',(9.94404760099994,12.2,-3.07384900800002));
#184173=CARTESIAN_POINT('Ctrl Pts',(9.94296136499995,12.2,-3.07336817300001));
#184174=CARTESIAN_POINT('Ctrl Pts',(9.94188276499995,12.2,-3.07289198100001));
#184175=CARTESIAN_POINT('Ctrl Pts',(9.94081182899994,12.2,-3.07242042600001));
#184176=CARTESIAN_POINT('Ctrl Pts',(9.93974858499995,12.2,-3.07195350200002));
#184177=CARTESIAN_POINT('Ctrl Pts',(9.93869306299995,12.2,-3.07149120200001));
#184178=CARTESIAN_POINT('Ctrl Pts',(9.93764528999994,12.2,-3.07103352400001));
#184179=CARTESIAN_POINT('Ctrl Pts',(9.93660529499994,12.2,-3.07058045900002));
#184180=CARTESIAN_POINT('Ctrl Pts',(9.93557310799994,12.2,-3.07013200400001));
#184181=CARTESIAN_POINT('Ctrl Pts',(9.93454875699994,12.2,-3.06968815200001));
#184182=CARTESIAN_POINT('Ctrl Pts',(9.93353226999995,12.2,-3.06924889800001));
#184183=CARTESIAN_POINT('Ctrl Pts',(9.93252367799995,12.2,-3.06881423400001));
#184184=CARTESIAN_POINT('Ctrl Pts',(9.93152301099995,12.2,-3.06838415800001));
#184185=CARTESIAN_POINT('Ctrl Pts',(9.93053029599994,12.2,-3.06795866100002));
#184186=CARTESIAN_POINT('Ctrl Pts',(9.92954556499994,12.2,-3.06753773800001));
#184187=CARTESIAN_POINT('Ctrl Pts',(9.92856884499994,12.2,-3.06712138300002));
#184188=CARTESIAN_POINT('Ctrl Pts',(9.92760016999994,12.2,-3.06670959200002));
#184189=CARTESIAN_POINT('Ctrl Pts',(9.92663956699994,12.2,-3.06630235600001));
#184190=CARTESIAN_POINT('Ctrl Pts',(9.92568706699995,12.2,-3.06589967100001));
#184191=CARTESIAN_POINT('Ctrl Pts',(9.92474269999994,12.2,-3.06550153000002));
#184192=CARTESIAN_POINT('Ctrl Pts',(9.92380649799994,12.2,-3.06510792800001));
#184193=CARTESIAN_POINT('Ctrl Pts',(9.92287849099995,12.2,-3.06471885700002));
#184194=CARTESIAN_POINT('Ctrl Pts',(9.92195870799994,12.2,-3.06433431200002));
#184195=CARTESIAN_POINT('Ctrl Pts',(9.92104718299995,12.2,-3.06395428600001));
#184196=CARTESIAN_POINT('Ctrl Pts',(9.92014394399994,12.2,-3.06357877400002));
#184197=CARTESIAN_POINT('Ctrl Pts',(9.91924902499994,12.2,-3.06320776900002));
#184198=CARTESIAN_POINT('Ctrl Pts',(9.91836245599995,12.2,-3.06284126300001));
#184199=CARTESIAN_POINT('Ctrl Pts',(9.91748426799995,12.2,-3.06247925400001));
#184200=CARTESIAN_POINT('Ctrl Pts',(9.91661449399994,12.2,-3.06212173000001));
#184201=CARTESIAN_POINT('Ctrl Pts',(9.91575316499994,12.2,-3.06176868700001));
#184202=CARTESIAN_POINT('Ctrl Pts',(9.91490522599995,12.2,-3.06142212700002));
#184203=CARTESIAN_POINT('Ctrl Pts',(9.91423456699994,12.2,-3.06114880300001));
#184204=CARTESIAN_POINT('Ctrl Pts',(9.91373655899995,12.2,-3.06094627500002));
#184205=CARTESIAN_POINT('Ctrl Pts',(9.91340782499995,12.2,-3.06081277600001));
#184206=CARTESIAN_POINT('Ctrl Pts',(9.91324626499994,12.2,-3.06074721200002));
#184207=CARTESIAN_POINT('Ctrl Pts',(9.91324626499994,15.2,-3.06074721200002));
#184208=CARTESIAN_POINT('Ctrl Pts',(9.91340782499995,15.2,-3.06081277600001));
#184209=CARTESIAN_POINT('Ctrl Pts',(9.91373655899995,15.2,-3.06094627500002));
#184210=CARTESIAN_POINT('Ctrl Pts',(9.91423456699994,15.2,-3.06114880300001));
#184211=CARTESIAN_POINT('Ctrl Pts',(9.91490522599995,15.2,-3.06142212700002));
#184212=CARTESIAN_POINT('Ctrl Pts',(9.91575316499994,15.2,-3.06176868700001));
#184213=CARTESIAN_POINT('Ctrl Pts',(9.91661449399994,15.2,-3.06212173000001));
#184214=CARTESIAN_POINT('Ctrl Pts',(9.91748426799995,15.2,-3.06247925400001));
#184215=CARTESIAN_POINT('Ctrl Pts',(9.91836245599995,15.2,-3.06284126300001));
#184216=CARTESIAN_POINT('Ctrl Pts',(9.91924902499994,15.2,-3.06320776900002));
#184217=CARTESIAN_POINT('Ctrl Pts',(9.92014394399994,15.2,-3.06357877400002));
#184218=CARTESIAN_POINT('Ctrl Pts',(9.92104718299995,15.2,-3.06395428600001));
#184219=CARTESIAN_POINT('Ctrl Pts',(9.92195870799994,15.2,-3.06433431200002));
#184220=CARTESIAN_POINT('Ctrl Pts',(9.92287849099995,15.2,-3.06471885700002));
#184221=CARTESIAN_POINT('Ctrl Pts',(9.92380649799994,15.2,-3.06510792800001));
#184222=CARTESIAN_POINT('Ctrl Pts',(9.92474269999994,15.2,-3.06550153000002));
#184223=CARTESIAN_POINT('Ctrl Pts',(9.92568706699995,15.2,-3.06589967100001));
#184224=CARTESIAN_POINT('Ctrl Pts',(9.92663956699994,15.2,-3.06630235600001));
#184225=CARTESIAN_POINT('Ctrl Pts',(9.92760016999994,15.2,-3.06670959200002));
#184226=CARTESIAN_POINT('Ctrl Pts',(9.92856884499994,15.2,-3.06712138300002));
#184227=CARTESIAN_POINT('Ctrl Pts',(9.92954556499994,15.2,-3.06753773800001));
#184228=CARTESIAN_POINT('Ctrl Pts',(9.93053029599994,15.2,-3.06795866100002));
#184229=CARTESIAN_POINT('Ctrl Pts',(9.93152301099995,15.2,-3.06838415800001));
#184230=CARTESIAN_POINT('Ctrl Pts',(9.93252367799995,15.2,-3.06881423400001));
#184231=CARTESIAN_POINT('Ctrl Pts',(9.93353226999995,15.2,-3.06924889800001));
#184232=CARTESIAN_POINT('Ctrl Pts',(9.93454875699994,15.2,-3.06968815200001));
#184233=CARTESIAN_POINT('Ctrl Pts',(9.93557310799994,15.2,-3.07013200400001));
#184234=CARTESIAN_POINT('Ctrl Pts',(9.93660529499994,15.2,-3.07058045900002));
#184235=CARTESIAN_POINT('Ctrl Pts',(9.93764528999994,15.2,-3.07103352400001));
#184236=CARTESIAN_POINT('Ctrl Pts',(9.93869306299995,15.2,-3.07149120200001));
#184237=CARTESIAN_POINT('Ctrl Pts',(9.93974858499995,15.2,-3.07195350200002));
#184238=CARTESIAN_POINT('Ctrl Pts',(9.94081182899994,15.2,-3.07242042600001));
#184239=CARTESIAN_POINT('Ctrl Pts',(9.94188276499995,15.2,-3.07289198100001));
#184240=CARTESIAN_POINT('Ctrl Pts',(9.94296136499995,15.2,-3.07336817300001));
#184241=CARTESIAN_POINT('Ctrl Pts',(9.94404760099994,15.2,-3.07384900800002));
#184242=CARTESIAN_POINT('Ctrl Pts',(9.94514144399995,15.2,-3.07433448900001));
#184243=CARTESIAN_POINT('Ctrl Pts',(9.94624286799995,15.2,-3.07482462300001));
#184244=CARTESIAN_POINT('Ctrl Pts',(9.94735184299994,15.2,-3.07531941600002));
#184245=CARTESIAN_POINT('Ctrl Pts',(9.94846834299994,15.2,-3.07581887100001));
#184246=CARTESIAN_POINT('Ctrl Pts',(9.94959233999994,15.2,-3.07632299600002));
#184247=CARTESIAN_POINT('Ctrl Pts',(9.95072380599994,15.2,-3.07683179400001));
#184248=CARTESIAN_POINT('Ctrl Pts',(9.95186271399995,15.2,-3.07734527000001));
#184249=CARTESIAN_POINT('Ctrl Pts',(9.95300903599994,15.2,-3.07786343200001));
#184250=CARTESIAN_POINT('Ctrl Pts',(9.95416274699994,15.2,-3.07838628200001));
#184251=CARTESIAN_POINT('Ctrl Pts',(9.95532381799995,15.2,-3.07891382600001));
#184252=CARTESIAN_POINT('Ctrl Pts',(9.95649222199994,15.2,-3.07944607000001));
#184253=CARTESIAN_POINT('Ctrl Pts',(9.95766793399994,15.2,-3.07998301700001));
#184254=CARTESIAN_POINT('Ctrl Pts',(9.95885092599995,15.2,-3.08052467500001));
#184255=CARTESIAN_POINT('Ctrl Pts',(9.96004117299995,15.2,-3.08107104600001));
#184256=CARTESIAN_POINT('Ctrl Pts',(9.96123864599994,15.2,-3.08162213600002));
#184257=CARTESIAN_POINT('Ctrl Pts',(9.96244331999995,15.2,-3.08217795000001));
#184258=CARTESIAN_POINT('Ctrl Pts',(9.96365516999995,15.2,-3.08273849300001));
#184259=CARTESIAN_POINT('Ctrl Pts',(9.96487416899994,15.2,-3.08330376800001));
#184260=CARTESIAN_POINT('Ctrl Pts',(9.96610028899994,15.2,-3.08387378200001));
#184261=CARTESIAN_POINT('Ctrl Pts',(9.96733350799994,15.2,-3.08444853900002));
#184262=CARTESIAN_POINT('Ctrl Pts',(9.96857379799994,15.2,-3.08502804400002));
#184263=CARTESIAN_POINT('Ctrl Pts',(9.96982113299994,15.2,-3.08561230000001));
#184264=CARTESIAN_POINT('Ctrl Pts',(9.97107548799995,15.2,-3.08620131400001));
#184265=CARTESIAN_POINT('Ctrl Pts',(9.97233683899994,15.2,-3.08679508900001));
#184266=CARTESIAN_POINT('Ctrl Pts',(9.97360515799994,15.2,-3.08739362900001));
#184267=CARTESIAN_POINT('Ctrl Pts',(9.97488042199994,15.2,-3.08799693900002));
#184268=CARTESIAN_POINT('Ctrl Pts',(9.97616260499995,15.2,-3.08860502500002));
#184269=CARTESIAN_POINT('Ctrl Pts',(9.97745168099994,15.2,-3.08921789100001));
#184270=CARTESIAN_POINT('Ctrl Pts',(9.97874762699994,15.2,-3.08983553900001));
#184271=CARTESIAN_POINT('Ctrl Pts',(9.98005041699994,15.2,-3.09045797700001));
#184272=CARTESIAN_POINT('Ctrl Pts',(9.98136002599994,15.2,-3.09108520600001));
#184273=CARTESIAN_POINT('Ctrl Pts',(9.98267643199994,15.2,-3.09171723300001));
#184274=CARTESIAN_POINT('Ctrl Pts',(9.98399960699994,15.2,-3.09235406000001));
#184275=CARTESIAN_POINT('Ctrl Pts',(9.98532952799994,15.2,-3.09299569400002));
#184276=CARTESIAN_POINT('Ctrl Pts',(9.98666617099994,15.2,-3.09364213600002));
#184277=CARTESIAN_POINT('Ctrl Pts',(9.98800951199994,15.2,-3.09429339200001));
#184278=CARTESIAN_POINT('Ctrl Pts',(9.98935952599994,15.2,-3.09494946600001));
#184279=CARTESIAN_POINT('Ctrl Pts',(9.99071618799995,15.2,-3.09561036200002));
#184280=CARTESIAN_POINT('Ctrl Pts',(9.99207947699994,15.2,-3.09627608500001));
#184281=CARTESIAN_POINT('Ctrl Pts',(9.99344936799995,15.2,-3.09694663700002));
#184282=CARTESIAN_POINT('Ctrl Pts',(9.99482583599995,15.2,-3.09762202400002));
#184283=CARTESIAN_POINT('Ctrl Pts',(9.99620885899994,15.2,-3.09830225000002));
#184284=CARTESIAN_POINT('Ctrl Pts',(9.99759841199995,15.2,-3.09898731700001));
#184285=CARTESIAN_POINT('Ctrl Pts',(9.99899447199994,15.2,-3.09967723100002));
#184286=CARTESIAN_POINT('Ctrl Pts',(10.0003970159999,15.2,-3.10037199500002));
#184287=CARTESIAN_POINT('Ctrl Pts',(10.0018060209999,15.2,-3.10107161300001));
#184288=CARTESIAN_POINT('Ctrl Pts',(10.0032214629999,15.2,-3.10177609000001));
#184289=CARTESIAN_POINT('Ctrl Pts',(10.0046433189999,15.2,-3.10248542800001));
#184290=CARTESIAN_POINT('Ctrl Pts',(10.0060715669999,15.2,-3.10319963200001));
#184291=CARTESIAN_POINT('Ctrl Pts',(10.0075061829999,15.2,-3.10391870500001));
#184292=CARTESIAN_POINT('Ctrl Pts',(10.0089471439999,15.2,-3.10464265200002));
#184293=CARTESIAN_POINT('Ctrl Pts',(10.0103944279999,15.2,-3.10537147600002));
#184294=CARTESIAN_POINT('Ctrl Pts',(10.0118480119999,15.2,-3.10610517900002));
#184295=CARTESIAN_POINT('Ctrl Pts',(10.0133078739999,15.2,-3.10684376900001));
#184296=CARTESIAN_POINT('Ctrl Pts',(10.0147739889999,15.2,-3.10758724500001));
#184297=CARTESIAN_POINT('Ctrl Pts',(10.0162463389999,15.2,-3.10833561400001));
#184298=CARTESIAN_POINT('Ctrl Pts',(10.0177248989999,15.2,-3.10908887700001));
#184299=CARTESIAN_POINT('Ctrl Pts',(10.0192096459999,15.2,-3.10984703900001));
#184300=CARTESIAN_POINT('Ctrl Pts',(10.0207005589999,15.2,-3.11061010400001));
#184301=CARTESIAN_POINT('Ctrl Pts',(10.0221976149999,15.2,-3.11137807500002));
#184302=CARTESIAN_POINT('Ctrl Pts',(10.0237007949999,15.2,-3.11215095500001));
#184303=CARTESIAN_POINT('Ctrl Pts',(10.0252100719999,15.2,-3.11292874700001));
#184304=CARTESIAN_POINT('Ctrl Pts',(10.0267254279999,15.2,-3.11371145700001));
#184305=CARTESIAN_POINT('Ctrl Pts',(10.0282468409999,15.2,-3.11449908600002));
#184306=CARTESIAN_POINT('Ctrl Pts',(10.0297742879999,15.2,-3.11529163800001));
#184307=CARTESIAN_POINT('Ctrl Pts',(10.0313077479999,15.2,-3.11608911700001));
#184308=CARTESIAN_POINT('Ctrl Pts',(10.0328471999999,15.2,-3.11689152500001));
#184309=CARTESIAN_POINT('Ctrl Pts',(10.0343926209999,15.2,-3.11769886700001));
#184310=CARTESIAN_POINT('Ctrl Pts',(10.0359439909999,15.2,-3.11851114600001));
#184311=CARTESIAN_POINT('Ctrl Pts',(10.0375012879999,15.2,-3.11932836300001));
#184312=CARTESIAN_POINT('Ctrl Pts',(10.0390644919999,15.2,-3.12015052400001));
#184313=CARTESIAN_POINT('Ctrl Pts',(10.0406335799999,15.2,-3.12097763100001));
#184314=CARTESIAN_POINT('Ctrl Pts',(10.0422085329999,15.2,-3.12180968700002));
#184315=CARTESIAN_POINT('Ctrl Pts',(10.0437893269999,15.2,-3.12264669700001));
#184316=CARTESIAN_POINT('Ctrl Pts',(10.0453759449999,15.2,-3.12348866100002));
#184317=CARTESIAN_POINT('Ctrl Pts',(10.0469683629999,15.2,-3.12433558500001));
#184318=CARTESIAN_POINT('Ctrl Pts',(10.0485665629999,15.2,-3.12518747000002));
#184319=CARTESIAN_POINT('Ctrl Pts',(10.0501705219999,15.2,-3.12604432200001));
#184320=CARTESIAN_POINT('Ctrl Pts',(10.0517802179999,15.2,-3.12690614000001));
#184321=CARTESIAN_POINT('Ctrl Pts',(10.0533956349999,15.2,-3.12777293000002));
#184322=CARTESIAN_POINT('Ctrl Pts',(10.0550167499999,15.2,-3.12864469400001));
#184323=CARTESIAN_POINT('Ctrl Pts',(10.0566435409999,15.2,-3.12952143500001));
#184324=CARTESIAN_POINT('Ctrl Pts',(10.0582759909999,15.2,-3.13040315700002));
#184325=CARTESIAN_POINT('Ctrl Pts',(10.0599140779999,15.2,-3.13128986000001));
#184326=CARTESIAN_POINT('Ctrl Pts',(10.0615577799999,15.2,-3.13218155100001));
#184327=CARTESIAN_POINT('Ctrl Pts',(10.0632070809999,15.2,-3.13307822900001));
#184328=CARTESIAN_POINT('Ctrl Pts',(10.0648619579999,15.2,-3.13397990000002));
#184329=CARTESIAN_POINT('Ctrl Pts',(10.0665223919999,15.2,-3.13488656500001));
#184330=CARTESIAN_POINT('Ctrl Pts',(10.0681883619999,15.2,-3.13579822800001));
#184331=CARTESIAN_POINT('Ctrl Pts',(10.0698598489999,15.2,-3.13671489000001));
#184332=CARTESIAN_POINT('Ctrl Pts',(10.0715368339999,15.2,-3.13763655600001));
#184333=CARTESIAN_POINT('Ctrl Pts',(10.0732192959999,15.2,-3.13856322800001));
#184334=CARTESIAN_POINT('Ctrl Pts',(10.0749072159999,15.2,-3.13949490700002));
#184335=CARTESIAN_POINT('Ctrl Pts',(10.0766005729999,15.2,-3.14043159900002));
#184336=CARTESIAN_POINT('Ctrl Pts',(10.0782993499999,15.2,-3.14137330300001));
#184337=CARTESIAN_POINT('Ctrl Pts',(10.0800035259999,15.2,-3.14232002500002));
#184338=CARTESIAN_POINT('Ctrl Pts',(10.0817130829999,15.2,-3.14327176500001));
#184339=CARTESIAN_POINT('Ctrl Pts',(10.0834279989999,15.2,-3.14422852800002));
#184340=CARTESIAN_POINT('Ctrl Pts',(10.0851482559999,15.2,-3.14519031400001));
#184341=CARTESIAN_POINT('Ctrl Pts',(10.0868738369999,15.2,-3.14615712900002));
#184342=CARTESIAN_POINT('Ctrl Pts',(10.0886047199999,15.2,-3.14712897300002));
#184343=CARTESIAN_POINT('Ctrl Pts',(10.0903408869999,15.2,-3.14810584800002));
#184344=CARTESIAN_POINT('Ctrl Pts',(10.0920823179999,15.2,-3.14908775800002));
#184345=CARTESIAN_POINT('Ctrl Pts',(10.0938289959999,15.2,-3.15007470700001));
#184346=CARTESIAN_POINT('Ctrl Pts',(10.0955808999999,15.2,-3.15106669300001));
#184347=CARTESIAN_POINT('Ctrl Pts',(10.0973380129999,15.2,-3.15206372300001));
#184348=CARTESIAN_POINT('Ctrl Pts',(10.0991003149999,15.2,-3.15306579700001));
#184349=CARTESIAN_POINT('Ctrl Pts',(10.1008677879999,15.2,-3.15407291900001));
#184350=CARTESIAN_POINT('Ctrl Pts',(10.1026404129999,15.2,-3.15508509000002));
#184351=CARTESIAN_POINT('Ctrl Pts',(10.1044181719999,15.2,-3.15610231100001));
#184352=CARTESIAN_POINT('Ctrl Pts',(10.1062010459999,15.2,-3.15712458800002));
#184353=CARTESIAN_POINT('Ctrl Pts',(10.1079890159999,15.2,-3.15815192100001));
#184354=CARTESIAN_POINT('Ctrl Pts',(10.1097820639999,15.2,-3.15918431300001));
#184355=CARTESIAN_POINT('Ctrl Pts',(10.1115801729999,15.2,-3.16022176700002));
#184356=CARTESIAN_POINT('Ctrl Pts',(10.1133833219999,15.2,-3.16126428300001));
#184357=CARTESIAN_POINT('Ctrl Pts',(10.1151914959999,15.2,-3.16231186600001));
#184358=CARTESIAN_POINT('Ctrl Pts',(10.1170046749999,15.2,-3.16336451600002));
#184359=CARTESIAN_POINT('Ctrl Pts',(10.1188228389999,15.2,-3.16442223800002));
#184360=CARTESIAN_POINT('Ctrl Pts',(10.1206459739999,15.2,-3.16548503000002));
#184361=CARTESIAN_POINT('Ctrl Pts',(10.1224740599999,15.2,-3.16655289800002));
#184362=CARTESIAN_POINT('Ctrl Pts',(10.1243070779999,15.2,-3.16762584300001));
#184363=CARTESIAN_POINT('Ctrl Pts',(10.1261450119999,15.2,-3.16870386600002));
#184364=CARTESIAN_POINT('Ctrl Pts',(10.1279878419999,15.2,-3.16978697100001));
#184365=CARTESIAN_POINT('Ctrl Pts',(10.1298355529999,15.2,-3.17087516000001));
#184366=CARTESIAN_POINT('Ctrl Pts',(10.1316881249999,15.2,-3.17196843300001));
#184367=CARTESIAN_POINT('Ctrl Pts',(10.1335455409999,15.2,-3.17306679400001));
#184368=CARTESIAN_POINT('Ctrl Pts',(10.1354077839999,15.2,-3.17417024400001));
#184369=CARTESIAN_POINT('Ctrl Pts',(10.1372748349999,15.2,-3.17527878600002));
#184370=CARTESIAN_POINT('Ctrl Pts',(10.1391466789999,15.2,-3.17639242200002));
#184371=CARTESIAN_POINT('Ctrl Pts',(10.1410232959999,15.2,-3.17751115200001));
#184372=CARTESIAN_POINT('Ctrl Pts',(10.1429046699999,15.2,-3.17863498200001));
#184373=CARTESIAN_POINT('Ctrl Pts',(10.1447907829999,15.2,-3.17976391000002));
#184374=CARTESIAN_POINT('Ctrl Pts',(10.1466816179999,15.2,-3.18089793900001));
#184375=CARTESIAN_POINT('Ctrl Pts',(10.1485771589999,15.2,-3.18203707400002));
#184376=CARTESIAN_POINT('Ctrl Pts',(10.1504773859999,15.2,-3.18318131200002));
#184377=CARTESIAN_POINT('Ctrl Pts',(10.1523822839999,15.2,-3.18433065800001));
#184378=CARTESIAN_POINT('Ctrl Pts',(10.1542918349999,15.2,-3.18548511300001));
#184379=CARTESIAN_POINT('Ctrl Pts',(10.1562060229999,15.2,-3.18664468000001));
#184380=CARTESIAN_POINT('Ctrl Pts',(10.1581248299999,15.2,-3.18780935900001));
#184381=CARTESIAN_POINT('Ctrl Pts',(10.1600482389999,15.2,-3.18897915400001));
#184382=CARTESIAN_POINT('Ctrl Pts',(10.1619762339999,15.2,-3.19015406500001));
#184383=CARTESIAN_POINT('Ctrl Pts',(10.1639087969999,15.2,-3.19133409300001));
#184384=CARTESIAN_POINT('Ctrl Pts',(10.1658459129999,15.2,-3.19251924300001));
#184385=CARTESIAN_POINT('Ctrl Pts',(10.1677875629999,15.2,-3.19370951400002));
#184386=CARTESIAN_POINT('Ctrl Pts',(10.1697337309999,15.2,-3.19490490900002));
#184387=CARTESIAN_POINT('Ctrl Pts',(10.1716844029999,15.2,-3.19610542900001));
#184388=CARTESIAN_POINT('Ctrl Pts',(10.1736395589999,15.2,-3.19731107700001));
#184389=CARTESIAN_POINT('Ctrl Pts',(10.1755991829999,15.2,-3.19852185400002));
#184390=CARTESIAN_POINT('Ctrl Pts',(10.1775632609999,15.2,-3.19973776100001));
#184391=CARTESIAN_POINT('Ctrl Pts',(10.1795317729999,15.2,-3.20095880100002));
#184392=CARTESIAN_POINT('Ctrl Pts',(10.1815047049999,15.2,-3.20218497500001));
#184393=CARTESIAN_POINT('Ctrl Pts',(10.1834820399999,15.2,-3.20341628300001));
#184394=CARTESIAN_POINT('Ctrl Pts',(10.1854637609999,15.2,-3.20465272900002));
#184395=CARTESIAN_POINT('Ctrl Pts',(10.1874498539999,15.2,-3.20589431400002));
#184396=CARTESIAN_POINT('Ctrl Pts',(10.1894402999999,15.2,-3.20714104000002));
#184397=CARTESIAN_POINT('Ctrl Pts',(10.1914350849999,15.2,-3.20839290800001));
#184398=CARTESIAN_POINT('Ctrl Pts',(10.1934341909999,15.2,-3.20964991800002));
#184399=CARTESIAN_POINT('Ctrl Pts',(10.1954376039999,15.2,-3.21091207400002));
#184400=CARTESIAN_POINT('Ctrl Pts',(10.1974453069999,15.2,-3.21217937700002));
#184401=CARTESIAN_POINT('Ctrl Pts',(10.1994572829999,15.2,-3.21345182800002));
#184402=CARTESIAN_POINT('Ctrl Pts',(10.2014735169999,15.2,-3.21472942900002));
#184403=CARTESIAN_POINT('Ctrl Pts',(10.2034939929999,15.2,-3.21601218000001));
#184404=CARTESIAN_POINT('Ctrl Pts',(10.2055186959999,15.2,-3.21730008500001));
#184405=CARTESIAN_POINT('Ctrl Pts',(10.2075476089999,15.2,-3.21859314200001));
#184406=CARTESIAN_POINT('Ctrl Pts',(10.2095807169999,15.2,-3.21989135600001));
#184407=CARTESIAN_POINT('Ctrl Pts',(10.2116180039999,15.2,-3.22119472700001));
#184408=CARTESIAN_POINT('Ctrl Pts',(10.2136594529999,15.2,-3.22250325600002));
#184409=CARTESIAN_POINT('Ctrl Pts',(10.2157050509999,15.2,-3.22381694500002));
#184410=CARTESIAN_POINT('Ctrl Pts',(10.2177547809999,15.2,-3.22513579400002));
#184411=CARTESIAN_POINT('Ctrl Pts',(10.2198086269999,15.2,-3.22645980700001));
#184412=CARTESIAN_POINT('Ctrl Pts',(10.2218665749999,15.2,-3.22778898400002));
#184413=CARTESIAN_POINT('Ctrl Pts',(10.2239286079999,15.2,-3.22912332500001));
#184414=CARTESIAN_POINT('Ctrl Pts',(10.2259947109999,15.2,-3.23046283300001));
#184415=CARTESIAN_POINT('Ctrl Pts',(10.2280648689999,15.2,-3.23180750800002));
#184416=CARTESIAN_POINT('Ctrl Pts',(10.2301390659999,15.2,-3.23315735300001));
#184417=CARTESIAN_POINT('Ctrl Pts',(10.2322172889999,15.2,-3.23451236800001));
#184418=CARTESIAN_POINT('Ctrl Pts',(10.2342995189999,15.2,-3.23587255500001));
#184419=CARTESIAN_POINT('Ctrl Pts',(10.2363857439999,15.2,-3.23723791500001));
#184420=CARTESIAN_POINT('Ctrl Pts',(10.2384759469999,15.2,-3.23860844800001));
#184421=CARTESIAN_POINT('Ctrl Pts',(10.2405701139999,15.2,-3.23998415800002));
#184422=CARTESIAN_POINT('Ctrl Pts',(10.2426682289999,15.2,-3.24136504400002));
#184423=CARTESIAN_POINT('Ctrl Pts',(10.2447702779999,15.2,-3.24275110800002));
#184424=CARTESIAN_POINT('Ctrl Pts',(10.2468762449999,15.2,-3.24414235000001));
#184425=CARTESIAN_POINT('Ctrl Pts',(10.2489861149999,15.2,-3.24553877200001));
#184426=CARTESIAN_POINT('Ctrl Pts',(10.2510998739999,15.2,-3.24694037600001));
#184427=CARTESIAN_POINT('Ctrl Pts',(10.2532175069999,15.2,-3.24834716200002));
#184428=CARTESIAN_POINT('Ctrl Pts',(10.2553389979999,15.2,-3.24975913200001));
#184429=CARTESIAN_POINT('Ctrl Pts',(10.2574643339999,15.2,-3.25117628600001));
#184430=CARTESIAN_POINT('Ctrl Pts',(10.2595934979999,15.2,-3.25259862700001));
#184431=CARTESIAN_POINT('Ctrl Pts',(10.2617264769999,15.2,-3.25402615300002));
#184432=CARTESIAN_POINT('Ctrl Pts',(10.2638632559999,15.2,-3.25545886800001));
#184433=CARTESIAN_POINT('Ctrl Pts',(10.2660038209999,15.2,-3.25689677200002));
#184434=CARTESIAN_POINT('Ctrl Pts',(10.2681481549999,15.2,-3.25833986600002));
#184435=CARTESIAN_POINT('Ctrl Pts',(10.2702962469999,15.2,-3.25978815000001));
#184436=CARTESIAN_POINT('Ctrl Pts',(10.2724480789999,15.2,-3.26124162800001));
#184437=CARTESIAN_POINT('Ctrl Pts',(10.2746036379999,15.2,-3.26270029800002));
#184438=CARTESIAN_POINT('Ctrl Pts',(10.2767629099999,15.2,-3.26416416200002));
#184439=CARTESIAN_POINT('Ctrl Pts',(10.2789258799999,15.2,-3.26563322100001));
#184440=CARTESIAN_POINT('Ctrl Pts',(10.2810925339999,15.2,-3.26710747600002));
#184441=CARTESIAN_POINT('Ctrl Pts',(10.2832628569999,15.2,-3.26858692800001));
#184442=CARTESIAN_POINT('Ctrl Pts',(10.2854368349999,15.2,-3.27007157800002));
#184443=CARTESIAN_POINT('Ctrl Pts',(10.2876144549999,15.2,-3.27156142700002));
#184444=CARTESIAN_POINT('Ctrl Pts',(10.2897957009999,15.2,-3.27305647500001));
#184445=CARTESIAN_POINT('Ctrl Pts',(10.2919805579999,15.2,-3.27455672400002));
#184446=CARTESIAN_POINT('Ctrl Pts',(10.2941690149999,15.2,-3.27606217500001));
#184447=CARTESIAN_POINT('Ctrl Pts',(10.2963610559999,15.2,-3.27757282800002));
#184448=CARTESIAN_POINT('Ctrl Pts',(10.2985566669999,15.2,-3.27908868400002));
#184449=CARTESIAN_POINT('Ctrl Pts',(10.3007558329999,15.2,-3.28060974400001));
#184450=CARTESIAN_POINT('Ctrl Pts',(10.3029585419999,15.2,-3.28213601000002));
#184451=CARTESIAN_POINT('Ctrl Pts',(10.3051647789999,15.2,-3.28366748100001));
#184452=CARTESIAN_POINT('Ctrl Pts',(10.3073745299999,15.2,-3.28520415900002));
#184453=CARTESIAN_POINT('Ctrl Pts',(10.3095877799999,15.2,-3.28674604500002));
#184454=CARTESIAN_POINT('Ctrl Pts',(10.3118045179999,15.2,-3.28829313800002));
#184455=CARTESIAN_POINT('Ctrl Pts',(10.3140247269999,15.2,-3.28984544000001));
#184456=CARTESIAN_POINT('Ctrl Pts',(10.3162483959999,15.2,-3.29140295300002));
#184457=CARTESIAN_POINT('Ctrl Pts',(10.3184755079999,15.2,-3.29296567500001));
#184458=CARTESIAN_POINT('Ctrl Pts',(10.3207060529999,15.2,-3.29453360900001));
#184459=CARTESIAN_POINT('Ctrl Pts',(10.3229400139999,15.2,-3.29610675500001));
#184460=CARTESIAN_POINT('Ctrl Pts',(10.3251773799999,15.2,-3.29768511400002));
#184461=CARTESIAN_POINT('Ctrl Pts',(10.3274181339999,15.2,-3.29926868600001));
#184462=CARTESIAN_POINT('Ctrl Pts',(10.3296622669999,15.2,-3.30085747200001));
#184463=CARTESIAN_POINT('Ctrl Pts',(10.3319097619999,15.2,-3.30245147300001));
#184464=CARTESIAN_POINT('Ctrl Pts',(10.3341606059999,15.2,-3.30405069000001));
#184465=CARTESIAN_POINT('Ctrl Pts',(10.3364147869999,15.2,-3.30565512200002));
#184466=CARTESIAN_POINT('Ctrl Pts',(10.3386722889999,15.2,-3.30726477100002));
#184467=CARTESIAN_POINT('Ctrl Pts',(10.3409331009999,15.2,-3.30887963800001));
#184468=CARTESIAN_POINT('Ctrl Pts',(10.3431972079999,15.2,-3.31049972300002));
#184469=CARTESIAN_POINT('Ctrl Pts',(10.3454645979999,15.2,-3.31212502700001));
#184470=CARTESIAN_POINT('Ctrl Pts',(10.3477352559999,15.2,-3.31375555000001));
#184471=CARTESIAN_POINT('Ctrl Pts',(10.3500091699999,15.2,-3.31539129200001));
#184472=CARTESIAN_POINT('Ctrl Pts',(10.3522863269999,15.2,-3.31703225500001));
#184473=CARTESIAN_POINT('Ctrl Pts',(10.3545667119999,15.2,-3.31867843900001));
#184474=CARTESIAN_POINT('Ctrl Pts',(10.3568503129999,15.2,-3.32032984500001));
#184475=CARTESIAN_POINT('Ctrl Pts',(10.3591371169999,15.2,-3.32198647300002));
#184476=CARTESIAN_POINT('Ctrl Pts',(10.3614271109999,15.2,-3.32364832300001));
#184477=CARTESIAN_POINT('Ctrl Pts',(10.3637202799999,15.2,-3.32531539600001));
#184478=CARTESIAN_POINT('Ctrl Pts',(10.3660166129999,15.2,-3.32698769300002));
#184479=CARTESIAN_POINT('Ctrl Pts',(10.3683160969999,15.2,-3.32866521600002));
#184480=CARTESIAN_POINT('Ctrl Pts',(10.3706187169999,15.2,-3.33034796100002));
#184481=CARTESIAN_POINT('Ctrl Pts',(10.3729244619999,15.2,-3.33203593300002));
#184482=CARTESIAN_POINT('Ctrl Pts',(10.3752333189999,15.2,-3.33372913000002));
#184483=CARTESIAN_POINT('Ctrl Pts',(10.3775452729999,15.2,-3.33542755200002));
#184484=CARTESIAN_POINT('Ctrl Pts',(10.3798603139999,15.2,-3.33713120100001));
#184485=CARTESIAN_POINT('Ctrl Pts',(10.3821784259999,15.2,-3.33884007800001));
#184486=CARTESIAN_POINT('Ctrl Pts',(10.3844995979999,15.2,-3.34055418200002));
#184487=CARTESIAN_POINT('Ctrl Pts',(10.3868238179999,15.2,-3.34227351400001));
#184488=CARTESIAN_POINT('Ctrl Pts',(10.3891510709999,15.2,-3.34399807300001));
#184489=CARTESIAN_POINT('Ctrl Pts',(10.3914813469999,15.2,-3.34572786200001));
#184490=CARTESIAN_POINT('Ctrl Pts',(10.3938146309999,15.2,-3.34746287900002));
#184491=CARTESIAN_POINT('Ctrl Pts',(10.3961509099999,15.2,-3.34920312600001));
#184492=CARTESIAN_POINT('Ctrl Pts',(10.3984901739999,15.2,-3.35094860300002));
#184493=CARTESIAN_POINT('Ctrl Pts',(10.4008324069999,15.2,-3.35269930900001));
#184494=CARTESIAN_POINT('Ctrl Pts',(10.4031775999999,15.2,-3.35445524600001));
#184495=CARTESIAN_POINT('Ctrl Pts',(10.4055257379999,15.2,-3.35621641400001));
#184496=CARTESIAN_POINT('Ctrl Pts',(10.4078768069999,15.2,-3.35798281300002));
#184497=CARTESIAN_POINT('Ctrl Pts',(10.4102307989999,15.2,-3.35975444400002));
#184498=CARTESIAN_POINT('Ctrl Pts',(10.4125876979999,15.2,-3.36153130600001));
#184499=CARTESIAN_POINT('Ctrl Pts',(10.4149474929999,15.2,-3.36331340000001));
#184500=CARTESIAN_POINT('Ctrl Pts',(10.4173101699999,15.2,-3.36510072600001));
#184501=CARTESIAN_POINT('Ctrl Pts',(10.4196757189999,15.2,-3.36689328500002));
#184502=CARTESIAN_POINT('Ctrl Pts',(10.4220441259999,15.2,-3.36869107600001));
#184503=CARTESIAN_POINT('Ctrl Pts',(10.4244153789999,15.2,-3.37049410100001));
#184504=CARTESIAN_POINT('Ctrl Pts',(10.4267894639999,15.2,-3.37230235900002));
#184505=CARTESIAN_POINT('Ctrl Pts',(10.4291663729999,15.2,-3.37411585000002));
#184506=CARTESIAN_POINT('Ctrl Pts',(10.4315460899999,15.2,-3.37593457500001));
#184507=CARTESIAN_POINT('Ctrl Pts',(10.4339286029999,15.2,-3.37775853500001));
#184508=CARTESIAN_POINT('Ctrl Pts',(10.4363139019999,15.2,-3.37958772900001));
#184509=CARTESIAN_POINT('Ctrl Pts',(10.4387019739999,15.2,-3.38142215600001));
#184510=CARTESIAN_POINT('Ctrl Pts',(10.4410928049999,15.2,-3.38326181800001));
#184511=CARTESIAN_POINT('Ctrl Pts',(10.4434863849999,15.2,-3.38510671600002));
#184512=CARTESIAN_POINT('Ctrl Pts',(10.4458826999999,15.2,-3.38695684700001));
#184513=CARTESIAN_POINT('Ctrl Pts',(10.4482817399999,15.2,-3.38881221500001));
#184514=CARTESIAN_POINT('Ctrl Pts',(10.4506834919999,15.2,-3.39067281600002));
#184515=CARTESIAN_POINT('Ctrl Pts',(10.4530879439999,15.2,-3.39253865400002));
#184516=CARTESIAN_POINT('Ctrl Pts',(10.4554950839999,15.2,-3.39440972700002));
#184517=CARTESIAN_POINT('Ctrl Pts',(10.4579048999999,15.2,-3.39628603500001));
#184518=CARTESIAN_POINT('Ctrl Pts',(10.4603173799999,15.2,-3.39816757900001));
#184519=CARTESIAN_POINT('Ctrl Pts',(10.4627325119999,15.2,-3.40005435900002));
#184520=CARTESIAN_POINT('Ctrl Pts',(10.4651502849999,15.2,-3.40194637400002));
#184521=CARTESIAN_POINT('Ctrl Pts',(10.4675706859999,15.2,-3.40384362500001));
#184522=CARTESIAN_POINT('Ctrl Pts',(10.4699937039999,15.2,-3.40574611300001));
#184523=CARTESIAN_POINT('Ctrl Pts',(10.4724193259999,15.2,-3.40765383700001));
#184524=CARTESIAN_POINT('Ctrl Pts',(10.4748475419999,15.2,-3.40956679600001));
#184525=CARTESIAN_POINT('Ctrl Pts',(10.4772783389999,15.2,-3.41148499200001));
#184526=CARTESIAN_POINT('Ctrl Pts',(10.4797117049999,15.2,-3.41340842300002));
#184527=CARTESIAN_POINT('Ctrl Pts',(10.4821476289999,15.2,-3.41533709100001));
#184528=CARTESIAN_POINT('Ctrl Pts',(10.4845860999999,15.2,-3.41727099600002));
#184529=CARTESIAN_POINT('Ctrl Pts',(10.4870271039999,15.2,-3.41921013700001));
#184530=CARTESIAN_POINT('Ctrl Pts',(10.4894706319999,15.2,-3.42115451300002));
#184531=CARTESIAN_POINT('Ctrl Pts',(10.4919166709999,15.2,-3.42310412600002));
#184532=CARTESIAN_POINT('Ctrl Pts',(10.4943652099999,15.2,-3.42505897500001));
#184533=CARTESIAN_POINT('Ctrl Pts',(10.4968162359999,15.2,-3.42701906000002));
#184534=CARTESIAN_POINT('Ctrl Pts',(10.4992697399999,15.2,-3.42898438100002));
#184535=CARTESIAN_POINT('Ctrl Pts',(10.5017257079999,15.2,-3.43095493800002));
#184536=CARTESIAN_POINT('Ctrl Pts',(10.5041841299999,15.2,-3.43293073100002));
#184537=CARTESIAN_POINT('Ctrl Pts',(10.5066449939999,15.2,-3.43491176000001));
#184538=CARTESIAN_POINT('Ctrl Pts',(10.5091082899999,15.2,-3.43689802500001));
#184539=CARTESIAN_POINT('Ctrl Pts',(10.5115740039999,15.2,-3.43888952500001));
#184540=CARTESIAN_POINT('Ctrl Pts',(10.5140421269999,15.2,-3.44088626100001));
#184541=CARTESIAN_POINT('Ctrl Pts',(10.5165126449999,15.2,-3.44288823300001));
#184542=CARTESIAN_POINT('Ctrl Pts',(10.5189855499999,15.2,-3.44489544000002));
#184543=CARTESIAN_POINT('Ctrl Pts',(10.5214608269999,15.2,-3.44690788300001));
#184544=CARTESIAN_POINT('Ctrl Pts',(10.5239384669999,15.2,-3.44892556000001));
#184545=CARTESIAN_POINT('Ctrl Pts',(10.5264184599999,15.2,-3.45094847300001));
#184546=CARTESIAN_POINT('Ctrl Pts',(10.5289007929999,15.2,-3.45297662100001));
#184547=CARTESIAN_POINT('Ctrl Pts',(10.5313854529999,15.2,-3.45501000300001));
#184548=CARTESIAN_POINT('Ctrl Pts',(10.5338724319999,15.2,-3.45704862000002));
#184549=CARTESIAN_POINT('Ctrl Pts',(10.5363617169999,15.2,-3.45909247100002));
#184550=CARTESIAN_POINT('Ctrl Pts',(10.5388532969999,15.2,-3.46114155700001));
#184551=CARTESIAN_POINT('Ctrl Pts',(10.5413471629999,15.2,-3.46319587600001));
#184552=CARTESIAN_POINT('Ctrl Pts',(10.5438433009999,15.2,-3.46525543000002));
#184553=CARTESIAN_POINT('Ctrl Pts',(10.5463417019999,15.2,-3.46732021700001));
#184554=CARTESIAN_POINT('Ctrl Pts',(10.5488423529999,15.2,-3.46939023800001));
#184555=CARTESIAN_POINT('Ctrl Pts',(10.5513452449999,15.2,-3.47146549100001));
#184556=CARTESIAN_POINT('Ctrl Pts',(10.5538503639999,15.2,-3.47354597800001));
#184557=CARTESIAN_POINT('Ctrl Pts',(10.5563577029999,15.2,-3.47563169800001));
#184558=CARTESIAN_POINT('Ctrl Pts',(10.5588672479999,15.2,-3.47772265000001));
#184559=CARTESIAN_POINT('Ctrl Pts',(10.5613789899999,15.2,-3.47981883400001));
#184560=CARTESIAN_POINT('Ctrl Pts',(10.5638929169999,15.2,-3.48192025000001));
#184561=CARTESIAN_POINT('Ctrl Pts',(10.5664090179999,15.2,-3.48402689800002));
#184562=CARTESIAN_POINT('Ctrl Pts',(10.5689272829999,15.2,-3.48613877700001));
#184563=CARTESIAN_POINT('Ctrl Pts',(10.5714476989999,15.2,-3.48825588800001));
#184564=CARTESIAN_POINT('Ctrl Pts',(10.5739702579999,15.2,-3.49037822900002));
#184565=CARTESIAN_POINT('Ctrl Pts',(10.5764949479999,15.2,-3.49250580000001));
#184566=CARTESIAN_POINT('Ctrl Pts',(10.5790217569999,15.2,-3.49463860200002));
#184567=CARTESIAN_POINT('Ctrl Pts',(10.5815506769999,15.2,-3.49677663500001));
#184568=CARTESIAN_POINT('Ctrl Pts',(10.5840816949999,15.2,-3.49891989600001));
#184569=CARTESIAN_POINT('Ctrl Pts',(10.5866147999999,15.2,-3.50106838700002));
#184570=CARTESIAN_POINT('Ctrl Pts',(10.5891499829999,15.2,-3.50322210700002));
#184571=CARTESIAN_POINT('Ctrl Pts',(10.5916872319999,15.2,-3.50538105500001));
#184572=CARTESIAN_POINT('Ctrl Pts',(10.5942265379999,15.2,-3.50754523200001));
#184573=CARTESIAN_POINT('Ctrl Pts',(10.5967678879999,15.2,-3.50971463600001));
#184574=CARTESIAN_POINT('Ctrl Pts',(10.5993112729999,15.2,-3.51188926900001));
#184575=CARTESIAN_POINT('Ctrl Pts',(10.6018566829999,15.2,-3.51406912700002));
#184576=CARTESIAN_POINT('Ctrl Pts',(10.6044041049999,15.2,-3.51625421300001));
#184577=CARTESIAN_POINT('Ctrl Pts',(10.6069535309999,15.2,-3.51844452500002));
#184578=CARTESIAN_POINT('Ctrl Pts',(10.6095049489999,15.2,-3.52064006300001));
#184579=CARTESIAN_POINT('Ctrl Pts',(10.6120583479999,15.2,-3.52284082600002));
#184580=CARTESIAN_POINT('Ctrl Pts',(10.6146137189999,15.2,-3.52504681400001));
#184581=CARTESIAN_POINT('Ctrl Pts',(10.6171710509999,15.2,-3.52725802700002));
#184582=CARTESIAN_POINT('Ctrl Pts',(10.6197303339999,15.2,-3.52947446500002));
#184583=CARTESIAN_POINT('Ctrl Pts',(10.6222915559999,15.2,-3.53169612600002));
#184584=CARTESIAN_POINT('Ctrl Pts',(10.6248547079999,15.2,-3.53392301000001));
#184585=CARTESIAN_POINT('Ctrl Pts',(10.6274197799999,15.2,-3.53615511700001));
#184586=CARTESIAN_POINT('Ctrl Pts',(10.6299867589999,15.2,-3.53839244700001));
#184587=CARTESIAN_POINT('Ctrl Pts',(10.6325556389999,15.2,-3.54063499900001));
#184588=CARTESIAN_POINT('Ctrl Pts',(10.6351264049999,15.2,-3.54288277200002));
#184589=CARTESIAN_POINT('Ctrl Pts',(10.6376990499999,15.2,-3.54513576600001));
#184590=CARTESIAN_POINT('Ctrl Pts',(10.6402735619999,15.2,-3.54739398000001));
#184591=CARTESIAN_POINT('Ctrl Pts',(10.6428499309999,15.2,-3.54965741400001));
#184592=CARTESIAN_POINT('Ctrl Pts',(10.6454281479999,15.2,-3.55192606900002));
#184593=CARTESIAN_POINT('Ctrl Pts',(10.6480082019999,15.2,-3.55419994100002));
#184594=CARTESIAN_POINT('Ctrl Pts',(10.6505900819999,15.2,-3.55647903300001));
#184595=CARTESIAN_POINT('Ctrl Pts',(10.6531737789999,15.2,-3.55876334200001));
#184596=CARTESIAN_POINT('Ctrl Pts',(10.6557592819999,15.2,-3.56105286800001));
#184597=CARTESIAN_POINT('Ctrl Pts',(10.6583465819999,15.2,-3.56334761200001));
#184598=CARTESIAN_POINT('Ctrl Pts',(10.6609356659999,15.2,-3.56564757100001));
#184599=CARTESIAN_POINT('Ctrl Pts',(10.6635265279999,15.2,-3.56795274600001));
#184600=CARTESIAN_POINT('Ctrl Pts',(10.6661191539999,15.2,-3.57026313700001));
#184601=CARTESIAN_POINT('Ctrl Pts',(10.6687135369999,15.2,-3.57257874200001));
#184602=CARTESIAN_POINT('Ctrl Pts',(10.6713096659999,15.2,-3.57489956100002));
#184603=CARTESIAN_POINT('Ctrl Pts',(10.6739075299999,15.2,-3.57722559400001));
#184604=CARTESIAN_POINT('Ctrl Pts',(10.6765071199999,15.2,-3.57955683900002));
#184605=CARTESIAN_POINT('Ctrl Pts',(10.6791084249999,15.2,-3.58189329600001));
#184606=CARTESIAN_POINT('Ctrl Pts',(10.6817114369999,15.2,-3.58423496500002));
#184607=CARTESIAN_POINT('Ctrl Pts',(10.6843161429999,15.2,-3.58658184500001));
#184608=CARTESIAN_POINT('Ctrl Pts',(10.6869225359999,15.2,-3.58893393500002));
#184609=CARTESIAN_POINT('Ctrl Pts',(10.6895306049999,15.2,-3.59129123500002));
#184610=CARTESIAN_POINT('Ctrl Pts',(10.6921403399999,15.2,-3.59365374400001));
#184611=CARTESIAN_POINT('Ctrl Pts',(10.6947517299999,15.2,-3.59602146200002));
#184612=CARTESIAN_POINT('Ctrl Pts',(10.6973647669999,15.2,-3.59839438800002));
#184613=CARTESIAN_POINT('Ctrl Pts',(10.6999794399999,15.2,-3.60077252100002));
#184614=CARTESIAN_POINT('Ctrl Pts',(10.7025957399999,15.2,-3.60315585900001));
#184615=CARTESIAN_POINT('Ctrl Pts',(10.7052136559999,15.2,-3.60554440400001));
#184616=CARTESIAN_POINT('Ctrl Pts',(10.7078331809999,15.2,-3.60793815500001));
#184617=CARTESIAN_POINT('Ctrl Pts',(10.7104543019999,15.2,-3.61033710900001));
#184618=CARTESIAN_POINT('Ctrl Pts',(10.7130770099999,15.2,-3.61274126800001));
#184619=CARTESIAN_POINT('Ctrl Pts',(10.7157012959999,15.2,-3.61515062900001));
#184620=CARTESIAN_POINT('Ctrl Pts',(10.7183271499999,15.2,-3.61756519200001));
#184621=CARTESIAN_POINT('Ctrl Pts',(10.7209545619999,15.2,-3.61998495800002));
#184622=CARTESIAN_POINT('Ctrl Pts',(10.7235835239999,15.2,-3.62240992500002));
#184623=CARTESIAN_POINT('Ctrl Pts',(10.7262140239999,15.2,-3.62484009100001));
#184624=CARTESIAN_POINT('Ctrl Pts',(10.7288460529999,15.2,-3.62727545700002));
#184625=CARTESIAN_POINT('Ctrl Pts',(10.7314796019999,15.2,-3.62971602300002));
#184626=CARTESIAN_POINT('Ctrl Pts',(10.7341146619999,15.2,-3.63216178500001));
#184627=CARTESIAN_POINT('Ctrl Pts',(10.7367512209999,15.2,-3.63461274500001));
#184628=CARTESIAN_POINT('Ctrl Pts',(10.7393892719999,15.2,-3.63706890200001));
#184629=CARTESIAN_POINT('Ctrl Pts',(10.7420288039999,15.2,-3.63953025500001));
#184630=CARTESIAN_POINT('Ctrl Pts',(10.7446698079999,15.2,-3.64199680200001));
#184631=CARTESIAN_POINT('Ctrl Pts',(10.7473122739999,15.2,-3.64446854400001));
#184632=CARTESIAN_POINT('Ctrl Pts',(10.7499561929999,15.2,-3.64694547900001));
#184633=CARTESIAN_POINT('Ctrl Pts',(10.7526015559999,15.2,-3.64942760700002));
#184634=CARTESIAN_POINT('Ctrl Pts',(10.7552483519999,15.2,-3.65191492600001));
#184635=CARTESIAN_POINT('Ctrl Pts',(10.7578965719999,15.2,-3.65440743700002));
#184636=CARTESIAN_POINT('Ctrl Pts',(10.7605462079999,15.2,-3.65690513800002));
#184637=CARTESIAN_POINT('Ctrl Pts',(10.7631972489999,15.2,-3.65940802800001));
#184638=CARTESIAN_POINT('Ctrl Pts',(10.7658496859999,15.2,-3.66191610700001));
#184639=CARTESIAN_POINT('Ctrl Pts',(10.7685035109999,15.2,-3.66442937400001));
#184640=CARTESIAN_POINT('Ctrl Pts',(10.7711587129999,15.2,-3.66694782800002));
#184641=CARTESIAN_POINT('Ctrl Pts',(10.7738152829999,15.2,-3.66947146800001));
#184642=CARTESIAN_POINT('Ctrl Pts',(10.7764732109999,15.2,-3.67200029300002));
#184643=CARTESIAN_POINT('Ctrl Pts',(10.7791324889999,15.2,-3.67453430200001));
#184644=CARTESIAN_POINT('Ctrl Pts',(10.7817931069999,15.2,-3.67707349500002));
#184645=CARTESIAN_POINT('Ctrl Pts',(10.7844550569999,15.2,-3.67961787200001));
#184646=CARTESIAN_POINT('Ctrl Pts',(10.7871183259999,15.2,-3.68216742900001));
#184647=CARTESIAN_POINT('Ctrl Pts',(10.7897829079999,15.2,-3.68472216800001));
#184648=CARTESIAN_POINT('Ctrl Pts',(10.7924487949999,15.2,-3.68728208700002));
#184649=CARTESIAN_POINT('Ctrl Pts',(10.7951159729999,15.2,-3.68984718400001));
#184650=CARTESIAN_POINT('Ctrl Pts',(10.7977844379999,15.2,-3.69241746100001));
#184651=CARTESIAN_POINT('Ctrl Pts',(10.8004541779999,15.2,-3.69499291500002));
#184652=CARTESIAN_POINT('Ctrl Pts',(10.8031251839999,15.2,-3.69757354500001));
#184653=CARTESIAN_POINT('Ctrl Pts',(10.8057974489999,15.2,-3.70015935000001));
#184654=CARTESIAN_POINT('Ctrl Pts',(10.8084709609999,15.2,-3.70275033200001));
#184655=CARTESIAN_POINT('Ctrl Pts',(10.8111457129999,15.2,-3.70534648600001));
#184656=CARTESIAN_POINT('Ctrl Pts',(10.8138216939999,15.2,-3.70794781300001));
#184657=CARTESIAN_POINT('Ctrl Pts',(10.8164988939999,15.2,-3.71055431200002));
#184658=CARTESIAN_POINT('Ctrl Pts',(10.8191773059999,15.2,-3.71316598200002));
#184659=CARTESIAN_POINT('Ctrl Pts',(10.8218569179999,15.2,-3.71578282200002));
#184660=CARTESIAN_POINT('Ctrl Pts',(10.8245377239999,15.2,-3.71840483100002));
#184661=CARTESIAN_POINT('Ctrl Pts',(10.8272197149999,15.2,-3.72103200700002));
#184662=CARTESIAN_POINT('Ctrl Pts',(10.8299028829999,15.2,-3.72366435100002));
#184663=CARTESIAN_POINT('Ctrl Pts',(10.8325872199999,15.2,-3.72630186200002));
#184664=CARTESIAN_POINT('Ctrl Pts',(10.8352727169999,15.2,-3.72894453800001));
#184665=CARTESIAN_POINT('Ctrl Pts',(10.8379593649999,15.2,-3.73159237800001));
#184666=CARTESIAN_POINT('Ctrl Pts',(10.8406471529999,15.2,-3.73424538200001));
#184667=CARTESIAN_POINT('Ctrl Pts',(10.8433360699999,15.2,-3.73690354800001));
#184668=CARTESIAN_POINT('Ctrl Pts',(10.8460261069999,15.2,-3.73956687500002));
#184669=CARTESIAN_POINT('Ctrl Pts',(10.8487172499999,15.2,-3.74223536100001));
#184670=CARTESIAN_POINT('Ctrl Pts',(10.8514094899999,15.2,-3.74490900600001));
#184671=CARTESIAN_POINT('Ctrl Pts',(10.8541028209999,15.2,-3.74758780800001));
#184672=CARTESIAN_POINT('Ctrl Pts',(10.8567972349999,15.2,-3.75027176800002));
#184673=CARTESIAN_POINT('Ctrl Pts',(10.8594927299999,15.2,-3.75296088400002));
#184674=CARTESIAN_POINT('Ctrl Pts',(10.8621893019999,15.2,-3.75565515600002));
#184675=CARTESIAN_POINT('Ctrl Pts',(10.8643474199999,15.2,-3.75781469800001));
#184676=CARTESIAN_POINT('Ctrl Pts',(10.8659664939999,15.2,-3.75943667400001));
#184677=CARTESIAN_POINT('Ctrl Pts',(10.8670460909999,15.2,-3.76051902400001));
#184678=CARTESIAN_POINT('Ctrl Pts',(10.8675859439999,15.2,-3.76106045600002));
#184679=CARTESIAN_POINT('Origin',(-5.66257110645729E-14,15.2,-1.77635683940025E-14));
#184680=CARTESIAN_POINT('',(10.0330625574591,15.2,-2.64164356403315));
#184681=CARTESIAN_POINT('',(10.0330625574591,12.2,-2.64164356403315));
#184682=CARTESIAN_POINT('',(10.0330625569999,15.2,-2.64164356400002));
#184683=CARTESIAN_POINT('Origin',(-5.66257110645729E-14,12.2,-1.77635683940025E-14));
#184684=CARTESIAN_POINT('Origin',(-5.66257110645729E-14,15.2,-1.77635683940025E-14));
#184685=CARTESIAN_POINT('Origin',(-5.66257110645729E-14,15.2,-1.77635683940025E-14));
#184686=CARTESIAN_POINT('',(11.2133565919999,15.2,-2.55159439000002));
#184687=CARTESIAN_POINT('',(11.2922242989999,15.2,-2.17615954700001));
#184688=CARTESIAN_POINT('Origin',(-5.66257110645729E-14,15.2,-1.77635683940025E-14));
#184689=CARTESIAN_POINT('',(11.2922242989999,12.2,-2.17615954700001));
#184690=CARTESIAN_POINT('',(11.2922242989999,15.2,-2.17615954700001));
#184691=CARTESIAN_POINT('',(11.2133565919999,12.2,-2.55159439000002));
#184692=CARTESIAN_POINT('Origin',(-5.66257110645729E-14,12.2,-1.77635683940025E-14));
#184693=CARTESIAN_POINT('',(11.2133565919999,15.2,-2.55159439000002));
#184694=CARTESIAN_POINT('Ctrl Pts',(11.2922242989999,15.2,-2.17615954700001));
#184695=CARTESIAN_POINT('Ctrl Pts',(11.2922242989999,11.6,-2.17615954700001));
#184696=CARTESIAN_POINT('Ctrl Pts',(11.2916128879999,15.2,-2.17570045500001));
#184697=CARTESIAN_POINT('Ctrl Pts',(11.2916128879999,11.6,-2.17570045500001));
#184698=CARTESIAN_POINT('Ctrl Pts',(11.2903902449999,15.2,-2.17478276600001));
#184699=CARTESIAN_POINT('Ctrl Pts',(11.2903902449999,11.6,-2.17478276600001));
#184700=CARTESIAN_POINT('Ctrl Pts',(11.2885568199999,15.2,-2.17340771600002));
#184701=CARTESIAN_POINT('Ctrl Pts',(11.2885568199999,11.6,-2.17340771600002));
#184702=CARTESIAN_POINT('Ctrl Pts',(11.2861133329999,15.2,-2.17157728800002));
#184703=CARTESIAN_POINT('Ctrl Pts',(11.2861133329999,11.6,-2.17157728800002));
#184704=CARTESIAN_POINT('Ctrl Pts',(11.2830607729999,15.2,-2.16929420200001));
#184705=CARTESIAN_POINT('Ctrl Pts',(11.2830607729999,11.6,-2.16929420200001));
#184706=CARTESIAN_POINT('Ctrl Pts',(11.2800100139999,15.2,-2.16701606700001));
#184707=CARTESIAN_POINT('Ctrl Pts',(11.2800100139999,11.6,-2.16701606700001));
#184708=CARTESIAN_POINT('Ctrl Pts',(11.2769610569999,15.2,-2.16474288000001));
#184709=CARTESIAN_POINT('Ctrl Pts',(11.2769610569999,11.6,-2.16474288000002));
#184710=CARTESIAN_POINT('Ctrl Pts',(11.2739139069999,15.2,-2.16247464600002));
#184711=CARTESIAN_POINT('Ctrl Pts',(11.2739139069999,11.6,-2.16247464600002));
#184712=CARTESIAN_POINT('Ctrl Pts',(11.2708685709999,15.2,-2.16021135900001));
#184713=CARTESIAN_POINT('Ctrl Pts',(11.2708685709999,11.6,-2.16021135900002));
#184714=CARTESIAN_POINT('Ctrl Pts',(11.2678250539999,15.2,-2.15795302400001));
#184715=CARTESIAN_POINT('Ctrl Pts',(11.2678250539999,11.6,-2.15795302400001));
#184716=CARTESIAN_POINT('Ctrl Pts',(11.2647833679999,15.2,-2.15569963800001));
#184717=CARTESIAN_POINT('Ctrl Pts',(11.2647833679999,11.6,-2.15569963800002));
#184718=CARTESIAN_POINT('Ctrl Pts',(11.2617435239999,15.2,-2.15345120200002));
#184719=CARTESIAN_POINT('Ctrl Pts',(11.2617435239999,11.6,-2.15345120200002));
#184720=CARTESIAN_POINT('Ctrl Pts',(11.2587055319999,15.2,-2.15120771400001));
#184721=CARTESIAN_POINT('Ctrl Pts',(11.2587055319999,11.6,-2.15120771400001));
#184722=CARTESIAN_POINT('Ctrl Pts',(11.2556694029999,15.2,-2.14896917500001));
#184723=CARTESIAN_POINT('Ctrl Pts',(11.2556694029999,11.6,-2.14896917500001));
#184724=CARTESIAN_POINT('Ctrl Pts',(11.2526351489999,15.2,-2.14673558300001));
#184725=CARTESIAN_POINT('Ctrl Pts',(11.2526351489999,11.6,-2.14673558300001));
#184726=CARTESIAN_POINT('Ctrl Pts',(11.2496027769999,15.2,-2.14450693900002));
#184727=CARTESIAN_POINT('Ctrl Pts',(11.2496027769999,11.6,-2.14450693900002));
#184728=CARTESIAN_POINT('Ctrl Pts',(11.2465722989999,15.2,-2.14228324400001));
#184729=CARTESIAN_POINT('Ctrl Pts',(11.2465722989999,11.6,-2.14228324400001));
#184730=CARTESIAN_POINT('Ctrl Pts',(11.2435437199999,15.2,-2.14006449500001));
#184731=CARTESIAN_POINT('Ctrl Pts',(11.2435437199999,11.6,-2.14006449500001));
#184732=CARTESIAN_POINT('Ctrl Pts',(11.2405170499999,15.2,-2.13785069200001));
#184733=CARTESIAN_POINT('Ctrl Pts',(11.2405170499999,11.6,-2.13785069200001));
#184734=CARTESIAN_POINT('Ctrl Pts',(11.2374922969999,15.2,-2.13564183800001));
#184735=CARTESIAN_POINT('Ctrl Pts',(11.2374922969999,11.6,-2.13564183800001));
#184736=CARTESIAN_POINT('Ctrl Pts',(11.2344694679999,15.2,-2.13343792800002));
#184737=CARTESIAN_POINT('Ctrl Pts',(11.2344694679999,11.6,-2.13343792800002));
#184738=CARTESIAN_POINT('Ctrl Pts',(11.2314485739999,15.2,-2.13123896500001));
#184739=CARTESIAN_POINT('Ctrl Pts',(11.2314485739999,11.6,-2.13123896500001));
#184740=CARTESIAN_POINT('Ctrl Pts',(11.2284296229999,15.2,-2.12904494700001));
#184741=CARTESIAN_POINT('Ctrl Pts',(11.2284296229999,11.6,-2.12904494700001));
#184742=CARTESIAN_POINT('Ctrl Pts',(11.2254126259999,15.2,-2.12685587500001));
#184743=CARTESIAN_POINT('Ctrl Pts',(11.2254126259999,11.6,-2.12685587500001));
#184744=CARTESIAN_POINT('Ctrl Pts',(11.2223975909999,15.2,-2.12467174800001));
#184745=CARTESIAN_POINT('Ctrl Pts',(11.2223975909999,11.6,-2.12467174800001));
#184746=CARTESIAN_POINT('Ctrl Pts',(11.2193845279999,15.2,-2.12249256400002));
#184747=CARTESIAN_POINT('Ctrl Pts',(11.2193845279999,11.6,-2.12249256400002));
#184748=CARTESIAN_POINT('Ctrl Pts',(11.2163734459999,15.2,-2.12031832500001));
#184749=CARTESIAN_POINT('Ctrl Pts',(11.2163734459999,11.6,-2.12031832500002));
#184750=CARTESIAN_POINT('Ctrl Pts',(11.2133643549999,15.2,-2.11814902900001));
#184751=CARTESIAN_POINT('Ctrl Pts',(11.2133643549999,11.6,-2.11814902900001));
#184752=CARTESIAN_POINT('Ctrl Pts',(11.2103572639999,15.2,-2.11598467700002));
#184753=CARTESIAN_POINT('Ctrl Pts',(11.2103572639999,11.6,-2.11598467700002));
#184754=CARTESIAN_POINT('Ctrl Pts',(11.2073521809999,15.2,-2.11382526700001));
#184755=CARTESIAN_POINT('Ctrl Pts',(11.2073521809999,11.6,-2.11382526700001));
#184756=CARTESIAN_POINT('Ctrl Pts',(11.2043491159999,15.2,-2.11167080000001));
#184757=CARTESIAN_POINT('Ctrl Pts',(11.2043491159999,11.6,-2.11167080000001));
#184758=CARTESIAN_POINT('Ctrl Pts',(11.2013480779999,15.2,-2.10952127400001));
#184759=CARTESIAN_POINT('Ctrl Pts',(11.2013480779999,11.6,-2.10952127400002));
#184760=CARTESIAN_POINT('Ctrl Pts',(11.1983490759999,15.2,-2.10737669000002));
#184761=CARTESIAN_POINT('Ctrl Pts',(11.1983490759999,11.6,-2.10737669000002));
#184762=CARTESIAN_POINT('Ctrl Pts',(11.1953521189999,15.2,-2.10523704700002));
#184763=CARTESIAN_POINT('Ctrl Pts',(11.1953521189999,11.6,-2.10523704700002));
#184764=CARTESIAN_POINT('Ctrl Pts',(11.1923572179999,15.2,-2.10310234400001));
#184765=CARTESIAN_POINT('Ctrl Pts',(11.1923572179999,11.6,-2.10310234400001));
#184766=CARTESIAN_POINT('Ctrl Pts',(11.1893643799999,15.2,-2.10097258200001));
#184767=CARTESIAN_POINT('Ctrl Pts',(11.1893643799999,11.6,-2.10097258200001));
#184768=CARTESIAN_POINT('Ctrl Pts',(11.1863736159999,15.2,-2.09884776000001));
#184769=CARTESIAN_POINT('Ctrl Pts',(11.1863736159999,11.6,-2.09884776000001));
#184770=CARTESIAN_POINT('Ctrl Pts',(11.1833849349999,15.2,-2.09672787600002));
#184771=CARTESIAN_POINT('Ctrl Pts',(11.1833849349999,11.6,-2.09672787600002));
#184772=CARTESIAN_POINT('Ctrl Pts',(11.1803983459999,15.2,-2.09461293100001));
#184773=CARTESIAN_POINT('Ctrl Pts',(11.1803983459999,11.6,-2.09461293100001));
#184774=CARTESIAN_POINT('Ctrl Pts',(11.1774138589999,15.2,-2.09250292400001));
#184775=CARTESIAN_POINT('Ctrl Pts',(11.1774138589999,11.6,-2.09250292400002));
#184776=CARTESIAN_POINT('Ctrl Pts',(11.1744314829999,15.2,-2.09039785500002));
#184777=CARTESIAN_POINT('Ctrl Pts',(11.1744314829999,11.6,-2.09039785500002));
#184778=CARTESIAN_POINT('Ctrl Pts',(11.1714512269999,15.2,-2.08829772200001));
#184779=CARTESIAN_POINT('Ctrl Pts',(11.1714512269999,11.6,-2.08829772200001));
#184780=CARTESIAN_POINT('Ctrl Pts',(11.1684731009999,15.2,-2.08620252800001));
#184781=CARTESIAN_POINT('Ctrl Pts',(11.1684731009999,11.6,-2.08620252800001));
#184782=CARTESIAN_POINT('Ctrl Pts',(11.1654971139999,15.2,-2.08411226800001));
#184783=CARTESIAN_POINT('Ctrl Pts',(11.1654971139999,11.6,-2.08411226800001));
#184784=CARTESIAN_POINT('Ctrl Pts',(11.1625232759999,15.2,-2.08202694400001));
#184785=CARTESIAN_POINT('Ctrl Pts',(11.1625232759999,11.6,-2.08202694400002));
#184786=CARTESIAN_POINT('Ctrl Pts',(11.1595515959999,15.2,-2.07994655500002));
#184787=CARTESIAN_POINT('Ctrl Pts',(11.1595515959999,11.6,-2.07994655500002));
#184788=CARTESIAN_POINT('Ctrl Pts',(11.1565820829999,15.2,-2.07787110100002));
#184789=CARTESIAN_POINT('Ctrl Pts',(11.1565820829999,11.6,-2.07787110100002));
#184790=CARTESIAN_POINT('Ctrl Pts',(11.1536147479999,15.2,-2.07580058000001));
#184791=CARTESIAN_POINT('Ctrl Pts',(11.1536147479999,11.6,-2.07580058000001));
#184792=CARTESIAN_POINT('Ctrl Pts',(11.1506495989999,15.2,-2.07373499200001));
#184793=CARTESIAN_POINT('Ctrl Pts',(11.1506495989999,11.6,-2.07373499200001));
#184794=CARTESIAN_POINT('Ctrl Pts',(11.1476866469999,15.2,-2.07167433800001));
#184795=CARTESIAN_POINT('Ctrl Pts',(11.1476866469999,11.6,-2.07167433800001));
#184796=CARTESIAN_POINT('Ctrl Pts',(11.1447258999999,15.2,-2.06961861400002));
#184797=CARTESIAN_POINT('Ctrl Pts',(11.1447258999999,11.6,-2.06961861400002));
#184798=CARTESIAN_POINT('Ctrl Pts',(11.1417673689999,15.2,-2.06756782300001));
#184799=CARTESIAN_POINT('Ctrl Pts',(11.1417673689999,11.6,-2.06756782300001));
#184800=CARTESIAN_POINT('Ctrl Pts',(11.1388110619999,15.2,-2.06552196300001));
#184801=CARTESIAN_POINT('Ctrl Pts',(11.1388110619999,11.6,-2.06552196300001));
#184802=CARTESIAN_POINT('Ctrl Pts',(11.1358569909999,15.2,-2.06348103200002));
#184803=CARTESIAN_POINT('Ctrl Pts',(11.1358569909999,11.6,-2.06348103200002));
#184804=CARTESIAN_POINT('Ctrl Pts',(11.1329051619999,15.2,-2.06144503100001));
#184805=CARTESIAN_POINT('Ctrl Pts',(11.1329051619999,11.6,-2.06144503100001));
#184806=CARTESIAN_POINT('Ctrl Pts',(11.1299555879999,15.2,-2.05941396000001));
#184807=CARTESIAN_POINT('Ctrl Pts',(11.1299555879999,11.6,-2.05941396000001));
#184808=CARTESIAN_POINT('Ctrl Pts',(11.1270082769999,15.2,-2.05738781600001));
#184809=CARTESIAN_POINT('Ctrl Pts',(11.1270082769999,11.6,-2.05738781600001));
#184810=CARTESIAN_POINT('Ctrl Pts',(11.1240632389999,15.2,-2.05536660000002));
#184811=CARTESIAN_POINT('Ctrl Pts',(11.1240632389999,11.6,-2.05536660000002));
#184812=CARTESIAN_POINT('Ctrl Pts',(11.1211204849999,15.2,-2.05335031100002));
#184813=CARTESIAN_POINT('Ctrl Pts',(11.1211204849999,11.6,-2.05335031100002));
#184814=CARTESIAN_POINT('Ctrl Pts',(11.1181800219999,15.2,-2.05133894900001));
#184815=CARTESIAN_POINT('Ctrl Pts',(11.1181800219999,11.6,-2.05133894900001));
#184816=CARTESIAN_POINT('Ctrl Pts',(11.1152418619999,15.2,-2.04933251100002));
#184817=CARTESIAN_POINT('Ctrl Pts',(11.1152418619999,11.6,-2.04933251100002));
#184818=CARTESIAN_POINT('Ctrl Pts',(11.1123060129999,15.2,-2.04733099900002));
#184819=CARTESIAN_POINT('Ctrl Pts',(11.1123060129999,11.6,-2.04733099900002));
#184820=CARTESIAN_POINT('Ctrl Pts',(11.1093724859999,15.2,-2.04533441000001));
#184821=CARTESIAN_POINT('Ctrl Pts',(11.1093724859999,11.6,-2.04533441000002));
#184822=CARTESIAN_POINT('Ctrl Pts',(11.1064412909999,15.2,-2.04334274600001));
#184823=CARTESIAN_POINT('Ctrl Pts',(11.1064412909999,11.6,-2.04334274600001));
#184824=CARTESIAN_POINT('Ctrl Pts',(11.1035124359999,15.2,-2.04135600400001));
#184825=CARTESIAN_POINT('Ctrl Pts',(11.1035124359999,11.6,-2.04135600400001));
#184826=CARTESIAN_POINT('Ctrl Pts',(11.1005859329999,15.2,-2.03937418500002));
#184827=CARTESIAN_POINT('Ctrl Pts',(11.1005859329999,11.6,-2.03937418500002));
#184828=CARTESIAN_POINT('Ctrl Pts',(11.0976617909999,15.2,-2.03739728600001));
#184829=CARTESIAN_POINT('Ctrl Pts',(11.0976617909999,11.6,-2.03739728600001));
#184830=CARTESIAN_POINT('Ctrl Pts',(11.0947400189999,15.2,-2.03542530800001));
#184831=CARTESIAN_POINT('Ctrl Pts',(11.0947400189999,11.6,-2.03542530800001));
#184832=CARTESIAN_POINT('Ctrl Pts',(11.0918206279999,15.2,-2.03345825000001));
#184833=CARTESIAN_POINT('Ctrl Pts',(11.0918206279999,11.6,-2.03345825000001));
#184834=CARTESIAN_POINT('Ctrl Pts',(11.0889036269999,15.2,-2.03149611000002));
#184835=CARTESIAN_POINT('Ctrl Pts',(11.0889036269999,11.6,-2.03149611000002));
#184836=CARTESIAN_POINT('Ctrl Pts',(11.0859890259999,15.2,-2.02953888900002));
#184837=CARTESIAN_POINT('Ctrl Pts',(11.0859890259999,11.6,-2.02953888900002));
#184838=CARTESIAN_POINT('Ctrl Pts',(11.0830768349999,15.2,-2.02758658500001));
#184839=CARTESIAN_POINT('Ctrl Pts',(11.0830768349999,11.6,-2.02758658500001));
#184840=CARTESIAN_POINT('Ctrl Pts',(11.0801670649999,15.2,-2.02563919800001));
#184841=CARTESIAN_POINT('Ctrl Pts',(11.0801670649999,11.6,-2.02563919800001));
#184842=CARTESIAN_POINT('Ctrl Pts',(11.0772597239999,15.2,-2.02369672700002));
#184843=CARTESIAN_POINT('Ctrl Pts',(11.0772597239999,11.6,-2.02369672700002));
#184844=CARTESIAN_POINT('Ctrl Pts',(11.0743548239999,15.2,-2.02175917000002));
#184845=CARTESIAN_POINT('Ctrl Pts',(11.0743548239999,11.6,-2.02175917000002));
#184846=CARTESIAN_POINT('Ctrl Pts',(11.0714523729999,15.2,-2.01982652800002));
#184847=CARTESIAN_POINT('Ctrl Pts',(11.0714523729999,11.6,-2.01982652800002));
#184848=CARTESIAN_POINT('Ctrl Pts',(11.0685523819999,15.2,-2.01789879900002));
#184849=CARTESIAN_POINT('Ctrl Pts',(11.0685523819999,11.6,-2.01789879900002));
#184850=CARTESIAN_POINT('Ctrl Pts',(11.0656548619999,15.2,-2.01597598400001));
#184851=CARTESIAN_POINT('Ctrl Pts',(11.0656548619999,11.6,-2.01597598400001));
#184852=CARTESIAN_POINT('Ctrl Pts',(11.0627598219999,15.2,-2.01405807900001));
#184853=CARTESIAN_POINT('Ctrl Pts',(11.0627598219999,11.6,-2.01405807900001));
#184854=CARTESIAN_POINT('Ctrl Pts',(11.0598672709999,15.2,-2.01214508500001));
#184855=CARTESIAN_POINT('Ctrl Pts',(11.0598672709999,11.6,-2.01214508500001));
#184856=CARTESIAN_POINT('Ctrl Pts',(11.0569772199999,15.2,-2.01023700100002));
#184857=CARTESIAN_POINT('Ctrl Pts',(11.0569772199999,11.6,-2.01023700100002));
#184858=CARTESIAN_POINT('Ctrl Pts',(11.0540896799999,15.2,-2.00833382500001));
#184859=CARTESIAN_POINT('Ctrl Pts',(11.0540896799999,11.6,-2.00833382500001));
#184860=CARTESIAN_POINT('Ctrl Pts',(11.0512046609999,15.2,-2.00643555900001));
#184861=CARTESIAN_POINT('Ctrl Pts',(11.0512046609999,11.6,-2.00643555900002));
#184862=CARTESIAN_POINT('Ctrl Pts',(11.0483221709999,15.2,-2.00454219900001));
#184863=CARTESIAN_POINT('Ctrl Pts',(11.0483221709999,11.6,-2.00454219900001));
#184864=CARTESIAN_POINT('Ctrl Pts',(11.0454422219999,15.2,-2.00265374600002));
#184865=CARTESIAN_POINT('Ctrl Pts',(11.0454422219999,11.6,-2.00265374600002));
#184866=CARTESIAN_POINT('Ctrl Pts',(11.0425648239999,15.2,-2.00077019700001));
#184867=CARTESIAN_POINT('Ctrl Pts',(11.0425648239999,11.6,-2.00077019700002));
#184868=CARTESIAN_POINT('Ctrl Pts',(11.0396899859999,15.2,-1.99889155300002));
#184869=CARTESIAN_POINT('Ctrl Pts',(11.0396899859999,11.6,-1.99889155300002));
#184870=CARTESIAN_POINT('Ctrl Pts',(11.0368177199999,15.2,-1.99701781300002));
#184871=CARTESIAN_POINT('Ctrl Pts',(11.0368177199999,11.6,-1.99701781300002));
#184872=CARTESIAN_POINT('Ctrl Pts',(11.0339480349999,15.2,-1.99514897500002));
#184873=CARTESIAN_POINT('Ctrl Pts',(11.0339480349999,11.6,-1.99514897500002));
#184874=CARTESIAN_POINT('Ctrl Pts',(11.0310809409999,15.2,-1.99328503900002));
#184875=CARTESIAN_POINT('Ctrl Pts',(11.0310809409999,11.6,-1.99328503900002));
#184876=CARTESIAN_POINT('Ctrl Pts',(11.0282164499999,15.2,-1.99142600400001));
#184877=CARTESIAN_POINT('Ctrl Pts',(11.0282164499999,11.6,-1.99142600400001));
#184878=CARTESIAN_POINT('Ctrl Pts',(11.0253545699999,15.2,-1.98957186700001));
#184879=CARTESIAN_POINT('Ctrl Pts',(11.0253545699999,11.6,-1.98957186700001));
#184880=CARTESIAN_POINT('Ctrl Pts',(11.0224953139999,15.2,-1.98772263000001));
#184881=CARTESIAN_POINT('Ctrl Pts',(11.0224953139999,11.6,-1.98772263000001));
#184882=CARTESIAN_POINT('Ctrl Pts',(11.0196386889999,15.2,-1.98587829000001));
#184883=CARTESIAN_POINT('Ctrl Pts',(11.0196386889999,11.6,-1.98587829000001));
#184884=CARTESIAN_POINT('Ctrl Pts',(11.0167847069999,15.2,-1.98403884600001));
#184885=CARTESIAN_POINT('Ctrl Pts',(11.0167847069999,11.6,-1.98403884600001));
#184886=CARTESIAN_POINT('Ctrl Pts',(11.0139333789999,15.2,-1.98220429900001));
#184887=CARTESIAN_POINT('Ctrl Pts',(11.0139333789999,11.6,-1.98220429900001));
#184888=CARTESIAN_POINT('Ctrl Pts',(11.0110847139999,15.2,-1.98037464500001));
#184889=CARTESIAN_POINT('Ctrl Pts',(11.0110847139999,11.6,-1.98037464500001));
#184890=CARTESIAN_POINT('Ctrl Pts',(11.0082387239999,15.2,-1.97854988600001));
#184891=CARTESIAN_POINT('Ctrl Pts',(11.0082387239999,11.6,-1.97854988600001));
#184892=CARTESIAN_POINT('Ctrl Pts',(11.0053954179999,15.2,-1.97673001800001));
#184893=CARTESIAN_POINT('Ctrl Pts',(11.0053954179999,11.6,-1.97673001800002));
#184894=CARTESIAN_POINT('Ctrl Pts',(11.0025548069999,15.2,-1.97491504200002));
#184895=CARTESIAN_POINT('Ctrl Pts',(11.0025548069999,11.6,-1.97491504200002));
#184896=CARTESIAN_POINT('Ctrl Pts',(10.9997169009999,15.2,-1.97310495600002));
#184897=CARTESIAN_POINT('Ctrl Pts',(10.9997169009999,11.6,-1.97310495600002));
#184898=CARTESIAN_POINT('Ctrl Pts',(10.9968817109999,15.2,-1.97129976000001));
#184899=CARTESIAN_POINT('Ctrl Pts',(10.9968817109999,11.6,-1.97129976000001));
#184900=CARTESIAN_POINT('Ctrl Pts',(10.9940492479999,15.2,-1.96949945100001));
#184901=CARTESIAN_POINT('Ctrl Pts',(10.9940492479999,11.6,-1.96949945100001));
#184902=CARTESIAN_POINT('Ctrl Pts',(10.9912195209999,15.2,-1.96770403000002));
#184903=CARTESIAN_POINT('Ctrl Pts',(10.9912195209999,11.6,-1.96770403000002));
#184904=CARTESIAN_POINT('Ctrl Pts',(10.9883925419999,15.2,-1.96591349300002));
#184905=CARTESIAN_POINT('Ctrl Pts',(10.9883925419999,11.6,-1.96591349300002));
#184906=CARTESIAN_POINT('Ctrl Pts',(10.9855683189999,15.2,-1.96412784200001));
#184907=CARTESIAN_POINT('Ctrl Pts',(10.9855683189999,11.6,-1.96412784200001));
#184908=CARTESIAN_POINT('Ctrl Pts',(10.9827468659999,15.2,-1.96234707600001));
#184909=CARTESIAN_POINT('Ctrl Pts',(10.9827468659999,11.6,-1.96234707600001));
#184910=CARTESIAN_POINT('Ctrl Pts',(10.9799281919999,15.2,-1.96057119000002));
#184911=CARTESIAN_POINT('Ctrl Pts',(10.9799281919999,11.6,-1.96057119000002));
#184912=CARTESIAN_POINT('Ctrl Pts',(10.9771123069999,15.2,-1.95880018600001));
#184913=CARTESIAN_POINT('Ctrl Pts',(10.9771123069999,11.6,-1.95880018600001));
#184914=CARTESIAN_POINT('Ctrl Pts',(10.9742992229999,15.2,-1.95703406200002));
#184915=CARTESIAN_POINT('Ctrl Pts',(10.9742992229999,11.6,-1.95703406200002));
#184916=CARTESIAN_POINT('Ctrl Pts',(10.9714889499999,15.2,-1.95527281700001));
#184917=CARTESIAN_POINT('Ctrl Pts',(10.9714889499999,11.6,-1.95527281700001));
#184918=CARTESIAN_POINT('Ctrl Pts',(10.9686814969999,15.2,-1.95351645000001));
#184919=CARTESIAN_POINT('Ctrl Pts',(10.9686814969999,11.6,-1.95351645000002));
#184920=CARTESIAN_POINT('Ctrl Pts',(10.9658768769999,15.2,-1.95176496000002));
#184921=CARTESIAN_POINT('Ctrl Pts',(10.9658768769999,11.6,-1.95176496000002));
#184922=CARTESIAN_POINT('Ctrl Pts',(10.9630750999999,15.2,-1.95001834400002));
#184923=CARTESIAN_POINT('Ctrl Pts',(10.9630750999999,11.6,-1.95001834400002));
#184924=CARTESIAN_POINT('Ctrl Pts',(10.9602761759999,15.2,-1.94827660300001));
#184925=CARTESIAN_POINT('Ctrl Pts',(10.9602761759999,11.6,-1.94827660300001));
#184926=CARTESIAN_POINT('Ctrl Pts',(10.9574801169999,15.2,-1.94653973400001));
#184927=CARTESIAN_POINT('Ctrl Pts',(10.9574801169999,11.6,-1.94653973400001));
#184928=CARTESIAN_POINT('Ctrl Pts',(10.9546869339999,15.2,-1.94480773700001));
#184929=CARTESIAN_POINT('Ctrl Pts',(10.9546869339999,11.6,-1.94480773700001));
#184930=CARTESIAN_POINT('Ctrl Pts',(10.9518966359999,15.2,-1.94308061000001));
#184931=CARTESIAN_POINT('Ctrl Pts',(10.9518966359999,11.6,-1.94308061000001));
#184932=CARTESIAN_POINT('Ctrl Pts',(10.9491092339999,15.2,-1.94135835200001));
#184933=CARTESIAN_POINT('Ctrl Pts',(10.9491092339999,11.6,-1.94135835200001));
#184934=CARTESIAN_POINT('Ctrl Pts',(10.9463247409999,15.2,-1.93964096300002));
#184935=CARTESIAN_POINT('Ctrl Pts',(10.9463247409999,11.6,-1.93964096300002));
#184936=CARTESIAN_POINT('Ctrl Pts',(10.9435431659999,15.2,-1.93792843900002));
#184937=CARTESIAN_POINT('Ctrl Pts',(10.9435431659999,11.6,-1.93792843900002));
#184938=CARTESIAN_POINT('Ctrl Pts',(10.9407645199999,15.2,-1.93622078000002));
#184939=CARTESIAN_POINT('Ctrl Pts',(10.9407645199999,11.6,-1.93622078000002));
#184940=CARTESIAN_POINT('Ctrl Pts',(10.9379888129999,15.2,-1.93451798600002));
#184941=CARTESIAN_POINT('Ctrl Pts',(10.9379888129999,11.6,-1.93451798600002));
#184942=CARTESIAN_POINT('Ctrl Pts',(10.9352160579999,15.2,-1.93282005400001));
#184943=CARTESIAN_POINT('Ctrl Pts',(10.9352160579999,11.6,-1.93282005400001));
#184944=CARTESIAN_POINT('Ctrl Pts',(10.9324462649999,15.2,-1.93112698300002));
#184945=CARTESIAN_POINT('Ctrl Pts',(10.9324462649999,11.6,-1.93112698300002));
#184946=CARTESIAN_POINT('Ctrl Pts',(10.9296794449999,15.2,-1.92943877200001));
#184947=CARTESIAN_POINT('Ctrl Pts',(10.9296794449999,11.6,-1.92943877200001));
#184948=CARTESIAN_POINT('Ctrl Pts',(10.9269156089999,15.2,-1.92775541900001));
#184949=CARTESIAN_POINT('Ctrl Pts',(10.9269156089999,11.6,-1.92775541900002));
#184950=CARTESIAN_POINT('Ctrl Pts',(10.9241547679999,15.2,-1.92607692400002));
#184951=CARTESIAN_POINT('Ctrl Pts',(10.9241547679999,11.6,-1.92607692400002));
#184952=CARTESIAN_POINT('Ctrl Pts',(10.9213969329999,15.2,-1.92440328400002));
#184953=CARTESIAN_POINT('Ctrl Pts',(10.9213969329999,11.6,-1.92440328400002));
#184954=CARTESIAN_POINT('Ctrl Pts',(10.9186421139999,15.2,-1.92273449800001));
#184955=CARTESIAN_POINT('Ctrl Pts',(10.9186421139999,11.6,-1.92273449800001));
#184956=CARTESIAN_POINT('Ctrl Pts',(10.9158903239999,15.2,-1.92107056500001));
#184957=CARTESIAN_POINT('Ctrl Pts',(10.9158903239999,11.6,-1.92107056500001));
#184958=CARTESIAN_POINT('Ctrl Pts',(10.9131415729999,15.2,-1.91941148400002));
#184959=CARTESIAN_POINT('Ctrl Pts',(10.9131415729999,11.6,-1.91941148400002));
#184960=CARTESIAN_POINT('Ctrl Pts',(10.9103958719999,15.2,-1.91775725300001));
#184961=CARTESIAN_POINT('Ctrl Pts',(10.9103958719999,11.6,-1.91775725300001));
#184962=CARTESIAN_POINT('Ctrl Pts',(10.9076532319999,15.2,-1.91610787000001));
#184963=CARTESIAN_POINT('Ctrl Pts',(10.9076532319999,11.6,-1.91610787000001));
#184964=CARTESIAN_POINT('Ctrl Pts',(10.9049136649999,15.2,-1.91446333400001));
#184965=CARTESIAN_POINT('Ctrl Pts',(10.9049136649999,11.6,-1.91446333400001));
#184966=CARTESIAN_POINT('Ctrl Pts',(10.9021771809999,15.2,-1.91282364500001));
#184967=CARTESIAN_POINT('Ctrl Pts',(10.9021771809999,11.6,-1.91282364500002));
#184968=CARTESIAN_POINT('Ctrl Pts',(10.8994437919999,15.2,-1.91118879900001));
#184969=CARTESIAN_POINT('Ctrl Pts',(10.8994437919999,11.6,-1.91118879900001));
#184970=CARTESIAN_POINT('Ctrl Pts',(10.8967135099999,15.2,-1.90955879600001));
#184971=CARTESIAN_POINT('Ctrl Pts',(10.8967135099999,11.6,-1.90955879600002));
#184972=CARTESIAN_POINT('Ctrl Pts',(10.8939863439999,15.2,-1.90793363400001));
#184973=CARTESIAN_POINT('Ctrl Pts',(10.8939863439999,11.6,-1.90793363400001));
#184974=CARTESIAN_POINT('Ctrl Pts',(10.8912623069999,15.2,-1.90631331100001));
#184975=CARTESIAN_POINT('Ctrl Pts',(10.8912623069999,11.6,-1.90631331100001));
#184976=CARTESIAN_POINT('Ctrl Pts',(10.8885414099999,15.2,-1.90469782700001));
#184977=CARTESIAN_POINT('Ctrl Pts',(10.8885414099999,11.6,-1.90469782700002));
#184978=CARTESIAN_POINT('Ctrl Pts',(10.8858236639999,15.2,-1.90308718000002));
#184979=CARTESIAN_POINT('Ctrl Pts',(10.8858236639999,11.6,-1.90308718000002));
#184980=CARTESIAN_POINT('Ctrl Pts',(10.8831090799999,15.2,-1.90148136800001));
#184981=CARTESIAN_POINT('Ctrl Pts',(10.8831090799999,11.6,-1.90148136800001));
#184982=CARTESIAN_POINT('Ctrl Pts',(10.8803976699999,15.2,-1.89988038900001));
#184983=CARTESIAN_POINT('Ctrl Pts',(10.8803976699999,11.6,-1.89988038900002));
#184984=CARTESIAN_POINT('Ctrl Pts',(10.8776894459999,15.2,-1.89828424200002));
#184985=CARTESIAN_POINT('Ctrl Pts',(10.8776894459999,11.6,-1.89828424200002));
#184986=CARTESIAN_POINT('Ctrl Pts',(10.8749844169999,15.2,-1.89669292500001));
#184987=CARTESIAN_POINT('Ctrl Pts',(10.8749844169999,11.6,-1.89669292500001));
#184988=CARTESIAN_POINT('Ctrl Pts',(10.8722825979999,15.2,-1.89510643700002));
#184989=CARTESIAN_POINT('Ctrl Pts',(10.8722825979999,11.6,-1.89510643700002));
#184990=CARTESIAN_POINT('Ctrl Pts',(10.8695839969999,15.2,-1.89352477600002));
#184991=CARTESIAN_POINT('Ctrl Pts',(10.8695839969999,11.6,-1.89352477600002));
#184992=CARTESIAN_POINT('Ctrl Pts',(10.8668886269999,15.2,-1.89194794100001));
#184993=CARTESIAN_POINT('Ctrl Pts',(10.8668886269999,11.6,-1.89194794100001));
#184994=CARTESIAN_POINT('Ctrl Pts',(10.8641964999999,15.2,-1.89037593000001));
#184995=CARTESIAN_POINT('Ctrl Pts',(10.8641964999999,11.6,-1.89037593000001));
#184996=CARTESIAN_POINT('Ctrl Pts',(10.8615076259999,15.2,-1.88880873900001));
#184997=CARTESIAN_POINT('Ctrl Pts',(10.8615076259999,11.6,-1.88880873900001));
#184998=CARTESIAN_POINT('Ctrl Pts',(10.8588220189999,15.2,-1.88724637100002));
#184999=CARTESIAN_POINT('Ctrl Pts',(10.8588220189999,11.6,-1.88724637100002));
#185000=CARTESIAN_POINT('Ctrl Pts',(10.8561396869999,15.2,-1.88568882100002));
#185001=CARTESIAN_POINT('Ctrl Pts',(10.8561396869999,11.6,-1.88568882100002));
#185002=CARTESIAN_POINT('Ctrl Pts',(10.8534606449999,15.2,-1.88413608800001));
#185003=CARTESIAN_POINT('Ctrl Pts',(10.8534606449999,11.6,-1.88413608800001));
#185004=CARTESIAN_POINT('Ctrl Pts',(10.8507849019999,15.2,-1.88258817100001));
#185005=CARTESIAN_POINT('Ctrl Pts',(10.8507849019999,11.6,-1.88258817100001));
#185006=CARTESIAN_POINT('Ctrl Pts',(10.8481124719999,15.2,-1.88104506700002));
#185007=CARTESIAN_POINT('Ctrl Pts',(10.8481124719999,11.6,-1.88104506700002));
#185008=CARTESIAN_POINT('Ctrl Pts',(10.8454433649999,15.2,-1.87950677600002));
#185009=CARTESIAN_POINT('Ctrl Pts',(10.8454433649999,11.6,-1.87950677600002));
#185010=CARTESIAN_POINT('Ctrl Pts',(10.8427775919999,15.2,-1.87797329500001));
#185011=CARTESIAN_POINT('Ctrl Pts',(10.8427775919999,11.6,-1.87797329500001));
#185012=CARTESIAN_POINT('Ctrl Pts',(10.8401151679999,15.2,-1.87644462300002));
#185013=CARTESIAN_POINT('Ctrl Pts',(10.8401151679999,11.6,-1.87644462300002));
#185014=CARTESIAN_POINT('Ctrl Pts',(10.8374561019999,15.2,-1.87492075600002));
#185015=CARTESIAN_POINT('Ctrl Pts',(10.8374561019999,11.6,-1.87492075600002));
#185016=CARTESIAN_POINT('Ctrl Pts',(10.8348004049999,15.2,-1.87340169600001));
#185017=CARTESIAN_POINT('Ctrl Pts',(10.8348004049999,11.6,-1.87340169600001));
#185018=CARTESIAN_POINT('Ctrl Pts',(10.8321480909999,15.2,-1.87188743700001));
#185019=CARTESIAN_POINT('Ctrl Pts',(10.8321480909999,11.6,-1.87188743700002));
#185020=CARTESIAN_POINT('Ctrl Pts',(10.8294991699999,15.2,-1.87037798100001));
#185021=CARTESIAN_POINT('Ctrl Pts',(10.8294991699999,11.6,-1.87037798100001));
#185022=CARTESIAN_POINT('Ctrl Pts',(10.8268536559999,15.2,-1.86887332500001));
#185023=CARTESIAN_POINT('Ctrl Pts',(10.8268536559999,11.6,-1.86887332500001));
#185024=CARTESIAN_POINT('Ctrl Pts',(10.8242115599999,15.2,-1.86737346600002));
#185025=CARTESIAN_POINT('Ctrl Pts',(10.8242115599999,11.6,-1.86737346600002));
#185026=CARTESIAN_POINT('Ctrl Pts',(10.8215728919999,15.2,-1.86587840300001));
#185027=CARTESIAN_POINT('Ctrl Pts',(10.8215728919999,11.6,-1.86587840300001));
#185028=CARTESIAN_POINT('Ctrl Pts',(10.8189376659999,15.2,-1.86438813400001));
#185029=CARTESIAN_POINT('Ctrl Pts',(10.8189376659999,11.6,-1.86438813400002));
#185030=CARTESIAN_POINT('Ctrl Pts',(10.8163058929999,15.2,-1.86290265800002));
#185031=CARTESIAN_POINT('Ctrl Pts',(10.8163058929999,11.6,-1.86290265800002));
#185032=CARTESIAN_POINT('Ctrl Pts',(10.8136775859999,15.2,-1.86142197100001));
#185033=CARTESIAN_POINT('Ctrl Pts',(10.8136775859999,11.6,-1.86142197100002));
#185034=CARTESIAN_POINT('Ctrl Pts',(10.8110527559999,15.2,-1.85994607300001));
#185035=CARTESIAN_POINT('Ctrl Pts',(10.8110527559999,11.6,-1.85994607300001));
#185036=CARTESIAN_POINT('Ctrl Pts',(10.8084314149999,15.2,-1.85847496100001));
#185037=CARTESIAN_POINT('Ctrl Pts',(10.8084314149999,11.6,-1.85847496100001));
#185038=CARTESIAN_POINT('Ctrl Pts',(10.8058135739999,15.2,-1.85700863500001));
#185039=CARTESIAN_POINT('Ctrl Pts',(10.8058135739999,11.6,-1.85700863500002));
#185040=CARTESIAN_POINT('Ctrl Pts',(10.8031992479999,15.2,-1.85554709000002));
#185041=CARTESIAN_POINT('Ctrl Pts',(10.8031992479999,11.6,-1.85554709000002));
#185042=CARTESIAN_POINT('Ctrl Pts',(10.8005884479999,15.2,-1.85409032700001));
#185043=CARTESIAN_POINT('Ctrl Pts',(10.8005884479999,11.6,-1.85409032700001));
#185044=CARTESIAN_POINT('Ctrl Pts',(10.7979811829999,15.2,-1.85263834300001));
#185045=CARTESIAN_POINT('Ctrl Pts',(10.7979811829999,11.6,-1.85263834300002));
#185046=CARTESIAN_POINT('Ctrl Pts',(10.7953774699999,15.2,-1.85119113400001));
#185047=CARTESIAN_POINT('Ctrl Pts',(10.7953774699999,11.6,-1.85119113400001));
#185048=CARTESIAN_POINT('Ctrl Pts',(10.7927773169999,15.2,-1.84974870100001));
#185049=CARTESIAN_POINT('Ctrl Pts',(10.7927773169999,11.6,-1.84974870100001));
#185050=CARTESIAN_POINT('Ctrl Pts',(10.7901807389999,15.2,-1.84831104100001));
#185051=CARTESIAN_POINT('Ctrl Pts',(10.7901807389999,11.6,-1.84831104100002));
#185052=CARTESIAN_POINT('Ctrl Pts',(10.7875877469999,15.2,-1.84687815000002));
#185053=CARTESIAN_POINT('Ctrl Pts',(10.7875877469999,11.6,-1.84687815000002));
#185054=CARTESIAN_POINT('Ctrl Pts',(10.7849983529999,15.2,-1.84545003000002));
#185055=CARTESIAN_POINT('Ctrl Pts',(10.7849983529999,11.6,-1.84545003000002));
#185056=CARTESIAN_POINT('Ctrl Pts',(10.7824125699999,15.2,-1.84402667500001));
#185057=CARTESIAN_POINT('Ctrl Pts',(10.7824125699999,11.6,-1.84402667500001));
#185058=CARTESIAN_POINT('Ctrl Pts',(10.7798304099999,15.2,-1.84260808500001));
#185059=CARTESIAN_POINT('Ctrl Pts',(10.7798304099999,11.6,-1.84260808500001));
#185060=CARTESIAN_POINT('Ctrl Pts',(10.7772518849999,15.2,-1.84119425700001));
#185061=CARTESIAN_POINT('Ctrl Pts',(10.7772518849999,11.6,-1.84119425700001));
#185062=CARTESIAN_POINT('Ctrl Pts',(10.7746770079999,15.2,-1.83978519100001));
#185063=CARTESIAN_POINT('Ctrl Pts',(10.7746770079999,11.6,-1.83978519100001));
#185064=CARTESIAN_POINT('Ctrl Pts',(10.7721057909999,15.2,-1.83838088200002));
#185065=CARTESIAN_POINT('Ctrl Pts',(10.7721057909999,11.6,-1.83838088200002));
#185066=CARTESIAN_POINT('Ctrl Pts',(10.7695382459999,15.2,-1.83698133000001));
#185067=CARTESIAN_POINT('Ctrl Pts',(10.7695382459999,11.6,-1.83698133000001));
#185068=CARTESIAN_POINT('Ctrl Pts',(10.7669743859999,15.2,-1.83558653200001));
#185069=CARTESIAN_POINT('Ctrl Pts',(10.7669743859999,11.6,-1.83558653200001));
#185070=CARTESIAN_POINT('Ctrl Pts',(10.7644142219999,15.2,-1.83419648500001));
#185071=CARTESIAN_POINT('Ctrl Pts',(10.7644142219999,11.6,-1.83419648500002));
#185072=CARTESIAN_POINT('Ctrl Pts',(10.7618577699999,15.2,-1.83281118900001));
#185073=CARTESIAN_POINT('Ctrl Pts',(10.7618577699999,11.6,-1.83281118900001));
#185074=CARTESIAN_POINT('Ctrl Pts',(10.7593050389999,15.2,-1.83143064000001));
#185075=CARTESIAN_POINT('Ctrl Pts',(10.7593050389999,11.6,-1.83143064000001));
#185076=CARTESIAN_POINT('Ctrl Pts',(10.7567560429999,15.2,-1.83005483600001));
#185077=CARTESIAN_POINT('Ctrl Pts',(10.7567560429999,11.6,-1.83005483600002));
#185078=CARTESIAN_POINT('Ctrl Pts',(10.7542107949999,15.2,-1.82868377600002));
#185079=CARTESIAN_POINT('Ctrl Pts',(10.7542107949999,11.6,-1.82868377600002));
#185080=CARTESIAN_POINT('Ctrl Pts',(10.7516693049999,15.2,-1.82731745700002));
#185081=CARTESIAN_POINT('Ctrl Pts',(10.7516693049999,11.6,-1.82731745700002));
#185082=CARTESIAN_POINT('Ctrl Pts',(10.7491315889999,15.2,-1.82595587600002));
#185083=CARTESIAN_POINT('Ctrl Pts',(10.7491315889999,11.6,-1.82595587600002));
#185084=CARTESIAN_POINT('Ctrl Pts',(10.7465976589999,15.2,-1.82459903200002));
#185085=CARTESIAN_POINT('Ctrl Pts',(10.7465976589999,11.6,-1.82459903200002));
#185086=CARTESIAN_POINT('Ctrl Pts',(10.7440675249999,15.2,-1.82324692100002));
#185087=CARTESIAN_POINT('Ctrl Pts',(10.7440675249999,11.6,-1.82324692100002));
#185088=CARTESIAN_POINT('Ctrl Pts',(10.7415412029999,15.2,-1.82189954400001));
#185089=CARTESIAN_POINT('Ctrl Pts',(10.7415412029999,11.6,-1.82189954400001));
#185090=CARTESIAN_POINT('Ctrl Pts',(10.7390187039999,15.2,-1.82055689500002));
#185091=CARTESIAN_POINT('Ctrl Pts',(10.7390187039999,11.6,-1.82055689500002));
#185092=CARTESIAN_POINT('Ctrl Pts',(10.7365000409999,15.2,-1.81921897400001));
#185093=CARTESIAN_POINT('Ctrl Pts',(10.7365000409999,11.6,-1.81921897400001));
#185094=CARTESIAN_POINT('Ctrl Pts',(10.7339852259999,15.2,-1.81788577800001));
#185095=CARTESIAN_POINT('Ctrl Pts',(10.7339852259999,11.6,-1.81788577800001));
#185096=CARTESIAN_POINT('Ctrl Pts',(10.7314742729999,15.2,-1.81655730500001));
#185097=CARTESIAN_POINT('Ctrl Pts',(10.7314742729999,11.6,-1.81655730500002));
#185098=CARTESIAN_POINT('Ctrl Pts',(10.7289671959999,15.2,-1.81523355200001));
#185099=CARTESIAN_POINT('Ctrl Pts',(10.7289671959999,11.6,-1.81523355200001));
#185100=CARTESIAN_POINT('Ctrl Pts',(10.7264640049999,15.2,-1.81391451700001));
#185101=CARTESIAN_POINT('Ctrl Pts',(10.7264640049999,11.6,-1.81391451700002));
#185102=CARTESIAN_POINT('Ctrl Pts',(10.7239647149999,15.2,-1.81260019700002));
#185103=CARTESIAN_POINT('Ctrl Pts',(10.7239647149999,11.6,-1.81260019700002));
#185104=CARTESIAN_POINT('Ctrl Pts',(10.7214693369999,15.2,-1.81129059100002));
#185105=CARTESIAN_POINT('Ctrl Pts',(10.7214693369999,11.6,-1.81129059100002));
#185106=CARTESIAN_POINT('Ctrl Pts',(10.7189778869999,15.2,-1.80998569500002));
#185107=CARTESIAN_POINT('Ctrl Pts',(10.7189778869999,11.6,-1.80998569500002));
#185108=CARTESIAN_POINT('Ctrl Pts',(10.7164903759999,15.2,-1.80868550800001));
#185109=CARTESIAN_POINT('Ctrl Pts',(10.7164903759999,11.6,-1.80868550800001));
#185110=CARTESIAN_POINT('Ctrl Pts',(10.7140068169999,15.2,-1.80739002600002));
#185111=CARTESIAN_POINT('Ctrl Pts',(10.7140068169999,11.6,-1.80739002600002));
#185112=CARTESIAN_POINT('Ctrl Pts',(10.7115272219999,15.2,-1.80609924900001));
#185113=CARTESIAN_POINT('Ctrl Pts',(10.7115272219999,11.6,-1.80609924900002));
#185114=CARTESIAN_POINT('Ctrl Pts',(10.7090516069999,15.2,-1.80481317100002));
#185115=CARTESIAN_POINT('Ctrl Pts',(10.7090516069999,11.6,-1.80481317100002));
#185116=CARTESIAN_POINT('Ctrl Pts',(10.7065799829999,15.2,-1.80353179300001));
#185117=CARTESIAN_POINT('Ctrl Pts',(10.7065799829999,11.6,-1.80353179300001));
#185118=CARTESIAN_POINT('Ctrl Pts',(10.7041123629999,15.2,-1.80225511000002));
#185119=CARTESIAN_POINT('Ctrl Pts',(10.7041123629999,11.6,-1.80225511000002));
#185120=CARTESIAN_POINT('Ctrl Pts',(10.7016487619999,15.2,-1.80098312100001));
#185121=CARTESIAN_POINT('Ctrl Pts',(10.7016487619999,11.6,-1.80098312100002));
#185122=CARTESIAN_POINT('Ctrl Pts',(10.6991891909999,15.2,-1.79971582200002));
#185123=CARTESIAN_POINT('Ctrl Pts',(10.6991891909999,11.6,-1.79971582200002));
#185124=CARTESIAN_POINT('Ctrl Pts',(10.6967336649999,15.2,-1.79845321200002));
#185125=CARTESIAN_POINT('Ctrl Pts',(10.6967336649999,11.6,-1.79845321200002));
#185126=CARTESIAN_POINT('Ctrl Pts',(10.6942821969999,15.2,-1.79719528800002));
#185127=CARTESIAN_POINT('Ctrl Pts',(10.6942821969999,11.6,-1.79719528800002));
#185128=CARTESIAN_POINT('Ctrl Pts',(10.6918347989999,15.2,-1.79594204600001));
#185129=CARTESIAN_POINT('Ctrl Pts',(10.6918347989999,11.6,-1.79594204600001));
#185130=CARTESIAN_POINT('Ctrl Pts',(10.6893914849999,15.2,-1.79469348500001));
#185131=CARTESIAN_POINT('Ctrl Pts',(10.6893914849999,11.6,-1.79469348500001));
#185132=CARTESIAN_POINT('Ctrl Pts',(10.6869522689999,15.2,-1.79344960200002));
#185133=CARTESIAN_POINT('Ctrl Pts',(10.6869522689999,11.6,-1.79344960200002));
#185134=CARTESIAN_POINT('Ctrl Pts',(10.6845171639999,15.2,-1.79221039500002));
#185135=CARTESIAN_POINT('Ctrl Pts',(10.6845171639999,11.6,-1.79221039500002));
#185136=CARTESIAN_POINT('Ctrl Pts',(10.6820861829999,15.2,-1.79097585900001));
#185137=CARTESIAN_POINT('Ctrl Pts',(10.6820861829999,11.6,-1.79097585900002));
#185138=CARTESIAN_POINT('Ctrl Pts',(10.6796593399999,15.2,-1.78974599400001));
#185139=CARTESIAN_POINT('Ctrl Pts',(10.6796593399999,11.6,-1.78974599400001));
#185140=CARTESIAN_POINT('Ctrl Pts',(10.6772366489999,15.2,-1.78852079700001));
#185141=CARTESIAN_POINT('Ctrl Pts',(10.6772366489999,11.6,-1.78852079700001));
#185142=CARTESIAN_POINT('Ctrl Pts',(10.6748181209999,15.2,-1.78730026200002));
#185143=CARTESIAN_POINT('Ctrl Pts',(10.6748181209999,11.6,-1.78730026200002));
#185144=CARTESIAN_POINT('Ctrl Pts',(10.6724037739999,15.2,-1.78608439100001));
#185145=CARTESIAN_POINT('Ctrl Pts',(10.6724037739999,11.6,-1.78608439100001));
#185146=CARTESIAN_POINT('Ctrl Pts',(10.6699936169999,15.2,-1.78487317800001));
#185147=CARTESIAN_POINT('Ctrl Pts',(10.6699936169999,11.6,-1.78487317800002));
#185148=CARTESIAN_POINT('Ctrl Pts',(10.6675876659999,15.2,-1.78366662200002));
#185149=CARTESIAN_POINT('Ctrl Pts',(10.6675876659999,11.6,-1.78366662200002));
#185150=CARTESIAN_POINT('Ctrl Pts',(10.6651859349999,15.2,-1.78246471900001));
#185151=CARTESIAN_POINT('Ctrl Pts',(10.6651859349999,11.6,-1.78246471900001));
#185152=CARTESIAN_POINT('Ctrl Pts',(10.6627884359999,15.2,-1.78126746700002));
#185153=CARTESIAN_POINT('Ctrl Pts',(10.6627884359999,11.6,-1.78126746700002));
#185154=CARTESIAN_POINT('Ctrl Pts',(10.6603951839999,15.2,-1.78007486200002));
#185155=CARTESIAN_POINT('Ctrl Pts',(10.6603951839999,11.6,-1.78007486200002));
#185156=CARTESIAN_POINT('Ctrl Pts',(10.6580061929999,15.2,-1.77888690400001));
#185157=CARTESIAN_POINT('Ctrl Pts',(10.6580061929999,11.6,-1.77888690400001));
#185158=CARTESIAN_POINT('Ctrl Pts',(10.6556214759999,15.2,-1.77770358600001));
#185159=CARTESIAN_POINT('Ctrl Pts',(10.6556214759999,11.6,-1.77770358600001));
#185160=CARTESIAN_POINT('Ctrl Pts',(10.6532410469999,15.2,-1.77652490900002));
#185161=CARTESIAN_POINT('Ctrl Pts',(10.6532410469999,11.6,-1.77652490900002));
#185162=CARTESIAN_POINT('Ctrl Pts',(10.6508649199999,15.2,-1.77535086800002));
#185163=CARTESIAN_POINT('Ctrl Pts',(10.6508649199999,11.6,-1.77535086800002));
#185164=CARTESIAN_POINT('Ctrl Pts',(10.6484931079999,15.2,-1.77418146100001));
#185165=CARTESIAN_POINT('Ctrl Pts',(10.6484931079999,11.6,-1.77418146100001));
#185166=CARTESIAN_POINT('Ctrl Pts',(10.6461256269999,15.2,-1.77301668400001));
#185167=CARTESIAN_POINT('Ctrl Pts',(10.6461256269999,11.6,-1.77301668400002));
#185168=CARTESIAN_POINT('Ctrl Pts',(10.6437624889999,15.2,-1.77185653600001));
#185169=CARTESIAN_POINT('Ctrl Pts',(10.6437624889999,11.6,-1.77185653600001));
#185170=CARTESIAN_POINT('Ctrl Pts',(10.6414037079999,15.2,-1.77070101100002));
#185171=CARTESIAN_POINT('Ctrl Pts',(10.6414037079999,11.6,-1.77070101100002));
#185172=CARTESIAN_POINT('Ctrl Pts',(10.6390492989999,15.2,-1.76955010900001));
#185173=CARTESIAN_POINT('Ctrl Pts',(10.6390492989999,11.6,-1.76955010900001));
#185174=CARTESIAN_POINT('Ctrl Pts',(10.6366992769999,15.2,-1.76840382600002));
#185175=CARTESIAN_POINT('Ctrl Pts',(10.6366992769999,11.6,-1.76840382600002));
#185176=CARTESIAN_POINT('Ctrl Pts',(10.6343536529999,15.2,-1.76726215800001));
#185177=CARTESIAN_POINT('Ctrl Pts',(10.6343536529999,11.6,-1.76726215800001));
#185178=CARTESIAN_POINT('Ctrl Pts',(10.6320124439999,15.2,-1.76612510300002));
#185179=CARTESIAN_POINT('Ctrl Pts',(10.6320124439999,11.6,-1.76612510300002));
#185180=CARTESIAN_POINT('Ctrl Pts',(10.6296756629999,15.2,-1.76499265800001));
#185181=CARTESIAN_POINT('Ctrl Pts',(10.6296756629999,11.6,-1.76499265800001));
#185182=CARTESIAN_POINT('Ctrl Pts',(10.6273433229999,15.2,-1.76386482000002));
#185183=CARTESIAN_POINT('Ctrl Pts',(10.6273433229999,11.6,-1.76386482000002));
#185184=CARTESIAN_POINT('Ctrl Pts',(10.6250154409999,15.2,-1.76274158600001));
#185185=CARTESIAN_POINT('Ctrl Pts',(10.6250154409999,11.6,-1.76274158600001));
#185186=CARTESIAN_POINT('Ctrl Pts',(10.6226920299999,15.2,-1.76162295100001));
#185187=CARTESIAN_POINT('Ctrl Pts',(10.6226920299999,11.6,-1.76162295100002));
#185188=CARTESIAN_POINT('Ctrl Pts',(10.6203731039999,15.2,-1.76050891500001));
#185189=CARTESIAN_POINT('Ctrl Pts',(10.6203731039999,11.6,-1.76050891500001));
#185190=CARTESIAN_POINT('Ctrl Pts',(10.6180586769999,15.2,-1.75939947300002));
#185191=CARTESIAN_POINT('Ctrl Pts',(10.6180586769999,11.6,-1.75939947300002));
#185192=CARTESIAN_POINT('Ctrl Pts',(10.6157487639999,15.2,-1.75829462200001));
#185193=CARTESIAN_POINT('Ctrl Pts',(10.6157487639999,11.6,-1.75829462200001));
#185194=CARTESIAN_POINT('Ctrl Pts',(10.6134433789999,15.2,-1.75719435900001));
#185195=CARTESIAN_POINT('Ctrl Pts',(10.6134433789999,11.6,-1.75719435900001));
#185196=CARTESIAN_POINT('Ctrl Pts',(10.6111425369999,15.2,-1.75609868000001));
#185197=CARTESIAN_POINT('Ctrl Pts',(10.6111425369999,11.6,-1.75609868000001));
#185198=CARTESIAN_POINT('Ctrl Pts',(10.6088462529999,15.2,-1.75500758300001));
#185199=CARTESIAN_POINT('Ctrl Pts',(10.6088462529999,11.6,-1.75500758300001));
#185200=CARTESIAN_POINT('Ctrl Pts',(10.6065545399999,15.2,-1.75392106500002));
#185201=CARTESIAN_POINT('Ctrl Pts',(10.6065545399999,11.6,-1.75392106500002));
#185202=CARTESIAN_POINT('Ctrl Pts',(10.6042674129999,15.2,-1.75283912300001));
#185203=CARTESIAN_POINT('Ctrl Pts',(10.6042674129999,11.6,-1.75283912300001));
#185204=CARTESIAN_POINT('Ctrl Pts',(10.6019848869999,15.2,-1.75176175100002));
#185205=CARTESIAN_POINT('Ctrl Pts',(10.6019848869999,11.6,-1.75176175100002));
#185206=CARTESIAN_POINT('Ctrl Pts',(10.5997069769999,15.2,-1.75068894800001));
#185207=CARTESIAN_POINT('Ctrl Pts',(10.5997069769999,11.6,-1.75068894800001));
#185208=CARTESIAN_POINT('Ctrl Pts',(10.5974336969999,15.2,-1.74962071100001));
#185209=CARTESIAN_POINT('Ctrl Pts',(10.5974336969999,11.6,-1.74962071100001));
#185210=CARTESIAN_POINT('Ctrl Pts',(10.5951650619999,15.2,-1.74855703600001));
#185211=CARTESIAN_POINT('Ctrl Pts',(10.5951650619999,11.6,-1.74855703600001));
#185212=CARTESIAN_POINT('Ctrl Pts',(10.5929010879999,15.2,-1.74749791900001));
#185213=CARTESIAN_POINT('Ctrl Pts',(10.5929010879999,11.6,-1.74749791900001));
#185214=CARTESIAN_POINT('Ctrl Pts',(10.5906417869999,15.2,-1.74644335800001));
#185215=CARTESIAN_POINT('Ctrl Pts',(10.5906417869999,11.6,-1.74644335800001));
#185216=CARTESIAN_POINT('Ctrl Pts',(10.5883871749999,15.2,-1.74539334800001));
#185217=CARTESIAN_POINT('Ctrl Pts',(10.5883871749999,11.6,-1.74539334800001));
#185218=CARTESIAN_POINT('Ctrl Pts',(10.5861372679999,15.2,-1.74434788600002));
#185219=CARTESIAN_POINT('Ctrl Pts',(10.5861372679999,11.6,-1.74434788600002));
#185220=CARTESIAN_POINT('Ctrl Pts',(10.5838920789999,15.2,-1.74330697000002));
#185221=CARTESIAN_POINT('Ctrl Pts',(10.5838920789999,11.6,-1.74330697000002));
#185222=CARTESIAN_POINT('Ctrl Pts',(10.5816516249999,15.2,-1.74227059600002));
#185223=CARTESIAN_POINT('Ctrl Pts',(10.5816516249999,11.6,-1.74227059600002));
#185224=CARTESIAN_POINT('Ctrl Pts',(10.5794159199999,15.2,-1.74123876000001));
#185225=CARTESIAN_POINT('Ctrl Pts',(10.5794159199999,11.6,-1.74123876000001));
#185226=CARTESIAN_POINT('Ctrl Pts',(10.5771849789999,15.2,-1.74021145700001));
#185227=CARTESIAN_POINT('Ctrl Pts',(10.5771849789999,11.6,-1.74021145700001));
#185228=CARTESIAN_POINT('Ctrl Pts',(10.5749588169999,15.2,-1.73918868600001));
#185229=CARTESIAN_POINT('Ctrl Pts',(10.5749588169999,11.6,-1.73918868600001));
#185230=CARTESIAN_POINT('Ctrl Pts',(10.5727374489999,15.2,-1.73817044400002));
#185231=CARTESIAN_POINT('Ctrl Pts',(10.5727374489999,11.6,-1.73817044400002));
#185232=CARTESIAN_POINT('Ctrl Pts',(10.5705208909999,15.2,-1.73715672500002));
#185233=CARTESIAN_POINT('Ctrl Pts',(10.5705208909999,11.6,-1.73715672500002));
#185234=CARTESIAN_POINT('Ctrl Pts',(10.5683091569999,15.2,-1.73614752600002));
#185235=CARTESIAN_POINT('Ctrl Pts',(10.5683091569999,11.6,-1.73614752600002));
#185236=CARTESIAN_POINT('Ctrl Pts',(10.5661022619999,15.2,-1.73514284500001));
#185237=CARTESIAN_POINT('Ctrl Pts',(10.5661022619999,11.6,-1.73514284500001));
#185238=CARTESIAN_POINT('Ctrl Pts',(10.5639002229999,15.2,-1.73414267600001));
#185239=CARTESIAN_POINT('Ctrl Pts',(10.5639002229999,11.6,-1.73414267600001));
#185240=CARTESIAN_POINT('Ctrl Pts',(10.5617030549999,15.2,-1.73314701800001));
#185241=CARTESIAN_POINT('Ctrl Pts',(10.5617030549999,11.6,-1.73314701800001));
#185242=CARTESIAN_POINT('Ctrl Pts',(10.5595107719999,15.2,-1.73215586600001));
#185243=CARTESIAN_POINT('Ctrl Pts',(10.5595107719999,11.6,-1.73215586600001));
#185244=CARTESIAN_POINT('Ctrl Pts',(10.5573233899999,15.2,-1.73116921600001));
#185245=CARTESIAN_POINT('Ctrl Pts',(10.5573233899999,11.6,-1.73116921600002));
#185246=CARTESIAN_POINT('Ctrl Pts',(10.5551409249999,15.2,-1.73018706400001));
#185247=CARTESIAN_POINT('Ctrl Pts',(10.5551409249999,11.6,-1.73018706400002));
#185248=CARTESIAN_POINT('Ctrl Pts',(10.5529633919999,15.2,-1.72920940800001));
#185249=CARTESIAN_POINT('Ctrl Pts',(10.5529633919999,11.6,-1.72920940800001));
#185250=CARTESIAN_POINT('Ctrl Pts',(10.5507908049999,15.2,-1.72823624300001));
#185251=CARTESIAN_POINT('Ctrl Pts',(10.5507908049999,11.6,-1.72823624300001));
#185252=CARTESIAN_POINT('Ctrl Pts',(10.5486231829999,15.2,-1.72726756600001));
#185253=CARTESIAN_POINT('Ctrl Pts',(10.5486231829999,11.6,-1.72726756600001));
#185254=CARTESIAN_POINT('Ctrl Pts',(10.5464605389999,15.2,-1.72630337200002));
#185255=CARTESIAN_POINT('Ctrl Pts',(10.5464605389999,11.6,-1.72630337200002));
#185256=CARTESIAN_POINT('Ctrl Pts',(10.5443028889999,15.2,-1.72534365700002));
#185257=CARTESIAN_POINT('Ctrl Pts',(10.5443028889999,11.6,-1.72534365700002));
#185258=CARTESIAN_POINT('Ctrl Pts',(10.5421502479999,15.2,-1.72438842000001));
#185259=CARTESIAN_POINT('Ctrl Pts',(10.5421502479999,11.6,-1.72438842000001));
#185260=CARTESIAN_POINT('Ctrl Pts',(10.5400026339999,15.2,-1.72343765400001));
#185261=CARTESIAN_POINT('Ctrl Pts',(10.5400026339999,11.6,-1.72343765400001));
#185262=CARTESIAN_POINT('Ctrl Pts',(10.5378600619999,15.2,-1.72249135700001));
#185263=CARTESIAN_POINT('Ctrl Pts',(10.5378600619999,11.6,-1.72249135700001));
#185264=CARTESIAN_POINT('Ctrl Pts',(10.5357225459999,15.2,-1.72154952500001));
#185265=CARTESIAN_POINT('Ctrl Pts',(10.5357225459999,11.6,-1.72154952500002));
#185266=CARTESIAN_POINT('Ctrl Pts',(10.5335901039999,15.2,-1.72061215300001));
#185267=CARTESIAN_POINT('Ctrl Pts',(10.5335901039999,11.6,-1.72061215300001));
#185268=CARTESIAN_POINT('Ctrl Pts',(10.5314627509999,15.2,-1.71967923800001));
#185269=CARTESIAN_POINT('Ctrl Pts',(10.5314627509999,11.6,-1.71967923800001));
#185270=CARTESIAN_POINT('Ctrl Pts',(10.5293405029999,15.2,-1.71875077500002));
#185271=CARTESIAN_POINT('Ctrl Pts',(10.5293405029999,11.6,-1.71875077500002));
#185272=CARTESIAN_POINT('Ctrl Pts',(10.5272233759999,15.2,-1.71782676100001));
#185273=CARTESIAN_POINT('Ctrl Pts',(10.5272233759999,11.6,-1.71782676100001));
#185274=CARTESIAN_POINT('Ctrl Pts',(10.5251113859999,15.2,-1.71690719200001));
#185275=CARTESIAN_POINT('Ctrl Pts',(10.5251113859999,11.6,-1.71690719200001));
#185276=CARTESIAN_POINT('Ctrl Pts',(10.5230045489999,15.2,-1.71599206300002));
#185277=CARTESIAN_POINT('Ctrl Pts',(10.5230045489999,11.6,-1.71599206300002));
#185278=CARTESIAN_POINT('Ctrl Pts',(10.5209028819999,15.2,-1.71508137300002));
#185279=CARTESIAN_POINT('Ctrl Pts',(10.5209028819999,11.6,-1.71508137300002));
#185280=CARTESIAN_POINT('Ctrl Pts',(10.5188063989999,15.2,-1.71417511400001));
#185281=CARTESIAN_POINT('Ctrl Pts',(10.5188063989999,11.6,-1.71417511400001));
#185282=CARTESIAN_POINT('Ctrl Pts',(10.5167151179999,15.2,-1.71327328300002));
#185283=CARTESIAN_POINT('Ctrl Pts',(10.5167151179999,11.6,-1.71327328300002));
#185284=CARTESIAN_POINT('Ctrl Pts',(10.5146290569999,15.2,-1.71237587700002));
#185285=CARTESIAN_POINT('Ctrl Pts',(10.5146290569999,11.6,-1.71237587700002));
#185286=CARTESIAN_POINT('Ctrl Pts',(10.5125482279999,15.2,-1.71148289200001));
#185287=CARTESIAN_POINT('Ctrl Pts',(10.5125482279999,11.6,-1.71148289200001));
#185288=CARTESIAN_POINT('Ctrl Pts',(10.5104726499999,15.2,-1.71059432200002));
#185289=CARTESIAN_POINT('Ctrl Pts',(10.5104726499999,11.6,-1.71059432200002));
#185290=CARTESIAN_POINT('Ctrl Pts',(10.5084023389999,15.2,-1.70971016400001));
#185291=CARTESIAN_POINT('Ctrl Pts',(10.5084023389999,11.6,-1.70971016400001));
#185292=CARTESIAN_POINT('Ctrl Pts',(10.5063373119999,15.2,-1.70883041400002));
#185293=CARTESIAN_POINT('Ctrl Pts',(10.5063373119999,11.6,-1.70883041400002));
#185294=CARTESIAN_POINT('Ctrl Pts',(10.5042775849999,15.2,-1.70795506700001));
#185295=CARTESIAN_POINT('Ctrl Pts',(10.5042775849999,11.6,-1.70795506700001));
#185296=CARTESIAN_POINT('Ctrl Pts',(10.5022231739999,15.2,-1.70708412100002));
#185297=CARTESIAN_POINT('Ctrl Pts',(10.5022231739999,11.6,-1.70708412100002));
#185298=CARTESIAN_POINT('Ctrl Pts',(10.5001740959999,15.2,-1.70621756800001));
#185299=CARTESIAN_POINT('Ctrl Pts',(10.5001740959999,11.6,-1.70621756800002));
#185300=CARTESIAN_POINT('Ctrl Pts',(10.4981303679999,15.2,-1.70535540700001));
#185301=CARTESIAN_POINT('Ctrl Pts',(10.4981303679999,11.6,-1.70535540700001));
#185302=CARTESIAN_POINT('Ctrl Pts',(10.4960920059999,15.2,-1.70449763100001));
#185303=CARTESIAN_POINT('Ctrl Pts',(10.4960920059999,11.6,-1.70449763100002));
#185304=CARTESIAN_POINT('Ctrl Pts',(10.4940590279999,15.2,-1.70364423800001));
#185305=CARTESIAN_POINT('Ctrl Pts',(10.4940590279999,11.6,-1.70364423800002));
#185306=CARTESIAN_POINT('Ctrl Pts',(10.4920314479999,15.2,-1.70279522300001));
#185307=CARTESIAN_POINT('Ctrl Pts',(10.4920314479999,11.6,-1.70279522300001));
#185308=CARTESIAN_POINT('Ctrl Pts',(10.4900092879999,15.2,-1.70195058100001));
#185309=CARTESIAN_POINT('Ctrl Pts',(10.4900092879999,11.6,-1.70195058100001));
#185310=CARTESIAN_POINT('Ctrl Pts',(10.4879925589999,15.2,-1.70111030700001));
#185311=CARTESIAN_POINT('Ctrl Pts',(10.4879925589999,11.6,-1.70111030700001));
#185312=CARTESIAN_POINT('Ctrl Pts',(10.4859812819999,15.2,-1.70027439800001));
#185313=CARTESIAN_POINT('Ctrl Pts',(10.4859812819999,11.6,-1.70027439800002));
#185314=CARTESIAN_POINT('Ctrl Pts',(10.4839754719999,15.2,-1.69944284800001));
#185315=CARTESIAN_POINT('Ctrl Pts',(10.4839754719999,11.6,-1.69944284800001));
#185316=CARTESIAN_POINT('Ctrl Pts',(10.4819751459999,15.2,-1.69861565400002));
#185317=CARTESIAN_POINT('Ctrl Pts',(10.4819751459999,11.6,-1.69861565400002));
#185318=CARTESIAN_POINT('Ctrl Pts',(10.4799803229999,15.2,-1.69779281100002));
#185319=CARTESIAN_POINT('Ctrl Pts',(10.4799803229999,11.6,-1.69779281100002));
#185320=CARTESIAN_POINT('Ctrl Pts',(10.4779910179999,15.2,-1.69697431400001));
#185321=CARTESIAN_POINT('Ctrl Pts',(10.4779910179999,11.6,-1.69697431400001));
#185322=CARTESIAN_POINT('Ctrl Pts',(10.4760072489999,15.2,-1.69616015900001));
#185323=CARTESIAN_POINT('Ctrl Pts',(10.4760072489999,11.6,-1.69616015900001));
#185324=CARTESIAN_POINT('Ctrl Pts',(10.4740290339999,15.2,-1.69535034000001));
#185325=CARTESIAN_POINT('Ctrl Pts',(10.4740290339999,11.6,-1.69535034000001));
#185326=CARTESIAN_POINT('Ctrl Pts',(10.4720563889999,15.2,-1.69454485500002));
#185327=CARTESIAN_POINT('Ctrl Pts',(10.4720563889999,11.6,-1.69454485500002));
#185328=CARTESIAN_POINT('Ctrl Pts',(10.4700893329999,15.2,-1.69374369700002));
#185329=CARTESIAN_POINT('Ctrl Pts',(10.4700893329999,11.6,-1.69374369700002));
#185330=CARTESIAN_POINT('Ctrl Pts',(10.4681278809999,15.2,-1.69294686200002));
#185331=CARTESIAN_POINT('Ctrl Pts',(10.4681278809999,11.6,-1.69294686200002));
#185332=CARTESIAN_POINT('Ctrl Pts',(10.4661720519999,15.2,-1.69215434500002));
#185333=CARTESIAN_POINT('Ctrl Pts',(10.4661720519999,11.6,-1.69215434500002));
#185334=CARTESIAN_POINT('Ctrl Pts',(10.4642218629999,15.2,-1.69136614200001));
#185335=CARTESIAN_POINT('Ctrl Pts',(10.4642218629999,11.6,-1.69136614200002));
#185336=CARTESIAN_POINT('Ctrl Pts',(10.4622773339999,15.2,-1.69058224900001));
#185337=CARTESIAN_POINT('Ctrl Pts',(10.4622773339999,11.6,-1.69058224900001));
#185338=CARTESIAN_POINT('Ctrl Pts',(10.4603384779999,15.2,-1.68980265900001));
#185339=CARTESIAN_POINT('Ctrl Pts',(10.4603384779999,11.6,-1.68980265900002));
#185340=CARTESIAN_POINT('Ctrl Pts',(10.4584053159999,15.2,-1.68902736800002));
#185341=CARTESIAN_POINT('Ctrl Pts',(10.4584053159999,11.6,-1.68902736800002));
#185342=CARTESIAN_POINT('Ctrl Pts',(10.4564778639999,15.2,-1.68825637300001));
#185343=CARTESIAN_POINT('Ctrl Pts',(10.4564778639999,11.6,-1.68825637300001));
#185344=CARTESIAN_POINT('Ctrl Pts',(10.4545561419999,15.2,-1.68748966700001));
#185345=CARTESIAN_POINT('Ctrl Pts',(10.4545561419999,11.6,-1.68748966700001));
#185346=CARTESIAN_POINT('Ctrl Pts',(10.4526401659999,15.2,-1.68672724400002));
#185347=CARTESIAN_POINT('Ctrl Pts',(10.4526401659999,11.6,-1.68672724400002));
#185348=CARTESIAN_POINT('Ctrl Pts',(10.4507299549999,15.2,-1.68596910300002));
#185349=CARTESIAN_POINT('Ctrl Pts',(10.4507299549999,11.6,-1.68596910300002));
#185350=CARTESIAN_POINT('Ctrl Pts',(10.4488255249999,15.2,-1.68521523500001));
#185351=CARTESIAN_POINT('Ctrl Pts',(10.4488255249999,11.6,-1.68521523500001));
#185352=CARTESIAN_POINT('Ctrl Pts',(10.4469268959999,15.2,-1.68446563800002));
#185353=CARTESIAN_POINT('Ctrl Pts',(10.4469268959999,11.6,-1.68446563800002));
#185354=CARTESIAN_POINT('Ctrl Pts',(10.4450340849999,15.2,-1.68372030600001));
#185355=CARTESIAN_POINT('Ctrl Pts',(10.4450340849999,11.6,-1.68372030600001));
#185356=CARTESIAN_POINT('Ctrl Pts',(10.4431471089999,15.2,-1.68297923300001));
#185357=CARTESIAN_POINT('Ctrl Pts',(10.4431471089999,11.6,-1.68297923300001));
#185358=CARTESIAN_POINT('Ctrl Pts',(10.4412659899999,15.2,-1.68224241600001));
#185359=CARTESIAN_POINT('Ctrl Pts',(10.4412659899999,11.6,-1.68224241600001));
#185360=CARTESIAN_POINT('Ctrl Pts',(10.4393907419999,15.2,-1.68150984700001));
#185361=CARTESIAN_POINT('Ctrl Pts',(10.4393907419999,11.6,-1.68150984700001));
#185362=CARTESIAN_POINT('Ctrl Pts',(10.4375213869999,15.2,-1.68078152300001));
#185363=CARTESIAN_POINT('Ctrl Pts',(10.4375213869999,11.6,-1.68078152300001));
#185364=CARTESIAN_POINT('Ctrl Pts',(10.4356579399999,15.2,-1.68005743800002));
#185365=CARTESIAN_POINT('Ctrl Pts',(10.4356579399999,11.6,-1.68005743800002));
#185366=CARTESIAN_POINT('Ctrl Pts',(10.4338004199999,15.2,-1.67933758800002));
#185367=CARTESIAN_POINT('Ctrl Pts',(10.4338004199999,11.6,-1.67933758800002));
#185368=CARTESIAN_POINT('Ctrl Pts',(10.4319488479999,15.2,-1.67862196700002));
#185369=CARTESIAN_POINT('Ctrl Pts',(10.4319488479999,11.6,-1.67862196700002));
#185370=CARTESIAN_POINT('Ctrl Pts',(10.4301032399999,15.2,-1.67791057000001));
#185371=CARTESIAN_POINT('Ctrl Pts',(10.4301032399999,11.6,-1.67791057000001));
#185372=CARTESIAN_POINT('Ctrl Pts',(10.4282636149999,15.2,-1.67720339000001));
#185373=CARTESIAN_POINT('Ctrl Pts',(10.4282636149999,11.6,-1.67720339000002));
#185374=CARTESIAN_POINT('Ctrl Pts',(10.4264299929999,15.2,-1.67650042400001));
#185375=CARTESIAN_POINT('Ctrl Pts',(10.4264299929999,11.6,-1.67650042400001));
#185376=CARTESIAN_POINT('Ctrl Pts',(10.4246023919999,15.2,-1.67580166600001));
#185377=CARTESIAN_POINT('Ctrl Pts',(10.4246023919999,11.6,-1.67580166600001));
#185378=CARTESIAN_POINT('Ctrl Pts',(10.4227808289999,15.2,-1.67510711000002));
#185379=CARTESIAN_POINT('Ctrl Pts',(10.4227808289999,11.6,-1.67510711000002));
#185380=CARTESIAN_POINT('Ctrl Pts',(10.4209653239999,15.2,-1.67441675200001));
#185381=CARTESIAN_POINT('Ctrl Pts',(10.4209653239999,11.6,-1.67441675200001));
#185382=CARTESIAN_POINT('Ctrl Pts',(10.4191558969999,15.2,-1.67373058500001));
#185383=CARTESIAN_POINT('Ctrl Pts',(10.4191558969999,11.6,-1.67373058500001));
#185384=CARTESIAN_POINT('Ctrl Pts',(10.4173525659999,15.2,-1.67304860400002));
#185385=CARTESIAN_POINT('Ctrl Pts',(10.4173525659999,11.6,-1.67304860400002));
#185386=CARTESIAN_POINT('Ctrl Pts',(10.4155553499999,15.2,-1.67237080400001));
#185387=CARTESIAN_POINT('Ctrl Pts',(10.4155553499999,11.6,-1.67237080400001));
#185388=CARTESIAN_POINT('Ctrl Pts',(10.4137642679999,15.2,-1.67169718000002));
#185389=CARTESIAN_POINT('Ctrl Pts',(10.4137642679999,11.6,-1.67169718000002));
#185390=CARTESIAN_POINT('Ctrl Pts',(10.4119793389999,15.2,-1.67102772400002));
#185391=CARTESIAN_POINT('Ctrl Pts',(10.4119793389999,11.6,-1.67102772400002));
#185392=CARTESIAN_POINT('Ctrl Pts',(10.4102005829999,15.2,-1.67036243400001));
#185393=CARTESIAN_POINT('Ctrl Pts',(10.4102005829999,11.6,-1.67036243400001));
#185394=CARTESIAN_POINT('Ctrl Pts',(10.4084280179999,15.2,-1.66970130200002));
#185395=CARTESIAN_POINT('Ctrl Pts',(10.4084280179999,11.6,-1.66970130200002));
#185396=CARTESIAN_POINT('Ctrl Pts',(10.4066616649999,15.2,-1.66904432200001));
#185397=CARTESIAN_POINT('Ctrl Pts',(10.4066616649999,11.6,-1.66904432200001));
#185398=CARTESIAN_POINT('Ctrl Pts',(10.4049015419999,15.2,-1.66839149000001));
#185399=CARTESIAN_POINT('Ctrl Pts',(10.4049015419999,11.6,-1.66839149000001));
#185400=CARTESIAN_POINT('Ctrl Pts',(10.4031476679999,15.2,-1.66774280000002));
#185401=CARTESIAN_POINT('Ctrl Pts',(10.4031476679999,11.6,-1.66774280000002));
#185402=CARTESIAN_POINT('Ctrl Pts',(10.4014000639999,15.2,-1.66709824500002));
#185403=CARTESIAN_POINT('Ctrl Pts',(10.4014000639999,11.6,-1.66709824500002));
#185404=CARTESIAN_POINT('Ctrl Pts',(10.3996587479999,15.2,-1.66645782000002));
#185405=CARTESIAN_POINT('Ctrl Pts',(10.3996587479999,11.6,-1.66645782000002));
#185406=CARTESIAN_POINT('Ctrl Pts',(10.3979237409999,15.2,-1.66582151900001));
#185407=CARTESIAN_POINT('Ctrl Pts',(10.3979237409999,11.6,-1.66582151900002));
#185408=CARTESIAN_POINT('Ctrl Pts',(10.3961950619999,15.2,-1.66518933700001));
#185409=CARTESIAN_POINT('Ctrl Pts',(10.3961950619999,11.6,-1.66518933700001));
#185410=CARTESIAN_POINT('Ctrl Pts',(10.3944727309999,15.2,-1.66456126800002));
#185411=CARTESIAN_POINT('Ctrl Pts',(10.3944727309999,11.6,-1.66456126800002));
#185412=CARTESIAN_POINT('Ctrl Pts',(10.3927567679999,15.2,-1.66393730500001));
#185413=CARTESIAN_POINT('Ctrl Pts',(10.3927567679999,11.6,-1.66393730500001));
#185414=CARTESIAN_POINT('Ctrl Pts',(10.3910471929999,15.2,-1.66331744300001));
#185415=CARTESIAN_POINT('Ctrl Pts',(10.3910471929999,11.6,-1.66331744300001));
#185416=CARTESIAN_POINT('Ctrl Pts',(10.3893440259999,15.2,-1.66270167600001));
#185417=CARTESIAN_POINT('Ctrl Pts',(10.3893440259999,11.6,-1.66270167600001));
#185418=CARTESIAN_POINT('Ctrl Pts',(10.3876472859999,15.2,-1.66208999800002));
#185419=CARTESIAN_POINT('Ctrl Pts',(10.3876472859999,11.6,-1.66208999800002));
#185420=CARTESIAN_POINT('Ctrl Pts',(10.3859569939999,15.2,-1.66148240200001));
#185421=CARTESIAN_POINT('Ctrl Pts',(10.3859569939999,11.6,-1.66148240200001));
#185422=CARTESIAN_POINT('Ctrl Pts',(10.3842731709999,15.2,-1.66087888300002));
#185423=CARTESIAN_POINT('Ctrl Pts',(10.3842731709999,11.6,-1.66087888300002));
#185424=CARTESIAN_POINT('Ctrl Pts',(10.3825958339999,15.2,-1.66027943500001));
#185425=CARTESIAN_POINT('Ctrl Pts',(10.3825958339999,11.6,-1.66027943500001));
#185426=CARTESIAN_POINT('Ctrl Pts',(10.3809250079999,15.2,-1.65968405100001));
#185427=CARTESIAN_POINT('Ctrl Pts',(10.3809250079999,11.6,-1.65968405100001));
#185428=CARTESIAN_POINT('Ctrl Pts',(10.3792607089999,15.2,-1.65909272500001));
#185429=CARTESIAN_POINT('Ctrl Pts',(10.3792607089999,11.6,-1.65909272500001));
#185430=CARTESIAN_POINT('Ctrl Pts',(10.3776029619999,15.2,-1.65850545200001));
#185431=CARTESIAN_POINT('Ctrl Pts',(10.3776029619999,11.6,-1.65850545200001));
#185432=CARTESIAN_POINT('Ctrl Pts',(10.3759517829999,15.2,-1.65792222500002));
#185433=CARTESIAN_POINT('Ctrl Pts',(10.3759517829999,11.6,-1.65792222500002));
#185434=CARTESIAN_POINT('Ctrl Pts',(10.3743071949999,15.2,-1.65734303700001));
#185435=CARTESIAN_POINT('Ctrl Pts',(10.3743071949999,11.6,-1.65734303700001));
#185436=CARTESIAN_POINT('Ctrl Pts',(10.3726692179999,15.2,-1.65676788300001));
#185437=CARTESIAN_POINT('Ctrl Pts',(10.3726692179999,11.6,-1.65676788300001));
#185438=CARTESIAN_POINT('Ctrl Pts',(10.3710378729999,15.2,-1.65619675500002));
#185439=CARTESIAN_POINT('Ctrl Pts',(10.3710378729999,11.6,-1.65619675500002));
#185440=CARTESIAN_POINT('Ctrl Pts',(10.3694131819999,15.2,-1.65562964900001));
#185441=CARTESIAN_POINT('Ctrl Pts',(10.3694131819999,11.6,-1.65562964900001));
#185442=CARTESIAN_POINT('Ctrl Pts',(10.3677951629999,15.2,-1.65506655600002));
#185443=CARTESIAN_POINT('Ctrl Pts',(10.3677951629999,11.6,-1.65506655600002));
#185444=CARTESIAN_POINT('Ctrl Pts',(10.3661838399999,15.2,-1.65450747100001));
#185445=CARTESIAN_POINT('Ctrl Pts',(10.3661838399999,11.6,-1.65450747100001));
#185446=CARTESIAN_POINT('Ctrl Pts',(10.3645792329999,15.2,-1.65395238800001));
#185447=CARTESIAN_POINT('Ctrl Pts',(10.3645792329999,11.6,-1.65395238800001));
#185448=CARTESIAN_POINT('Ctrl Pts',(10.3629813619999,15.2,-1.65340129900001));
#185449=CARTESIAN_POINT('Ctrl Pts',(10.3629813619999,11.6,-1.65340129900002));
#185450=CARTESIAN_POINT('Ctrl Pts',(10.3613902499999,15.2,-1.65285419800002));
#185451=CARTESIAN_POINT('Ctrl Pts',(10.3613902499999,11.6,-1.65285419800002));
#185452=CARTESIAN_POINT('Ctrl Pts',(10.3598059159999,15.2,-1.65231108000001));
#185453=CARTESIAN_POINT('Ctrl Pts',(10.3598059159999,11.6,-1.65231108000001));
#185454=CARTESIAN_POINT('Ctrl Pts',(10.3582283849999,15.2,-1.65177193600002));
#185455=CARTESIAN_POINT('Ctrl Pts',(10.3582283849999,11.6,-1.65177193600002));
#185456=CARTESIAN_POINT('Ctrl Pts',(10.3566576739999,15.2,-1.65123676100002));
#185457=CARTESIAN_POINT('Ctrl Pts',(10.3566576739999,11.6,-1.65123676100002));
#185458=CARTESIAN_POINT('Ctrl Pts',(10.3550938079999,15.2,-1.65070554700002));
#185459=CARTESIAN_POINT('Ctrl Pts',(10.3550938079999,11.6,-1.65070554700002));
#185460=CARTESIAN_POINT('Ctrl Pts',(10.3535368059999,15.2,-1.65017828800002));
#185461=CARTESIAN_POINT('Ctrl Pts',(10.3535368059999,11.6,-1.65017828800002));
#185462=CARTESIAN_POINT('Ctrl Pts',(10.3519866919999,15.2,-1.64965497700001));
#185463=CARTESIAN_POINT('Ctrl Pts',(10.3519866919999,11.6,-1.64965497700001));
#185464=CARTESIAN_POINT('Ctrl Pts',(10.3504434859999,15.2,-1.64913560700001));
#185465=CARTESIAN_POINT('Ctrl Pts',(10.3504434859999,11.6,-1.64913560700001));
#185466=CARTESIAN_POINT('Ctrl Pts',(10.3489072109999,15.2,-1.64862017200001));
#185467=CARTESIAN_POINT('Ctrl Pts',(10.3489072109999,11.6,-1.64862017200001));
#185468=CARTESIAN_POINT('Ctrl Pts',(10.3473778879999,15.2,-1.64810866500002));
#185469=CARTESIAN_POINT('Ctrl Pts',(10.3473778879999,11.6,-1.64810866500002));
#185470=CARTESIAN_POINT('Ctrl Pts',(10.3458555399999,15.2,-1.64760107700001));
#185471=CARTESIAN_POINT('Ctrl Pts',(10.3458555399999,11.6,-1.64760107700001));
#185472=CARTESIAN_POINT('Ctrl Pts',(10.3443401869999,15.2,-1.64709740400002));
#185473=CARTESIAN_POINT('Ctrl Pts',(10.3443401869999,11.6,-1.64709740400002));
#185474=CARTESIAN_POINT('Ctrl Pts',(10.3428318549999,15.2,-1.64659763700001));
#185475=CARTESIAN_POINT('Ctrl Pts',(10.3428318549999,11.6,-1.64659763700001));
#185476=CARTESIAN_POINT('Ctrl Pts',(10.3413305619999,15.2,-1.64610176900001));
#185477=CARTESIAN_POINT('Ctrl Pts',(10.3413305619999,11.6,-1.64610176900002));
#185478=CARTESIAN_POINT('Ctrl Pts',(10.3398363339999,15.2,-1.64560979500001));
#185479=CARTESIAN_POINT('Ctrl Pts',(10.3398363339999,11.6,-1.64560979500001));
#185480=CARTESIAN_POINT('Ctrl Pts',(10.3383491889999,15.2,-1.64512170500001));
#185481=CARTESIAN_POINT('Ctrl Pts',(10.3383491889999,11.6,-1.64512170500001));
#185482=CARTESIAN_POINT('Ctrl Pts',(10.3368691539999,15.2,-1.64463749400001));
#185483=CARTESIAN_POINT('Ctrl Pts',(10.3368691539999,11.6,-1.64463749400001));
#185484=CARTESIAN_POINT('Ctrl Pts',(10.3353962489999,15.2,-1.64415715300001));
#185485=CARTESIAN_POINT('Ctrl Pts',(10.3353962489999,11.6,-1.64415715300001));
#185486=CARTESIAN_POINT('Ctrl Pts',(10.3339304969999,15.2,-1.64368067500002));
#185487=CARTESIAN_POINT('Ctrl Pts',(10.3339304969999,11.6,-1.64368067500002));
#185488=CARTESIAN_POINT('Ctrl Pts',(10.3324719229999,15.2,-1.64320805500001));
#185489=CARTESIAN_POINT('Ctrl Pts',(10.3324719229999,11.6,-1.64320805500001));
#185490=CARTESIAN_POINT('Ctrl Pts',(10.3310205459999,15.2,-1.64273928400001));
#185491=CARTESIAN_POINT('Ctrl Pts',(10.3310205459999,11.6,-1.64273928400001));
#185492=CARTESIAN_POINT('Ctrl Pts',(10.3295763909999,15.2,-1.64227435400001));
#185493=CARTESIAN_POINT('Ctrl Pts',(10.3295763909999,11.6,-1.64227435400001));
#185494=CARTESIAN_POINT('Ctrl Pts',(10.3281394819999,15.2,-1.64181325700001));
#185495=CARTESIAN_POINT('Ctrl Pts',(10.3281394819999,11.6,-1.64181325700001));
#185496=CARTESIAN_POINT('Ctrl Pts',(10.3267098399999,15.2,-1.64135598800002));
#185497=CARTESIAN_POINT('Ctrl Pts',(10.3267098399999,11.6,-1.64135598800002));
#185498=CARTESIAN_POINT('Ctrl Pts',(10.3252874889999,15.2,-1.64090253800001));
#185499=CARTESIAN_POINT('Ctrl Pts',(10.3252874889999,11.6,-1.64090253800001));
#185500=CARTESIAN_POINT('Ctrl Pts',(10.3238724529999,15.2,-1.64045290000002));
#185501=CARTESIAN_POINT('Ctrl Pts',(10.3238724529999,11.6,-1.64045290000002));
#185502=CARTESIAN_POINT('Ctrl Pts',(10.3224647549999,15.2,-1.64000706600001));
#185503=CARTESIAN_POINT('Ctrl Pts',(10.3224647549999,11.6,-1.64000706600001));
#185504=CARTESIAN_POINT('Ctrl Pts',(10.3210644169999,15.2,-1.63956502700001));
#185505=CARTESIAN_POINT('Ctrl Pts',(10.3210644169999,11.6,-1.63956502700001));
#185506=CARTESIAN_POINT('Ctrl Pts',(10.3196714649999,15.2,-1.63912677800001));
#185507=CARTESIAN_POINT('Ctrl Pts',(10.3196714649999,11.6,-1.63912677800001));
#185508=CARTESIAN_POINT('Ctrl Pts',(10.3182859209999,15.2,-1.63869230900001));
#185509=CARTESIAN_POINT('Ctrl Pts',(10.3182859209999,11.6,-1.63869230900001));
#185510=CARTESIAN_POINT('Ctrl Pts',(10.3169078099999,15.2,-1.63826161400001));
#185511=CARTESIAN_POINT('Ctrl Pts',(10.3169078099999,11.6,-1.63826161400001));
#185512=CARTESIAN_POINT('Ctrl Pts',(10.3155371549999,15.2,-1.63783468500001));
#185513=CARTESIAN_POINT('Ctrl Pts',(10.3155371549999,11.6,-1.63783468500002));
#185514=CARTESIAN_POINT('Ctrl Pts',(10.3141739779999,15.2,-1.63741151200002));
#185515=CARTESIAN_POINT('Ctrl Pts',(10.3141739779999,11.6,-1.63741151200002));
#185516=CARTESIAN_POINT('Ctrl Pts',(10.3128183069999,15.2,-1.63699208900002));
#185517=CARTESIAN_POINT('Ctrl Pts',(10.3128183069999,11.6,-1.63699208900002));
#185518=CARTESIAN_POINT('Ctrl Pts',(10.3114701629999,15.2,-1.63657640900002));
#185519=CARTESIAN_POINT('Ctrl Pts',(10.3114701629999,11.6,-1.63657640900002));
#185520=CARTESIAN_POINT('Ctrl Pts',(10.3101295719999,15.2,-1.63616446000002));
#185521=CARTESIAN_POINT('Ctrl Pts',(10.3101295719999,11.6,-1.63616446000002));
#185522=CARTESIAN_POINT('Ctrl Pts',(10.3087965579999,15.2,-1.63575623800002));
#185523=CARTESIAN_POINT('Ctrl Pts',(10.3087965579999,11.6,-1.63575623800002));
#185524=CARTESIAN_POINT('Ctrl Pts',(10.3074711439999,15.2,-1.63535173400001));
#185525=CARTESIAN_POINT('Ctrl Pts',(10.3074711439999,11.6,-1.63535173400001));
#185526=CARTESIAN_POINT('Ctrl Pts',(10.3061533569999,15.2,-1.63495093800002));
#185527=CARTESIAN_POINT('Ctrl Pts',(10.3061533569999,11.6,-1.63495093800002));
#185528=CARTESIAN_POINT('Ctrl Pts',(10.3048432199999,15.2,-1.63455384400002));
#185529=CARTESIAN_POINT('Ctrl Pts',(10.3048432199999,11.6,-1.63455384400002));
#185530=CARTESIAN_POINT('Ctrl Pts',(10.3035407569999,15.2,-1.63416044200002));
#185531=CARTESIAN_POINT('Ctrl Pts',(10.3035407569999,11.6,-1.63416044200002));
#185532=CARTESIAN_POINT('Ctrl Pts',(10.3022459949999,15.2,-1.63377072600001));
#185533=CARTESIAN_POINT('Ctrl Pts',(10.3022459949999,11.6,-1.63377072600001));
#185534=CARTESIAN_POINT('Ctrl Pts',(10.3009589569999,15.2,-1.63338468500001));
#185535=CARTESIAN_POINT('Ctrl Pts',(10.3009589569999,11.6,-1.63338468500001));
#185536=CARTESIAN_POINT('Ctrl Pts',(10.2996796679999,15.2,-1.63300231200001));
#185537=CARTESIAN_POINT('Ctrl Pts',(10.2996796679999,11.6,-1.63300231200001));
#185538=CARTESIAN_POINT('Ctrl Pts',(10.2984081549999,15.2,-1.63262359900001));
#185539=CARTESIAN_POINT('Ctrl Pts',(10.2984081549999,11.6,-1.63262359900001));
#185540=CARTESIAN_POINT('Ctrl Pts',(10.2971444419999,15.2,-1.63224853600001));
#185541=CARTESIAN_POINT('Ctrl Pts',(10.2971444419999,11.6,-1.63224853600001));
#185542=CARTESIAN_POINT('Ctrl Pts',(10.2958885549999,15.2,-1.63187711700001));
#185543=CARTESIAN_POINT('Ctrl Pts',(10.2958885549999,11.6,-1.63187711700001));
#185544=CARTESIAN_POINT('Ctrl Pts',(10.2946405169999,15.2,-1.63150933000002));
#185545=CARTESIAN_POINT('Ctrl Pts',(10.2946405169999,11.6,-1.63150933000002));
#185546=CARTESIAN_POINT('Ctrl Pts',(10.2934003569999,15.2,-1.63114516800002));
#185547=CARTESIAN_POINT('Ctrl Pts',(10.2934003569999,11.6,-1.63114516800002));
#185548=CARTESIAN_POINT('Ctrl Pts',(10.2921680989999,15.2,-1.63078462400001));
#185549=CARTESIAN_POINT('Ctrl Pts',(10.2921680989999,11.6,-1.63078462400002));
#185550=CARTESIAN_POINT('Ctrl Pts',(10.2909437679999,15.2,-1.63042768700001));
#185551=CARTESIAN_POINT('Ctrl Pts',(10.2909437679999,11.6,-1.63042768700001));
#185552=CARTESIAN_POINT('Ctrl Pts',(10.2897273919999,15.2,-1.63007434800001));
#185553=CARTESIAN_POINT('Ctrl Pts',(10.2897273919999,11.6,-1.63007434800001));
#185554=CARTESIAN_POINT('Ctrl Pts',(10.2885189949999,15.2,-1.62972460000002));
#185555=CARTESIAN_POINT('Ctrl Pts',(10.2885189949999,11.6,-1.62972460000002));
#185556=CARTESIAN_POINT('Ctrl Pts',(10.2873186039999,15.2,-1.62937843300002));
#185557=CARTESIAN_POINT('Ctrl Pts',(10.2873186039999,11.6,-1.62937843300002));
#185558=CARTESIAN_POINT('Ctrl Pts',(10.2861262449999,15.2,-1.62903583900002));
#185559=CARTESIAN_POINT('Ctrl Pts',(10.2861262449999,11.6,-1.62903583900002));
#185560=CARTESIAN_POINT('Ctrl Pts',(10.2849419449999,15.2,-1.62869680700001));
#185561=CARTESIAN_POINT('Ctrl Pts',(10.2849419449999,11.6,-1.62869680700001));
#185562=CARTESIAN_POINT('Ctrl Pts',(10.2837657299999,15.2,-1.62836132900001));
#185563=CARTESIAN_POINT('Ctrl Pts',(10.2837657299999,11.6,-1.62836132900001));
#185564=CARTESIAN_POINT('Ctrl Pts',(10.2825976249999,15.2,-1.62802939700001));
#185565=CARTESIAN_POINT('Ctrl Pts',(10.2825976249999,11.6,-1.62802939700002));
#185566=CARTESIAN_POINT('Ctrl Pts',(10.2814376589999,15.2,-1.62770100000001));
#185567=CARTESIAN_POINT('Ctrl Pts',(10.2814376589999,11.6,-1.62770100000001));
#185568=CARTESIAN_POINT('Ctrl Pts',(10.2802858579999,15.2,-1.62737613100001));
#185569=CARTESIAN_POINT('Ctrl Pts',(10.2802858579999,11.6,-1.62737613100001));
#185570=CARTESIAN_POINT('Ctrl Pts',(10.2791422489999,15.2,-1.62705477900001));
#185571=CARTESIAN_POINT('Ctrl Pts',(10.2791422489999,11.6,-1.62705477900001));
#185572=CARTESIAN_POINT('Ctrl Pts',(10.2780068579999,15.2,-1.62673693400002));
#185573=CARTESIAN_POINT('Ctrl Pts',(10.2780068579999,11.6,-1.62673693400002));
#185574=CARTESIAN_POINT('Ctrl Pts',(10.2768797139999,15.2,-1.62642258900001));
#185575=CARTESIAN_POINT('Ctrl Pts',(10.2768797139999,11.6,-1.62642258900001));
#185576=CARTESIAN_POINT('Ctrl Pts',(10.2757608429999,15.2,-1.62611173200002));
#185577=CARTESIAN_POINT('Ctrl Pts',(10.2757608429999,11.6,-1.62611173200002));
#185578=CARTESIAN_POINT('Ctrl Pts',(10.2746502719999,15.2,-1.62580435500002));
#185579=CARTESIAN_POINT('Ctrl Pts',(10.2746502719999,11.6,-1.62580435500002));
#185580=CARTESIAN_POINT('Ctrl Pts',(10.2735480289999,15.2,-1.62550044900001));
#185581=CARTESIAN_POINT('Ctrl Pts',(10.2735480289999,11.6,-1.62550044900002));
#185582=CARTESIAN_POINT('Ctrl Pts',(10.2724541419999,15.2,-1.62520000200002));
#185583=CARTESIAN_POINT('Ctrl Pts',(10.2724541419999,11.6,-1.62520000200002));
#185584=CARTESIAN_POINT('Ctrl Pts',(10.2713686389999,15.2,-1.62490300700001));
#185585=CARTESIAN_POINT('Ctrl Pts',(10.2713686389999,11.6,-1.62490300700001));
#185586=CARTESIAN_POINT('Ctrl Pts',(10.2702915479999,15.2,-1.62460945400001));
#185587=CARTESIAN_POINT('Ctrl Pts',(10.2702915479999,11.6,-1.62460945400001));
#185588=CARTESIAN_POINT('Ctrl Pts',(10.2692228959999,15.2,-1.62431933100001));
#185589=CARTESIAN_POINT('Ctrl Pts',(10.2692228959999,11.6,-1.62431933100002));
#185590=CARTESIAN_POINT('Ctrl Pts',(10.2681627099999,15.2,-1.62403262900002));
#185591=CARTESIAN_POINT('Ctrl Pts',(10.2681627099999,11.6,-1.62403262900002));
#185592=CARTESIAN_POINT('Ctrl Pts',(10.2671110219999,15.2,-1.62374934000002));
#185593=CARTESIAN_POINT('Ctrl Pts',(10.2671110219999,11.6,-1.62374934000002));
#185594=CARTESIAN_POINT('Ctrl Pts',(10.2660678569999,15.2,-1.62346945200001));
#185595=CARTESIAN_POINT('Ctrl Pts',(10.2660678569999,11.6,-1.62346945200001));
#185596=CARTESIAN_POINT('Ctrl Pts',(10.2650332449999,15.2,-1.62319295600001));
#185597=CARTESIAN_POINT('Ctrl Pts',(10.2650332449999,11.6,-1.62319295600002));
#185598=CARTESIAN_POINT('Ctrl Pts',(10.2640072149999,15.2,-1.62291984100001));
#185599=CARTESIAN_POINT('Ctrl Pts',(10.2640072149999,11.6,-1.62291984100001));
#185600=CARTESIAN_POINT('Ctrl Pts',(10.2629897939999,15.2,-1.62265009700001));
#185601=CARTESIAN_POINT('Ctrl Pts',(10.2629897939999,11.6,-1.62265009700001));
#185602=CARTESIAN_POINT('Ctrl Pts',(10.2619810129999,15.2,-1.62238371500001));
#185603=CARTESIAN_POINT('Ctrl Pts',(10.2619810129999,11.6,-1.62238371500001));
#185604=CARTESIAN_POINT('Ctrl Pts',(10.2609808999999,15.2,-1.62212068400001));
#185605=CARTESIAN_POINT('Ctrl Pts',(10.2609808999999,11.6,-1.62212068400002));
#185606=CARTESIAN_POINT('Ctrl Pts',(10.2599894849999,15.2,-1.62186099200001));
#185607=CARTESIAN_POINT('Ctrl Pts',(10.2599894849999,11.6,-1.62186099200001));
#185608=CARTESIAN_POINT('Ctrl Pts',(10.2590067959999,15.2,-1.62160463100002));
#185609=CARTESIAN_POINT('Ctrl Pts',(10.2590067959999,11.6,-1.62160463100002));
#185610=CARTESIAN_POINT('Ctrl Pts',(10.2580328639999,15.2,-1.62135159000002));
#185611=CARTESIAN_POINT('Ctrl Pts',(10.2580328639999,11.6,-1.62135159000002));
#185612=CARTESIAN_POINT('Ctrl Pts',(10.2570677169999,15.2,-1.62110185800001));
#185613=CARTESIAN_POINT('Ctrl Pts',(10.2570677169999,11.6,-1.62110185800001));
#185614=CARTESIAN_POINT('Ctrl Pts',(10.2561113859999,15.2,-1.62085542400002));
#185615=CARTESIAN_POINT('Ctrl Pts',(10.2561113859999,11.6,-1.62085542400002));
#185616=CARTESIAN_POINT('Ctrl Pts',(10.2551638999999,15.2,-1.62061227900002));
#185617=CARTESIAN_POINT('Ctrl Pts',(10.2551638999999,11.6,-1.62061227900002));
#185618=CARTESIAN_POINT('Ctrl Pts',(10.2542252899999,15.2,-1.62037241000001));
#185619=CARTESIAN_POINT('Ctrl Pts',(10.2542252899999,11.6,-1.62037241000002));
#185620=CARTESIAN_POINT('Ctrl Pts',(10.2532955859999,15.2,-1.62013580700001));
#185621=CARTESIAN_POINT('Ctrl Pts',(10.2532955859999,11.6,-1.62013580700001));
#185622=CARTESIAN_POINT('Ctrl Pts',(10.2523748169999,15.2,-1.61990246000002));
#185623=CARTESIAN_POINT('Ctrl Pts',(10.2523748169999,11.6,-1.61990246000002));
#185624=CARTESIAN_POINT('Ctrl Pts',(10.2514630149999,15.2,-1.61967235800001));
#185625=CARTESIAN_POINT('Ctrl Pts',(10.2514630149999,11.6,-1.61967235800002));
#185626=CARTESIAN_POINT('Ctrl Pts',(10.2505602109999,15.2,-1.61944548900002));
#185627=CARTESIAN_POINT('Ctrl Pts',(10.2505602109999,11.6,-1.61944548900002));
#185628=CARTESIAN_POINT('Ctrl Pts',(10.2496715819999,15.2,-1.61922313000002));
#185629=CARTESIAN_POINT('Ctrl Pts',(10.2496715819999,11.6,-1.61922313000002));
#185630=CARTESIAN_POINT('Ctrl Pts',(10.2489688509999,15.2,-1.61904803300001));
#185631=CARTESIAN_POINT('Ctrl Pts',(10.2489688509999,11.6,-1.61904803300001));
#185632=CARTESIAN_POINT('Ctrl Pts',(10.2484470889999,15.2,-1.61891844100001));
#185633=CARTESIAN_POINT('Ctrl Pts',(10.2484470889999,11.6,-1.61891844100001));
#185634=CARTESIAN_POINT('Ctrl Pts',(10.2481027029999,15.2,-1.61883308400002));
#185635=CARTESIAN_POINT('Ctrl Pts',(10.2481027029999,11.6,-1.61883308400002));
#185636=CARTESIAN_POINT('Ctrl Pts',(10.2479334559999,15.2,-1.61879118000002));
#185637=CARTESIAN_POINT('Ctrl Pts',(10.2479334559999,11.6,-1.61879118000002));
#185638=CARTESIAN_POINT('',(10.2479334559999,12.2,-1.61879118000002));
#185639=CARTESIAN_POINT('',(10.2479334559999,15.2,-1.61879118000002));
#185640=CARTESIAN_POINT('',(10.2479334559999,12.2,-1.61879118000002));
#185641=CARTESIAN_POINT('Ctrl Pts',(11.2922242989999,12.2,-2.17615954700001));
#185642=CARTESIAN_POINT('Ctrl Pts',(11.2891672434446,12.2,-2.17386408658301));
#185643=CARTESIAN_POINT('Ctrl Pts',(11.2861128828178,12.2,-2.17157605041022));
#185644=CARTESIAN_POINT('Ctrl Pts',(11.2830612235708,12.2,-2.16929543995597));
#185645=CARTESIAN_POINT('Ctrl Pts',(11.2800095643238,12.2,-2.16701482950172));
#185646=CARTESIAN_POINT('Ctrl Pts',(11.2769606036145,12.2,-2.16474164385347));
#185647=CARTESIAN_POINT('Ctrl Pts',(11.2739143610727,12.2,-2.16247588328007));
#185648=CARTESIAN_POINT('Ctrl Pts',(11.2708681185308,12.2,-2.16021012270667));
#185649=CARTESIAN_POINT('Ctrl Pts',(11.2678245931694,12.2,-2.15795178692656));
#185650=CARTESIAN_POINT('Ctrl Pts',(11.2647838291545,12.2,-2.15570087596567));
#185651=CARTESIAN_POINT('Ctrl Pts',(11.2617430645872,12.2,-2.15344996459586));
#185652=CARTESIAN_POINT('Ctrl Pts',(11.2587050621956,12.2,-2.15120647715313));
#185653=CARTESIAN_POINT('Ctrl Pts',(11.2556698710466,12.2,-2.14897041128751));
#185654=CARTESIAN_POINT('Ctrl Pts',(11.2526346804489,12.2,-2.1467343458281));
#185655=CARTESIAN_POINT('Ctrl Pts',(11.2496023012261,12.2,-2.14450570232663));
#185656=CARTESIAN_POINT('Ctrl Pts',(11.2465727734614,12.2,-2.14228448028298));
#185657=CARTESIAN_POINT('Ctrl Pts',(11.2435432456967,12.2,-2.14006325823933));
#185658=CARTESIAN_POINT('Ctrl Pts',(11.2405165681844,12.2,-2.13784945607778));
#185659=CARTESIAN_POINT('Ctrl Pts',(11.2374927780305,12.2,-2.13564307406463));
#185660=CARTESIAN_POINT('Ctrl Pts',(11.2334610580085,12.2,-2.13270123151403));
#185661=CARTESIAN_POINT('Ctrl Pts',(11.2294344705125,12.2,-2.12977257764798));
#185662=CARTESIAN_POINT('Ctrl Pts',(11.2254131171741,12.2,-2.12685711171831));
#185663=CARTESIAN_POINT('Ctrl Pts',(11.2223971014853,12.2,-2.12467051177452));
#185664=CARTESIAN_POINT('Ctrl Pts',(11.2193840292308,12.2,-2.12249132815782));
#185665=CARTESIAN_POINT('Ctrl Pts',(11.2163739430854,12.2,-2.12031956030152));
#185666=CARTESIAN_POINT('Ctrl Pts',(11.2133638574868,12.2,-2.11814779283977));
#185667=CARTESIAN_POINT('Ctrl Pts',(11.2103567582631,12.2,-2.11598344095264));
#185668=CARTESIAN_POINT('Ctrl Pts',(11.2073526851642,12.2,-2.11382650248998));
#185669=CARTESIAN_POINT('Ctrl Pts',(11.2043486120653,12.2,-2.11166956402733));
#185670=CARTESIAN_POINT('Ctrl Pts',(11.2013475658352,12.2,-2.10952003876322));
#185671=CARTESIAN_POINT('Ctrl Pts',(11.1983495872639,12.2,-2.10737792524802));
#185672=CARTESIAN_POINT('Ctrl Pts',(11.1953516086925,12.2,-2.10523581173282));
#185673=CARTESIAN_POINT('Ctrl Pts',(11.1923566985575,12.2,-2.10310110905096));
#185674=CARTESIAN_POINT('Ctrl Pts',(11.189364898486,12.2,-2.10097381699356));
#185675=CARTESIAN_POINT('Ctrl Pts',(11.1863730984144,12.2,-2.09884652493616));
#185676=CARTESIAN_POINT('Ctrl Pts',(11.1833844089172,12.2,-2.09672664170424));
#185677=CARTESIAN_POINT('Ctrl Pts',(11.1803988718171,12.2,-2.09461416573868));
#185678=CARTESIAN_POINT('Ctrl Pts',(11.1774133347169,12.2,-2.09250168977312));
#185679=CARTESIAN_POINT('Ctrl Pts',(11.1744309502416,12.2,-2.09039662064872));
#185680=CARTESIAN_POINT('Ctrl Pts',(11.1714517601411,12.2,-2.08829895714059));
#185681=CARTESIAN_POINT('Ctrl Pts',(11.1684725694993,12.2,-2.08620129325139));
#185682=CARTESIAN_POINT('Ctrl Pts',(11.1654965735335,12.2,-2.08411103414762));
#185683=CARTESIAN_POINT('Ctrl Pts',(11.1625238148519,12.2,-2.08202817730424));
#185684=CARTESIAN_POINT('Ctrl Pts',(11.1595510567103,12.2,-2.07994532083926));
#185685=CARTESIAN_POINT('Ctrl Pts',(11.1565815351994,12.2,-2.07786986734391));
#185686=CARTESIAN_POINT('Ctrl Pts',(11.1536152939511,12.2,-2.07580181285825));
#185687=CARTESIAN_POINT('Ctrl Pts',(11.1506490527027,12.2,-2.07373375837259));
#185688=CARTESIAN_POINT('Ctrl Pts',(11.1476860917529,12.2,-2.0716731043677));
#185689=CARTESIAN_POINT('Ctrl Pts',(11.1447264536524,12.2,-2.06961984698462));
#185690=CARTESIAN_POINT('Ctrl Pts',(11.1417668155519,12.2,-2.06756658960153));
#185691=CARTESIAN_POINT('Ctrl Pts',(11.1388105006593,12.2,-2.0655207303759));
#185692=CARTESIAN_POINT('Ctrl Pts',(11.1358575515583,12.2,-2.06348226449162));
#185693=CARTESIAN_POINT('Ctrl Pts',(11.1329046024572,12.2,-2.06144379860735));
#185694=CARTESIAN_POINT('Ctrl Pts',(11.1299550190977,12.2,-2.05941272813111));
#185695=CARTESIAN_POINT('Ctrl Pts',(11.1270088455794,12.2,-2.057389048204));
#185696=CARTESIAN_POINT('Ctrl Pts',(11.1240626720612,12.2,-2.05536536827689));
#185697=CARTESIAN_POINT('Ctrl Pts',(11.1211199089177,12.2,-2.05334908044925));
#185698=CARTESIAN_POINT('Ctrl Pts',(11.1181805983574,12.2,-2.05134018047958));
#185699=CARTESIAN_POINT('Ctrl Pts',(11.115241287263,12.2,-2.04933128014495));
#185700=CARTESIAN_POINT('Ctrl Pts',(11.1123054290197,12.2,-2.04732976760407));
#185701=CARTESIAN_POINT('Ctrl Pts',(11.109373068344,12.2,-2.04533564077359));
#185702=CARTESIAN_POINT('Ctrl Pts',(11.106440708201,12.2,-2.04334151430537));
#185703=CARTESIAN_POINT('Ctrl Pts',(11.1035118444734,12.2,-2.04135477375985));
#185704=CARTESIAN_POINT('Ctrl Pts',(11.100586522684,12.2,-2.03937541465041));
#185705=CARTESIAN_POINT('Ctrl Pts',(11.0976612008945,12.2,-2.03739605554096));
#185706=CARTESIAN_POINT('Ctrl Pts',(11.0947394202922,12.2,-2.03542407828059));
#185707=CARTESIAN_POINT('Ctrl Pts',(11.0918212251902,12.2,-2.03345947931095));
#185708=CARTESIAN_POINT('Ctrl Pts',(11.0889030300882,12.2,-2.0314948803413));
#185709=CARTESIAN_POINT('Ctrl Pts',(11.0859884198275,12.2,-2.02953765971245));
#185710=CARTESIAN_POINT('Ctrl Pts',(11.0830774402249,12.2,-2.02758781424162));
#185711=CARTESIAN_POINT('Ctrl Pts',(11.0801664606223,12.2,-2.0256379687708));
#185712=CARTESIAN_POINT('Ctrl Pts',(11.0772591111946,12.2,-2.02369549840801));
#185713=CARTESIAN_POINT('Ctrl Pts',(11.0743554365915,12.2,-2.02176039893602));
#185714=CARTESIAN_POINT('Ctrl Pts',(11.0714517619883,12.2,-2.01982529946402));
#185715=CARTESIAN_POINT('Ctrl Pts',(11.0685517618502,12.2,-2.01789757206525));
#185716=CARTESIAN_POINT('Ctrl Pts',(11.0656554825603,12.2,-2.01597721191324));
#185717=CARTESIAN_POINT('Ctrl Pts',(11.0627592032704,12.2,-2.01405685176123));
#185718=CARTESIAN_POINT('Ctrl Pts',(11.0598666428919,12.2,-2.0121438583805));
#185719=CARTESIAN_POINT('Ctrl Pts',(11.0569778483713,12.2,-2.01023822844873));
#185720=CARTESIAN_POINT('Ctrl Pts',(11.054089053326,12.2,-2.00833259817078));
#185721=CARTESIAN_POINT('Ctrl Pts',(11.0512040246067,12.2,-2.00643433216156));
#185722=CARTESIAN_POINT('Ctrl Pts',(11.0483228056052,12.2,-2.00454342530442));
#185723=CARTESIAN_POINT('Ctrl Pts',(11.0444811811421,12.2,-2.00202221673409));
#185724=CARTESIAN_POINT('Ctrl Pts',(11.0406463315365,12.2,-1.99951409062871));
#185725=CARTESIAN_POINT('Ctrl Pts',(11.0368183655713,12.2,-1.99701903872073));
#185726=CARTESIAN_POINT('Ctrl Pts',(11.0339473909669,12.2,-1.99514774970476));
#185727=CARTESIAN_POINT('Ctrl Pts',(11.0310802880101,12.2,-1.99328381496872));
#185728=CARTESIAN_POINT('Ctrl Pts',(11.0282171033456,12.2,-1.99142722890091));
#185729=CARTESIAN_POINT('Ctrl Pts',(11.0253539186811,12.2,-1.9895706428331));
#185730=CARTESIAN_POINT('Ctrl Pts',(11.0224946528025,12.2,-1.98772140635225));
#185731=CARTESIAN_POINT('Ctrl Pts',(11.019639350364,12.2,-1.98587951441817));
#185732=CARTESIAN_POINT('Ctrl Pts',(11.0167840474069,12.2,-1.98403762214947));
#185733=CARTESIAN_POINT('Ctrl Pts',(11.0139327091425,12.2,-1.98220307514953));
#185734=CARTESIAN_POINT('Ctrl Pts',(11.0110853821042,12.2,-1.98037586830164));
#185735=CARTESIAN_POINT('Ctrl Pts',(11.0072889469153,12.2,-1.97793959305769));
#185736=CARTESIAN_POINT('Ctrl Pts',(11.0034996427782,12.2,-1.97551636664261));
#185737=CARTESIAN_POINT('Ctrl Pts',(10.9997175803092,12.2,-1.97310617867212));
#185738=CARTESIAN_POINT('Ctrl Pts',(10.9968810333285,12.2,-1.97129853761216));
#185739=CARTESIAN_POINT('Ctrl Pts',(10.9940485607195,12.2,-1.96949823050554));
#185740=CARTESIAN_POINT('Ctrl Pts',(10.9912202085138,12.2,-1.96770525139693));
#185741=CARTESIAN_POINT('Ctrl Pts',(10.9883918563082,12.2,-1.96591227228832));
#185742=CARTESIAN_POINT('Ctrl Pts',(10.9855676239795,12.2,-1.96412662250736));
#185743=CARTESIAN_POINT('Ctrl Pts',(10.982747561373,12.2,-1.96234829644598));
#185744=CARTESIAN_POINT('Ctrl Pts',(10.9789874775562,12.2,-1.95997719481543));
#185745=CARTESIAN_POINT('Ctrl Pts',(10.9752348046818,12.2,-1.95761911140555));
#185746=CARTESIAN_POINT('Ctrl Pts',(10.9714896550332,12.2,-1.95527403649996));
#185747=CARTESIAN_POINT('Ctrl Pts',(10.9677445053847,12.2,-1.95292896159437));
#185748=CARTESIAN_POINT('Ctrl Pts',(10.9640068792231,12.2,-1.95059689427086));
#185749=CARTESIAN_POINT('Ctrl Pts',(10.9602768916317,12.2,-1.9482778206458));
#185750=CARTESIAN_POINT('Ctrl Pts',(10.9565469045485,12.2,-1.94595874733671));
#185751=CARTESIAN_POINT('Ctrl Pts',(10.9528245563768,12.2,-1.94365266726341));
#185752=CARTESIAN_POINT('Ctrl Pts',(10.9491099612191,12.2,-1.9413595692182));
#185753=CARTESIAN_POINT('Ctrl Pts',(10.9453953655553,12.2,-1.93906647086055));
#185754=CARTESIAN_POINT('Ctrl Pts',(10.9416885239598,12.2,-1.93678635215709));
#185755=CARTESIAN_POINT('Ctrl Pts',(10.9379895503701,12.2,-1.93451920114596));
#185756=CARTESIAN_POINT('Ctrl Pts',(10.9342905772844,12.2,-1.93225205044372));
#185757=CARTESIAN_POINT('Ctrl Pts',(10.9305994745283,12.2,-1.9299978656426));
#185758=CARTESIAN_POINT('Ctrl Pts',(10.9269163580511,12.2,-1.92775663365831));
#185759=CARTESIAN_POINT('Ctrl Pts',(10.923233241072,12.2,-1.92551540136864));
#185760=CARTESIAN_POINT('Ctrl Pts',(10.9195581097752,12.2,-1.92328712073386));
#185761=CARTESIAN_POINT('Ctrl Pts',(10.9158910832262,12.2,-1.92107177767024));
#185762=CARTESIAN_POINT('Ctrl Pts',(10.9122240571768,12.2,-1.91885643490846));
#185763=CARTESIAN_POINT('Ctrl Pts',(10.9085651352116,12.2,-1.91665402927315));
#185764=CARTESIAN_POINT('Ctrl Pts',(10.9049144360651,12.2,-1.91446454589574));
#185765=CARTESIAN_POINT('Ctrl Pts',(10.9012637364212,12.2,-1.91227506222002));
#185766=CARTESIAN_POINT('Ctrl Pts',(10.8976212601338,12.2,-1.91009850048474));
#185767=CARTESIAN_POINT('Ctrl Pts',(10.8939871259362,12.2,-1.90793484358987));
#185768=CARTESIAN_POINT('Ctrl Pts',(10.8903529922338,12.2,-1.9057711869898));
#185769=CARTESIAN_POINT('Ctrl Pts',(10.8867272019106,12.2,-1.90362043733507));
#185770=CARTESIAN_POINT('Ctrl Pts',(10.8831098740249,12.2,-1.90148257656859));
#185771=CARTESIAN_POINT('Ctrl Pts',(10.8794925456463,12.2,-1.89934471551082));
#185772=CARTESIAN_POINT('Ctrl Pts',(10.8758836812763,12.2,-1.89721974320003));
#185773=CARTESIAN_POINT('Ctrl Pts',(10.8722834022473,12.2,-1.89510764358576));
#185774=CARTESIAN_POINT('Ctrl Pts',(10.8686831237089,12.2,-1.89299554425926));
#185775=CARTESIAN_POINT('Ctrl Pts',(10.8650914291048,12.2,-1.89089631763295));
#185776=CARTESIAN_POINT('Ctrl Pts',(10.8615084432857,12.2,-1.88880994502443));
#185777=CARTESIAN_POINT('Ctrl Pts',(10.8579254569785,12.2,-1.88672357213163));
#185778=CARTESIAN_POINT('Ctrl Pts',(10.854351177758,12.2,-1.88465005522851));
#185779=CARTESIAN_POINT('Ctrl Pts',(10.8507857302142,12.2,-1.88258937427356));
#185780=CARTESIAN_POINT('Ctrl Pts',(10.8472202831561,12.2,-1.88052869359938));
#185781=CARTESIAN_POINT('Ctrl Pts',(10.8436636666964,12.2,-1.87848085057874));
#185782=CARTESIAN_POINT('Ctrl Pts',(10.8401160080966,12.2,-1.87644582463269));
#185783=CARTESIAN_POINT('Ctrl Pts',(10.8365683490135,12.2,-1.87441079840937));
#185784=CARTESIAN_POINT('Ctrl Pts',(10.8330296438617,12.2,-1.87238858944281));
#185785=CARTESIAN_POINT('Ctrl Pts',(10.8295000217249,12.2,-1.87037918099996));
#185786=CARTESIAN_POINT('Ctrl Pts',(10.8259703995881,12.2,-1.86836977255711));
#185787=CARTESIAN_POINT('Ctrl Pts',(10.8224498602162,12.2,-1.8663731622852));
#185788=CARTESIAN_POINT('Ctrl Pts',(10.8189385286925,12.2,-1.86438933190062));
#185789=CARTESIAN_POINT('Ctrl Pts',(10.8154271976471,12.2,-1.86240550178633));
#185790=CARTESIAN_POINT('Ctrl Pts',(10.8119250765895,12.2,-1.86043444973703));
#185791=CARTESIAN_POINT('Ctrl Pts',(10.8084322903189,12.2,-1.85847615761851));
#185792=CARTESIAN_POINT('Ctrl Pts',(10.8049395035723,12.2,-1.85651786523317));
#185793=CARTESIAN_POINT('Ctrl Pts',(10.8014560547274,12.2,-1.85457233221203));
#185794=CARTESIAN_POINT('Ctrl Pts',(10.7979820704209,12.2,-1.85263953651124));
#185795=CARTESIAN_POINT('Ctrl Pts',(10.7945080865877,12.2,-1.85070674107379));
#185796=CARTESIAN_POINT('Ctrl Pts',(10.7910435691201,12.2,-1.84878668357314));
#185797=CARTESIAN_POINT('Ctrl Pts',(10.7875886467908,12.2,-1.84687934283934));
#185798=CARTESIAN_POINT('Ctrl Pts',(10.7841337239907,12.2,-1.84497200184567));
#185799=CARTESIAN_POINT('Ctrl Pts',(10.7806883968419,12.2,-1.84307737701742));
#185800=CARTESIAN_POINT('Ctrl Pts',(10.7772527967108,12.2,-1.84119544730457));
#185801=CARTESIAN_POINT('Ctrl Pts',(10.7738171970479,12.2,-1.83931351784814));
#185802=CARTESIAN_POINT('Ctrl Pts',(10.7703913249296,12.2,-1.83744428348651));
#185803=CARTESIAN_POINT('Ctrl Pts',(10.7669753105373,12.2,-1.83558772004443));
#185804=CARTESIAN_POINT('Ctrl Pts',(10.7635592956796,12.2,-1.8337311563494));
#185805=CARTESIAN_POINT('Ctrl Pts',(10.7601531412707,12.2,-1.83188726482158));
#185806=CARTESIAN_POINT('Ctrl Pts',(10.7567569796974,12.2,-1.83005602183371));
#185807=CARTESIAN_POINT('Ctrl Pts',(10.7533608185868,12.2,-1.82822477909535));
#185808=CARTESIAN_POINT('Ctrl Pts',(10.7499746495492,12.2,-1.82640618560724));
#185809=CARTESIAN_POINT('Ctrl Pts',(10.7465986086019,12.2,-1.82460021558692));
#185810=CARTESIAN_POINT('Ctrl Pts',(10.7432225671946,12.2,-1.82279424532054));
#185811=CARTESIAN_POINT('Ctrl Pts',(10.7398566537679,12.2,-1.82100090030663));
#185812=CARTESIAN_POINT('Ctrl Pts',(10.7365010030143,12.2,-1.81922015525709));
#185813=CARTESIAN_POINT('Ctrl Pts',(10.7331453527178,12.2,-1.81743941045017));
#185814=CARTESIAN_POINT('Ctrl Pts',(10.7297999663791,12.2,-1.81567126613366));
#185815=CARTESIAN_POINT('Ctrl Pts',(10.7264649807619,12.2,-1.81391569605368));
#185816=CARTESIAN_POINT('Ctrl Pts',(10.7231299946902,12.2,-1.8121601257345));
#185817=CARTESIAN_POINT('Ctrl Pts',(10.71980540945,12.2,-1.81041713059982));
#185818=CARTESIAN_POINT('Ctrl Pts',(10.7164913639916,12.2,-1.80868668428329));
#185819=CARTESIAN_POINT('Ctrl Pts',(10.7131773185332,12.2,-1.80695623796676));
#185820=CARTESIAN_POINT('Ctrl Pts',(10.7098738114344,12.2,-1.80523834092947));
#185821=CARTESIAN_POINT('Ctrl Pts',(10.7065809834782,12.2,-1.80353296650448));
#185822=CARTESIAN_POINT('Ctrl Pts',(10.7032881559707,12.2,-1.80182759231183));
#185823=CARTESIAN_POINT('Ctrl Pts',(10.7000060071857,12.2,-1.80013473975198));
#185824=CARTESIAN_POINT('Ctrl Pts',(10.6967346794938,12.2,-1.79845438349278));
#185825=CARTESIAN_POINT('Ctrl Pts',(10.6934633513562,12.2,-1.79677402700463));
#185826=CARTESIAN_POINT('Ctrl Pts',(10.6902028422835,12.2,-1.79510616451548));
#185827=CARTESIAN_POINT('Ctrl Pts',(10.6869532962186,12.2,-1.79345077070432));
#185828=CARTESIAN_POINT('Ctrl Pts',(10.6828913638589,12.2,-1.79138152855314));
#185829=CARTESIAN_POINT('Ctrl Pts',(10.678846559605,12.2,-1.78933176627727));
#185830=CARTESIAN_POINT('Ctrl Pts',(10.6748191656481,12.2,-1.78730142766774));
#185831=CARTESIAN_POINT('Ctrl Pts',(10.671597250746,12.2,-1.7856771569129));
#185832=CARTESIAN_POINT('Ctrl Pts',(10.6683864779468,12.2,-1.78406531861094));
#185833=CARTESIAN_POINT('Ctrl Pts',(10.6651869930271,12.2,-1.78246588173439));
#185834=CARTESIAN_POINT('Ctrl Pts',(10.6619875076715,12.2,-1.78086644463992));
#185835=CARTESIAN_POINT('Ctrl Pts',(10.6587993100969,12.2,-1.77927940958262));
#185836=CARTESIAN_POINT('Ctrl Pts',(10.6556225474805,12.2,-1.77770474594252));
#185837=CARTESIAN_POINT('Ctrl Pts',(10.6524457852969,12.2,-1.77613008251696));
#185838=CARTESIAN_POINT('Ctrl Pts',(10.649280457323,12.2,-1.77456779159811));
#185839=CARTESIAN_POINT('Ctrl Pts',(10.6461267130245,12.2,-1.77301784133512));
#185840=CARTESIAN_POINT('Ctrl Pts',(10.6429729682963,12.2,-1.77146789086096));
#185841=CARTESIAN_POINT('Ctrl Pts',(10.6398308055328,12.2,-1.76993028070364));
#185842=CARTESIAN_POINT('Ctrl Pts',(10.6367003760957,12.2,-1.76840497954537));
#185843=CARTESIAN_POINT('Ctrl Pts',(10.6335699470851,12.2,-1.76687967859492));
#185844=CARTESIAN_POINT('Ctrl Pts',(10.6304512504675,12.2,-1.76536668609533));
#185845=CARTESIAN_POINT('Ctrl Pts',(10.6273444377207,12.2,-1.7638659711061));
#185846=CARTESIAN_POINT('Ctrl Pts',(10.6242376245506,12.2,-1.7623652559124));
#185847=CARTESIAN_POINT('Ctrl Pts',(10.6211426971291,12.2,-1.76087681637573));
#185848=CARTESIAN_POINT('Ctrl Pts',(10.6180598052397,12.2,-1.7594006206294));
#185849=CARTESIAN_POINT('Ctrl Pts',(10.6149769137702,12.2,-1.75792442508422));
#185850=CARTESIAN_POINT('Ctrl Pts',(10.6119060592254,12.2,-1.75646047158226));
#185851=CARTESIAN_POINT('Ctrl Pts',(10.6088473962105,12.2,-1.75500872796069));
#185852=CARTESIAN_POINT('Ctrl Pts',(10.6057887327788,12.2,-1.75355698414132));
#185853=CARTESIAN_POINT('Ctrl Pts',(10.6027422594804,12.2,-1.75211744984096));
#185854=CARTESIAN_POINT('Ctrl Pts',(10.5997081342603,12.2,-1.75069008937506));
#185855=CARTESIAN_POINT('Ctrl Pts',(10.5966740094536,12.2,-1.74926272910364));
#185856=CARTESIAN_POINT('Ctrl Pts',(10.5936522330527,12.2,-1.74784754366035));
#185857=CARTESIAN_POINT('Ctrl Pts',(10.5906429597419,12.2,-1.74644449599604));
#185858=CARTESIAN_POINT('Ctrl Pts',(10.5868813677959,12.2,-1.74469068627227));
#185859=CARTESIAN_POINT('Ctrl Pts',(10.5831393145361,12.2,-1.74295584315294));
#185860=CARTESIAN_POINT('Ctrl Pts',(10.5794171114321,12.2,-1.74123989348256));
#185861=CARTESIAN_POINT('Ctrl Pts',(10.575694908328,12.2,-1.73952394381218));
#185862=CARTESIAN_POINT('Ctrl Pts',(10.5719925556196,12.2,-1.73782688946638));
#185863=CARTESIAN_POINT('Ctrl Pts',(10.5683103670075,12.2,-1.73614865557651));
#185864=CARTESIAN_POINT('Ctrl Pts',(10.5646281783953,12.2,-1.73447042168664));
#185865=CARTESIAN_POINT('Ctrl Pts',(10.5609661564948,12.2,-1.73281100937503));
#185866=CARTESIAN_POINT('Ctrl Pts',(10.5573246194798,12.2,-1.73117034062405));
#185867=CARTESIAN_POINT('Ctrl Pts',(10.5536830824649,12.2,-1.72952967187307));
#185868=CARTESIAN_POINT('Ctrl Pts',(10.5500620305754,12.2,-1.72790774972813));
#185869=CARTESIAN_POINT('Ctrl Pts',(10.5464617877271,12.2,-1.72630449187994));
#185870=CARTESIAN_POINT('Ctrl Pts',(10.5428615448789,12.2,-1.72470123403175));
#185871=CARTESIAN_POINT('Ctrl Pts',(10.5392821105347,12.2,-1.72311664391354));
#185872=CARTESIAN_POINT('Ctrl Pts',(10.5357238144768,12.2,-1.72155064001749));
#185873=CARTESIAN_POINT('Ctrl Pts',(10.532165518419,12.2,-1.71998463612144));
#185874=CARTESIAN_POINT('Ctrl Pts',(10.5286283611332,12.2,-1.71843721744996));
#185875=CARTESIAN_POINT('Ctrl Pts',(10.5251126742582,12.2,-1.7169083020333));
#185876=CARTESIAN_POINT('Ctrl Pts',(10.5215969873832,12.2,-1.71537938661663));
#185877=CARTESIAN_POINT('Ctrl Pts',(10.5181027712526,12.2,-1.71386897543366));
#185878=CARTESIAN_POINT('Ctrl Pts',(10.5146303650563,12.2,-1.71237698223249));
#185879=CARTESIAN_POINT('Ctrl Pts',(10.5111579588601,12.2,-1.71088498903132));
#185880=CARTESIAN_POINT('Ctrl Pts',(10.5077073598247,12.2,-1.70941141196506));
#185881=CARTESIAN_POINT('Ctrl Pts',(10.5042789137841,12.2,-1.70795616710491));
#185882=CARTESIAN_POINT('Ctrl Pts',(10.5008504677436,12.2,-1.70650092224475));
#185883=CARTESIAN_POINT('Ctrl Pts',(10.4974441731775,12.2,-1.70506400643413));
#185884=CARTESIAN_POINT('Ctrl Pts',(10.4940603773454,12.2,-1.7036453324073));
#185885=CARTESIAN_POINT('Ctrl Pts',(10.4906765815132,12.2,-1.70222665838047));
#185886=CARTESIAN_POINT('Ctrl Pts',(10.4873152869609,12.2,-1.70082622411292));
#185887=CARTESIAN_POINT('Ctrl Pts',(10.4839768426291,12.2,-1.69944393682291));
#185888=CARTESIAN_POINT('Ctrl Pts',(10.4806383982972,12.2,-1.69806164953289));
#185889=CARTESIAN_POINT('Ctrl Pts',(10.4773228069951,12.2,-1.69669751057243));
#185890=CARTESIAN_POINT('Ctrl Pts',(10.4740304260943,12.2,-1.69535142328224));
#185891=CARTESIAN_POINT('Ctrl Pts',(10.4700795691567,12.2,-1.69373611859271));
#185892=CARTESIAN_POINT('Ctrl Pts',(10.4661621343579,12.2,-1.69214680864117));
#185893=CARTESIAN_POINT('Ctrl Pts',(10.4622787523148,12.2,-1.69058332477426));
#185894=CARTESIAN_POINT('Ctrl Pts',(10.4590426004946,12.2,-1.68928042150451));
#185895=CARTESIAN_POINT('Ctrl Pts',(10.4558300937513,12.2,-1.68799545171071));
#185896=CARTESIAN_POINT('Ctrl Pts',(10.4526416070165,12.2,-1.68672831435054));
#185897=CARTESIAN_POINT('Ctrl Pts',(10.4494531202817,12.2,-1.68546117699037));
#185898=CARTESIAN_POINT('Ctrl Pts',(10.4462886496434,12.2,-1.68421187264083));
#185899=CARTESIAN_POINT('Ctrl Pts',(10.443148572978,12.2,-1.68298029687786));
#185900=CARTESIAN_POINT('Ctrl Pts',(10.4400084963126,12.2,-1.6817487211149));
#185901=CARTESIAN_POINT('Ctrl Pts',(10.4368928141828,12.2,-1.68053487177526));
#185902=CARTESIAN_POINT('Ctrl Pts',(10.4338019065995,12.2,-1.67933864511951));
#185903=CARTESIAN_POINT('Ctrl Pts',(10.4294746362525,12.2,-1.67766392790576));
#185904=CARTESIAN_POINT('Ctrl Pts',(10.4251959272567,12.2,-1.67602374681866));
#185905=CARTESIAN_POINT('Ctrl Pts',(10.4209668438783,12.2,-1.67441779991668));
#185906=CARTESIAN_POINT('Ctrl Pts',(10.417341914845,12.2,-1.67304127383994));
#185907=CARTESIAN_POINT('Ctrl Pts',(10.4137534485502,12.2,-1.67168989669216));
#185908=CARTESIAN_POINT('Ctrl Pts',(10.4102021304314,12.2,-1.67036347338839));
#185909=CARTESIAN_POINT('Ctrl Pts',(10.4066508126352,12.2,-1.66903705020509));
#185910=CARTESIAN_POINT('Ctrl Pts',(10.4031366447736,12.2,-1.66773557787858));
#185911=CARTESIAN_POINT('Ctrl Pts',(10.3996603252332,12.2,-1.6664588510083));
#185912=CARTESIAN_POINT('Ctrl Pts',(10.3961840056929,12.2,-1.66518212413803));
#185913=CARTESIAN_POINT('Ctrl Pts',(10.3927455368108,12.2,-1.66393014446191));
#185914=CARTESIAN_POINT('Ctrl Pts',(10.3893456330955,12.2,-1.66270269836044));
#185915=CARTESIAN_POINT('Ctrl Pts',(10.3859457290715,12.2,-1.66147525214747));
#185916=CARTESIAN_POINT('Ctrl Pts',(10.3825843893245,12.2,-1.66027233816742));
#185917=CARTESIAN_POINT('Ctrl Pts',(10.3792623465628,12.2,-1.65909373810484));
#185918=CARTESIAN_POINT('Ctrl Pts',(10.3759403041029,12.2,-1.65791513814932));
#185919=CARTESIAN_POINT('Ctrl Pts',(10.3726575564452,12.2,-1.65676085241348));
#185920=CARTESIAN_POINT('Ctrl Pts',(10.3694148500484,12.2,-1.65563065228279));
#185921=CARTESIAN_POINT('Ctrl Pts',(10.3661721436516,12.2,-1.65450045215211));
#185922=CARTESIAN_POINT('Ctrl Pts',(10.3629694782426,12.2,-1.65339433672077));
#185923=CARTESIAN_POINT('Ctrl Pts',(10.3598076168557,12.2,-1.65231207359239));
#185924=CARTESIAN_POINT('Ctrl Pts',(10.3566457551816,12.2,-1.6512298103657));
#185925=CARTESIAN_POINT('Ctrl Pts',(10.3535246958959,12.2,-1.65017139676697));
#185926=CARTESIAN_POINT('Ctrl Pts',(10.3504452183975,12.2,-1.64913659062885));
#185927=CARTESIAN_POINT('Ctrl Pts',(10.3473657411789,12.2,-1.64810178458472));
#185928=CARTESIAN_POINT('Ctrl Pts',(10.3443278454199,12.2,-1.6470905856764));
#185929=CARTESIAN_POINT('Ctrl Pts',(10.3413323281818,12.2,-1.64610274245786));
#185930=CARTESIAN_POINT('Ctrl Pts',(10.3383368109438,12.2,-1.64511489923932));
#185931=CARTESIAN_POINT('Ctrl Pts',(10.3353836696881,12.2,-1.64415040969318));
#185932=CARTESIAN_POINT('Ctrl Pts',(10.3324737224586,12.2,-1.64320901730971));
#185933=CARTESIAN_POINT('Ctrl Pts',(10.3295637749649,12.2,-1.64226762484074));
#185934=CARTESIAN_POINT('Ctrl Pts',(10.3266970175847,12.2,-1.64134932435795));
#185935=CARTESIAN_POINT('Ctrl Pts',(10.3238742871839,12.2,-1.64045385089404));
#185936=CARTESIAN_POINT('Ctrl Pts',(10.3210515570394,12.2,-1.63955837751147));
#185937=CARTESIAN_POINT('Ctrl Pts',(10.3182728521331,12.2,-1.63868572728853));
#185938=CARTESIAN_POINT('Ctrl Pts',(10.3155390244011,12.2,-1.63783562398707));
#185939=CARTESIAN_POINT('Ctrl Pts',(10.312805196669,12.2,-1.63698552068561));
#185940=CARTESIAN_POINT('Ctrl Pts',(10.3101162476,12.2,-1.63615796238233));
#185941=CARTESIAN_POINT('Ctrl Pts',(10.3074730508608,12.2,-1.63535266107729));
#185942=CARTESIAN_POINT('Ctrl Pts',(10.3048298541215,12.2,-1.63454735977225));
#185943=CARTESIAN_POINT('Ctrl Pts',(10.3022324099134,12.2,-1.63376431454012));
#185944=CARTESIAN_POINT('Ctrl Pts',(10.2996816122529,12.2,-1.63300322706627));
#185945=CARTESIAN_POINT('Ctrl Pts',(10.2971308143607,12.2,-1.63224213952329));
#185946=CARTESIAN_POINT('Ctrl Pts',(10.2946266653563,12.2,-1.63150300843246));
#185947=CARTESIAN_POINT('Ctrl Pts',(10.2921700806412,12.2,-1.63078552572763));
#185948=CARTESIAN_POINT('Ctrl Pts',(10.2897134961492,12.2,-1.63006804308798));
#185949=CARTESIAN_POINT('Ctrl Pts',(10.2873044769177,12.2,-1.62937220681223));
#185950=CARTESIAN_POINT('Ctrl Pts',(10.2849439662426,12.2,-1.62869769550029));
#185951=CARTESIAN_POINT('Ctrl Pts',(10.2825834555675,12.2,-1.62802318418834));
#185952=CARTESIAN_POINT('Ctrl Pts',(10.2802714503093,12.2,-1.62737000058902));
#185953=CARTESIAN_POINT('Ctrl Pts',(10.2780089199715,12.2,-1.62673780902723));
#185954=CARTESIAN_POINT('Ctrl Pts',(10.2757463894281,12.2,-1.62610561740801));
#185955=CARTESIAN_POINT('Ctrl Pts',(10.2735333314221,12.2,-1.62549441732006));
#185956=CARTESIAN_POINT('Ctrl Pts',(10.2713707417824,12.2,-1.62490386742623));
#185957=CARTESIAN_POINT('Ctrl Pts',(10.2692081523392,12.2,-1.62431331758605));
#185958=CARTESIAN_POINT('Ctrl Pts',(10.2670960277416,12.2,-1.62374341398834));
#185959=CARTESIAN_POINT('Ctrl Pts',(10.2650353904832,12.2,-1.62319380125831));
#185960=CARTESIAN_POINT('Ctrl Pts',(10.2629747532247,12.2,-1.62264418852828));
#185961=CARTESIAN_POINT('Ctrl Pts',(10.2609656015273,12.2,-1.62211486489073));
#185962=CARTESIAN_POINT('Ctrl Pts',(10.2590089854143,12.2,-1.62160546104931));
#185963=CARTESIAN_POINT('Ctrl Pts',(10.2570523691235,12.2,-1.62109605716161));
#185964=CARTESIAN_POINT('Ctrl Pts',(10.255148287587,12.2,-1.62060657271471));
#185965=CARTESIAN_POINT('Ctrl Pts',(10.2532978195732,12.2,-1.62013662094043));
#185966=CARTESIAN_POINT('Ctrl Pts',(10.2514562326224,12.2,-1.61966892463414));
#185967=CARTESIAN_POINT('Ctrl Pts',(10.2496677474645,12.2,-1.61922057460985));
#185968=CARTESIAN_POINT('Ctrl Pts',(10.2479334559999,12.2,-1.61879118000002));
#185969=CARTESIAN_POINT('Ctrl Pts',(10.2479334559999,15.2,-1.61879118000002));
#185970=CARTESIAN_POINT('Ctrl Pts',(10.2496677474645,15.2,-1.61922057460985));
#185971=CARTESIAN_POINT('Ctrl Pts',(10.2514562326224,15.2,-1.61966892463414));
#185972=CARTESIAN_POINT('Ctrl Pts',(10.2532978195732,15.2,-1.62013662094043));
#185973=CARTESIAN_POINT('Ctrl Pts',(10.2551482875871,15.2,-1.62060657271471));
#185974=CARTESIAN_POINT('Ctrl Pts',(10.2570523691235,15.2,-1.62109605716161));
#185975=CARTESIAN_POINT('Ctrl Pts',(10.2590089854143,15.2,-1.62160546104931));
#185976=CARTESIAN_POINT('Ctrl Pts',(10.2609656015273,15.2,-1.62211486489073));
#185977=CARTESIAN_POINT('Ctrl Pts',(10.2629747532247,15.2,-1.62264418852828));
#185978=CARTESIAN_POINT('Ctrl Pts',(10.2650353904832,15.2,-1.62319380125831));
#185979=CARTESIAN_POINT('Ctrl Pts',(10.2670960277416,15.2,-1.62374341398834));
#185980=CARTESIAN_POINT('Ctrl Pts',(10.2692081523392,15.2,-1.62431331758605));
#185981=CARTESIAN_POINT('Ctrl Pts',(10.2713707417824,15.2,-1.62490386742623));
#185982=CARTESIAN_POINT('Ctrl Pts',(10.2735333314221,15.2,-1.62549441732006));
#185983=CARTESIAN_POINT('Ctrl Pts',(10.2757463894281,15.2,-1.62610561740801));
#185984=CARTESIAN_POINT('Ctrl Pts',(10.2780089199715,15.2,-1.62673780902722));
#185985=CARTESIAN_POINT('Ctrl Pts',(10.2802714503093,15.2,-1.62737000058902));
#185986=CARTESIAN_POINT('Ctrl Pts',(10.2825834555675,15.2,-1.62802318418834));
#185987=CARTESIAN_POINT('Ctrl Pts',(10.2849439662426,15.2,-1.62869769550028));
#185988=CARTESIAN_POINT('Ctrl Pts',(10.2873044769177,15.2,-1.62937220681223));
#185989=CARTESIAN_POINT('Ctrl Pts',(10.2897134961492,15.2,-1.63006804308797));
#185990=CARTESIAN_POINT('Ctrl Pts',(10.2921700806412,15.2,-1.63078552572763));
#185991=CARTESIAN_POINT('Ctrl Pts',(10.2946266653563,15.2,-1.63150300843246));
#185992=CARTESIAN_POINT('Ctrl Pts',(10.2971308143607,15.2,-1.6322421395233));
#185993=CARTESIAN_POINT('Ctrl Pts',(10.2996816122529,15.2,-1.63300322706627));
#185994=CARTESIAN_POINT('Ctrl Pts',(10.3022324099134,15.2,-1.63376431454011));
#185995=CARTESIAN_POINT('Ctrl Pts',(10.3048298541215,15.2,-1.63454735977225));
#185996=CARTESIAN_POINT('Ctrl Pts',(10.3074730508608,15.2,-1.63535266107729));
#185997=CARTESIAN_POINT('Ctrl Pts',(10.3101162476,15.2,-1.63615796238233));
#185998=CARTESIAN_POINT('Ctrl Pts',(10.312805196669,15.2,-1.63698552068561));
#185999=CARTESIAN_POINT('Ctrl Pts',(10.3155390244011,15.2,-1.63783562398707));
#186000=CARTESIAN_POINT('Ctrl Pts',(10.3182728521331,15.2,-1.63868572728853));
#186001=CARTESIAN_POINT('Ctrl Pts',(10.3210515570394,15.2,-1.63955837751146));
#186002=CARTESIAN_POINT('Ctrl Pts',(10.3238742871839,15.2,-1.64045385089404));
#186003=CARTESIAN_POINT('Ctrl Pts',(10.3266970175847,15.2,-1.64134932435796));
#186004=CARTESIAN_POINT('Ctrl Pts',(10.3295637749648,15.2,-1.64226762484073));
#186005=CARTESIAN_POINT('Ctrl Pts',(10.3324737224586,15.2,-1.64320901730971));
#186006=CARTESIAN_POINT('Ctrl Pts',(10.3353836696881,15.2,-1.64415040969318));
#186007=CARTESIAN_POINT('Ctrl Pts',(10.3383368109438,15.2,-1.64511489923932));
#186008=CARTESIAN_POINT('Ctrl Pts',(10.3413323281818,15.2,-1.64610274245786));
#186009=CARTESIAN_POINT('Ctrl Pts',(10.3443278454199,15.2,-1.64709058567641));
#186010=CARTESIAN_POINT('Ctrl Pts',(10.3473657411789,15.2,-1.64810178458472));
#186011=CARTESIAN_POINT('Ctrl Pts',(10.3504452183975,15.2,-1.64913659062885));
#186012=CARTESIAN_POINT('Ctrl Pts',(10.3535246958959,15.2,-1.65017139676697));
#186013=CARTESIAN_POINT('Ctrl Pts',(10.3566457551816,15.2,-1.6512298103657));
#186014=CARTESIAN_POINT('Ctrl Pts',(10.3598076168557,15.2,-1.65231207359239));
#186015=CARTESIAN_POINT('Ctrl Pts',(10.3629694782426,15.2,-1.65339433672077));
#186016=CARTESIAN_POINT('Ctrl Pts',(10.3661721436516,15.2,-1.65450045215211));
#186017=CARTESIAN_POINT('Ctrl Pts',(10.3694148500484,15.2,-1.65563065228279));
#186018=CARTESIAN_POINT('Ctrl Pts',(10.3726575564452,15.2,-1.65676085241347));
#186019=CARTESIAN_POINT('Ctrl Pts',(10.3759403041029,15.2,-1.65791513814932));
#186020=CARTESIAN_POINT('Ctrl Pts',(10.3792623465628,15.2,-1.65909373810484));
#186021=CARTESIAN_POINT('Ctrl Pts',(10.3825843893245,15.2,-1.66027233816742));
#186022=CARTESIAN_POINT('Ctrl Pts',(10.3859457290715,15.2,-1.66147525214747));
#186023=CARTESIAN_POINT('Ctrl Pts',(10.3893456330955,15.2,-1.66270269836044));
#186024=CARTESIAN_POINT('Ctrl Pts',(10.3927455368108,15.2,-1.66393014446192));
#186025=CARTESIAN_POINT('Ctrl Pts',(10.3961840056929,15.2,-1.66518212413802));
#186026=CARTESIAN_POINT('Ctrl Pts',(10.3996603252332,15.2,-1.6664588510083));
#186027=CARTESIAN_POINT('Ctrl Pts',(10.4031366447736,15.2,-1.66773557787858));
#186028=CARTESIAN_POINT('Ctrl Pts',(10.4066508126352,15.2,-1.66903705020509));
#186029=CARTESIAN_POINT('Ctrl Pts',(10.4102021304314,15.2,-1.67036347338839));
#186030=CARTESIAN_POINT('Ctrl Pts',(10.4137534485502,15.2,-1.67168989669217));
#186031=CARTESIAN_POINT('Ctrl Pts',(10.417341914845,15.2,-1.67304127383995));
#186032=CARTESIAN_POINT('Ctrl Pts',(10.4209668438783,15.2,-1.67441779991668));
#186033=CARTESIAN_POINT('Ctrl Pts',(10.4258000822603,15.2,-1.67625316789396));
#186034=CARTESIAN_POINT('Ctrl Pts',(10.4306981370547,15.2,-1.67813324902336));
#186035=CARTESIAN_POINT('Ctrl Pts',(10.4356594221266,15.2,-1.68005849687305));
#186036=CARTESIAN_POINT('Ctrl Pts',(10.4387602253388,15.2,-1.6812617767955));
#186037=CARTESIAN_POINT('Ctrl Pts',(10.4418857244099,15.2,-1.6824826994772));
#186038=CARTESIAN_POINT('Ctrl Pts',(10.4450355442036,15.2,-1.68372137093699));
#186039=CARTESIAN_POINT('Ctrl Pts',(10.4481853639972,15.2,-1.68496004239679));
#186040=CARTESIAN_POINT('Ctrl Pts',(10.4513594997051,15.2,-1.68621646330408));
#186041=CARTESIAN_POINT('Ctrl Pts',(10.4545575789432,15.2,-1.68749073795832));
#186042=CARTESIAN_POINT('Ctrl Pts',(10.4577556578327,15.2,-1.68876501247365));
#186043=CARTESIAN_POINT('Ctrl Pts',(10.4609776818311,15.2,-1.69005713868399));
#186044=CARTESIAN_POINT('Ctrl Pts',(10.464223277517,15.2,-1.69136721930362));
#186045=CARTESIAN_POINT('Ctrl Pts',(10.4674688735568,15.2,-1.69267730006604));
#186046=CARTESIAN_POINT('Ctrl Pts',(10.4707380451934,15.2,-1.69400533599205));
#186047=CARTESIAN_POINT('Ctrl Pts',(10.4740304260942,15.2,-1.69535142328224));
#186048=CARTESIAN_POINT('Ctrl Pts',(10.4773228069951,15.2,-1.69669751057243));
#186049=CARTESIAN_POINT('Ctrl Pts',(10.4806383982972,15.2,-1.69806164953288));
#186050=CARTESIAN_POINT('Ctrl Pts',(10.4839768426291,15.2,-1.6994439368229));
#186051=CARTESIAN_POINT('Ctrl Pts',(10.487315286961,15.2,-1.70082622411293));
#186052=CARTESIAN_POINT('Ctrl Pts',(10.4906765815132,15.2,-1.70222665838047));
#186053=CARTESIAN_POINT('Ctrl Pts',(10.4940603773454,15.2,-1.7036453324073));
#186054=CARTESIAN_POINT('Ctrl Pts',(10.4974441731776,15.2,-1.70506400643413));
#186055=CARTESIAN_POINT('Ctrl Pts',(10.5008504677436,15.2,-1.70650092224475));
#186056=CARTESIAN_POINT('Ctrl Pts',(10.5042789137841,15.2,-1.7079561671049));
#186057=CARTESIAN_POINT('Ctrl Pts',(10.5077073598246,15.2,-1.70941141196506));
#186058=CARTESIAN_POINT('Ctrl Pts',(10.5111579588601,15.2,-1.71088498903132));
#186059=CARTESIAN_POINT('Ctrl Pts',(10.5146303650563,15.2,-1.71237698223249));
#186060=CARTESIAN_POINT('Ctrl Pts',(10.5187972523405,15.2,-1.71416737400885));
#186061=CARTESIAN_POINT('Ctrl Pts',(10.5229955456113,15.2,-1.71598428835948));
#186062=CARTESIAN_POINT('Ctrl Pts',(10.5272246597889,15.2,-1.71782787204069));
#186063=CARTESIAN_POINT('Ctrl Pts',(10.5307489217316,15.2,-1.71936419183085));
#186064=CARTESIAN_POINT('Ctrl Pts',(10.5342945876647,15.2,-1.7209190315234));
#186065=CARTESIAN_POINT('Ctrl Pts',(10.5378613256193,15.2,-1.72249247305905));
#186066=CARTESIAN_POINT('Ctrl Pts',(10.5414280635738,15.2,-1.72406591459469));
#186067=CARTESIAN_POINT('Ctrl Pts',(10.545015874304,15.2,-1.72565796019572));
#186068=CARTESIAN_POINT('Ctrl Pts',(10.548624427289,15.2,-1.72726868665307));
#186069=CARTESIAN_POINT('Ctrl Pts',(10.5536764015467,15.2,-1.72952370372847));
#186070=CARTESIAN_POINT('Ctrl Pts',(10.5587690353144,15.2,-1.73181533826371));
#186071=CARTESIAN_POINT('Ctrl Pts',(10.5639014407416,15.2,-1.73414380371663));
#186072=CARTESIAN_POINT('Ctrl Pts',(10.568300645165,15.2,-1.73613963114411));
#186073=CARTESIAN_POINT('Ctrl Pts',(10.5727290727597,15.2,-1.73816251542536));
#186074=CARTESIAN_POINT('Ctrl Pts',(10.5771861733188,15.2,-1.74021258978505));
#186075=CARTESIAN_POINT('Ctrl Pts',(10.5809004239196,15.2,-1.74192098514686));
#186076=CARTESIAN_POINT('Ctrl Pts',(10.5846345871611,15.2,-1.74364825788131));
#186077=CARTESIAN_POINT('Ctrl Pts',(10.5883883509795,15.2,-1.74539448489421));
#186078=CARTESIAN_POINT('Ctrl Pts',(10.5921421147979,15.2,-1.74714071190711));
#186079=CARTESIAN_POINT('Ctrl Pts',(10.5959154779418,15.2,-1.74890588888993));
#186080=CARTESIAN_POINT('Ctrl Pts',(10.5997081342603,15.2,-1.75069008937506));
#186081=CARTESIAN_POINT('Ctrl Pts',(10.6027422594805,15.2,-1.75211744984096));
#186082=CARTESIAN_POINT('Ctrl Pts',(10.6057887327788,15.2,-1.75355698414132));
#186083=CARTESIAN_POINT('Ctrl Pts',(10.6088473962105,15.2,-1.75500872796069));
#186084=CARTESIAN_POINT('Ctrl Pts',(10.6119060592254,15.2,-1.75646047158226));
#186085=CARTESIAN_POINT('Ctrl Pts',(10.6149769137702,15.2,-1.75792442508421));
#186086=CARTESIAN_POINT('Ctrl Pts',(10.6180598052397,15.2,-1.7594006206294));
#186087=CARTESIAN_POINT('Ctrl Pts',(10.6211426971291,15.2,-1.76087681637573));
#186088=CARTESIAN_POINT('Ctrl Pts',(10.6242376245506,15.2,-1.7623652559124));
#186089=CARTESIAN_POINT('Ctrl Pts',(10.6273444377207,15.2,-1.7638659711061));
#186090=CARTESIAN_POINT('Ctrl Pts',(10.6304512504675,15.2,-1.76536668609533));
#186091=CARTESIAN_POINT('Ctrl Pts',(10.6335699470852,15.2,-1.76687967859493));
#186092=CARTESIAN_POINT('Ctrl Pts',(10.6367003760957,15.2,-1.76840497954537));
#186093=CARTESIAN_POINT('Ctrl Pts',(10.6398308055328,15.2,-1.76993028070363));
#186094=CARTESIAN_POINT('Ctrl Pts',(10.6429729682963,15.2,-1.77146789086095));
#186095=CARTESIAN_POINT('Ctrl Pts',(10.6461267130245,15.2,-1.77301784133512));
#186096=CARTESIAN_POINT('Ctrl Pts',(10.649280457323,15.2,-1.77456779159811));
#186097=CARTESIAN_POINT('Ctrl Pts',(10.6524457852969,15.2,-1.77613008251696));
#186098=CARTESIAN_POINT('Ctrl Pts',(10.6556225474805,15.2,-1.77770474594252));
#186099=CARTESIAN_POINT('Ctrl Pts',(10.6587993100969,15.2,-1.77927940958262));
#186100=CARTESIAN_POINT('Ctrl Pts',(10.6619875076715,15.2,-1.78086644463991));
#186101=CARTESIAN_POINT('Ctrl Pts',(10.6651869930271,15.2,-1.78246588173439));
#186102=CARTESIAN_POINT('Ctrl Pts',(10.6683864779468,15.2,-1.78406531861095));
#186103=CARTESIAN_POINT('Ctrl Pts',(10.671597250746,15.2,-1.7856771569129));
#186104=CARTESIAN_POINT('Ctrl Pts',(10.6748191656481,15.2,-1.78730142766774));
#186105=CARTESIAN_POINT('Ctrl Pts',(10.678846559605,15.2,-1.78933176627727));
#186106=CARTESIAN_POINT('Ctrl Pts',(10.6828913638589,15.2,-1.79138152855313));
#186107=CARTESIAN_POINT('Ctrl Pts',(10.6869532962186,15.2,-1.79345077070432));
#186108=CARTESIAN_POINT('Ctrl Pts',(10.6902028422835,15.2,-1.79510616451548));
#186109=CARTESIAN_POINT('Ctrl Pts',(10.6934633513562,15.2,-1.79677402700464));
#186110=CARTESIAN_POINT('Ctrl Pts',(10.6967346794938,15.2,-1.79845438349278));
#186111=CARTESIAN_POINT('Ctrl Pts',(10.7000060071857,15.2,-1.80013473975198));
#186112=CARTESIAN_POINT('Ctrl Pts',(10.7032881559707,15.2,-1.80182759231183));
#186113=CARTESIAN_POINT('Ctrl Pts',(10.7065809834782,15.2,-1.80353296650448));
#186114=CARTESIAN_POINT('Ctrl Pts',(10.7106970181991,15.2,-1.80566468441955));
#186115=CARTESIAN_POINT('Ctrl Pts',(10.7148297387252,15.2,-1.80781596909539));
#186116=CARTESIAN_POINT('Ctrl Pts',(10.7189788712239,15.2,-1.80998687194102));
#186117=CARTESIAN_POINT('Ctrl Pts',(10.7222981774037,15.2,-1.81172359431217));
#186118=CARTESIAN_POINT('Ctrl Pts',(10.7256279900688,15.2,-1.81347287244432));
#186119=CARTESIAN_POINT('Ctrl Pts',(10.7289681675438,15.2,-1.81523473149283));
#186120=CARTESIAN_POINT('Ctrl Pts',(10.7323083445638,15.2,-1.81699659030129));
#186121=CARTESIAN_POINT('Ctrl Pts',(10.7356588894401,15.2,-1.81877102999683));
#186122=CARTESIAN_POINT('Ctrl Pts',(10.7390196624421,15.2,-1.82055807668279));
#186123=CARTESIAN_POINT('Ctrl Pts',(10.743220629038,15.2,-1.82279188522286));
#186124=CARTESIAN_POINT('Ctrl Pts',(10.747437578192,15.2,-1.82504539094313));
#186125=CARTESIAN_POINT('Ctrl Pts',(10.7516702479129,15.2,-1.8273186412193));
#186126=CARTESIAN_POINT('Ctrl Pts',(10.7559029176339,15.2,-1.82959189149547));
#186127=CARTESIAN_POINT('Ctrl Pts',(10.7601513043042,15.2,-1.83188488622295));
#186128=CARTESIAN_POINT('Ctrl Pts',(10.7644151494467,15.2,-1.83419767244822));
#186129=CARTESIAN_POINT('Ctrl Pts',(10.7678262257466,15.2,-1.83604790152928));
#186130=CARTESIAN_POINT('Ctrl Pts',(10.7712471950929,15.2,-1.83791079673092));
#186131=CARTESIAN_POINT('Ctrl Pts',(10.7746779232805,15.2,-1.83978638044508));
#186132=CARTESIAN_POINT('Ctrl Pts',(10.7781086510006,15.2,-1.84166196390369));
#186133=CARTESIAN_POINT('Ctrl Pts',(10.7815491388494,15.2,-1.8435502374792));
#186134=CARTESIAN_POINT('Ctrl Pts',(10.7849992551775,15.2,-1.84545122098916));
#186135=CARTESIAN_POINT('Ctrl Pts',(10.7884493719756,15.2,-1.84735220475813));
#186136=CARTESIAN_POINT('Ctrl Pts',(10.7919091171335,15.2,-1.84926589974306));
#186137=CARTESIAN_POINT('Ctrl Pts',(10.7953783600606,15.2,-1.85119232796794));
#186138=CARTESIAN_POINT('Ctrl Pts',(10.798847602515,15.2,-1.85311875593035));
#186139=CARTESIAN_POINT('Ctrl Pts',(10.8023263425435,15.2,-1.85505791591948));
#186140=CARTESIAN_POINT('Ctrl Pts',(10.8058144521463,15.2,-1.85700982998083));
#186141=CARTESIAN_POINT('Ctrl Pts',(10.8093025622243,15.2,-1.85896174430813));
#186142=CARTESIAN_POINT('Ctrl Pts',(10.8128000406254,15.2,-1.8609264129533));
#186143=CARTESIAN_POINT('Ctrl Pts',(10.8163067594832,15.2,-1.86290385528329));
#186144=CARTESIAN_POINT('Ctrl Pts',(10.8215668372922,15.2,-1.86587001850886));
#186145=CARTESIAN_POINT('Ctrl Pts',(10.8268477058994,15.2,-1.86886492240721));
#186146=CARTESIAN_POINT('Ctrl Pts',(10.8321489387054,15.2,-1.87188863737872));
#186147=CARTESIAN_POINT('Ctrl Pts',(10.8356830942304,15.2,-1.87390444754283));
#186148=CARTESIAN_POINT('Ctrl Pts',(10.8392262989926,15.2,-1.87593306149467));
#186149=CARTESIAN_POINT('Ctrl Pts',(10.8427784292023,15.2,-1.87797449722636));
#186150=CARTESIAN_POINT('Ctrl Pts',(10.8463305589281,15.2,-1.8800159326799));
#186151=CARTESIAN_POINT('Ctrl Pts',(10.8498916141118,15.2,-1.88207019159341));
#186152=CARTESIAN_POINT('Ctrl Pts',(10.8534614692079,15.2,-1.88413729164533));
#186153=CARTESIAN_POINT('Ctrl Pts',(10.8579237884429,15.2,-1.88672116692147));
#186154=CARTESIAN_POINT('Ctrl Pts',(10.8623998578415,15.2,-1.88932510789172));
#186155=CARTESIAN_POINT('Ctrl Pts',(10.866889437146,15.2,-1.89194914664008));
#186156=CARTESIAN_POINT('Ctrl Pts',(10.8713790164505,15.2,-1.89457318538844));
#186157=CARTESIAN_POINT('Ctrl Pts',(10.8758821055176,15.2,-1.89721732467573));
#186158=CARTESIAN_POINT('Ctrl Pts',(10.8803984659507,15.2,-1.89988159668242));
#186159=CARTESIAN_POINT('Ctrl Pts',(10.884011554494,15.2,-1.90201301440394));
#186160=CARTESIAN_POINT('Ctrl Pts',(10.8876331373206,15.2,-1.90415731601359));
#186161=CARTESIAN_POINT('Ctrl Pts',(10.8912630922967,15.2,-1.90631452090977));
#186162=CARTESIAN_POINT('Ctrl Pts',(10.8948930467783,15.2,-1.90847172551203));
#186163=CARTESIAN_POINT('Ctrl Pts',(10.898531373786,15.2,-1.91064183205061));
#186164=CARTESIAN_POINT('Ctrl Pts',(10.9021779541537,15.2,-1.91282485542638));
#186165=CARTESIAN_POINT('Ctrl Pts',(10.9058245350183,15.2,-1.91500787909959));
#186166=CARTESIAN_POINT('Ctrl Pts',(10.9094793685083,15.2,-1.91720382148212));
#186167=CARTESIAN_POINT('Ctrl Pts',(10.9131423355024,15.2,-1.91941269650147));
#186168=CARTESIAN_POINT('Ctrl Pts',(10.9168053019974,15.2,-1.92162157121986));
#186169=CARTESIAN_POINT('Ctrl Pts',(10.920476403025,15.2,-1.92384338069638));
#186170=CARTESIAN_POINT('Ctrl Pts',(10.9241555188901,15.2,-1.92607813740126));
#186171=CARTESIAN_POINT('Ctrl Pts',(10.9287544140974,15.2,-1.92887158351071));
#186172=CARTESIAN_POINT('Ctrl Pts',(10.933365833635,15.2,-1.93168526253651));
#186173=CARTESIAN_POINT('Ctrl Pts',(10.9379895503701,15.2,-1.93451920114596));
#186174=CARTESIAN_POINT('Ctrl Pts',(10.9416885239598,15.2,-1.93678635215708));
#186175=CARTESIAN_POINT('Ctrl Pts',(10.9453953655553,15.2,-1.93906647086055));
#186176=CARTESIAN_POINT('Ctrl Pts',(10.9491099612191,15.2,-1.94135956921819));
#186177=CARTESIAN_POINT('Ctrl Pts',(10.9528245563768,15.2,-1.9436526672634));
#186178=CARTESIAN_POINT('Ctrl Pts',(10.9565469045485,15.2,-1.94595874733671));
#186179=CARTESIAN_POINT('Ctrl Pts',(10.9602768916317,15.2,-1.9482778206458));
#186180=CARTESIAN_POINT('Ctrl Pts',(10.9640068792231,15.2,-1.95059689427087));
#186181=CARTESIAN_POINT('Ctrl Pts',(10.9677445053847,15.2,-1.95292896159437));
#186182=CARTESIAN_POINT('Ctrl Pts',(10.9714896550332,15.2,-1.95527403649996));
#186183=CARTESIAN_POINT('Ctrl Pts',(10.9752348046818,15.2,-1.95761911140555));
#186184=CARTESIAN_POINT('Ctrl Pts',(10.9789874775562,15.2,-1.95997719481541));
#186185=CARTESIAN_POINT('Ctrl Pts',(10.982747561373,15.2,-1.96234829644598));
#186186=CARTESIAN_POINT('Ctrl Pts',(10.9855676239795,15.2,-1.96412662250737));
#186187=CARTESIAN_POINT('Ctrl Pts',(10.9883918563082,15.2,-1.96591227228832));
#186188=CARTESIAN_POINT('Ctrl Pts',(10.9912202085138,15.2,-1.96770525139694));
#186189=CARTESIAN_POINT('Ctrl Pts',(10.9940485607195,15.2,-1.96949823050555));
#186190=CARTESIAN_POINT('Ctrl Pts',(10.9968810333286,15.2,-1.97129853761216));
#186191=CARTESIAN_POINT('Ctrl Pts',(10.9997175803092,15.2,-1.97310617867212));
#186192=CARTESIAN_POINT('Ctrl Pts',(11.0025541272898,15.2,-1.97491381973208));
#186193=CARTESIAN_POINT('Ctrl Pts',(11.0053947479533,15.2,-1.97672879523283));
#186194=CARTESIAN_POINT('Ctrl Pts',(11.0082393950166,15.2,-1.97855110879162));
#186195=CARTESIAN_POINT('Ctrl Pts',(11.0110840420799,15.2,-1.98037342235041));
#186196=CARTESIAN_POINT('Ctrl Pts',(11.0139327161097,15.2,-1.98220307445057));
#186197=CARTESIAN_POINT('Ctrl Pts',(11.0167853701724,15.2,-1.98404007000819));
#186198=CARTESIAN_POINT('Ctrl Pts',(11.0205889092681,15.2,-1.98648939764082));
#186199=CARTESIAN_POINT('Ctrl Pts',(11.0243995234462,15.2,-1.98895178058563));
#186200=CARTESIAN_POINT('Ctrl Pts',(11.0282171033456,15.2,-1.9914272289009));
#186201=CARTESIAN_POINT('Ctrl Pts',(11.03108028801,15.2,-1.99328381496872));
#186202=CARTESIAN_POINT('Ctrl Pts',(11.0339473909669,15.2,-1.99514774970475));
#186203=CARTESIAN_POINT('Ctrl Pts',(11.0368183655713,15.2,-1.99701903872073));
#186204=CARTESIAN_POINT('Ctrl Pts',(11.0406463315365,15.2,-1.99951409062871));
#186205=CARTESIAN_POINT('Ctrl Pts',(11.0444811811421,15.2,-2.00202221673409));
#186206=CARTESIAN_POINT('Ctrl Pts',(11.0483228056052,15.2,-2.00454342530442));
#186207=CARTESIAN_POINT('Ctrl Pts',(11.0512040246067,15.2,-2.00643433216157));
#186208=CARTESIAN_POINT('Ctrl Pts',(11.054089053326,15.2,-2.00833259817077));
#186209=CARTESIAN_POINT('Ctrl Pts',(11.0569778483713,15.2,-2.01023822844873));
#186210=CARTESIAN_POINT('Ctrl Pts',(11.0598666428919,15.2,-2.0121438583805));
#186211=CARTESIAN_POINT('Ctrl Pts',(11.0627592032704,15.2,-2.01405685176123));
#186212=CARTESIAN_POINT('Ctrl Pts',(11.0656554825603,15.2,-2.01597721191324));
#186213=CARTESIAN_POINT('Ctrl Pts',(11.0685517618502,15.2,-2.01789757206525));
#186214=CARTESIAN_POINT('Ctrl Pts',(11.0714517619883,15.2,-2.01982529946402));
#186215=CARTESIAN_POINT('Ctrl Pts',(11.0743554365915,15.2,-2.02176039893602));
#186216=CARTESIAN_POINT('Ctrl Pts',(11.0772591111946,15.2,-2.02369549840801));
#186217=CARTESIAN_POINT('Ctrl Pts',(11.0801664606224,15.2,-2.0256379687708));
#186218=CARTESIAN_POINT('Ctrl Pts',(11.0830774402249,15.2,-2.02758781424162));
#186219=CARTESIAN_POINT('Ctrl Pts',(11.0869587467142,15.2,-2.03018760843886));
#186220=CARTESIAN_POINT('Ctrl Pts',(11.0908465071015,15.2,-2.03280051410986));
#186221=CARTESIAN_POINT('Ctrl Pts',(11.0947406148699,15.2,-2.03542653842099));
#186222=CARTESIAN_POINT('Ctrl Pts',(11.0996082487847,15.2,-2.03870906827322));
#186223=CARTESIAN_POINT('Ctrl Pts',(11.1044858017942,15.2,-2.04201209690141));
#186224=CARTESIAN_POINT('Ctrl Pts',(11.109373068344,15.2,-2.04533564077359));
#186225=CARTESIAN_POINT('Ctrl Pts',(11.1123054290197,15.2,-2.04732976760406));
#186226=CARTESIAN_POINT('Ctrl Pts',(11.115241287263,15.2,-2.04933128014494));
#186227=CARTESIAN_POINT('Ctrl Pts',(11.1181805983574,15.2,-2.05134018047957));
#186228=CARTESIAN_POINT('Ctrl Pts',(11.1211199089177,15.2,-2.05334908044926));
#186229=CARTESIAN_POINT('Ctrl Pts',(11.1240626720612,15.2,-2.05536536827688));
#186230=CARTESIAN_POINT('Ctrl Pts',(11.1270088455794,15.2,-2.057389048204));
#186231=CARTESIAN_POINT('Ctrl Pts',(11.1299550190977,15.2,-2.05941272813112));
#186232=CARTESIAN_POINT('Ctrl Pts',(11.1329046024572,15.2,-2.06144379860736));
#186233=CARTESIAN_POINT('Ctrl Pts',(11.1358575515583,15.2,-2.06348226449163));
#186234=CARTESIAN_POINT('Ctrl Pts',(11.1388105006593,15.2,-2.0655207303759));
#186235=CARTESIAN_POINT('Ctrl Pts',(11.1417668155519,15.2,-2.06756658960153));
#186236=CARTESIAN_POINT('Ctrl Pts',(11.1447264536524,15.2,-2.06961984698462));
#186237=CARTESIAN_POINT('Ctrl Pts',(11.1486726381448,15.2,-2.07235752374407));
#186238=CARTESIAN_POINT('Ctrl Pts',(11.1526247300242,15.2,-2.07510835093346));
#186239=CARTESIAN_POINT('Ctrl Pts',(11.1565826280493,15.2,-2.07787233466777));
#186240=CARTESIAN_POINT('Ctrl Pts',(11.160540525535,15.2,-2.08063631802549));
#186241=CARTESIAN_POINT('Ctrl Pts',(11.1645042281476,15.2,-2.08341345872595));
#186242=CARTESIAN_POINT('Ctrl Pts',(11.1684736354338,15.2,-2.08620376133031));
#186243=CARTESIAN_POINT('Ctrl Pts',(11.1714506910337,15.2,-2.08829648837863));
#186244=CARTESIAN_POINT('Ctrl Pts',(11.1744309554584,15.2,-2.09039662001811));
#186245=CARTESIAN_POINT('Ctrl Pts',(11.1774143860995,15.2,-2.09250415802386));
#186246=CARTESIAN_POINT('Ctrl Pts',(11.1823867706822,15.2,-2.09601672149441));
#186247=CARTESIAN_POINT('Ctrl Pts',(11.1873679517054,15.2,-2.0995498578114));
#186248=CARTESIAN_POINT('Ctrl Pts',(11.192357733204,15.2,-2.10310357882084));
#186249=CARTESIAN_POINT('Ctrl Pts',(11.1953516019945,15.2,-2.10523581134903));
#186250=CARTESIAN_POINT('Ctrl Pts',(11.1983485672053,15.2,-2.10737545409427));
#186251=CARTESIAN_POINT('Ctrl Pts',(11.2013485863459,15.2,-2.10952250901525));
#186252=CARTESIAN_POINT('Ctrl Pts',(11.2043486060315,15.2,-2.11166956432628));
#186253=CARTESIAN_POINT('Ctrl Pts',(11.2073516799846,15.2,-2.11382403163939));
#186254=CARTESIAN_POINT('Ctrl Pts',(11.2103577666719,15.2,-2.11598591299626));
#186255=CARTESIAN_POINT('Ctrl Pts',(11.2133638528131,15.2,-2.11814779396038));
#186256=CARTESIAN_POINT('Ctrl Pts',(11.2163729519875,15.2,-2.12031708903246));
#186257=CARTESIAN_POINT('Ctrl Pts',(11.2193850235866,15.2,-2.12249380045402));
#186258=CARTESIAN_POINT('Ctrl Pts',(11.2223970951858,15.2,-2.12467051187558));
#186259=CARTESIAN_POINT('Ctrl Pts',(11.2254121383653,15.2,-2.12685463855492));
#186260=CARTESIAN_POINT('Ctrl Pts',(11.2284301114777,15.2,-2.12904618348529));
#186261=CARTESIAN_POINT('Ctrl Pts',(11.2314480845901,15.2,-2.13123772841565));
#186262=CARTESIAN_POINT('Ctrl Pts',(11.2344689878767,15.2,-2.13343669205148));
#186263=CARTESIAN_POINT('Ctrl Pts',(11.2374927780305,15.2,-2.13564307406463));
#186264=CARTESIAN_POINT('Ctrl Pts',(11.2405165681844,15.2,-2.13784945607777));
#186265=CARTESIAN_POINT('Ctrl Pts',(11.2435432456968,15.2,-2.14006325823933));
#186266=CARTESIAN_POINT('Ctrl Pts',(11.2465727734614,15.2,-2.14228448028297));
#186267=CARTESIAN_POINT('Ctrl Pts',(11.2496023012261,15.2,-2.14450570232662));
#186268=CARTESIAN_POINT('Ctrl Pts',(11.2526346804489,15.2,-2.14673434582808));
#186269=CARTESIAN_POINT('Ctrl Pts',(11.2556698710466,15.2,-2.14897041128751));
#186270=CARTESIAN_POINT('Ctrl Pts',(11.2597167922111,15.2,-2.15195183217089));
#186271=CARTESIAN_POINT('Ctrl Pts',(11.2637687107826,15.2,-2.1549464469966));
#186272=CARTESIAN_POINT('Ctrl Pts',(11.2678255117444,15.2,-2.15795426128535));
#186273=CARTESIAN_POINT('Ctrl Pts',(11.2718823121534,15.2,-2.16096207516428));
#186274=CARTESIAN_POINT('Ctrl Pts',(11.2759439872013,15.2,-2.16398308926437));
#186275=CARTESIAN_POINT('Ctrl Pts',(11.2800104638684,15.2,-2.16701730357055));
#186276=CARTESIAN_POINT('Ctrl Pts',(11.2840769410895,15.2,-2.17005151829013));
#186277=CARTESIAN_POINT('Ctrl Pts',(11.2881482245559,15.2,-2.17309893283267));
#186278=CARTESIAN_POINT('Ctrl Pts',(11.2922242989999,15.2,-2.17615954700001));
#186279=CARTESIAN_POINT('Ctrl Pts',(10.0330625579999,15.2,-2.64164356400002));
#186280=CARTESIAN_POINT('Ctrl Pts',(10.0330625579999,11.6,-2.64164356400002));
#186281=CARTESIAN_POINT('Ctrl Pts',(10.0332343599999,15.2,-2.64167330400001));
#186282=CARTESIAN_POINT('Ctrl Pts',(10.0332343599999,11.6,-2.64167330400001));
#186283=CARTESIAN_POINT('Ctrl Pts',(10.0335839819999,15.2,-2.64173373800002));
#186284=CARTESIAN_POINT('Ctrl Pts',(10.0335839819999,11.6,-2.64173373800002));
#186285=CARTESIAN_POINT('Ctrl Pts',(10.0341137859999,15.2,-2.64182504800001));
#186286=CARTESIAN_POINT('Ctrl Pts',(10.0341137859999,11.6,-2.64182504800001));
#186287=CARTESIAN_POINT('Ctrl Pts',(10.0348275719999,15.2,-2.64194751900002));
#186288=CARTESIAN_POINT('Ctrl Pts',(10.0348275719999,11.6,-2.64194751900002));
#186289=CARTESIAN_POINT('Ctrl Pts',(10.0357305589999,15.2,-2.64210152600001));
#186290=CARTESIAN_POINT('Ctrl Pts',(10.0357305589999,11.6,-2.64210152600001));
#186291=CARTESIAN_POINT('Ctrl Pts',(10.0366483389999,15.2,-2.64225710800002));
#186292=CARTESIAN_POINT('Ctrl Pts',(10.0366483389999,11.6,-2.64225710800002));
#186293=CARTESIAN_POINT('Ctrl Pts',(10.0375756569999,15.2,-2.64241335000001));
#186294=CARTESIAN_POINT('Ctrl Pts',(10.0375756569999,11.6,-2.64241335000001));
#186295=CARTESIAN_POINT('Ctrl Pts',(10.0385124889999,15.2,-2.64257022900001));
#186296=CARTESIAN_POINT('Ctrl Pts',(10.0385124889999,11.6,-2.64257022900001));
#186297=CARTESIAN_POINT('Ctrl Pts',(10.0394588109999,15.2,-2.64272772400002));
#186298=CARTESIAN_POINT('Ctrl Pts',(10.0394588109999,11.6,-2.64272772400002));
#186299=CARTESIAN_POINT('Ctrl Pts',(10.0404146009999,15.2,-2.64288581300002));
#186300=CARTESIAN_POINT('Ctrl Pts',(10.0404146009999,11.6,-2.64288581300002));
#186301=CARTESIAN_POINT('Ctrl Pts',(10.0413798349999,15.2,-2.64304447300002));
#186302=CARTESIAN_POINT('Ctrl Pts',(10.0413798349999,11.6,-2.64304447300002));
#186303=CARTESIAN_POINT('Ctrl Pts',(10.0423544889999,15.2,-2.64320368200002));
#186304=CARTESIAN_POINT('Ctrl Pts',(10.0423544889999,11.6,-2.64320368200002));
#186305=CARTESIAN_POINT('Ctrl Pts',(10.0433385409999,15.2,-2.64336341800002));
#186306=CARTESIAN_POINT('Ctrl Pts',(10.0433385409999,11.6,-2.64336341800002));
#186307=CARTESIAN_POINT('Ctrl Pts',(10.0443319679999,15.2,-2.64352366000002));
#186308=CARTESIAN_POINT('Ctrl Pts',(10.0443319679999,11.6,-2.64352366000002));
#186309=CARTESIAN_POINT('Ctrl Pts',(10.0453347469999,15.2,-2.64368438700001));
#186310=CARTESIAN_POINT('Ctrl Pts',(10.0453347469999,11.6,-2.64368438700001));
#186311=CARTESIAN_POINT('Ctrl Pts',(10.0463468539999,15.2,-2.64384557600001));
#186312=CARTESIAN_POINT('Ctrl Pts',(10.0463468539999,11.6,-2.64384557600002));
#186313=CARTESIAN_POINT('Ctrl Pts',(10.0473682679999,15.2,-2.64400720800001));
#186314=CARTESIAN_POINT('Ctrl Pts',(10.0473682679999,11.6,-2.64400720800001));
#186315=CARTESIAN_POINT('Ctrl Pts',(10.0483989659999,15.2,-2.64416925900001));
#186316=CARTESIAN_POINT('Ctrl Pts',(10.0483989659999,11.6,-2.64416925900001));
#186317=CARTESIAN_POINT('Ctrl Pts',(10.0494389259999,15.2,-2.64433171000002));
#186318=CARTESIAN_POINT('Ctrl Pts',(10.0494389259999,11.6,-2.64433171000002));
#186319=CARTESIAN_POINT('Ctrl Pts',(10.0504881239999,15.2,-2.64449453900002));
#186320=CARTESIAN_POINT('Ctrl Pts',(10.0504881239999,11.6,-2.64449453900002));
#186321=CARTESIAN_POINT('Ctrl Pts',(10.0515465379999,15.2,-2.64465772600001));
#186322=CARTESIAN_POINT('Ctrl Pts',(10.0515465379999,11.6,-2.64465772600001));
#186323=CARTESIAN_POINT('Ctrl Pts',(10.0526141479999,15.2,-2.64482124900002));
#186324=CARTESIAN_POINT('Ctrl Pts',(10.0526141479999,11.6,-2.64482124900002));
#186325=CARTESIAN_POINT('Ctrl Pts',(10.0536909299999,15.2,-2.64498508700001));
#186326=CARTESIAN_POINT('Ctrl Pts',(10.0536909299999,11.6,-2.64498508700001));
#186327=CARTESIAN_POINT('Ctrl Pts',(10.0547768619999,15.2,-2.64514922200001));
#186328=CARTESIAN_POINT('Ctrl Pts',(10.0547768619999,11.6,-2.64514922200001));
#186329=CARTESIAN_POINT('Ctrl Pts',(10.0558719239999,15.2,-2.64531363100001));
#186330=CARTESIAN_POINT('Ctrl Pts',(10.0558719239999,11.6,-2.64531363100002));
#186331=CARTESIAN_POINT('Ctrl Pts',(10.0569760909999,15.2,-2.64547829500001));
#186332=CARTESIAN_POINT('Ctrl Pts',(10.0569760909999,11.6,-2.64547829500001));
#186333=CARTESIAN_POINT('Ctrl Pts',(10.0580893439999,15.2,-2.64564319300002));
#186334=CARTESIAN_POINT('Ctrl Pts',(10.0580893439999,11.6,-2.64564319300002));
#186335=CARTESIAN_POINT('Ctrl Pts',(10.0592116599999,15.2,-2.64580830600002));
#186336=CARTESIAN_POINT('Ctrl Pts',(10.0592116599999,11.6,-2.64580830600002));
#186337=CARTESIAN_POINT('Ctrl Pts',(10.0603430189999,15.2,-2.64597361200002));
#186338=CARTESIAN_POINT('Ctrl Pts',(10.0603430189999,11.6,-2.64597361200002));
#186339=CARTESIAN_POINT('Ctrl Pts',(10.0614833969999,15.2,-2.64613909300001));
#186340=CARTESIAN_POINT('Ctrl Pts',(10.0614833969999,11.6,-2.64613909300001));
#186341=CARTESIAN_POINT('Ctrl Pts',(10.0626327749999,15.2,-2.64630472800001));
#186342=CARTESIAN_POINT('Ctrl Pts',(10.0626327749999,11.6,-2.64630472800001));
#186343=CARTESIAN_POINT('Ctrl Pts',(10.0637911309999,15.2,-2.64647049800002));
#186344=CARTESIAN_POINT('Ctrl Pts',(10.0637911309999,11.6,-2.64647049800002));
#186345=CARTESIAN_POINT('Ctrl Pts',(10.0649584439999,15.2,-2.64663638300001));
#186346=CARTESIAN_POINT('Ctrl Pts',(10.0649584439999,11.6,-2.64663638300001));
#186347=CARTESIAN_POINT('Ctrl Pts',(10.0661346919999,15.2,-2.64680236400002));
#186348=CARTESIAN_POINT('Ctrl Pts',(10.0661346919999,11.6,-2.64680236400002));
#186349=CARTESIAN_POINT('Ctrl Pts',(10.0673198549999,15.2,-2.64696842100001));
#186350=CARTESIAN_POINT('Ctrl Pts',(10.0673198549999,11.6,-2.64696842100001));
#186351=CARTESIAN_POINT('Ctrl Pts',(10.0685139109999,15.2,-2.64713453500002));
#186352=CARTESIAN_POINT('Ctrl Pts',(10.0685139109999,11.6,-2.64713453500002));
#186353=CARTESIAN_POINT('Ctrl Pts',(10.0697168409999,15.2,-2.64730068700001));
#186354=CARTESIAN_POINT('Ctrl Pts',(10.0697168409999,11.6,-2.64730068700001));
#186355=CARTESIAN_POINT('Ctrl Pts',(10.0709286239999,15.2,-2.64746685700001));
#186356=CARTESIAN_POINT('Ctrl Pts',(10.0709286239999,11.6,-2.64746685700001));
#186357=CARTESIAN_POINT('Ctrl Pts',(10.0721492369999,15.2,-2.64763302600001));
#186358=CARTESIAN_POINT('Ctrl Pts',(10.0721492369999,11.6,-2.64763302600001));
#186359=CARTESIAN_POINT('Ctrl Pts',(10.0733786619999,15.2,-2.64779917600002));
#186360=CARTESIAN_POINT('Ctrl Pts',(10.0733786619999,11.6,-2.64779917600002));
#186361=CARTESIAN_POINT('Ctrl Pts',(10.0746168779999,15.2,-2.64796528800002));
#186362=CARTESIAN_POINT('Ctrl Pts',(10.0746168779999,11.6,-2.64796528800002));
#186363=CARTESIAN_POINT('Ctrl Pts',(10.0758638629999,15.2,-2.64813134200002));
#186364=CARTESIAN_POINT('Ctrl Pts',(10.0758638629999,11.6,-2.64813134200002));
#186365=CARTESIAN_POINT('Ctrl Pts',(10.0771195969999,15.2,-2.64829732100001));
#186366=CARTESIAN_POINT('Ctrl Pts',(10.0771195969999,11.6,-2.64829732100001));
#186367=CARTESIAN_POINT('Ctrl Pts',(10.0783840629999,15.2,-2.64846320600002));
#186368=CARTESIAN_POINT('Ctrl Pts',(10.0783840629999,11.6,-2.64846320600002));
#186369=CARTESIAN_POINT('Ctrl Pts',(10.0796572369999,15.2,-2.64862897800001));
#186370=CARTESIAN_POINT('Ctrl Pts',(10.0796572369999,11.6,-2.64862897800001));
#186371=CARTESIAN_POINT('Ctrl Pts',(10.0809390999999,15.2,-2.64879461900001));
#186372=CARTESIAN_POINT('Ctrl Pts',(10.0809390999999,11.6,-2.64879461900001));
#186373=CARTESIAN_POINT('Ctrl Pts',(10.0822296339999,15.2,-2.64896011100001));
#186374=CARTESIAN_POINT('Ctrl Pts',(10.0822296339999,11.6,-2.64896011100001));
#186375=CARTESIAN_POINT('Ctrl Pts',(10.0835288159999,15.2,-2.64912543500001));
#186376=CARTESIAN_POINT('Ctrl Pts',(10.0835288159999,11.6,-2.64912543500001));
#186377=CARTESIAN_POINT('Ctrl Pts',(10.0848366279999,15.2,-2.64929057400002));
#186378=CARTESIAN_POINT('Ctrl Pts',(10.0848366279999,11.6,-2.64929057400002));
#186379=CARTESIAN_POINT('Ctrl Pts',(10.0861530489999,15.2,-2.64945550800002));
#186380=CARTESIAN_POINT('Ctrl Pts',(10.0861530489999,11.6,-2.64945550800002));
#186381=CARTESIAN_POINT('Ctrl Pts',(10.0874780619999,15.2,-2.64962022200002));
#186382=CARTESIAN_POINT('Ctrl Pts',(10.0874780619999,11.6,-2.64962022200002));
#186383=CARTESIAN_POINT('Ctrl Pts',(10.0888116439999,15.2,-2.64978469600001));
#186384=CARTESIAN_POINT('Ctrl Pts',(10.0888116439999,11.6,-2.64978469600001));
#186385=CARTESIAN_POINT('Ctrl Pts',(10.0901537779999,15.2,-2.64994891200002));
#186386=CARTESIAN_POINT('Ctrl Pts',(10.0901537779999,11.6,-2.64994891200002));
#186387=CARTESIAN_POINT('Ctrl Pts',(10.0915044419999,15.2,-2.65011285400002));
#186388=CARTESIAN_POINT('Ctrl Pts',(10.0915044419999,11.6,-2.65011285400002));
#186389=CARTESIAN_POINT('Ctrl Pts',(10.0928636199999,15.2,-2.65027650400001));
#186390=CARTESIAN_POINT('Ctrl Pts',(10.0928636199999,11.6,-2.65027650400001));
#186391=CARTESIAN_POINT('Ctrl Pts',(10.0942312899999,15.2,-2.65043984300001));
#186392=CARTESIAN_POINT('Ctrl Pts',(10.0942312899999,11.6,-2.65043984300001));
#186393=CARTESIAN_POINT('Ctrl Pts',(10.0956074329999,15.2,-2.65060285500001));
#186394=CARTESIAN_POINT('Ctrl Pts',(10.0956074329999,11.6,-2.65060285500002));
#186395=CARTESIAN_POINT('Ctrl Pts',(10.0969920309999,15.2,-2.65076552200001));
#186396=CARTESIAN_POINT('Ctrl Pts',(10.0969920309999,11.6,-2.65076552200001));
#186397=CARTESIAN_POINT('Ctrl Pts',(10.0983850649999,15.2,-2.65092782800001));
#186398=CARTESIAN_POINT('Ctrl Pts',(10.0983850649999,11.6,-2.65092782800001));
#186399=CARTESIAN_POINT('Ctrl Pts',(10.0997865139999,15.2,-2.65108975600001));
#186400=CARTESIAN_POINT('Ctrl Pts',(10.0997865139999,11.6,-2.65108975600001));
#186401=CARTESIAN_POINT('Ctrl Pts',(10.1011963619999,15.2,-2.65125128600001));
#186402=CARTESIAN_POINT('Ctrl Pts',(10.1011963619999,11.6,-2.65125128600001));
#186403=CARTESIAN_POINT('Ctrl Pts',(10.1026145869999,15.2,-2.65141240300002));
#186404=CARTESIAN_POINT('Ctrl Pts',(10.1026145869999,11.6,-2.65141240300002));
#186405=CARTESIAN_POINT('Ctrl Pts',(10.1040411729999,15.2,-2.65157309000001));
#186406=CARTESIAN_POINT('Ctrl Pts',(10.1040411729999,11.6,-2.65157309000001));
#186407=CARTESIAN_POINT('Ctrl Pts',(10.1054760989999,15.2,-2.65173333000002));
#186408=CARTESIAN_POINT('Ctrl Pts',(10.1054760989999,11.6,-2.65173333000002));
#186409=CARTESIAN_POINT('Ctrl Pts',(10.1069193469999,15.2,-2.65189310700002));
#186410=CARTESIAN_POINT('Ctrl Pts',(10.1069193469999,11.6,-2.65189310700002));
#186411=CARTESIAN_POINT('Ctrl Pts',(10.1083708989999,15.2,-2.65205240400002));
#186412=CARTESIAN_POINT('Ctrl Pts',(10.1083708989999,11.6,-2.65205240400002));
#186413=CARTESIAN_POINT('Ctrl Pts',(10.1098307359999,15.2,-2.65221120400001));
#186414=CARTESIAN_POINT('Ctrl Pts',(10.1098307359999,11.6,-2.65221120400001));
#186415=CARTESIAN_POINT('Ctrl Pts',(10.1112988399999,15.2,-2.65236949000001));
#186416=CARTESIAN_POINT('Ctrl Pts',(10.1112988399999,11.6,-2.65236949000002));
#186417=CARTESIAN_POINT('Ctrl Pts',(10.1127751919999,15.2,-2.65252724600002));
#186418=CARTESIAN_POINT('Ctrl Pts',(10.1127751919999,11.6,-2.65252724600002));
#186419=CARTESIAN_POINT('Ctrl Pts',(10.1142597739999,15.2,-2.65268445700002));
#186420=CARTESIAN_POINT('Ctrl Pts',(10.1142597739999,11.6,-2.65268445700002));
#186421=CARTESIAN_POINT('Ctrl Pts',(10.1157525679999,15.2,-2.65284110400001));
#186422=CARTESIAN_POINT('Ctrl Pts',(10.1157525679999,11.6,-2.65284110400001));
#186423=CARTESIAN_POINT('Ctrl Pts',(10.1172535539999,15.2,-2.65299717300001));
#186424=CARTESIAN_POINT('Ctrl Pts',(10.1172535539999,11.6,-2.65299717300001));
#186425=CARTESIAN_POINT('Ctrl Pts',(10.1187627169999,15.2,-2.65315264700002));
#186426=CARTESIAN_POINT('Ctrl Pts',(10.1187627169999,11.6,-2.65315264700002));
#186427=CARTESIAN_POINT('Ctrl Pts',(10.1202800349999,15.2,-2.65330750900001));
#186428=CARTESIAN_POINT('Ctrl Pts',(10.1202800349999,11.6,-2.65330750900001));
#186429=CARTESIAN_POINT('Ctrl Pts',(10.1218054939999,15.2,-2.65346174700001));
#186430=CARTESIAN_POINT('Ctrl Pts',(10.1218054939999,11.6,-2.65346174700001));
#186431=CARTESIAN_POINT('Ctrl Pts',(10.1233390739999,15.2,-2.65361533900002));
#186432=CARTESIAN_POINT('Ctrl Pts',(10.1233390739999,11.6,-2.65361533900002));
#186433=CARTESIAN_POINT('Ctrl Pts',(10.1248807569999,15.2,-2.65376827500001));
#186434=CARTESIAN_POINT('Ctrl Pts',(10.1248807569999,11.6,-2.65376827500001));
#186435=CARTESIAN_POINT('Ctrl Pts',(10.1264305249999,15.2,-2.65392053400001));
#186436=CARTESIAN_POINT('Ctrl Pts',(10.1264305249999,11.6,-2.65392053400001));
#186437=CARTESIAN_POINT('Ctrl Pts',(10.1279883609999,15.2,-2.65407210400001));
#186438=CARTESIAN_POINT('Ctrl Pts',(10.1279883609999,11.6,-2.65407210400001));
#186439=CARTESIAN_POINT('Ctrl Pts',(10.1295542479999,15.2,-2.65422296900002));
#186440=CARTESIAN_POINT('Ctrl Pts',(10.1295542479999,11.6,-2.65422296900002));
#186441=CARTESIAN_POINT('Ctrl Pts',(10.1311281659999,15.2,-2.65437311200001));
#186442=CARTESIAN_POINT('Ctrl Pts',(10.1311281659999,11.6,-2.65437311200001));
#186443=CARTESIAN_POINT('Ctrl Pts',(10.1327100999999,15.2,-2.65452251800002));
#186444=CARTESIAN_POINT('Ctrl Pts',(10.1327100999999,11.6,-2.65452251800002));
#186445=CARTESIAN_POINT('Ctrl Pts',(10.1343000309999,15.2,-2.65467117300001));
#186446=CARTESIAN_POINT('Ctrl Pts',(10.1343000309999,11.6,-2.65467117300001));
#186447=CARTESIAN_POINT('Ctrl Pts',(10.1358979419999,15.2,-2.65481905900002));
#186448=CARTESIAN_POINT('Ctrl Pts',(10.1358979419999,11.6,-2.65481905900002));
#186449=CARTESIAN_POINT('Ctrl Pts',(10.1375038149999,15.2,-2.65496616300001));
#186450=CARTESIAN_POINT('Ctrl Pts',(10.1375038149999,11.6,-2.65496616300001));
#186451=CARTESIAN_POINT('Ctrl Pts',(10.1391176329999,15.2,-2.65511246900001));
#186452=CARTESIAN_POINT('Ctrl Pts',(10.1391176329999,11.6,-2.65511246900001));
#186453=CARTESIAN_POINT('Ctrl Pts',(10.1407393799999,15.2,-2.65525796100002));
#186454=CARTESIAN_POINT('Ctrl Pts',(10.1407393799999,11.6,-2.65525796100002));
#186455=CARTESIAN_POINT('Ctrl Pts',(10.1423690359999,15.2,-2.65540262600001));
#186456=CARTESIAN_POINT('Ctrl Pts',(10.1423690359999,11.6,-2.65540262600001));
#186457=CARTESIAN_POINT('Ctrl Pts',(10.1440065869999,15.2,-2.65554644800002));
#186458=CARTESIAN_POINT('Ctrl Pts',(10.1440065869999,11.6,-2.65554644800002));
#186459=CARTESIAN_POINT('Ctrl Pts',(10.1456520129999,15.2,-2.65568941000002));
#186460=CARTESIAN_POINT('Ctrl Pts',(10.1456520129999,11.6,-2.65568941000002));
#186461=CARTESIAN_POINT('Ctrl Pts',(10.1473052979999,15.2,-2.65583150200001));
#186462=CARTESIAN_POINT('Ctrl Pts',(10.1473052979999,11.6,-2.65583150200001));
#186463=CARTESIAN_POINT('Ctrl Pts',(10.1489664269999,15.2,-2.65597270400002));
#186464=CARTESIAN_POINT('Ctrl Pts',(10.1489664269999,11.6,-2.65597270400002));
#186465=CARTESIAN_POINT('Ctrl Pts',(10.1506353799999,15.2,-2.65611300300002));
#186466=CARTESIAN_POINT('Ctrl Pts',(10.1506353799999,11.6,-2.65611300300002));
#186467=CARTESIAN_POINT('Ctrl Pts',(10.1523121419999,15.2,-2.65625238700002));
#186468=CARTESIAN_POINT('Ctrl Pts',(10.1523121419999,11.6,-2.65625238700002));
#186469=CARTESIAN_POINT('Ctrl Pts',(10.1539966949999,15.2,-2.65639083800002));
#186470=CARTESIAN_POINT('Ctrl Pts',(10.1539966949999,11.6,-2.65639083800002));
#186471=CARTESIAN_POINT('Ctrl Pts',(10.1556890229999,15.2,-2.65652834200001));
#186472=CARTESIAN_POINT('Ctrl Pts',(10.1556890229999,11.6,-2.65652834200001));
#186473=CARTESIAN_POINT('Ctrl Pts',(10.1573891099999,15.2,-2.65666488700001));
#186474=CARTESIAN_POINT('Ctrl Pts',(10.1573891099999,11.6,-2.65666488700001));
#186475=CARTESIAN_POINT('Ctrl Pts',(10.1590969379999,15.2,-2.65680045500002));
#186476=CARTESIAN_POINT('Ctrl Pts',(10.1590969379999,11.6,-2.65680045500002));
#186477=CARTESIAN_POINT('Ctrl Pts',(10.1608124909999,15.2,-2.65693503500001));
#186478=CARTESIAN_POINT('Ctrl Pts',(10.1608124909999,11.6,-2.65693503500001));
#186479=CARTESIAN_POINT('Ctrl Pts',(10.1625357519999,15.2,-2.65706861000002));
#186480=CARTESIAN_POINT('Ctrl Pts',(10.1625357519999,11.6,-2.65706861000002));
#186481=CARTESIAN_POINT('Ctrl Pts',(10.1642667059999,15.2,-2.65720116800002));
#186482=CARTESIAN_POINT('Ctrl Pts',(10.1642667059999,11.6,-2.65720116800002));
#186483=CARTESIAN_POINT('Ctrl Pts',(10.1660053339999,15.2,-2.65733269300001));
#186484=CARTESIAN_POINT('Ctrl Pts',(10.1660053339999,11.6,-2.65733269300001));
#186485=CARTESIAN_POINT('Ctrl Pts',(10.1677516209999,15.2,-2.65746317300001));
#186486=CARTESIAN_POINT('Ctrl Pts',(10.1677516209999,11.6,-2.65746317300001));
#186487=CARTESIAN_POINT('Ctrl Pts',(10.1695055519999,15.2,-2.65759259200001));
#186488=CARTESIAN_POINT('Ctrl Pts',(10.1695055519999,11.6,-2.65759259200001));
#186489=CARTESIAN_POINT('Ctrl Pts',(10.1712671079999,15.2,-2.65772093700001));
#186490=CARTESIAN_POINT('Ctrl Pts',(10.1712671079999,11.6,-2.65772093700001));
#186491=CARTESIAN_POINT('Ctrl Pts',(10.1730362739999,15.2,-2.65784819400002));
#186492=CARTESIAN_POINT('Ctrl Pts',(10.1730362739999,11.6,-2.65784819400002));
#186493=CARTESIAN_POINT('Ctrl Pts',(10.1748130349999,15.2,-2.65797434800001));
#186494=CARTESIAN_POINT('Ctrl Pts',(10.1748130349999,11.6,-2.65797434800001));
#186495=CARTESIAN_POINT('Ctrl Pts',(10.1765973729999,15.2,-2.65809938700002));
#186496=CARTESIAN_POINT('Ctrl Pts',(10.1765973729999,11.6,-2.65809938700002));
#186497=CARTESIAN_POINT('Ctrl Pts',(10.1783892739999,15.2,-2.65822329700002));
#186498=CARTESIAN_POINT('Ctrl Pts',(10.1783892739999,11.6,-2.65822329700002));
#186499=CARTESIAN_POINT('Ctrl Pts',(10.1801887189999,15.2,-2.65834606300002));
#186500=CARTESIAN_POINT('Ctrl Pts',(10.1801887189999,11.6,-2.65834606300002));
#186501=CARTESIAN_POINT('Ctrl Pts',(10.1819956949999,15.2,-2.65846767300001));
#186502=CARTESIAN_POINT('Ctrl Pts',(10.1819956949999,11.6,-2.65846767300001));
#186503=CARTESIAN_POINT('Ctrl Pts',(10.1838101829999,15.2,-2.65858811100002));
#186504=CARTESIAN_POINT('Ctrl Pts',(10.1838101829999,11.6,-2.65858811100002));
#186505=CARTESIAN_POINT('Ctrl Pts',(10.1856321709999,15.2,-2.65870736700001));
#186506=CARTESIAN_POINT('Ctrl Pts',(10.1856321709999,11.6,-2.65870736700002));
#186507=CARTESIAN_POINT('Ctrl Pts',(10.1874616389999,15.2,-2.65882542500002));
#186508=CARTESIAN_POINT('Ctrl Pts',(10.1874616389999,11.6,-2.65882542500002));
#186509=CARTESIAN_POINT('Ctrl Pts',(10.1892985749999,15.2,-2.65894227200001));
#186510=CARTESIAN_POINT('Ctrl Pts',(10.1892985749999,11.6,-2.65894227200001));
#186511=CARTESIAN_POINT('Ctrl Pts',(10.1911429609999,15.2,-2.65905789600001));
#186512=CARTESIAN_POINT('Ctrl Pts',(10.1911429609999,11.6,-2.65905789600001));
#186513=CARTESIAN_POINT('Ctrl Pts',(10.1929947809999,15.2,-2.65917228300002));
#186514=CARTESIAN_POINT('Ctrl Pts',(10.1929947809999,11.6,-2.65917228300002));
#186515=CARTESIAN_POINT('Ctrl Pts',(10.1948540199999,15.2,-2.65928541800001));
#186516=CARTESIAN_POINT('Ctrl Pts',(10.1948540199999,11.6,-2.65928541800002));
#186517=CARTESIAN_POINT('Ctrl Pts',(10.1967206629999,15.2,-2.65939729100001));
#186518=CARTESIAN_POINT('Ctrl Pts',(10.1967206629999,11.6,-2.65939729100001));
#186519=CARTESIAN_POINT('Ctrl Pts',(10.1985946949999,15.2,-2.65950788700001));
#186520=CARTESIAN_POINT('Ctrl Pts',(10.1985946949999,11.6,-2.65950788700001));
#186521=CARTESIAN_POINT('Ctrl Pts',(10.2004760989999,15.2,-2.65961719300002));
#186522=CARTESIAN_POINT('Ctrl Pts',(10.2004760989999,11.6,-2.65961719300002));
#186523=CARTESIAN_POINT('Ctrl Pts',(10.2023648589999,15.2,-2.65972519600002));
#186524=CARTESIAN_POINT('Ctrl Pts',(10.2023648589999,11.6,-2.65972519600002));
#186525=CARTESIAN_POINT('Ctrl Pts',(10.2042609619999,15.2,-2.65983188400002));
#186526=CARTESIAN_POINT('Ctrl Pts',(10.2042609619999,11.6,-2.65983188400002));
#186527=CARTESIAN_POINT('Ctrl Pts',(10.2061643889999,15.2,-2.65993724300001));
#186528=CARTESIAN_POINT('Ctrl Pts',(10.2061643889999,11.6,-2.65993724300001));
#186529=CARTESIAN_POINT('Ctrl Pts',(10.2080751289999,15.2,-2.66004126100002));
#186530=CARTESIAN_POINT('Ctrl Pts',(10.2080751289999,11.6,-2.66004126100002));
#186531=CARTESIAN_POINT('Ctrl Pts',(10.2099931639999,15.2,-2.66014392600002));
#186532=CARTESIAN_POINT('Ctrl Pts',(10.2099931639999,11.6,-2.66014392600002));
#186533=CARTESIAN_POINT('Ctrl Pts',(10.2119184799999,15.2,-2.66024522300001));
#186534=CARTESIAN_POINT('Ctrl Pts',(10.2119184799999,11.6,-2.66024522300001));
#186535=CARTESIAN_POINT('Ctrl Pts',(10.2138510599999,15.2,-2.66034514000001));
#186536=CARTESIAN_POINT('Ctrl Pts',(10.2138510599999,11.6,-2.66034514000001));
#186537=CARTESIAN_POINT('Ctrl Pts',(10.2157908909999,15.2,-2.66044366600001));
#186538=CARTESIAN_POINT('Ctrl Pts',(10.2157908909999,11.6,-2.66044366600001));
#186539=CARTESIAN_POINT('Ctrl Pts',(10.2177379569999,15.2,-2.66054078700002));
#186540=CARTESIAN_POINT('Ctrl Pts',(10.2177379569999,11.6,-2.66054078700002));
#186541=CARTESIAN_POINT('Ctrl Pts',(10.2196922419999,15.2,-2.66063649100001));
#186542=CARTESIAN_POINT('Ctrl Pts',(10.2196922419999,11.6,-2.66063649100001));
#186543=CARTESIAN_POINT('Ctrl Pts',(10.2216537329999,15.2,-2.66073076600001));
#186544=CARTESIAN_POINT('Ctrl Pts',(10.2216537329999,11.6,-2.66073076600002));
#186545=CARTESIAN_POINT('Ctrl Pts',(10.2236224129999,15.2,-2.66082359800001));
#186546=CARTESIAN_POINT('Ctrl Pts',(10.2236224129999,11.6,-2.66082359800001));
#186547=CARTESIAN_POINT('Ctrl Pts',(10.2255982689999,15.2,-2.66091497700002));
#186548=CARTESIAN_POINT('Ctrl Pts',(10.2255982689999,11.6,-2.66091497700002));
#186549=CARTESIAN_POINT('Ctrl Pts',(10.2275812839999,15.2,-2.66100488900001));
#186550=CARTESIAN_POINT('Ctrl Pts',(10.2275812839999,11.6,-2.66100488900001));
#186551=CARTESIAN_POINT('Ctrl Pts',(10.2295714459999,15.2,-2.66109332200001));
#186552=CARTESIAN_POINT('Ctrl Pts',(10.2295714459999,11.6,-2.66109332200001));
#186553=CARTESIAN_POINT('Ctrl Pts',(10.2315687369999,15.2,-2.66118026400001));
#186554=CARTESIAN_POINT('Ctrl Pts',(10.2315687369999,11.6,-2.66118026400001));
#186555=CARTESIAN_POINT('Ctrl Pts',(10.2335731439999,15.2,-2.66126570200001));
#186556=CARTESIAN_POINT('Ctrl Pts',(10.2335731439999,11.6,-2.66126570200001));
#186557=CARTESIAN_POINT('Ctrl Pts',(10.2355846529999,15.2,-2.66134962600002));
#186558=CARTESIAN_POINT('Ctrl Pts',(10.2355846529999,11.6,-2.66134962600002));
#186559=CARTESIAN_POINT('Ctrl Pts',(10.2376032469999,15.2,-2.66143202200002));
#186560=CARTESIAN_POINT('Ctrl Pts',(10.2376032469999,11.6,-2.66143202200002));
#186561=CARTESIAN_POINT('Ctrl Pts',(10.2396289129999,15.2,-2.66151288000001));
#186562=CARTESIAN_POINT('Ctrl Pts',(10.2396289129999,11.6,-2.66151288000001));
#186563=CARTESIAN_POINT('Ctrl Pts',(10.2416616369999,15.2,-2.66159218500002));
#186564=CARTESIAN_POINT('Ctrl Pts',(10.2416616369999,11.6,-2.66159218500002));
#186565=CARTESIAN_POINT('Ctrl Pts',(10.2437014029999,15.2,-2.66166992700001));
#186566=CARTESIAN_POINT('Ctrl Pts',(10.2437014029999,11.6,-2.66166992700001));
#186567=CARTESIAN_POINT('Ctrl Pts',(10.2457481969999,15.2,-2.66174609500001));
#186568=CARTESIAN_POINT('Ctrl Pts',(10.2457481969999,11.6,-2.66174609500002));
#186569=CARTESIAN_POINT('Ctrl Pts',(10.2478020049999,15.2,-2.66182067600001));
#186570=CARTESIAN_POINT('Ctrl Pts',(10.2478020049999,11.6,-2.66182067600001));
#186571=CARTESIAN_POINT('Ctrl Pts',(10.2498628119999,15.2,-2.66189365800001));
#186572=CARTESIAN_POINT('Ctrl Pts',(10.2498628119999,11.6,-2.66189365800001));
#186573=CARTESIAN_POINT('Ctrl Pts',(10.2519306029999,15.2,-2.66196503000002));
#186574=CARTESIAN_POINT('Ctrl Pts',(10.2519306029999,11.6,-2.66196503000002));
#186575=CARTESIAN_POINT('Ctrl Pts',(10.2540053659999,15.2,-2.66203478000001));
#186576=CARTESIAN_POINT('Ctrl Pts',(10.2540053659999,11.6,-2.66203478000001));
#186577=CARTESIAN_POINT('Ctrl Pts',(10.2560870839999,15.2,-2.66210289700001));
#186578=CARTESIAN_POINT('Ctrl Pts',(10.2560870839999,11.6,-2.66210289700001));
#186579=CARTESIAN_POINT('Ctrl Pts',(10.2581757429999,15.2,-2.66216936800001));
#186580=CARTESIAN_POINT('Ctrl Pts',(10.2581757429999,11.6,-2.66216936800001));
#186581=CARTESIAN_POINT('Ctrl Pts',(10.2602713319999,15.2,-2.66223418300001));
#186582=CARTESIAN_POINT('Ctrl Pts',(10.2602713319999,11.6,-2.66223418300001));
#186583=CARTESIAN_POINT('Ctrl Pts',(10.2623738329999,15.2,-2.66229733000001));
#186584=CARTESIAN_POINT('Ctrl Pts',(10.2623738329999,11.6,-2.66229733000001));
#186585=CARTESIAN_POINT('Ctrl Pts',(10.2644832329999,15.2,-2.66235879800002));
#186586=CARTESIAN_POINT('Ctrl Pts',(10.2644832329999,11.6,-2.66235879800002));
#186587=CARTESIAN_POINT('Ctrl Pts',(10.2665995189999,15.2,-2.66241857400002));
#186588=CARTESIAN_POINT('Ctrl Pts',(10.2665995189999,11.6,-2.66241857400002));
#186589=CARTESIAN_POINT('Ctrl Pts',(10.2687226749999,15.2,-2.66247664800002));
#186590=CARTESIAN_POINT('Ctrl Pts',(10.2687226749999,11.6,-2.66247664800002));
#186591=CARTESIAN_POINT('Ctrl Pts',(10.2708526889999,15.2,-2.66253300900001));
#186592=CARTESIAN_POINT('Ctrl Pts',(10.2708526889999,11.6,-2.66253300900001));
#186593=CARTESIAN_POINT('Ctrl Pts',(10.2729895449999,15.2,-2.66258764600002));
#186594=CARTESIAN_POINT('Ctrl Pts',(10.2729895449999,11.6,-2.66258764600002));
#186595=CARTESIAN_POINT('Ctrl Pts',(10.2751332309999,15.2,-2.66264054600001));
#186596=CARTESIAN_POINT('Ctrl Pts',(10.2751332309999,11.6,-2.66264054600002));
#186597=CARTESIAN_POINT('Ctrl Pts',(10.2772837319999,15.2,-2.66269169900001));
#186598=CARTESIAN_POINT('Ctrl Pts',(10.2772837319999,11.6,-2.66269169900002));
#186599=CARTESIAN_POINT('Ctrl Pts',(10.2794410339999,15.2,-2.66274109400001));
#186600=CARTESIAN_POINT('Ctrl Pts',(10.2794410339999,11.6,-2.66274109400001));
#186601=CARTESIAN_POINT('Ctrl Pts',(10.2816051239999,15.2,-2.66278872000001));
#186602=CARTESIAN_POINT('Ctrl Pts',(10.2816051239999,11.6,-2.66278872000001));
#186603=CARTESIAN_POINT('Ctrl Pts',(10.2837759869999,15.2,-2.66283456600001));
#186604=CARTESIAN_POINT('Ctrl Pts',(10.2837759869999,11.6,-2.66283456600001));
#186605=CARTESIAN_POINT('Ctrl Pts',(10.2859536089999,15.2,-2.66287862000001));
#186606=CARTESIAN_POINT('Ctrl Pts',(10.2859536089999,11.6,-2.66287862000001));
#186607=CARTESIAN_POINT('Ctrl Pts',(10.2881379789999,15.2,-2.66292087100001));
#186608=CARTESIAN_POINT('Ctrl Pts',(10.2881379789999,11.6,-2.66292087100001));
#186609=CARTESIAN_POINT('Ctrl Pts',(10.2903290789999,15.2,-2.66296131100002));
#186610=CARTESIAN_POINT('Ctrl Pts',(10.2903290789999,11.6,-2.66296131100002));
#186611=CARTESIAN_POINT('Ctrl Pts',(10.2925268989999,15.2,-2.66299992600001));
#186612=CARTESIAN_POINT('Ctrl Pts',(10.2925268989999,11.6,-2.66299992600001));
#186613=CARTESIAN_POINT('Ctrl Pts',(10.2947314239999,15.2,-2.66303670600001));
#186614=CARTESIAN_POINT('Ctrl Pts',(10.2947314239999,11.6,-2.66303670600002));
#186615=CARTESIAN_POINT('Ctrl Pts',(10.2969426399999,15.2,-2.66307164000001));
#186616=CARTESIAN_POINT('Ctrl Pts',(10.2969426399999,11.6,-2.66307164000001));
#186617=CARTESIAN_POINT('Ctrl Pts',(10.2991605329999,15.2,-2.66310471900002));
#186618=CARTESIAN_POINT('Ctrl Pts',(10.2991605329999,11.6,-2.66310471900002));
#186619=CARTESIAN_POINT('Ctrl Pts',(10.3013850909999,15.2,-2.66313593100001));
#186620=CARTESIAN_POINT('Ctrl Pts',(10.3013850909999,11.6,-2.66313593100001));
#186621=CARTESIAN_POINT('Ctrl Pts',(10.3036162999999,15.2,-2.66316526500002));
#186622=CARTESIAN_POINT('Ctrl Pts',(10.3036162999999,11.6,-2.66316526500002));
#186623=CARTESIAN_POINT('Ctrl Pts',(10.3058541459999,15.2,-2.66319271100001));
#186624=CARTESIAN_POINT('Ctrl Pts',(10.3058541459999,11.6,-2.66319271100001));
#186625=CARTESIAN_POINT('Ctrl Pts',(10.3080986159999,15.2,-2.66321825900001));
#186626=CARTESIAN_POINT('Ctrl Pts',(10.3080986159999,11.6,-2.66321825900001));
#186627=CARTESIAN_POINT('Ctrl Pts',(10.3103496959999,15.2,-2.66324189700001));
#186628=CARTESIAN_POINT('Ctrl Pts',(10.3103496959999,11.6,-2.66324189700002));
#186629=CARTESIAN_POINT('Ctrl Pts',(10.3126073739999,15.2,-2.66326361500001));
#186630=CARTESIAN_POINT('Ctrl Pts',(10.3126073739999,11.6,-2.66326361500001));
#186631=CARTESIAN_POINT('Ctrl Pts',(10.3148716349999,15.2,-2.66328340400001));
#186632=CARTESIAN_POINT('Ctrl Pts',(10.3148716349999,11.6,-2.66328340400001));
#186633=CARTESIAN_POINT('Ctrl Pts',(10.3171424659999,15.2,-2.66330125200001));
#186634=CARTESIAN_POINT('Ctrl Pts',(10.3171424659999,11.6,-2.66330125200001));
#186635=CARTESIAN_POINT('Ctrl Pts',(10.3194198549999,15.2,-2.66331714900002));
#186636=CARTESIAN_POINT('Ctrl Pts',(10.3194198549999,11.6,-2.66331714900002));
#186637=CARTESIAN_POINT('Ctrl Pts',(10.3217037879999,15.2,-2.66333108500001));
#186638=CARTESIAN_POINT('Ctrl Pts',(10.3217037879999,11.6,-2.66333108500001));
#186639=CARTESIAN_POINT('Ctrl Pts',(10.3239942509999,15.2,-2.66334305000001));
#186640=CARTESIAN_POINT('Ctrl Pts',(10.3239942509999,11.6,-2.66334305000001));
#186641=CARTESIAN_POINT('Ctrl Pts',(10.3262912319999,15.2,-2.66335303400002));
#186642=CARTESIAN_POINT('Ctrl Pts',(10.3262912319999,11.6,-2.66335303400002));
#186643=CARTESIAN_POINT('Ctrl Pts',(10.3285947179999,15.2,-2.66336102400002));
#186644=CARTESIAN_POINT('Ctrl Pts',(10.3285947179999,11.6,-2.66336102400002));
#186645=CARTESIAN_POINT('Ctrl Pts',(10.3309046949999,15.2,-2.66336701400002));
#186646=CARTESIAN_POINT('Ctrl Pts',(10.3309046949999,11.6,-2.66336701400002));
#186647=CARTESIAN_POINT('Ctrl Pts',(10.3332211489999,15.2,-2.66337099000001));
#186648=CARTESIAN_POINT('Ctrl Pts',(10.3332211489999,11.6,-2.66337099000001));
#186649=CARTESIAN_POINT('Ctrl Pts',(10.3355440699999,15.2,-2.66337294600001));
#186650=CARTESIAN_POINT('Ctrl Pts',(10.3355440699999,11.6,-2.66337294600001));
#186651=CARTESIAN_POINT('Ctrl Pts',(10.3378734419999,15.2,-2.66337286900002));
#186652=CARTESIAN_POINT('Ctrl Pts',(10.3378734419999,11.6,-2.66337286900002));
#186653=CARTESIAN_POINT('Ctrl Pts',(10.3402092539999,15.2,-2.66337074900001));
#186654=CARTESIAN_POINT('Ctrl Pts',(10.3402092539999,11.6,-2.66337074900001));
#186655=CARTESIAN_POINT('Ctrl Pts',(10.3425514919999,15.2,-2.66336657700001));
#186656=CARTESIAN_POINT('Ctrl Pts',(10.3425514919999,11.6,-2.66336657700002));
#186657=CARTESIAN_POINT('Ctrl Pts',(10.3449001429999,15.2,-2.66336034300001));
#186658=CARTESIAN_POINT('Ctrl Pts',(10.3449001429999,11.6,-2.66336034300001));
#186659=CARTESIAN_POINT('Ctrl Pts',(10.3472551949999,15.2,-2.66335203800002));
#186660=CARTESIAN_POINT('Ctrl Pts',(10.3472551949999,11.6,-2.66335203800002));
#186661=CARTESIAN_POINT('Ctrl Pts',(10.3496166339999,15.2,-2.66334165000002));
#186662=CARTESIAN_POINT('Ctrl Pts',(10.3496166339999,11.6,-2.66334165000002));
#186663=CARTESIAN_POINT('Ctrl Pts',(10.3519844489999,15.2,-2.66332917100002));
#186664=CARTESIAN_POINT('Ctrl Pts',(10.3519844489999,11.6,-2.66332917100002));
#186665=CARTESIAN_POINT('Ctrl Pts',(10.3543586239999,15.2,-2.66331459100002));
#186666=CARTESIAN_POINT('Ctrl Pts',(10.3543586239999,11.6,-2.66331459100002));
#186667=CARTESIAN_POINT('Ctrl Pts',(10.3567391499999,15.2,-2.66329790000002));
#186668=CARTESIAN_POINT('Ctrl Pts',(10.3567391499999,11.6,-2.66329790000002));
#186669=CARTESIAN_POINT('Ctrl Pts',(10.3591260109999,15.2,-2.66327908600001));
#186670=CARTESIAN_POINT('Ctrl Pts',(10.3591260109999,11.6,-2.66327908600001));
#186671=CARTESIAN_POINT('Ctrl Pts',(10.3615191969999,15.2,-2.66325814300002));
#186672=CARTESIAN_POINT('Ctrl Pts',(10.3615191969999,11.6,-2.66325814300002));
#186673=CARTESIAN_POINT('Ctrl Pts',(10.3639186939999,15.2,-2.66323506100001));
#186674=CARTESIAN_POINT('Ctrl Pts',(10.3639186939999,11.6,-2.66323506100001));
#186675=CARTESIAN_POINT('Ctrl Pts',(10.3663244889999,15.2,-2.66320982800002));
#186676=CARTESIAN_POINT('Ctrl Pts',(10.3663244889999,11.6,-2.66320982800002));
#186677=CARTESIAN_POINT('Ctrl Pts',(10.3687365709999,15.2,-2.66318243600002));
#186678=CARTESIAN_POINT('Ctrl Pts',(10.3687365709999,11.6,-2.66318243600002));
#186679=CARTESIAN_POINT('Ctrl Pts',(10.3711549249999,15.2,-2.66315287500001));
#186680=CARTESIAN_POINT('Ctrl Pts',(10.3711549249999,11.6,-2.66315287500001));
#186681=CARTESIAN_POINT('Ctrl Pts',(10.3735795409999,15.2,-2.66312113600002));
#186682=CARTESIAN_POINT('Ctrl Pts',(10.3735795409999,11.6,-2.66312113600002));
#186683=CARTESIAN_POINT('Ctrl Pts',(10.3760104039999,15.2,-2.66308720900001));
#186684=CARTESIAN_POINT('Ctrl Pts',(10.3760104039999,11.6,-2.66308720900002));
#186685=CARTESIAN_POINT('Ctrl Pts',(10.3784475029999,15.2,-2.66305108600001));
#186686=CARTESIAN_POINT('Ctrl Pts',(10.3784475029999,11.6,-2.66305108600001));
#186687=CARTESIAN_POINT('Ctrl Pts',(10.3808908259999,15.2,-2.66301275600001));
#186688=CARTESIAN_POINT('Ctrl Pts',(10.3808908259999,11.6,-2.66301275600001));
#186689=CARTESIAN_POINT('Ctrl Pts',(10.3833403579999,15.2,-2.66297221000002));
#186690=CARTESIAN_POINT('Ctrl Pts',(10.3833403579999,11.6,-2.66297221000002));
#186691=CARTESIAN_POINT('Ctrl Pts',(10.3857960899999,15.2,-2.66292943900002));
#186692=CARTESIAN_POINT('Ctrl Pts',(10.3857960899999,11.6,-2.66292943900002));
#186693=CARTESIAN_POINT('Ctrl Pts',(10.3882580069999,15.2,-2.66288443300001));
#186694=CARTESIAN_POINT('Ctrl Pts',(10.3882580069999,11.6,-2.66288443300001));
#186695=CARTESIAN_POINT('Ctrl Pts',(10.3907260989999,15.2,-2.66283718400001));
#186696=CARTESIAN_POINT('Ctrl Pts',(10.3907260989999,11.6,-2.66283718400001));
#186697=CARTESIAN_POINT('Ctrl Pts',(10.3932003519999,15.2,-2.66278768200001));
#186698=CARTESIAN_POINT('Ctrl Pts',(10.3932003519999,11.6,-2.66278768200001));
#186699=CARTESIAN_POINT('Ctrl Pts',(10.3956807539999,15.2,-2.66273591800001));
#186700=CARTESIAN_POINT('Ctrl Pts',(10.3956807539999,11.6,-2.66273591800001));
#186701=CARTESIAN_POINT('Ctrl Pts',(10.3981672919999,15.2,-2.66268188300002));
#186702=CARTESIAN_POINT('Ctrl Pts',(10.3981672919999,11.6,-2.66268188300002));
#186703=CARTESIAN_POINT('Ctrl Pts',(10.4006599549999,15.2,-2.66262556800001));
#186704=CARTESIAN_POINT('Ctrl Pts',(10.4006599549999,11.6,-2.66262556800001));
#186705=CARTESIAN_POINT('Ctrl Pts',(10.4031587299999,15.2,-2.66256696400001));
#186706=CARTESIAN_POINT('Ctrl Pts',(10.4031587299999,11.6,-2.66256696400002));
#186707=CARTESIAN_POINT('Ctrl Pts',(10.4056636059999,15.2,-2.66250606100002));
#186708=CARTESIAN_POINT('Ctrl Pts',(10.4056636059999,11.6,-2.66250606100002));
#186709=CARTESIAN_POINT('Ctrl Pts',(10.4081745689999,15.2,-2.66244285100001));
#186710=CARTESIAN_POINT('Ctrl Pts',(10.4081745689999,11.6,-2.66244285100001));
#186711=CARTESIAN_POINT('Ctrl Pts',(10.4106916089999,15.2,-2.66237732400001));
#186712=CARTESIAN_POINT('Ctrl Pts',(10.4106916089999,11.6,-2.66237732400001));
#186713=CARTESIAN_POINT('Ctrl Pts',(10.4132147119999,15.2,-2.66230947300001));
#186714=CARTESIAN_POINT('Ctrl Pts',(10.4132147119999,11.6,-2.66230947300001));
#186715=CARTESIAN_POINT('Ctrl Pts',(10.4157438659999,15.2,-2.66223928800001));
#186716=CARTESIAN_POINT('Ctrl Pts',(10.4157438659999,11.6,-2.66223928800001));
#186717=CARTESIAN_POINT('Ctrl Pts',(10.4182790609999,15.2,-2.66216675900001));
#186718=CARTESIAN_POINT('Ctrl Pts',(10.4182790609999,11.6,-2.66216675900001));
#186719=CARTESIAN_POINT('Ctrl Pts',(10.4208202819999,15.2,-2.66209187800001));
#186720=CARTESIAN_POINT('Ctrl Pts',(10.4208202819999,11.6,-2.66209187800001));
#186721=CARTESIAN_POINT('Ctrl Pts',(10.4233675199999,15.2,-2.66201463800002));
#186722=CARTESIAN_POINT('Ctrl Pts',(10.4233675199999,11.6,-2.66201463800002));
#186723=CARTESIAN_POINT('Ctrl Pts',(10.4259207609999,15.2,-2.66193502800002));
#186724=CARTESIAN_POINT('Ctrl Pts',(10.4259207609999,11.6,-2.66193502800002));
#186725=CARTESIAN_POINT('Ctrl Pts',(10.4284799939999,15.2,-2.66185304000001));
#186726=CARTESIAN_POINT('Ctrl Pts',(10.4284799939999,11.6,-2.66185304000001));
#186727=CARTESIAN_POINT('Ctrl Pts',(10.4310452059999,15.2,-2.66176866400002));
#186728=CARTESIAN_POINT('Ctrl Pts',(10.4310452059999,11.6,-2.66176866400002));
#186729=CARTESIAN_POINT('Ctrl Pts',(10.4336163859999,15.2,-2.66168189400001));
#186730=CARTESIAN_POINT('Ctrl Pts',(10.4336163859999,11.6,-2.66168189400001));
#186731=CARTESIAN_POINT('Ctrl Pts',(10.4361935219999,15.2,-2.66159272000001));
#186732=CARTESIAN_POINT('Ctrl Pts',(10.4361935219999,11.6,-2.66159272000001));
#186733=CARTESIAN_POINT('Ctrl Pts',(10.4387766019999,15.2,-2.66150113300001));
#186734=CARTESIAN_POINT('Ctrl Pts',(10.4387766019999,11.6,-2.66150113300002));
#186735=CARTESIAN_POINT('Ctrl Pts',(10.4413656149999,15.2,-2.66140712400002));
#186736=CARTESIAN_POINT('Ctrl Pts',(10.4413656149999,11.6,-2.66140712400002));
#186737=CARTESIAN_POINT('Ctrl Pts',(10.4439605469999,15.2,-2.66131068600002));
#186738=CARTESIAN_POINT('Ctrl Pts',(10.4439605469999,11.6,-2.66131068600002));
#186739=CARTESIAN_POINT('Ctrl Pts',(10.4465613889999,15.2,-2.66121180900001));
#186740=CARTESIAN_POINT('Ctrl Pts',(10.4465613889999,11.6,-2.66121180900001));
#186741=CARTESIAN_POINT('Ctrl Pts',(10.4491681279999,15.2,-2.66111048600001));
#186742=CARTESIAN_POINT('Ctrl Pts',(10.4491681279999,11.6,-2.66111048600001));
#186743=CARTESIAN_POINT('Ctrl Pts',(10.4517807519999,15.2,-2.66100670700002));
#186744=CARTESIAN_POINT('Ctrl Pts',(10.4517807519999,11.6,-2.66100670700002));
#186745=CARTESIAN_POINT('Ctrl Pts',(10.4543992489999,15.2,-2.66090046400001));
#186746=CARTESIAN_POINT('Ctrl Pts',(10.4543992489999,11.6,-2.66090046400001));
#186747=CARTESIAN_POINT('Ctrl Pts',(10.4570236089999,15.2,-2.66079175000002));
#186748=CARTESIAN_POINT('Ctrl Pts',(10.4570236089999,11.6,-2.66079175000002));
#186749=CARTESIAN_POINT('Ctrl Pts',(10.4596538179999,15.2,-2.66068055600002));
#186750=CARTESIAN_POINT('Ctrl Pts',(10.4596538179999,11.6,-2.66068055600002));
#186751=CARTESIAN_POINT('Ctrl Pts',(10.4622898669999,15.2,-2.66056687100001));
#186752=CARTESIAN_POINT('Ctrl Pts',(10.4622898669999,11.6,-2.66056687100001));
#186753=CARTESIAN_POINT('Ctrl Pts',(10.4649317429999,15.2,-2.66045069100001));
#186754=CARTESIAN_POINT('Ctrl Pts',(10.4649317429999,11.6,-2.66045069100001));
#186755=CARTESIAN_POINT('Ctrl Pts',(10.4675794329999,15.2,-2.66033200500001));
#186756=CARTESIAN_POINT('Ctrl Pts',(10.4675794329999,11.6,-2.66033200500001));
#186757=CARTESIAN_POINT('Ctrl Pts',(10.4702329269999,15.2,-2.66021080500002));
#186758=CARTESIAN_POINT('Ctrl Pts',(10.4702329269999,11.6,-2.66021080500002));
#186759=CARTESIAN_POINT('Ctrl Pts',(10.4728922149999,15.2,-2.66008708400001));
#186760=CARTESIAN_POINT('Ctrl Pts',(10.4728922149999,11.6,-2.66008708400001));
#186761=CARTESIAN_POINT('Ctrl Pts',(10.4755572819999,15.2,-2.65996083200001));
#186762=CARTESIAN_POINT('Ctrl Pts',(10.4755572819999,11.6,-2.65996083200001));
#186763=CARTESIAN_POINT('Ctrl Pts',(10.4782281199999,15.2,-2.65983204300001));
#186764=CARTESIAN_POINT('Ctrl Pts',(10.4782281199999,11.6,-2.65983204300001));
#186765=CARTESIAN_POINT('Ctrl Pts',(10.4809047149999,15.2,-2.65970070700002));
#186766=CARTESIAN_POINT('Ctrl Pts',(10.4809047149999,11.6,-2.65970070700002));
#186767=CARTESIAN_POINT('Ctrl Pts',(10.4835870569999,15.2,-2.65956681700001));
#186768=CARTESIAN_POINT('Ctrl Pts',(10.4835870569999,11.6,-2.65956681700001));
#186769=CARTESIAN_POINT('Ctrl Pts',(10.4862751339999,15.2,-2.65943036500001));
#186770=CARTESIAN_POINT('Ctrl Pts',(10.4862751339999,11.6,-2.65943036500001));
#186771=CARTESIAN_POINT('Ctrl Pts',(10.4889689349999,15.2,-2.65929134100002));
#186772=CARTESIAN_POINT('Ctrl Pts',(10.4889689349999,11.6,-2.65929134100002));
#186773=CARTESIAN_POINT('Ctrl Pts',(10.4916684479999,15.2,-2.65914974000002));
#186774=CARTESIAN_POINT('Ctrl Pts',(10.4916684479999,11.6,-2.65914974000002));
#186775=CARTESIAN_POINT('Ctrl Pts',(10.4943736619999,15.2,-2.65900555300002));
#186776=CARTESIAN_POINT('Ctrl Pts',(10.4943736619999,11.6,-2.65900555300002));
#186777=CARTESIAN_POINT('Ctrl Pts',(10.4970845659999,15.2,-2.65885877000001));
#186778=CARTESIAN_POINT('Ctrl Pts',(10.4970845659999,11.6,-2.65885877000001));
#186779=CARTESIAN_POINT('Ctrl Pts',(10.4998011489999,15.2,-2.65870938600001));
#186780=CARTESIAN_POINT('Ctrl Pts',(10.4998011489999,11.6,-2.65870938600001));
#186781=CARTESIAN_POINT('Ctrl Pts',(10.5025233979999,15.2,-2.65855739100001));
#186782=CARTESIAN_POINT('Ctrl Pts',(10.5025233979999,11.6,-2.65855739100001));
#186783=CARTESIAN_POINT('Ctrl Pts',(10.5052513029999,15.2,-2.65840277900002));
#186784=CARTESIAN_POINT('Ctrl Pts',(10.5052513029999,11.6,-2.65840277900002));
#186785=CARTESIAN_POINT('Ctrl Pts',(10.5079848529999,15.2,-2.65824554000002));
#186786=CARTESIAN_POINT('Ctrl Pts',(10.5079848529999,11.6,-2.65824554000002));
#186787=CARTESIAN_POINT('Ctrl Pts',(10.5107240369999,15.2,-2.65808566900001));
#186788=CARTESIAN_POINT('Ctrl Pts',(10.5107240369999,11.6,-2.65808566900001));
#186789=CARTESIAN_POINT('Ctrl Pts',(10.5134688429999,15.2,-2.65792315500001));
#186790=CARTESIAN_POINT('Ctrl Pts',(10.5134688429999,11.6,-2.65792315500002));
#186791=CARTESIAN_POINT('Ctrl Pts',(10.5162192599999,15.2,-2.65775799100001));
#186792=CARTESIAN_POINT('Ctrl Pts',(10.5162192599999,11.6,-2.65775799100001));
#186793=CARTESIAN_POINT('Ctrl Pts',(10.5189752759999,15.2,-2.65759017200002));
#186794=CARTESIAN_POINT('Ctrl Pts',(10.5189752759999,11.6,-2.65759017200002));
#186795=CARTESIAN_POINT('Ctrl Pts',(10.5217368829999,15.2,-2.65741968800001));
#186796=CARTESIAN_POINT('Ctrl Pts',(10.5217368829999,11.6,-2.65741968800001));
#186797=CARTESIAN_POINT('Ctrl Pts',(10.5245040669999,15.2,-2.65724653000001));
#186798=CARTESIAN_POINT('Ctrl Pts',(10.5245040669999,11.6,-2.65724653000001));
#186799=CARTESIAN_POINT('Ctrl Pts',(10.5272768169999,15.2,-2.65707069400001));
#186800=CARTESIAN_POINT('Ctrl Pts',(10.5272768169999,11.6,-2.65707069400001));
#186801=CARTESIAN_POINT('Ctrl Pts',(10.5300551229999,15.2,-2.65689217000002));
#186802=CARTESIAN_POINT('Ctrl Pts',(10.5300551229999,11.6,-2.65689217000002));
#186803=CARTESIAN_POINT('Ctrl Pts',(10.5328389739999,15.2,-2.65671095100001));
#186804=CARTESIAN_POINT('Ctrl Pts',(10.5328389739999,11.6,-2.65671095100001));
#186805=CARTESIAN_POINT('Ctrl Pts',(10.5356283589999,15.2,-2.65652702800002));
#186806=CARTESIAN_POINT('Ctrl Pts',(10.5356283589999,11.6,-2.65652702800002));
#186807=CARTESIAN_POINT('Ctrl Pts',(10.5384232659999,15.2,-2.65634039600001));
#186808=CARTESIAN_POINT('Ctrl Pts',(10.5384232659999,11.6,-2.65634039600001));
#186809=CARTESIAN_POINT('Ctrl Pts',(10.5412236849999,15.2,-2.65615104500001));
#186810=CARTESIAN_POINT('Ctrl Pts',(10.5412236849999,11.6,-2.65615104500002));
#186811=CARTESIAN_POINT('Ctrl Pts',(10.5440296059999,15.2,-2.65595897000001));
#186812=CARTESIAN_POINT('Ctrl Pts',(10.5440296059999,11.6,-2.65595897000001));
#186813=CARTESIAN_POINT('Ctrl Pts',(10.5468410149999,15.2,-2.65576416200001));
#186814=CARTESIAN_POINT('Ctrl Pts',(10.5468410149999,11.6,-2.65576416200001));
#186815=CARTESIAN_POINT('Ctrl Pts',(10.5496579039999,15.2,-2.65556661400002));
#186816=CARTESIAN_POINT('Ctrl Pts',(10.5496579039999,11.6,-2.65556661400002));
#186817=CARTESIAN_POINT('Ctrl Pts',(10.5524802599999,15.2,-2.65536631800002));
#186818=CARTESIAN_POINT('Ctrl Pts',(10.5524802599999,11.6,-2.65536631800002));
#186819=CARTESIAN_POINT('Ctrl Pts',(10.5553080749999,15.2,-2.65516326700002));
#186820=CARTESIAN_POINT('Ctrl Pts',(10.5553080749999,11.6,-2.65516326700002));
#186821=CARTESIAN_POINT('Ctrl Pts',(10.5581413349999,15.2,-2.65495745500001));
#186822=CARTESIAN_POINT('Ctrl Pts',(10.5581413349999,11.6,-2.65495745500001));
#186823=CARTESIAN_POINT('Ctrl Pts',(10.5609800309999,15.2,-2.65474887200002));
#186824=CARTESIAN_POINT('Ctrl Pts',(10.5609800309999,11.6,-2.65474887200002));
#186825=CARTESIAN_POINT('Ctrl Pts',(10.5638241519999,15.2,-2.65453751200001));
#186826=CARTESIAN_POINT('Ctrl Pts',(10.5638241519999,11.6,-2.65453751200001));
#186827=CARTESIAN_POINT('Ctrl Pts',(10.5666736869999,15.2,-2.65432336900002));
#186828=CARTESIAN_POINT('Ctrl Pts',(10.5666736869999,11.6,-2.65432336900002));
#186829=CARTESIAN_POINT('Ctrl Pts',(10.5695286259999,15.2,-2.65410643300001));
#186830=CARTESIAN_POINT('Ctrl Pts',(10.5695286259999,11.6,-2.65410643300001));
#186831=CARTESIAN_POINT('Ctrl Pts',(10.5723889559999,15.2,-2.65388670000001));
#186832=CARTESIAN_POINT('Ctrl Pts',(10.5723889559999,11.6,-2.65388670000001));
#186833=CARTESIAN_POINT('Ctrl Pts',(10.5752546689999,15.2,-2.65366416100001));
#186834=CARTESIAN_POINT('Ctrl Pts',(10.5752546689999,11.6,-2.65366416100001));
#186835=CARTESIAN_POINT('Ctrl Pts',(10.5781257519999,15.2,-2.65343880800001));
#186836=CARTESIAN_POINT('Ctrl Pts',(10.5781257519999,11.6,-2.65343880800002));
#186837=CARTESIAN_POINT('Ctrl Pts',(10.5810021969999,15.2,-2.65321063600001));
#186838=CARTESIAN_POINT('Ctrl Pts',(10.5810021969999,11.6,-2.65321063600001));
#186839=CARTESIAN_POINT('Ctrl Pts',(10.5838839899999,15.2,-2.65297963500001));
#186840=CARTESIAN_POINT('Ctrl Pts',(10.5838839899999,11.6,-2.65297963500001));
#186841=CARTESIAN_POINT('Ctrl Pts',(10.5867711239999,15.2,-2.65274580100002));
#186842=CARTESIAN_POINT('Ctrl Pts',(10.5867711239999,11.6,-2.65274580100002));
#186843=CARTESIAN_POINT('Ctrl Pts',(10.5896635859999,15.2,-2.65250912500001));
#186844=CARTESIAN_POINT('Ctrl Pts',(10.5896635859999,11.6,-2.65250912500001));
#186845=CARTESIAN_POINT('Ctrl Pts',(10.5925613649999,15.2,-2.65226960100001));
#186846=CARTESIAN_POINT('Ctrl Pts',(10.5925613649999,11.6,-2.65226960100002));
#186847=CARTESIAN_POINT('Ctrl Pts',(10.5954644519999,15.2,-2.65202722100002));
#186848=CARTESIAN_POINT('Ctrl Pts',(10.5954644519999,11.6,-2.65202722100002));
#186849=CARTESIAN_POINT('Ctrl Pts',(10.5983728359999,15.2,-2.65178197900001));
#186850=CARTESIAN_POINT('Ctrl Pts',(10.5983728359999,11.6,-2.65178197900001));
#186851=CARTESIAN_POINT('Ctrl Pts',(10.6012865059999,15.2,-2.65153386700002));
#186852=CARTESIAN_POINT('Ctrl Pts',(10.6012865059999,11.6,-2.65153386700002));
#186853=CARTESIAN_POINT('Ctrl Pts',(10.6042054519999,15.2,-2.65128287800001));
#186854=CARTESIAN_POINT('Ctrl Pts',(10.6042054519999,11.6,-2.65128287800001));
#186855=CARTESIAN_POINT('Ctrl Pts',(10.6071296629999,15.2,-2.65102900700001));
#186856=CARTESIAN_POINT('Ctrl Pts',(10.6071296629999,11.6,-2.65102900700001));
#186857=CARTESIAN_POINT('Ctrl Pts',(10.6100591289999,15.2,-2.65077224400001));
#186858=CARTESIAN_POINT('Ctrl Pts',(10.6100591289999,11.6,-2.65077224400002));
#186859=CARTESIAN_POINT('Ctrl Pts',(10.6129938389999,15.2,-2.65051258500002));
#186860=CARTESIAN_POINT('Ctrl Pts',(10.6129938389999,11.6,-2.65051258500002));
#186861=CARTESIAN_POINT('Ctrl Pts',(10.6159337839999,15.2,-2.65025002200002));
#186862=CARTESIAN_POINT('Ctrl Pts',(10.6159337839999,11.6,-2.65025002200002));
#186863=CARTESIAN_POINT('Ctrl Pts',(10.6188789509999,15.2,-2.64998454800002));
#186864=CARTESIAN_POINT('Ctrl Pts',(10.6188789509999,11.6,-2.64998454800002));
#186865=CARTESIAN_POINT('Ctrl Pts',(10.6218293329999,15.2,-2.64971615600002));
#186866=CARTESIAN_POINT('Ctrl Pts',(10.6218293329999,11.6,-2.64971615600002));
#186867=CARTESIAN_POINT('Ctrl Pts',(10.6247849159999,15.2,-2.64944484000001));
#186868=CARTESIAN_POINT('Ctrl Pts',(10.6247849159999,11.6,-2.64944484000001));
#186869=CARTESIAN_POINT('Ctrl Pts',(10.6277456919999,15.2,-2.64917059200001));
#186870=CARTESIAN_POINT('Ctrl Pts',(10.6277456919999,11.6,-2.64917059200001));
#186871=CARTESIAN_POINT('Ctrl Pts',(10.6307116499999,15.2,-2.64889340600002));
#186872=CARTESIAN_POINT('Ctrl Pts',(10.6307116499999,11.6,-2.64889340600002));
#186873=CARTESIAN_POINT('Ctrl Pts',(10.6336827789999,15.2,-2.64861327700002));
#186874=CARTESIAN_POINT('Ctrl Pts',(10.6336827789999,11.6,-2.64861327700002));
#186875=CARTESIAN_POINT('Ctrl Pts',(10.6366590699999,15.2,-2.64833019500001));
#186876=CARTESIAN_POINT('Ctrl Pts',(10.6366590699999,11.6,-2.64833019500002));
#186877=CARTESIAN_POINT('Ctrl Pts',(10.6396405129999,15.2,-2.64804415600001));
#186878=CARTESIAN_POINT('Ctrl Pts',(10.6396405129999,11.6,-2.64804415600001));
#186879=CARTESIAN_POINT('Ctrl Pts',(10.6426270949999,15.2,-2.64775515100002));
#186880=CARTESIAN_POINT('Ctrl Pts',(10.6426270949999,11.6,-2.64775515100002));
#186881=CARTESIAN_POINT('Ctrl Pts',(10.6456188079999,15.2,-2.64746317600002));
#186882=CARTESIAN_POINT('Ctrl Pts',(10.6456188079999,11.6,-2.64746317600002));
#186883=CARTESIAN_POINT('Ctrl Pts',(10.6486156409999,15.2,-2.64716822200001));
#186884=CARTESIAN_POINT('Ctrl Pts',(10.6486156409999,11.6,-2.64716822200001));
#186885=CARTESIAN_POINT('Ctrl Pts',(10.6516175849999,15.2,-2.64687028400001));
#186886=CARTESIAN_POINT('Ctrl Pts',(10.6516175849999,11.6,-2.64687028400001));
#186887=CARTESIAN_POINT('Ctrl Pts',(10.6546246289999,15.2,-2.64656935600001));
#186888=CARTESIAN_POINT('Ctrl Pts',(10.6546246289999,11.6,-2.64656935600002));
#186889=CARTESIAN_POINT('Ctrl Pts',(10.6576367619999,15.2,-2.64626542900002));
#186890=CARTESIAN_POINT('Ctrl Pts',(10.6576367619999,11.6,-2.64626542900002));
#186891=CARTESIAN_POINT('Ctrl Pts',(10.6606539749999,15.2,-2.64595849900001));
#186892=CARTESIAN_POINT('Ctrl Pts',(10.6606539749999,11.6,-2.64595849900001));
#186893=CARTESIAN_POINT('Ctrl Pts',(10.6636762569999,15.2,-2.64564855800002));
#186894=CARTESIAN_POINT('Ctrl Pts',(10.6636762569999,11.6,-2.64564855800002));
#186895=CARTESIAN_POINT('Ctrl Pts',(10.6667035989999,15.2,-2.64533559900002));
#186896=CARTESIAN_POINT('Ctrl Pts',(10.6667035989999,11.6,-2.64533559900002));
#186897=CARTESIAN_POINT('Ctrl Pts',(10.6697359889999,15.2,-2.64501961700002));
#186898=CARTESIAN_POINT('Ctrl Pts',(10.6697359889999,11.6,-2.64501961700002));
#186899=CARTESIAN_POINT('Ctrl Pts',(10.6727734179999,15.2,-2.64470060600001));
#186900=CARTESIAN_POINT('Ctrl Pts',(10.6727734179999,11.6,-2.64470060600001));
#186901=CARTESIAN_POINT('Ctrl Pts',(10.6758158769999,15.2,-2.64437855800002));
#186902=CARTESIAN_POINT('Ctrl Pts',(10.6758158769999,11.6,-2.64437855800002));
#186903=CARTESIAN_POINT('Ctrl Pts',(10.6788633539999,15.2,-2.64405346800002));
#186904=CARTESIAN_POINT('Ctrl Pts',(10.6788633539999,11.6,-2.64405346800002));
#186905=CARTESIAN_POINT('Ctrl Pts',(10.6819158399999,15.2,-2.64372532800001));
#186906=CARTESIAN_POINT('Ctrl Pts',(10.6819158399999,11.6,-2.64372532800001));
#186907=CARTESIAN_POINT('Ctrl Pts',(10.6849733239999,15.2,-2.64339413300001));
#186908=CARTESIAN_POINT('Ctrl Pts',(10.6849733239999,11.6,-2.64339413300001));
#186909=CARTESIAN_POINT('Ctrl Pts',(10.6880357989999,15.2,-2.64305987600002));
#186910=CARTESIAN_POINT('Ctrl Pts',(10.6880357989999,11.6,-2.64305987600002));
#186911=CARTESIAN_POINT('Ctrl Pts',(10.6911032509999,15.2,-2.64272255200002));
#186912=CARTESIAN_POINT('Ctrl Pts',(10.6911032509999,11.6,-2.64272255200002));
#186913=CARTESIAN_POINT('Ctrl Pts',(10.6941756719999,15.2,-2.64238215300002));
#186914=CARTESIAN_POINT('Ctrl Pts',(10.6941756719999,11.6,-2.64238215300002));
#186915=CARTESIAN_POINT('Ctrl Pts',(10.6972530529999,15.2,-2.64203867300001));
#186916=CARTESIAN_POINT('Ctrl Pts',(10.6972530529999,11.6,-2.64203867300001));
#186917=CARTESIAN_POINT('Ctrl Pts',(10.7003353819999,15.2,-2.64169210700001));
#186918=CARTESIAN_POINT('Ctrl Pts',(10.7003353819999,11.6,-2.64169210700001));
#186919=CARTESIAN_POINT('Ctrl Pts',(10.7034226499999,15.2,-2.64134244800001));
#186920=CARTESIAN_POINT('Ctrl Pts',(10.7034226499999,11.6,-2.64134244800002));
#186921=CARTESIAN_POINT('Ctrl Pts',(10.7065148479999,15.2,-2.64098969000001));
#186922=CARTESIAN_POINT('Ctrl Pts',(10.7065148479999,11.6,-2.64098969000001));
#186923=CARTESIAN_POINT('Ctrl Pts',(10.7096119649999,15.2,-2.64063382700002));
#186924=CARTESIAN_POINT('Ctrl Pts',(10.7096119649999,11.6,-2.64063382700002));
#186925=CARTESIAN_POINT('Ctrl Pts',(10.7127139909999,15.2,-2.64027485300002));
#186926=CARTESIAN_POINT('Ctrl Pts',(10.7127139909999,11.6,-2.64027485300002));
#186927=CARTESIAN_POINT('Ctrl Pts',(10.7158209159999,15.2,-2.63991276000001));
#186928=CARTESIAN_POINT('Ctrl Pts',(10.7158209159999,11.6,-2.63991276000001));
#186929=CARTESIAN_POINT('Ctrl Pts',(10.7189327309999,15.2,-2.63954754400002));
#186930=CARTESIAN_POINT('Ctrl Pts',(10.7189327309999,11.6,-2.63954754400002));
#186931=CARTESIAN_POINT('Ctrl Pts',(10.7220494259999,15.2,-2.63917919900001));
#186932=CARTESIAN_POINT('Ctrl Pts',(10.7220494259999,11.6,-2.63917919900001));
#186933=CARTESIAN_POINT('Ctrl Pts',(10.7251709909999,15.2,-2.63880771700002));
#186934=CARTESIAN_POINT('Ctrl Pts',(10.7251709909999,11.6,-2.63880771700002));
#186935=CARTESIAN_POINT('Ctrl Pts',(10.7282974159999,15.2,-2.63843309400002));
#186936=CARTESIAN_POINT('Ctrl Pts',(10.7282974159999,11.6,-2.63843309400002));
#186937=CARTESIAN_POINT('Ctrl Pts',(10.7314286909999,15.2,-2.63805532300001));
#186938=CARTESIAN_POINT('Ctrl Pts',(10.7314286909999,11.6,-2.63805532300002));
#186939=CARTESIAN_POINT('Ctrl Pts',(10.7345648079999,15.2,-2.63767439800001));
#186940=CARTESIAN_POINT('Ctrl Pts',(10.7345648079999,11.6,-2.63767439800001));
#186941=CARTESIAN_POINT('Ctrl Pts',(10.7377057549999,15.2,-2.63729031300001));
#186942=CARTESIAN_POINT('Ctrl Pts',(10.7377057549999,11.6,-2.63729031300001));
#186943=CARTESIAN_POINT('Ctrl Pts',(10.7408515229999,15.2,-2.63690306300001));
#186944=CARTESIAN_POINT('Ctrl Pts',(10.7408515229999,11.6,-2.63690306300001));
#186945=CARTESIAN_POINT('Ctrl Pts',(10.7440021029999,15.2,-2.63651264000002));
#186946=CARTESIAN_POINT('Ctrl Pts',(10.7440021029999,11.6,-2.63651264000002));
#186947=CARTESIAN_POINT('Ctrl Pts',(10.7471574849999,15.2,-2.63611904100001));
#186948=CARTESIAN_POINT('Ctrl Pts',(10.7471574849999,11.6,-2.63611904100001));
#186949=CARTESIAN_POINT('Ctrl Pts',(10.7503176589999,15.2,-2.63572225700001));
#186950=CARTESIAN_POINT('Ctrl Pts',(10.7503176589999,11.6,-2.63572225700001));
#186951=CARTESIAN_POINT('Ctrl Pts',(10.7534826149999,15.2,-2.63532228500001));
#186952=CARTESIAN_POINT('Ctrl Pts',(10.7534826149999,11.6,-2.63532228500001));
#186953=CARTESIAN_POINT('Ctrl Pts',(10.7566523439999,15.2,-2.63491911700001));
#186954=CARTESIAN_POINT('Ctrl Pts',(10.7566523439999,11.6,-2.63491911700001));
#186955=CARTESIAN_POINT('Ctrl Pts',(10.7598268359999,15.2,-2.63451274700001));
#186956=CARTESIAN_POINT('Ctrl Pts',(10.7598268359999,11.6,-2.63451274700001));
#186957=CARTESIAN_POINT('Ctrl Pts',(10.7630060819999,15.2,-2.63410317200002));
#186958=CARTESIAN_POINT('Ctrl Pts',(10.7630060819999,11.6,-2.63410317200002));
#186959=CARTESIAN_POINT('Ctrl Pts',(10.7661900709999,15.2,-2.63369038300001));
#186960=CARTESIAN_POINT('Ctrl Pts',(10.7661900709999,11.6,-2.63369038300001));
#186961=CARTESIAN_POINT('Ctrl Pts',(10.7693787949999,15.2,-2.63327437600001));
#186962=CARTESIAN_POINT('Ctrl Pts',(10.7693787949999,11.6,-2.63327437600001));
#186963=CARTESIAN_POINT('Ctrl Pts',(10.7725722439999,15.2,-2.63285514400001));
#186964=CARTESIAN_POINT('Ctrl Pts',(10.7725722439999,11.6,-2.63285514400002));
#186965=CARTESIAN_POINT('Ctrl Pts',(10.7757704079999,15.2,-2.63243268200001));
#186966=CARTESIAN_POINT('Ctrl Pts',(10.7757704079999,11.6,-2.63243268200001));
#186967=CARTESIAN_POINT('Ctrl Pts',(10.7789732769999,15.2,-2.63200698600001));
#186968=CARTESIAN_POINT('Ctrl Pts',(10.7789732769999,11.6,-2.63200698600001));
#186969=CARTESIAN_POINT('Ctrl Pts',(10.7821808439999,15.2,-2.63157804700001));
#186970=CARTESIAN_POINT('Ctrl Pts',(10.7821808439999,11.6,-2.63157804700001));
#186971=CARTESIAN_POINT('Ctrl Pts',(10.7853930959999,15.2,-2.63114586100002));
#186972=CARTESIAN_POINT('Ctrl Pts',(10.7853930959999,11.6,-2.63114586100002));
#186973=CARTESIAN_POINT('Ctrl Pts',(10.7886100249999,15.2,-2.63071042400002));
#186974=CARTESIAN_POINT('Ctrl Pts',(10.7886100249999,11.6,-2.63071042400002));
#186975=CARTESIAN_POINT('Ctrl Pts',(10.7918316229999,15.2,-2.63027172700002));
#186976=CARTESIAN_POINT('Ctrl Pts',(10.7918316229999,11.6,-2.63027172700002));
#186977=CARTESIAN_POINT('Ctrl Pts',(10.7950578779999,15.2,-2.62982976600002));
#186978=CARTESIAN_POINT('Ctrl Pts',(10.7950578779999,11.6,-2.62982976600002));
#186979=CARTESIAN_POINT('Ctrl Pts',(10.7982887819999,15.2,-2.62938453500002));
#186980=CARTESIAN_POINT('Ctrl Pts',(10.7982887819999,11.6,-2.62938453500002));
#186981=CARTESIAN_POINT('Ctrl Pts',(10.8015243249999,15.2,-2.62893603000002));
#186982=CARTESIAN_POINT('Ctrl Pts',(10.8015243249999,11.6,-2.62893603000002));
#186983=CARTESIAN_POINT('Ctrl Pts',(10.8047644979999,15.2,-2.62848424300001));
#186984=CARTESIAN_POINT('Ctrl Pts',(10.8047644979999,11.6,-2.62848424300001));
#186985=CARTESIAN_POINT('Ctrl Pts',(10.8080092919999,15.2,-2.62802917000001));
#186986=CARTESIAN_POINT('Ctrl Pts',(10.8080092919999,11.6,-2.62802917000002));
#186987=CARTESIAN_POINT('Ctrl Pts',(10.8112586969999,15.2,-2.62757080500001));
#186988=CARTESIAN_POINT('Ctrl Pts',(10.8112586969999,11.6,-2.62757080500002));
#186989=CARTESIAN_POINT('Ctrl Pts',(10.8145127039999,15.2,-2.62710914400001));
#186990=CARTESIAN_POINT('Ctrl Pts',(10.8145127039999,11.6,-2.62710914400001));
#186991=CARTESIAN_POINT('Ctrl Pts',(10.8177713029999,15.2,-2.62664417900002));
#186992=CARTESIAN_POINT('Ctrl Pts',(10.8177713029999,11.6,-2.62664417900002));
#186993=CARTESIAN_POINT('Ctrl Pts',(10.8210344849999,15.2,-2.62617590500001));
#186994=CARTESIAN_POINT('Ctrl Pts',(10.8210344849999,11.6,-2.62617590500001));
#186995=CARTESIAN_POINT('Ctrl Pts',(10.8243022389999,15.2,-2.62570431800001));
#186996=CARTESIAN_POINT('Ctrl Pts',(10.8243022389999,11.6,-2.62570431800001));
#186997=CARTESIAN_POINT('Ctrl Pts',(10.8275745599999,15.2,-2.62522941200002));
#186998=CARTESIAN_POINT('Ctrl Pts',(10.8275745599999,11.6,-2.62522941200002));
#186999=CARTESIAN_POINT('Ctrl Pts',(10.8308514339999,15.2,-2.62475118200001));
#187000=CARTESIAN_POINT('Ctrl Pts',(10.8308514339999,11.6,-2.62475118200001));
#187001=CARTESIAN_POINT('Ctrl Pts',(10.8341328539999,15.2,-2.62426962100001));
#187002=CARTESIAN_POINT('Ctrl Pts',(10.8341328539999,11.6,-2.62426962100002));
#187003=CARTESIAN_POINT('Ctrl Pts',(10.8374188119999,15.2,-2.62378472500002));
#187004=CARTESIAN_POINT('Ctrl Pts',(10.8374188119999,11.6,-2.62378472500002));
#187005=CARTESIAN_POINT('Ctrl Pts',(10.8407092959999,15.2,-2.62329648600002));
#187006=CARTESIAN_POINT('Ctrl Pts',(10.8407092959999,11.6,-2.62329648600002));
#187007=CARTESIAN_POINT('Ctrl Pts',(10.8440042969999,15.2,-2.62280490300002));
#187008=CARTESIAN_POINT('Ctrl Pts',(10.8440042969999,11.6,-2.62280490300002));
#187009=CARTESIAN_POINT('Ctrl Pts',(10.8473038089999,15.2,-2.62230996900001));
#187010=CARTESIAN_POINT('Ctrl Pts',(10.8473038089999,11.6,-2.62230996900001));
#187011=CARTESIAN_POINT('Ctrl Pts',(10.8506078189999,15.2,-2.62181167700001));
#187012=CARTESIAN_POINT('Ctrl Pts',(10.8506078189999,11.6,-2.62181167700001));
#187013=CARTESIAN_POINT('Ctrl Pts',(10.8539163189999,15.2,-2.62131002300002));
#187014=CARTESIAN_POINT('Ctrl Pts',(10.8539163189999,11.6,-2.62131002300002));
#187015=CARTESIAN_POINT('Ctrl Pts',(10.8572292999999,15.2,-2.62080500200002));
#187016=CARTESIAN_POINT('Ctrl Pts',(10.8572292999999,11.6,-2.62080500200002));
#187017=CARTESIAN_POINT('Ctrl Pts',(10.8605467539999,15.2,-2.62029660800001));
#187018=CARTESIAN_POINT('Ctrl Pts',(10.8605467539999,11.6,-2.62029660800001));
#187019=CARTESIAN_POINT('Ctrl Pts',(10.8638686699999,15.2,-2.61978483700001));
#187020=CARTESIAN_POINT('Ctrl Pts',(10.8638686699999,11.6,-2.61978483700001));
#187021=CARTESIAN_POINT('Ctrl Pts',(10.8671950389999,15.2,-2.61926968300001));
#187022=CARTESIAN_POINT('Ctrl Pts',(10.8671950389999,11.6,-2.61926968300001));
#187023=CARTESIAN_POINT('Ctrl Pts',(10.8705258539999,15.2,-2.61875113900001));
#187024=CARTESIAN_POINT('Ctrl Pts',(10.8705258539999,11.6,-2.61875113900001));
#187025=CARTESIAN_POINT('Ctrl Pts',(10.8738611029999,15.2,-2.61822920300002));
#187026=CARTESIAN_POINT('Ctrl Pts',(10.8738611029999,11.6,-2.61822920300002));
#187027=CARTESIAN_POINT('Ctrl Pts',(10.8772007789999,15.2,-2.61770386800002));
#187028=CARTESIAN_POINT('Ctrl Pts',(10.8772007789999,11.6,-2.61770386800002));
#187029=CARTESIAN_POINT('Ctrl Pts',(10.8805448709999,15.2,-2.61717512900002));
#187030=CARTESIAN_POINT('Ctrl Pts',(10.8805448709999,11.6,-2.61717512900002));
#187031=CARTESIAN_POINT('Ctrl Pts',(10.8838933719999,15.2,-2.61664298100001));
#187032=CARTESIAN_POINT('Ctrl Pts',(10.8838933719999,11.6,-2.61664298100001));
#187033=CARTESIAN_POINT('Ctrl Pts',(10.8872462719999,15.2,-2.61610741800002));
#187034=CARTESIAN_POINT('Ctrl Pts',(10.8872462719999,11.6,-2.61610741800002));
#187035=CARTESIAN_POINT('Ctrl Pts',(10.8906035619999,15.2,-2.61556843700002));
#187036=CARTESIAN_POINT('Ctrl Pts',(10.8906035619999,11.6,-2.61556843700002));
#187037=CARTESIAN_POINT('Ctrl Pts',(10.8939652319999,15.2,-2.61502603200002));
#187038=CARTESIAN_POINT('Ctrl Pts',(10.8939652319999,11.6,-2.61502603200002));
#187039=CARTESIAN_POINT('Ctrl Pts',(10.8973312739999,15.2,-2.61448019700001));
#187040=CARTESIAN_POINT('Ctrl Pts',(10.8973312739999,11.6,-2.61448019700001));
#187041=CARTESIAN_POINT('Ctrl Pts',(10.9007016779999,15.2,-2.61393092800001));
#187042=CARTESIAN_POINT('Ctrl Pts',(10.9007016779999,11.6,-2.61393092800001));
#187043=CARTESIAN_POINT('Ctrl Pts',(10.9040764379999,15.2,-2.61337822000002));
#187044=CARTESIAN_POINT('Ctrl Pts',(10.9040764379999,11.6,-2.61337822000002));
#187045=CARTESIAN_POINT('Ctrl Pts',(10.9074555409999,15.2,-2.61282206600002));
#187046=CARTESIAN_POINT('Ctrl Pts',(10.9074555409999,11.6,-2.61282206600002));
#187047=CARTESIAN_POINT('Ctrl Pts',(10.9108389799999,15.2,-2.61226246400001));
#187048=CARTESIAN_POINT('Ctrl Pts',(10.9108389799999,11.6,-2.61226246400002));
#187049=CARTESIAN_POINT('Ctrl Pts',(10.9142267459999,15.2,-2.61169940700002));
#187050=CARTESIAN_POINT('Ctrl Pts',(10.9142267459999,11.6,-2.61169940700002));
#187051=CARTESIAN_POINT('Ctrl Pts',(10.9176188299999,15.2,-2.61113289100001));
#187052=CARTESIAN_POINT('Ctrl Pts',(10.9176188299999,11.6,-2.61113289100001));
#187053=CARTESIAN_POINT('Ctrl Pts',(10.9210152229999,15.2,-2.61056291100001));
#187054=CARTESIAN_POINT('Ctrl Pts',(10.9210152229999,11.6,-2.61056291100001));
#187055=CARTESIAN_POINT('Ctrl Pts',(10.9244159159999,15.2,-2.60998946000001));
#187056=CARTESIAN_POINT('Ctrl Pts',(10.9244159159999,11.6,-2.60998946000001));
#187057=CARTESIAN_POINT('Ctrl Pts',(10.9278208999999,15.2,-2.60941253700001));
#187058=CARTESIAN_POINT('Ctrl Pts',(10.9278208999999,11.6,-2.60941253700001));
#187059=CARTESIAN_POINT('Ctrl Pts',(10.9312301659999,15.2,-2.60883213400001));
#187060=CARTESIAN_POINT('Ctrl Pts',(10.9312301659999,11.6,-2.60883213400001));
#187061=CARTESIAN_POINT('Ctrl Pts',(10.9346437049999,15.2,-2.60824824600002));
#187062=CARTESIAN_POINT('Ctrl Pts',(10.9346437049999,11.6,-2.60824824600002));
#187063=CARTESIAN_POINT('Ctrl Pts',(10.9380615099999,15.2,-2.60766087000002));
#187064=CARTESIAN_POINT('Ctrl Pts',(10.9380615099999,11.6,-2.60766087000002));
#187065=CARTESIAN_POINT('Ctrl Pts',(10.9414835689999,15.2,-2.60707000100002));
#187066=CARTESIAN_POINT('Ctrl Pts',(10.9414835689999,11.6,-2.60707000100002));
#187067=CARTESIAN_POINT('Ctrl Pts',(10.9449098759999,15.2,-2.60647563300001));
#187068=CARTESIAN_POINT('Ctrl Pts',(10.9449098759999,11.6,-2.60647563300001));
#187069=CARTESIAN_POINT('Ctrl Pts',(10.9483404199999,15.2,-2.60587776100001));
#187070=CARTESIAN_POINT('Ctrl Pts',(10.9483404199999,11.6,-2.60587776100001));
#187071=CARTESIAN_POINT('Ctrl Pts',(10.9517751929999,15.2,-2.60527638200001));
#187072=CARTESIAN_POINT('Ctrl Pts',(10.9517751929999,11.6,-2.60527638200002));
#187073=CARTESIAN_POINT('Ctrl Pts',(10.9552141859999,15.2,-2.60467148900001));
#187074=CARTESIAN_POINT('Ctrl Pts',(10.9552141859999,11.6,-2.60467148900001));
#187075=CARTESIAN_POINT('Ctrl Pts',(10.9586573909999,15.2,-2.60406307900002));
#187076=CARTESIAN_POINT('Ctrl Pts',(10.9586573909999,11.6,-2.60406307900002));
#187077=CARTESIAN_POINT('Ctrl Pts',(10.9621047989999,15.2,-2.60345114600002));
#187078=CARTESIAN_POINT('Ctrl Pts',(10.9621047989999,11.6,-2.60345114600002));
#187079=CARTESIAN_POINT('Ctrl Pts',(10.9655563999999,15.2,-2.60283568600002));
#187080=CARTESIAN_POINT('Ctrl Pts',(10.9655563999999,11.6,-2.60283568600002));
#187081=CARTESIAN_POINT('Ctrl Pts',(10.9690121869999,15.2,-2.60221669400002));
#187082=CARTESIAN_POINT('Ctrl Pts',(10.9690121869999,11.6,-2.60221669400002));
#187083=CARTESIAN_POINT('Ctrl Pts',(10.9724721499999,15.2,-2.60159416500001));
#187084=CARTESIAN_POINT('Ctrl Pts',(10.9724721499999,11.6,-2.60159416500001));
#187085=CARTESIAN_POINT('Ctrl Pts',(10.9759362809999,15.2,-2.60096809500002));
#187086=CARTESIAN_POINT('Ctrl Pts',(10.9759362809999,11.6,-2.60096809500002));
#187087=CARTESIAN_POINT('Ctrl Pts',(10.9794045699999,15.2,-2.60033848000001));
#187088=CARTESIAN_POINT('Ctrl Pts',(10.9794045699999,11.6,-2.60033848000001));
#187089=CARTESIAN_POINT('Ctrl Pts',(10.9828770099999,15.2,-2.59970531200001));
#187090=CARTESIAN_POINT('Ctrl Pts',(10.9828770099999,11.6,-2.59970531200001));
#187091=CARTESIAN_POINT('Ctrl Pts',(10.9863535909999,15.2,-2.59906859100001));
#187092=CARTESIAN_POINT('Ctrl Pts',(10.9863535909999,11.6,-2.59906859100001));
#187093=CARTESIAN_POINT('Ctrl Pts',(10.9898343049999,15.2,-2.59842830900002));
#187094=CARTESIAN_POINT('Ctrl Pts',(10.9898343049999,11.6,-2.59842830900002));
#187095=CARTESIAN_POINT('Ctrl Pts',(10.9933191429999,15.2,-2.59778446200002));
#187096=CARTESIAN_POINT('Ctrl Pts',(10.9933191429999,11.6,-2.59778446200002));
#187097=CARTESIAN_POINT('Ctrl Pts',(10.9968080969999,15.2,-2.59713704600002));
#187098=CARTESIAN_POINT('Ctrl Pts',(10.9968080969999,11.6,-2.59713704600002));
#187099=CARTESIAN_POINT('Ctrl Pts',(11.0003011569999,15.2,-2.59648605600002));
#187100=CARTESIAN_POINT('Ctrl Pts',(11.0003011569999,11.6,-2.59648605600002));
#187101=CARTESIAN_POINT('Ctrl Pts',(11.0037983149999,15.2,-2.59583148900001));
#187102=CARTESIAN_POINT('Ctrl Pts',(11.0037983149999,11.6,-2.59583148900001));
#187103=CARTESIAN_POINT('Ctrl Pts',(11.0072995639999,15.2,-2.59517333800002));
#187104=CARTESIAN_POINT('Ctrl Pts',(11.0072995639999,11.6,-2.59517333800002));
#187105=CARTESIAN_POINT('Ctrl Pts',(11.0108048919999,15.2,-2.59451160000001));
#187106=CARTESIAN_POINT('Ctrl Pts',(11.0108048919999,11.6,-2.59451160000001));
#187107=CARTESIAN_POINT('Ctrl Pts',(11.0143142939999,15.2,-2.59384627000002));
#187108=CARTESIAN_POINT('Ctrl Pts',(11.0143142939999,11.6,-2.59384627000002));
#187109=CARTESIAN_POINT('Ctrl Pts',(11.0178277579999,15.2,-2.59317734300001));
#187110=CARTESIAN_POINT('Ctrl Pts',(11.0178277579999,11.6,-2.59317734300002));
#187111=CARTESIAN_POINT('Ctrl Pts',(11.0213452789999,15.2,-2.59250481600001));
#187112=CARTESIAN_POINT('Ctrl Pts',(11.0213452789999,11.6,-2.59250481600001));
#187113=CARTESIAN_POINT('Ctrl Pts',(11.0248668449999,15.2,-2.59182868300002));
#187114=CARTESIAN_POINT('Ctrl Pts',(11.0248668449999,11.6,-2.59182868300002));
#187115=CARTESIAN_POINT('Ctrl Pts',(11.0283924499999,15.2,-2.59114894000001));
#187116=CARTESIAN_POINT('Ctrl Pts',(11.0283924499999,11.6,-2.59114894000001));
#187117=CARTESIAN_POINT('Ctrl Pts',(11.0319220829999,15.2,-2.59046558300001));
#187118=CARTESIAN_POINT('Ctrl Pts',(11.0319220829999,11.6,-2.59046558300001));
#187119=CARTESIAN_POINT('Ctrl Pts',(11.0354557389999,15.2,-2.58977860600002));
#187120=CARTESIAN_POINT('Ctrl Pts',(11.0354557389999,11.6,-2.58977860600002));
#187121=CARTESIAN_POINT('Ctrl Pts',(11.0389934059999,15.2,-2.58908800800001));
#187122=CARTESIAN_POINT('Ctrl Pts',(11.0389934059999,11.6,-2.58908800800001));
#187123=CARTESIAN_POINT('Ctrl Pts',(11.0425350769999,15.2,-2.58839378100001));
#187124=CARTESIAN_POINT('Ctrl Pts',(11.0425350769999,11.6,-2.58839378100001));
#187125=CARTESIAN_POINT('Ctrl Pts',(11.0460807439999,15.2,-2.58769592200002));
#187126=CARTESIAN_POINT('Ctrl Pts',(11.0460807439999,11.6,-2.58769592200002));
#187127=CARTESIAN_POINT('Ctrl Pts',(11.0496303969999,15.2,-2.58699442700001));
#187128=CARTESIAN_POINT('Ctrl Pts',(11.0496303969999,11.6,-2.58699442700001));
#187129=CARTESIAN_POINT('Ctrl Pts',(11.0531840289999,15.2,-2.58628929200002));
#187130=CARTESIAN_POINT('Ctrl Pts',(11.0531840289999,11.6,-2.58628929200002));
#187131=CARTESIAN_POINT('Ctrl Pts',(11.0567416309999,15.2,-2.58558051000001));
#187132=CARTESIAN_POINT('Ctrl Pts',(11.0567416309999,11.6,-2.58558051000001));
#187133=CARTESIAN_POINT('Ctrl Pts',(11.0603031939999,15.2,-2.58486808000002));
#187134=CARTESIAN_POINT('Ctrl Pts',(11.0603031939999,11.6,-2.58486808000002));
#187135=CARTESIAN_POINT('Ctrl Pts',(11.0638687099999,15.2,-2.58415199700002));
#187136=CARTESIAN_POINT('Ctrl Pts',(11.0638687099999,11.6,-2.58415199700002));
#187137=CARTESIAN_POINT('Ctrl Pts',(11.0674381719999,15.2,-2.58343225400001));
#187138=CARTESIAN_POINT('Ctrl Pts',(11.0674381719999,11.6,-2.58343225400001));
#187139=CARTESIAN_POINT('Ctrl Pts',(11.0710115679999,15.2,-2.58270885000002));
#187140=CARTESIAN_POINT('Ctrl Pts',(11.0710115679999,11.6,-2.58270885000002));
#187141=CARTESIAN_POINT('Ctrl Pts',(11.0745888929999,15.2,-2.58198177900002));
#187142=CARTESIAN_POINT('Ctrl Pts',(11.0745888929999,11.6,-2.58198177900002));
#187143=CARTESIAN_POINT('Ctrl Pts',(11.0781701369999,15.2,-2.58125103800001));
#187144=CARTESIAN_POINT('Ctrl Pts',(11.0781701369999,11.6,-2.58125103800001));
#187145=CARTESIAN_POINT('Ctrl Pts',(11.0817552919999,15.2,-2.58051662100002));
#187146=CARTESIAN_POINT('Ctrl Pts',(11.0817552919999,11.6,-2.58051662100002));
#187147=CARTESIAN_POINT('Ctrl Pts',(11.0853443499999,15.2,-2.57977852500002));
#187148=CARTESIAN_POINT('Ctrl Pts',(11.0853443499999,11.6,-2.57977852500002));
#187149=CARTESIAN_POINT('Ctrl Pts',(11.0889373019999,15.2,-2.57903674500001));
#187150=CARTESIAN_POINT('Ctrl Pts',(11.0889373019999,11.6,-2.57903674500001));
#187151=CARTESIAN_POINT('Ctrl Pts',(11.0925341399999,15.2,-2.57829127800001));
#187152=CARTESIAN_POINT('Ctrl Pts',(11.0925341399999,11.6,-2.57829127800001));
#187153=CARTESIAN_POINT('Ctrl Pts',(11.0961348549999,15.2,-2.57754211900002));
#187154=CARTESIAN_POINT('Ctrl Pts',(11.0961348549999,11.6,-2.57754211900002));
#187155=CARTESIAN_POINT('Ctrl Pts',(11.0997394399999,15.2,-2.57678926400001));
#187156=CARTESIAN_POINT('Ctrl Pts',(11.0997394399999,11.6,-2.57678926400001));
#187157=CARTESIAN_POINT('Ctrl Pts',(11.1033478849999,15.2,-2.57603270800002));
#187158=CARTESIAN_POINT('Ctrl Pts',(11.1033478849999,11.6,-2.57603270800002));
#187159=CARTESIAN_POINT('Ctrl Pts',(11.1069601819999,15.2,-2.57527244800002));
#187160=CARTESIAN_POINT('Ctrl Pts',(11.1069601819999,11.6,-2.57527244800002));
#187161=CARTESIAN_POINT('Ctrl Pts',(11.1105763249999,15.2,-2.57450847900001));
#187162=CARTESIAN_POINT('Ctrl Pts',(11.1105763249999,11.6,-2.57450847900001));
#187163=CARTESIAN_POINT('Ctrl Pts',(11.1141963019999,15.2,-2.57374079800002));
#187164=CARTESIAN_POINT('Ctrl Pts',(11.1141963019999,11.6,-2.57374079800002));
#187165=CARTESIAN_POINT('Ctrl Pts',(11.1178201069999,15.2,-2.57296939900002));
#187166=CARTESIAN_POINT('Ctrl Pts',(11.1178201069999,11.6,-2.57296939900002));
#187167=CARTESIAN_POINT('Ctrl Pts',(11.1214477319999,15.2,-2.57219428100001));
#187168=CARTESIAN_POINT('Ctrl Pts',(11.1214477319999,11.6,-2.57219428100001));
#187169=CARTESIAN_POINT('Ctrl Pts',(11.1250791699999,15.2,-2.57141543700001));
#187170=CARTESIAN_POINT('Ctrl Pts',(11.1250791699999,11.6,-2.57141543700001));
#187171=CARTESIAN_POINT('Ctrl Pts',(11.1287144089999,15.2,-2.57063286400002));
#187172=CARTESIAN_POINT('Ctrl Pts',(11.1287144089999,11.6,-2.57063286400002));
#187173=CARTESIAN_POINT('Ctrl Pts',(11.1323534439999,15.2,-2.56984655900002));
#187174=CARTESIAN_POINT('Ctrl Pts',(11.1323534439999,11.6,-2.56984655900002));
#187175=CARTESIAN_POINT('Ctrl Pts',(11.1359962649999,15.2,-2.56905651800002));
#187176=CARTESIAN_POINT('Ctrl Pts',(11.1359962649999,11.6,-2.56905651800002));
#187177=CARTESIAN_POINT('Ctrl Pts',(11.1396428639999,15.2,-2.56826273300002));
#187178=CARTESIAN_POINT('Ctrl Pts',(11.1396428639999,11.6,-2.56826273300002));
#187179=CARTESIAN_POINT('Ctrl Pts',(11.1432932319999,15.2,-2.56746520500001));
#187180=CARTESIAN_POINT('Ctrl Pts',(11.1432932319999,11.6,-2.56746520500002));
#187181=CARTESIAN_POINT('Ctrl Pts',(11.1469473609999,15.2,-2.56666392500001));
#187182=CARTESIAN_POINT('Ctrl Pts',(11.1469473609999,11.6,-2.56666392500001));
#187183=CARTESIAN_POINT('Ctrl Pts',(11.1506052429999,15.2,-2.56585889300001));
#187184=CARTESIAN_POINT('Ctrl Pts',(11.1506052429999,11.6,-2.56585889300002));
#187185=CARTESIAN_POINT('Ctrl Pts',(11.1542668699999,15.2,-2.56505010300002));
#187186=CARTESIAN_POINT('Ctrl Pts',(11.1542668699999,11.6,-2.56505010300002));
#187187=CARTESIAN_POINT('Ctrl Pts',(11.1579322339999,15.2,-2.56423755300001));
#187188=CARTESIAN_POINT('Ctrl Pts',(11.1579322339999,11.6,-2.56423755300002));
#187189=CARTESIAN_POINT('Ctrl Pts',(11.1616013289999,15.2,-2.56342123900001));
#187190=CARTESIAN_POINT('Ctrl Pts',(11.1616013289999,11.6,-2.56342123900001));
#187191=CARTESIAN_POINT('Ctrl Pts',(11.1652741469999,15.2,-2.56260115600002));
#187192=CARTESIAN_POINT('Ctrl Pts',(11.1652741469999,11.6,-2.56260115600002));
#187193=CARTESIAN_POINT('Ctrl Pts',(11.1689506789999,15.2,-2.56177730200001));
#187194=CARTESIAN_POINT('Ctrl Pts',(11.1689506789999,11.6,-2.56177730200001));
#187195=CARTESIAN_POINT('Ctrl Pts',(11.1726309199999,15.2,-2.56094967200001));
#187196=CARTESIAN_POINT('Ctrl Pts',(11.1726309199999,11.6,-2.56094967200002));
#187197=CARTESIAN_POINT('Ctrl Pts',(11.1763148559999,15.2,-2.56011826200002));
#187198=CARTESIAN_POINT('Ctrl Pts',(11.1763148559999,11.6,-2.56011826200002));
#187199=CARTESIAN_POINT('Ctrl Pts',(11.1800024799999,15.2,-2.55928306600001));
#187200=CARTESIAN_POINT('Ctrl Pts',(11.1800024799999,11.6,-2.55928306600001));
#187201=CARTESIAN_POINT('Ctrl Pts',(11.1836937809999,15.2,-2.55844408100002));
#187202=CARTESIAN_POINT('Ctrl Pts',(11.1836937809999,11.6,-2.55844408100002));
#187203=CARTESIAN_POINT('Ctrl Pts',(11.1873887489999,15.2,-2.55760130200001));
#187204=CARTESIAN_POINT('Ctrl Pts',(11.1873887489999,11.6,-2.55760130200001));
#187205=CARTESIAN_POINT('Ctrl Pts',(11.1910873769999,15.2,-2.55675472300001));
#187206=CARTESIAN_POINT('Ctrl Pts',(11.1910873769999,11.6,-2.55675472300001));
#187207=CARTESIAN_POINT('Ctrl Pts',(11.1947896549999,15.2,-2.55590434200001));
#187208=CARTESIAN_POINT('Ctrl Pts',(11.1947896549999,11.6,-2.55590434200002));
#187209=CARTESIAN_POINT('Ctrl Pts',(11.1984955799999,15.2,-2.55505015600002));
#187210=CARTESIAN_POINT('Ctrl Pts',(11.1984955799999,11.6,-2.55505015600002));
#187211=CARTESIAN_POINT('Ctrl Pts',(11.2022051459999,15.2,-2.55419216300002));
#187212=CARTESIAN_POINT('Ctrl Pts',(11.2022051459999,11.6,-2.55419216300002));
#187213=CARTESIAN_POINT('Ctrl Pts',(11.2059183529999,15.2,-2.55333036400001));
#187214=CARTESIAN_POINT('Ctrl Pts',(11.2059183529999,11.6,-2.55333036400002));
#187215=CARTESIAN_POINT('Ctrl Pts',(11.2088918289999,15.2,-2.55263787800001));
#187216=CARTESIAN_POINT('Ctrl Pts',(11.2088918289999,11.6,-2.55263787800002));
#187217=CARTESIAN_POINT('Ctrl Pts',(11.2111235739999,15.2,-2.55211680100001));
#187218=CARTESIAN_POINT('Ctrl Pts',(11.2111235739999,11.6,-2.55211680100001));
#187219=CARTESIAN_POINT('Ctrl Pts',(11.2126121319999,15.2,-2.55176865400002));
#187220=CARTESIAN_POINT('Ctrl Pts',(11.2126121319999,11.6,-2.55176865400002));
#187221=CARTESIAN_POINT('Ctrl Pts',(11.2133565919999,15.2,-2.55159439000002));
#187222=CARTESIAN_POINT('Ctrl Pts',(11.2133565919999,11.6,-2.55159439000002));
#187223=CARTESIAN_POINT('Ctrl Pts',(10.0330625579999,15.2,-2.64164356400002));
#187224=CARTESIAN_POINT('Ctrl Pts',(10.0348230291495,15.2,-2.6419483125593));
#187225=CARTESIAN_POINT('Ctrl Pts',(10.0366407489629,15.2,-2.64225752130091));
#187226=CARTESIAN_POINT('Ctrl Pts',(10.0385148613113,15.2,-2.64257038295741));
#187227=CARTESIAN_POINT('Ctrl Pts',(10.0403980115767,15.2,-2.64288475339096));
#187228=CARTESIAN_POINT('Ctrl Pts',(10.0423381038896,15.2,-2.64320281589738));
#187229=CARTESIAN_POINT('Ctrl Pts',(10.0443343061848,15.2,-2.6435237812644));
#187230=CARTESIAN_POINT('Ctrl Pts',(10.0463305082985,15.2,-2.64384474660228));
#187231=CARTESIAN_POINT('Ctrl Pts',(10.0483828195931,15.2,-2.64416861599519));
#187232=CARTESIAN_POINT('Ctrl Pts',(10.0504904280165,15.2,-2.64449462848334));
#187233=CARTESIAN_POINT('Ctrl Pts',(10.0525980364399,15.2,-2.64482064097149));
#187234=CARTESIAN_POINT('Ctrl Pts',(10.0547609457251,15.1999999999999,-2.64514879481373));
#187235=CARTESIAN_POINT('Ctrl Pts',(10.0569783622521,15.2,-2.6454783534848));
#187236=CARTESIAN_POINT('Ctrl Pts',(10.0591957789806,15.2,-2.64580791218582));
#187237=CARTESIAN_POINT('Ctrl Pts',(10.061467704948,15.2,-2.64613887502637));
#187238=CARTESIAN_POINT('Ctrl Pts',(10.063793370495,15.2,-2.6464705267945));
#187239=CARTESIAN_POINT('Ctrl Pts',(10.0661190358309,15.2,-2.6468021785325));
#187240=CARTESIAN_POINT('Ctrl Pts',(10.0684984390365,15.2,-2.6471345208524));
#187241=CARTESIAN_POINT('Ctrl Pts',(10.0709308315426,15.2,-2.6474668567585));
#187242=CARTESIAN_POINT('Ctrl Pts',(10.0737686229471,15.2,-2.64785458200241));
#187243=CARTESIAN_POINT('Ctrl Pts',(10.0766785365834,15.2,-2.64824230028018));
#187244=CARTESIAN_POINT('Ctrl Pts',(10.0796594095367,15.2,-2.64862894528614));
#187245=CARTESIAN_POINT('Ctrl Pts',(10.0822144433641,15.2,-2.64896035527404));
#187246=CARTESIAN_POINT('Ctrl Pts',(10.0848216127188,15.2,-2.64929097719397));
#187247=CARTESIAN_POINT('Ctrl Pts',(10.0874802043011,15.2,-2.64962016201683));
#187248=CARTESIAN_POINT('Ctrl Pts',(10.0901387958833,15.2,-2.6499493468397));
#187249=CARTESIAN_POINT('Ctrl Pts',(10.0928488087771,15.2,-2.650277092594));
#187250=CARTESIAN_POINT('Ctrl Pts',(10.0956095465913,15.2,-2.65060276874893));
#187251=CARTESIAN_POINT('Ctrl Pts',(10.0983702846562,15.2,-2.65092844493343));
#187252=CARTESIAN_POINT('Ctrl Pts',(10.1011817494274,15.2,-2.65125205402602));
#187253=CARTESIAN_POINT('Ctrl Pts',(10.1040432583368,15.2,-2.65157297829333));
#187254=CARTESIAN_POINT('Ctrl Pts',(10.1069047669862,15.2,-2.65189390253149));
#187255=CARTESIAN_POINT('Ctrl Pts',(10.1098163187669,15.2,-2.65221214557876));
#187256=CARTESIAN_POINT('Ctrl Pts',(10.1127772496614,15.2,-2.65252710973384));
#187257=CARTESIAN_POINT('Ctrl Pts',(10.115738180556,15.2,-2.65284207388892));
#187258=CARTESIAN_POINT('Ctrl Pts',(10.11874848838,15.2,-2.65315375826091));
#187259=CARTESIAN_POINT('Ctrl Pts',(10.1218075241,15.2,-2.65346158558323));
#187260=CARTESIAN_POINT('Ctrl Pts',(10.1248665598201,15.2,-2.65376941290554));
#187261=CARTESIAN_POINT('Ctrl Pts',(10.1279743205738,15.2,-2.65407338115295));
#187262=CARTESIAN_POINT('Ctrl Pts',(10.1311301696225,15.2,-2.6543729277257));
#187263=CARTESIAN_POINT('Ctrl Pts',(10.1342860189579,15.2,-2.65467247432566));
#187264=CARTESIAN_POINT('Ctrl Pts',(10.1374899571313,15.2,-2.65496759964189));
#187265=CARTESIAN_POINT('Ctrl Pts',(10.1407413574773,15.2,-2.65525775424082));
#187266=CARTESIAN_POINT('Ctrl Pts',(10.1445346577332,15.2,-2.65559626792639));
#187267=CARTESIAN_POINT('Ctrl Pts',(10.148392559207,15.2,-2.65592801608681));
#187268=CARTESIAN_POINT('Ctrl Pts',(10.1523140901329,15.2,-2.65625215381364));
#187269=CARTESIAN_POINT('Ctrl Pts',(10.1556754021806,15.2,-2.6565299861365));
#187270=CARTESIAN_POINT('Ctrl Pts',(10.1590834633618,15.2,-2.65680222507444));
#187271=CARTESIAN_POINT('Ctrl Pts',(10.162537675405,15.2,-2.65706835573117));
#187272=CARTESIAN_POINT('Ctrl Pts',(10.1665675896645,15.2,-2.65737884151348));
#187273=CARTESIAN_POINT('Ctrl Pts',(10.1706603172142,15.2,-2.65768101328449));
#187274=CARTESIAN_POINT('Ctrl Pts',(10.1748149296714,15.2,-2.65797406926074));
#187275=CARTESIAN_POINT('Ctrl Pts',(10.1783760258784,15.2,-2.65822526008449));
#187276=CARTESIAN_POINT('Ctrl Pts',(10.1819825880631,15.2,-2.65846975596353));
#187277=CARTESIAN_POINT('Ctrl Pts',(10.1856340412657,15.2,-2.65870706753793));
#187278=CARTESIAN_POINT('Ctrl Pts',(10.1892854944683,15.2,-2.65894437911233));
#187279=CARTESIAN_POINT('Ctrl Pts',(10.192981837834,15.2,-2.65917450509562));
#187280=CARTESIAN_POINT('Ctrl Pts',(10.1967225100295,15.2,-2.65939697175454));
#187281=CARTESIAN_POINT('Ctrl Pts',(10.200463182225,15.2,-2.65961943841345));
#187282=CARTESIAN_POINT('Ctrl Pts',(10.2042481801746,15.2,-2.65983424195945));
#187283=CARTESIAN_POINT('Ctrl Pts',(10.2080769523659,15.2,-2.6600409227025));
#187284=CARTESIAN_POINT('Ctrl Pts',(10.2119057249049,15.2,-2.66024760346432));
#187285=CARTESIAN_POINT('Ctrl Pts',(10.2157782699648,15.2,-2.66044615690037));
#187286=CARTESIAN_POINT('Ctrl Pts',(10.2196940436801,15.2,-2.66063613374368));
#187287=CARTESIAN_POINT('Ctrl Pts',(10.2236098170397,15.2,-2.66082611056973));
#187288=CARTESIAN_POINT('Ctrl Pts',(10.2275688203671,15.2,-2.66100750994708));
#187289=CARTESIAN_POINT('Ctrl Pts',(10.2315705159897,15.2,-2.66117988802495));
#187290=CARTESIAN_POINT('Ctrl Pts',(10.2349052624631,15.2,-2.6613235364284));
#187291=CARTESIAN_POINT('Ctrl Pts',(10.2382696579332,15.2,-2.66146092320003));
#187292=CARTESIAN_POINT('Ctrl Pts',(10.2416633975165,15.2,-2.6615917942417));
#187293=CARTESIAN_POINT('Ctrl Pts',(10.2450571370999,15.2,-2.66172266528337));
#187294=CARTESIAN_POINT('Ctrl Pts',(10.2484802196249,15.2,-2.66184702443847));
#187295=CARTESIAN_POINT('Ctrl Pts',(10.2519323459601,15.2,-2.66196462450843));
#187296=CARTESIAN_POINT('Ctrl Pts',(10.2553844722953,15.2,-2.66208222457839));
#187297=CARTESIAN_POINT('Ctrl Pts',(10.2588656422836,15.2,-2.66219306607381));
#187298=CARTESIAN_POINT('Ctrl Pts',(10.2623755579796,15.2,-2.66229691024011));
#187299=CARTESIAN_POINT('Ctrl Pts',(10.2658854736755,15.2,-2.66240075440641));
#187300=CARTESIAN_POINT('Ctrl Pts',(10.2694241362485,15.2,-2.66249759921178));
#187301=CARTESIAN_POINT('Ctrl Pts',(10.2729912527083,15.2,-2.66258721178085));
#187302=CARTESIAN_POINT('Ctrl Pts',(10.2765583691681,15.2,-2.66267682434992));
#187303=CARTESIAN_POINT('Ctrl Pts',(10.2801539412488,15.2,-2.66275920294437));
#187304=CARTESIAN_POINT('Ctrl Pts',(10.2837776771956,15.2,-2.66283411801704));
#187305=CARTESIAN_POINT('Ctrl Pts',(10.2874014131425,15.2,-2.66290903308971));
#187306=CARTESIAN_POINT('Ctrl Pts',(10.2910533150067,15.2,-2.66297648424737));
#187307=CARTESIAN_POINT('Ctrl Pts',(10.2947330972312,15.2,-2.66303624452451));
#187308=CARTESIAN_POINT('Ctrl Pts',(10.2984128794557,15.2,-2.66309600480166));
#187309=CARTESIAN_POINT('Ctrl Pts',(10.3021205410195,15.2,-2.6631480763509));
#187310=CARTESIAN_POINT('Ctrl Pts',(10.3058558024801,15.2,-2.66319223648914));
#187311=CARTESIAN_POINT('Ctrl Pts',(10.3095910635336,15.2,-2.66323639662256));
#187312=CARTESIAN_POINT('Ctrl Pts',(10.313353923875,15.2,-2.66327264480431));
#187313=CARTESIAN_POINT('Ctrl Pts',(10.3171441049875,15.2,-2.66330076424635));
#187314=CARTESIAN_POINT('Ctrl Pts',(10.320934286513,15.2,-2.66332888369147));
#187315=CARTESIAN_POINT('Ctrl Pts',(10.3247517896936,15.2,-2.66334887532005));
#187316=CARTESIAN_POINT('Ctrl Pts',(10.328596340247,15.2,-2.66336052393184));
#187317=CARTESIAN_POINT('Ctrl Pts',(10.3324408908004,15.2,-2.66337217254364));
#187318=CARTESIAN_POINT('Ctrl Pts',(10.3363124867379,15.2,-2.66337548064473));
#187319=CARTESIAN_POINT('Ctrl Pts',(10.3402108600558,15.2,-2.66337023599228));
#187320=CARTESIAN_POINT('Ctrl Pts',(10.3441092333737,15.2,-2.66336499133984));
#187321=CARTESIAN_POINT('Ctrl Pts',(10.3480343822041,15.2,-2.66335119630656));
#187322=CARTESIAN_POINT('Ctrl Pts',(10.3519860387999,15.2,-2.66332864575146));
#187323=CARTESIAN_POINT('Ctrl Pts',(10.3559376953958,15.2,-2.66330609519636));
#187324=CARTESIAN_POINT('Ctrl Pts',(10.3599158599229,15.2,-2.66327478717437));
#187325=CARTESIAN_POINT('Ctrl Pts',(10.3639202682548,15.2,-2.66323452328595));
#187326=CARTESIAN_POINT('Ctrl Pts',(10.3679246765868,15.2,-2.66319425939753));
#187327=CARTESIAN_POINT('Ctrl Pts',(10.371955329325,15.2,-2.66314503629776));
#187328=CARTESIAN_POINT('Ctrl Pts',(10.3760119627264,15.2,-2.6630866599788));
#187329=CARTESIAN_POINT('Ctrl Pts',(10.3800685961278,15.2,-2.66302828365983));
#187330=CARTESIAN_POINT('Ctrl Pts',(10.3841512115291,15.2,-2.6629607526504));
#187331=CARTESIAN_POINT('Ctrl Pts',(10.3882595507143,15.2,-2.66288387223341));
#187332=CARTESIAN_POINT('Ctrl Pts',(10.3923678898996,15.2,-2.66280699181642));
#187333=CARTESIAN_POINT('Ctrl Pts',(10.3965019530165,15.2,-2.66272076289449));
#187334=CARTESIAN_POINT('Ctrl Pts',(10.4006614830165,15.2,-2.66262499574171));
#187335=CARTESIAN_POINT('Ctrl Pts',(10.4039891071979,15.2,-2.66254838201531));
#187336=CARTESIAN_POINT('Ctrl Pts',(10.4073330312423,15.2,-2.66246566257709));
#187337=CARTESIAN_POINT('Ctrl Pts',(10.4106931253159,15.2,-2.6623767429605));
#187338=CARTESIAN_POINT('Ctrl Pts',(10.4140532189318,15.2,-2.66228782335602));
#187339=CARTESIAN_POINT('Ctrl Pts',(10.4174294817457,15.2,-2.66219270320892));
#187340=CARTESIAN_POINT('Ctrl Pts',(10.4208217862059,15.2,-2.66209128821677));
#187341=CARTESIAN_POINT('Ctrl Pts',(10.4242140911284,15.2,-2.66198987321081));
#187342=CARTESIAN_POINT('Ctrl Pts',(10.4276224383076,15.2,-2.66188216367714));
#187343=CARTESIAN_POINT('Ctrl Pts',(10.4310466985514,15.2,-2.66176806544805));
#187344=CARTESIAN_POINT('Ctrl Pts',(10.4344709583287,15.2,-2.6616539672345));
#187345=CARTESIAN_POINT('Ctrl Pts',(10.4379111327372,15.2,-2.66153348233567));
#187346=CARTESIAN_POINT('Ctrl Pts',(10.4413670945092,15.2,-2.66140651673536));
#187347=CARTESIAN_POINT('Ctrl Pts',(10.444823056752,15.2,-2.66127955111776));
#187348=CARTESIAN_POINT('Ctrl Pts',(10.4482948076293,15.2,-2.66114610650321));
#187349=CARTESIAN_POINT('Ctrl Pts',(10.4517822207727,15.2,-2.66100609098802));
#187350=CARTESIAN_POINT('Ctrl Pts',(10.4552696334409,15.2,-2.6608660754919));
#187351=CARTESIAN_POINT('Ctrl Pts',(10.4587727085288,15.2,-2.66071949135787));
#187352=CARTESIAN_POINT('Ctrl Pts',(10.4622913234624,15.2,-2.66056624720417));
#187353=CARTESIAN_POINT('Ctrl Pts',(10.4658099388754,15.2,-2.66041300302959));
#187354=CARTESIAN_POINT('Ctrl Pts',(10.4693440911819,15.2,-2.66025310083476));
#187355=CARTESIAN_POINT('Ctrl Pts',(10.4728936600985,15.2,-2.66008645126969));
#187356=CARTESIAN_POINT('Ctrl Pts',(10.4764432285316,15.2,-2.65991980172731));
#187357=CARTESIAN_POINT('Ctrl Pts',(10.4800082122984,15.2,-2.65974640550317));
#187358=CARTESIAN_POINT('Ctrl Pts',(10.4835884902388,15.2,-2.65956617650949));
#187359=CARTESIAN_POINT('Ctrl Pts',(10.487168768667,15.2,-2.65938594749125));
#187360=CARTESIAN_POINT('Ctrl Pts',(10.4907643404863,15.2,-2.65919888487014));
#187361=CARTESIAN_POINT('Ctrl Pts',(10.4943750847952,15.2,-2.65900490402579));
#187362=CARTESIAN_POINT('Ctrl Pts',(10.4979858286121,15.2,-2.65881092320786));
#187363=CARTESIAN_POINT('Ctrl Pts',(10.501611745176,15.2,-2.65861002380798));
#187364=CARTESIAN_POINT('Ctrl Pts',(10.5052527136546,15.2,-2.6584021223257));
#187365=CARTESIAN_POINT('Ctrl Pts',(10.5088936826293,15.2,-2.65819422081508));
#187366=CARTESIAN_POINT('Ctrl Pts',(10.5125497053467,15.2,-2.65797931672135));
#187367=CARTESIAN_POINT('Ctrl Pts',(10.5162206597857,15.2,-2.65775732720822));
#187368=CARTESIAN_POINT('Ctrl Pts',(10.5198916137246,15.2,-2.65753533772534));
#187369=CARTESIAN_POINT('Ctrl Pts',(10.5235775028572,15.2,-2.65730626298806));
#187370=CARTESIAN_POINT('Ctrl Pts',(10.5272782053865,15.2,-2.65707002206366));
#187371=CARTESIAN_POINT('Ctrl Pts',(10.53097890842,15.2,-2.65683378110708));
#187372=CARTESIAN_POINT('Ctrl Pts',(10.5346944275744,15.2,-2.65659037247204));
#187373=CARTESIAN_POINT('Ctrl Pts',(10.5384246439999,15.2,-2.65633971629171));
#187374=CARTESIAN_POINT('Ctrl Pts',(10.5421548604254,15.2,-2.65608906011138));
#187375=CARTESIAN_POINT('Ctrl Pts',(10.5458997756999,15.2,-2.65583115714687));
#187376=CARTESIAN_POINT('Ctrl Pts',(10.5496592714062,15.2,-2.65556592696501));
#187377=CARTESIAN_POINT('Ctrl Pts',(10.5534187666004,15.2,-2.65530069681928));
#187378=CARTESIAN_POINT('Ctrl Pts',(10.5571928440954,15.2,-2.65502814039526));
#187379=CARTESIAN_POINT('Ctrl Pts',(10.5609813872473,15.2,-2.65474817775023));
#187380=CARTESIAN_POINT('Ctrl Pts',(10.5647699309154,15.2,-2.65446821506707));
#187381=CARTESIAN_POINT('Ctrl Pts',(10.5685729412895,15.2,-2.65418084742145));
#187382=CARTESIAN_POINT('Ctrl Pts',(10.5723903023324,15.2,-2.65388599846017));
#187383=CARTESIAN_POINT('Ctrl Pts',(10.5771620033759,15.2,-2.65351743727865));
#187384=CARTESIAN_POINT('Ctrl Pts',(10.5819561283114,15.2,-2.65313718318306));
#187385=CARTESIAN_POINT('Ctrl Pts',(10.5867724566465,15.2,-2.65274509047376));
#187386=CARTESIAN_POINT('Ctrl Pts',(10.5906255189997,15.2,-2.65243141633196));
#187387=CARTESIAN_POINT('Ctrl Pts',(10.5944927896386,15.2,-2.65211016498318));
#187388=CARTESIAN_POINT('Ctrl Pts',(10.5983741575056,15.2,-2.6517812615086));
#187389=CARTESIAN_POINT('Ctrl Pts',(10.6032258677359,15.2,-2.65137013213177));
#187390=CARTESIAN_POINT('Ctrl Pts',(10.608099603411,15.2,-2.65094704505005));
#187391=CARTESIAN_POINT('Ctrl Pts',(10.6129951477165,15.2,-2.65051185900838));
#187392=CARTESIAN_POINT('Ctrl Pts',(10.6169115833744,15.2,-2.65016371015607));
#187393=CARTESIAN_POINT('Ctrl Pts',(10.6208419763756,15.2,-2.64980781708898));
#187394=CARTESIAN_POINT('Ctrl Pts',(10.6247862148698,15.2,-2.64944410695724));
#187395=CARTESIAN_POINT('Ctrl Pts',(10.6287304528265,15.2,-2.64908039687506));
#187396=CARTESIAN_POINT('Ctrl Pts',(10.63268853689,15.2,-2.64870887040154));
#187397=CARTESIAN_POINT('Ctrl Pts',(10.6366603579722,15.2,-2.64832945570864));
#187398=CARTESIAN_POINT('Ctrl Pts',(10.6406321795955,15.2,-2.64795004096404));
#187399=CARTESIAN_POINT('Ctrl Pts',(10.6446177356122,15.2,-2.64756273789388));
#187400=CARTESIAN_POINT('Ctrl Pts',(10.6486169193871,15.2,-2.64716747592708));
#187401=CARTESIAN_POINT('Ctrl Pts',(10.6526161026171,15.2,-2.64677221401414));
#187402=CARTESIAN_POINT('Ctrl Pts',(10.6566289133787,15.2,-2.64636899442445));
#187403=CARTESIAN_POINT('Ctrl Pts',(10.6606552419375,15.2,-2.64595774629192));
#187404=CARTESIAN_POINT('Ctrl Pts',(10.664681571045,15.2,-2.64554649810337));
#187405=CARTESIAN_POINT('Ctrl Pts',(10.6687214180846,15.2,-2.64512722015274));
#187406=CARTESIAN_POINT('Ctrl Pts',(10.6727746758064,15.2,-2.64469984674003));
#187407=CARTESIAN_POINT('Ctrl Pts',(10.6768279329759,15.2,-2.64427247338555));
#187408=CARTESIAN_POINT('Ctrl Pts',(10.6808945997305,15.2,-2.64383700289956));
#187409=CARTESIAN_POINT('Ctrl Pts',(10.6849745710996,15.2,-2.64339336758104));
#187410=CARTESIAN_POINT('Ctrl Pts',(10.6890545430246,15.2,-2.64294973220208));
#187411=CARTESIAN_POINT('Ctrl Pts',(10.6931478179694,15.2,-2.64249793280464));
#187412=CARTESIAN_POINT('Ctrl Pts',(10.6972542903607,15.2,-2.64203790144569));
#187413=CARTESIAN_POINT('Ctrl Pts',(10.7013607621925,15.2,-2.64157787014943));
#187414=CARTESIAN_POINT('Ctrl Pts',(10.7054804310245,15.2,-2.64110960804926));
#187415=CARTESIAN_POINT('Ctrl Pts',(10.7096131915742,15.2,-2.64063304931129));
#187416=CARTESIAN_POINT('Ctrl Pts',(10.713745952687,15.2,-2.64015649050839));
#187417=CARTESIAN_POINT('Ctrl Pts',(10.7178918043683,15.2,-2.63967163347886));
#187418=CARTESIAN_POINT('Ctrl Pts',(10.7220506435027,15.2,-2.63917841478304));
#187419=CARTESIAN_POINT('Ctrl Pts',(10.7272491921375,15.2,-2.63856189144688));
#187420=CARTESIAN_POINT('Ctrl Pts',(10.7324680326749,15.2,-2.63793230175307));
#187421=CARTESIAN_POINT('Ctrl Pts',(10.7377069605926,15.2,-2.63728952168293));
#187422=CARTESIAN_POINT('Ctrl Pts',(10.7418981025842,15.2,-2.63677529766886));
#187423=CARTESIAN_POINT('Ctrl Pts',(10.746102101887,15.2,-2.6362526312787));
#187424=CARTESIAN_POINT('Ctrl Pts',(10.7503188538188,15.2,-2.63572146004522));
#187425=CARTESIAN_POINT('Ctrl Pts',(10.7545356063251,15.2,-2.63519028873936));
#187426=CARTESIAN_POINT('Ctrl Pts',(10.7587651119162,15.2,-2.63465061196263));
#187427=CARTESIAN_POINT('Ctrl Pts',(10.7630072677778,15.2,-2.63410236854134));
#187428=CARTESIAN_POINT('Ctrl Pts',(10.7672494230614,15.2,-2.63355412519475));
#187429=CARTESIAN_POINT('Ctrl Pts',(10.7715042295384,15.2,-2.63299731289261));
#187430=CARTESIAN_POINT('Ctrl Pts',(10.7757715835772,15.2,-2.63243187355083));
#187431=CARTESIAN_POINT('Ctrl Pts',(10.7800389381974,15.2,-2.631866434132));
#187432=CARTESIAN_POINT('Ctrl Pts',(10.7843188417604,15.2,-2.63129236579571));
#187433=CARTESIAN_POINT('Ctrl Pts',(10.7886111922166,15.2,-2.63070960904172));
#187434=CARTESIAN_POINT('Ctrl Pts',(10.7929035426727,15.2,-2.63012685228774));
#187435=CARTESIAN_POINT('Ctrl Pts',(10.7972083399692,15.2,-2.62953540480219));
#187436=CARTESIAN_POINT('Ctrl Pts',(10.8015254832058,15.2,-2.62893520943525));
#187437=CARTESIAN_POINT('Ctrl Pts',(10.8058426258541,15.2,-2.62833501415008));
#187438=CARTESIAN_POINT('Ctrl Pts',(10.8101721160628,15.2,-2.62772606936663));
#187439=CARTESIAN_POINT('Ctrl Pts',(10.8145138520053,15.2,-2.62710831802547));
#187440=CARTESIAN_POINT('Ctrl Pts',(10.8188555885394,15.2,-2.62649056660014));
#187441=CARTESIAN_POINT('Ctrl Pts',(10.8232095699496,15.2,-2.62586400558169));
#187442=CARTESIAN_POINT('Ctrl Pts',(10.8275756990221,15.2,-2.62522858087949));
#187443=CARTESIAN_POINT('Ctrl Pts',(10.8319418274997,15.2,-2.62459315626386));
#187444=CARTESIAN_POINT('Ctrl Pts',(10.8363201027758,15.2,-2.6239488650605));
#187445=CARTESIAN_POINT('Ctrl Pts',(10.8407104249161,15.2,-2.62329565000337));
#187446=CARTESIAN_POINT('Ctrl Pts',(10.8440031666709,15.2,-2.62280573868827));
#187447=CARTESIAN_POINT('Ctrl Pts',(10.847302686516,15.2,-2.62231080996962));
#187448=CARTESIAN_POINT('Ctrl Pts',(10.850608940852,15.2,-2.6218108365884));
#187449=CARTESIAN_POINT('Ctrl Pts',(10.855017280367,15.2,-2.62114420535288));
#187450=CARTESIAN_POINT('Ctrl Pts',(10.8594375942756,15.2,-2.62046860861245));
#187451=CARTESIAN_POINT('Ctrl Pts',(10.863869783629,15.2,-2.61978399118566));
#187452=CARTESIAN_POINT('Ctrl Pts',(10.8671939253422,15.2,-2.61927052816221));
#187453=CARTESIAN_POINT('Ctrl Pts',(10.8705247480878,15.2,-2.61875198924769));
#187454=CARTESIAN_POINT('Ctrl Pts',(10.8738622097166,15.2,-2.61822835326672));
#187455=CARTESIAN_POINT('Ctrl Pts',(10.8783121589591,15.2,-2.61753017189534));
#187456=CARTESIAN_POINT('Ctrl Pts',(10.8827739110335,15.2,-2.61682292656456));
#187457=CARTESIAN_POINT('Ctrl Pts',(10.887247370223,15.2,-2.61610656335792));
#187458=CARTESIAN_POINT('Ctrl Pts',(10.8906024643103,15.2,-2.61556929100174));
#187459=CARTESIAN_POINT('Ctrl Pts',(10.893964142805,15.2,-2.61502689076879));
#187460=CARTESIAN_POINT('Ctrl Pts',(10.897332365185,15.2,-2.61447933838573));
#187461=CARTESIAN_POINT('Ctrl Pts',(10.900700587565,15.2,-2.61393178600267));
#187462=CARTESIAN_POINT('Ctrl Pts',(10.9040753551409,15.2,-2.61337908225267));
#187463=CARTESIAN_POINT('Ctrl Pts',(10.9074566253519,15.2,-2.61282120389749));
#187464=CARTESIAN_POINT('Ctrl Pts',(10.910837895563,15.2,-2.61226332554231));
#187465=CARTESIAN_POINT('Ctrl Pts',(10.9142256696232,15.2,-2.61170027346274));
#187466=CARTESIAN_POINT('Ctrl Pts',(10.9176199072499,15.2,-2.61113202498339));
#187467=CARTESIAN_POINT('Ctrl Pts',(10.9221455578299,15.2,-2.61037436027543));
#187468=CARTESIAN_POINT('Ctrl Pts',(10.9266826989834,15.2,-2.6096074571275));
#187469=CARTESIAN_POINT('Ctrl Pts',(10.9312312350103,15.2,-2.6088312626398));
#187470=CARTESIAN_POINT('Ctrl Pts',(10.9346426367205,15.2,-2.60824911682691));
#187471=CARTESIAN_POINT('Ctrl Pts',(10.9380604492817,15.2,-2.6076617451107));
#187472=CARTESIAN_POINT('Ctrl Pts',(10.9414846316208,15.2,-2.60706912614368));
#187473=CARTESIAN_POINT('Ctrl Pts',(10.9471916023932,15.2,-2.60608142782943));
#187474=CARTESIAN_POINT('Ctrl Pts',(10.9529162663107,15.2,-2.60507915132934));
#187475=CARTESIAN_POINT('Ctrl Pts',(10.9586584424927,15.2,-2.6040621981337));
#187476=CARTESIAN_POINT('Ctrl Pts',(10.9621037480767,15.2,-2.60345202623848));
#187477=CARTESIAN_POINT('Ctrl Pts',(10.9655553572687,15.2,-2.60283657054354));
#187478=CARTESIAN_POINT('Ctrl Pts',(10.9690132313936,15.2,-2.60221580969063));
#187479=CARTESIAN_POINT('Ctrl Pts',(10.9724711055185,15.2,-2.60159504883773));
#187480=CARTESIAN_POINT('Ctrl Pts',(10.9759352440467,15.2,-2.60096898362943));
#187481=CARTESIAN_POINT('Ctrl Pts',(10.9794056077281,15.2,-2.60033759181614));
#187482=CARTESIAN_POINT('Ctrl Pts',(10.9828759714094,15.2,-2.59970620000286));
#187483=CARTESIAN_POINT('Ctrl Pts',(10.9863525608242,15.2,-2.59906948256353));
#187484=CARTESIAN_POINT('Ctrl Pts',(10.9898353360051,15.2,-2.59842741775064));
#187485=CARTESIAN_POINT('Ctrl Pts',(10.993318111186,15.2,-2.59778535293774));
#187486=CARTESIAN_POINT('Ctrl Pts',(10.9968070728799,15.2,-2.59713794068027));
#187487=CARTESIAN_POINT('Ctrl Pts',(11.0003021811274,15.2,-2.59648516178778));
#187488=CARTESIAN_POINT('Ctrl Pts',(11.0037972893748,15.2,-2.5958323828953));
#187489=CARTESIAN_POINT('Ctrl Pts',(11.0072985455136,15.2,-2.59517423653652));
#187490=CARTESIAN_POINT('Ctrl Pts',(11.010805909677,15.2,-2.5945107021447));
#187491=CARTESIAN_POINT('Ctrl Pts',(11.0143132744775,15.2,-2.59384716763233));
#187492=CARTESIAN_POINT('Ctrl Pts',(11.0178267478048,15.2,-2.59317824488512));
#187493=CARTESIAN_POINT('Ctrl Pts',(11.0213462910672,15.2,-2.59250391436971));
#187494=CARTESIAN_POINT('Ctrl Pts',(11.0248658336901,15.2,-2.59182958397681));
#187495=CARTESIAN_POINT('Ctrl Pts',(11.0283914454127,15.2,-2.59114984523419));
#187496=CARTESIAN_POINT('Ctrl Pts',(11.0319230890766,15.2,-2.59046467796694));
#187497=CARTESIAN_POINT('Ctrl Pts',(11.0354547327405,15.2,-2.5897795106997));
#187498=CARTESIAN_POINT('Ctrl Pts',(11.0389924078491,15.2,-2.58908891626064));
#187499=CARTESIAN_POINT('Ctrl Pts',(11.0425360759865,15.2,-2.58839287299108));
#187500=CARTESIAN_POINT('Ctrl Pts',(11.0460797441238,15.2,-2.58769682972152));
#187501=CARTESIAN_POINT('Ctrl Pts',(11.0496294053597,15.2,-2.58699533911152));
#187502=CARTESIAN_POINT('Ctrl Pts',(11.0531850214967,15.2,-2.58628838030069));
#187503=CARTESIAN_POINT('Ctrl Pts',(11.0579258434432,15.2,-2.5853457684673));
#187504=CARTESIAN_POINT('Ctrl Pts',(11.0626772516873,15.2,-2.5843934369934));
#187505=CARTESIAN_POINT('Ctrl Pts',(11.0674391563368,15.2,-2.58343133855108));
#187506=CARTESIAN_POINT('Ctrl Pts',(11.0710105844995,15.2,-2.58270976478488));
#187507=CARTESIAN_POINT('Ctrl Pts',(11.0745879164369,15.2,-2.58198269829397));
#187508=CARTESIAN_POINT('Ctrl Pts',(11.0781711151406,15.2,-2.58125011894511));
#187509=CARTESIAN_POINT('Ctrl Pts',(11.0817543138442,15.2,-2.58051753959624));
#187510=CARTESIAN_POINT('Ctrl Pts',(11.0853433793174,15.2,-2.57977944704243));
#187511=CARTESIAN_POINT('Ctrl Pts',(11.0889382734948,15.2,-2.57903582323271));
#187512=CARTESIAN_POINT('Ctrl Pts',(11.0925331676723,15.2,-2.57829219942299));
#187513=CARTESIAN_POINT('Ctrl Pts',(11.096133890878,15.2,-2.57754304457672));
#187514=CARTESIAN_POINT('Ctrl Pts',(11.0997404050133,15.2,-2.5767883387674));
#187515=CARTESIAN_POINT('Ctrl Pts',(11.1033469191486,15.2,-2.57603363295809));
#187516=CARTESIAN_POINT('Ctrl Pts',(11.1069592240376,15.2,-2.57527337640512));
#187517=CARTESIAN_POINT('Ctrl Pts',(11.1105772831556,15.2,-2.57450755105843));
#187518=CARTESIAN_POINT('Ctrl Pts',(11.1141953422737,15.2,-2.57374172571175));
#187519=CARTESIAN_POINT('Ctrl Pts',(11.1178191538413,15.2,-2.57297033109044));
#187520=CARTESIAN_POINT('Ctrl Pts',(11.121448684417,15.2,-2.57219334970276));
#187521=CARTESIAN_POINT('Ctrl Pts',(11.125078215652,15.2,-2.57141636817394));
#187522=CARTESIAN_POINT('Ctrl Pts',(11.1287134635304,15.2,-2.57063379841021));
#187523=CARTESIAN_POINT('Ctrl Pts',(11.1323543913103,15.2,-2.56984562479489));
#187524=CARTESIAN_POINT('Ctrl Pts',(11.1372089605811,15.2,-2.56879472687978));
#187525=CARTESIAN_POINT('Ctrl Pts',(11.1420736265119,15.2,-2.56773386186806));
#187526=CARTESIAN_POINT('Ctrl Pts',(11.1469482992466,15.2,-2.56666298695078));
#187527=CARTESIAN_POINT('Ctrl Pts',(11.1506043039637,15.2,-2.56585983072634));
#187528=CARTESIAN_POINT('Ctrl Pts',(11.1542659375507,15.2,-2.56505104442532));
#187529=CARTESIAN_POINT('Ctrl Pts',(11.1579331663336,15.2,-2.5642366120804));
#187530=CARTESIAN_POINT('Ctrl Pts',(11.1616003951165,15.2,-2.56342217973548));
#187531=CARTESIAN_POINT('Ctrl Pts',(11.1652732197991,15.2,-2.56260210053262));
#187532=CARTESIAN_POINT('Ctrl Pts',(11.168951605373,15.2,-2.56177635818839));
#187533=CARTESIAN_POINT('Ctrl Pts',(11.1726299916152,15.2,-2.56095061569416));
#187534=CARTESIAN_POINT('Ctrl Pts',(11.1763139379006,15.2,-2.56011920950666));
#187535=CARTESIAN_POINT('Ctrl Pts',(11.1800034000625,15.2,-2.5592821185509));
#187536=CARTESIAN_POINT('Ctrl Pts',(11.1836928615542,15.2,-2.5584450277472));
#187537=CARTESIAN_POINT('Ctrl Pts',(11.1873878377649,15.2,-2.55760225254806));
#187538=CARTESIAN_POINT('Ctrl Pts',(11.1910882902742,15.2,-2.5567537723275));
#187539=CARTESIAN_POINT('Ctrl Pts',(11.1947887427836,15.2,-2.55590529210695));
#187540=CARTESIAN_POINT('Ctrl Pts',(11.1984946703957,15.2,-2.55505110740725));
#187541=CARTESIAN_POINT('Ctrl Pts',(11.2022060566279,15.2,-2.55419121137746));
#187542=CARTESIAN_POINT('Ctrl Pts',(11.20591744286,15.2,-2.55333131534767));
#187543=CARTESIAN_POINT('Ctrl Pts',(11.2096342913237,15.2,-2.5524657101583));
#187544=CARTESIAN_POINT('Ctrl Pts',(11.2133565919999,15.2,-2.55159439000002));
#187545=CARTESIAN_POINT('Ctrl Pts',(10.0330625579999,12.2,-2.64164356400002));
#187546=CARTESIAN_POINT('Ctrl Pts',(10.0348230291495,12.2,-2.6419483125593));
#187547=CARTESIAN_POINT('Ctrl Pts',(10.0366407489629,12.2,-2.64225752130091));
#187548=CARTESIAN_POINT('Ctrl Pts',(10.0385148613113,12.2,-2.64257038295741));
#187549=CARTESIAN_POINT('Ctrl Pts',(10.0403980115767,12.2,-2.64288475339096));
#187550=CARTESIAN_POINT('Ctrl Pts',(10.0423381038896,12.2,-2.64320281589738));
#187551=CARTESIAN_POINT('Ctrl Pts',(10.0443343061848,12.2,-2.6435237812644));
#187552=CARTESIAN_POINT('Ctrl Pts',(10.0463305082985,12.2,-2.64384474660227));
#187553=CARTESIAN_POINT('Ctrl Pts',(10.0483828195931,12.2,-2.64416861599519));
#187554=CARTESIAN_POINT('Ctrl Pts',(10.0504904280165,12.2,-2.64449462848334));
#187555=CARTESIAN_POINT('Ctrl Pts',(10.0525980364399,12.2,-2.6448206409715));
#187556=CARTESIAN_POINT('Ctrl Pts',(10.0547609457251,12.2,-2.64514879481372));
#187557=CARTESIAN_POINT('Ctrl Pts',(10.0569783622521,12.2,-2.6454783534848));
#187558=CARTESIAN_POINT('Ctrl Pts',(10.0591957789806,12.2,-2.64580791218581));
#187559=CARTESIAN_POINT('Ctrl Pts',(10.061467704948,12.2,-2.64613887502637));
#187560=CARTESIAN_POINT('Ctrl Pts',(10.063793370495,12.2,-2.6464705267945));
#187561=CARTESIAN_POINT('Ctrl Pts',(10.0661190358309,12.2,-2.64680217853249));
#187562=CARTESIAN_POINT('Ctrl Pts',(10.0684984390365,12.2,-2.6471345208524));
#187563=CARTESIAN_POINT('Ctrl Pts',(10.0709308315426,12.2,-2.6474668567585));
#187564=CARTESIAN_POINT('Ctrl Pts',(10.0733632240487,12.2,-2.6477991926646));
#187565=CARTESIAN_POINT('Ctrl Pts',(10.0758486035812,12.2,-2.64813152383563));
#187566=CARTESIAN_POINT('Ctrl Pts',(10.0783862399034,12.2,-2.64846317774027));
#187567=CARTESIAN_POINT('Ctrl Pts',(10.0809238764561,12.2,-2.64879483167505));
#187568=CARTESIAN_POINT('Ctrl Pts',(10.0835137664236,12.2,-2.64912580789308));
#187569=CARTESIAN_POINT('Ctrl Pts',(10.0861551972378,12.2,-2.64945545299428));
#187570=CARTESIAN_POINT('Ctrl Pts',(10.088796627812,12.2,-2.64978509806555));
#187571=CARTESIAN_POINT('Ctrl Pts',(10.0914895985887,12.2,-2.65011341309641));
#187572=CARTESIAN_POINT('Ctrl Pts',(10.0942334084079,12.2,-2.65043976125113));
#187573=CARTESIAN_POINT('Ctrl Pts',(10.0969772182271,12.2,-2.65076610940585));
#187574=CARTESIAN_POINT('Ctrl Pts',(10.0997718692422,12.2,-2.65109049432738));
#187575=CARTESIAN_POINT('Ctrl Pts',(10.1026166770534,12.2,-2.65141229548247));
#187576=CARTESIAN_POINT('Ctrl Pts',(10.1054614848645,12.2,-2.65173409663756));
#187577=CARTESIAN_POINT('Ctrl Pts',(10.1083564488809,12.2,-2.65205331806851));
#187578=CARTESIAN_POINT('Ctrl Pts',(10.1113009016873,12.2,-2.65236935747391));
#187579=CARTESIAN_POINT('Ctrl Pts',(10.114245354761,12.2,-2.65268539690801));
#187580=CARTESIAN_POINT('Ctrl Pts',(10.1172392960313,12.2,-2.65299825575017));
#187581=CARTESIAN_POINT('Ctrl Pts',(10.1202820703659,12.2,-2.65330735293352));
#187582=CARTESIAN_POINT('Ctrl Pts',(10.1233248444241,12.2,-2.65361645008879));
#187583=CARTESIAN_POINT('Ctrl Pts',(10.1264164538067,12.2,-2.65392178319278));
#187584=CARTESIAN_POINT('Ctrl Pts',(10.1295562557901,12.2,-2.65422278851655));
#187585=CARTESIAN_POINT('Ctrl Pts',(10.1326960577735,12.2,-2.65452379384033));
#187586=CARTESIAN_POINT('Ctrl Pts',(10.1358840529847,12.2,-2.65482046992015));
#187587=CARTESIAN_POINT('Ctrl Pts',(10.1391196148639,12.2,-2.65511226549322));
#187588=CARTESIAN_POINT('Ctrl Pts',(10.142355177037,12.2,-2.65540406109279));
#187589=CARTESIAN_POINT('Ctrl Pts',(10.1456383039564,12.2,-2.6556909793419));
#187590=CARTESIAN_POINT('Ctrl Pts',(10.1489683832232,12.2,-2.65597247827368));
#187591=CARTESIAN_POINT('Ctrl Pts',(10.1522984621876,12.2,-2.65625397717988));
#187592=CARTESIAN_POINT('Ctrl Pts',(10.1556754910989,12.2,-2.65653006229181));
#187593=CARTESIAN_POINT('Ctrl Pts',(10.15909886924,12.2,-2.6568002079499));
#187594=CARTESIAN_POINT('Ctrl Pts',(10.162522247381,12.2,-2.657070353608));
#187595=CARTESIAN_POINT('Ctrl Pts',(10.1659919738642,12.2,-2.65733456172252));
#187596=CARTESIAN_POINT('Ctrl Pts',(10.1695074579,12.2,-2.65759232346359));
#187597=CARTESIAN_POINT('Ctrl Pts',(10.1730229422551,12.2,-2.65785008522808));
#187598=CARTESIAN_POINT('Ctrl Pts',(10.1765841833362,12.2,-2.65810140029853));
#187599=CARTESIAN_POINT('Ctrl Pts',(10.1801906020489,12.2,-2.65834577399032));
#187600=CARTESIAN_POINT('Ctrl Pts',(10.1837970204339,12.2,-2.65859014765991));
#187601=CARTESIAN_POINT('Ctrl Pts',(10.1874486162258,12.2,-2.65882757816672));
#187602=CARTESIAN_POINT('Ctrl Pts',(10.1911448195082,12.2,-2.6590575867417));
#187603=CARTESIAN_POINT('Ctrl Pts',(10.1948410227905,12.2,-2.65928759531668));
#187604=CARTESIAN_POINT('Ctrl Pts',(10.1985818339515,12.2,-2.65951017837586));
#187605=CARTESIAN_POINT('Ctrl Pts',(10.2023666943338,12.2,-2.65972486721258));
#187606=CARTESIAN_POINT('Ctrl Pts',(10.20615155506,12.2,-2.65993955606879));
#187607=CARTESIAN_POINT('Ctrl Pts',(10.2099804643496,12.2,-2.66014635131974));
#187608=CARTESIAN_POINT('Ctrl Pts',(10.213852873147,12.2,-2.66034479224666));
#187609=CARTESIAN_POINT('Ctrl Pts',(10.2177252815926,12.2,-2.66054323315555));
#187610=CARTESIAN_POINT('Ctrl Pts',(10.2216411903358,12.2,-2.66073332143923));
#187611=CARTESIAN_POINT('Ctrl Pts',(10.2256000587933,12.2,-2.66091461026678));
#187612=CARTESIAN_POINT('Ctrl Pts',(10.2302187389002,12.2,-2.6611261139099));
#187613=CARTESIAN_POINT('Ctrl Pts',(10.2348958924318,12.2,-2.6613256374042));
#187614=CARTESIAN_POINT('Ctrl Pts',(10.2396306779256,12.2,-2.66151249180915));
#187615=CARTESIAN_POINT('Ctrl Pts',(10.2430126675113,12.2,-2.66164595923918));
#187616=CARTESIAN_POINT('Ctrl Pts',(10.2464240620142,12.2,-2.6617729621052));
#187617=CARTESIAN_POINT('Ctrl Pts',(10.2498645584749,12.2,-2.66189325550743));
#187618=CARTESIAN_POINT('Ctrl Pts',(10.2533050545606,12.2,-2.66201354889655));
#187619=CARTESIAN_POINT('Ctrl Pts',(10.2567746537871,12.2,-2.66212713260269));
#187620=CARTESIAN_POINT('Ctrl Pts',(10.260273059584,12.2,-2.66223376599441));
#187621=CARTESIAN_POINT('Ctrl Pts',(10.2637714657622,12.2,-2.66234039939776));
#187622=CARTESIAN_POINT('Ctrl Pts',(10.2672986760149,12.2,-2.66244008130401));
#187623=CARTESIAN_POINT('Ctrl Pts',(10.2708543990681,12.2,-2.66253257797127));
#187624=CARTESIAN_POINT('Ctrl Pts',(10.2744101221214,12.2,-2.66262507463852));
#187625=CARTESIAN_POINT('Ctrl Pts',(10.277994357841,12.2,-2.66271038324212));
#187626=CARTESIAN_POINT('Ctrl Pts',(10.281606816839,12.2,-2.66278827498263));
#187627=CARTESIAN_POINT('Ctrl Pts',(10.2852192758369,12.2,-2.66286616672315));
#187628=CARTESIAN_POINT('Ctrl Pts',(10.2888599562005,12.2,-2.66293663952882));
#187629=CARTESIAN_POINT('Ctrl Pts',(10.2925285750184,12.2,-2.66299946723755));
#187630=CARTESIAN_POINT('Ctrl Pts',(10.2961971938364,12.2,-2.66306229494628));
#187631=CARTESIAN_POINT('Ctrl Pts',(10.2998937483913,12.2,-2.66311747771871));
#187632=CARTESIAN_POINT('Ctrl Pts',(10.3036179590148,12.2,-2.66316479299689));
#187633=CARTESIAN_POINT('Ctrl Pts',(10.3080870116007,12.2,-2.66322157132866));
#187634=CARTESIAN_POINT('Ctrl Pts',(10.3125958873221,12.2,-2.66326702091345));
#187635=CARTESIAN_POINT('Ctrl Pts',(10.3171441049875,12.2,-2.66330076424635));
#187636=CARTESIAN_POINT('Ctrl Pts',(10.320934286513,12.2,-2.66332888369147));
#187637=CARTESIAN_POINT('Ctrl Pts',(10.3247517896936,12.2,-2.66334887532005));
#187638=CARTESIAN_POINT('Ctrl Pts',(10.328596340247,12.2,-2.66336052393185));
#187639=CARTESIAN_POINT('Ctrl Pts',(10.3332098011625,12.2,-2.66337450226676));
#187640=CARTESIAN_POINT('Ctrl Pts',(10.3378622083032,12.2,-2.66337646909247));
#187641=CARTESIAN_POINT('Ctrl Pts',(10.3425530957121,12.2,-2.66336606150733));
#187642=CARTESIAN_POINT('Ctrl Pts',(10.3464621683398,12.2,-2.66335738852019));
#187643=CARTESIAN_POINT('Ctrl Pts',(10.3503979631104,12.2,-2.66334012392512));
#187644=CARTESIAN_POINT('Ctrl Pts',(10.3543602122098,12.2,-2.66331406322996));
#187645=CARTESIAN_POINT('Ctrl Pts',(10.3583224613092,12.2,-2.6632880025348));
#187646=CARTESIAN_POINT('Ctrl Pts',(10.3623111655451,12.2,-2.66325314364504));
#187647=CARTESIAN_POINT('Ctrl Pts',(10.3663260612417,12.2,-2.66320928822763));
#187648=CARTESIAN_POINT('Ctrl Pts',(10.3703409569383,12.2,-2.66316543281023));
#187649=CARTESIAN_POINT('Ctrl Pts',(10.3743820430464,12.2,-2.66311257981489));
#187650=CARTESIAN_POINT('Ctrl Pts',(10.3784490595069,12.2,-2.66305053425859));
#187651=CARTESIAN_POINT('Ctrl Pts',(10.382516075524,12.2,-2.66298848870904));
#187652=CARTESIAN_POINT('Ctrl Pts',(10.3866090201511,12.2,-2.66291724791214));
#187653=CARTESIAN_POINT('Ctrl Pts',(10.3907276387278,12.2,-2.66283662076891));
#187654=CARTESIAN_POINT('Ctrl Pts',(10.3948462577535,12.2,-2.6627559936169));
#187655=CARTESIAN_POINT('Ctrl Pts',(10.398990547251,12.2,-2.66266597969561));
#187656=CARTESIAN_POINT('Ctrl Pts',(10.4031602546795,12.2,-2.66256638927973));
#187657=CARTESIAN_POINT('Ctrl Pts',(10.4064960208041,12.2,-2.66248671694268));
#187658=CARTESIAN_POINT('Ctrl Pts',(10.4098480544588,12.2,-2.66240091461654));
#187659=CARTESIAN_POINT('Ctrl Pts',(10.4132162247688,12.2,-2.66230888949997));
#187660=CARTESIAN_POINT('Ctrl Pts',(10.41658439462,12.2,-2.66221686439595));
#187661=CARTESIAN_POINT('Ctrl Pts',(10.4199687025541,12.2,-2.66211861325516));
#187662=CARTESIAN_POINT('Ctrl Pts',(10.4233690202189,12.2,-2.66201404554213));
#187663=CARTESIAN_POINT('Ctrl Pts',(10.4267693383471,12.2,-2.66190947781486));
#187664=CARTESIAN_POINT('Ctrl Pts',(10.4301856654795,12.2,-2.66179859007033));
#187665=CARTESIAN_POINT('Ctrl Pts',(10.4336178749999,12.2,-2.66168129300838));
#187666=CARTESIAN_POINT('Ctrl Pts',(10.4370500845203,12.2,-2.66156399594643));
#187667=CARTESIAN_POINT('Ctrl Pts',(10.4404981767314,12.2,-2.66144028720596));
#187668=CARTESIAN_POINT('Ctrl Pts',(10.4439620250329,12.2,-2.66131007625375));
#187669=CARTESIAN_POINT('Ctrl Pts',(10.4474258728624,12.2,-2.66117986531928));
#187670=CARTESIAN_POINT('Ctrl Pts',(10.4509054783174,12.2,-2.66104315177794));
#187671=CARTESIAN_POINT('Ctrl Pts',(10.4544007147142,12.2,-2.66089984623347));
#187672=CARTESIAN_POINT('Ctrl Pts',(10.4578959515872,12.2,-2.66075654066948));
#187673=CARTESIAN_POINT('Ctrl Pts',(10.4614068208521,12.2,-2.66060664289754));
#187674=CARTESIAN_POINT('Ctrl Pts',(10.4649331971015,12.2,-2.66045006449944));
#187675=CARTESIAN_POINT('Ctrl Pts',(10.4684595728703,12.2,-2.66029348612266));
#187676=CARTESIAN_POINT('Ctrl Pts',(10.4720014559233,12.2,-2.66013022593842));
#187677=CARTESIAN_POINT('Ctrl Pts',(10.4755587244092,12.2,-2.65996019773054));
#187678=CARTESIAN_POINT('Ctrl Pts',(10.4791159933799,12.2,-2.6597901694995));
#187679=CARTESIAN_POINT('Ctrl Pts',(10.4826886477473,12.2,-2.6596133735348));
#187680=CARTESIAN_POINT('Ctrl Pts',(10.4862765655123,12.2,-2.65942972201502));
#187681=CARTESIAN_POINT('Ctrl Pts',(10.4898644827884,12.2,-2.65924607052027));
#187682=CARTESIAN_POINT('Ctrl Pts',(10.493467662401,12.2,-2.65905556520786));
#187683=CARTESIAN_POINT('Ctrl Pts',(10.4970859854376,12.2,-2.65885811972445));
#187684=CARTESIAN_POINT('Ctrl Pts',(10.5007043089671,12.2,-2.65866067421414));
#187685=CARTESIAN_POINT('Ctrl Pts',(10.5043377735346,12.2,-2.65845628950023));
#187686=CARTESIAN_POINT('Ctrl Pts',(10.50798626179,12.2,-2.6582448819327));
#187687=CARTESIAN_POINT('Ctrl Pts',(10.5125468718606,12.2,-2.65798062248768));
#187688=CARTESIAN_POINT('Ctrl Pts',(10.5171309534808,12.2,-2.65770538875962));
#187689=CARTESIAN_POINT('Ctrl Pts',(10.5217382778098,12.2,-2.65741901950843));
#187690=CARTESIAN_POINT('Ctrl Pts',(10.5254241369717,12.2,-2.6571899241262));
#187691=CARTESIAN_POINT('Ctrl Pts',(10.5291248681038,12.2,-2.65695370381061));
#187692=CARTESIAN_POINT('Ctrl Pts',(10.532840357188,12.2,-2.65671027505321));
#187693=CARTESIAN_POINT('Ctrl Pts',(10.5365558467784,12.2,-2.65646684626264));
#187694=CARTESIAN_POINT('Ctrl Pts',(10.5402860927067,12.2,-2.65621620964898));
#187695=CARTESIAN_POINT('Ctrl Pts',(10.5440309783562,12.2,-2.65595828674555));
#187696=CARTESIAN_POINT('Ctrl Pts',(10.5477758634954,12.2,-2.65570036387728));
#187697=CARTESIAN_POINT('Ctrl Pts',(10.551535387143,12.2,-2.65543515296914));
#187698=CARTESIAN_POINT('Ctrl Pts',(10.555309435744,12.2,-2.65516257675622));
#187699=CARTESIAN_POINT('Ctrl Pts',(10.5590834848592,12.2,-2.65489000050617));
#187700=CARTESIAN_POINT('Ctrl Pts',(10.5628720566888,12.2,-2.65461005757041));
#187701=CARTESIAN_POINT('Ctrl Pts',(10.5666750382859,12.2,-2.65432267077648));
#187702=CARTESIAN_POINT('Ctrl Pts',(10.5704780193649,12.2,-2.65403528402171));
#187703=CARTESIAN_POINT('Ctrl Pts',(10.574295408027,12.2,-2.65374045406565));
#187704=CARTESIAN_POINT('Ctrl Pts',(10.5781270918234,12.2,-2.65343810325781));
#187705=CARTESIAN_POINT('Ctrl Pts',(10.5819587761419,12.2,-2.65313575240877));
#187706=CARTESIAN_POINT('Ctrl Pts',(10.5858047554857,12.2,-2.65282588044637));
#187707=CARTESIAN_POINT('Ctrl Pts',(10.5896649152692,12.2,-2.65250841298316));
#187708=CARTESIAN_POINT('Ctrl Pts',(10.5935250745268,12.2,-2.6521909455632));
#187709=CARTESIAN_POINT('Ctrl Pts',(10.5973994151751,12.2,-2.65186588245979));
#187710=CARTESIAN_POINT('Ctrl Pts',(10.6012878243558,12.2,-2.65153314782111));
#187711=CARTESIAN_POINT('Ctrl Pts',(10.606148336229,12.2,-2.65111722948876));
#187712=CARTESIAN_POINT('Ctrl Pts',(10.6110308302991,12.2,-2.65068932611216));
#187713=CARTESIAN_POINT('Ctrl Pts',(10.6159350889084,12.2,-2.6502492943076));
#187714=CARTESIAN_POINT('Ctrl Pts',(10.6198584960097,12.2,-2.64989726884476));
#187715=CARTESIAN_POINT('Ctrl Pts',(10.6237958324915,12.2,-2.64953748080764));
#187716=CARTESIAN_POINT('Ctrl Pts',(10.6277469875026,12.2,-2.64916985750813));
#187717=CARTESIAN_POINT('Ctrl Pts',(10.6316981419753,12.2,-2.64880223425871));
#187718=CARTESIAN_POINT('Ctrl Pts',(10.635663115301,12.2,-2.64842677796113));
#187719=CARTESIAN_POINT('Ctrl Pts',(10.6396417971411,12.2,-2.64804341460439));
#187720=CARTESIAN_POINT('Ctrl Pts',(10.6436204795231,12.2,-2.64766005119542));
#187721=CARTESIAN_POINT('Ctrl Pts',(10.6476128690038,12.2,-2.64726878133014));
#187722=CARTESIAN_POINT('Ctrl Pts',(10.6516188599999,12.2,-2.64686953647505));
#187723=CARTESIAN_POINT('Ctrl Pts',(10.6566263484721,12.2,-2.64637048043338));
#187724=CARTESIAN_POINT('Ctrl Pts',(10.6616550858166,12.2,-2.64585896150561));
#187725=CARTESIAN_POINT('Ctrl Pts',(10.6667048610249,12.2,-2.64533484324172));
#187726=CARTESIAN_POINT('Ctrl Pts',(10.6707446814117,12.2,-2.64491554860775));
#187727=CARTESIAN_POINT('Ctrl Pts',(10.6747979657862,12.2,-2.6444881928673));
#187728=CARTESIAN_POINT('Ctrl Pts',(10.6788646068981,12.2,-2.64405270545384));
#187729=CARTESIAN_POINT('Ctrl Pts',(10.6829312474559,12.2,-2.64361721809972));
#187730=CARTESIAN_POINT('Ctrl Pts',(10.6870112458326,12.2,-2.64317359934322));
#187731=CARTESIAN_POINT('Ctrl Pts',(10.6911044932388,12.2,-2.64272178326702));
#187732=CARTESIAN_POINT('Ctrl Pts',(10.6951977412026,12.2,-2.64226996712926));
#187733=CARTESIAN_POINT('Ctrl Pts',(10.699304240042,12.2,-2.64180995186651));
#187734=CARTESIAN_POINT('Ctrl Pts',(10.7034238831568,12.2,-2.64134167317348));
#187735=CARTESIAN_POINT('Ctrl Pts',(10.7075435257102,12.2,-2.64087339454425));
#187736=CARTESIAN_POINT('Ctrl Pts',(10.7116763128814,12.2,-2.64039685245498));
#187737=CARTESIAN_POINT('Ctrl Pts',(10.7158221381528,12.2,-2.63991197927294));
#187738=CARTESIAN_POINT('Ctrl Pts',(10.719967963989,12.2,-2.63942710602484));
#187739=CARTESIAN_POINT('Ctrl Pts',(10.7241268296851,12.2,-2.6389339037109));
#187740=CARTESIAN_POINT('Ctrl Pts',(10.728298629122,12.2,-2.63843230693555));
#187741=CARTESIAN_POINT('Ctrl Pts',(10.7324704279905,12.2,-2.63793071022855));
#187742=CARTESIAN_POINT('Ctrl Pts',(10.7366551617147,12.2,-2.63742071906886));
#187743=CARTESIAN_POINT('Ctrl Pts',(10.7408527256485,12.2,-2.63690226983402));
#187744=CARTESIAN_POINT('Ctrl Pts',(10.7450502901542,12.2,-2.63638382052854));
#187745=CARTESIAN_POINT('Ctrl Pts',(10.7492606860782,12.2,-2.63585691344704));
#187746=CARTESIAN_POINT('Ctrl Pts',(10.7534838085869,12.2,-2.63532148597286));
#187747=CARTESIAN_POINT('Ctrl Pts',(10.7577069305203,12.2,-2.63478605857163));
#187748=CARTESIAN_POINT('Ctrl Pts',(10.7619427799196,12.2,-2.63424210981464));
#187749=CARTESIAN_POINT('Ctrl Pts',(10.7661912541168,12.2,-2.63368957855518));
#187750=CARTESIAN_POINT('Ctrl Pts',(10.7704397288928,12.2,-2.63313704722043));
#187751=CARTESIAN_POINT('Ctrl Pts',(10.7747008286768,12.2,-2.63257593266556));
#187752=CARTESIAN_POINT('Ctrl Pts',(10.7789744517994,12.2,-2.63200617524506));
#187753=CARTESIAN_POINT('Ctrl Pts',(10.7832480743397,12.2,-2.63143641790218));
#187754=CARTESIAN_POINT('Ctrl Pts',(10.7875342193775,12.2,-2.63085801691937));
#187755=CARTESIAN_POINT('Ctrl Pts',(10.7918327865804,12.2,-2.63027091107937));
#187756=CARTESIAN_POINT('Ctrl Pts',(10.796131354369,12.2,-2.62968380515938));
#187757=CARTESIAN_POINT('Ctrl Pts',(10.8004423427114,12.2,-2.62908799540758));
#187758=CARTESIAN_POINT('Ctrl Pts',(10.8047656532445,12.2,-2.62848342148297));
#187759=CARTESIAN_POINT('Ctrl Pts',(10.8090889631885,12.2,-2.62787884764073));
#187760=CARTESIAN_POINT('Ctrl Pts',(10.8134245954902,12.2,-2.62726551164167));
#187761=CARTESIAN_POINT('Ctrl Pts',(10.8177724480224,12.2,-2.6266433518601));
#187762=CARTESIAN_POINT('Ctrl Pts',(10.822120301147,12.2,-2.62602119199376));
#187763=CARTESIAN_POINT('Ctrl Pts',(10.8264803750866,12.2,-2.6253902105877));
#187764=CARTESIAN_POINT('Ctrl Pts',(10.8308525704916,12.2,-2.62475034927505));
#187765=CARTESIAN_POINT('Ctrl Pts',(10.8363178144499,12.2,-2.62395052267783));
#187766=CARTESIAN_POINT('Ctrl Pts',(10.8418019999779,12.2,-2.62313681862562));
#187767=CARTESIAN_POINT('Ctrl Pts',(10.8473049335446,12.2,-2.6223091295246));
#187768=CARTESIAN_POINT('Ctrl Pts',(10.8506066935646,12.2,-2.62181251608203));
#187769=CARTESIAN_POINT('Ctrl Pts',(10.853915201619,12.2,-2.62131086666771));
#187770=CARTESIAN_POINT('Ctrl Pts',(10.8572304182219,12.2,-2.62080415876718));
#187771=CARTESIAN_POINT('Ctrl Pts',(10.8605456348248,12.2,-2.62029745086664));
#187772=CARTESIAN_POINT('Ctrl Pts',(10.8638675590087,12.2,-2.61978568495375));
#187773=CARTESIAN_POINT('Ctrl Pts',(10.8671961500955,12.2,-2.61926883559797));
#187774=CARTESIAN_POINT('Ctrl Pts',(10.8705247411823,12.2,-2.61875198624219));
#187775=CARTESIAN_POINT('Ctrl Pts',(10.873859999177,12.2,-2.61823005451176));
#187776=CARTESIAN_POINT('Ctrl Pts',(10.8772018823047,12.2,-2.61770301711494));
#187777=CARTESIAN_POINT('Ctrl Pts',(10.8805437660395,12.2,-2.61717597962238));
#187778=CARTESIAN_POINT('Ctrl Pts',(10.8838922755261,12.2,-2.6166438358117));
#187779=CARTESIAN_POINT('Ctrl Pts',(10.887247370223,12.2,-2.61610656335792));
#187780=CARTESIAN_POINT('Ctrl Pts',(10.8906024643103,12.2,-2.61556929100174));
#187781=CARTESIAN_POINT('Ctrl Pts',(10.893964142805,12.2,-2.61502689076879));
#187782=CARTESIAN_POINT('Ctrl Pts',(10.897332365185,12.2,-2.61447933838573));
#187783=CARTESIAN_POINT('Ctrl Pts',(10.9007005875649,12.2,-2.61393178600267));
#187784=CARTESIAN_POINT('Ctrl Pts',(10.9040753551409,12.2,-2.61337908225267));
#187785=CARTESIAN_POINT('Ctrl Pts',(10.9074566253519,12.2,-2.61282120389749));
#187786=CARTESIAN_POINT('Ctrl Pts',(10.910837895563,12.2,-2.61226332554231));
#187787=CARTESIAN_POINT('Ctrl Pts',(10.9142256696232,12.2,-2.61170027346274));
#187788=CARTESIAN_POINT('Ctrl Pts',(10.9176199072499,12.2,-2.61113202498339));
#187789=CARTESIAN_POINT('Ctrl Pts',(10.9210141448766,12.2,-2.61056377650403));
#187790=CARTESIAN_POINT('Ctrl Pts',(10.924414846003,12.2,-2.60999033060822));
#187791=CARTESIAN_POINT('Ctrl Pts',(10.9278219701286,12.2,-2.60941166708804));
#187792=CARTESIAN_POINT('Ctrl Pts',(10.9312290942543,12.2,-2.60883300356785));
#187793=CARTESIAN_POINT('Ctrl Pts',(10.9346426415924,12.2,-2.6082491198214));
#187794=CARTESIAN_POINT('Ctrl Pts',(10.9380625728883,12.2,-2.60765999685565));
#187795=CARTESIAN_POINT('Ctrl Pts',(10.9414825041842,12.2,-2.6070708738899));
#187796=CARTESIAN_POINT('Ctrl Pts',(10.9449088188272,12.2,-2.60647651024159));
#187797=CARTESIAN_POINT('Ctrl Pts',(10.9483414764933,12.2,-2.60587688434743));
#187798=CARTESIAN_POINT('Ctrl Pts',(10.9517741347829,12.2,-2.60527725834434));
#187799=CARTESIAN_POINT('Ctrl Pts',(10.9552131362827,12.2,-2.60467237013976));
#187800=CARTESIAN_POINT('Ctrl Pts',(10.9586584424927,12.2,-2.6040621981337));
#187801=CARTESIAN_POINT('Ctrl Pts',(10.9621037480767,12.2,-2.60345202623848));
#187802=CARTESIAN_POINT('Ctrl Pts',(10.9655553572687,12.2,-2.60283657054354));
#187803=CARTESIAN_POINT('Ctrl Pts',(10.9690132313936,12.2,-2.60221580969063));
#187804=CARTESIAN_POINT('Ctrl Pts',(10.9724711055185,12.2,-2.60159504883773));
#187805=CARTESIAN_POINT('Ctrl Pts',(10.9759352440467,12.2,-2.60096898362943));
#187806=CARTESIAN_POINT('Ctrl Pts',(10.9794056077281,12.2,-2.60033759181614));
#187807=CARTESIAN_POINT('Ctrl Pts',(10.9840327590931,12.2,-2.59949573610333));
#187808=CARTESIAN_POINT('Ctrl Pts',(10.9886709779376,12.2,-2.59864441231112));
#187809=CARTESIAN_POINT('Ctrl Pts',(10.9933201712231,12.2,-2.59778356988246));
#187810=CARTESIAN_POINT('Ctrl Pts',(10.996807066979,12.2,-2.59713793791436));
#187811=CARTESIAN_POINT('Ctrl Pts',(11.0003001352533,12.2,-2.59648695240308));
#187812=CARTESIAN_POINT('Ctrl Pts',(11.0037993384711,12.2,-2.59583059289029));
#187813=CARTESIAN_POINT('Ctrl Pts',(11.0072985410531,12.2,-2.59517423349675));
#187814=CARTESIAN_POINT('Ctrl Pts',(11.0108038777765,12.2,-2.59451249950347));
#187815=CARTESIAN_POINT('Ctrl Pts',(11.0143153099411,12.2,-2.59384537069391));
#187816=CARTESIAN_POINT('Ctrl Pts',(11.0178267421057,12.2,-2.59317824188435));
#187817=CARTESIAN_POINT('Ctrl Pts',(11.0213442700446,12.2,-2.59250571880876));
#187818=CARTESIAN_POINT('Ctrl Pts',(11.0248678547082,12.2,-2.59182778050006));
#187819=CARTESIAN_POINT('Ctrl Pts',(11.0283914393719,12.2,-2.59114984219136));
#187820=CARTESIAN_POINT('Ctrl Pts',(11.0319210808269,12.2,-2.59046648861621));
#187821=CARTESIAN_POINT('Ctrl Pts',(11.0354567414063,12.2,-2.58977770076671));
#187822=CARTESIAN_POINT('Ctrl Pts',(11.0389924019856,12.2,-2.58908891291721));
#187823=CARTESIAN_POINT('Ctrl Pts',(11.0425340804993,12.2,-2.5883946904776));
#187824=CARTESIAN_POINT('Ctrl Pts',(11.0460817398386,12.2,-2.58769501313537));
#187825=CARTESIAN_POINT('Ctrl Pts',(11.0496293991779,12.2,-2.58699533579314));
#187826=CARTESIAN_POINT('Ctrl Pts',(11.0531830388207,12.2,-2.58629020434506));
#187827=CARTESIAN_POINT('Ctrl Pts',(11.0567426204823,12.2,-2.58557959812163));
#187828=CARTESIAN_POINT('Ctrl Pts',(11.0626752568003,12.2,-2.58439525437287));
#187829=CARTESIAN_POINT('Ctrl Pts',(11.0686243990709,12.2,-2.58319570559104));
#187830=CARTESIAN_POINT('Ctrl Pts',(11.0745898719863,12.2,-2.58198086163395));
#187831=CARTESIAN_POINT('Ctrl Pts',(11.0781691562557,12.2,-2.58125195515377));
#187832=CARTESIAN_POINT('Ctrl Pts',(11.0817543194767,12.2,-2.58051754229703));
#187833=CARTESIAN_POINT('Ctrl Pts',(11.0853453242911,12.2,-2.57977760385541));
#187834=CARTESIAN_POINT('Ctrl Pts',(11.0889363284531,12.2,-2.57903766554821));
#187835=CARTESIAN_POINT('Ctrl Pts',(11.0925331738306,12.2,-2.57829220223224));
#187836=CARTESIAN_POINT('Ctrl Pts',(11.096135823172,12.2,-2.57754119484637));
#187837=CARTESIAN_POINT('Ctrl Pts',(11.0997384725134,12.2,-2.57679018746049));
#187838=CARTESIAN_POINT('Ctrl Pts',(11.1033469247248,12.2,-2.57603363548969));
#187839=CARTESIAN_POINT('Ctrl Pts',(11.106961143844,12.2,-2.57527152068356));
#187840=CARTESIAN_POINT('Ctrl Pts',(11.1105753629631,12.2,-2.57450940587743));
#187841=CARTESIAN_POINT('Ctrl Pts',(11.114195347765,12.2,-2.5737417280053));
#187842=CARTESIAN_POINT('Ctrl Pts',(11.1178210620082,12.2,-2.57296846920006));
#187843=CARTESIAN_POINT('Ctrl Pts',(11.1214467762515,12.2,-2.57219521039482));
#187844=CARTESIAN_POINT('Ctrl Pts',(11.1250782213195,12.2,-2.57141637033981));
#187845=CARTESIAN_POINT('Ctrl Pts',(11.1287153575619,12.2,-2.57063193107713));
#187846=CARTESIAN_POINT('Ctrl Pts',(11.1323524938042,12.2,-2.56984749181445));
#187847=CARTESIAN_POINT('Ctrl Pts',(11.1359953227117,12.2,-2.56905745416413));
#187848=CARTESIAN_POINT('Ctrl Pts',(11.1396438055524,12.2,-2.56826179732061));
#187849=CARTESIAN_POINT('Ctrl Pts',(11.1432922883931,12.2,-2.56746614047708));
#187850=CARTESIAN_POINT('Ctrl Pts',(11.1469464247525,12.2,-2.56666486501253));
#187851=CARTESIAN_POINT('Ctrl Pts',(11.1506061784521,12.2,-2.56585795370929));
#187852=CARTESIAN_POINT('Ctrl Pts',(11.1542659328165,12.2,-2.56505104225945));
#187853=CARTESIAN_POINT('Ctrl Pts',(11.1579313042159,12.2,-2.56423849550803));
#187854=CARTESIAN_POINT('Ctrl Pts',(11.1616022605418,12.2,-2.56342029659668));
#187855=CARTESIAN_POINT('Ctrl Pts',(11.1652732162009,12.2,-2.56260209783397));
#187856=CARTESIAN_POINT('Ctrl Pts',(11.168949756718,12.2,-2.5617782472799));
#187857=CARTESIAN_POINT('Ctrl Pts',(11.1726318442097,12.2,-2.56094872689288));
#187858=CARTESIAN_POINT('Ctrl Pts',(11.1763139317014,12.2,-2.56011920650586));
#187859=CARTESIAN_POINT('Ctrl Pts',(11.180001564104,12.2,-2.55928401492258));
#187860=CARTESIAN_POINT('Ctrl Pts',(11.1836946977783,12.2,-2.55844313249096));
#187861=CARTESIAN_POINT('Ctrl Pts',(11.1873878314526,12.2,-2.55760225005933));
#187862=CARTESIAN_POINT('Ctrl Pts',(11.1910864657143,12.2,-2.55675567444037));
#187863=CARTESIAN_POINT('Ctrl Pts',(11.1947905667215,12.2,-2.55590339075916));
#187864=CARTESIAN_POINT('Ctrl Pts',(11.2009640686245,12.2,-2.55448291790553));
#187865=CARTESIAN_POINT('Ctrl Pts',(11.2071527573142,12.2,-2.55304659031659));
#187866=CARTESIAN_POINT('Ctrl Pts',(11.2133565919999,12.2,-2.55159439000002));
#187867=CARTESIAN_POINT('Origin',(-5.66257110645729E-14,15.2,-1.77635683940025E-14));
#187868=CARTESIAN_POINT('',(10.3068855235888,15.2,-1.18690176536278));
#187869=CARTESIAN_POINT('',(10.3068855235888,12.2,-1.18690176536278));
#187870=CARTESIAN_POINT('',(10.3068855229999,15.2,-1.18690176500001));
#187871=CARTESIAN_POINT('Origin',(-5.66257110645729E-14,12.2,-1.77635683940025E-14));
#187872=CARTESIAN_POINT('Origin',(-5.66257110645729E-14,15.2,-1.77635683940025E-14));
#187873=CARTESIAN_POINT('Origin',(-5.66257110645729E-14,15.2,-1.77635683940025E-14));
#187874=CARTESIAN_POINT('',(11.4623505329999,15.2,-0.929795809000016));
#187875=CARTESIAN_POINT('',(11.4869855316539,15.2,-0.54695830599941));
#187876=CARTESIAN_POINT('Origin',(-5.66257110645729E-14,15.2,-1.77635683940025E-14));
#187877=CARTESIAN_POINT('',(11.4869855316539,12.2,-0.54695830599941));
#187878=CARTESIAN_POINT('',(11.4869855319999,15.2,-0.546958306000014));
#187879=CARTESIAN_POINT('',(11.4623505329999,12.2,-0.929795809000016));
#187880=CARTESIAN_POINT('Origin',(-5.66257110645729E-14,12.2,-1.77635683940025E-14));
#187881=CARTESIAN_POINT('',(11.4623505329999,15.2,-0.929795809000016));
#187882=CARTESIAN_POINT('Ctrl Pts',(10.3068855239999,15.2,-1.18690176600001));
#187883=CARTESIAN_POINT('Ctrl Pts',(10.3068855239999,11.6,-1.18690176600001));
#187884=CARTESIAN_POINT('Ctrl Pts',(10.3070598099999,15.2,-1.18690675400002));
#187885=CARTESIAN_POINT('Ctrl Pts',(10.3070598099999,11.6,-1.18690675400002));
#187886=CARTESIAN_POINT('Ctrl Pts',(10.3074144739999,15.2,-1.18691681500001));
#187887=CARTESIAN_POINT('Ctrl Pts',(10.3074144739999,11.6,-1.18691681500001));
#187888=CARTESIAN_POINT('Ctrl Pts',(10.3079518789999,15.2,-1.18693179700001));
#187889=CARTESIAN_POINT('Ctrl Pts',(10.3079518789999,11.6,-1.18693179700002));
#187890=CARTESIAN_POINT('Ctrl Pts',(10.3086758299999,15.2,-1.18695143900001));
#187891=CARTESIAN_POINT('Ctrl Pts',(10.3086758299999,11.6,-1.18695143900002));
#187892=CARTESIAN_POINT('Ctrl Pts',(10.3095915439999,15.2,-1.18697537100001));
#187893=CARTESIAN_POINT('Ctrl Pts',(10.3095915439999,11.6,-1.18697537100001));
#187894=CARTESIAN_POINT('Ctrl Pts',(10.3105221239999,15.2,-1.18699875500001));
#187895=CARTESIAN_POINT('Ctrl Pts',(10.3105221239999,11.6,-1.18699875500001));
#187896=CARTESIAN_POINT('Ctrl Pts',(10.3114622379999,15.2,-1.18702143600002));
#187897=CARTESIAN_POINT('Ctrl Pts',(10.3114622379999,11.6,-1.18702143600002));
#187898=CARTESIAN_POINT('Ctrl Pts',(10.3124118609999,15.2,-1.18704339300002));
#187899=CARTESIAN_POINT('Ctrl Pts',(10.3124118609999,11.6,-1.18704339300002));
#187900=CARTESIAN_POINT('Ctrl Pts',(10.3133709649999,15.2,-1.18706461000002));
#187901=CARTESIAN_POINT('Ctrl Pts',(10.3133709649999,11.6,-1.18706461000002));
#187902=CARTESIAN_POINT('Ctrl Pts',(10.3143395239999,15.2,-1.18708506500001));
#187903=CARTESIAN_POINT('Ctrl Pts',(10.3143395239999,11.6,-1.18708506500001));
#187904=CARTESIAN_POINT('Ctrl Pts',(10.3153175129999,15.2,-1.18710474300002));
#187905=CARTESIAN_POINT('Ctrl Pts',(10.3153175129999,11.6,-1.18710474300002));
#187906=CARTESIAN_POINT('Ctrl Pts',(10.3163049049999,15.2,-1.18712362400001));
#187907=CARTESIAN_POINT('Ctrl Pts',(10.3163049049999,11.6,-1.18712362400002));
#187908=CARTESIAN_POINT('Ctrl Pts',(10.3173016729999,15.2,-1.18714169000001));
#187909=CARTESIAN_POINT('Ctrl Pts',(10.3173016729999,11.6,-1.18714169000001));
#187910=CARTESIAN_POINT('Ctrl Pts',(10.3183077929999,15.2,-1.18715892100001));
#187911=CARTESIAN_POINT('Ctrl Pts',(10.3183077929999,11.6,-1.18715892100001));
#187912=CARTESIAN_POINT('Ctrl Pts',(10.3193232389999,15.2,-1.18717530300001));
#187913=CARTESIAN_POINT('Ctrl Pts',(10.3193232389999,11.6,-1.18717530300001));
#187914=CARTESIAN_POINT('Ctrl Pts',(10.3203479849999,15.2,-1.18719081300001));
#187915=CARTESIAN_POINT('Ctrl Pts',(10.3203479849999,11.6,-1.18719081300001));
#187916=CARTESIAN_POINT('Ctrl Pts',(10.3213820039999,15.2,-1.18720543700002));
#187917=CARTESIAN_POINT('Ctrl Pts',(10.3213820039999,11.6,-1.18720543700002));
#187918=CARTESIAN_POINT('Ctrl Pts',(10.3224252739999,15.2,-1.18721915500001));
#187919=CARTESIAN_POINT('Ctrl Pts',(10.3224252739999,11.6,-1.18721915500001));
#187920=CARTESIAN_POINT('Ctrl Pts',(10.3234777669999,15.2,-1.18723195000001));
#187921=CARTESIAN_POINT('Ctrl Pts',(10.3234777669999,11.6,-1.18723195000001));
#187922=CARTESIAN_POINT('Ctrl Pts',(10.3245394589999,15.2,-1.18724380600002));
#187923=CARTESIAN_POINT('Ctrl Pts',(10.3245394589999,11.6,-1.18724380600002));
#187924=CARTESIAN_POINT('Ctrl Pts',(10.3256103239999,15.2,-1.18725470300001));
#187925=CARTESIAN_POINT('Ctrl Pts',(10.3256103239999,11.6,-1.18725470300001));
#187926=CARTESIAN_POINT('Ctrl Pts',(10.3266903399999,15.2,-1.18726462500002));
#187927=CARTESIAN_POINT('Ctrl Pts',(10.3266903399999,11.6,-1.18726462500002));
#187928=CARTESIAN_POINT('Ctrl Pts',(10.3277794779999,15.2,-1.18727355500001));
#187929=CARTESIAN_POINT('Ctrl Pts',(10.3277794779999,11.6,-1.18727355500001));
#187930=CARTESIAN_POINT('Ctrl Pts',(10.3288777159999,15.2,-1.18728147400001));
#187931=CARTESIAN_POINT('Ctrl Pts',(10.3288777159999,11.6,-1.18728147400002));
#187932=CARTESIAN_POINT('Ctrl Pts',(10.3299850289999,15.2,-1.18728836600001));
#187933=CARTESIAN_POINT('Ctrl Pts',(10.3299850289999,11.6,-1.18728836600001));
#187934=CARTESIAN_POINT('Ctrl Pts',(10.3311013919999,15.2,-1.18729421400001));
#187935=CARTESIAN_POINT('Ctrl Pts',(10.3311013919999,11.6,-1.18729421400001));
#187936=CARTESIAN_POINT('Ctrl Pts',(10.3322267799999,15.2,-1.18729900100002));
#187937=CARTESIAN_POINT('Ctrl Pts',(10.3322267799999,11.6,-1.18729900100002));
#187938=CARTESIAN_POINT('Ctrl Pts',(10.3333611709999,15.2,-1.18730271200001));
#187939=CARTESIAN_POINT('Ctrl Pts',(10.3333611709999,11.6,-1.18730271200001));
#187940=CARTESIAN_POINT('Ctrl Pts',(10.3345045389999,15.2,-1.18730532600001));
#187941=CARTESIAN_POINT('Ctrl Pts',(10.3345045389999,11.6,-1.18730532600001));
#187942=CARTESIAN_POINT('Ctrl Pts',(10.3356568609999,15.2,-1.18730683000001));
#187943=CARTESIAN_POINT('Ctrl Pts',(10.3356568609999,11.6,-1.18730683000001));
#187944=CARTESIAN_POINT('Ctrl Pts',(10.3368181129999,15.2,-1.18730720600002));
#187945=CARTESIAN_POINT('Ctrl Pts',(10.3368181129999,11.6,-1.18730720600002));
#187946=CARTESIAN_POINT('Ctrl Pts',(10.3379882699999,15.2,-1.18730643700002));
#187947=CARTESIAN_POINT('Ctrl Pts',(10.3379882699999,11.6,-1.18730643700002));
#187948=CARTESIAN_POINT('Ctrl Pts',(10.3391673089999,15.2,-1.18730450800001));
#187949=CARTESIAN_POINT('Ctrl Pts',(10.3391673089999,11.6,-1.18730450800001));
#187950=CARTESIAN_POINT('Ctrl Pts',(10.3403552059999,15.2,-1.18730140200002));
#187951=CARTESIAN_POINT('Ctrl Pts',(10.3403552059999,11.6,-1.18730140200002));
#187952=CARTESIAN_POINT('Ctrl Pts',(10.3415519369999,15.2,-1.18729710200002));
#187953=CARTESIAN_POINT('Ctrl Pts',(10.3415519369999,11.6,-1.18729710200002));
#187954=CARTESIAN_POINT('Ctrl Pts',(10.3427574809999,15.2,-1.18729159300001));
#187955=CARTESIAN_POINT('Ctrl Pts',(10.3427574809999,11.6,-1.18729159300001));
#187956=CARTESIAN_POINT('Ctrl Pts',(10.3439718129999,15.2,-1.18728485900002));
#187957=CARTESIAN_POINT('Ctrl Pts',(10.3439718129999,11.6,-1.18728485900002));
#187958=CARTESIAN_POINT('Ctrl Pts',(10.3451949089999,15.2,-1.18727688200002));
#187959=CARTESIAN_POINT('Ctrl Pts',(10.3451949089999,11.6,-1.18727688200002));
#187960=CARTESIAN_POINT('Ctrl Pts',(10.3464267469999,15.2,-1.18726764900002));
#187961=CARTESIAN_POINT('Ctrl Pts',(10.3464267469999,11.6,-1.18726764900002));
#187962=CARTESIAN_POINT('Ctrl Pts',(10.3476673029999,15.2,-1.18725714300002));
#187963=CARTESIAN_POINT('Ctrl Pts',(10.3476673029999,11.6,-1.18725714300002));
#187964=CARTESIAN_POINT('Ctrl Pts',(10.3489165549999,15.2,-1.18724534800001));
#187965=CARTESIAN_POINT('Ctrl Pts',(10.3489165549999,11.6,-1.18724534800001));
#187966=CARTESIAN_POINT('Ctrl Pts',(10.3501744809999,15.2,-1.18723224800001));
#187967=CARTESIAN_POINT('Ctrl Pts',(10.3501744809999,11.6,-1.18723224800001));
#187968=CARTESIAN_POINT('Ctrl Pts',(10.3514410549999,15.2,-1.18721782700002));
#187969=CARTESIAN_POINT('Ctrl Pts',(10.3514410549999,11.6,-1.18721782700002));
#187970=CARTESIAN_POINT('Ctrl Pts',(10.3527162579999,15.2,-1.18720207200001));
#187971=CARTESIAN_POINT('Ctrl Pts',(10.3527162579999,11.6,-1.18720207200001));
#187972=CARTESIAN_POINT('Ctrl Pts',(10.3540000639999,15.2,-1.18718496500001));
#187973=CARTESIAN_POINT('Ctrl Pts',(10.3540000639999,11.6,-1.18718496500001));
#187974=CARTESIAN_POINT('Ctrl Pts',(10.3552924529999,15.2,-1.18716649100001));
#187975=CARTESIAN_POINT('Ctrl Pts',(10.3552924529999,11.6,-1.18716649100001));
#187976=CARTESIAN_POINT('Ctrl Pts',(10.3565934029999,15.2,-1.18714663700001));
#187977=CARTESIAN_POINT('Ctrl Pts',(10.3565934029999,11.6,-1.18714663700001));
#187978=CARTESIAN_POINT('Ctrl Pts',(10.3579028899999,15.2,-1.18712538500001));
#187979=CARTESIAN_POINT('Ctrl Pts',(10.3579028899999,11.6,-1.18712538500001));
#187980=CARTESIAN_POINT('Ctrl Pts',(10.3592208919999,15.2,-1.18710272100001));
#187981=CARTESIAN_POINT('Ctrl Pts',(10.3592208919999,11.6,-1.18710272100001));
#187982=CARTESIAN_POINT('Ctrl Pts',(10.3605473869999,15.2,-1.18707863200001));
#187983=CARTESIAN_POINT('Ctrl Pts',(10.3605473869999,11.6,-1.18707863200001));
#187984=CARTESIAN_POINT('Ctrl Pts',(10.3618823529999,15.2,-1.18705310000002));
#187985=CARTESIAN_POINT('Ctrl Pts',(10.3618823529999,11.6,-1.18705310000002));
#187986=CARTESIAN_POINT('Ctrl Pts',(10.3632257689999,15.2,-1.18702611100002));
#187987=CARTESIAN_POINT('Ctrl Pts',(10.3632257689999,11.6,-1.18702611100002));
#187988=CARTESIAN_POINT('Ctrl Pts',(10.3645776119999,15.2,-1.18699765000001));
#187989=CARTESIAN_POINT('Ctrl Pts',(10.3645776119999,11.6,-1.18699765000002));
#187990=CARTESIAN_POINT('Ctrl Pts',(10.3659378599999,15.2,-1.18696770300001));
#187991=CARTESIAN_POINT('Ctrl Pts',(10.3659378599999,11.6,-1.18696770300002));
#187992=CARTESIAN_POINT('Ctrl Pts',(10.3673064919999,15.2,-1.18693625600002));
#187993=CARTESIAN_POINT('Ctrl Pts',(10.3673064919999,11.6,-1.18693625600002));
#187994=CARTESIAN_POINT('Ctrl Pts',(10.3686834869999,15.2,-1.18690329300001));
#187995=CARTESIAN_POINT('Ctrl Pts',(10.3686834869999,11.6,-1.18690329300001));
#187996=CARTESIAN_POINT('Ctrl Pts',(10.3700688229999,15.2,-1.18686880000002));
#187997=CARTESIAN_POINT('Ctrl Pts',(10.3700688229999,11.6,-1.18686880000002));
#187998=CARTESIAN_POINT('Ctrl Pts',(10.3714624779999,15.2,-1.18683276400001));
#187999=CARTESIAN_POINT('Ctrl Pts',(10.3714624779999,11.6,-1.18683276400001));
#188000=CARTESIAN_POINT('Ctrl Pts',(10.3728644309999,15.2,-1.18679516800002));
#188001=CARTESIAN_POINT('Ctrl Pts',(10.3728644309999,11.6,-1.18679516800002));
#188002=CARTESIAN_POINT('Ctrl Pts',(10.3742746599999,15.2,-1.18675600000001));
#188003=CARTESIAN_POINT('Ctrl Pts',(10.3742746599999,11.6,-1.18675600000001));
#188004=CARTESIAN_POINT('Ctrl Pts',(10.3756931459999,15.2,-1.18671524300002));
#188005=CARTESIAN_POINT('Ctrl Pts',(10.3756931459999,11.6,-1.18671524300002));
#188006=CARTESIAN_POINT('Ctrl Pts',(10.3771198649999,15.2,-1.18667288700002));
#188007=CARTESIAN_POINT('Ctrl Pts',(10.3771198649999,11.6,-1.18667288700002));
#188008=CARTESIAN_POINT('Ctrl Pts',(10.3785547979999,15.2,-1.18662891400001));
#188009=CARTESIAN_POINT('Ctrl Pts',(10.3785547979999,11.6,-1.18662891400001));
#188010=CARTESIAN_POINT('Ctrl Pts',(10.3799979229999,15.2,-1.18658331200002));
#188011=CARTESIAN_POINT('Ctrl Pts',(10.3799979229999,11.6,-1.18658331200002));
#188012=CARTESIAN_POINT('Ctrl Pts',(10.3814492199999,15.2,-1.18653606700001));
#188013=CARTESIAN_POINT('Ctrl Pts',(10.3814492199999,11.6,-1.18653606700002));
#188014=CARTESIAN_POINT('Ctrl Pts',(10.3829086669999,15.2,-1.18648716400001));
#188015=CARTESIAN_POINT('Ctrl Pts',(10.3829086669999,11.6,-1.18648716400001));
#188016=CARTESIAN_POINT('Ctrl Pts',(10.3843762449999,15.2,-1.18643659100002));
#188017=CARTESIAN_POINT('Ctrl Pts',(10.3843762449999,11.6,-1.18643659100002));
#188018=CARTESIAN_POINT('Ctrl Pts',(10.3858519319999,15.2,-1.18638433300001));
#188019=CARTESIAN_POINT('Ctrl Pts',(10.3858519319999,11.6,-1.18638433300002));
#188020=CARTESIAN_POINT('Ctrl Pts',(10.3873357079999,15.2,-1.18633037800001));
#188021=CARTESIAN_POINT('Ctrl Pts',(10.3873357079999,11.6,-1.18633037800001));
#188022=CARTESIAN_POINT('Ctrl Pts',(10.3888275529999,15.2,-1.18627470900002));
#188023=CARTESIAN_POINT('Ctrl Pts',(10.3888275529999,11.6,-1.18627470900002));
#188024=CARTESIAN_POINT('Ctrl Pts',(10.3903274449999,15.2,-1.18621731600001));
#188025=CARTESIAN_POINT('Ctrl Pts',(10.3903274449999,11.6,-1.18621731600001));
#188026=CARTESIAN_POINT('Ctrl Pts',(10.3918353649999,15.2,-1.18615818300002));
#188027=CARTESIAN_POINT('Ctrl Pts',(10.3918353649999,11.6,-1.18615818300002));
#188028=CARTESIAN_POINT('Ctrl Pts',(10.3933512919999,15.2,-1.18609729900002));
#188029=CARTESIAN_POINT('Ctrl Pts',(10.3933512919999,11.6,-1.18609729900002));
#188030=CARTESIAN_POINT('Ctrl Pts',(10.3948752069999,15.2,-1.18603464900001));
#188031=CARTESIAN_POINT('Ctrl Pts',(10.3948752069999,11.6,-1.18603464900001));
#188032=CARTESIAN_POINT('Ctrl Pts',(10.3964070879999,15.2,-1.18597021900001));
#188033=CARTESIAN_POINT('Ctrl Pts',(10.3964070879999,11.6,-1.18597021900001));
#188034=CARTESIAN_POINT('Ctrl Pts',(10.3979469159999,15.2,-1.18590399800001));
#188035=CARTESIAN_POINT('Ctrl Pts',(10.3979469159999,11.6,-1.18590399800001));
#188036=CARTESIAN_POINT('Ctrl Pts',(10.3994946729999,15.2,-1.18583597200002));
#188037=CARTESIAN_POINT('Ctrl Pts',(10.3994946729999,11.6,-1.18583597200002));
#188038=CARTESIAN_POINT('Ctrl Pts',(10.4010503359999,15.2,-1.18576612800001));
#188039=CARTESIAN_POINT('Ctrl Pts',(10.4010503359999,11.6,-1.18576612800001));
#188040=CARTESIAN_POINT('Ctrl Pts',(10.4026138859999,15.2,-1.18569445100002));
#188041=CARTESIAN_POINT('Ctrl Pts',(10.4026138859999,11.6,-1.18569445100002));
#188042=CARTESIAN_POINT('Ctrl Pts',(10.4041853039999,15.2,-1.18562093200001));
#188043=CARTESIAN_POINT('Ctrl Pts',(10.4041853039999,11.6,-1.18562093200001));
#188044=CARTESIAN_POINT('Ctrl Pts',(10.4057645699999,15.2,-1.18554555400001));
#188045=CARTESIAN_POINT('Ctrl Pts',(10.4057645699999,11.6,-1.18554555400001));
#188046=CARTESIAN_POINT('Ctrl Pts',(10.4073516649999,15.2,-1.18546830700001));
#188047=CARTESIAN_POINT('Ctrl Pts',(10.4073516649999,11.6,-1.18546830700002));
#188048=CARTESIAN_POINT('Ctrl Pts',(10.4089465679999,15.2,-1.18538917800001));
#188049=CARTESIAN_POINT('Ctrl Pts',(10.4089465679999,11.6,-1.18538917800001));
#188050=CARTESIAN_POINT('Ctrl Pts',(10.4105492599999,15.2,-1.18530815300002));
#188051=CARTESIAN_POINT('Ctrl Pts',(10.4105492599999,11.6,-1.18530815300002));
#188052=CARTESIAN_POINT('Ctrl Pts',(10.4121597229999,15.2,-1.18522521900001));
#188053=CARTESIAN_POINT('Ctrl Pts',(10.4121597229999,11.6,-1.18522521900001));
#188054=CARTESIAN_POINT('Ctrl Pts',(10.4137779369999,15.2,-1.18514036600001));
#188055=CARTESIAN_POINT('Ctrl Pts',(10.4137779369999,11.6,-1.18514036600002));
#188056=CARTESIAN_POINT('Ctrl Pts',(10.4154038819999,15.2,-1.18505358000002));
#188057=CARTESIAN_POINT('Ctrl Pts',(10.4154038819999,11.6,-1.18505358000002));
#188058=CARTESIAN_POINT('Ctrl Pts',(10.4170375389999,15.2,-1.18496484700001));
#188059=CARTESIAN_POINT('Ctrl Pts',(10.4170375389999,11.6,-1.18496484700001));
#188060=CARTESIAN_POINT('Ctrl Pts',(10.4186788889999,15.2,-1.18487415700002));
#188061=CARTESIAN_POINT('Ctrl Pts',(10.4186788889999,11.6,-1.18487415700002));
#188062=CARTESIAN_POINT('Ctrl Pts',(10.4203279129999,15.2,-1.18478149600001));
#188063=CARTESIAN_POINT('Ctrl Pts',(10.4203279129999,11.6,-1.18478149600001));
#188064=CARTESIAN_POINT('Ctrl Pts',(10.4219845919999,15.2,-1.18468685300002));
#188065=CARTESIAN_POINT('Ctrl Pts',(10.4219845919999,11.6,-1.18468685300002));
#188066=CARTESIAN_POINT('Ctrl Pts',(10.4236489079999,15.2,-1.18459021500001));
#188067=CARTESIAN_POINT('Ctrl Pts',(10.4236489079999,11.6,-1.18459021500001));
#188068=CARTESIAN_POINT('Ctrl Pts',(10.4253208399999,15.2,-1.18449157100001));
#188069=CARTESIAN_POINT('Ctrl Pts',(10.4253208399999,11.6,-1.18449157100002));
#188070=CARTESIAN_POINT('Ctrl Pts',(10.4270003709999,15.2,-1.18439090700001));
#188071=CARTESIAN_POINT('Ctrl Pts',(10.4270003709999,11.6,-1.18439090700001));
#188072=CARTESIAN_POINT('Ctrl Pts',(10.4286874819999,15.2,-1.18428821100002));
#188073=CARTESIAN_POINT('Ctrl Pts',(10.4286874819999,11.6,-1.18428821100002));
#188074=CARTESIAN_POINT('Ctrl Pts',(10.4303821539999,15.2,-1.18418347300001));
#188075=CARTESIAN_POINT('Ctrl Pts',(10.4303821539999,11.6,-1.18418347300001));
#188076=CARTESIAN_POINT('Ctrl Pts',(10.4320843689999,15.2,-1.18407668000001));
#188077=CARTESIAN_POINT('Ctrl Pts',(10.4320843689999,11.6,-1.18407668000002));
#188078=CARTESIAN_POINT('Ctrl Pts',(10.4337941069999,15.2,-1.18396782000001));
#188079=CARTESIAN_POINT('Ctrl Pts',(10.4337941069999,11.6,-1.18396782000001));
#188080=CARTESIAN_POINT('Ctrl Pts',(10.4355113499999,15.2,-1.18385688100001));
#188081=CARTESIAN_POINT('Ctrl Pts',(10.4355113499999,11.6,-1.18385688100001));
#188082=CARTESIAN_POINT('Ctrl Pts',(10.4372360809999,15.2,-1.18374385200001));
#188083=CARTESIAN_POINT('Ctrl Pts',(10.4372360809999,11.6,-1.18374385200001));
#188084=CARTESIAN_POINT('Ctrl Pts',(10.4389682809999,15.2,-1.18362871900001));
#188085=CARTESIAN_POINT('Ctrl Pts',(10.4389682809999,11.6,-1.18362871900001));
#188086=CARTESIAN_POINT('Ctrl Pts',(10.4407079299999,15.2,-1.18351147300002));
#188087=CARTESIAN_POINT('Ctrl Pts',(10.4407079299999,11.6,-1.18351147300002));
#188088=CARTESIAN_POINT('Ctrl Pts',(10.4424550129999,15.2,-1.18339210200002));
#188089=CARTESIAN_POINT('Ctrl Pts',(10.4424550129999,11.6,-1.18339210200002));
#188090=CARTESIAN_POINT('Ctrl Pts',(10.4442095079999,15.2,-1.18327059300002));
#188091=CARTESIAN_POINT('Ctrl Pts',(10.4442095079999,11.6,-1.18327059300002));
#188092=CARTESIAN_POINT('Ctrl Pts',(10.4459713999999,15.2,-1.18314693600002));
#188093=CARTESIAN_POINT('Ctrl Pts',(10.4459713999999,11.6,-1.18314693600002));
#188094=CARTESIAN_POINT('Ctrl Pts',(10.4477406689999,15.2,-1.18302111900002));
#188095=CARTESIAN_POINT('Ctrl Pts',(10.4477406689999,11.6,-1.18302111900002));
#188096=CARTESIAN_POINT('Ctrl Pts',(10.4495172989999,15.2,-1.18289313000002));
#188097=CARTESIAN_POINT('Ctrl Pts',(10.4495172989999,11.6,-1.18289313000002));
#188098=CARTESIAN_POINT('Ctrl Pts',(10.4513012699999,15.2,-1.18276295800001));
#188099=CARTESIAN_POINT('Ctrl Pts',(10.4513012699999,11.6,-1.18276295800001));
#188100=CARTESIAN_POINT('Ctrl Pts',(10.4530925649999,15.2,-1.18263059300002));
#188101=CARTESIAN_POINT('Ctrl Pts',(10.4530925649999,11.6,-1.18263059300002));
#188102=CARTESIAN_POINT('Ctrl Pts',(10.4548911669999,15.2,-1.18249602100001));
#188103=CARTESIAN_POINT('Ctrl Pts',(10.4548911669999,11.6,-1.18249602100002));
#188104=CARTESIAN_POINT('Ctrl Pts',(10.4566970559999,15.2,-1.18235923400002));
#188105=CARTESIAN_POINT('Ctrl Pts',(10.4566970559999,11.6,-1.18235923400002));
#188106=CARTESIAN_POINT('Ctrl Pts',(10.4585102169999,15.2,-1.18222021800001));
#188107=CARTESIAN_POINT('Ctrl Pts',(10.4585102169999,11.6,-1.18222021800001));
#188108=CARTESIAN_POINT('Ctrl Pts',(10.4603306309999,15.2,-1.18207896400001));
#188109=CARTESIAN_POINT('Ctrl Pts',(10.4603306309999,11.6,-1.18207896400001));
#188110=CARTESIAN_POINT('Ctrl Pts',(10.4621582789999,15.2,-1.18193546000001));
#188111=CARTESIAN_POINT('Ctrl Pts',(10.4621582789999,11.6,-1.18193546000001));
#188112=CARTESIAN_POINT('Ctrl Pts',(10.4639931469999,15.2,-1.18178969500002));
#188113=CARTESIAN_POINT('Ctrl Pts',(10.4639931469999,11.6,-1.18178969500002));
#188114=CARTESIAN_POINT('Ctrl Pts',(10.4658352139999,15.2,-1.18164165800001));
#188115=CARTESIAN_POINT('Ctrl Pts',(10.4658352139999,11.6,-1.18164165800001));
#188116=CARTESIAN_POINT('Ctrl Pts',(10.4676844649999,15.2,-1.18149133900001));
#188117=CARTESIAN_POINT('Ctrl Pts',(10.4676844649999,11.6,-1.18149133900001));
#188118=CARTESIAN_POINT('Ctrl Pts',(10.4695408809999,15.2,-1.18133872700001));
#188119=CARTESIAN_POINT('Ctrl Pts',(10.4695408809999,11.6,-1.18133872700001));
#188120=CARTESIAN_POINT('Ctrl Pts',(10.4714044449999,15.2,-1.18118380800002));
#188121=CARTESIAN_POINT('Ctrl Pts',(10.4714044449999,11.6,-1.18118380800002));
#188122=CARTESIAN_POINT('Ctrl Pts',(10.4732751399999,15.2,-1.18102657700002));
#188123=CARTESIAN_POINT('Ctrl Pts',(10.4732751399999,11.6,-1.18102657700002));
#188124=CARTESIAN_POINT('Ctrl Pts',(10.4751529499999,15.2,-1.18086701800001));
#188125=CARTESIAN_POINT('Ctrl Pts',(10.4751529499999,11.6,-1.18086701800001));
#188126=CARTESIAN_POINT('Ctrl Pts',(10.4770378569999,15.2,-1.18070512400001));
#188127=CARTESIAN_POINT('Ctrl Pts',(10.4770378569999,11.6,-1.18070512400001));
#188128=CARTESIAN_POINT('Ctrl Pts',(10.4789298419999,15.2,-1.18054088200001));
#188129=CARTESIAN_POINT('Ctrl Pts',(10.4789298419999,11.6,-1.18054088200001));
#188130=CARTESIAN_POINT('Ctrl Pts',(10.4808288909999,15.2,-1.18037428300001));
#188131=CARTESIAN_POINT('Ctrl Pts',(10.4808288909999,11.6,-1.18037428300001));
#188132=CARTESIAN_POINT('Ctrl Pts',(10.4827349849999,15.2,-1.18020531600001));
#188133=CARTESIAN_POINT('Ctrl Pts',(10.4827349849999,11.6,-1.18020531600001));
#188134=CARTESIAN_POINT('Ctrl Pts',(10.4846481079999,15.2,-1.18003397000002));
#188135=CARTESIAN_POINT('Ctrl Pts',(10.4846481079999,11.6,-1.18003397000002));
#188136=CARTESIAN_POINT('Ctrl Pts',(10.4865682419999,15.2,-1.17986023500002));
#188137=CARTESIAN_POINT('Ctrl Pts',(10.4865682419999,11.6,-1.17986023500002));
#188138=CARTESIAN_POINT('Ctrl Pts',(10.4884953719999,15.2,-1.17968410100001));
#188139=CARTESIAN_POINT('Ctrl Pts',(10.4884953719999,11.6,-1.17968410100001));
#188140=CARTESIAN_POINT('Ctrl Pts',(10.4904294789999,15.2,-1.17950555700002));
#188141=CARTESIAN_POINT('Ctrl Pts',(10.4904294789999,11.6,-1.17950555700002));
#188142=CARTESIAN_POINT('Ctrl Pts',(10.4923705489999,15.2,-1.17932459300001));
#188143=CARTESIAN_POINT('Ctrl Pts',(10.4923705489999,11.6,-1.17932459300001));
#188144=CARTESIAN_POINT('Ctrl Pts',(10.4943185629999,15.2,-1.17914119900002));
#188145=CARTESIAN_POINT('Ctrl Pts',(10.4943185629999,11.6,-1.17914119900002));
#188146=CARTESIAN_POINT('Ctrl Pts',(10.4962735059999,15.2,-1.17895536500002));
#188147=CARTESIAN_POINT('Ctrl Pts',(10.4962735059999,11.6,-1.17895536500002));
#188148=CARTESIAN_POINT('Ctrl Pts',(10.4982353589999,15.2,-1.17876708100002));
#188149=CARTESIAN_POINT('Ctrl Pts',(10.4982353589999,11.6,-1.17876708100002));
#188150=CARTESIAN_POINT('Ctrl Pts',(10.5002041069999,15.2,-1.17857633500002));
#188151=CARTESIAN_POINT('Ctrl Pts',(10.5002041069999,11.6,-1.17857633500002));
#188152=CARTESIAN_POINT('Ctrl Pts',(10.5021797349999,15.2,-1.17838311900002));
#188153=CARTESIAN_POINT('Ctrl Pts',(10.5021797349999,11.6,-1.17838311900002));
#188154=CARTESIAN_POINT('Ctrl Pts',(10.5041622239999,15.2,-1.17818742300001));
#188155=CARTESIAN_POINT('Ctrl Pts',(10.5041622239999,11.6,-1.17818742300001));
#188156=CARTESIAN_POINT('Ctrl Pts',(10.5061515589999,15.2,-1.17798923500001));
#188157=CARTESIAN_POINT('Ctrl Pts',(10.5061515589999,11.6,-1.17798923500001));
#188158=CARTESIAN_POINT('Ctrl Pts',(10.5081477229999,15.2,-1.17778854800001));
#188159=CARTESIAN_POINT('Ctrl Pts',(10.5081477229999,11.6,-1.17778854800001));
#188160=CARTESIAN_POINT('Ctrl Pts',(10.5101507009999,15.2,-1.17758535000001));
#188161=CARTESIAN_POINT('Ctrl Pts',(10.5101507009999,11.6,-1.17758535000001));
#188162=CARTESIAN_POINT('Ctrl Pts',(10.5121604749999,15.2,-1.17737963100002));
#188163=CARTESIAN_POINT('Ctrl Pts',(10.5121604749999,11.6,-1.17737963100002));
#188164=CARTESIAN_POINT('Ctrl Pts',(10.5141770299999,15.2,-1.17717138300002));
#188165=CARTESIAN_POINT('Ctrl Pts',(10.5141770299999,11.6,-1.17717138300002));
#188166=CARTESIAN_POINT('Ctrl Pts',(10.5162003509999,15.2,-1.17696059400001));
#188167=CARTESIAN_POINT('Ctrl Pts',(10.5162003509999,11.6,-1.17696059400001));
#188168=CARTESIAN_POINT('Ctrl Pts',(10.5182304179999,15.2,-1.17674725700001));
#188169=CARTESIAN_POINT('Ctrl Pts',(10.5182304179999,11.6,-1.17674725700002));
#188170=CARTESIAN_POINT('Ctrl Pts',(10.5202672189999,15.2,-1.17653135900001));
#188171=CARTESIAN_POINT('Ctrl Pts',(10.5202672189999,11.6,-1.17653135900001));
#188172=CARTESIAN_POINT('Ctrl Pts',(10.5223107349999,15.2,-1.17631289400002));
#188173=CARTESIAN_POINT('Ctrl Pts',(10.5223107349999,11.6,-1.17631289400002));
#188174=CARTESIAN_POINT('Ctrl Pts',(10.5243609529999,15.2,-1.17609185000001));
#188175=CARTESIAN_POINT('Ctrl Pts',(10.5243609529999,11.6,-1.17609185000001));
#188176=CARTESIAN_POINT('Ctrl Pts',(10.5264178549999,15.2,-1.17586821900002));
#188177=CARTESIAN_POINT('Ctrl Pts',(10.5264178549999,11.6,-1.17586821900002));
#188178=CARTESIAN_POINT('Ctrl Pts',(10.5284814249999,15.2,-1.17564198900002));
#188179=CARTESIAN_POINT('Ctrl Pts',(10.5284814249999,11.6,-1.17564198900002));
#188180=CARTESIAN_POINT('Ctrl Pts',(10.5305516489999,15.2,-1.17541315300001));
#188181=CARTESIAN_POINT('Ctrl Pts',(10.5305516489999,11.6,-1.17541315300001));
#188182=CARTESIAN_POINT('Ctrl Pts',(10.5326285089999,15.2,-1.17518170100002));
#188183=CARTESIAN_POINT('Ctrl Pts',(10.5326285089999,11.6,-1.17518170100002));
#188184=CARTESIAN_POINT('Ctrl Pts',(10.5347119909999,15.2,-1.17494762200002));
#188185=CARTESIAN_POINT('Ctrl Pts',(10.5347119909999,11.6,-1.17494762200002));
#188186=CARTESIAN_POINT('Ctrl Pts',(10.5368020779999,15.2,-1.17471091000001));
#188187=CARTESIAN_POINT('Ctrl Pts',(10.5368020779999,11.6,-1.17471091000001));
#188188=CARTESIAN_POINT('Ctrl Pts',(10.5388987559999,15.2,-1.17447155300002));
#188189=CARTESIAN_POINT('Ctrl Pts',(10.5388987559999,11.6,-1.17447155300002));
#188190=CARTESIAN_POINT('Ctrl Pts',(10.5410020069999,15.2,-1.17422954100002));
#188191=CARTESIAN_POINT('Ctrl Pts',(10.5410020069999,11.6,-1.17422954100002));
#188192=CARTESIAN_POINT('Ctrl Pts',(10.5431118179999,15.2,-1.17398486800001));
#188193=CARTESIAN_POINT('Ctrl Pts',(10.5431118179999,11.6,-1.17398486800001));
#188194=CARTESIAN_POINT('Ctrl Pts',(10.5452281719999,15.2,-1.17373752300002));
#188195=CARTESIAN_POINT('Ctrl Pts',(10.5452281719999,11.6,-1.17373752300002));
#188196=CARTESIAN_POINT('Ctrl Pts',(10.5473510539999,15.2,-1.17348749700001));
#188197=CARTESIAN_POINT('Ctrl Pts',(10.5473510539999,11.6,-1.17348749700001));
#188198=CARTESIAN_POINT('Ctrl Pts',(10.5494804499999,15.2,-1.17323478000001));
#188199=CARTESIAN_POINT('Ctrl Pts',(10.5494804499999,11.6,-1.17323478000001));
#188200=CARTESIAN_POINT('Ctrl Pts',(10.5516163409999,15.2,-1.17297936500002));
#188201=CARTESIAN_POINT('Ctrl Pts',(10.5516163409999,11.6,-1.17297936500002));
#188202=CARTESIAN_POINT('Ctrl Pts',(10.5537587149999,15.2,-1.17272124100001));
#188203=CARTESIAN_POINT('Ctrl Pts',(10.5537587149999,11.6,-1.17272124100001));
#188204=CARTESIAN_POINT('Ctrl Pts',(10.5559075549999,15.2,-1.17246040000001));
#188205=CARTESIAN_POINT('Ctrl Pts',(10.5559075549999,11.6,-1.17246040000001));
#188206=CARTESIAN_POINT('Ctrl Pts',(10.5580628449999,15.2,-1.17219683300001));
#188207=CARTESIAN_POINT('Ctrl Pts',(10.5580628449999,11.6,-1.17219683300001));
#188208=CARTESIAN_POINT('Ctrl Pts',(10.5602245729999,15.2,-1.17193053100001));
#188209=CARTESIAN_POINT('Ctrl Pts',(10.5602245729999,11.6,-1.17193053100001));
#188210=CARTESIAN_POINT('Ctrl Pts',(10.5623927209999,15.2,-1.17166148400001));
#188211=CARTESIAN_POINT('Ctrl Pts',(10.5623927209999,11.6,-1.17166148400001));
#188212=CARTESIAN_POINT('Ctrl Pts',(10.5645672749999,15.2,-1.17138968500001));
#188213=CARTESIAN_POINT('Ctrl Pts',(10.5645672749999,11.6,-1.17138968500001));
#188214=CARTESIAN_POINT('Ctrl Pts',(10.5667482189999,15.2,-1.17111512500002));
#188215=CARTESIAN_POINT('Ctrl Pts',(10.5667482189999,11.6,-1.17111512500002));
#188216=CARTESIAN_POINT('Ctrl Pts',(10.5689355399999,15.2,-1.17083779400001));
#188217=CARTESIAN_POINT('Ctrl Pts',(10.5689355399999,11.6,-1.17083779400002));
#188218=CARTESIAN_POINT('Ctrl Pts',(10.5711292199999,15.2,-1.17055768500002));
#188219=CARTESIAN_POINT('Ctrl Pts',(10.5711292199999,11.6,-1.17055768500002));
#188220=CARTESIAN_POINT('Ctrl Pts',(10.5733292469999,15.2,-1.17027478700001));
#188221=CARTESIAN_POINT('Ctrl Pts',(10.5733292469999,11.6,-1.17027478700001));
#188222=CARTESIAN_POINT('Ctrl Pts',(10.5755356029999,15.2,-1.16998909400001));
#188223=CARTESIAN_POINT('Ctrl Pts',(10.5755356029999,11.6,-1.16998909400001));
#188224=CARTESIAN_POINT('Ctrl Pts',(10.5777482769999,15.2,-1.16970059500002));
#188225=CARTESIAN_POINT('Ctrl Pts',(10.5777482769999,11.6,-1.16970059500002));
#188226=CARTESIAN_POINT('Ctrl Pts',(10.5799672509999,15.2,-1.16940928300002));
#188227=CARTESIAN_POINT('Ctrl Pts',(10.5799672509999,11.6,-1.16940928300002));
#188228=CARTESIAN_POINT('Ctrl Pts',(10.5821925109999,15.2,-1.16911515000002));
#188229=CARTESIAN_POINT('Ctrl Pts',(10.5821925109999,11.6,-1.16911515000002));
#188230=CARTESIAN_POINT('Ctrl Pts',(10.5844240429999,15.2,-1.16881818500001));
#188231=CARTESIAN_POINT('Ctrl Pts',(10.5844240429999,11.6,-1.16881818500001));
#188232=CARTESIAN_POINT('Ctrl Pts',(10.5866618309999,15.2,-1.16851838200001));
#188233=CARTESIAN_POINT('Ctrl Pts',(10.5866618309999,11.6,-1.16851838200001));
#188234=CARTESIAN_POINT('Ctrl Pts',(10.5889058619999,15.2,-1.16821573000002));
#188235=CARTESIAN_POINT('Ctrl Pts',(10.5889058619999,11.6,-1.16821573000002));
#188236=CARTESIAN_POINT('Ctrl Pts',(10.5911561199999,15.2,-1.16791022400001));
#188237=CARTESIAN_POINT('Ctrl Pts',(10.5911561199999,11.6,-1.16791022400002));
#188238=CARTESIAN_POINT('Ctrl Pts',(10.5934125899999,15.2,-1.16760185300001));
#188239=CARTESIAN_POINT('Ctrl Pts',(10.5934125899999,11.6,-1.16760185300001));
#188240=CARTESIAN_POINT('Ctrl Pts',(10.5956752579999,15.2,-1.16729060900001));
#188241=CARTESIAN_POINT('Ctrl Pts',(10.5956752579999,11.6,-1.16729060900001));
#188242=CARTESIAN_POINT('Ctrl Pts',(10.5979441109999,15.2,-1.16697648600002));
#188243=CARTESIAN_POINT('Ctrl Pts',(10.5979441109999,11.6,-1.16697648600002));
#188244=CARTESIAN_POINT('Ctrl Pts',(10.6002191329999,15.2,-1.16665947300001));
#188245=CARTESIAN_POINT('Ctrl Pts',(10.6002191329999,11.6,-1.16665947300001));
#188246=CARTESIAN_POINT('Ctrl Pts',(10.6025003099999,15.2,-1.16633956200001));
#188247=CARTESIAN_POINT('Ctrl Pts',(10.6025003099999,11.6,-1.16633956200001));
#188248=CARTESIAN_POINT('Ctrl Pts',(10.6047876269999,15.2,-1.16601674700001));
#188249=CARTESIAN_POINT('Ctrl Pts',(10.6047876269999,11.6,-1.16601674700001));
#188250=CARTESIAN_POINT('Ctrl Pts',(10.6070810689999,15.2,-1.16569101700001));
#188251=CARTESIAN_POINT('Ctrl Pts',(10.6070810689999,11.6,-1.16569101700001));
#188252=CARTESIAN_POINT('Ctrl Pts',(10.6093806239999,15.2,-1.16536236600002));
#188253=CARTESIAN_POINT('Ctrl Pts',(10.6093806239999,11.6,-1.16536236600002));
#188254=CARTESIAN_POINT('Ctrl Pts',(10.6116862759999,15.2,-1.16503078600001));
#188255=CARTESIAN_POINT('Ctrl Pts',(10.6116862759999,11.6,-1.16503078600001));
#188256=CARTESIAN_POINT('Ctrl Pts',(10.6139980099999,15.2,-1.16469626700002));
#188257=CARTESIAN_POINT('Ctrl Pts',(10.6139980099999,11.6,-1.16469626700002));
#188258=CARTESIAN_POINT('Ctrl Pts',(10.6163158139999,15.2,-1.16435880300001));
#188259=CARTESIAN_POINT('Ctrl Pts',(10.6163158139999,11.6,-1.16435880300001));
#188260=CARTESIAN_POINT('Ctrl Pts',(10.6186396719999,15.2,-1.16401838500002));
#188261=CARTESIAN_POINT('Ctrl Pts',(10.6186396719999,11.6,-1.16401838500002));
#188262=CARTESIAN_POINT('Ctrl Pts',(10.6209695709999,15.2,-1.16367500400001));
#188263=CARTESIAN_POINT('Ctrl Pts',(10.6209695709999,11.6,-1.16367500400001));
#188264=CARTESIAN_POINT('Ctrl Pts',(10.6233054959999,15.2,-1.16332865400001));
#188265=CARTESIAN_POINT('Ctrl Pts',(10.6233054959999,11.6,-1.16332865400001));
#188266=CARTESIAN_POINT('Ctrl Pts',(10.6256474329999,15.2,-1.16297932800002));
#188267=CARTESIAN_POINT('Ctrl Pts',(10.6256474329999,11.6,-1.16297932800002));
#188268=CARTESIAN_POINT('Ctrl Pts',(10.6279953679999,15.2,-1.16262701600002));
#188269=CARTESIAN_POINT('Ctrl Pts',(10.6279953679999,11.6,-1.16262701600002));
#188270=CARTESIAN_POINT('Ctrl Pts',(10.6303492879999,15.2,-1.16227170900002));
#188271=CARTESIAN_POINT('Ctrl Pts',(10.6303492879999,11.6,-1.16227170900002));
#188272=CARTESIAN_POINT('Ctrl Pts',(10.6327091779999,15.2,-1.16191340300002));
#188273=CARTESIAN_POINT('Ctrl Pts',(10.6327091779999,11.6,-1.16191340300002));
#188274=CARTESIAN_POINT('Ctrl Pts',(10.6350750239999,15.2,-1.16155208700001));
#188275=CARTESIAN_POINT('Ctrl Pts',(10.6350750239999,11.6,-1.16155208700001));
#188276=CARTESIAN_POINT('Ctrl Pts',(10.6374468119999,15.2,-1.16118775500002));
#188277=CARTESIAN_POINT('Ctrl Pts',(10.6374468119999,11.6,-1.16118775500002));
#188278=CARTESIAN_POINT('Ctrl Pts',(10.6398245289999,15.2,-1.16082039900002));
#188279=CARTESIAN_POINT('Ctrl Pts',(10.6398245289999,11.6,-1.16082039900002));
#188280=CARTESIAN_POINT('Ctrl Pts',(10.6422081599999,15.2,-1.16045001000002));
#188281=CARTESIAN_POINT('Ctrl Pts',(10.6422081599999,11.6,-1.16045001000002));
#188282=CARTESIAN_POINT('Ctrl Pts',(10.6445976929999,15.2,-1.16007658200001));
#188283=CARTESIAN_POINT('Ctrl Pts',(10.6445976929999,11.6,-1.16007658200001));
#188284=CARTESIAN_POINT('Ctrl Pts',(10.6469931119999,15.2,-1.15970010800002));
#188285=CARTESIAN_POINT('Ctrl Pts',(10.6469931119999,11.6,-1.15970010800002));
#188286=CARTESIAN_POINT('Ctrl Pts',(10.6493944039999,15.2,-1.15932057900002));
#188287=CARTESIAN_POINT('Ctrl Pts',(10.6493944039999,11.6,-1.15932057900002));
#188288=CARTESIAN_POINT('Ctrl Pts',(10.6518015559999,15.2,-1.15893798700001));
#188289=CARTESIAN_POINT('Ctrl Pts',(10.6518015559999,11.6,-1.15893798700002));
#188290=CARTESIAN_POINT('Ctrl Pts',(10.6542145539999,15.2,-1.15855232600001));
#188291=CARTESIAN_POINT('Ctrl Pts',(10.6542145539999,11.6,-1.15855232600001));
#188292=CARTESIAN_POINT('Ctrl Pts',(10.6566333849999,15.2,-1.15816358900001));
#188293=CARTESIAN_POINT('Ctrl Pts',(10.6566333849999,11.6,-1.15816358900001));
#188294=CARTESIAN_POINT('Ctrl Pts',(10.6590580339999,15.2,-1.15777176500002));
#188295=CARTESIAN_POINT('Ctrl Pts',(10.6590580339999,11.6,-1.15777176500002));
#188296=CARTESIAN_POINT('Ctrl Pts',(10.6614884869999,15.2,-1.15737685100001));
#188297=CARTESIAN_POINT('Ctrl Pts',(10.6614884869999,11.6,-1.15737685100001));
#188298=CARTESIAN_POINT('Ctrl Pts',(10.6639247329999,15.2,-1.15697883600001));
#188299=CARTESIAN_POINT('Ctrl Pts',(10.6639247329999,11.6,-1.15697883600001));
#188300=CARTESIAN_POINT('Ctrl Pts',(10.6663667569999,15.2,-1.15657771500001));
#188301=CARTESIAN_POINT('Ctrl Pts',(10.6663667569999,11.6,-1.15657771500001));
#188302=CARTESIAN_POINT('Ctrl Pts',(10.6688145439999,15.2,-1.15617348100002));
#188303=CARTESIAN_POINT('Ctrl Pts',(10.6688145439999,11.6,-1.15617348100002));
#188304=CARTESIAN_POINT('Ctrl Pts',(10.6712680829999,15.2,-1.15576612400002));
#188305=CARTESIAN_POINT('Ctrl Pts',(10.6712680829999,11.6,-1.15576612400002));
#188306=CARTESIAN_POINT('Ctrl Pts',(10.6737273609999,15.2,-1.15535563900002));
#188307=CARTESIAN_POINT('Ctrl Pts',(10.6737273609999,11.6,-1.15535563900002));
#188308=CARTESIAN_POINT('Ctrl Pts',(10.6761923619999,15.2,-1.15494201900002));
#188309=CARTESIAN_POINT('Ctrl Pts',(10.6761923619999,11.6,-1.15494201900002));
#188310=CARTESIAN_POINT('Ctrl Pts',(10.6786630739999,15.2,-1.15452525500002));
#188311=CARTESIAN_POINT('Ctrl Pts',(10.6786630739999,11.6,-1.15452525500002));
#188312=CARTESIAN_POINT('Ctrl Pts',(10.6811394829999,15.2,-1.15410534100001));
#188313=CARTESIAN_POINT('Ctrl Pts',(10.6811394829999,11.6,-1.15410534100001));
#188314=CARTESIAN_POINT('Ctrl Pts',(10.6836215769999,15.2,-1.15368227000001));
#188315=CARTESIAN_POINT('Ctrl Pts',(10.6836215769999,11.6,-1.15368227000001));
#188316=CARTESIAN_POINT('Ctrl Pts',(10.6861093419999,15.2,-1.15325603400001));
#188317=CARTESIAN_POINT('Ctrl Pts',(10.6861093419999,11.6,-1.15325603400001));
#188318=CARTESIAN_POINT('Ctrl Pts',(10.6886027649999,15.2,-1.15282662600002));
#188319=CARTESIAN_POINT('Ctrl Pts',(10.6886027649999,11.6,-1.15282662600002));
#188320=CARTESIAN_POINT('Ctrl Pts',(10.6911018329999,15.2,-1.15239404100001));
#188321=CARTESIAN_POINT('Ctrl Pts',(10.6911018329999,11.6,-1.15239404100001));
#188322=CARTESIAN_POINT('Ctrl Pts',(10.6936065319999,15.2,-1.15195826900001));
#188323=CARTESIAN_POINT('Ctrl Pts',(10.6936065319999,11.6,-1.15195826900001));
#188324=CARTESIAN_POINT('Ctrl Pts',(10.6961168509999,15.2,-1.15151930500001));
#188325=CARTESIAN_POINT('Ctrl Pts',(10.6961168509999,11.6,-1.15151930500002));
#188326=CARTESIAN_POINT('Ctrl Pts',(10.6986327729999,15.2,-1.15107714100001));
#188327=CARTESIAN_POINT('Ctrl Pts',(10.6986327729999,11.6,-1.15107714100001));
#188328=CARTESIAN_POINT('Ctrl Pts',(10.7011542889999,15.2,-1.15063177000001));
#188329=CARTESIAN_POINT('Ctrl Pts',(10.7011542889999,11.6,-1.15063177000002));
#188330=CARTESIAN_POINT('Ctrl Pts',(10.7036813819999,15.2,-1.15018318700002));
#188331=CARTESIAN_POINT('Ctrl Pts',(10.7036813819999,11.6,-1.15018318700002));
#188332=CARTESIAN_POINT('Ctrl Pts',(10.7062140429999,15.2,-1.14973138100002));
#188333=CARTESIAN_POINT('Ctrl Pts',(10.7062140429999,11.6,-1.14973138100002));
#188334=CARTESIAN_POINT('Ctrl Pts',(10.7087522569999,15.2,-1.14927635000001));
#188335=CARTESIAN_POINT('Ctrl Pts',(10.7087522569999,11.6,-1.14927635000001));
#188336=CARTESIAN_POINT('Ctrl Pts',(10.7112960109999,15.2,-1.14881808400002));
#188337=CARTESIAN_POINT('Ctrl Pts',(10.7112960109999,11.6,-1.14881808400002));
#188338=CARTESIAN_POINT('Ctrl Pts',(10.7138452919999,15.2,-1.14835657800001));
#188339=CARTESIAN_POINT('Ctrl Pts',(10.7138452919999,11.6,-1.14835657800001));
#188340=CARTESIAN_POINT('Ctrl Pts',(10.7164000879999,15.2,-1.14789182400001));
#188341=CARTESIAN_POINT('Ctrl Pts',(10.7164000879999,11.6,-1.14789182400001));
#188342=CARTESIAN_POINT('Ctrl Pts',(10.7189603849999,15.2,-1.14742381500001));
#188343=CARTESIAN_POINT('Ctrl Pts',(10.7189603849999,11.6,-1.14742381500002));
#188344=CARTESIAN_POINT('Ctrl Pts',(10.7215261719999,15.2,-1.14695254600001));
#188345=CARTESIAN_POINT('Ctrl Pts',(10.7215261719999,11.6,-1.14695254600001));
#188346=CARTESIAN_POINT('Ctrl Pts',(10.7240974329999,15.2,-1.14647800800002));
#188347=CARTESIAN_POINT('Ctrl Pts',(10.7240974329999,11.6,-1.14647800800002));
#188348=CARTESIAN_POINT('Ctrl Pts',(10.7266741579999,15.2,-1.14600019600001));
#188349=CARTESIAN_POINT('Ctrl Pts',(10.7266741579999,11.6,-1.14600019600001));
#188350=CARTESIAN_POINT('Ctrl Pts',(10.7292563339999,15.2,-1.14551910300001));
#188351=CARTESIAN_POINT('Ctrl Pts',(10.7292563339999,11.6,-1.14551910300001));
#188352=CARTESIAN_POINT('Ctrl Pts',(10.7318439469999,15.2,-1.14503472200001));
#188353=CARTESIAN_POINT('Ctrl Pts',(10.7318439469999,11.6,-1.14503472200001));
#188354=CARTESIAN_POINT('Ctrl Pts',(10.7344369859999,15.2,-1.14454704700002));
#188355=CARTESIAN_POINT('Ctrl Pts',(10.7344369859999,11.6,-1.14454704700002));
#188356=CARTESIAN_POINT('Ctrl Pts',(10.7370354359999,15.2,-1.14405607000001));
#188357=CARTESIAN_POINT('Ctrl Pts',(10.7370354359999,11.6,-1.14405607000002));
#188358=CARTESIAN_POINT('Ctrl Pts',(10.7396392859999,15.2,-1.14356178700001));
#188359=CARTESIAN_POINT('Ctrl Pts',(10.7396392859999,11.6,-1.14356178700001));
#188360=CARTESIAN_POINT('Ctrl Pts',(10.7422485239999,15.2,-1.14306418900001));
#188361=CARTESIAN_POINT('Ctrl Pts',(10.7422485239999,11.6,-1.14306418900001));
#188362=CARTESIAN_POINT('Ctrl Pts',(10.7448631359999,15.2,-1.14256327100001));
#188363=CARTESIAN_POINT('Ctrl Pts',(10.7448631359999,11.6,-1.14256327100001));
#188364=CARTESIAN_POINT('Ctrl Pts',(10.7474831099999,15.2,-1.14205902600002));
#188365=CARTESIAN_POINT('Ctrl Pts',(10.7474831099999,11.6,-1.14205902600002));
#188366=CARTESIAN_POINT('Ctrl Pts',(10.7501084329999,15.2,-1.14155144700002));
#188367=CARTESIAN_POINT('Ctrl Pts',(10.7501084329999,11.6,-1.14155144700002));
#188368=CARTESIAN_POINT('Ctrl Pts',(10.7527390939999,15.2,-1.14104053000001));
#188369=CARTESIAN_POINT('Ctrl Pts',(10.7527390939999,11.6,-1.14104053000002));
#188370=CARTESIAN_POINT('Ctrl Pts',(10.7553750779999,15.2,-1.14052626500001));
#188371=CARTESIAN_POINT('Ctrl Pts',(10.7553750779999,11.6,-1.14052626500001));
#188372=CARTESIAN_POINT('Ctrl Pts',(10.7580163749999,15.2,-1.14000864800001));
#188373=CARTESIAN_POINT('Ctrl Pts',(10.7580163749999,11.6,-1.14000864800001));
#188374=CARTESIAN_POINT('Ctrl Pts',(10.7606629729999,15.2,-1.13948767300001));
#188375=CARTESIAN_POINT('Ctrl Pts',(10.7606629729999,11.6,-1.13948767300002));
#188376=CARTESIAN_POINT('Ctrl Pts',(10.7633148559999,15.2,-1.13896333100001));
#188377=CARTESIAN_POINT('Ctrl Pts',(10.7633148559999,11.6,-1.13896333100001));
#188378=CARTESIAN_POINT('Ctrl Pts',(10.7659720149999,15.2,-1.13843562000001));
#188379=CARTESIAN_POINT('Ctrl Pts',(10.7659720149999,11.6,-1.13843562000001));
#188380=CARTESIAN_POINT('Ctrl Pts',(10.7686344369999,15.2,-1.13790452900002));
#188381=CARTESIAN_POINT('Ctrl Pts',(10.7686344369999,11.6,-1.13790452900002));
#188382=CARTESIAN_POINT('Ctrl Pts',(10.7713021079999,15.2,-1.13737005600001));
#188383=CARTESIAN_POINT('Ctrl Pts',(10.7713021079999,11.6,-1.13737005600001));
#188384=CARTESIAN_POINT('Ctrl Pts',(10.7739750179999,15.2,-1.13683219200002));
#188385=CARTESIAN_POINT('Ctrl Pts',(10.7739750179999,11.6,-1.13683219200002));
#188386=CARTESIAN_POINT('Ctrl Pts',(10.7766531539999,15.2,-1.13629093100001));
#188387=CARTESIAN_POINT('Ctrl Pts',(10.7766531539999,11.6,-1.13629093100002));
#188388=CARTESIAN_POINT('Ctrl Pts',(10.7793365029999,15.2,-1.13574626900002));
#188389=CARTESIAN_POINT('Ctrl Pts',(10.7793365029999,11.6,-1.13574626900002));
#188390=CARTESIAN_POINT('Ctrl Pts',(10.7820250529999,15.2,-1.13519819700001));
#188391=CARTESIAN_POINT('Ctrl Pts',(10.7820250529999,11.6,-1.13519819700001));
#188392=CARTESIAN_POINT('Ctrl Pts',(10.7847187929999,15.2,-1.13464671100001));
#188393=CARTESIAN_POINT('Ctrl Pts',(10.7847187929999,11.6,-1.13464671100001));
#188394=CARTESIAN_POINT('Ctrl Pts',(10.7874177099999,15.2,-1.13409180400001));
#188395=CARTESIAN_POINT('Ctrl Pts',(10.7874177099999,11.6,-1.13409180400002));
#188396=CARTESIAN_POINT('Ctrl Pts',(10.7901217899999,15.2,-1.13353347000002));
#188397=CARTESIAN_POINT('Ctrl Pts',(10.7901217899999,11.6,-1.13353347000002));
#188398=CARTESIAN_POINT('Ctrl Pts',(10.7928310259999,15.2,-1.13297170300001));
#188399=CARTESIAN_POINT('Ctrl Pts',(10.7928310259999,11.6,-1.13297170300001));
#188400=CARTESIAN_POINT('Ctrl Pts',(10.7955453999999,15.2,-1.13240649900002));
#188401=CARTESIAN_POINT('Ctrl Pts',(10.7955453999999,11.6,-1.13240649900002));
#188402=CARTESIAN_POINT('Ctrl Pts',(10.7982649039999,15.2,-1.13183784800002));
#188403=CARTESIAN_POINT('Ctrl Pts',(10.7982649039999,11.6,-1.13183784800002));
#188404=CARTESIAN_POINT('Ctrl Pts',(10.8009895249999,15.2,-1.13126574700001));
#188405=CARTESIAN_POINT('Ctrl Pts',(10.8009895249999,11.6,-1.13126574700001));
#188406=CARTESIAN_POINT('Ctrl Pts',(10.8037192499999,15.2,-1.13069018800001));
#188407=CARTESIAN_POINT('Ctrl Pts',(10.8037192499999,11.6,-1.13069018800001));
#188408=CARTESIAN_POINT('Ctrl Pts',(10.8064540679999,15.2,-1.13011116700001));
#188409=CARTESIAN_POINT('Ctrl Pts',(10.8064540679999,11.6,-1.13011116700001));
#188410=CARTESIAN_POINT('Ctrl Pts',(10.8091939669999,15.2,-1.12952867800002));
#188411=CARTESIAN_POINT('Ctrl Pts',(10.8091939669999,11.6,-1.12952867800002));
#188412=CARTESIAN_POINT('Ctrl Pts',(10.8119389339999,15.2,-1.12894271400001));
#188413=CARTESIAN_POINT('Ctrl Pts',(10.8119389339999,11.6,-1.12894271400001));
#188414=CARTESIAN_POINT('Ctrl Pts',(10.8146889589999,15.2,-1.12835326900001));
#188415=CARTESIAN_POINT('Ctrl Pts',(10.8146889589999,11.6,-1.12835326900001));
#188416=CARTESIAN_POINT('Ctrl Pts',(10.8174440279999,15.2,-1.12776033900001));
#188417=CARTESIAN_POINT('Ctrl Pts',(10.8174440279999,11.6,-1.12776033900001));
#188418=CARTESIAN_POINT('Ctrl Pts',(10.8202041309999,15.2,-1.12716391700001));
#188419=CARTESIAN_POINT('Ctrl Pts',(10.8202041309999,11.6,-1.12716391700001));
#188420=CARTESIAN_POINT('Ctrl Pts',(10.8229692549999,15.2,-1.12656399600001));
#188421=CARTESIAN_POINT('Ctrl Pts',(10.8229692549999,11.6,-1.12656399600001));
#188422=CARTESIAN_POINT('Ctrl Pts',(10.8257393889999,15.2,-1.12596057200001));
#188423=CARTESIAN_POINT('Ctrl Pts',(10.8257393889999,11.6,-1.12596057200001));
#188424=CARTESIAN_POINT('Ctrl Pts',(10.8285145199999,15.2,-1.12535363900002));
#188425=CARTESIAN_POINT('Ctrl Pts',(10.8285145199999,11.6,-1.12535363900002));
#188426=CARTESIAN_POINT('Ctrl Pts',(10.8312946379999,15.2,-1.12474319100001));
#188427=CARTESIAN_POINT('Ctrl Pts',(10.8312946379999,11.6,-1.12474319100001));
#188428=CARTESIAN_POINT('Ctrl Pts',(10.8340797309999,15.2,-1.12412922200001));
#188429=CARTESIAN_POINT('Ctrl Pts',(10.8340797309999,11.6,-1.12412922200001));
#188430=CARTESIAN_POINT('Ctrl Pts',(10.8368697859999,15.2,-1.12351172700001));
#188431=CARTESIAN_POINT('Ctrl Pts',(10.8368697859999,11.6,-1.12351172700001));
#188432=CARTESIAN_POINT('Ctrl Pts',(10.8396647919999,15.2,-1.12289070000001));
#188433=CARTESIAN_POINT('Ctrl Pts',(10.8396647919999,11.6,-1.12289070000001));
#188434=CARTESIAN_POINT('Ctrl Pts',(10.8424647369999,15.2,-1.12226613600001));
#188435=CARTESIAN_POINT('Ctrl Pts',(10.8424647369999,11.6,-1.12226613600001));
#188436=CARTESIAN_POINT('Ctrl Pts',(10.8452696099999,15.2,-1.12163802800001));
#188437=CARTESIAN_POINT('Ctrl Pts',(10.8452696099999,11.6,-1.12163802800001));
#188438=CARTESIAN_POINT('Ctrl Pts',(10.8480793999999,15.2,-1.12100637100002));
#188439=CARTESIAN_POINT('Ctrl Pts',(10.8480793999999,11.6,-1.12100637100002));
#188440=CARTESIAN_POINT('Ctrl Pts',(10.8508940929999,15.2,-1.12037116000002));
#188441=CARTESIAN_POINT('Ctrl Pts',(10.8508940929999,11.6,-1.12037116000002));
#188442=CARTESIAN_POINT('Ctrl Pts',(10.8537136799999,15.2,-1.11973239000001));
#188443=CARTESIAN_POINT('Ctrl Pts',(10.8537136799999,11.6,-1.11973239000001));
#188444=CARTESIAN_POINT('Ctrl Pts',(10.8565381479999,15.2,-1.11909005300001));
#188445=CARTESIAN_POINT('Ctrl Pts',(10.8565381479999,11.6,-1.11909005300001));
#188446=CARTESIAN_POINT('Ctrl Pts',(10.8593674859999,15.2,-1.11844414700002));
#188447=CARTESIAN_POINT('Ctrl Pts',(10.8593674859999,11.6,-1.11844414700002));
#188448=CARTESIAN_POINT('Ctrl Pts',(10.8622016829999,15.2,-1.11779466300002));
#188449=CARTESIAN_POINT('Ctrl Pts',(10.8622016829999,11.6,-1.11779466300002));
#188450=CARTESIAN_POINT('Ctrl Pts',(10.8650407269999,15.2,-1.11714159800002));
#188451=CARTESIAN_POINT('Ctrl Pts',(10.8650407269999,11.6,-1.11714159800002));
#188452=CARTESIAN_POINT('Ctrl Pts',(10.8678846049999,15.2,-1.11648494500002));
#188453=CARTESIAN_POINT('Ctrl Pts',(10.8678846049999,11.6,-1.11648494500002));
#188454=CARTESIAN_POINT('Ctrl Pts',(10.8707333089999,15.2,-1.11582470100001));
#188455=CARTESIAN_POINT('Ctrl Pts',(10.8707333089999,11.6,-1.11582470100001));
#188456=CARTESIAN_POINT('Ctrl Pts',(10.8735868239999,15.2,-1.11516085700002));
#188457=CARTESIAN_POINT('Ctrl Pts',(10.8735868239999,11.6,-1.11516085700002));
#188458=CARTESIAN_POINT('Ctrl Pts',(10.8764451419999,15.2,-1.11449341100001));
#188459=CARTESIAN_POINT('Ctrl Pts',(10.8764451419999,11.6,-1.11449341100002));
#188460=CARTESIAN_POINT('Ctrl Pts',(10.8793082489999,15.2,-1.11382235600002));
#188461=CARTESIAN_POINT('Ctrl Pts',(10.8793082489999,11.6,-1.11382235600002));
#188462=CARTESIAN_POINT('Ctrl Pts',(10.8821761349999,15.2,-1.11314768700002));
#188463=CARTESIAN_POINT('Ctrl Pts',(10.8821761349999,11.6,-1.11314768700002));
#188464=CARTESIAN_POINT('Ctrl Pts',(10.8850487879999,15.2,-1.11246939900001));
#188465=CARTESIAN_POINT('Ctrl Pts',(10.8850487879999,11.6,-1.11246939900001));
#188466=CARTESIAN_POINT('Ctrl Pts',(10.8879261969999,15.2,-1.11178748600001));
#188467=CARTESIAN_POINT('Ctrl Pts',(10.8879261969999,11.6,-1.11178748600001));
#188468=CARTESIAN_POINT('Ctrl Pts',(10.8908083519999,15.2,-1.11110194200001));
#188469=CARTESIAN_POINT('Ctrl Pts',(10.8908083519999,11.6,-1.11110194200001));
#188470=CARTESIAN_POINT('Ctrl Pts',(10.8936952389999,15.2,-1.11041276400002));
#188471=CARTESIAN_POINT('Ctrl Pts',(10.8936952389999,11.6,-1.11041276400002));
#188472=CARTESIAN_POINT('Ctrl Pts',(10.8965868489999,15.2,-1.10971994600002));
#188473=CARTESIAN_POINT('Ctrl Pts',(10.8965868489999,11.6,-1.10971994600002));
#188474=CARTESIAN_POINT('Ctrl Pts',(10.8994831699999,15.2,-1.10902348200002));
#188475=CARTESIAN_POINT('Ctrl Pts',(10.8994831699999,11.6,-1.10902348200002));
#188476=CARTESIAN_POINT('Ctrl Pts',(10.9023841919999,15.2,-1.10832336700001));
#188477=CARTESIAN_POINT('Ctrl Pts',(10.9023841919999,11.6,-1.10832336700002));
#188478=CARTESIAN_POINT('Ctrl Pts',(10.9052899019999,15.2,-1.10761959600001));
#188479=CARTESIAN_POINT('Ctrl Pts',(10.9052899019999,11.6,-1.10761959600001));
#188480=CARTESIAN_POINT('Ctrl Pts',(10.9082002889999,15.2,-1.10691216500001));
#188481=CARTESIAN_POINT('Ctrl Pts',(10.9082002889999,11.6,-1.10691216500001));
#188482=CARTESIAN_POINT('Ctrl Pts',(10.9111153429999,15.2,-1.10620106900001));
#188483=CARTESIAN_POINT('Ctrl Pts',(10.9111153429999,11.6,-1.10620106900001));
#188484=CARTESIAN_POINT('Ctrl Pts',(10.9140350519999,15.2,-1.10548629900002));
#188485=CARTESIAN_POINT('Ctrl Pts',(10.9140350519999,11.6,-1.10548629900002));
#188486=CARTESIAN_POINT('Ctrl Pts',(10.9169594059999,15.2,-1.10476785400001));
#188487=CARTESIAN_POINT('Ctrl Pts',(10.9169594059999,11.6,-1.10476785400001));
#188488=CARTESIAN_POINT('Ctrl Pts',(10.9198883929999,15.2,-1.10404572800002));
#188489=CARTESIAN_POINT('Ctrl Pts',(10.9198883929999,11.6,-1.10404572800002));
#188490=CARTESIAN_POINT('Ctrl Pts',(10.9228220029999,15.2,-1.10331991500002));
#188491=CARTESIAN_POINT('Ctrl Pts',(10.9228220029999,11.6,-1.10331991500002));
#188492=CARTESIAN_POINT('Ctrl Pts',(10.9257602229999,15.2,-1.10259041100001));
#188493=CARTESIAN_POINT('Ctrl Pts',(10.9257602229999,11.6,-1.10259041100001));
#188494=CARTESIAN_POINT('Ctrl Pts',(10.9287030449999,15.2,-1.10185721000001));
#188495=CARTESIAN_POINT('Ctrl Pts',(10.9287030449999,11.6,-1.10185721000002));
#188496=CARTESIAN_POINT('Ctrl Pts',(10.9316504549999,15.2,-1.10112030800002));
#188497=CARTESIAN_POINT('Ctrl Pts',(10.9316504549999,11.6,-1.10112030800002));
#188498=CARTESIAN_POINT('Ctrl Pts',(10.9346024439999,15.2,-1.10037969900001));
#188499=CARTESIAN_POINT('Ctrl Pts',(10.9346024439999,11.6,-1.10037969900001));
#188500=CARTESIAN_POINT('Ctrl Pts',(10.9375589989999,15.2,-1.09963538000001));
#188501=CARTESIAN_POINT('Ctrl Pts',(10.9375589989999,11.6,-1.09963538000002));
#188502=CARTESIAN_POINT('Ctrl Pts',(10.9405201119999,15.2,-1.09888734500001));
#188503=CARTESIAN_POINT('Ctrl Pts',(10.9405201119999,11.6,-1.09888734500002));
#188504=CARTESIAN_POINT('Ctrl Pts',(10.9434857709999,15.2,-1.09813558700001));
#188505=CARTESIAN_POINT('Ctrl Pts',(10.9434857709999,11.6,-1.09813558700001));
#188506=CARTESIAN_POINT('Ctrl Pts',(10.9464559649999,15.2,-1.09738010500001));
#188507=CARTESIAN_POINT('Ctrl Pts',(10.9464559649999,11.6,-1.09738010500001));
#188508=CARTESIAN_POINT('Ctrl Pts',(10.9494306809999,15.2,-1.09662089000001));
#188509=CARTESIAN_POINT('Ctrl Pts',(10.9494306809999,11.6,-1.09662089000001));
#188510=CARTESIAN_POINT('Ctrl Pts',(10.9524099109999,15.2,-1.09585794100001));
#188511=CARTESIAN_POINT('Ctrl Pts',(10.9524099109999,11.6,-1.09585794100001));
#188512=CARTESIAN_POINT('Ctrl Pts',(10.9553936439999,15.2,-1.09509125200002));
#188513=CARTESIAN_POINT('Ctrl Pts',(10.9553936439999,11.6,-1.09509125200002));
#188514=CARTESIAN_POINT('Ctrl Pts',(10.9583818679999,15.2,-1.09432081700001));
#188515=CARTESIAN_POINT('Ctrl Pts',(10.9583818679999,11.6,-1.09432081700001));
#188516=CARTESIAN_POINT('Ctrl Pts',(10.9613745729999,15.2,-1.09354663200001));
#188517=CARTESIAN_POINT('Ctrl Pts',(10.9613745729999,11.6,-1.09354663200001));
#188518=CARTESIAN_POINT('Ctrl Pts',(10.9643717479999,15.2,-1.09276869100002));
#188519=CARTESIAN_POINT('Ctrl Pts',(10.9643717479999,11.6,-1.09276869100002));
#188520=CARTESIAN_POINT('Ctrl Pts',(10.9673733819999,15.2,-1.09198699100002));
#188521=CARTESIAN_POINT('Ctrl Pts',(10.9673733819999,11.6,-1.09198699100002));
#188522=CARTESIAN_POINT('Ctrl Pts',(10.9703794639999,15.2,-1.09120152700001));
#188523=CARTESIAN_POINT('Ctrl Pts',(10.9703794639999,11.6,-1.09120152700001));
#188524=CARTESIAN_POINT('Ctrl Pts',(10.9733899849999,15.2,-1.09041229500002));
#188525=CARTESIAN_POINT('Ctrl Pts',(10.9733899849999,11.6,-1.09041229500002));
#188526=CARTESIAN_POINT('Ctrl Pts',(10.9764049329999,15.2,-1.08961928800001));
#188527=CARTESIAN_POINT('Ctrl Pts',(10.9764049329999,11.6,-1.08961928800001));
#188528=CARTESIAN_POINT('Ctrl Pts',(10.9794242969999,15.2,-1.08882250200002));
#188529=CARTESIAN_POINT('Ctrl Pts',(10.9794242969999,11.6,-1.08882250200002));
#188530=CARTESIAN_POINT('Ctrl Pts',(10.9824480679999,15.2,-1.08802193400001));
#188531=CARTESIAN_POINT('Ctrl Pts',(10.9824480679999,11.6,-1.08802193400001));
#188532=CARTESIAN_POINT('Ctrl Pts',(10.9854762329999,15.2,-1.08721757800001));
#188533=CARTESIAN_POINT('Ctrl Pts',(10.9854762329999,11.6,-1.08721757800002));
#188534=CARTESIAN_POINT('Ctrl Pts',(10.9885087839999,15.2,-1.08640943000001));
#188535=CARTESIAN_POINT('Ctrl Pts',(10.9885087839999,11.6,-1.08640943000002));
#188536=CARTESIAN_POINT('Ctrl Pts',(10.9915457079999,15.2,-1.08559748400001));
#188537=CARTESIAN_POINT('Ctrl Pts',(10.9915457079999,11.6,-1.08559748400001));
#188538=CARTESIAN_POINT('Ctrl Pts',(10.9945869969999,15.2,-1.08478173800002));
#188539=CARTESIAN_POINT('Ctrl Pts',(10.9945869969999,11.6,-1.08478173800002));
#188540=CARTESIAN_POINT('Ctrl Pts',(10.9976326369999,15.2,-1.08396218400001));
#188541=CARTESIAN_POINT('Ctrl Pts',(10.9976326369999,11.6,-1.08396218400001));
#188542=CARTESIAN_POINT('Ctrl Pts',(11.0006826209999,15.2,-1.08313882100001));
#188543=CARTESIAN_POINT('Ctrl Pts',(11.0006826209999,11.6,-1.08313882100001));
#188544=CARTESIAN_POINT('Ctrl Pts',(11.0037369369999,15.2,-1.08231164300001));
#188545=CARTESIAN_POINT('Ctrl Pts',(11.0037369369999,11.6,-1.08231164300001));
#188546=CARTESIAN_POINT('Ctrl Pts',(11.0067955739999,15.2,-1.08148064400002));
#188547=CARTESIAN_POINT('Ctrl Pts',(11.0067955739999,11.6,-1.08148064400002));
#188548=CARTESIAN_POINT('Ctrl Pts',(11.0098585239999,15.2,-1.08064582200001));
#188549=CARTESIAN_POINT('Ctrl Pts',(11.0098585239999,11.6,-1.08064582200001));
#188550=CARTESIAN_POINT('Ctrl Pts',(11.0129257729999,15.2,-1.07980717100002));
#188551=CARTESIAN_POINT('Ctrl Pts',(11.0129257729999,11.6,-1.07980717100002));
#188552=CARTESIAN_POINT('Ctrl Pts',(11.0159973129999,15.2,-1.07896468600002));
#188553=CARTESIAN_POINT('Ctrl Pts',(11.0159973129999,11.6,-1.07896468600002));
#188554=CARTESIAN_POINT('Ctrl Pts',(11.0190731309999,15.2,-1.07811836400002));
#188555=CARTESIAN_POINT('Ctrl Pts',(11.0190731309999,11.6,-1.07811836400002));
#188556=CARTESIAN_POINT('Ctrl Pts',(11.0221532199999,15.2,-1.07726820000002));
#188557=CARTESIAN_POINT('Ctrl Pts',(11.0221532199999,11.6,-1.07726820000002));
#188558=CARTESIAN_POINT('Ctrl Pts',(11.0252375679999,15.2,-1.07641419000001));
#188559=CARTESIAN_POINT('Ctrl Pts',(11.0252375679999,11.6,-1.07641419000002));
#188560=CARTESIAN_POINT('Ctrl Pts',(11.0283261659999,15.2,-1.07555632900001));
#188561=CARTESIAN_POINT('Ctrl Pts',(11.0283261659999,11.6,-1.07555632900001));
#188562=CARTESIAN_POINT('Ctrl Pts',(11.0314190009999,15.2,-1.07469461300001));
#188563=CARTESIAN_POINT('Ctrl Pts',(11.0314190009999,11.6,-1.07469461300001));
#188564=CARTESIAN_POINT('Ctrl Pts',(11.0345160639999,15.2,-1.07382903800001));
#188565=CARTESIAN_POINT('Ctrl Pts',(11.0345160639999,11.6,-1.07382903800001));
#188566=CARTESIAN_POINT('Ctrl Pts',(11.0376173449999,15.2,-1.07295959800001));
#188567=CARTESIAN_POINT('Ctrl Pts',(11.0376173449999,11.6,-1.07295959800001));
#188568=CARTESIAN_POINT('Ctrl Pts',(11.0407228349999,15.2,-1.07208629100001));
#188569=CARTESIAN_POINT('Ctrl Pts',(11.0407228349999,11.6,-1.07208629100001));
#188570=CARTESIAN_POINT('Ctrl Pts',(11.0438325199999,15.2,-1.07120911000001));
#188571=CARTESIAN_POINT('Ctrl Pts',(11.0438325199999,11.6,-1.07120911000001));
#188572=CARTESIAN_POINT('Ctrl Pts',(11.0469463939999,15.2,-1.07032805400001));
#188573=CARTESIAN_POINT('Ctrl Pts',(11.0469463939999,11.6,-1.07032805400001));
#188574=CARTESIAN_POINT('Ctrl Pts',(11.0500644439999,15.2,-1.06944311600001));
#188575=CARTESIAN_POINT('Ctrl Pts',(11.0500644439999,11.6,-1.06944311600001));
#188576=CARTESIAN_POINT('Ctrl Pts',(11.0531866599999,15.2,-1.06855429300001));
#188577=CARTESIAN_POINT('Ctrl Pts',(11.0531866599999,11.6,-1.06855429300001));
#188578=CARTESIAN_POINT('Ctrl Pts',(11.0563130319999,15.2,-1.06766158000001));
#188579=CARTESIAN_POINT('Ctrl Pts',(11.0563130319999,11.6,-1.06766158000001));
#188580=CARTESIAN_POINT('Ctrl Pts',(11.0594435509999,15.2,-1.06676497400001));
#188581=CARTESIAN_POINT('Ctrl Pts',(11.0594435509999,11.6,-1.06676497400001));
#188582=CARTESIAN_POINT('Ctrl Pts',(11.0625782069999,15.2,-1.06586447000002));
#188583=CARTESIAN_POINT('Ctrl Pts',(11.0625782069999,11.6,-1.06586447000002));
#188584=CARTESIAN_POINT('Ctrl Pts',(11.0657169879999,15.2,-1.06496006400001));
#188585=CARTESIAN_POINT('Ctrl Pts',(11.0657169879999,11.6,-1.06496006400001));
#188586=CARTESIAN_POINT('Ctrl Pts',(11.0688598849999,15.2,-1.06405175100001));
#188587=CARTESIAN_POINT('Ctrl Pts',(11.0688598849999,11.6,-1.06405175100001));
#188588=CARTESIAN_POINT('Ctrl Pts',(11.0720068879999,15.2,-1.06313952900001));
#188589=CARTESIAN_POINT('Ctrl Pts',(11.0720068879999,11.6,-1.06313952900001));
#188590=CARTESIAN_POINT('Ctrl Pts',(11.0751579869999,15.2,-1.06222339000002));
#188591=CARTESIAN_POINT('Ctrl Pts',(11.0751579869999,11.6,-1.06222339000002));
#188592=CARTESIAN_POINT('Ctrl Pts',(11.0783131709999,15.2,-1.06130333400001));
#188593=CARTESIAN_POINT('Ctrl Pts',(11.0783131709999,11.6,-1.06130333400001));
#188594=CARTESIAN_POINT('Ctrl Pts',(11.0814724299999,15.2,-1.06037935500002));
#188595=CARTESIAN_POINT('Ctrl Pts',(11.0814724299999,11.6,-1.06037935500002));
#188596=CARTESIAN_POINT('Ctrl Pts',(11.0846357549999,15.2,-1.05945144900002));
#188597=CARTESIAN_POINT('Ctrl Pts',(11.0846357549999,11.6,-1.05945144900002));
#188598=CARTESIAN_POINT('Ctrl Pts',(11.0878031359999,15.2,-1.05851961200001));
#188599=CARTESIAN_POINT('Ctrl Pts',(11.0878031359999,11.6,-1.05851961200001));
#188600=CARTESIAN_POINT('Ctrl Pts',(11.0909745619999,15.2,-1.05758384000001));
#188601=CARTESIAN_POINT('Ctrl Pts',(11.0909745619999,11.6,-1.05758384000001));
#188602=CARTESIAN_POINT('Ctrl Pts',(11.0941500229999,15.2,-1.05664412900001));
#188603=CARTESIAN_POINT('Ctrl Pts',(11.0941500229999,11.6,-1.05664412900001));
#188604=CARTESIAN_POINT('Ctrl Pts',(11.0973295109999,15.2,-1.05570047500001));
#188605=CARTESIAN_POINT('Ctrl Pts',(11.0973295109999,11.6,-1.05570047500001));
#188606=CARTESIAN_POINT('Ctrl Pts',(11.1005130129999,15.2,-1.05475287300001));
#188607=CARTESIAN_POINT('Ctrl Pts',(11.1005130129999,11.6,-1.05475287300001));
#188608=CARTESIAN_POINT('Ctrl Pts',(11.1037005219999,15.2,-1.05380132100001));
#188609=CARTESIAN_POINT('Ctrl Pts',(11.1037005219999,11.6,-1.05380132100001));
#188610=CARTESIAN_POINT('Ctrl Pts',(11.1068920249999,15.2,-1.05284581400001));
#188611=CARTESIAN_POINT('Ctrl Pts',(11.1068920249999,11.6,-1.05284581400001));
#188612=CARTESIAN_POINT('Ctrl Pts',(11.1100875149999,15.2,-1.05188634700002));
#188613=CARTESIAN_POINT('Ctrl Pts',(11.1100875149999,11.6,-1.05188634700002));
#188614=CARTESIAN_POINT('Ctrl Pts',(11.1132869809999,15.2,-1.05092291700001));
#188615=CARTESIAN_POINT('Ctrl Pts',(11.1132869809999,11.6,-1.05092291700001));
#188616=CARTESIAN_POINT('Ctrl Pts',(11.1164904129999,15.2,-1.04995552100001));
#188617=CARTESIAN_POINT('Ctrl Pts',(11.1164904129999,11.6,-1.04995552100001));
#188618=CARTESIAN_POINT('Ctrl Pts',(11.1196978009999,15.2,-1.04898415400001));
#188619=CARTESIAN_POINT('Ctrl Pts',(11.1196978009999,11.6,-1.04898415400001));
#188620=CARTESIAN_POINT('Ctrl Pts',(11.1229091349999,15.2,-1.04800881300001));
#188621=CARTESIAN_POINT('Ctrl Pts',(11.1229091349999,11.6,-1.04800881300001));
#188622=CARTESIAN_POINT('Ctrl Pts',(11.1261244069999,15.2,-1.04702949200002));
#188623=CARTESIAN_POINT('Ctrl Pts',(11.1261244069999,11.6,-1.04702949200002));
#188624=CARTESIAN_POINT('Ctrl Pts',(11.1293436049999,15.2,-1.04604618900002));
#188625=CARTESIAN_POINT('Ctrl Pts',(11.1293436049999,11.6,-1.04604618900002));
#188626=CARTESIAN_POINT('Ctrl Pts',(11.1325667189999,15.2,-1.04505890000001));
#188627=CARTESIAN_POINT('Ctrl Pts',(11.1325667189999,11.6,-1.04505890000001));
#188628=CARTESIAN_POINT('Ctrl Pts',(11.1357937419999,15.2,-1.04406762000002));
#188629=CARTESIAN_POINT('Ctrl Pts',(11.1357937419999,11.6,-1.04406762000002));
#188630=CARTESIAN_POINT('Ctrl Pts',(11.1390246609999,15.2,-1.04307234700002));
#188631=CARTESIAN_POINT('Ctrl Pts',(11.1390246609999,11.6,-1.04307234700002));
#188632=CARTESIAN_POINT('Ctrl Pts',(11.1422594689999,15.2,-1.04207307500001));
#188633=CARTESIAN_POINT('Ctrl Pts',(11.1422594689999,11.6,-1.04207307500001));
#188634=CARTESIAN_POINT('Ctrl Pts',(11.1454981539999,15.2,-1.04106980300001));
#188635=CARTESIAN_POINT('Ctrl Pts',(11.1454981539999,11.6,-1.04106980300001));
#188636=CARTESIAN_POINT('Ctrl Pts',(11.1487407069999,15.2,-1.04006252500001));
#188637=CARTESIAN_POINT('Ctrl Pts',(11.1487407069999,11.6,-1.04006252500001));
#188638=CARTESIAN_POINT('Ctrl Pts',(11.1519871189999,15.2,-1.03905123800001));
#188639=CARTESIAN_POINT('Ctrl Pts',(11.1519871189999,11.6,-1.03905123800002));
#188640=CARTESIAN_POINT('Ctrl Pts',(11.1552373799999,15.2,-1.03803593800002));
#188641=CARTESIAN_POINT('Ctrl Pts',(11.1552373799999,11.6,-1.03803593800002));
#188642=CARTESIAN_POINT('Ctrl Pts',(11.1584914799999,15.2,-1.03701662100002));
#188643=CARTESIAN_POINT('Ctrl Pts',(11.1584914799999,11.6,-1.03701662100002));
#188644=CARTESIAN_POINT('Ctrl Pts',(11.1617494109999,15.2,-1.03599328400001));
#188645=CARTESIAN_POINT('Ctrl Pts',(11.1617494109999,11.6,-1.03599328400001));
#188646=CARTESIAN_POINT('Ctrl Pts',(11.1650111599999,15.2,-1.03496592300001));
#188647=CARTESIAN_POINT('Ctrl Pts',(11.1650111599999,11.6,-1.03496592300001));
#188648=CARTESIAN_POINT('Ctrl Pts',(11.1682767209999,15.2,-1.03393453400002));
#188649=CARTESIAN_POINT('Ctrl Pts',(11.1682767209999,11.6,-1.03393453400002));
#188650=CARTESIAN_POINT('Ctrl Pts',(11.1715460819999,15.2,-1.03289911400001));
#188651=CARTESIAN_POINT('Ctrl Pts',(11.1715460819999,11.6,-1.03289911400001));
#188652=CARTESIAN_POINT('Ctrl Pts',(11.1748192339999,15.2,-1.03185965900002));
#188653=CARTESIAN_POINT('Ctrl Pts',(11.1748192339999,11.6,-1.03185965900002));
#188654=CARTESIAN_POINT('Ctrl Pts',(11.1780961679999,15.2,-1.03081616500001));
#188655=CARTESIAN_POINT('Ctrl Pts',(11.1780961679999,11.6,-1.03081616500001));
#188656=CARTESIAN_POINT('Ctrl Pts',(11.1813768729999,15.2,-1.02976862900002));
#188657=CARTESIAN_POINT('Ctrl Pts',(11.1813768729999,11.6,-1.02976862900002));
#188658=CARTESIAN_POINT('Ctrl Pts',(11.1846613419999,15.2,-1.02871704700001));
#188659=CARTESIAN_POINT('Ctrl Pts',(11.1846613419999,11.6,-1.02871704700001));
#188660=CARTESIAN_POINT('Ctrl Pts',(11.1879495629999,15.2,-1.02766141500001));
#188661=CARTESIAN_POINT('Ctrl Pts',(11.1879495629999,11.6,-1.02766141500001));
#188662=CARTESIAN_POINT('Ctrl Pts',(11.1912415279999,15.2,-1.02660173100002));
#188663=CARTESIAN_POINT('Ctrl Pts',(11.1912415279999,11.6,-1.02660173100002));
#188664=CARTESIAN_POINT('Ctrl Pts',(11.1945372269999,15.2,-1.02553798900002));
#188665=CARTESIAN_POINT('Ctrl Pts',(11.1945372269999,11.6,-1.02553798900002));
#188666=CARTESIAN_POINT('Ctrl Pts',(11.1978366499999,15.2,-1.02447018800001));
#188667=CARTESIAN_POINT('Ctrl Pts',(11.1978366499999,11.6,-1.02447018800001));
#188668=CARTESIAN_POINT('Ctrl Pts',(11.2011397889999,15.2,-1.02339832200002));
#188669=CARTESIAN_POINT('Ctrl Pts',(11.2011397889999,11.6,-1.02339832200002));
#188670=CARTESIAN_POINT('Ctrl Pts',(11.2044466319999,15.2,-1.02232239100001));
#188671=CARTESIAN_POINT('Ctrl Pts',(11.2044466319999,11.6,-1.02232239100001));
#188672=CARTESIAN_POINT('Ctrl Pts',(11.2077571719999,15.2,-1.02124238700001));
#188673=CARTESIAN_POINT('Ctrl Pts',(11.2077571719999,11.6,-1.02124238700001));
#188674=CARTESIAN_POINT('Ctrl Pts',(11.2110713989999,15.2,-1.02015830900001));
#188675=CARTESIAN_POINT('Ctrl Pts',(11.2110713989999,11.6,-1.02015830900001));
#188676=CARTESIAN_POINT('Ctrl Pts',(11.2143893039999,15.2,-1.01907015400001));
#188677=CARTESIAN_POINT('Ctrl Pts',(11.2143893039999,11.6,-1.01907015400002));
#188678=CARTESIAN_POINT('Ctrl Pts',(11.2177108769999,15.2,-1.01797791700001));
#188679=CARTESIAN_POINT('Ctrl Pts',(11.2177108769999,11.6,-1.01797791700002));
#188680=CARTESIAN_POINT('Ctrl Pts',(11.2210361069999,15.2,-1.01688159500001));
#188681=CARTESIAN_POINT('Ctrl Pts',(11.2210361069999,11.6,-1.01688159500001));
#188682=CARTESIAN_POINT('Ctrl Pts',(11.2243649869999,15.2,-1.01578118600001));
#188683=CARTESIAN_POINT('Ctrl Pts',(11.2243649869999,11.6,-1.01578118600001));
#188684=CARTESIAN_POINT('Ctrl Pts',(11.2276975069999,15.2,-1.01467668400002));
#188685=CARTESIAN_POINT('Ctrl Pts',(11.2276975069999,11.6,-1.01467668400002));
#188686=CARTESIAN_POINT('Ctrl Pts',(11.2310336579999,15.2,-1.01356808800002));
#188687=CARTESIAN_POINT('Ctrl Pts',(11.2310336579999,11.6,-1.01356808800002));
#188688=CARTESIAN_POINT('Ctrl Pts',(11.2343734289999,15.2,-1.01245539300002));
#188689=CARTESIAN_POINT('Ctrl Pts',(11.2343734289999,11.6,-1.01245539300002));
#188690=CARTESIAN_POINT('Ctrl Pts',(11.2377168129999,15.2,-1.01133859700001));
#188691=CARTESIAN_POINT('Ctrl Pts',(11.2377168129999,11.6,-1.01133859700001));
#188692=CARTESIAN_POINT('Ctrl Pts',(11.2410637989999,15.2,-1.01021769500001));
#188693=CARTESIAN_POINT('Ctrl Pts',(11.2410637989999,11.6,-1.01021769500001));
#188694=CARTESIAN_POINT('Ctrl Pts',(11.2444143789999,15.2,-1.00909268500001));
#188695=CARTESIAN_POINT('Ctrl Pts',(11.2444143789999,11.6,-1.00909268500002));
#188696=CARTESIAN_POINT('Ctrl Pts',(11.2477685419999,15.2,-1.00796356400001));
#188697=CARTESIAN_POINT('Ctrl Pts',(11.2477685419999,11.6,-1.00796356400001));
#188698=CARTESIAN_POINT('Ctrl Pts',(11.2511262799999,15.2,-1.00683032600001));
#188699=CARTESIAN_POINT('Ctrl Pts',(11.2511262799999,11.6,-1.00683032600001));
#188700=CARTESIAN_POINT('Ctrl Pts',(11.2544875849999,15.2,-1.00569297000002));
#188701=CARTESIAN_POINT('Ctrl Pts',(11.2544875849999,11.6,-1.00569297000002));
#188702=CARTESIAN_POINT('Ctrl Pts',(11.2578524459999,15.2,-1.00455149200001));
#188703=CARTESIAN_POINT('Ctrl Pts',(11.2578524459999,11.6,-1.00455149200001));
#188704=CARTESIAN_POINT('Ctrl Pts',(11.2612208539999,15.2,-1.00340589000002));
#188705=CARTESIAN_POINT('Ctrl Pts',(11.2612208539999,11.6,-1.00340589000002));
#188706=CARTESIAN_POINT('Ctrl Pts',(11.2645927989999,15.2,-1.00225615800001));
#188707=CARTESIAN_POINT('Ctrl Pts',(11.2645927989999,11.6,-1.00225615800001));
#188708=CARTESIAN_POINT('Ctrl Pts',(11.2679682739999,15.2,-1.00110229500002));
#188709=CARTESIAN_POINT('Ctrl Pts',(11.2679682739999,11.6,-1.00110229500002));
#188710=CARTESIAN_POINT('Ctrl Pts',(11.2713472679999,15.2,-0.999944297000015));
#188711=CARTESIAN_POINT('Ctrl Pts',(11.2713472679999,11.6,-0.999944297000015));
#188712=CARTESIAN_POINT('Ctrl Pts',(11.2747297729999,15.2,-0.998782161000014));
#188713=CARTESIAN_POINT('Ctrl Pts',(11.2747297729999,11.6,-0.998782161000014));
#188714=CARTESIAN_POINT('Ctrl Pts',(11.2781157789999,15.2,-0.997615884000016));
#188715=CARTESIAN_POINT('Ctrl Pts',(11.2781157789999,11.6,-0.997615884000016));
#188716=CARTESIAN_POINT('Ctrl Pts',(11.2815052779999,15.2,-0.996445462000013));
#188717=CARTESIAN_POINT('Ctrl Pts',(11.2815052779999,11.6,-0.996445462000013));
#188718=CARTESIAN_POINT('Ctrl Pts',(11.2848982589999,15.2,-0.995270892000013));
#188719=CARTESIAN_POINT('Ctrl Pts',(11.2848982589999,11.6,-0.995270892000014));
#188720=CARTESIAN_POINT('Ctrl Pts',(11.2882947149999,15.2,-0.994092171000016));
#188721=CARTESIAN_POINT('Ctrl Pts',(11.2882947149999,11.6,-0.994092171000017));
#188722=CARTESIAN_POINT('Ctrl Pts',(11.2916946349999,15.2,-0.992909297000013));
#188723=CARTESIAN_POINT('Ctrl Pts',(11.2916946349999,11.6,-0.992909297000014));
#188724=CARTESIAN_POINT('Ctrl Pts',(11.2950980119999,15.2,-0.991722263000017));
#188725=CARTESIAN_POINT('Ctrl Pts',(11.2950980119999,11.6,-0.991722263000017));
#188726=CARTESIAN_POINT('Ctrl Pts',(11.2985048339999,15.2,-0.990531071000014));
#188727=CARTESIAN_POINT('Ctrl Pts',(11.2985048339999,11.6,-0.990531071000014));
#188728=CARTESIAN_POINT('Ctrl Pts',(11.3019150959999,15.2,-0.989335715000017));
#188729=CARTESIAN_POINT('Ctrl Pts',(11.3019150959999,11.6,-0.989335715000017));
#188730=CARTESIAN_POINT('Ctrl Pts',(11.3053287859999,15.2,-0.988136191000013));
#188731=CARTESIAN_POINT('Ctrl Pts',(11.3053287859999,11.6,-0.988136191000013));
#188732=CARTESIAN_POINT('Ctrl Pts',(11.3087458949999,15.2,-0.986932498000015));
#188733=CARTESIAN_POINT('Ctrl Pts',(11.3087458949999,11.6,-0.986932498000015));
#188734=CARTESIAN_POINT('Ctrl Pts',(11.3121664159999,15.2,-0.985724632000018));
#188735=CARTESIAN_POINT('Ctrl Pts',(11.3121664159999,11.6,-0.985724632000018));
#188736=CARTESIAN_POINT('Ctrl Pts',(11.3155903389999,15.2,-0.984512590000013));
#188737=CARTESIAN_POINT('Ctrl Pts',(11.3155903389999,11.6,-0.984512590000013));
#188738=CARTESIAN_POINT('Ctrl Pts',(11.3190176529999,15.2,-0.983296370000013));
#188739=CARTESIAN_POINT('Ctrl Pts',(11.3190176529999,11.6,-0.983296370000013));
#188740=CARTESIAN_POINT('Ctrl Pts',(11.3224483519999,15.2,-0.982075966000018));
#188741=CARTESIAN_POINT('Ctrl Pts',(11.3224483519999,11.6,-0.982075966000018));
#188742=CARTESIAN_POINT('Ctrl Pts',(11.3258824259999,15.2,-0.980851377000014));
#188743=CARTESIAN_POINT('Ctrl Pts',(11.3258824259999,11.6,-0.980851377000014));
#188744=CARTESIAN_POINT('Ctrl Pts',(11.3293198659999,15.2,-0.979622601000014));
#188745=CARTESIAN_POINT('Ctrl Pts',(11.3293198659999,11.6,-0.979622601000015));
#188746=CARTESIAN_POINT('Ctrl Pts',(11.3327606619999,15.2,-0.978389632000014));
#188747=CARTESIAN_POINT('Ctrl Pts',(11.3327606619999,11.6,-0.978389632000014));
#188748=CARTESIAN_POINT('Ctrl Pts',(11.3362048069999,15.2,-0.977152470000018));
#188749=CARTESIAN_POINT('Ctrl Pts',(11.3362048069999,11.6,-0.977152470000018));
#188750=CARTESIAN_POINT('Ctrl Pts',(11.3396522919999,15.2,-0.975911111000016));
#188751=CARTESIAN_POINT('Ctrl Pts',(11.3396522919999,11.6,-0.975911111000017));
#188752=CARTESIAN_POINT('Ctrl Pts',(11.3431031069999,15.2,-0.974665551000014));
#188753=CARTESIAN_POINT('Ctrl Pts',(11.3431031069999,11.6,-0.974665551000014));
#188754=CARTESIAN_POINT('Ctrl Pts',(11.3465572429999,15.2,-0.973415788000014));
#188755=CARTESIAN_POINT('Ctrl Pts',(11.3465572429999,11.6,-0.973415788000014));
#188756=CARTESIAN_POINT('Ctrl Pts',(11.3500146919999,15.2,-0.972161819000017));
#188757=CARTESIAN_POINT('Ctrl Pts',(11.3500146919999,11.6,-0.972161819000017));
#188758=CARTESIAN_POINT('Ctrl Pts',(11.3534754439999,15.2,-0.970903641000014));
#188759=CARTESIAN_POINT('Ctrl Pts',(11.3534754439999,11.6,-0.970903641000014));
#188760=CARTESIAN_POINT('Ctrl Pts',(11.3569394909999,15.2,-0.969641251000013));
#188761=CARTESIAN_POINT('Ctrl Pts',(11.3569394909999,11.6,-0.969641251000013));
#188762=CARTESIAN_POINT('Ctrl Pts',(11.3604068239999,15.2,-0.968374645000014));
#188763=CARTESIAN_POINT('Ctrl Pts',(11.3604068239999,11.6,-0.968374645000015));
#188764=CARTESIAN_POINT('Ctrl Pts',(11.3638774359999,15.2,-0.967103822000013));
#188765=CARTESIAN_POINT('Ctrl Pts',(11.3638774359999,11.6,-0.967103822000013));
#188766=CARTESIAN_POINT('Ctrl Pts',(11.3673513139999,15.2,-0.965828778000013));
#188767=CARTESIAN_POINT('Ctrl Pts',(11.3673513139999,11.6,-0.965828778000013));
#188768=CARTESIAN_POINT('Ctrl Pts',(11.3708284529999,15.2,-0.964549510000015));
#188769=CARTESIAN_POINT('Ctrl Pts',(11.3708284529999,11.6,-0.964549510000015));
#188770=CARTESIAN_POINT('Ctrl Pts',(11.3743088439999,15.2,-0.963266017000013));
#188771=CARTESIAN_POINT('Ctrl Pts',(11.3743088439999,11.6,-0.963266017000013));
#188772=CARTESIAN_POINT('Ctrl Pts',(11.3777924759999,15.2,-0.961978293000012));
#188773=CARTESIAN_POINT('Ctrl Pts',(11.3777924759999,11.6,-0.961978293000012));
#188774=CARTESIAN_POINT('Ctrl Pts',(11.3812793429999,15.2,-0.960686338000016));
#188775=CARTESIAN_POINT('Ctrl Pts',(11.3812793429999,11.6,-0.960686338000017));
#188776=CARTESIAN_POINT('Ctrl Pts',(11.3847694349999,15.2,-0.959390147000012));
#188777=CARTESIAN_POINT('Ctrl Pts',(11.3847694349999,11.6,-0.959390147000013));
#188778=CARTESIAN_POINT('Ctrl Pts',(11.3882627429999,15.2,-0.958089719000017));
#188779=CARTESIAN_POINT('Ctrl Pts',(11.3882627429999,11.6,-0.958089719000017));
#188780=CARTESIAN_POINT('Ctrl Pts',(11.3917592569999,15.2,-0.956785049000013));
#188781=CARTESIAN_POINT('Ctrl Pts',(11.3917592569999,11.6,-0.956785049000013));
#188782=CARTESIAN_POINT('Ctrl Pts',(11.3952589699999,15.2,-0.955476136000013));
#188783=CARTESIAN_POINT('Ctrl Pts',(11.3952589699999,11.6,-0.955476136000013));
#188784=CARTESIAN_POINT('Ctrl Pts',(11.3987618709999,15.2,-0.954162977000017));
#188785=CARTESIAN_POINT('Ctrl Pts',(11.3987618709999,11.6,-0.954162977000018));
#188786=CARTESIAN_POINT('Ctrl Pts',(11.4022679529999,15.2,-0.952845568000011));
#188787=CARTESIAN_POINT('Ctrl Pts',(11.4022679529999,11.6,-0.952845568000012));
#188788=CARTESIAN_POINT('Ctrl Pts',(11.4057772069999,15.2,-0.951523906000014));
#188789=CARTESIAN_POINT('Ctrl Pts',(11.4057772069999,11.6,-0.951523906000014));
#188790=CARTESIAN_POINT('Ctrl Pts',(11.4092896249999,15.2,-0.950197991000015));
#188791=CARTESIAN_POINT('Ctrl Pts',(11.4092896249999,11.6,-0.950197991000015));
#188792=CARTESIAN_POINT('Ctrl Pts',(11.4128051999999,15.2,-0.948867819000014));
#188793=CARTESIAN_POINT('Ctrl Pts',(11.4128051999999,11.6,-0.948867819000015));
#188794=CARTESIAN_POINT('Ctrl Pts',(11.4163239239999,15.2,-0.947533387000017));
#188795=CARTESIAN_POINT('Ctrl Pts',(11.4163239239999,11.6,-0.947533387000017));
#188796=CARTESIAN_POINT('Ctrl Pts',(11.4198457879999,15.2,-0.946194694000013));
#188797=CARTESIAN_POINT('Ctrl Pts',(11.4198457879999,11.6,-0.946194694000014));
#188798=CARTESIAN_POINT('Ctrl Pts',(11.4233707839999,15.2,-0.944851734000016));
#188799=CARTESIAN_POINT('Ctrl Pts',(11.4233707839999,11.6,-0.944851734000017));
#188800=CARTESIAN_POINT('Ctrl Pts',(11.4268989019999,15.2,-0.943504507000017));
#188801=CARTESIAN_POINT('Ctrl Pts',(11.4268989019999,11.6,-0.943504507000017));
#188802=CARTESIAN_POINT('Ctrl Pts',(11.4304301309999,15.2,-0.942153010000015));
#188803=CARTESIAN_POINT('Ctrl Pts',(11.4304301309999,11.6,-0.942153010000016));
#188804=CARTESIAN_POINT('Ctrl Pts',(11.4339644589999,15.2,-0.940797237000015));
#188805=CARTESIAN_POINT('Ctrl Pts',(11.4339644589999,11.6,-0.940797237000015));
#188806=CARTESIAN_POINT('Ctrl Pts',(11.4375018779999,15.2,-0.939437187000016));
#188807=CARTESIAN_POINT('Ctrl Pts',(11.4375018779999,11.6,-0.939437187000017));
#188808=CARTESIAN_POINT('Ctrl Pts',(11.4410423789999,15.2,-0.938072856000014));
#188809=CARTESIAN_POINT('Ctrl Pts',(11.4410423789999,11.6,-0.938072856000014));
#188810=CARTESIAN_POINT('Ctrl Pts',(11.4445859519999,15.2,-0.936704241000013));
#188811=CARTESIAN_POINT('Ctrl Pts',(11.4445859519999,11.6,-0.936704241000013));
#188812=CARTESIAN_POINT('Ctrl Pts',(11.4481325909999,15.2,-0.935331342000012));
#188813=CARTESIAN_POINT('Ctrl Pts',(11.4481325909999,11.6,-0.935331342000012));
#188814=CARTESIAN_POINT('Ctrl Pts',(11.4516822949999,15.2,-0.933954156000016));
#188815=CARTESIAN_POINT('Ctrl Pts',(11.4516822949999,11.6,-0.933954156000017));
#188816=CARTESIAN_POINT('Ctrl Pts',(11.4552350599999,15.2,-0.932572684000017));
#188817=CARTESIAN_POINT('Ctrl Pts',(11.4552350599999,11.6,-0.932572684000017));
#188818=CARTESIAN_POINT('Ctrl Pts',(11.4580797199999,15.2,-0.931464077000013));
#188819=CARTESIAN_POINT('Ctrl Pts',(11.4580797199999,11.6,-0.931464077000013));
#188820=CARTESIAN_POINT('Ctrl Pts',(11.4602145909999,15.2,-0.930630693000012));
#188821=CARTESIAN_POINT('Ctrl Pts',(11.4602145909999,11.6,-0.930630693000012));
#188822=CARTESIAN_POINT('Ctrl Pts',(11.4616384499999,15.2,-0.930074246000014));
#188823=CARTESIAN_POINT('Ctrl Pts',(11.4616384499999,11.6,-0.930074246000015));
#188824=CARTESIAN_POINT('Ctrl Pts',(11.4623505329999,15.2,-0.929795809000016));
#188825=CARTESIAN_POINT('Ctrl Pts',(11.4623505329999,11.6,-0.929795809000016));
#188826=CARTESIAN_POINT('Ctrl Pts',(10.3068855239999,15.2,-1.18690176600001));
#188827=CARTESIAN_POINT('Ctrl Pts',(10.3086714467389,15.2,-1.1869528784395));
#188828=CARTESIAN_POINT('Ctrl Pts',(10.3105146691063,15.2,-1.18700024430173));
#188829=CARTESIAN_POINT('Ctrl Pts',(10.3124142310585,15.2,-1.18704320794532));
#188830=CARTESIAN_POINT('Ctrl Pts',(10.3143229536586,15.2,-1.18708637878131));
#188831=CARTESIAN_POINT('Ctrl Pts',(10.3162885628145,15.2,-1.18712509875838));
#188832=CARTESIAN_POINT('Ctrl Pts',(10.3183101246955,15.2,-1.18715870867826));
#188833=CARTESIAN_POINT('Ctrl Pts',(10.3206686132814,15.2,-1.18719792024688));
#188834=CARTESIAN_POINT('Ctrl Pts',(10.3231032554094,15.2,-1.18723017361547));
#188835=CARTESIAN_POINT('Ctrl Pts',(10.3256126114571,15.2,-1.18725445923942));
#188836=CARTESIAN_POINT('Ctrl Pts',(10.3277634883206,15.2,-1.18727527549095));
#188837=CARTESIAN_POINT('Ctrl Pts',(10.3299692556961,15.2,-1.18729023695032));
#188838=CARTESIAN_POINT('Ctrl Pts',(10.3322290309353,15.2,-1.18729873195083));
#188839=CARTESIAN_POINT('Ctrl Pts',(10.3344888059692,15.2,-1.18730722695057));
#188840=CARTESIAN_POINT('Ctrl Pts',(10.3368025915859,15.2,-1.18730925158318));
#188841=CARTESIAN_POINT('Ctrl Pts',(10.3391695234998,15.2,-1.18730421375003));
#188842=CARTESIAN_POINT('Ctrl Pts',(10.3419309442095,15.2,-1.18729833627771));
#188843=CARTESIAN_POINT('Ctrl Pts',(10.3447647053247,15.2,-1.18728284169453));
#188844=CARTESIAN_POINT('Ctrl Pts',(10.3476694772408,15.2,-1.18725682074785));
#188845=CARTESIAN_POINT('Ctrl Pts',(10.3501592816111,15.2,-1.18723451708043));
#188846=CARTESIAN_POINT('Ctrl Pts',(10.3527012581607,15.2,-1.1872044765403));
#188847=CARTESIAN_POINT('Ctrl Pts',(10.3552945932332,15.2,-1.18716614595836));
#188848=CARTESIAN_POINT('Ctrl Pts',(10.3578879283056,15.2,-1.18712781537642));
#188849=CARTESIAN_POINT('Ctrl Pts',(10.3605326202138,15.2,-1.18708119543062));
#188850=CARTESIAN_POINT('Ctrl Pts',(10.3632278754976,15.2,-1.18702574301371));
#188851=CARTESIAN_POINT('Ctrl Pts',(10.3659231310262,15.2,-1.18697029059176));
#188852=CARTESIAN_POINT('Ctrl Pts',(10.3686689482239,15.2,-1.18690600845499));
#188853=CARTESIAN_POINT('Ctrl Pts',(10.3714645527963,15.2,-1.18683237403367));
#188854=CARTESIAN_POINT('Ctrl Pts',(10.3742601571147,15.2,-1.18675873961904));
#188855=CARTESIAN_POINT('Ctrl Pts',(10.3771055475764,15.2,-1.18667575065539));
#188856=CARTESIAN_POINT('Ctrl Pts',(10.3799999659845,15.2,-1.18658290124166));
#188857=CARTESIAN_POINT('Ctrl Pts',(10.3828943843926,15.2,-1.18649005182792));
#188858=CARTESIAN_POINT('Ctrl Pts',(10.3858378311395,15.2,-1.18638734211826));
#188859=CARTESIAN_POINT('Ctrl Pts',(10.388829564612,15.2,-1.18627427795615));
#188860=CARTESIAN_POINT('Ctrl Pts',(10.3918212983563,15.2,-1.18616121378377));
#188861=CARTESIAN_POINT('Ctrl Pts',(10.3948613167899,15.2,-1.18603779600178));
#188862=CARTESIAN_POINT('Ctrl Pts',(10.3979488985448,15.2,-1.18590354674373));
#188863=CARTESIAN_POINT('Ctrl Pts',(10.4010364800191,15.2,-1.18576929749787));
#188864=CARTESIAN_POINT('Ctrl Pts',(10.4041716226371,15.2,-1.18562421472794));
#188865=CARTESIAN_POINT('Ctrl Pts',(10.4073536171901,15.2,-1.18546783648313));
#188866=CARTESIAN_POINT('Ctrl Pts',(10.4105356117432,15.2,-1.18531145823832));
#188867=CARTESIAN_POINT('Ctrl Pts',(10.4137644583592,15.2,-1.1851437827194));
#188868=CARTESIAN_POINT('Ctrl Pts',(10.4170394620716,15.2,-1.18496435772643));
#188869=CARTESIAN_POINT('Ctrl Pts',(10.4214061337872,15.2,-1.18472512439704));
#188870=CARTESIAN_POINT('Ctrl Pts',(10.4258548607992,15.2,-1.18446500339921));
#188871=CARTESIAN_POINT('Ctrl Pts',(10.4303840394047,15.2,-1.1841829592788));
#188872=CARTESIAN_POINT('Ctrl Pts',(10.4343470708002,15.2,-1.18393617066624));
#188873=CARTESIAN_POINT('Ctrl Pts',(10.4383716952584,15.2,-1.18367259643219));
#188874=CARTESIAN_POINT('Ctrl Pts',(10.4424568660582,15.2,-1.18339156752504));
#188875=CARTESIAN_POINT('Ctrl Pts',(10.4465420368579,15.2,-1.18311053861789));
#188876=CARTESIAN_POINT('Ctrl Pts',(10.4506877527646,15.2,-1.18281205483429));
#188877=CARTESIAN_POINT('Ctrl Pts',(10.4548929891403,15.2,-1.18249546717376));
#188878=CARTESIAN_POINT('Ctrl Pts',(10.4584974772753,15.2,-1.18222410633595));
#188879=CARTESIAN_POINT('Ctrl Pts',(10.462145694934,15.2,-1.18193944523087));
#188880=CARTESIAN_POINT('Ctrl Pts',(10.4658370099665,15.2,-1.18164108749171));
#188881=CARTESIAN_POINT('Ctrl Pts',(10.4701435443947,15.2,-1.18129300344462));
#188882=CARTESIAN_POINT('Ctrl Pts',(10.4745087382407,15.2,-1.18092627583869));
#188883=CARTESIAN_POINT('Ctrl Pts',(10.478931608325,15.2,-1.18054029270133));
#188884=CARTESIAN_POINT('Ctrl Pts',(10.4827226396292,15.2,-1.18020945002934));
#188885=CARTESIAN_POINT('Ctrl Pts',(10.486556045599,15.2,-1.17986446165365));
#188886=CARTESIAN_POINT('Ctrl Pts',(10.4904312197082,15.2,-1.17950495200004));
#188887=CARTESIAN_POINT('Ctrl Pts',(10.496243980872,15.2,-1.17896568751964));
#188888=CARTESIAN_POINT('Ctrl Pts',(10.5021507173861,15.2,-1.17839375053718));
#188889=CARTESIAN_POINT('Ctrl Pts',(10.508149426039,15.2,-1.17778792031073));
#188890=CARTESIAN_POINT('Ctrl Pts',(10.5121485655041,15.2,-1.17738403345641));
#188891=CARTESIAN_POINT('Ctrl Pts',(10.516188583465,15.2,-1.17696508170065));
#188892=CARTESIAN_POINT('Ctrl Pts',(10.5202688980224,15.2,-1.1765307171763));
#188893=CARTESIAN_POINT('Ctrl Pts',(10.5250292644502,15.2,-1.17602395862375));
#188894=CARTESIAN_POINT('Ctrl Pts',(10.5298444813069,15.2,-1.17549622163256));
#188895=CARTESIAN_POINT('Ctrl Pts',(10.53471364182,15.2,-1.17494696375136));
#188896=CARTESIAN_POINT('Ctrl Pts',(10.5388872084614,15.2,-1.17447617122677));
#188897=CARTESIAN_POINT('Ctrl Pts',(10.5431004072067,15.2,-1.17398956869235));
#188898=CARTESIAN_POINT('Ctrl Pts',(10.5473526826901,15.2,-1.17348682424757));
#188899=CARTESIAN_POINT('Ctrl Pts',(10.5516049577873,15.2,-1.17298407984847));
#188900=CARTESIAN_POINT('Ctrl Pts',(10.5558963048357,15.2,-1.17246519517489));
#188901=CARTESIAN_POINT('Ctrl Pts',(10.5602261780312,15.2,-1.17192984477528));
#188902=CARTESIAN_POINT('Ctrl Pts',(10.5645560512268,15.2,-1.17139449437567));
#188903=CARTESIAN_POINT('Ctrl Pts',(10.5689244484073,15.2,-1.17084268066522));
#188904=CARTESIAN_POINT('Ctrl Pts',(10.5733308288279,15.2,-1.17027408827035));
#188905=CARTESIAN_POINT('Ctrl Pts',(10.5777372096488,15.2,-1.16970549582383));
#188906=CARTESIAN_POINT('Ctrl Pts',(10.5821815751048,15.2,-1.16912012613898));
#188907=CARTESIAN_POINT('Ctrl Pts',(10.5866633921585,15.2,-1.16851766974172));
#188908=CARTESIAN_POINT('Ctrl Pts',(10.5903982394997,15.2,-1.16801562277137));
#188909=CARTESIAN_POINT('Ctrl Pts',(10.5941590933431,15.2,-1.16750171144334));
#188910=CARTESIAN_POINT('Ctrl Pts',(10.5979456537618,15.2,-1.16697576345625));
#188911=CARTESIAN_POINT('Ctrl Pts',(10.6024895260993,15.2,-1.16634462589466));
#188912=CARTESIAN_POINT('Ctrl Pts',(10.6070704129237,15.2,-1.16569615159527));
#188913=CARTESIAN_POINT('Ctrl Pts',(10.611687796527,15.2,-1.16503005128308));
#188914=CARTESIAN_POINT('Ctrl Pts',(10.6170747443438,15.2,-1.16425293421184));
#188915=CARTESIAN_POINT('Ctrl Pts',(10.6225113698796,15.2,-1.16345182399275));
#188916=CARTESIAN_POINT('Ctrl Pts',(10.6279968647457,15.2,-1.16262626721458));
#188917=CARTESIAN_POINT('Ctrl Pts',(10.632698717244,15.2,-1.16191864715573));
#188918=CARTESIAN_POINT('Ctrl Pts',(10.6374364739733,15.2,-1.16119306829803));
#188919=CARTESIAN_POINT('Ctrl Pts',(10.6422096354665,15.2,-1.16044925024172));
#188920=CARTESIAN_POINT('Ctrl Pts',(10.6469827969598,15.2,-1.15970543218541));
#188921=CARTESIAN_POINT('Ctrl Pts',(10.6517913613925,15.2,-1.1589433795684));
#188922=CARTESIAN_POINT('Ctrl Pts',(10.6566348390398,15.2,-1.15816281739218));
#188923=CARTESIAN_POINT('Ctrl Pts',(10.6606710705592,15.2,-1.15751234888836));
#188924=CARTESIAN_POINT('Ctrl Pts',(10.6647315450508,15.2,-1.15684902721018));
#188925=CARTESIAN_POINT('Ctrl Pts',(10.6688159817162,15.2,-1.15617270033587));
#188926=CARTESIAN_POINT('Ctrl Pts',(10.6729004183816,15.2,-1.15549637346155));
#188927=CARTESIAN_POINT('Ctrl Pts',(10.6770088199366,15.2,-1.15480704032856));
#188928=CARTESIAN_POINT('Ctrl Pts',(10.6811409039631,15.2,-1.15410455178758));
#188929=CARTESIAN_POINT('Ctrl Pts',(10.6844465713645,15.2,-1.15354256092416));
#188930=CARTESIAN_POINT('Ctrl Pts',(10.6877673976315,15.2,-1.15297214976888));
#188931=CARTESIAN_POINT('Ctrl Pts',(10.691103241259,15.2,-1.15239324420766));
#188932=CARTESIAN_POINT('Ctrl Pts',(10.6952730455662,15.2,-1.15166961229559));
#188933=CARTESIAN_POINT('Ctrl Pts',(10.6994663144995,15.2,-1.15093270629744));
#188934=CARTESIAN_POINT('Ctrl Pts',(10.7036827745014,15.2,-1.1501823812269));
#188935=CARTESIAN_POINT('Ctrl Pts',(10.7070559422272,15.2,-1.14958212121954));
#188936=CARTESIAN_POINT('Ctrl Pts',(10.7104439541788,15.2,-1.14897327350774));
#188937=CARTESIAN_POINT('Ctrl Pts',(10.7138466704552,15.2,-1.14835576605878));
#188938=CARTESIAN_POINT('Ctrl Pts',(10.7172493871952,15.2,-1.14773825852569));
#188939=CARTESIAN_POINT('Ctrl Pts',(10.7206668097243,15.2,-1.14711209012495));
#188940=CARTESIAN_POINT('Ctrl Pts',(10.724098799473,15.2,-1.14647718939121));
#188941=CARTESIAN_POINT('Ctrl Pts',(10.727530788754,15.2,-1.14584228874397));
#188942=CARTESIAN_POINT('Ctrl Pts',(10.7309773475621,15.2,-1.14519865686606));
#188943=CARTESIAN_POINT('Ctrl Pts',(10.7344383385004,15.2,-1.14454622158664));
#188944=CARTESIAN_POINT('Ctrl Pts',(10.7396298256153,15.2,-1.14356756853417));
#188945=CARTESIAN_POINT('Ctrl Pts',(10.7448537859175,15.2,-1.14256910956257));
#188946=CARTESIAN_POINT('Ctrl Pts',(10.7501097680395,15.2,-1.14155061233903));
#188947=CARTESIAN_POINT('Ctrl Pts',(10.7536137556434,15.2,-1.14087161428251));
#188948=CARTESIAN_POINT('Ctrl Pts',(10.7571319753008,15.2,-1.14018370986613));
#188949=CARTESIAN_POINT('Ctrl Pts',(10.7606642943058,15.2,-1.13948683130886));
#188950=CARTESIAN_POINT('Ctrl Pts',(10.7641966137921,15.2,-1.13878995265663));
#188951=CARTESIAN_POINT('Ctrl Pts',(10.767743032056,15.2,-1.13808410036471));
#188952=CARTESIAN_POINT('Ctrl Pts',(10.771303418307,15.2,-1.13736920815816));
#188953=CARTESIAN_POINT('Ctrl Pts',(10.7757539008782,15.2,-1.13647559294867));
#188954=CARTESIAN_POINT('Ctrl Pts',(10.7802262088693,15.2,-1.13556785070839));
#188955=CARTESIAN_POINT('Ctrl Pts',(10.7847200878294,15.2,-1.13464585563778));
#188956=CARTESIAN_POINT('Ctrl Pts',(10.7883151907035,15.2,-1.13390825964159));
#188957=CARTESIAN_POINT('Ctrl Pts',(10.7919240985688,15.2,-1.13316154130606));
#188958=CARTESIAN_POINT('Ctrl Pts',(10.7955466824558,15.2,-1.1324056373089));
#188959=CARTESIAN_POINT('Ctrl Pts',(10.7991692668363,15.2,-1.13164973320875));
#188960=CARTESIAN_POINT('Ctrl Pts',(10.8028055286936,15.2,-1.13088464063048));
#188961=CARTESIAN_POINT('Ctrl Pts',(10.8064553388383,15.2,-1.13011029986511));
#188962=CARTESIAN_POINT('Ctrl Pts',(10.8101051484858,15.2,-1.12933595920524));
#188963=CARTESIAN_POINT('Ctrl Pts',(10.8137685064204,15.2,-1.12855236811046));
#188964=CARTESIAN_POINT('Ctrl Pts',(10.8174452861744,15.2,-1.12775946606478));
#188965=CARTESIAN_POINT('Ctrl Pts',(10.8229604560561,15.2,-1.12657011294224));
#188966=CARTESIAN_POINT('Ctrl Pts',(10.8285058251134,15.2,-1.12535980549642));
#188967=CARTESIAN_POINT('Ctrl Pts',(10.8340809709089,15.2,-1.12412834062594));
#188968=CARTESIAN_POINT('Ctrl Pts',(10.8396561172107,15.2,-1.1228968756436));
#188969=CARTESIAN_POINT('Ctrl Pts',(10.8452610382988,15.2,-1.12164425230923));
#188970=CARTESIAN_POINT('Ctrl Pts',(10.8508953167738,15.2,-1.12037027015553));
#188971=CARTESIAN_POINT('Ctrl Pts',(10.8555905485804,15.2,-1.11930861841864));
#188972=CARTESIAN_POINT('Ctrl Pts',(10.8603061689784,15.2,-1.11823213332331));
#188973=CARTESIAN_POINT('Ctrl Pts',(10.8650419360914,15.2,-1.11714070090664));
#188974=CARTESIAN_POINT('Ctrl Pts',(10.8688305494721,15.2,-1.11626755504467));
#188975=CARTESIAN_POINT('Ctrl Pts',(10.8726320572842,15.2,-1.11538484343267));
#188976=CARTESIAN_POINT('Ctrl Pts',(10.8764463389715,15.2,-1.11449250883958));
#188977=CARTESIAN_POINT('Ctrl Pts',(10.8812141914705,15.2,-1.11337709050703));
#188978=CARTESIAN_POINT('Ctrl Pts',(10.8860020013255,15.2,-1.11224663584076));
#188979=CARTESIAN_POINT('Ctrl Pts',(10.8908095347273,15.2,-1.11110103354988));
#188980=CARTESIAN_POINT('Ctrl Pts',(10.895617068129,15.2,-1.10995543125901));
#188981=CARTESIAN_POINT('Ctrl Pts',(10.9004443251919,15.2,-1.10879468328933));
#188982=CARTESIAN_POINT('Ctrl Pts',(10.9052910712556,15.2,-1.10761868099236));
#188983=CARTESIAN_POINT('Ctrl Pts',(10.9091684683178,15.2,-1.10667787910351));
#188984=CARTESIAN_POINT('Ctrl Pts',(10.9130583385795,15.2,-1.1057273149797));
#188985=CARTESIAN_POINT('Ctrl Pts',(10.9169605649046,15.2,-1.10476693359302));
#188986=CARTESIAN_POINT('Ctrl Pts',(10.920862790698,15.2,-1.1038065523372));
#188987=CARTESIAN_POINT('Ctrl Pts',(10.9247773719869,15.2,-1.10283635395487));
#188988=CARTESIAN_POINT('Ctrl Pts',(10.9287041917207,15.2,-1.10185628481341));
#188989=CARTESIAN_POINT('Ctrl Pts',(10.9355761269235,15.2,-1.10014116364895));
#188990=CARTESIAN_POINT('Ctrl Pts',(10.9424855408517,15.2,-1.09839581517403));
#188991=CARTESIAN_POINT('Ctrl Pts',(10.9494318094776,15.2,-1.09661995645769));
#188992=CARTESIAN_POINT('Ctrl Pts',(10.9563780781035,15.2,-1.09484409774136));
#188993=CARTESIAN_POINT('Ctrl Pts',(10.9633612061443,15.2,-1.09303773123659));
#188994=CARTESIAN_POINT('Ctrl Pts',(10.9703805743807,15.2,-1.09120058480341));
#188995=CARTESIAN_POINT('Ctrl Pts',(10.974391641554,15.2,-1.09015078694376));
#188996=CARTESIAN_POINT('Ctrl Pts',(10.9784145437091,15.2,-1.08909093690485));
#188997=CARTESIAN_POINT('Ctrl Pts',(10.9824491662118,15.2,-1.08802098710409));
#188998=CARTESIAN_POINT('Ctrl Pts',(10.9874924447526,15.2,-1.08668354974381));
#188999=CARTESIAN_POINT('Ctrl Pts',(10.9925540375852,15.2,-1.08533032970142));
#189000=CARTESIAN_POINT('Ctrl Pts',(10.9976337229555,15.2,-1.08396123170913));
#189001=CARTESIAN_POINT('Ctrl Pts',(11.0016974714731,15.2,-1.08286595325561));
#189002=CARTESIAN_POINT('Ctrl Pts',(11.0057728011331,15.2,-1.0817605139156));
#189003=CARTESIAN_POINT('Ctrl Pts',(11.0098595994681,15.2,-1.08064486457597));
#189004=CARTESIAN_POINT('Ctrl Pts',(11.0139463972463,15.2,-1.07952921538835));
#189005=CARTESIAN_POINT('Ctrl Pts',(11.0180446612757,15.2,-1.07840335499095));
#189006=CARTESIAN_POINT('Ctrl Pts',(11.0221542844391,15.2,-1.0772672385845));
#189007=CARTESIAN_POINT('Ctrl Pts',(11.0262639081623,15.2,-1.07613112202326));
#189008=CARTESIAN_POINT('Ctrl Pts',(11.0303848903975,15.2,-1.07498474884832));
#189009=CARTESIAN_POINT('Ctrl Pts',(11.0345171191079,15.2,-1.07382807161549));
#189010=CARTESIAN_POINT('Ctrl Pts',(11.0386493472553,15.2,-1.07267139454025));
#189011=CARTESIAN_POINT('Ctrl Pts',(11.0427928233035,15.2,-1.0715044134215));
#189012=CARTESIAN_POINT('Ctrl Pts',(11.0469474376854,15.2,-1.07032708362953));
#189013=CARTESIAN_POINT('Ctrl Pts',(11.0511020526333,15.2,-1.06914975367716));
#189014=CARTESIAN_POINT('Ctrl Pts',(11.0552678032353,15.2,-1.06796207330966));
#189015=CARTESIAN_POINT('Ctrl Pts',(11.0594445855748,15.2,-1.06676399941035));
#189016=CARTESIAN_POINT('Ctrl Pts',(11.0646655632146,15.2,-1.06526640711783));
#189017=CARTESIAN_POINT('Ctrl Pts',(11.0699037742296,15.2,-1.06375257351661));
#189018=CARTESIAN_POINT('Ctrl Pts',(11.0751590088683,15.2,-1.06222241052237));
#189019=CARTESIAN_POINT('Ctrl Pts',(11.0804142435071,15.2,-1.06069224752812));
#189020=CARTESIAN_POINT('Ctrl Pts',(11.085686500207,15.2,-1.05914575810252));
#189021=CARTESIAN_POINT('Ctrl Pts',(11.0909755714584,15.2,-1.05758285504562));
#189022=CARTESIAN_POINT('Ctrl Pts',(11.0962646427098,15.2,-1.05601995198873));
#189023=CARTESIAN_POINT('Ctrl Pts',(11.1015705294947,15.2,-1.05444063603155));
#189024=CARTESIAN_POINT('Ctrl Pts',(11.1068930224128,15.2,-1.05284482380798));
#189025=CARTESIAN_POINT('Ctrl Pts',(11.1100865180475,15.2,-1.05188733650863));
#189026=CARTESIAN_POINT('Ctrl Pts',(11.1132859934091,15.2,-1.05092390992634));
#189027=CARTESIAN_POINT('Ctrl Pts',(11.1164914026201,15.2,-1.04995452807911));
#189028=CARTESIAN_POINT('Ctrl Pts',(11.1196968118311,15.2,-1.04898514623188));
#189029=CARTESIAN_POINT('Ctrl Pts',(11.1229081549004,15.2,-1.04800980859119));
#189030=CARTESIAN_POINT('Ctrl Pts',(11.1261253888673,15.2,-1.04702849637633));
#189031=CARTESIAN_POINT('Ctrl Pts',(11.1304150339618,15.2,-1.04572008014927));
#189032=CARTESIAN_POINT('Ctrl Pts',(11.1347151492458,15.2,-1.04440104445489));
#189033=CARTESIAN_POINT('Ctrl Pts',(11.1390256325035,15.2,-1.04307134750912));
#189034=CARTESIAN_POINT('Ctrl Pts',(11.1422584956809,15.2,-1.04207407457334));
#189035=CARTESIAN_POINT('Ctrl Pts',(11.1454971902682,15.2,-1.04107080546086));
#189036=CARTESIAN_POINT('Ctrl Pts',(11.1487416724489,15.2,-1.04006152252169));
#189037=CARTESIAN_POINT('Ctrl Pts',(11.1530676477074,15.2,-1.03871581224173));
#189038=CARTESIAN_POINT('Ctrl Pts',(11.1574039136131,15.2,-1.03735941033984));
#189039=CARTESIAN_POINT('Ctrl Pts',(11.1617503655553,15.2,-1.03599227800099));
#189040=CARTESIAN_POINT('Ctrl Pts',(11.1660968180896,15.2,-1.03462514547586));
#189041=CARTESIAN_POINT('Ctrl Pts',(11.1704534570693,15.2,-1.03324728216368));
#189042=CARTESIAN_POINT('Ctrl Pts',(11.1748201801972,15.2,-1.03185864903134));
#189043=CARTESIAN_POINT('Ctrl Pts',(11.1780952222457,15.2,-1.03081717427669));
#189044=CARTESIAN_POINT('Ctrl Pts',(11.1813759363438,15.2,-1.02976964161403));
#189045=CARTESIAN_POINT('Ctrl Pts',(11.1846622803915,15.2,-1.02871603440178));
#189046=CARTESIAN_POINT('Ctrl Pts',(11.1890440722562,15.2,-1.02731122484925));
#189047=CARTESIAN_POINT('Ctrl Pts',(11.1934358715798,15.2,-1.02589561696069));
#189048=CARTESIAN_POINT('Ctrl Pts',(11.1978375783279,15.2,-1.02446917200698));
#189049=CARTESIAN_POINT('Ctrl Pts',(11.2011388585389,15.2,-1.02339933824311));
#189050=CARTESIAN_POINT('Ctrl Pts',(11.2044457104489,15.2,-1.02232340984579));
#189051=CARTESIAN_POINT('Ctrl Pts',(11.2077580930361,15.2,-1.02124136871927));
#189052=CARTESIAN_POINT('Ctrl Pts',(11.2121746035536,15.2,-1.0197986470862));
#189053=CARTESIAN_POINT('Ctrl Pts',(11.2166009468442,15.2,-1.01834506107432));
#189054=CARTESIAN_POINT('Ctrl Pts',(11.2210370194749,15.2,-1.01688057321673));
#189055=CARTESIAN_POINT('Ctrl Pts',(11.2243640736457,15.2,-1.0157822074233));
#189056=CARTESIAN_POINT('Ctrl Pts',(11.2276966025412,15.2,-1.01467770914679));
#189057=CARTESIAN_POINT('Ctrl Pts',(11.2310345626695,15.2,-1.01356706339602));
#189058=CARTESIAN_POINT('Ctrl Pts',(11.2354851765781,15.2,-1.01208620226047));
#189059=CARTESIAN_POINT('Ctrl Pts',(11.2399454473447,15.2,-1.01059441166486));
#189060=CARTESIAN_POINT('Ctrl Pts',(11.2444152754236,15.2,-1.00909165700694));
#189061=CARTESIAN_POINT('Ctrl Pts',(11.2500025602176,15.2,-1.00721321378691));
#189062=CARTESIAN_POINT('Ctrl Pts',(11.2556047793556,15.2,-1.00531763611238));
#189063=CARTESIAN_POINT('Ctrl Pts',(11.2612217390096,15.2,-1.00340485729153));
#189064=CARTESIAN_POINT('Ctrl Pts',(11.2657153063654,15.2,-1.00187463435994));
#189065=CARTESIAN_POINT('Ctrl Pts',(11.2702183086006,15.2,-1.00033340146312));
#189066=CARTESIAN_POINT('Ctrl Pts',(11.2747306478978,15.2,-0.998781125868518));
#189067=CARTESIAN_POINT('Ctrl Pts',(11.2803710724804,15.2,-0.99684078121664));
#189068=CARTESIAN_POINT('Ctrl Pts',(11.2860260859911,15.2,-0.994883180883756));
#189069=CARTESIAN_POINT('Ctrl Pts',(11.2916954988375,15.2,-0.992908257204114));
#189070=CARTESIAN_POINT('Ctrl Pts',(11.2950971464218,15.2,-0.991723303039382));
#189071=CARTESIAN_POINT('Ctrl Pts',(11.2985039771939,15.2,-0.990532113480597));
#189072=CARTESIAN_POINT('Ctrl Pts',(11.3019159523648,15.2,-0.989334673256673));
#189073=CARTESIAN_POINT('Ctrl Pts',(11.3064652530059,15.2,-0.987738086146419));
#189074=CARTESIAN_POINT('Ctrl Pts',(11.3110236965266,15.2,-0.986130387201012));
#189075=CARTESIAN_POINT('Ctrl Pts',(11.3155911871651,15.2,-0.984511545334278));
#189076=CARTESIAN_POINT('Ctrl Pts',(11.3190168048327,15.2,-0.983297414044511));
#189077=CARTESIAN_POINT('Ctrl Pts',(11.3224475114081,15.2,-0.982077013005494));
#189078=CARTESIAN_POINT('Ctrl Pts',(11.3258832674916,15.2,-0.980850330216728));
#189079=CARTESIAN_POINT('Ctrl Pts',(11.330464276019,15.2,-0.979214753016476));
#189080=CARTESIAN_POINT('Ctrl Pts',(11.3350542593975,15.2,-0.977568006920488));
#189081=CARTESIAN_POINT('Ctrl Pts',(11.3396531252602,15.2,-0.975910060495646));
#189082=CARTESIAN_POINT('Ctrl Pts',(11.3431022743439,15.2,-0.974666600789963));
#189083=CARTESIAN_POINT('Ctrl Pts',(11.3465564186382,15.2,-0.973416840274823));
#189084=CARTESIAN_POINT('Ctrl Pts',(11.3500155184359,15.2,-0.972160766506979));
#189085=CARTESIAN_POINT('Ctrl Pts',(11.35462765129,15.2,-0.970486001559251));
#189086=CARTESIAN_POINT('Ctrl Pts',(11.3592485935672,15.2,-0.968800011813104));
#189087=CARTESIAN_POINT('Ctrl Pts',(11.3638782521882,15.2,-0.967102766897035));
#189088=CARTESIAN_POINT('Ctrl Pts',(11.3673504963116,15.2,-0.96582983315217));
#189089=CARTESIAN_POINT('Ctrl Pts',(11.370827642868,15.2,-0.964550568282739));
#189090=CARTESIAN_POINT('Ctrl Pts',(11.3743096535325,15.2,-0.963264959580315));
#189091=CARTESIAN_POINT('Ctrl Pts',(11.3789523348402,15.2,-0.961550814488047));
#189092=CARTESIAN_POINT('Ctrl Pts',(11.383603663864,15.2,-0.95982539096812));
#189093=CARTESIAN_POINT('Ctrl Pts',(11.3882635445281,15.2,-0.958088658532206));
#189094=CARTESIAN_POINT('Ctrl Pts',(11.3917584547087,15.2,-0.956786109323585));
#189095=CARTESIAN_POINT('Ctrl Pts',(11.3952581755082,15.2,-0.955477198759407));
#189096=CARTESIAN_POINT('Ctrl Pts',(11.3987626662301,15.2,-0.954161914509585));
#189097=CARTESIAN_POINT('Ctrl Pts',(11.402267156952,15.2,-0.952846630259763));
#189098=CARTESIAN_POINT('Ctrl Pts',(11.4057764181117,15.2,-0.9515249706459));
#189099=CARTESIAN_POINT('Ctrl Pts',(11.4092904138586,15.2,-0.950196926903042));
#189100=CARTESIAN_POINT('Ctrl Pts',(11.4128044096055,15.2,-0.948868883160183));
#189101=CARTESIAN_POINT('Ctrl Pts',(11.4163231410938,15.2,-0.947534454292763));
#189102=CARTESIAN_POINT('Ctrl Pts',(11.4198465702151,15.2,-0.946193627592354));
#189103=CARTESIAN_POINT('Ctrl Pts',(11.4233699999766,15.2,-0.944852800648362));
#189104=CARTESIAN_POINT('Ctrl Pts',(11.4268981283727,15.2,-0.9435055762359));
#189105=CARTESIAN_POINT('Ctrl Pts',(11.4304309065534,15.2,-0.942151940746629));
#189106=CARTESIAN_POINT('Ctrl Pts',(11.4339636840923,15.2,-0.940798305503269));
#189107=CARTESIAN_POINT('Ctrl Pts',(11.4375011113365,15.2,-0.939438257904982));
#189108=CARTESIAN_POINT('Ctrl Pts',(11.4410431477186,15.2,-0.938071784760617));
#189109=CARTESIAN_POINT('Ctrl Pts',(11.4445851841007,15.2,-0.936705311616251));
#189110=CARTESIAN_POINT('Ctrl Pts',(11.4481318265055,15.2,-0.935332413272528));
#189111=CARTESIAN_POINT('Ctrl Pts',(11.4516830606605,15.2,-0.933953084335651));
#189112=CARTESIAN_POINT('Ctrl Pts',(11.4552342948154,15.2,-0.932573755398775));
#189113=CARTESIAN_POINT('Ctrl Pts',(11.4587901173531,15.2,-0.931187994252923));
#189114=CARTESIAN_POINT('Ctrl Pts',(11.4623505329999,15.2,-0.929795809000016));
#189115=CARTESIAN_POINT('Ctrl Pts',(10.3068855239999,12.2,-1.18690176600001));
#189116=CARTESIAN_POINT('Ctrl Pts',(10.3086714467389,12.2,-1.1869528784395));
#189117=CARTESIAN_POINT('Ctrl Pts',(10.3105146691063,12.2,-1.18700024430173));
#189118=CARTESIAN_POINT('Ctrl Pts',(10.3124142310585,12.2,-1.18704320794532));
#189119=CARTESIAN_POINT('Ctrl Pts',(10.3143229536586,12.2,-1.18708637878131));
#189120=CARTESIAN_POINT('Ctrl Pts',(10.3162885628145,12.2,-1.18712509875838));
#189121=CARTESIAN_POINT('Ctrl Pts',(10.3183101246955,12.2,-1.18715870867826));
#189122=CARTESIAN_POINT('Ctrl Pts',(10.320331686393,12.2,-1.18719231859509));
#189123=CARTESIAN_POINT('Ctrl Pts',(10.3224091993606,12.2,-1.18722081628418));
#189124=CARTESIAN_POINT('Ctrl Pts',(10.3245417522832,12.2,-1.18724356628336));
#189125=CARTESIAN_POINT('Ctrl Pts',(10.3266743052057,12.2,-1.18726631628253));
#189126=CARTESIAN_POINT('Ctrl Pts',(10.3288619009474,12.2,-1.1872833164318));
#189127=CARTESIAN_POINT('Ctrl Pts',(10.3311036480581,12.2,-1.18729394876565));
#189128=CARTESIAN_POINT('Ctrl Pts',(10.3333453953725,12.2,-1.18730458110046));
#189129=CARTESIAN_POINT('Ctrl Pts',(10.3356412985326,12.2,-1.18730884765036));
#189130=CARTESIAN_POINT('Ctrl Pts',(10.3379904907476,12.2,-1.18730614698306));
#189131=CARTESIAN_POINT('Ctrl Pts',(10.3403396827492,12.2,-1.18730344631602));
#189132=CARTESIAN_POINT('Ctrl Pts',(10.3427421643956,12.2,-1.18729378046616));
#189133=CARTESIAN_POINT('Ctrl Pts',(10.3451970944843,12.2,-1.18727656796669));
#189134=CARTESIAN_POINT('Ctrl Pts',(10.347652024573,12.2,-1.18725935546722));
#189135=CARTESIAN_POINT('Ctrl Pts',(10.3501594035892,12.2,-1.18723459877524));
#189136=CARTESIAN_POINT('Ctrl Pts',(10.3527184086606,12.2,-1.18720173402679));
#189137=CARTESIAN_POINT('Ctrl Pts',(10.3557039147322,12.2,-1.18716339181826));
#189138=CARTESIAN_POINT('Ctrl Pts',(10.3587596906992,12.2,-1.18711401306237));
#189139=CARTESIAN_POINT('Ctrl Pts',(10.3618844654844,12.2,-1.18705273574167));
#189140=CARTESIAN_POINT('Ctrl Pts',(10.3645628437327,12.2,-1.18700021232666));
#189141=CARTESIAN_POINT('Ctrl Pts',(10.3672919152934,12.2,-1.18693894571754));
#189142=CARTESIAN_POINT('Ctrl Pts',(10.3700709026069,12.2,-1.1868684142205));
#189143=CARTESIAN_POINT('Ctrl Pts',(10.3747025482978,12.2,-1.18675086172117));
#189144=CARTESIAN_POINT('Ctrl Pts',(10.3794728364098,12.2,-1.18660755852582));
#189145=CARTESIAN_POINT('Ctrl Pts',(10.3843782722652,12.2,-1.18643616977508));
#189146=CARTESIAN_POINT('Ctrl Pts',(10.3878120774175,12.2,-1.18631619764769));
#189147=CARTESIAN_POINT('Ctrl Pts',(10.3913121072864,12.2,-1.18618246645147));
#189148=CARTESIAN_POINT('Ctrl Pts',(10.3948771986916,12.2,-1.18603420401806));
#189149=CARTESIAN_POINT('Ctrl Pts',(10.3984422898192,12.2,-1.1858859415962));
#189150=CARTESIAN_POINT('Ctrl Pts',(10.4020724431775,12.2,-1.18572315146579));
#189151=CARTESIAN_POINT('Ctrl Pts',(10.4057665268881,12.2,-1.18554508674167));
#189152=CARTESIAN_POINT('Ctrl Pts',(10.4094606108863,12.2,-1.18536702200368));
#189153=CARTESIAN_POINT('Ctrl Pts',(10.4132186242088,12.2,-1.18517368689576));
#189154=CARTESIAN_POINT('Ctrl Pts',(10.4170394620716,12.2,-1.18496435772643));
#189155=CARTESIAN_POINT('Ctrl Pts',(10.4203144660814,12.2,-1.18478493271717));
#189156=CARTESIAN_POINT('Ctrl Pts',(10.4236356273469,12.2,-1.18459376083978));
#189157=CARTESIAN_POINT('Ctrl Pts',(10.4270022663668,12.2,-1.18439039899453));
#189158=CARTESIAN_POINT('Ctrl Pts',(10.4303689050809,12.2,-1.18418703716776));
#189159=CARTESIAN_POINT('Ctrl Pts',(10.4337810208038,12.2,-1.18397148993814));
#189160=CARTESIAN_POINT('Ctrl Pts',(10.4372379484301,12.2,-1.18374332602921));
#189161=CARTESIAN_POINT('Ctrl Pts',(10.4406948760565,12.2,-1.18351516212029));
#189162=CARTESIAN_POINT('Ctrl Pts',(10.4441966131543,12.2,-1.18327438392903));
#189163=CARTESIAN_POINT('Ctrl Pts',(10.4477425090235,12.2,-1.18302057602215));
#189164=CARTESIAN_POINT('Ctrl Pts',(10.4512884048927,12.2,-1.18276676811527));
#189165=CARTESIAN_POINT('Ctrl Pts',(10.4548784581555,12.2,-1.18249993024449));
#189166=CARTESIAN_POINT('Ctrl Pts',(10.4585120298538,12.2,-1.18221965850558));
#189167=CARTESIAN_POINT('Ctrl Pts',(10.4621456018822,12.2,-1.18193938674122));
#189168=CARTESIAN_POINT('Ctrl Pts',(10.4658226908315,12.2,-1.18164568290891));
#189169=CARTESIAN_POINT('Ctrl Pts',(10.4695426682028,12.2,-1.18133815030822));
#189170=CARTESIAN_POINT('Ctrl Pts',(10.4738826412958,12.2,-1.18097936231598));
#189171=CARTESIAN_POINT('Ctrl Pts',(10.4782809922367,12.2,-1.1806017551446));
#189172=CARTESIAN_POINT('Ctrl Pts',(10.4827367418169,12.2,-1.18020472129546));
#189173=CARTESIAN_POINT('Ctrl Pts',(10.4865559561889,12.2,-1.17986440652789));
#189174=CARTESIAN_POINT('Ctrl Pts',(10.4904173410482,12.2,-1.17950981866728));
#189175=CARTESIAN_POINT('Ctrl Pts',(10.4943202954294,12.2,-1.17914058897986));
#189176=CARTESIAN_POINT('Ctrl Pts',(10.4982232494561,12.2,-1.17877135932597));
#189177=CARTESIAN_POINT('Ctrl Pts',(10.5021677700582,12.2,-1.17838748677917));
#189178=CARTESIAN_POINT('Ctrl Pts',(10.5061532662647,12.2,-1.17798861020855));
#189179=CARTESIAN_POINT('Ctrl Pts',(10.5101387624713,12.2,-1.17758973363794));
#189180=CARTESIAN_POINT('Ctrl Pts',(10.5141652357321,12.2,-1.17717585342185));
#189181=CARTESIAN_POINT('Ctrl Pts',(10.5182321009983,12.2,-1.17674661685516));
#189182=CARTESIAN_POINT('Ctrl Pts',(10.5216211555099,12.2,-1.17638891970325));
#189183=CARTESIAN_POINT('Ctrl Pts',(10.5250382617855,12.2,-1.17602056038444));
#189184=CARTESIAN_POINT('Ctrl Pts',(10.5284830880667,12.2,-1.17564133751903));
#189185=CARTESIAN_POINT('Ctrl Pts',(10.531927914348,12.2,-1.17526211465361));
#189186=CARTESIAN_POINT('Ctrl Pts',(10.5354004603837,12.2,-1.17487203125341));
#189187=CARTESIAN_POINT('Ctrl Pts',(10.5389003990628,12.2,-1.17447088930954));
#189188=CARTESIAN_POINT('Ctrl Pts',(10.5424003377419,12.2,-1.17406974736568));
#189189=CARTESIAN_POINT('Ctrl Pts',(10.5459276698968,12.2,-1.17365755007708));
#189190=CARTESIAN_POINT('Ctrl Pts',(10.5494820735759,12.2,-1.17323410549433));
#189191=CARTESIAN_POINT('Ctrl Pts',(10.5530364772551,12.2,-1.17281066091159));
#189192=CARTESIAN_POINT('Ctrl Pts',(10.5566179502372,12.2,-1.1723759701245));
#189193=CARTESIAN_POINT('Ctrl Pts',(10.5602261780312,12.2,-1.17192984477528));
#189194=CARTESIAN_POINT('Ctrl Pts',(10.5645560512268,12.2,-1.17139449437567));
#189195=CARTESIAN_POINT('Ctrl Pts',(10.5689244484073,12.2,-1.17084268066522));
#189196=CARTESIAN_POINT('Ctrl Pts',(10.5733308288279,12.2,-1.17027408827035));
#189197=CARTESIAN_POINT('Ctrl Pts',(10.5770028126452,12.2,-1.16980026125741));
#189198=CARTESIAN_POINT('Ctrl Pts',(10.5807011750889,12.2,-1.16931478338731));
#189199=CARTESIAN_POINT('Ctrl Pts',(10.5844256065926,12.2,-1.16881747551607));
#189200=CARTESIAN_POINT('Ctrl Pts',(10.5881500380963,12.2,-1.16832016764482));
#189201=CARTESIAN_POINT('Ctrl Pts',(10.5919005384933,12.2,-1.16781102958898));
#189202=CARTESIAN_POINT('Ctrl Pts',(10.5956768039781,12.2,-1.16728988924239));
#189203=CARTESIAN_POINT('Ctrl Pts',(10.6002083228068,12.2,-1.16666452079239));
#189204=CARTESIAN_POINT('Ctrl Pts',(10.6047769440901,12.2,-1.16602186619859));
#189205=CARTESIAN_POINT('Ctrl Pts',(10.6093821487602,12.2,-1.16536163366141));
#189206=CARTESIAN_POINT('Ctrl Pts',(10.6132198186912,12.2,-1.16481143997038));
#189207=CARTESIAN_POINT('Ctrl Pts',(10.6170828927727,12.2,-1.16424903848934));
#189208=CARTESIAN_POINT('Ctrl Pts',(10.6209710769996,12.2,-1.16367426181689));
#189209=CARTESIAN_POINT('Ctrl Pts',(10.6256368988348,12.2,-1.16298452969717));
#189210=CARTESIAN_POINT('Ctrl Pts',(10.6303388777568,12.2,-1.16227698215076));
#189211=CARTESIAN_POINT('Ctrl Pts',(10.6350765097666,12.2,-1.16155133294376));
#189212=CARTESIAN_POINT('Ctrl Pts',(10.6390245362262,12.2,-1.16094662530421));
#189213=CARTESIAN_POINT('Ctrl Pts',(10.6429973231491,12.2,-1.16032934789832));
#189214=CARTESIAN_POINT('Ctrl Pts',(10.6469945805114,12.2,-1.1596993442171));
#189215=CARTESIAN_POINT('Ctrl Pts',(10.6509918378738,12.2,-1.15906934053588));
#189216=CARTESIAN_POINT('Ctrl Pts',(10.6550135686936,12.2,-1.1584266083631));
#189217=CARTESIAN_POINT('Ctrl Pts',(10.6590594854946,12.2,-1.15777099235723));
#189218=CARTESIAN_POINT('Ctrl Pts',(10.6631054022957,12.2,-1.15711537635136));
#189219=CARTESIAN_POINT('Ctrl Pts',(10.6671755061057,12.2,-1.15644687772863));
#189220=CARTESIAN_POINT('Ctrl Pts',(10.6712695182604,12.2,-1.15576534189423));
#189221=CARTESIAN_POINT('Ctrl Pts',(10.6745447277164,12.2,-1.15522011327129));
#189222=CARTESIAN_POINT('Ctrl Pts',(10.6778352370121,12.2,-1.15466654257442));
#189223=CARTESIAN_POINT('Ctrl Pts',(10.6811409039631,12.2,-1.15410455178758));
#189224=CARTESIAN_POINT('Ctrl Pts',(10.6844465713645,12.2,-1.15354256092416));
#189225=CARTESIAN_POINT('Ctrl Pts',(10.6877673976315,12.2,-1.15297214976888));
#189226=CARTESIAN_POINT('Ctrl Pts',(10.691103241259,12.2,-1.15239324420766));
#189227=CARTESIAN_POINT('Ctrl Pts',(10.6944390844321,12.2,-1.15181433872533));
#189228=CARTESIAN_POINT('Ctrl Pts',(10.6977899454288,12.2,-1.15122693717163));
#189229=CARTESIAN_POINT('Ctrl Pts',(10.7011556830415,12.2,-1.15063096699869));
#189230=CARTESIAN_POINT('Ctrl Pts',(10.7045214211129,12.2,-1.15003499674455));
#189231=CARTESIAN_POINT('Ctrl Pts',(10.7079020375721,12.2,-1.14943045601438));
#189232=CARTESIAN_POINT('Ctrl Pts',(10.7112973930359,12.2,-1.14881727392484));
#189233=CARTESIAN_POINT('Ctrl Pts',(10.7146927480371,12.2,-1.14820409191885));
#189234=CARTESIAN_POINT('Ctrl Pts',(10.7181028429409,12.2,-1.1475822676318));
#189235=CARTESIAN_POINT('Ctrl Pts',(10.721527540053,12.2,-1.14695172887483));
#189236=CARTESIAN_POINT('Ctrl Pts',(10.7249522376317,12.2,-1.14632119003194));
#189237=CARTESIAN_POINT('Ctrl Pts',(10.7283915370043,12.2,-1.14568193657732));
#189238=CARTESIAN_POINT('Ctrl Pts',(10.731845303749,12.2,-1.14503389843032));
#189239=CARTESIAN_POINT('Ctrl Pts',(10.7352990700232,12.2,-1.14438586037162));
#189240=CARTESIAN_POINT('Ctrl Pts',(10.7387673020111,12.2,-1.14372903703689));
#189241=CARTESIAN_POINT('Ctrl Pts',(10.7422498669472,12.2,-1.14306335909222));
#189242=CARTESIAN_POINT('Ctrl Pts',(10.7457324323577,12.2,-1.14239768105684));
#189243=CARTESIAN_POINT('Ctrl Pts',(10.7492293293088,12.2,-1.14172314853441));
#189244=CARTESIAN_POINT('Ctrl Pts',(10.7527404247939,12.2,-1.14103969304958));
#189245=CARTESIAN_POINT('Ctrl Pts',(10.7562515198007,12.2,-1.14035623765788));
#189246=CARTESIAN_POINT('Ctrl Pts',(10.7597768145676,12.2,-1.13966385812035));
#189247=CARTESIAN_POINT('Ctrl Pts',(10.7633161743879,12.2,-1.13896248878972));
#189248=CARTESIAN_POINT('Ctrl Pts',(10.7668555346904,12.2,-1.13826111936352));
#189249=CARTESIAN_POINT('Ctrl Pts',(10.7704089617499,12.2,-1.13755076002815));
#189250=CARTESIAN_POINT('Ctrl Pts',(10.7739763244999,12.2,-1.13683134276672));
#189251=CARTESIAN_POINT('Ctrl Pts',(10.7775436872499,12.2,-1.13611192550529));
#189252=CARTESIAN_POINT('Ctrl Pts',(10.7811249844654,12.2,-1.13538345173447));
#189253=CARTESIAN_POINT('Ctrl Pts',(10.7847200878294,12.2,-1.13464585563778));
#189254=CARTESIAN_POINT('Ctrl Pts',(10.7883151907035,12.2,-1.13390825964159));
#189255=CARTESIAN_POINT('Ctrl Pts',(10.7919240985688,12.2,-1.13316154130606));
#189256=CARTESIAN_POINT('Ctrl Pts',(10.7955466824558,12.2,-1.1324056373089));
#189257=CARTESIAN_POINT('Ctrl Pts',(10.7991692668363,12.2,-1.13164973320875));
#189258=CARTESIAN_POINT('Ctrl Pts',(10.8028055286936,12.2,-1.13088464063048));
#189259=CARTESIAN_POINT('Ctrl Pts',(10.8064553388383,12.2,-1.13011029986511));
#189260=CARTESIAN_POINT('Ctrl Pts',(10.8101051484858,12.2,-1.12933595920524));
#189261=CARTESIAN_POINT('Ctrl Pts',(10.8137685064204,12.2,-1.12855236811046));
#189262=CARTESIAN_POINT('Ctrl Pts',(10.8174452861744,12.2,-1.12775946606478));
#189263=CARTESIAN_POINT('Ctrl Pts',(10.8211220664295,12.2,-1.12696656391107));
#189264=CARTESIAN_POINT('Ctrl Pts',(10.8248122687716,12.2,-1.12616434821782));
#189265=CARTESIAN_POINT('Ctrl Pts',(10.8285157672707,12.2,-1.12535276013223));
#189266=CARTESIAN_POINT('Ctrl Pts',(10.8322192652652,12.2,-1.12454117215722));
#189267=CARTESIAN_POINT('Ctrl Pts',(10.8359360607037,12.2,-1.12372021039935));
#189268=CARTESIAN_POINT('Ctrl Pts',(10.8396660264534,12.2,-1.12288981580118));
#189269=CARTESIAN_POINT('Ctrl Pts',(10.8433959927114,12.2,-1.12205942108987));
#189270=CARTESIAN_POINT('Ctrl Pts',(10.8471391311238,12.2,-1.12121959159133));
#189271=CARTESIAN_POINT('Ctrl Pts',(10.8508953167738,12.2,-1.12037027015553));
#189272=CARTESIAN_POINT('Ctrl Pts',(10.854651501912,12.2,-1.11952094883545));
#189273=CARTESIAN_POINT('Ctrl Pts',(10.8584207350364,12.2,-1.11866213436979));
#189274=CARTESIAN_POINT('Ctrl Pts',(10.8622028941928,12.2,-1.11779376784267));
#189275=CARTESIAN_POINT('Ctrl Pts',(10.8669305935248,12.2,-1.11670830959504));
#189276=CARTESIAN_POINT('Ctrl Pts',(10.8716784864726,12.2,-1.11560792717213));
#189277=CARTESIAN_POINT('Ctrl Pts',(10.8764463389715,12.2,-1.11449250883958));
#189278=CARTESIAN_POINT('Ctrl Pts',(10.8812141914705,12.2,-1.11337709050703));
#189279=CARTESIAN_POINT('Ctrl Pts',(10.8860020013255,12.2,-1.11224663584076));
#189280=CARTESIAN_POINT('Ctrl Pts',(10.8908095347273,12.2,-1.11110103354988));
#189281=CARTESIAN_POINT('Ctrl Pts',(10.8946555616583,12.2,-1.11018455166724));
#189282=CARTESIAN_POINT('Ctrl Pts',(10.8985142108396,12.2,-1.10925837747114));
#189283=CARTESIAN_POINT('Ctrl Pts',(10.9023853645784,12.2,-1.10832245287252));
#189284=CARTESIAN_POINT('Ctrl Pts',(10.9062565177897,12.2,-1.10738652840143));
#189285=CARTESIAN_POINT('Ctrl Pts',(10.9101401724564,12.2,-1.10644085726321));
#189286=CARTESIAN_POINT('Ctrl Pts',(10.9140362129148,12.2,-1.1054853802864));
#189287=CARTESIAN_POINT('Ctrl Pts',(10.9179322539042,12.2,-1.10452990317942));
#189288=CARTESIAN_POINT('Ctrl Pts',(10.9218406801116,12.2,-1.10356462396292));
#189289=CARTESIAN_POINT('Ctrl Pts',(10.9257613737705,12.2,-1.10258948668691));
#189290=CARTESIAN_POINT('Ctrl Pts',(10.9296820668953,12.2,-1.10161434954376));
#189291=CARTESIAN_POINT('Ctrl Pts',(10.9336150272564,12.2,-1.10062935446093));
#189292=CARTESIAN_POINT('Ctrl Pts',(10.9375601378215,12.2,-1.09963445115438));
#189293=CARTESIAN_POINT('Ctrl Pts',(10.9415052489242,12.2,-1.09863954771228));
#189294=CARTESIAN_POINT('Ctrl Pts',(10.9454625129654,12.2,-1.09763473290653));
#189295=CARTESIAN_POINT('Ctrl Pts',(10.9494318094776,12.2,-1.09661995645769));
#189296=CARTESIAN_POINT('Ctrl Pts',(10.953401105449,12.2,-1.09560518014712));
#189297=CARTESIAN_POINT('Ctrl Pts',(10.9573824380636,12.2,-1.09458044427528));
#189298=CARTESIAN_POINT('Ctrl Pts',(10.961375689847,12.2,-1.09354569319423));
#189299=CARTESIAN_POINT('Ctrl Pts',(10.9653689421745,12.2,-1.0925109419722));
#189300=CARTESIAN_POINT('Ctrl Pts',(10.9693741134838,12.2,-1.09146617794366));
#189301=CARTESIAN_POINT('Ctrl Pts',(10.9733910917582,12.2,-1.09041135127506));
#189302=CARTESIAN_POINT('Ctrl Pts',(10.9774080700327,12.2,-1.08935652460646));
#189303=CARTESIAN_POINT('Ctrl Pts',(10.9814368537308,12.2,-1.08829163308946));
#189304=CARTESIAN_POINT('Ctrl Pts',(10.9854773301189,12.2,-1.08721662980762));
#189305=CARTESIAN_POINT('Ctrl Pts',(10.9895178059564,12.2,-1.08614162667225));
#189306=CARTESIAN_POINT('Ctrl Pts',(10.9935699749915,12.2,-1.08505651001342));
#189307=CARTESIAN_POINT('Ctrl Pts',(10.9976337229555,12.2,-1.08396123170913));
#189308=CARTESIAN_POINT('Ctrl Pts',(11.0016974714731,12.2,-1.08286595325561));
#189309=CARTESIAN_POINT('Ctrl Pts',(11.0057728011331,12.2,-1.0817605139156));
#189310=CARTESIAN_POINT('Ctrl Pts',(11.0098595994681,12.2,-1.08064486457597));
#189311=CARTESIAN_POINT('Ctrl Pts',(11.0139463972463,12.2,-1.07952921538835));
#189312=CARTESIAN_POINT('Ctrl Pts',(11.0180446612757,12.2,-1.07840335499096));
#189313=CARTESIAN_POINT('Ctrl Pts',(11.0221542844391,12.2,-1.0772672385845));
#189314=CARTESIAN_POINT('Ctrl Pts',(11.0262639081623,12.2,-1.07613112202326));
#189315=CARTESIAN_POINT('Ctrl Pts',(11.0303848903975,12.2,-1.07498474884832));
#189316=CARTESIAN_POINT('Ctrl Pts',(11.0345171191079,12.2,-1.07382807161549));
#189317=CARTESIAN_POINT('Ctrl Pts',(11.0386493472553,12.2,-1.07267139454025));
#189318=CARTESIAN_POINT('Ctrl Pts',(11.0427928233035,12.2,-1.0715044134215));
#189319=CARTESIAN_POINT('Ctrl Pts',(11.0469474376854,12.2,-1.07032708362954));
#189320=CARTESIAN_POINT('Ctrl Pts',(11.0521407060873,12.2,-1.06885542126927));
#189321=CARTESIAN_POINT('Ctrl Pts',(11.0573513752257,12.2,-1.06736758688081));
#189322=CARTESIAN_POINT('Ctrl Pts',(11.0625792379331,12.2,-1.06586349458999));
#189323=CARTESIAN_POINT('Ctrl Pts',(11.066761528327,12.2,-1.06466022069176));
#189324=CARTESIAN_POINT('Ctrl Pts',(11.0709548209282,12.2,-1.06344654098448));
#189325=CARTESIAN_POINT('Ctrl Pts',(11.0751590088683,12.2,-1.06222241052237));
#189326=CARTESIAN_POINT('Ctrl Pts',(11.0793631962356,12.2,-1.06099828022705));
#189327=CARTESIAN_POINT('Ctrl Pts',(11.0835782770924,12.2,-1.05976370136038));
#189328=CARTESIAN_POINT('Ctrl Pts',(11.0878041469129,12.2,-1.05851862835174));
#189329=CARTESIAN_POINT('Ctrl Pts',(11.0930864846203,12.2,-1.05696228696371));
#189330=CARTESIAN_POINT('Ctrl Pts',(11.0983856782588,12.2,-1.05538954888081));
#189331=CARTESIAN_POINT('Ctrl Pts',(11.1037015202023,12.2,-1.05380033235389));
#189332=CARTESIAN_POINT('Ctrl Pts',(11.1068910252526,12.2,-1.05284680247239));
#189333=CARTESIAN_POINT('Ctrl Pts',(11.110086523671,12.2,-1.05188733901591));
#189334=CARTESIAN_POINT('Ctrl Pts',(11.1132879718806,12.2,-1.05092192567011));
#189335=CARTESIAN_POINT('Ctrl Pts',(11.1164894200902,12.2,-1.04995651232432));
#189336=CARTESIAN_POINT('Ctrl Pts',(11.119696816717,12.2,-1.04898514954345));
#189337=CARTESIAN_POINT('Ctrl Pts',(11.1229101187661,12.2,-1.04800781824644));
#189338=CARTESIAN_POINT('Ctrl Pts',(11.1261234213989,12.2,-1.04703048677189));
#189339=CARTESIAN_POINT('Ctrl Pts',(11.1293426287668,12.2,-1.04604718699565));
#189340=CARTESIAN_POINT('Ctrl Pts',(11.132567696903,12.2,-1.04505790205939));
#189341=CARTESIAN_POINT('Ctrl Pts',(11.1357927644532,12.2,-1.04406861730285));
#189342=CARTESIAN_POINT('Ctrl Pts',(11.1390236931199,12.2,-1.04307334710496));
#189343=CARTESIAN_POINT('Ctrl Pts',(11.1422604386278,12.2,-1.04207207484915));
#189344=CARTESIAN_POINT('Ctrl Pts',(11.1454971841357,12.2,-1.04107080259334));
#189345=CARTESIAN_POINT('Ctrl Pts',(11.1487397456894,12.2,-1.04006352855028));
#189346=CARTESIAN_POINT('Ctrl Pts',(11.1519880812529,12.2,-1.03905023474914));
#189347=CARTESIAN_POINT('Ctrl Pts',(11.1552364168163,12.2,-1.03803694094799));
#189348=CARTESIAN_POINT('Ctrl Pts',(11.1584905264506,12.2,-1.03701762730169));
#189349=CARTESIAN_POINT('Ctrl Pts',(11.1617503655553,12.2,-1.03599227800099));
#189350=CARTESIAN_POINT('Ctrl Pts',(11.1650102046599,12.2,-1.03496692870028));
#189351=CARTESIAN_POINT('Ctrl Pts',(11.1682757737628,12.2,-1.03393554315815));
#189352=CARTESIAN_POINT('Ctrl Pts',(11.1715470293934,12.2,-1.03289810536304));
#189353=CARTESIAN_POINT('Ctrl Pts',(11.1748182850241,12.2,-1.03186066756792));
#189354=CARTESIAN_POINT('Ctrl Pts',(11.1780952271543,12.2,-1.03081717702322));
#189355=CARTESIAN_POINT('Ctrl Pts',(11.1813778132426,12.2,-1.02976761772886));
#189356=CARTESIAN_POINT('Ctrl Pts',(11.1846603999273,12.2,-1.02871805824382));
#189357=CARTESIAN_POINT('Ctrl Pts',(11.1879486305718,12.2,-1.02766242975706));
#189358=CARTESIAN_POINT('Ctrl Pts',(11.191242462218,12.2,-1.02660071631026));
#189359=CARTESIAN_POINT('Ctrl Pts',(11.1945362932657,12.2,-1.02553900305635));
#189360=CARTESIAN_POINT('Ctrl Pts',(11.197835725427,12.2,-1.02447120432423));
#189361=CARTESIAN_POINT('Ctrl Pts',(11.2011407156811,12.2,-1.02339730547556));
#189362=CARTESIAN_POINT('Ctrl Pts',(11.2044457059351,12.2,-1.02232340662689));
#189363=CARTESIAN_POINT('Ctrl Pts',(11.2077562537648,12.2,-1.0212434064093));
#189364=CARTESIAN_POINT('Ctrl Pts',(11.2110723188531,12.2,-1.0201572896149));
#189365=CARTESIAN_POINT('Ctrl Pts',(11.2143883839414,12.2,-1.0190711728205));
#189366=CARTESIAN_POINT('Ctrl Pts',(11.2177099653041,12.2,-1.01797893901015));
#189367=CARTESIAN_POINT('Ctrl Pts',(11.2210370194749,12.2,-1.01688057321673));
#189368=CARTESIAN_POINT('Ctrl Pts',(11.2243640736457,12.2,-1.0157822074233));
#189369=CARTESIAN_POINT('Ctrl Pts',(11.2276966025412,12.2,-1.01467770914679));
#189370=CARTESIAN_POINT('Ctrl Pts',(11.2310345626695,12.2,-1.01356706339602));
#189371=CARTESIAN_POINT('Ctrl Pts',(11.2343725227977,12.2,-1.01245641764524));
#189372=CARTESIAN_POINT('Ctrl Pts',(11.2377159145737,12.2,-1.01133962443184));
#189373=CARTESIAN_POINT('Ctrl Pts',(11.2410646968271,12.2,-1.01021666820893));
#189374=CARTESIAN_POINT('Ctrl Pts',(11.2444134790804,12.2,-1.00909371198601));
#189375=CARTESIAN_POINT('Ctrl Pts',(11.247767650407,12.2,-1.00796459388879));
#189376=CARTESIAN_POINT('Ctrl Pts',(11.2511271709925,12.2,-1.00682929672255));
#189377=CARTESIAN_POINT('Ctrl Pts',(11.2544866921884,12.2,-1.00569399935006));
#189378=CARTESIAN_POINT('Ctrl Pts',(11.2578515627274,12.2,-1.00455252475083));
#189379=CARTESIAN_POINT('Ctrl Pts',(11.2612217390096,12.2,-1.00340485729153));
#189380=CARTESIAN_POINT('Ctrl Pts',(11.2657153063654,12.2,-1.00187463435994));
#189381=CARTESIAN_POINT('Ctrl Pts',(11.2702183086006,12.2,-1.00033340146312));
#189382=CARTESIAN_POINT('Ctrl Pts',(11.2747306478978,12.2,-0.998781125868519));
#189383=CARTESIAN_POINT('Ctrl Pts',(11.2781149025244,12.2,-0.997616919119692));
#189384=CARTESIAN_POINT('Ctrl Pts',(11.2815044093506,12.2,-0.996446500179626));
#189385=CARTESIAN_POINT('Ctrl Pts',(11.2848991269765,12.2,-0.995269854514894));
#189386=CARTESIAN_POINT('Ctrl Pts',(11.2882938452192,12.2,-0.994093208636405));
#189387=CARTESIAN_POINT('Ctrl Pts',(11.2916937747633,12.2,-0.992910336514494));
#189388=CARTESIAN_POINT('Ctrl Pts',(11.2950988740506,12.2,-0.991721223174159));
#189389=CARTESIAN_POINT('Ctrl Pts',(11.2985039727192,12.2,-0.990532110049847));
#189390=CARTESIAN_POINT('Ctrl Pts',(11.301914242547,12.2,-0.989336757217945));
#189391=CARTESIAN_POINT('Ctrl Pts',(11.3053296414274,12.2,-0.988135148492515));
#189392=CARTESIAN_POINT('Ctrl Pts',(11.3087450403079,12.2,-0.986933539767085));
#189393=CARTESIAN_POINT('Ctrl Pts',(11.3121655694974,12.2,-0.985725676624046));
#189394=CARTESIAN_POINT('Ctrl Pts',(11.3155911871651,12.2,-0.984511545334279));
#189395=CARTESIAN_POINT('Ctrl Pts',(11.3190168048327,12.2,-0.983297414044512));
#189396=CARTESIAN_POINT('Ctrl Pts',(11.3224475114081,12.2,-0.982077013005498));
#189397=CARTESIAN_POINT('Ctrl Pts',(11.3258832674916,12.2,-0.980850330216732));
#189398=CARTESIAN_POINT('Ctrl Pts',(11.3293190235751,12.2,-0.979623647427967));
#189399=CARTESIAN_POINT('Ctrl Pts',(11.3327598275334,12.2,-0.978390681672795));
#189400=CARTESIAN_POINT('Ctrl Pts',(11.3362056416161,12.2,-0.977151420885035));
#189401=CARTESIAN_POINT('Ctrl Pts',(11.3396514556988,12.2,-0.975912160097274));
#189402=CARTESIAN_POINT('Ctrl Pts',(11.3431022787682,12.2,-0.974666603008525));
#189403=CARTESIAN_POINT('Ctrl Pts',(11.3465580705647,12.2,-0.973414736742201));
#189404=CARTESIAN_POINT('Ctrl Pts',(11.3500138623612,12.2,-0.972162870475877));
#189405=CARTESIAN_POINT('Ctrl Pts',(11.3534746225543,12.2,-0.970904695462241));
#189406=CARTESIAN_POINT('Ctrl Pts',(11.3569403117611,12.2,-0.969640197300713));
#189407=CARTESIAN_POINT('Ctrl Pts',(11.3604060015974,12.2,-0.968375698909467));
#189408=CARTESIAN_POINT('Ctrl Pts',(11.3638766215518,12.2,-0.967104878091442));
#189409=CARTESIAN_POINT('Ctrl Pts',(11.3673521299742,12.2,-0.965827721738297));
#189410=CARTESIAN_POINT('Ctrl Pts',(11.3719861401519,12.2,-0.964124846987467));
#189411=CARTESIAN_POINT('Ctrl Pts',(11.3766288443144,12.2,-0.962410710032548));
#189412=CARTESIAN_POINT('Ctrl Pts',(11.3812801488781,12.2,-0.960685279174338));
#189413=CARTESIAN_POINT('Ctrl Pts',(11.3847686274593,12.2,-0.959391205971909));
#189414=CARTESIAN_POINT('Ctrl Pts',(11.3882619432427,12.2,-0.958090780169896));
#189415=CARTESIAN_POINT('Ctrl Pts',(11.3917600560398,12.2,-0.956783988486161));
#189416=CARTESIAN_POINT('Ctrl Pts',(11.3952581688369,12.2,-0.955477196802426));
#189417=CARTESIAN_POINT('Ctrl Pts',(11.39876107808,12.2,-0.9541640406389));
#189418=CARTESIAN_POINT('Ctrl Pts',(11.4022687452436,12.2,-0.952844505062712));
#189419=CARTESIAN_POINT('Ctrl Pts',(11.4057764130444,12.2,-0.951524969246809));
#189420=CARTESIAN_POINT('Ctrl Pts',(11.4092888387048,12.2,-0.950199056087446));
#189421=CARTESIAN_POINT('Ctrl Pts',(11.4128059880083,12.2,-0.948866753726278));
#189422=CARTESIAN_POINT('Ctrl Pts',(11.4163231366728,12.2,-0.947534451607146));
#189423=CARTESIAN_POINT('Ctrl Pts',(11.4198450088788,12.2,-0.94619576065502));
#189424=CARTESIAN_POINT('Ctrl Pts',(11.4233715648761,12.2,-0.944850667078338));
#189425=CARTESIAN_POINT('Ctrl Pts',(11.4268981208733,12.2,-0.943505573501657));
#189426=CARTESIAN_POINT('Ctrl Pts',(11.4304293590655,12.2,-0.942154079389015));
#189427=CARTESIAN_POINT('Ctrl Pts',(11.4339652317448,12.2,-0.940796167723825));
#189428=CARTESIAN_POINT('Ctrl Pts',(11.4375011044241,12.2,-0.939438256058633));
#189429=CARTESIAN_POINT('Ctrl Pts',(11.4410416129428,12.2,-0.938073927057691));
#189430=CARTESIAN_POINT('Ctrl Pts',(11.4445867185384,12.2,-0.936703169976301));
#189431=CARTESIAN_POINT('Ctrl Pts',(11.450495228079,12.2,-0.934418574757642));
#189432=CARTESIAN_POINT('Ctrl Pts',(11.4564165067063,12.2,-0.932116117839165));
#189433=CARTESIAN_POINT('Ctrl Pts',(11.4623505329999,12.2,-0.929795809000016));
#189434=CARTESIAN_POINT('Ctrl Pts',(11.4869855309999,15.2,-0.546958306000014));
#189435=CARTESIAN_POINT('Ctrl Pts',(11.4869855309999,11.6,-0.546958306000014));
#189436=CARTESIAN_POINT('Ctrl Pts',(11.4863150069999,15.2,-0.546590899000012));
#189437=CARTESIAN_POINT('Ctrl Pts',(11.4863150069999,11.6,-0.546590899000013));
#189438=CARTESIAN_POINT('Ctrl Pts',(11.4849742089999,15.2,-0.545856552000017));
#189439=CARTESIAN_POINT('Ctrl Pts',(11.4849742089999,11.6,-0.545856552000017));
#189440=CARTESIAN_POINT('Ctrl Pts',(11.4829637559999,15.2,-0.544756422000017));
#189441=CARTESIAN_POINT('Ctrl Pts',(11.4829637559999,11.6,-0.544756422000017));
#189442=CARTESIAN_POINT('Ctrl Pts',(11.4802846429999,15.2,-0.543292368000015));
#189443=CARTESIAN_POINT('Ctrl Pts',(11.4802846429999,11.6,-0.543292368000015));
#189444=CARTESIAN_POINT('Ctrl Pts',(11.4769382369999,15.2,-0.541466945000018));
#189445=CARTESIAN_POINT('Ctrl Pts',(11.4769382369999,11.6,-0.541466945000018));
#189446=CARTESIAN_POINT('Ctrl Pts',(11.4735943179999,15.2,-0.539646167000014));
#189447=CARTESIAN_POINT('Ctrl Pts',(11.4735943179999,11.6,-0.539646167000015));
#189448=CARTESIAN_POINT('Ctrl Pts',(11.4702528869999,15.2,-0.537830030000013));
#189449=CARTESIAN_POINT('Ctrl Pts',(11.4702528869999,11.6,-0.537830030000013));
#189450=CARTESIAN_POINT('Ctrl Pts',(11.4669139489999,15.2,-0.536018536000018));
#189451=CARTESIAN_POINT('Ctrl Pts',(11.4669139489999,11.6,-0.536018536000018));
#189452=CARTESIAN_POINT('Ctrl Pts',(11.4635775099999,15.2,-0.534211685000017));
#189453=CARTESIAN_POINT('Ctrl Pts',(11.4635775099999,11.6,-0.534211685000017));
#189454=CARTESIAN_POINT('Ctrl Pts',(11.4602435779999,15.2,-0.532409474000013));
#189455=CARTESIAN_POINT('Ctrl Pts',(11.4602435779999,11.6,-0.532409474000013));
#189456=CARTESIAN_POINT('Ctrl Pts',(11.4569121619999,15.2,-0.530611901000011));
#189457=CARTESIAN_POINT('Ctrl Pts',(11.4569121619999,11.6,-0.530611901000011));
#189458=CARTESIAN_POINT('Ctrl Pts',(11.4535832719999,15.2,-0.528818965000015));
#189459=CARTESIAN_POINT('Ctrl Pts',(11.4535832719999,11.6,-0.528818965000016));
#189460=CARTESIAN_POINT('Ctrl Pts',(11.4502569209999,15.2,-0.527030665000012));
#189461=CARTESIAN_POINT('Ctrl Pts',(11.4502569209999,11.6,-0.527030665000013));
#189462=CARTESIAN_POINT('Ctrl Pts',(11.4469331179999,15.2,-0.525246997000015));
#189463=CARTESIAN_POINT('Ctrl Pts',(11.4469331179999,11.6,-0.525246997000016));
#189464=CARTESIAN_POINT('Ctrl Pts',(11.4436118749999,15.2,-0.523467959000015));
#189465=CARTESIAN_POINT('Ctrl Pts',(11.4436118749999,11.6,-0.523467959000015));
#189466=CARTESIAN_POINT('Ctrl Pts',(11.4402931999999,15.2,-0.521693551000015));
#189467=CARTESIAN_POINT('Ctrl Pts',(11.4402931999999,11.6,-0.521693551000016));
#189468=CARTESIAN_POINT('Ctrl Pts',(11.4369771019999,15.2,-0.519923772000013));
#189469=CARTESIAN_POINT('Ctrl Pts',(11.4369771019999,11.6,-0.519923772000013));
#189470=CARTESIAN_POINT('Ctrl Pts',(11.4336635899999,15.2,-0.518158618000015));
#189471=CARTESIAN_POINT('Ctrl Pts',(11.4336635899999,11.6,-0.518158618000016));
#189472=CARTESIAN_POINT('Ctrl Pts',(11.4303526699999,15.2,-0.516398090000014));
#189473=CARTESIAN_POINT('Ctrl Pts',(11.4303526699999,11.6,-0.516398090000015));
#189474=CARTESIAN_POINT('Ctrl Pts',(11.4270443509999,15.2,-0.514642184000014));
#189475=CARTESIAN_POINT('Ctrl Pts',(11.4270443509999,11.6,-0.514642184000014));
#189476=CARTESIAN_POINT('Ctrl Pts',(11.4237386419999,15.2,-0.512890901000014));
#189477=CARTESIAN_POINT('Ctrl Pts',(11.4237386419999,11.6,-0.512890901000014));
#189478=CARTESIAN_POINT('Ctrl Pts',(11.4204355509999,15.2,-0.511144238000014));
#189479=CARTESIAN_POINT('Ctrl Pts',(11.4204355509999,11.6,-0.511144238000015));
#189480=CARTESIAN_POINT('Ctrl Pts',(11.4171350879999,15.2,-0.509402194000015));
#189481=CARTESIAN_POINT('Ctrl Pts',(11.4171350879999,11.6,-0.509402194000015));
#189482=CARTESIAN_POINT('Ctrl Pts',(11.4138372609999,15.2,-0.507664766000016));
#189483=CARTESIAN_POINT('Ctrl Pts',(11.4138372609999,11.6,-0.507664766000016));
#189484=CARTESIAN_POINT('Ctrl Pts',(11.4105420809999,15.2,-0.505931955000012));
#189485=CARTESIAN_POINT('Ctrl Pts',(11.4105420809999,11.6,-0.505931955000012));
#189486=CARTESIAN_POINT('Ctrl Pts',(11.4072495559999,15.2,-0.504203755000017));
#189487=CARTESIAN_POINT('Ctrl Pts',(11.4072495559999,11.6,-0.504203755000017));
#189488=CARTESIAN_POINT('Ctrl Pts',(11.4039596959999,15.2,-0.502480169000012));
#189489=CARTESIAN_POINT('Ctrl Pts',(11.4039596959999,11.6,-0.502480169000013));
#189490=CARTESIAN_POINT('Ctrl Pts',(11.4006725109999,15.2,-0.500761191000016));
#189491=CARTESIAN_POINT('Ctrl Pts',(11.4006725109999,11.6,-0.500761191000017));
#189492=CARTESIAN_POINT('Ctrl Pts',(11.3973880069999,15.2,-0.499046823000011));
#189493=CARTESIAN_POINT('Ctrl Pts',(11.3973880069999,11.6,-0.499046823000012));
#189494=CARTESIAN_POINT('Ctrl Pts',(11.3941061959999,15.2,-0.497337061000014));
#189495=CARTESIAN_POINT('Ctrl Pts',(11.3941061959999,11.6,-0.497337061000014));
#189496=CARTESIAN_POINT('Ctrl Pts',(11.3908270859999,15.2,-0.495631903000016));
#189497=CARTESIAN_POINT('Ctrl Pts',(11.3908270859999,11.6,-0.495631903000016));
#189498=CARTESIAN_POINT('Ctrl Pts',(11.3875506839999,15.2,-0.493931349000012));
#189499=CARTESIAN_POINT('Ctrl Pts',(11.3875506839999,11.6,-0.493931349000012));
#189500=CARTESIAN_POINT('Ctrl Pts',(11.3842770019999,15.2,-0.492235396000016));
#189501=CARTESIAN_POINT('Ctrl Pts',(11.3842770019999,11.6,-0.492235396000016));
#189502=CARTESIAN_POINT('Ctrl Pts',(11.3810060469999,15.2,-0.490544043000014));
#189503=CARTESIAN_POINT('Ctrl Pts',(11.3810060469999,11.6,-0.490544043000015));
#189504=CARTESIAN_POINT('Ctrl Pts',(11.3777378289999,15.2,-0.488857287000015));
#189505=CARTESIAN_POINT('Ctrl Pts',(11.3777378289999,11.6,-0.488857287000016));
#189506=CARTESIAN_POINT('Ctrl Pts',(11.3744723579999,15.2,-0.487175129000015));
#189507=CARTESIAN_POINT('Ctrl Pts',(11.3744723579999,11.6,-0.487175129000015));
#189508=CARTESIAN_POINT('Ctrl Pts',(11.3712096409999,15.2,-0.485497564000017));
#189509=CARTESIAN_POINT('Ctrl Pts',(11.3712096409999,11.6,-0.485497564000017));
#189510=CARTESIAN_POINT('Ctrl Pts',(11.3679496899999,15.2,-0.483824591000013));
#189511=CARTESIAN_POINT('Ctrl Pts',(11.3679496899999,11.6,-0.483824591000013));
#189512=CARTESIAN_POINT('Ctrl Pts',(11.3646925119999,15.2,-0.482156209000015));
#189513=CARTESIAN_POINT('Ctrl Pts',(11.3646925119999,11.6,-0.482156209000016));
#189514=CARTESIAN_POINT('Ctrl Pts',(11.3614381179999,15.2,-0.480492415000011));
#189515=CARTESIAN_POINT('Ctrl Pts',(11.3614381179999,11.6,-0.480492415000012));
#189516=CARTESIAN_POINT('Ctrl Pts',(11.3581865149999,15.2,-0.478833210000014));
#189517=CARTESIAN_POINT('Ctrl Pts',(11.3581865149999,11.6,-0.478833210000014));
#189518=CARTESIAN_POINT('Ctrl Pts',(11.3549377139999,15.2,-0.477178588000013));
#189519=CARTESIAN_POINT('Ctrl Pts',(11.3549377139999,11.6,-0.477178588000014));
#189520=CARTESIAN_POINT('Ctrl Pts',(11.3516917239999,15.2,-0.475528551000015));
#189521=CARTESIAN_POINT('Ctrl Pts',(11.3516917239999,11.6,-0.475528551000016));
#189522=CARTESIAN_POINT('Ctrl Pts',(11.3484485529999,15.2,-0.473883094000014));
#189523=CARTESIAN_POINT('Ctrl Pts',(11.3484485529999,11.6,-0.473883094000014));
#189524=CARTESIAN_POINT('Ctrl Pts',(11.3452082119999,15.2,-0.472242217000014));
#189525=CARTESIAN_POINT('Ctrl Pts',(11.3452082119999,11.6,-0.472242217000014));
#189526=CARTESIAN_POINT('Ctrl Pts',(11.3419707089999,15.2,-0.470605918000011));
#189527=CARTESIAN_POINT('Ctrl Pts',(11.3419707089999,11.6,-0.470605918000012));
#189528=CARTESIAN_POINT('Ctrl Pts',(11.3387360539999,15.2,-0.468974194000014));
#189529=CARTESIAN_POINT('Ctrl Pts',(11.3387360539999,11.6,-0.468974194000014));
#189530=CARTESIAN_POINT('Ctrl Pts',(11.3355042559999,15.2,-0.467347044000017));
#189531=CARTESIAN_POINT('Ctrl Pts',(11.3355042559999,11.6,-0.467347044000018));
#189532=CARTESIAN_POINT('Ctrl Pts',(11.3322753239999,15.2,-0.465724466000013));
#189533=CARTESIAN_POINT('Ctrl Pts',(11.3322753239999,11.6,-0.465724466000013));
#189534=CARTESIAN_POINT('Ctrl Pts',(11.3290492679999,15.2,-0.464106457000018));
#189535=CARTESIAN_POINT('Ctrl Pts',(11.3290492679999,11.6,-0.464106457000018));
#189536=CARTESIAN_POINT('Ctrl Pts',(11.3258260979999,15.2,-0.462493017000014));
#189537=CARTESIAN_POINT('Ctrl Pts',(11.3258260979999,11.6,-0.462493017000015));
#189538=CARTESIAN_POINT('Ctrl Pts',(11.3226058229999,15.2,-0.460884143000015));
#189539=CARTESIAN_POINT('Ctrl Pts',(11.3226058229999,11.6,-0.460884143000016));
#189540=CARTESIAN_POINT('Ctrl Pts',(11.3193884509999,15.2,-0.459279832000017));
#189541=CARTESIAN_POINT('Ctrl Pts',(11.3193884509999,11.6,-0.459279832000017));
#189542=CARTESIAN_POINT('Ctrl Pts',(11.3161739919999,15.2,-0.457680084000014));
#189543=CARTESIAN_POINT('Ctrl Pts',(11.3161739919999,11.6,-0.457680084000014));
#189544=CARTESIAN_POINT('Ctrl Pts',(11.3129624559999,15.2,-0.456084896000015));
#189545=CARTESIAN_POINT('Ctrl Pts',(11.3129624559999,11.6,-0.456084896000016));
#189546=CARTESIAN_POINT('Ctrl Pts',(11.3097538529999,15.2,-0.454494266000012));
#189547=CARTESIAN_POINT('Ctrl Pts',(11.3097538529999,11.6,-0.454494266000012));
#189548=CARTESIAN_POINT('Ctrl Pts',(11.3065481919999,15.2,-0.452908191000017));
#189549=CARTESIAN_POINT('Ctrl Pts',(11.3065481919999,11.6,-0.452908191000017));
#189550=CARTESIAN_POINT('Ctrl Pts',(11.3033454809999,15.2,-0.451326671000012));
#189551=CARTESIAN_POINT('Ctrl Pts',(11.3033454809999,11.6,-0.451326671000012));
#189552=CARTESIAN_POINT('Ctrl Pts',(11.3001457309999,15.2,-0.449749702000015));
#189553=CARTESIAN_POINT('Ctrl Pts',(11.3001457309999,11.6,-0.449749702000016));
#189554=CARTESIAN_POINT('Ctrl Pts',(11.2969489509999,15.2,-0.448177284000018));
#189555=CARTESIAN_POINT('Ctrl Pts',(11.2969489509999,11.6,-0.448177284000018));
#189556=CARTESIAN_POINT('Ctrl Pts',(11.2937551509999,15.2,-0.446609413000014));
#189557=CARTESIAN_POINT('Ctrl Pts',(11.2937551509999,11.6,-0.446609413000015));
#189558=CARTESIAN_POINT('Ctrl Pts',(11.2905643409999,15.2,-0.445046088000014));
#189559=CARTESIAN_POINT('Ctrl Pts',(11.2905643409999,11.6,-0.445046088000014));
#189560=CARTESIAN_POINT('Ctrl Pts',(11.2873765289999,15.2,-0.443487307000012));
#189561=CARTESIAN_POINT('Ctrl Pts',(11.2873765289999,11.6,-0.443487307000013));
#189562=CARTESIAN_POINT('Ctrl Pts',(11.2841917249999,15.2,-0.441933067000013));
#189563=CARTESIAN_POINT('Ctrl Pts',(11.2841917249999,11.6,-0.441933067000014));
#189564=CARTESIAN_POINT('Ctrl Pts',(11.2810099399999,15.2,-0.440383367000017));
#189565=CARTESIAN_POINT('Ctrl Pts',(11.2810099399999,11.6,-0.440383367000017));
#189566=CARTESIAN_POINT('Ctrl Pts',(11.2778311809999,15.2,-0.438838205000014));
#189567=CARTESIAN_POINT('Ctrl Pts',(11.2778311809999,11.6,-0.438838205000014));
#189568=CARTESIAN_POINT('Ctrl Pts',(11.2746554609999,15.2,-0.437297577000013));
#189569=CARTESIAN_POINT('Ctrl Pts',(11.2746554609999,11.6,-0.437297577000014));
#189570=CARTESIAN_POINT('Ctrl Pts',(11.2714827859999,15.2,-0.435761482000014));
#189571=CARTESIAN_POINT('Ctrl Pts',(11.2714827859999,11.6,-0.435761482000015));
#189572=CARTESIAN_POINT('Ctrl Pts',(11.2683131689999,15.2,-0.434229918000018));
#189573=CARTESIAN_POINT('Ctrl Pts',(11.2683131689999,11.6,-0.434229918000018));
#189574=CARTESIAN_POINT('Ctrl Pts',(11.2651466169999,15.2,-0.432702883000013));
#189575=CARTESIAN_POINT('Ctrl Pts',(11.2651466169999,11.6,-0.432702883000014));
#189576=CARTESIAN_POINT('Ctrl Pts',(11.2619831409999,15.2,-0.431180374000015));
#189577=CARTESIAN_POINT('Ctrl Pts',(11.2619831409999,11.6,-0.431180374000016));
#189578=CARTESIAN_POINT('Ctrl Pts',(11.2588227499999,15.2,-0.429662390000014));
#189579=CARTESIAN_POINT('Ctrl Pts',(11.2588227499999,11.6,-0.429662390000014));
#189580=CARTESIAN_POINT('Ctrl Pts',(11.2556654559999,15.2,-0.428148928000014));
#189581=CARTESIAN_POINT('Ctrl Pts',(11.2556654559999,11.6,-0.428148928000014));
#189582=CARTESIAN_POINT('Ctrl Pts',(11.2525112649999,15.2,-0.426639986000015));
#189583=CARTESIAN_POINT('Ctrl Pts',(11.2525112649999,11.6,-0.426639986000015));
#189584=CARTESIAN_POINT('Ctrl Pts',(11.2493601889999,15.2,-0.425135562000012));
#189585=CARTESIAN_POINT('Ctrl Pts',(11.2493601889999,11.6,-0.425135562000012));
#189586=CARTESIAN_POINT('Ctrl Pts',(11.2462122379999,15.2,-0.423635653000014));
#189587=CARTESIAN_POINT('Ctrl Pts',(11.2462122379999,11.6,-0.423635653000014));
#189588=CARTESIAN_POINT('Ctrl Pts',(11.2430674209999,15.2,-0.422140257000017));
#189589=CARTESIAN_POINT('Ctrl Pts',(11.2430674209999,11.6,-0.422140257000017));
#189590=CARTESIAN_POINT('Ctrl Pts',(11.2399257469999,15.2,-0.420649373000015));
#189591=CARTESIAN_POINT('Ctrl Pts',(11.2399257469999,11.6,-0.420649373000015));
#189592=CARTESIAN_POINT('Ctrl Pts',(11.2367872269999,15.2,-0.419162996000013));
#189593=CARTESIAN_POINT('Ctrl Pts',(11.2367872269999,11.6,-0.419162996000014));
#189594=CARTESIAN_POINT('Ctrl Pts',(11.2336518709999,15.2,-0.417681128000016));
#189595=CARTESIAN_POINT('Ctrl Pts',(11.2336518709999,11.6,-0.417681128000016));
#189596=CARTESIAN_POINT('Ctrl Pts',(11.2305196889999,15.2,-0.416203762000014));
#189597=CARTESIAN_POINT('Ctrl Pts',(11.2305196889999,11.6,-0.416203762000014));
#189598=CARTESIAN_POINT('Ctrl Pts',(11.2273906889999,15.2,-0.414730898000015));
#189599=CARTESIAN_POINT('Ctrl Pts',(11.2273906889999,11.6,-0.414730898000016));
#189600=CARTESIAN_POINT('Ctrl Pts',(11.2242648839999,15.2,-0.413262534000012));
#189601=CARTESIAN_POINT('Ctrl Pts',(11.2242648839999,11.6,-0.413262534000012));
#189602=CARTESIAN_POINT('Ctrl Pts',(11.2211422809999,15.2,-0.411798667000016));
#189603=CARTESIAN_POINT('Ctrl Pts',(11.2211422809999,11.6,-0.411798667000017));
#189604=CARTESIAN_POINT('Ctrl Pts',(11.2180228899999,15.2,-0.410339294000015));
#189605=CARTESIAN_POINT('Ctrl Pts',(11.2180228899999,11.6,-0.410339294000015));
#189606=CARTESIAN_POINT('Ctrl Pts',(11.2149067229999,15.2,-0.408884414000017));
#189607=CARTESIAN_POINT('Ctrl Pts',(11.2149067229999,11.6,-0.408884414000017));
#189608=CARTESIAN_POINT('Ctrl Pts',(11.2117937879999,15.2,-0.407434024000013));
#189609=CARTESIAN_POINT('Ctrl Pts',(11.2117937879999,11.6,-0.407434024000013));
#189610=CARTESIAN_POINT('Ctrl Pts',(11.2086840959999,15.2,-0.405988122000016));
#189611=CARTESIAN_POINT('Ctrl Pts',(11.2086840959999,11.6,-0.405988122000017));
#189612=CARTESIAN_POINT('Ctrl Pts',(11.2055776569999,15.2,-0.404546706000013));
#189613=CARTESIAN_POINT('Ctrl Pts',(11.2055776569999,11.6,-0.404546706000013));
#189614=CARTESIAN_POINT('Ctrl Pts',(11.2024744809999,15.2,-0.403109771000012));
#189615=CARTESIAN_POINT('Ctrl Pts',(11.2024744809999,11.6,-0.403109771000012));
#189616=CARTESIAN_POINT('Ctrl Pts',(11.1993745769999,15.2,-0.401677318000013));
#189617=CARTESIAN_POINT('Ctrl Pts',(11.1993745769999,11.6,-0.401677318000014));
#189618=CARTESIAN_POINT('Ctrl Pts',(11.1962779569999,15.2,-0.400249342000016));
#189619=CARTESIAN_POINT('Ctrl Pts',(11.1962779569999,11.6,-0.400249342000017));
#189620=CARTESIAN_POINT('Ctrl Pts',(11.1931846289999,15.2,-0.398825842000012));
#189621=CARTESIAN_POINT('Ctrl Pts',(11.1931846289999,11.6,-0.398825842000013));
#189622=CARTESIAN_POINT('Ctrl Pts',(11.1900946029999,15.2,-0.397406815000014));
#189623=CARTESIAN_POINT('Ctrl Pts',(11.1900946029999,11.6,-0.397406815000015));
#189624=CARTESIAN_POINT('Ctrl Pts',(11.1870078909999,15.2,-0.395992258000017));
#189625=CARTESIAN_POINT('Ctrl Pts',(11.1870078909999,11.6,-0.395992258000018));
#189626=CARTESIAN_POINT('Ctrl Pts',(11.1839245019999,15.2,-0.394582170000017));
#189627=CARTESIAN_POINT('Ctrl Pts',(11.1839245019999,11.6,-0.394582170000018));
#189628=CARTESIAN_POINT('Ctrl Pts',(11.1808444459999,15.2,-0.393176547000014));
#189629=CARTESIAN_POINT('Ctrl Pts',(11.1808444459999,11.6,-0.393176547000014));
#189630=CARTESIAN_POINT('Ctrl Pts',(11.1777677329999,15.2,-0.391775387000015));
#189631=CARTESIAN_POINT('Ctrl Pts',(11.1777677329999,11.6,-0.391775387000016));
#189632=CARTESIAN_POINT('Ctrl Pts',(11.1746943739999,15.2,-0.390378688000013));
#189633=CARTESIAN_POINT('Ctrl Pts',(11.1746943739999,11.6,-0.390378688000013));
#189634=CARTESIAN_POINT('Ctrl Pts',(11.1716243779999,15.2,-0.388986447000015));
#189635=CARTESIAN_POINT('Ctrl Pts',(11.1716243779999,11.6,-0.388986447000015));
#189636=CARTESIAN_POINT('Ctrl Pts',(11.1685577559999,15.2,-0.387598660000013));
#189637=CARTESIAN_POINT('Ctrl Pts',(11.1685577559999,11.6,-0.387598660000013));
#189638=CARTESIAN_POINT('Ctrl Pts',(11.1654945179999,15.2,-0.386215328000015));
#189639=CARTESIAN_POINT('Ctrl Pts',(11.1654945179999,11.6,-0.386215328000015));
#189640=CARTESIAN_POINT('Ctrl Pts',(11.1624346739999,15.2,-0.384836446000012));
#189641=CARTESIAN_POINT('Ctrl Pts',(11.1624346739999,11.6,-0.384836446000012));
#189642=CARTESIAN_POINT('Ctrl Pts',(11.1593782349999,15.2,-0.383462011000013));
#189643=CARTESIAN_POINT('Ctrl Pts',(11.1593782349999,11.6,-0.383462011000014));
#189644=CARTESIAN_POINT('Ctrl Pts',(11.1563252099999,15.2,-0.382092022000013));
#189645=CARTESIAN_POINT('Ctrl Pts',(11.1563252099999,11.6,-0.382092022000014));
#189646=CARTESIAN_POINT('Ctrl Pts',(11.1532756099999,15.2,-0.380726475000017));
#189647=CARTESIAN_POINT('Ctrl Pts',(11.1532756099999,11.6,-0.380726475000018));
#189648=CARTESIAN_POINT('Ctrl Pts',(11.1502294459999,15.2,-0.379365367000015));
#189649=CARTESIAN_POINT('Ctrl Pts',(11.1502294459999,11.6,-0.379365367000016));
#189650=CARTESIAN_POINT('Ctrl Pts',(11.1471867269999,15.2,-0.378008697000016));
#189651=CARTESIAN_POINT('Ctrl Pts',(11.1471867269999,11.6,-0.378008697000017));
#189652=CARTESIAN_POINT('Ctrl Pts',(11.1441474629999,15.2,-0.376656462000016));
#189653=CARTESIAN_POINT('Ctrl Pts',(11.1441474629999,11.6,-0.376656462000016));
#189654=CARTESIAN_POINT('Ctrl Pts',(11.1411116659999,15.2,-0.375308658000013));
#189655=CARTESIAN_POINT('Ctrl Pts',(11.1411116659999,11.6,-0.375308658000014));
#189656=CARTESIAN_POINT('Ctrl Pts',(11.1380793459999,15.2,-0.373965284000013));
#189657=CARTESIAN_POINT('Ctrl Pts',(11.1380793459999,11.6,-0.373965284000013));
#189658=CARTESIAN_POINT('Ctrl Pts',(11.1350505129999,15.2,-0.372626336000015));
#189659=CARTESIAN_POINT('Ctrl Pts',(11.1350505129999,11.6,-0.372626336000015));
#189660=CARTESIAN_POINT('Ctrl Pts',(11.1320251769999,15.2,-0.371291812000014));
#189661=CARTESIAN_POINT('Ctrl Pts',(11.1320251769999,11.6,-0.371291812000015));
#189662=CARTESIAN_POINT('Ctrl Pts',(11.1290033489999,15.2,-0.369961709000015));
#189663=CARTESIAN_POINT('Ctrl Pts',(11.1290033489999,11.6,-0.369961709000016));
#189664=CARTESIAN_POINT('Ctrl Pts',(11.1259850389999,15.2,-0.368636024000013));
#189665=CARTESIAN_POINT('Ctrl Pts',(11.1259850389999,11.6,-0.368636024000013));
#189666=CARTESIAN_POINT('Ctrl Pts',(11.1229702569999,15.2,-0.367314755000017));
#189667=CARTESIAN_POINT('Ctrl Pts',(11.1229702569999,11.6,-0.367314755000017));
#189668=CARTESIAN_POINT('Ctrl Pts',(11.1199590149999,15.2,-0.365997899000017));
#189669=CARTESIAN_POINT('Ctrl Pts',(11.1199590149999,11.6,-0.365997899000017));
#189670=CARTESIAN_POINT('Ctrl Pts',(11.1169513219999,15.2,-0.364685453000018));
#189671=CARTESIAN_POINT('Ctrl Pts',(11.1169513219999,11.6,-0.364685453000018));
#189672=CARTESIAN_POINT('Ctrl Pts',(11.1139471899999,15.2,-0.363377413000014));
#189673=CARTESIAN_POINT('Ctrl Pts',(11.1139471899999,11.6,-0.363377413000015));
#189674=CARTESIAN_POINT('Ctrl Pts',(11.1109466279999,15.2,-0.362073779000016));
#189675=CARTESIAN_POINT('Ctrl Pts',(11.1109466279999,11.6,-0.362073779000017));
#189676=CARTESIAN_POINT('Ctrl Pts',(11.1079496479999,15.2,-0.360774546000013));
#189677=CARTESIAN_POINT('Ctrl Pts',(11.1079496479999,11.6,-0.360774546000014));
#189678=CARTESIAN_POINT('Ctrl Pts',(11.1049562589999,15.2,-0.359479712000015));
#189679=CARTESIAN_POINT('Ctrl Pts',(11.1049562589999,11.6,-0.359479712000015));
#189680=CARTESIAN_POINT('Ctrl Pts',(11.1019664729999,15.2,-0.358189274000011));
#189681=CARTESIAN_POINT('Ctrl Pts',(11.1019664729999,11.6,-0.358189274000012));
#189682=CARTESIAN_POINT('Ctrl Pts',(11.0989802999999,15.2,-0.356903228000016));
#189683=CARTESIAN_POINT('Ctrl Pts',(11.0989802999999,11.6,-0.356903228000017));
#189684=CARTESIAN_POINT('Ctrl Pts',(11.0959977499999,15.2,-0.355621573000011));
#189685=CARTESIAN_POINT('Ctrl Pts',(11.0959977499999,11.6,-0.355621573000012));
#189686=CARTESIAN_POINT('Ctrl Pts',(11.0930188349999,15.2,-0.354344304000014));
#189687=CARTESIAN_POINT('Ctrl Pts',(11.0930188349999,11.6,-0.354344304000014));
#189688=CARTESIAN_POINT('Ctrl Pts',(11.0900435649999,15.2,-0.353071421000015));
#189689=CARTESIAN_POINT('Ctrl Pts',(11.0900435649999,11.6,-0.353071421000016));
#189690=CARTESIAN_POINT('Ctrl Pts',(11.0870719499999,15.2,-0.351802918000015));
#189691=CARTESIAN_POINT('Ctrl Pts',(11.0870719499999,11.6,-0.351802918000015));
#189692=CARTESIAN_POINT('Ctrl Pts',(11.0841040009999,15.2,-0.350538795000013));
#189693=CARTESIAN_POINT('Ctrl Pts',(11.0841040009999,11.6,-0.350538795000013));
#189694=CARTESIAN_POINT('Ctrl Pts',(11.0811397299999,15.2,-0.349279047000017));
#189695=CARTESIAN_POINT('Ctrl Pts',(11.0811397299999,11.6,-0.349279047000018));
#189696=CARTESIAN_POINT('Ctrl Pts',(11.0781791459999,15.2,-0.348023671000015));
#189697=CARTESIAN_POINT('Ctrl Pts',(11.0781791459999,11.6,-0.348023671000016));
#189698=CARTESIAN_POINT('Ctrl Pts',(11.0752222619999,15.2,-0.346772665000015));
#189699=CARTESIAN_POINT('Ctrl Pts',(11.0752222619999,11.6,-0.346772665000015));
#189700=CARTESIAN_POINT('Ctrl Pts',(11.0722690859999,15.2,-0.345526025000016));
#189701=CARTESIAN_POINT('Ctrl Pts',(11.0722690859999,11.6,-0.345526025000016));
#189702=CARTESIAN_POINT('Ctrl Pts',(11.0693196309999,15.2,-0.344283750000014));
#189703=CARTESIAN_POINT('Ctrl Pts',(11.0693196309999,11.6,-0.344283750000014));
#189704=CARTESIAN_POINT('Ctrl Pts',(11.0663739069999,15.2,-0.343045834000013));
#189705=CARTESIAN_POINT('Ctrl Pts',(11.0663739069999,11.6,-0.343045834000014));
#189706=CARTESIAN_POINT('Ctrl Pts',(11.0634319249999,15.2,-0.341812275000013));
#189707=CARTESIAN_POINT('Ctrl Pts',(11.0634319249999,11.6,-0.341812275000013));
#189708=CARTESIAN_POINT('Ctrl Pts',(11.0604936949999,15.2,-0.340583072000014));
#189709=CARTESIAN_POINT('Ctrl Pts',(11.0604936949999,11.6,-0.340583072000014));
#189710=CARTESIAN_POINT('Ctrl Pts',(11.0575592289999,15.2,-0.339358220000014));
#189711=CARTESIAN_POINT('Ctrl Pts',(11.0575592289999,11.6,-0.339358220000015));
#189712=CARTESIAN_POINT('Ctrl Pts',(11.0546285369999,15.2,-0.338137715000015));
#189713=CARTESIAN_POINT('Ctrl Pts',(11.0546285369999,11.6,-0.338137715000016));
#189714=CARTESIAN_POINT('Ctrl Pts',(11.0517016309999,15.2,-0.336921557000016));
#189715=CARTESIAN_POINT('Ctrl Pts',(11.0517016309999,11.6,-0.336921557000017));
#189716=CARTESIAN_POINT('Ctrl Pts',(11.0487785209999,15.2,-0.335709740000016));
#189717=CARTESIAN_POINT('Ctrl Pts',(11.0487785209999,11.6,-0.335709740000017));
#189718=CARTESIAN_POINT('Ctrl Pts',(11.0458592189999,15.2,-0.334502262000012));
#189719=CARTESIAN_POINT('Ctrl Pts',(11.0458592189999,11.6,-0.334502262000012));
#189720=CARTESIAN_POINT('Ctrl Pts',(11.0429437349999,15.2,-0.333299120000015));
#189721=CARTESIAN_POINT('Ctrl Pts',(11.0429437349999,11.6,-0.333299120000015));
#189722=CARTESIAN_POINT('Ctrl Pts',(11.0400320799999,15.2,-0.332100311000012));
#189723=CARTESIAN_POINT('Ctrl Pts',(11.0400320799999,11.6,-0.332100311000012));
#189724=CARTESIAN_POINT('Ctrl Pts',(11.0371242659999,15.2,-0.330905831000017));
#189725=CARTESIAN_POINT('Ctrl Pts',(11.0371242659999,11.6,-0.330905831000017));
#189726=CARTESIAN_POINT('Ctrl Pts',(11.0342203029999,15.2,-0.329715677000015));
#189727=CARTESIAN_POINT('Ctrl Pts',(11.0342203029999,11.6,-0.329715677000016));
#189728=CARTESIAN_POINT('Ctrl Pts',(11.0313202029999,15.2,-0.328529847000016));
#189729=CARTESIAN_POINT('Ctrl Pts',(11.0313202029999,11.6,-0.328529847000017));
#189730=CARTESIAN_POINT('Ctrl Pts',(11.0284239769999,15.2,-0.327348336000015));
#189731=CARTESIAN_POINT('Ctrl Pts',(11.0284239769999,11.6,-0.327348336000016));
#189732=CARTESIAN_POINT('Ctrl Pts',(11.0255316349999,15.2,-0.326171141000016));
#189733=CARTESIAN_POINT('Ctrl Pts',(11.0255316349999,11.6,-0.326171141000016));
#189734=CARTESIAN_POINT('Ctrl Pts',(11.0226431889999,15.2,-0.324998260000013));
#189735=CARTESIAN_POINT('Ctrl Pts',(11.0226431889999,11.6,-0.324998260000014));
#189736=CARTESIAN_POINT('Ctrl Pts',(11.0197586499999,15.2,-0.323829688000017));
#189737=CARTESIAN_POINT('Ctrl Pts',(11.0197586499999,11.6,-0.323829688000017));
#189738=CARTESIAN_POINT('Ctrl Pts',(11.0168780289999,15.2,-0.322665425000017));
#189739=CARTESIAN_POINT('Ctrl Pts',(11.0168780289999,11.6,-0.322665425000018));
#189740=CARTESIAN_POINT('Ctrl Pts',(11.0140013379999,15.2,-0.321505464000014));
#189741=CARTESIAN_POINT('Ctrl Pts',(11.0140013379999,11.6,-0.321505464000014));
#189742=CARTESIAN_POINT('Ctrl Pts',(11.0111285869999,15.2,-0.320349803000015));
#189743=CARTESIAN_POINT('Ctrl Pts',(11.0111285869999,11.6,-0.320349803000016));
#189744=CARTESIAN_POINT('Ctrl Pts',(11.0082597879999,15.2,-0.319198439000012));
#189745=CARTESIAN_POINT('Ctrl Pts',(11.0082597879999,11.6,-0.319198439000013));
#189746=CARTESIAN_POINT('Ctrl Pts',(11.0053949529999,15.2,-0.318051369000014));
#189747=CARTESIAN_POINT('Ctrl Pts',(11.0053949529999,11.6,-0.318051369000015));
#189748=CARTESIAN_POINT('Ctrl Pts',(11.0025340919999,15.2,-0.316908589000011));
#189749=CARTESIAN_POINT('Ctrl Pts',(11.0025340919999,11.6,-0.316908589000012));
#189750=CARTESIAN_POINT('Ctrl Pts',(10.9996772159999,15.2,-0.315770095000012));
#189751=CARTESIAN_POINT('Ctrl Pts',(10.9996772159999,11.6,-0.315770095000012));
#189752=CARTESIAN_POINT('Ctrl Pts',(10.9968243389999,15.2,-0.314635885000012));
#189753=CARTESIAN_POINT('Ctrl Pts',(10.9968243389999,11.6,-0.314635885000012));
#189754=CARTESIAN_POINT('Ctrl Pts',(10.9939754689999,15.2,-0.313505954000015));
#189755=CARTESIAN_POINT('Ctrl Pts',(10.9939754689999,11.6,-0.313505954000016));
#189756=CARTESIAN_POINT('Ctrl Pts',(10.9911306189999,15.2,-0.312380300000012));
#189757=CARTESIAN_POINT('Ctrl Pts',(10.9911306189999,11.6,-0.312380300000013));
#189758=CARTESIAN_POINT('Ctrl Pts',(10.9882897999999,15.2,-0.311258919000017));
#189759=CARTESIAN_POINT('Ctrl Pts',(10.9882897999999,11.6,-0.311258919000017));
#189760=CARTESIAN_POINT('Ctrl Pts',(10.9854530239999,15.2,-0.310141807000015));
#189761=CARTESIAN_POINT('Ctrl Pts',(10.9854530239999,11.6,-0.310141807000015));
#189762=CARTESIAN_POINT('Ctrl Pts',(10.9826203019999,15.2,-0.309028962000015));
#189763=CARTESIAN_POINT('Ctrl Pts',(10.9826203019999,11.6,-0.309028962000016));
#189764=CARTESIAN_POINT('Ctrl Pts',(10.9797916459999,15.2,-0.307920379000013));
#189765=CARTESIAN_POINT('Ctrl Pts',(10.9797916459999,11.6,-0.307920379000013));
#189766=CARTESIAN_POINT('Ctrl Pts',(10.9769670669999,15.2,-0.306816055000017));
#189767=CARTESIAN_POINT('Ctrl Pts',(10.9769670669999,11.6,-0.306816055000017));
#189768=CARTESIAN_POINT('Ctrl Pts',(10.9741465759999,15.2,-0.305715987000017));
#189769=CARTESIAN_POINT('Ctrl Pts',(10.9741465759999,11.6,-0.305715987000017));
#189770=CARTESIAN_POINT('Ctrl Pts',(10.9713301849999,15.2,-0.304620170000014));
#189771=CARTESIAN_POINT('Ctrl Pts',(10.9713301849999,11.6,-0.304620170000014));
#189772=CARTESIAN_POINT('Ctrl Pts',(10.9685179069999,15.2,-0.303528602000016));
#189773=CARTESIAN_POINT('Ctrl Pts',(10.9685179069999,11.6,-0.303528602000017));
#189774=CARTESIAN_POINT('Ctrl Pts',(10.9657097509999,15.2,-0.302441280000014));
#189775=CARTESIAN_POINT('Ctrl Pts',(10.9657097509999,11.6,-0.302441280000015));
#189776=CARTESIAN_POINT('Ctrl Pts',(10.9629057309999,15.2,-0.301358197000017));
#189777=CARTESIAN_POINT('Ctrl Pts',(10.9629057309999,11.6,-0.301358197000017));
#189778=CARTESIAN_POINT('Ctrl Pts',(10.9601058569999,15.2,-0.300279353000015));
#189779=CARTESIAN_POINT('Ctrl Pts',(10.9601058569999,11.6,-0.300279353000015));
#189780=CARTESIAN_POINT('Ctrl Pts',(10.9573101409999,15.2,-0.299204743000012));
#189781=CARTESIAN_POINT('Ctrl Pts',(10.9573101409999,11.6,-0.299204743000013));
#189782=CARTESIAN_POINT('Ctrl Pts',(10.9545185949999,15.2,-0.298134363000013));
#189783=CARTESIAN_POINT('Ctrl Pts',(10.9545185949999,11.6,-0.298134363000014));
#189784=CARTESIAN_POINT('Ctrl Pts',(10.9517312309999,15.2,-0.297068209000013));
#189785=CARTESIAN_POINT('Ctrl Pts',(10.9517312309999,11.6,-0.297068209000014));
#189786=CARTESIAN_POINT('Ctrl Pts',(10.9489480589999,15.2,-0.296006279000016));
#189787=CARTESIAN_POINT('Ctrl Pts',(10.9489480589999,11.6,-0.296006279000017));
#189788=CARTESIAN_POINT('Ctrl Pts',(10.9461690929999,15.2,-0.294948568000013));
#189789=CARTESIAN_POINT('Ctrl Pts',(10.9461690929999,11.6,-0.294948568000013));
#189790=CARTESIAN_POINT('Ctrl Pts',(10.9433943439999,15.2,-0.293895072000012));
#189791=CARTESIAN_POINT('Ctrl Pts',(10.9433943439999,11.6,-0.293895072000013));
#189792=CARTESIAN_POINT('Ctrl Pts',(10.9406238229999,15.2,-0.292845788000013));
#189793=CARTESIAN_POINT('Ctrl Pts',(10.9406238229999,11.6,-0.292845788000014));
#189794=CARTESIAN_POINT('Ctrl Pts',(10.9378575429999,15.2,-0.291800712000012));
#189795=CARTESIAN_POINT('Ctrl Pts',(10.9378575429999,11.6,-0.291800712000013));
#189796=CARTESIAN_POINT('Ctrl Pts',(10.9350955149999,15.2,-0.290759841000017));
#189797=CARTESIAN_POINT('Ctrl Pts',(10.9350955149999,11.6,-0.290759841000017));
#189798=CARTESIAN_POINT('Ctrl Pts',(10.9323377509999,15.2,-0.289723170000014));
#189799=CARTESIAN_POINT('Ctrl Pts',(10.9323377509999,11.6,-0.289723170000014));
#189800=CARTESIAN_POINT('Ctrl Pts',(10.9295842629999,15.2,-0.288690696000016));
#189801=CARTESIAN_POINT('Ctrl Pts',(10.9295842629999,11.6,-0.288690696000016));
#189802=CARTESIAN_POINT('Ctrl Pts',(10.9268350629999,15.2,-0.287662415000014));
#189803=CARTESIAN_POINT('Ctrl Pts',(10.9268350629999,11.6,-0.287662415000014));
#189804=CARTESIAN_POINT('Ctrl Pts',(10.9240901629999,15.2,-0.286638322000012));
#189805=CARTESIAN_POINT('Ctrl Pts',(10.9240901629999,11.6,-0.286638322000013));
#189806=CARTESIAN_POINT('Ctrl Pts',(10.9213495759999,15.2,-0.285618415000015));
#189807=CARTESIAN_POINT('Ctrl Pts',(10.9213495759999,11.6,-0.285618415000016));
#189808=CARTESIAN_POINT('Ctrl Pts',(10.9186133109999,15.2,-0.284602689000018));
#189809=CARTESIAN_POINT('Ctrl Pts',(10.9186133109999,11.6,-0.284602689000018));
#189810=CARTESIAN_POINT('Ctrl Pts',(10.9158813839999,15.2,-0.283591141000015));
#189811=CARTESIAN_POINT('Ctrl Pts',(10.9158813839999,11.6,-0.283591141000015));
#189812=CARTESIAN_POINT('Ctrl Pts',(10.9131538029999,15.2,-0.282583766000015));
#189813=CARTESIAN_POINT('Ctrl Pts',(10.9131538029999,11.6,-0.282583766000016));
#189814=CARTESIAN_POINT('Ctrl Pts',(10.9104305819999,15.2,-0.281580561000014));
#189815=CARTESIAN_POINT('Ctrl Pts',(10.9104305819999,11.6,-0.281580561000015));
#189816=CARTESIAN_POINT('Ctrl Pts',(10.9077117349999,15.2,-0.280581520000016));
#189817=CARTESIAN_POINT('Ctrl Pts',(10.9077117349999,11.6,-0.280581520000017));
#189818=CARTESIAN_POINT('Ctrl Pts',(10.9049972699999,15.2,-0.279586642000016));
#189819=CARTESIAN_POINT('Ctrl Pts',(10.9049972699999,11.6,-0.279586642000016));
#189820=CARTESIAN_POINT('Ctrl Pts',(10.9022872019999,15.2,-0.278595921000013));
#189821=CARTESIAN_POINT('Ctrl Pts',(10.9022872019999,11.6,-0.278595921000014));
#189822=CARTESIAN_POINT('Ctrl Pts',(10.8995815439999,15.2,-0.277609354000017));
#189823=CARTESIAN_POINT('Ctrl Pts',(10.8995815439999,11.6,-0.277609354000017));
#189824=CARTESIAN_POINT('Ctrl Pts',(10.8968803049999,15.2,-0.276626936000017));
#189825=CARTESIAN_POINT('Ctrl Pts',(10.8968803049999,11.6,-0.276626936000018));
#189826=CARTESIAN_POINT('Ctrl Pts',(10.8941834999999,15.2,-0.275648665000015));
#189827=CARTESIAN_POINT('Ctrl Pts',(10.8941834999999,11.6,-0.275648665000015));
#189828=CARTESIAN_POINT('Ctrl Pts',(10.8914911399999,15.2,-0.274674534000017));
#189829=CARTESIAN_POINT('Ctrl Pts',(10.8914911399999,11.6,-0.274674534000017));
#189830=CARTESIAN_POINT('Ctrl Pts',(10.8888032369999,15.2,-0.273704541000015));
#189831=CARTESIAN_POINT('Ctrl Pts',(10.8888032369999,11.6,-0.273704541000015));
#189832=CARTESIAN_POINT('Ctrl Pts',(10.8861198049999,15.2,-0.272738682000018));
#189833=CARTESIAN_POINT('Ctrl Pts',(10.8861198049999,11.6,-0.272738682000018));
#189834=CARTESIAN_POINT('Ctrl Pts',(10.8834408539999,15.2,-0.271776950000016));
#189835=CARTESIAN_POINT('Ctrl Pts',(10.8834408539999,11.6,-0.271776950000016));
#189836=CARTESIAN_POINT('Ctrl Pts',(10.8807663989999,15.2,-0.270819345000017));
#189837=CARTESIAN_POINT('Ctrl Pts',(10.8807663989999,11.6,-0.270819345000018));
#189838=CARTESIAN_POINT('Ctrl Pts',(10.8780964489999,15.2,-0.269865861000014));
#189839=CARTESIAN_POINT('Ctrl Pts',(10.8780964489999,11.6,-0.269865861000014));
#189840=CARTESIAN_POINT('Ctrl Pts',(10.8754310189999,15.2,-0.268916493000013));
#189841=CARTESIAN_POINT('Ctrl Pts',(10.8754310189999,11.6,-0.268916493000014));
#189842=CARTESIAN_POINT('Ctrl Pts',(10.8727701199999,15.2,-0.267971237000015));
#189843=CARTESIAN_POINT('Ctrl Pts',(10.8727701199999,11.6,-0.267971237000016));
#189844=CARTESIAN_POINT('Ctrl Pts',(10.8701137659999,15.2,-0.267030089000015));
#189845=CARTESIAN_POINT('Ctrl Pts',(10.8701137659999,11.6,-0.267030089000016));
#189846=CARTESIAN_POINT('Ctrl Pts',(10.8674619699999,15.2,-0.266093046000013));
#189847=CARTESIAN_POINT('Ctrl Pts',(10.8674619699999,11.6,-0.266093046000014));
#189848=CARTESIAN_POINT('Ctrl Pts',(10.8648147409999,15.2,-0.265160103000017));
#189849=CARTESIAN_POINT('Ctrl Pts',(10.8648147409999,11.6,-0.265160103000018));
#189850=CARTESIAN_POINT('Ctrl Pts',(10.8621720949999,15.2,-0.264231254000014));
#189851=CARTESIAN_POINT('Ctrl Pts',(10.8621720949999,11.6,-0.264231254000014));
#189852=CARTESIAN_POINT('Ctrl Pts',(10.8595340429999,15.2,-0.263306498000015));
#189853=CARTESIAN_POINT('Ctrl Pts',(10.8595340429999,11.6,-0.263306498000016));
#189854=CARTESIAN_POINT('Ctrl Pts',(10.8569005969999,15.2,-0.262385828000014));
#189855=CARTESIAN_POINT('Ctrl Pts',(10.8569005969999,11.6,-0.262385828000014));
#189856=CARTESIAN_POINT('Ctrl Pts',(10.8542717719999,15.2,-0.261469241000012));
#189857=CARTESIAN_POINT('Ctrl Pts',(10.8542717719999,11.6,-0.261469241000012));
#189858=CARTESIAN_POINT('Ctrl Pts',(10.8516475779999,15.2,-0.260556732000015));
#189859=CARTESIAN_POINT('Ctrl Pts',(10.8516475779999,11.6,-0.260556732000015));
#189860=CARTESIAN_POINT('Ctrl Pts',(10.8490280299999,15.2,-0.259648296000012));
#189861=CARTESIAN_POINT('Ctrl Pts',(10.8490280299999,11.6,-0.259648296000013));
#189862=CARTESIAN_POINT('Ctrl Pts',(10.8464131379999,15.2,-0.258743931000014));
#189863=CARTESIAN_POINT('Ctrl Pts',(10.8464131379999,11.6,-0.258743931000014));
#189864=CARTESIAN_POINT('Ctrl Pts',(10.8438029179999,15.2,-0.257843630000014));
#189865=CARTESIAN_POINT('Ctrl Pts',(10.8438029179999,11.6,-0.257843630000015));
#189866=CARTESIAN_POINT('Ctrl Pts',(10.8411973799999,15.2,-0.256947389000013));
#189867=CARTESIAN_POINT('Ctrl Pts',(10.8411973799999,11.6,-0.256947389000013));
#189868=CARTESIAN_POINT('Ctrl Pts',(10.8385965389999,15.2,-0.256055205000014));
#189869=CARTESIAN_POINT('Ctrl Pts',(10.8385965389999,11.6,-0.256055205000015));
#189870=CARTESIAN_POINT('Ctrl Pts',(10.8360004059999,15.2,-0.255167073000013));
#189871=CARTESIAN_POINT('Ctrl Pts',(10.8360004059999,11.6,-0.255167073000014));
#189872=CARTESIAN_POINT('Ctrl Pts',(10.8334089939999,15.2,-0.254282987000014));
#189873=CARTESIAN_POINT('Ctrl Pts',(10.8334089939999,11.6,-0.254282987000015));
#189874=CARTESIAN_POINT('Ctrl Pts',(10.8308223169999,15.2,-0.253402945000012));
#189875=CARTESIAN_POINT('Ctrl Pts',(10.8308223169999,11.6,-0.253402945000012));
#189876=CARTESIAN_POINT('Ctrl Pts',(10.8282403869999,15.2,-0.252526940000015));
#189877=CARTESIAN_POINT('Ctrl Pts',(10.8282403869999,11.6,-0.252526940000016));
#189878=CARTESIAN_POINT('Ctrl Pts',(10.8256632179999,15.2,-0.251654969000015));
#189879=CARTESIAN_POINT('Ctrl Pts',(10.8256632179999,11.6,-0.251654969000015));
#189880=CARTESIAN_POINT('Ctrl Pts',(10.8230908219999,15.2,-0.250787027000015));
#189881=CARTESIAN_POINT('Ctrl Pts',(10.8230908219999,11.6,-0.250787027000015));
#189882=CARTESIAN_POINT('Ctrl Pts',(10.8205232129999,15.2,-0.249923108000014));
#189883=CARTESIAN_POINT('Ctrl Pts',(10.8205232129999,11.6,-0.249923108000015));
#189884=CARTESIAN_POINT('Ctrl Pts',(10.8179604029999,15.2,-0.249063210000013));
#189885=CARTESIAN_POINT('Ctrl Pts',(10.8179604029999,11.6,-0.249063210000014));
#189886=CARTESIAN_POINT('Ctrl Pts',(10.8154024049999,15.2,-0.248207327000016));
#189887=CARTESIAN_POINT('Ctrl Pts',(10.8154024049999,11.6,-0.248207327000017));
#189888=CARTESIAN_POINT('Ctrl Pts',(10.8128492319999,15.2,-0.247355454000013));
#189889=CARTESIAN_POINT('Ctrl Pts',(10.8128492319999,11.6,-0.247355454000014));
#189890=CARTESIAN_POINT('Ctrl Pts',(10.8103008979999,15.2,-0.246507587000018));
#189891=CARTESIAN_POINT('Ctrl Pts',(10.8103008979999,11.6,-0.246507587000018));
#189892=CARTESIAN_POINT('Ctrl Pts',(10.8077574159999,15.2,-0.245663720000016));
#189893=CARTESIAN_POINT('Ctrl Pts',(10.8077574159999,11.6,-0.245663720000016));
#189894=CARTESIAN_POINT('Ctrl Pts',(10.8052187989999,15.2,-0.244823851000016));
#189895=CARTESIAN_POINT('Ctrl Pts',(10.8052187989999,11.6,-0.244823851000016));
#189896=CARTESIAN_POINT('Ctrl Pts',(10.8026850599999,15.2,-0.243987972000017));
#189897=CARTESIAN_POINT('Ctrl Pts',(10.8026850599999,11.6,-0.243987972000018));
#189898=CARTESIAN_POINT('Ctrl Pts',(10.8001562119999,15.2,-0.243156081000016));
#189899=CARTESIAN_POINT('Ctrl Pts',(10.8001562119999,11.6,-0.243156081000016));
#189900=CARTESIAN_POINT('Ctrl Pts',(10.7976322689999,15.2,-0.242328170000015));
#189901=CARTESIAN_POINT('Ctrl Pts',(10.7976322689999,11.6,-0.242328170000015));
#189902=CARTESIAN_POINT('Ctrl Pts',(10.7951132439999,15.2,-0.241504237000014));
#189903=CARTESIAN_POINT('Ctrl Pts',(10.7951132439999,11.6,-0.241504237000015));
#189904=CARTESIAN_POINT('Ctrl Pts',(10.7925991499999,15.2,-0.240684278000014));
#189905=CARTESIAN_POINT('Ctrl Pts',(10.7925991499999,11.6,-0.240684278000014));
#189906=CARTESIAN_POINT('Ctrl Pts',(10.7900900009999,15.2,-0.239868284000018));
#189907=CARTESIAN_POINT('Ctrl Pts',(10.7900900009999,11.6,-0.239868284000018));
#189908=CARTESIAN_POINT('Ctrl Pts',(10.7875858089999,15.2,-0.239056253000012));
#189909=CARTESIAN_POINT('Ctrl Pts',(10.7875858089999,11.6,-0.239056253000012));
#189910=CARTESIAN_POINT('Ctrl Pts',(10.7850865899999,15.2,-0.238248181000014));
#189911=CARTESIAN_POINT('Ctrl Pts',(10.7850865899999,11.6,-0.238248181000014));
#189912=CARTESIAN_POINT('Ctrl Pts',(10.7825923549999,15.2,-0.237444060000014));
#189913=CARTESIAN_POINT('Ctrl Pts',(10.7825923549999,11.6,-0.237444060000014));
#189914=CARTESIAN_POINT('Ctrl Pts',(10.7801031189999,15.2,-0.236643887000016));
#189915=CARTESIAN_POINT('Ctrl Pts',(10.7801031189999,11.6,-0.236643887000017));
#189916=CARTESIAN_POINT('Ctrl Pts',(10.7776188939999,15.2,-0.235847657000012));
#189917=CARTESIAN_POINT('Ctrl Pts',(10.7776188939999,11.6,-0.235847657000013));
#189918=CARTESIAN_POINT('Ctrl Pts',(10.7751396949999,15.2,-0.235055365000014));
#189919=CARTESIAN_POINT('Ctrl Pts',(10.7751396949999,11.6,-0.235055365000015));
#189920=CARTESIAN_POINT('Ctrl Pts',(10.7726655359999,15.2,-0.234267005000017));
#189921=CARTESIAN_POINT('Ctrl Pts',(10.7726655359999,11.6,-0.234267005000018));
#189922=CARTESIAN_POINT('Ctrl Pts',(10.7701964279999,15.2,-0.233482574000017));
#189923=CARTESIAN_POINT('Ctrl Pts',(10.7701964279999,11.6,-0.233482574000017));
#189924=CARTESIAN_POINT('Ctrl Pts',(10.7677323879999,15.2,-0.232702063000012));
#189925=CARTESIAN_POINT('Ctrl Pts',(10.7677323879999,11.6,-0.232702063000013));
#189926=CARTESIAN_POINT('Ctrl Pts',(10.7652734269999,15.2,-0.231925472000012));
#189927=CARTESIAN_POINT('Ctrl Pts',(10.7652734269999,11.6,-0.231925472000012));
#189928=CARTESIAN_POINT('Ctrl Pts',(10.7628195609999,15.2,-0.231152792000016));
#189929=CARTESIAN_POINT('Ctrl Pts',(10.7628195609999,11.6,-0.231152792000016));
#189930=CARTESIAN_POINT('Ctrl Pts',(10.7603708009999,15.2,-0.230384019000014));
#189931=CARTESIAN_POINT('Ctrl Pts',(10.7603708009999,11.6,-0.230384019000014));
#189932=CARTESIAN_POINT('Ctrl Pts',(10.7579271629999,15.2,-0.229619149000015));
#189933=CARTESIAN_POINT('Ctrl Pts',(10.7579271629999,11.6,-0.229619149000016));
#189934=CARTESIAN_POINT('Ctrl Pts',(10.7554886599999,15.2,-0.228858176000015));
#189935=CARTESIAN_POINT('Ctrl Pts',(10.7554886599999,11.6,-0.228858176000016));
#189936=CARTESIAN_POINT('Ctrl Pts',(10.7530553059999,15.2,-0.228101094000017));
#189937=CARTESIAN_POINT('Ctrl Pts',(10.7530553059999,11.6,-0.228101094000018));
#189938=CARTESIAN_POINT('Ctrl Pts',(10.7506271149999,15.2,-0.227347899000012));
#189939=CARTESIAN_POINT('Ctrl Pts',(10.7506271149999,11.6,-0.227347899000013));
#189940=CARTESIAN_POINT('Ctrl Pts',(10.7482041009999,15.2,-0.226598584000013));
#189941=CARTESIAN_POINT('Ctrl Pts',(10.7482041009999,11.6,-0.226598584000013));
#189942=CARTESIAN_POINT('Ctrl Pts',(10.7457862769999,15.2,-0.225853146000015));
#189943=CARTESIAN_POINT('Ctrl Pts',(10.7457862769999,11.6,-0.225853146000015));
#189944=CARTESIAN_POINT('Ctrl Pts',(10.7433736579999,15.2,-0.225111577000017));
#189945=CARTESIAN_POINT('Ctrl Pts',(10.7433736579999,11.6,-0.225111577000017));
#189946=CARTESIAN_POINT('Ctrl Pts',(10.7409662579999,15.2,-0.224373875000015));
#189947=CARTESIAN_POINT('Ctrl Pts',(10.7409662579999,11.6,-0.224373875000015));
#189948=CARTESIAN_POINT('Ctrl Pts',(10.7385640919999,15.2,-0.223640032000016));
#189949=CARTESIAN_POINT('Ctrl Pts',(10.7385640919999,11.6,-0.223640032000017));
#189950=CARTESIAN_POINT('Ctrl Pts',(10.7361671709999,15.2,-0.222910044000013));
#189951=CARTESIAN_POINT('Ctrl Pts',(10.7361671709999,11.6,-0.222910044000014));
#189952=CARTESIAN_POINT('Ctrl Pts',(10.7337755109999,15.2,-0.222183905000013));
#189953=CARTESIAN_POINT('Ctrl Pts',(10.7337755109999,11.6,-0.222183905000013));
#189954=CARTESIAN_POINT('Ctrl Pts',(10.7313891279999,15.2,-0.221461609000015));
#189955=CARTESIAN_POINT('Ctrl Pts',(10.7313891279999,11.6,-0.221461609000016));
#189956=CARTESIAN_POINT('Ctrl Pts',(10.7290080319999,15.2,-0.220743152000011));
#189957=CARTESIAN_POINT('Ctrl Pts',(10.7290080319999,11.6,-0.220743152000012));
#189958=CARTESIAN_POINT('Ctrl Pts',(10.7266322409999,15.2,-0.220028527000018));
#189959=CARTESIAN_POINT('Ctrl Pts',(10.7266322409999,11.6,-0.220028527000018));
#189960=CARTESIAN_POINT('Ctrl Pts',(10.7242617679999,15.2,-0.219317729000017));
#189961=CARTESIAN_POINT('Ctrl Pts',(10.7242617679999,11.6,-0.219317729000017));
#189962=CARTESIAN_POINT('Ctrl Pts',(10.7218966269999,15.2,-0.218610753000017));
#189963=CARTESIAN_POINT('Ctrl Pts',(10.7218966269999,11.6,-0.218610753000017));
#189964=CARTESIAN_POINT('Ctrl Pts',(10.7195368329999,15.2,-0.217907593000017));
#189965=CARTESIAN_POINT('Ctrl Pts',(10.7195368329999,11.6,-0.217907593000018));
#189966=CARTESIAN_POINT('Ctrl Pts',(10.7171823989999,15.2,-0.217208244000013));
#189967=CARTESIAN_POINT('Ctrl Pts',(10.7171823989999,11.6,-0.217208244000014));
#189968=CARTESIAN_POINT('Ctrl Pts',(10.7148333409999,15.2,-0.216512699000013));
#189969=CARTESIAN_POINT('Ctrl Pts',(10.7148333409999,11.6,-0.216512699000014));
#189970=CARTESIAN_POINT('Ctrl Pts',(10.7124896719999,15.2,-0.215820955000012));
#189971=CARTESIAN_POINT('Ctrl Pts',(10.7124896719999,11.6,-0.215820955000013));
#189972=CARTESIAN_POINT('Ctrl Pts',(10.7101514079999,15.2,-0.215133003000014));
#189973=CARTESIAN_POINT('Ctrl Pts',(10.7101514079999,11.6,-0.215133003000015));
#189974=CARTESIAN_POINT('Ctrl Pts',(10.7078185619999,15.2,-0.214448839000014));
#189975=CARTESIAN_POINT('Ctrl Pts',(10.7078185619999,11.6,-0.214448839000015));
#189976=CARTESIAN_POINT('Ctrl Pts',(10.7054911499999,15.2,-0.213768458000012));
#189977=CARTESIAN_POINT('Ctrl Pts',(10.7054911499999,11.6,-0.213768458000013));
#189978=CARTESIAN_POINT('Ctrl Pts',(10.7031691859999,15.2,-0.213091853000016));
#189979=CARTESIAN_POINT('Ctrl Pts',(10.7031691859999,11.6,-0.213091853000016));
#189980=CARTESIAN_POINT('Ctrl Pts',(10.7008526839999,15.2,-0.212419018000016));
#189981=CARTESIAN_POINT('Ctrl Pts',(10.7008526839999,11.6,-0.212419018000017));
#189982=CARTESIAN_POINT('Ctrl Pts',(10.6985416599999,15.2,-0.211749949000013));
#189983=CARTESIAN_POINT('Ctrl Pts',(10.6985416599999,11.6,-0.211749949000013));
#189984=CARTESIAN_POINT('Ctrl Pts',(10.6962361279999,15.2,-0.211084638000014));
#189985=CARTESIAN_POINT('Ctrl Pts',(10.6962361279999,11.6,-0.211084638000015));
#189986=CARTESIAN_POINT('Ctrl Pts',(10.6939361019999,15.2,-0.210423081000015));
#189987=CARTESIAN_POINT('Ctrl Pts',(10.6939361019999,11.6,-0.210423081000016));
#189988=CARTESIAN_POINT('Ctrl Pts',(10.6916415969999,15.2,-0.209765271000015));
#189989=CARTESIAN_POINT('Ctrl Pts',(10.6916415969999,11.6,-0.209765271000016));
#189990=CARTESIAN_POINT('Ctrl Pts',(10.6893526289999,15.2,-0.209111203000014));
#189991=CARTESIAN_POINT('Ctrl Pts',(10.6893526289999,11.6,-0.209111203000015));
#189992=CARTESIAN_POINT('Ctrl Pts',(10.6870692119999,15.2,-0.208460870000016));
#189993=CARTESIAN_POINT('Ctrl Pts',(10.6870692119999,11.6,-0.208460870000016));
#189994=CARTESIAN_POINT('Ctrl Pts',(10.6847913619999,15.2,-0.207814266000015));
#189995=CARTESIAN_POINT('Ctrl Pts',(10.6847913619999,11.6,-0.207814266000015));
#189996=CARTESIAN_POINT('Ctrl Pts',(10.6825190919999,15.2,-0.207171387000016));
#189997=CARTESIAN_POINT('Ctrl Pts',(10.6825190919999,11.6,-0.207171387000016));
#189998=CARTESIAN_POINT('Ctrl Pts',(10.6802524189999,15.2,-0.206532225000018));
#189999=CARTESIAN_POINT('Ctrl Pts',(10.6802524189999,11.6,-0.206532225000018));
#190000=CARTESIAN_POINT('Ctrl Pts',(10.6779913559999,15.2,-0.205896774000016));
#190001=CARTESIAN_POINT('Ctrl Pts',(10.6779913559999,11.6,-0.205896774000017));
#190002=CARTESIAN_POINT('Ctrl Pts',(10.6757359199999,15.2,-0.205265028000015));
#190003=CARTESIAN_POINT('Ctrl Pts',(10.6757359199999,11.6,-0.205265028000015));
#190004=CARTESIAN_POINT('Ctrl Pts',(10.6734861239999,15.2,-0.204636983000013));
#190005=CARTESIAN_POINT('Ctrl Pts',(10.6734861239999,11.6,-0.204636983000013));
#190006=CARTESIAN_POINT('Ctrl Pts',(10.6712419859999,15.2,-0.204012630000014));
#190007=CARTESIAN_POINT('Ctrl Pts',(10.6712419859999,11.6,-0.204012630000015));
#190008=CARTESIAN_POINT('Ctrl Pts',(10.6690035179999,15.2,-0.203391965000015));
#190009=CARTESIAN_POINT('Ctrl Pts',(10.6690035179999,11.6,-0.203391965000015));
#190010=CARTESIAN_POINT('Ctrl Pts',(10.6667707369999,15.2,-0.202774980000013));
#190011=CARTESIAN_POINT('Ctrl Pts',(10.6667707369999,11.6,-0.202774980000014));
#190012=CARTESIAN_POINT('Ctrl Pts',(10.6645436589999,15.2,-0.202161669000014));
#190013=CARTESIAN_POINT('Ctrl Pts',(10.6645436589999,11.6,-0.202161669000014));
#190014=CARTESIAN_POINT('Ctrl Pts',(10.6623222969999,15.2,-0.201552028000016));
#190015=CARTESIAN_POINT('Ctrl Pts',(10.6623222969999,11.6,-0.201552028000016));
#190016=CARTESIAN_POINT('Ctrl Pts',(10.6601066689999,15.2,-0.200946048000015));
#190017=CARTESIAN_POINT('Ctrl Pts',(10.6601066689999,11.6,-0.200946048000015));
#190018=CARTESIAN_POINT('Ctrl Pts',(10.6578967889999,15.2,-0.200343724000014));
#190019=CARTESIAN_POINT('Ctrl Pts',(10.6578967889999,11.6,-0.200343724000014));
#190020=CARTESIAN_POINT('Ctrl Pts',(10.6556926709999,15.2,-0.199745050000013));
#190021=CARTESIAN_POINT('Ctrl Pts',(10.6556926709999,11.6,-0.199745050000014));
#190022=CARTESIAN_POINT('Ctrl Pts',(10.6534943329999,15.2,-0.199150020000012));
#190023=CARTESIAN_POINT('Ctrl Pts',(10.6534943329999,11.6,-0.199150020000012));
#190024=CARTESIAN_POINT('Ctrl Pts',(10.6513017899999,15.2,-0.198558626000014));
#190025=CARTESIAN_POINT('Ctrl Pts',(10.6513017899999,11.6,-0.198558626000014));
#190026=CARTESIAN_POINT('Ctrl Pts',(10.6491150549999,15.2,-0.197970862000014));
#190027=CARTESIAN_POINT('Ctrl Pts',(10.6491150549999,11.6,-0.197970862000015));
#190028=CARTESIAN_POINT('Ctrl Pts',(10.6469341469999,15.2,-0.197386722000013));
#190029=CARTESIAN_POINT('Ctrl Pts',(10.6469341469999,11.6,-0.197386722000013));
#190030=CARTESIAN_POINT('Ctrl Pts',(10.6447590809999,15.2,-0.196806200000013));
#190031=CARTESIAN_POINT('Ctrl Pts',(10.6447590809999,11.6,-0.196806200000013));
#190032=CARTESIAN_POINT('Ctrl Pts',(10.6425898709999,15.2,-0.196229289000014));
#190033=CARTESIAN_POINT('Ctrl Pts',(10.6425898709999,11.6,-0.196229289000014));
#190034=CARTESIAN_POINT('Ctrl Pts',(10.6404265339999,15.2,-0.195655982000016));
#190035=CARTESIAN_POINT('Ctrl Pts',(10.6404265339999,11.6,-0.195655982000016));
#190036=CARTESIAN_POINT('Ctrl Pts',(10.6382690849999,15.2,-0.195086273000014));
#190037=CARTESIAN_POINT('Ctrl Pts',(10.6382690849999,11.6,-0.195086273000014));
#190038=CARTESIAN_POINT('Ctrl Pts',(10.6361175409999,15.2,-0.194520155000015));
#190039=CARTESIAN_POINT('Ctrl Pts',(10.6361175409999,11.6,-0.194520155000016));
#190040=CARTESIAN_POINT('Ctrl Pts',(10.6339719169999,15.2,-0.193957622000016));
#190041=CARTESIAN_POINT('Ctrl Pts',(10.6339719169999,11.6,-0.193957622000017));
#190042=CARTESIAN_POINT('Ctrl Pts',(10.6318322289999,15.2,-0.193398667000015));
#190043=CARTESIAN_POINT('Ctrl Pts',(10.6318322289999,11.6,-0.193398667000016));
#190044=CARTESIAN_POINT('Ctrl Pts',(10.6296984919999,15.2,-0.192843283000013));
#190045=CARTESIAN_POINT('Ctrl Pts',(10.6296984919999,11.6,-0.192843283000013));
#190046=CARTESIAN_POINT('Ctrl Pts',(10.6275707239999,15.2,-0.192291464000016));
#190047=CARTESIAN_POINT('Ctrl Pts',(10.6275707239999,11.6,-0.192291464000017));
#190048=CARTESIAN_POINT('Ctrl Pts',(10.6254489389999,15.2,-0.191743203000012));
#190049=CARTESIAN_POINT('Ctrl Pts',(10.6254489389999,11.6,-0.191743203000013));
#190050=CARTESIAN_POINT('Ctrl Pts',(10.6233331559999,15.2,-0.191198492000013));
#190051=CARTESIAN_POINT('Ctrl Pts',(10.6233331559999,11.6,-0.191198492000014));
#190052=CARTESIAN_POINT('Ctrl Pts',(10.6212233869999,15.2,-0.190657326000014));
#190053=CARTESIAN_POINT('Ctrl Pts',(10.6212233869999,11.6,-0.190657326000015));
#190054=CARTESIAN_POINT('Ctrl Pts',(10.6191196519999,15.2,-0.190119697000015));
#190055=CARTESIAN_POINT('Ctrl Pts',(10.6191196519999,11.6,-0.190119697000016));
#190056=CARTESIAN_POINT('Ctrl Pts',(10.6170219649999,15.2,-0.189585598000015));
#190057=CARTESIAN_POINT('Ctrl Pts',(10.6170219649999,11.6,-0.189585598000015));
#190058=CARTESIAN_POINT('Ctrl Pts',(10.6149303439999,15.2,-0.189055023000013));
#190059=CARTESIAN_POINT('Ctrl Pts',(10.6149303439999,11.6,-0.189055023000014));
#190060=CARTESIAN_POINT('Ctrl Pts',(10.6128448019999,15.2,-0.188527965000014));
#190061=CARTESIAN_POINT('Ctrl Pts',(10.6128448019999,11.6,-0.188527965000014));
#190062=CARTESIAN_POINT('Ctrl Pts',(10.6107653599999,15.2,-0.188004416000016));
#190063=CARTESIAN_POINT('Ctrl Pts',(10.6107653599999,11.6,-0.188004416000016));
#190064=CARTESIAN_POINT('Ctrl Pts',(10.6086920309999,15.2,-0.187484371000015));
#190065=CARTESIAN_POINT('Ctrl Pts',(10.6086920309999,11.6,-0.187484371000016));
#190066=CARTESIAN_POINT('Ctrl Pts',(10.6066248309999,15.2,-0.186967820000015));
#190067=CARTESIAN_POINT('Ctrl Pts',(10.6066248309999,11.6,-0.186967820000015));
#190068=CARTESIAN_POINT('Ctrl Pts',(10.6045637799999,15.2,-0.186454758000014));
#190069=CARTESIAN_POINT('Ctrl Pts',(10.6045637799999,11.6,-0.186454758000015));
#190070=CARTESIAN_POINT('Ctrl Pts',(10.6025088909999,15.2,-0.185945177000013));
#190071=CARTESIAN_POINT('Ctrl Pts',(10.6025088909999,11.6,-0.185945177000014));
#190072=CARTESIAN_POINT('Ctrl Pts',(10.6004601839999,15.2,-0.185439072000015));
#190073=CARTESIAN_POINT('Ctrl Pts',(10.6004601839999,11.6,-0.185439072000016));
#190074=CARTESIAN_POINT('Ctrl Pts',(10.5984176719999,15.2,-0.184936432000011));
#190075=CARTESIAN_POINT('Ctrl Pts',(10.5984176719999,11.6,-0.184936432000012));
#190076=CARTESIAN_POINT('Ctrl Pts',(10.5963813739999,15.2,-0.184437252000014));
#190077=CARTESIAN_POINT('Ctrl Pts',(10.5963813739999,11.6,-0.184437252000014));
#190078=CARTESIAN_POINT('Ctrl Pts',(10.5943513069999,15.2,-0.183941526000013));
#190079=CARTESIAN_POINT('Ctrl Pts',(10.5943513069999,11.6,-0.183941526000014));
#190080=CARTESIAN_POINT('Ctrl Pts',(10.5923274859999,15.2,-0.183449245000014));
#190081=CARTESIAN_POINT('Ctrl Pts',(10.5923274859999,11.6,-0.183449245000014));
#190082=CARTESIAN_POINT('Ctrl Pts',(10.5903099289999,15.2,-0.182960401000014));
#190083=CARTESIAN_POINT('Ctrl Pts',(10.5903099289999,11.6,-0.182960401000015));
#190084=CARTESIAN_POINT('Ctrl Pts',(10.5882986539999,15.2,-0.182474988000014));
#190085=CARTESIAN_POINT('Ctrl Pts',(10.5882986539999,11.6,-0.182474988000015));
#190086=CARTESIAN_POINT('Ctrl Pts',(10.5862936749999,15.2,-0.181992998000013));
#190087=CARTESIAN_POINT('Ctrl Pts',(10.5862936749999,11.6,-0.181992998000014));
#190088=CARTESIAN_POINT('Ctrl Pts',(10.5842950119999,15.2,-0.181514425000016));
#190089=CARTESIAN_POINT('Ctrl Pts',(10.5842950119999,11.6,-0.181514425000016));
#190090=CARTESIAN_POINT('Ctrl Pts',(10.5823026799999,15.2,-0.181039259000015));
#190091=CARTESIAN_POINT('Ctrl Pts',(10.5823026799999,11.6,-0.181039259000016));
#190092=CARTESIAN_POINT('Ctrl Pts',(10.5803166979999,15.2,-0.180567496000013));
#190093=CARTESIAN_POINT('Ctrl Pts',(10.5803166979999,11.6,-0.180567496000013));
#190094=CARTESIAN_POINT('Ctrl Pts',(10.5783370809999,15.2,-0.180099124000015));
#190095=CARTESIAN_POINT('Ctrl Pts',(10.5783370809999,11.6,-0.180099124000015));
#190096=CARTESIAN_POINT('Ctrl Pts',(10.5763638469999,15.2,-0.179634139000013));
#190097=CARTESIAN_POINT('Ctrl Pts',(10.5763638469999,11.6,-0.179634139000014));
#190098=CARTESIAN_POINT('Ctrl Pts',(10.5743970139999,15.2,-0.179172532000016));
#190099=CARTESIAN_POINT('Ctrl Pts',(10.5743970139999,11.6,-0.179172532000016));
#190100=CARTESIAN_POINT('Ctrl Pts',(10.5724365989999,15.2,-0.178714295000013));
#190101=CARTESIAN_POINT('Ctrl Pts',(10.5724365989999,11.6,-0.178714295000014));
#190102=CARTESIAN_POINT('Ctrl Pts',(10.5704826189999,15.2,-0.178259423000018));
#190103=CARTESIAN_POINT('Ctrl Pts',(10.5704826189999,11.6,-0.178259423000018));
#190104=CARTESIAN_POINT('Ctrl Pts',(10.5685350909999,15.2,-0.177807905000016));
#190105=CARTESIAN_POINT('Ctrl Pts',(10.5685350909999,11.6,-0.177807905000016));
#190106=CARTESIAN_POINT('Ctrl Pts',(10.5665940339999,15.2,-0.177359733000015));
#190107=CARTESIAN_POINT('Ctrl Pts',(10.5665940339999,11.6,-0.177359733000016));
#190108=CARTESIAN_POINT('Ctrl Pts',(10.5646594639999,15.2,-0.176914903000016));
#190109=CARTESIAN_POINT('Ctrl Pts',(10.5646594639999,11.6,-0.176914903000017));
#190110=CARTESIAN_POINT('Ctrl Pts',(10.5627313999999,15.2,-0.176473403000017));
#190111=CARTESIAN_POINT('Ctrl Pts',(10.5627313999999,11.6,-0.176473403000017));
#190112=CARTESIAN_POINT('Ctrl Pts',(10.5608098579999,15.2,-0.176035228000018));
#190113=CARTESIAN_POINT('Ctrl Pts',(10.5608098579999,11.6,-0.176035228000018));
#190114=CARTESIAN_POINT('Ctrl Pts',(10.5588948559999,15.2,-0.175600368000013));
#190115=CARTESIAN_POINT('Ctrl Pts',(10.5588948559999,11.6,-0.175600368000013));
#190116=CARTESIAN_POINT('Ctrl Pts',(10.5569864129999,15.2,-0.175168818000015));
#190117=CARTESIAN_POINT('Ctrl Pts',(10.5569864129999,11.6,-0.175168818000016));
#190118=CARTESIAN_POINT('Ctrl Pts',(10.5550845449999,15.2,-0.174740567000011));
#190119=CARTESIAN_POINT('Ctrl Pts',(10.5550845449999,11.6,-0.174740567000012));
#190120=CARTESIAN_POINT('Ctrl Pts',(10.5531892719999,15.2,-0.174315609000013));
#190121=CARTESIAN_POINT('Ctrl Pts',(10.5531892719999,11.6,-0.174315609000014));
#190122=CARTESIAN_POINT('Ctrl Pts',(10.5513006109999,15.2,-0.173893935000016));
#190123=CARTESIAN_POINT('Ctrl Pts',(10.5513006109999,11.6,-0.173893935000016));
#190124=CARTESIAN_POINT('Ctrl Pts',(10.5494185789999,15.2,-0.173475536000014));
#190125=CARTESIAN_POINT('Ctrl Pts',(10.5494185789999,11.6,-0.173475536000014));
#190126=CARTESIAN_POINT('Ctrl Pts',(10.5475431949999,15.2,-0.173060406000012));
#190127=CARTESIAN_POINT('Ctrl Pts',(10.5475431949999,11.6,-0.173060406000012));
#190128=CARTESIAN_POINT('Ctrl Pts',(10.5456744759999,15.2,-0.172648535000013));
#190129=CARTESIAN_POINT('Ctrl Pts',(10.5456744759999,11.6,-0.172648535000013));
#190130=CARTESIAN_POINT('Ctrl Pts',(10.5438124429999,15.2,-0.172239916000017));
#190131=CARTESIAN_POINT('Ctrl Pts',(10.5438124429999,11.6,-0.172239916000017));
#190132=CARTESIAN_POINT('Ctrl Pts',(10.5419571109999,15.2,-0.171834540000013));
#190133=CARTESIAN_POINT('Ctrl Pts',(10.5419571109999,11.6,-0.171834540000014));
#190134=CARTESIAN_POINT('Ctrl Pts',(10.5401084989999,15.2,-0.171432400000011));
#190135=CARTESIAN_POINT('Ctrl Pts',(10.5401084989999,11.6,-0.171432400000012));
#190136=CARTESIAN_POINT('Ctrl Pts',(10.5382666269999,15.2,-0.171033486000014));
#190137=CARTESIAN_POINT('Ctrl Pts',(10.5382666269999,11.6,-0.171033486000014));
#190138=CARTESIAN_POINT('Ctrl Pts',(10.5364315109999,15.2,-0.170637790000012));
#190139=CARTESIAN_POINT('Ctrl Pts',(10.5364315109999,11.6,-0.170637790000013));
#190140=CARTESIAN_POINT('Ctrl Pts',(10.5346031709999,15.2,-0.170245304000014));
#190141=CARTESIAN_POINT('Ctrl Pts',(10.5346031709999,11.6,-0.170245304000014));
#190142=CARTESIAN_POINT('Ctrl Pts',(10.5327816249999,15.2,-0.169856021000014));
#190143=CARTESIAN_POINT('Ctrl Pts',(10.5327816249999,11.6,-0.169856021000015));
#190144=CARTESIAN_POINT('Ctrl Pts',(10.5309668919999,15.2,-0.169469929000012));
#190145=CARTESIAN_POINT('Ctrl Pts',(10.5309668919999,11.6,-0.169469929000013));
#190146=CARTESIAN_POINT('Ctrl Pts',(10.5291589899999,15.2,-0.169087023000016));
#190147=CARTESIAN_POINT('Ctrl Pts',(10.5291589899999,11.6,-0.169087023000017));
#190148=CARTESIAN_POINT('Ctrl Pts',(10.5273579379999,15.2,-0.168707293000012));
#190149=CARTESIAN_POINT('Ctrl Pts',(10.5273579379999,11.6,-0.168707293000013));
#190150=CARTESIAN_POINT('Ctrl Pts',(10.5255637549999,15.2,-0.168330729000012));
#190151=CARTESIAN_POINT('Ctrl Pts',(10.5255637549999,11.6,-0.168330729000013));
#190152=CARTESIAN_POINT('Ctrl Pts',(10.5237764589999,15.2,-0.167957324000017));
#190153=CARTESIAN_POINT('Ctrl Pts',(10.5237764589999,11.6,-0.167957324000017));
#190154=CARTESIAN_POINT('Ctrl Pts',(10.5219960679999,15.2,-0.167587069000015));
#190155=CARTESIAN_POINT('Ctrl Pts',(10.5219960679999,11.6,-0.167587069000015));
#190156=CARTESIAN_POINT('Ctrl Pts',(10.5202226039999,15.2,-0.167219956000015));
#190157=CARTESIAN_POINT('Ctrl Pts',(10.5202226039999,11.6,-0.167219956000016));
#190158=CARTESIAN_POINT('Ctrl Pts',(10.5184560839999,15.2,-0.166855975000013));
#190159=CARTESIAN_POINT('Ctrl Pts',(10.5184560839999,11.6,-0.166855975000014));
#190160=CARTESIAN_POINT('Ctrl Pts',(10.5166965259999,15.2,-0.166495117000016));
#190161=CARTESIAN_POINT('Ctrl Pts',(10.5166965259999,11.6,-0.166495117000017));
#190162=CARTESIAN_POINT('Ctrl Pts',(10.5149439519999,15.2,-0.166137374000015));
#190163=CARTESIAN_POINT('Ctrl Pts',(10.5149439519999,11.6,-0.166137374000015));
#190164=CARTESIAN_POINT('Ctrl Pts',(10.5131983789999,15.2,-0.165782737000013));
#190165=CARTESIAN_POINT('Ctrl Pts',(10.5131983789999,11.6,-0.165782737000014));
#190166=CARTESIAN_POINT('Ctrl Pts',(10.5114598269999,15.2,-0.165431197000014));
#190167=CARTESIAN_POINT('Ctrl Pts',(10.5114598269999,11.6,-0.165431197000015));
#190168=CARTESIAN_POINT('Ctrl Pts',(10.5097283139999,15.2,-0.165082745000014));
#190169=CARTESIAN_POINT('Ctrl Pts',(10.5097283139999,11.6,-0.165082745000014));
#190170=CARTESIAN_POINT('Ctrl Pts',(10.5080038619999,15.2,-0.164737371000014));
#190171=CARTESIAN_POINT('Ctrl Pts',(10.5080038619999,11.6,-0.164737371000015));
#190172=CARTESIAN_POINT('Ctrl Pts',(10.5062864879999,15.2,-0.164395067000012));
#190173=CARTESIAN_POINT('Ctrl Pts',(10.5062864879999,11.6,-0.164395067000012));
#190174=CARTESIAN_POINT('Ctrl Pts',(10.5045762119999,15.2,-0.164055824000013));
#190175=CARTESIAN_POINT('Ctrl Pts',(10.5045762119999,11.6,-0.164055824000014));
#190176=CARTESIAN_POINT('Ctrl Pts',(10.5028730549999,15.2,-0.163719632000014));
#190177=CARTESIAN_POINT('Ctrl Pts',(10.5028730549999,11.6,-0.163719632000015));
#190178=CARTESIAN_POINT('Ctrl Pts',(10.5011770349999,15.2,-0.163386483000014));
#190179=CARTESIAN_POINT('Ctrl Pts',(10.5011770349999,11.6,-0.163386483000015));
#190180=CARTESIAN_POINT('Ctrl Pts',(10.4994881719999,15.2,-0.163056366000016));
#190181=CARTESIAN_POINT('Ctrl Pts',(10.4994881719999,11.6,-0.163056366000017));
#190182=CARTESIAN_POINT('Ctrl Pts',(10.4978064869999,15.2,-0.162729273000015));
#190183=CARTESIAN_POINT('Ctrl Pts',(10.4978064869999,11.6,-0.162729273000016));
#190184=CARTESIAN_POINT('Ctrl Pts',(10.4961319979999,15.2,-0.162405194000015));
#190185=CARTESIAN_POINT('Ctrl Pts',(10.4961319979999,11.6,-0.162405194000015));
#190186=CARTESIAN_POINT('Ctrl Pts',(10.4944647269999,15.2,-0.162084120000014));
#190187=CARTESIAN_POINT('Ctrl Pts',(10.4944647269999,11.6,-0.162084120000015));
#190188=CARTESIAN_POINT('Ctrl Pts',(10.4928046919999,15.2,-0.161766042000018));
#190189=CARTESIAN_POINT('Ctrl Pts',(10.4928046919999,11.6,-0.161766042000018));
#190190=CARTESIAN_POINT('Ctrl Pts',(10.4911519139999,15.2,-0.161450949000015));
#190191=CARTESIAN_POINT('Ctrl Pts',(10.4911519139999,11.6,-0.161450949000015));
#190192=CARTESIAN_POINT('Ctrl Pts',(10.4895064129999,15.2,-0.161138832000014));
#190193=CARTESIAN_POINT('Ctrl Pts',(10.4895064129999,11.6,-0.161138832000014));
#190194=CARTESIAN_POINT('Ctrl Pts',(10.4878682099999,15.2,-0.160829682000014));
#190195=CARTESIAN_POINT('Ctrl Pts',(10.4878682099999,11.6,-0.160829682000015));
#190196=CARTESIAN_POINT('Ctrl Pts',(10.4862373239999,15.2,-0.160523489000015));
#190197=CARTESIAN_POINT('Ctrl Pts',(10.4862373239999,11.6,-0.160523489000016));
#190198=CARTESIAN_POINT('Ctrl Pts',(10.4846137759999,15.2,-0.160220244000016));
#190199=CARTESIAN_POINT('Ctrl Pts',(10.4846137759999,11.6,-0.160220244000016));
#190200=CARTESIAN_POINT('Ctrl Pts',(10.4829975859999,15.2,-0.159919936000015));
#190201=CARTESIAN_POINT('Ctrl Pts',(10.4829975859999,11.6,-0.159919936000015));
#190202=CARTESIAN_POINT('Ctrl Pts',(10.4813887749999,15.2,-0.159622556000016));
#190203=CARTESIAN_POINT('Ctrl Pts',(10.4813887749999,11.6,-0.159622556000017));
#190204=CARTESIAN_POINT('Ctrl Pts',(10.4797873629999,15.2,-0.159328093000015));
#190205=CARTESIAN_POINT('Ctrl Pts',(10.4797873629999,11.6,-0.159328093000016));
#190206=CARTESIAN_POINT('Ctrl Pts',(10.4781933699999,15.2,-0.159036540000015));
#190207=CARTESIAN_POINT('Ctrl Pts',(10.4781933699999,11.6,-0.159036540000015));
#190208=CARTESIAN_POINT('Ctrl Pts',(10.4766068189999,15.2,-0.158747884000014));
#190209=CARTESIAN_POINT('Ctrl Pts',(10.4766068189999,11.6,-0.158747884000015));
#190210=CARTESIAN_POINT('Ctrl Pts',(10.4750277289999,15.2,-0.158462116000013));
#190211=CARTESIAN_POINT('Ctrl Pts',(10.4750277289999,11.6,-0.158462116000014));
#190212=CARTESIAN_POINT('Ctrl Pts',(10.4734561209999,15.2,-0.158179227000015));
#190213=CARTESIAN_POINT('Ctrl Pts',(10.4734561209999,11.6,-0.158179227000015));
#190214=CARTESIAN_POINT('Ctrl Pts',(10.4718920149999,15.2,-0.157899205000014));
#190215=CARTESIAN_POINT('Ctrl Pts',(10.4718920149999,11.6,-0.157899205000014));
#190216=CARTESIAN_POINT('Ctrl Pts',(10.4703354349999,15.2,-0.157622040000014));
#190217=CARTESIAN_POINT('Ctrl Pts',(10.4703354349999,11.6,-0.157622040000014));
#190218=CARTESIAN_POINT('Ctrl Pts',(10.4687863999999,15.2,-0.157347725000014));
#190219=CARTESIAN_POINT('Ctrl Pts',(10.4687863999999,11.6,-0.157347725000015));
#190220=CARTESIAN_POINT('Ctrl Pts',(10.4672449309999,15.2,-0.157076245000014));
#190221=CARTESIAN_POINT('Ctrl Pts',(10.4672449309999,11.6,-0.157076245000014));
#190222=CARTESIAN_POINT('Ctrl Pts',(10.4657110499999,15.2,-0.156807593000017));
#190223=CARTESIAN_POINT('Ctrl Pts',(10.4657110499999,11.6,-0.156807593000017));
#190224=CARTESIAN_POINT('Ctrl Pts',(10.4641847769999,15.2,-0.156541758000017));
#190225=CARTESIAN_POINT('Ctrl Pts',(10.4641847769999,11.6,-0.156541758000018));
#190226=CARTESIAN_POINT('Ctrl Pts',(10.4626661349999,15.2,-0.156278729000014));
#190227=CARTESIAN_POINT('Ctrl Pts',(10.4626661349999,11.6,-0.156278729000015));
#190228=CARTESIAN_POINT('Ctrl Pts',(10.4611551459999,15.2,-0.156018496000012));
#190229=CARTESIAN_POINT('Ctrl Pts',(10.4611551459999,11.6,-0.156018496000013));
#190230=CARTESIAN_POINT('Ctrl Pts',(10.4596518279999,15.2,-0.155761048000014));
#190231=CARTESIAN_POINT('Ctrl Pts',(10.4596518279999,11.6,-0.155761048000014));
#190232=CARTESIAN_POINT('Ctrl Pts',(10.4581562069999,15.2,-0.155506375000014));
#190233=CARTESIAN_POINT('Ctrl Pts',(10.4581562069999,11.6,-0.155506375000015));
#190234=CARTESIAN_POINT('Ctrl Pts',(10.4566683019999,15.2,-0.155254466000017));
#190235=CARTESIAN_POINT('Ctrl Pts',(10.4566683019999,11.6,-0.155254466000017));
#190236=CARTESIAN_POINT('Ctrl Pts',(10.4551881359999,15.2,-0.155005310000016));
#190237=CARTESIAN_POINT('Ctrl Pts',(10.4551881359999,11.6,-0.155005310000016));
#190238=CARTESIAN_POINT('Ctrl Pts',(10.4537157299999,15.2,-0.154758897000011));
#190239=CARTESIAN_POINT('Ctrl Pts',(10.4537157299999,11.6,-0.154758897000012));
#190240=CARTESIAN_POINT('Ctrl Pts',(10.4522511059999,15.2,-0.154515216000015));
#190241=CARTESIAN_POINT('Ctrl Pts',(10.4522511059999,11.6,-0.154515216000016));
#190242=CARTESIAN_POINT('Ctrl Pts',(10.4507942869999,15.2,-0.154274256000013));
#190243=CARTESIAN_POINT('Ctrl Pts',(10.4507942869999,11.6,-0.154274256000014));
#190244=CARTESIAN_POINT('Ctrl Pts',(10.4493452949999,15.2,-0.154036006000013));
#190245=CARTESIAN_POINT('Ctrl Pts',(10.4493452949999,11.6,-0.154036006000014));
#190246=CARTESIAN_POINT('Ctrl Pts',(10.4479041509999,15.2,-0.153800456000015));
#190247=CARTESIAN_POINT('Ctrl Pts',(10.4479041509999,11.6,-0.153800456000015));
#190248=CARTESIAN_POINT('Ctrl Pts',(10.4464708799999,15.2,-0.153567592000012));
#190249=CARTESIAN_POINT('Ctrl Pts',(10.4464708799999,11.6,-0.153567592000013));
#190250=CARTESIAN_POINT('Ctrl Pts',(10.4450455009999,15.2,-0.153337407000014));
#190251=CARTESIAN_POINT('Ctrl Pts',(10.4450455009999,11.6,-0.153337407000014));
#190252=CARTESIAN_POINT('Ctrl Pts',(10.4436280379999,15.2,-0.153109887000014));
#190253=CARTESIAN_POINT('Ctrl Pts',(10.4436280379999,11.6,-0.153109887000014));
#190254=CARTESIAN_POINT('Ctrl Pts',(10.4422185139999,15.2,-0.152885022000016));
#190255=CARTESIAN_POINT('Ctrl Pts',(10.4422185139999,11.6,-0.152885022000016));
#190256=CARTESIAN_POINT('Ctrl Pts',(10.4408169509999,15.2,-0.152662801000014));
#190257=CARTESIAN_POINT('Ctrl Pts',(10.4408169509999,11.6,-0.152662801000015));
#190258=CARTESIAN_POINT('Ctrl Pts',(10.4394233719999,15.2,-0.152443211000013));
#190259=CARTESIAN_POINT('Ctrl Pts',(10.4394233719999,11.6,-0.152443211000013));
#190260=CARTESIAN_POINT('Ctrl Pts',(10.4380377999999,15.2,-0.152226243000015));
#190261=CARTESIAN_POINT('Ctrl Pts',(10.4380377999999,11.6,-0.152226243000016));
#190262=CARTESIAN_POINT('Ctrl Pts',(10.4366602579999,15.2,-0.152011884000016));
#190263=CARTESIAN_POINT('Ctrl Pts',(10.4366602579999,11.6,-0.152011884000017));
#190264=CARTESIAN_POINT('Ctrl Pts',(10.4352907679999,15.2,-0.151800122000014));
#190265=CARTESIAN_POINT('Ctrl Pts',(10.4352907679999,11.6,-0.151800122000015));
#190266=CARTESIAN_POINT('Ctrl Pts',(10.4339293549999,15.2,-0.151590947000013));
#190267=CARTESIAN_POINT('Ctrl Pts',(10.4339293549999,11.6,-0.151590947000014));
#190268=CARTESIAN_POINT('Ctrl Pts',(10.4325760399999,15.2,-0.151384346000012));
#190269=CARTESIAN_POINT('Ctrl Pts',(10.4325760399999,11.6,-0.151384346000012));
#190270=CARTESIAN_POINT('Ctrl Pts',(10.4312308479999,15.2,-0.151180309000014));
#190271=CARTESIAN_POINT('Ctrl Pts',(10.4312308479999,11.6,-0.151180309000015));
#190272=CARTESIAN_POINT('Ctrl Pts',(10.4298938009999,15.2,-0.150978823000014));
#190273=CARTESIAN_POINT('Ctrl Pts',(10.4298938009999,11.6,-0.150978823000015));
#190274=CARTESIAN_POINT('Ctrl Pts',(10.4285649239999,15.2,-0.150779877000016));
#190275=CARTESIAN_POINT('Ctrl Pts',(10.4285649239999,11.6,-0.150779877000016));
#190276=CARTESIAN_POINT('Ctrl Pts',(10.4272442399999,15.2,-0.150583457000018));
#190277=CARTESIAN_POINT('Ctrl Pts',(10.4272442399999,11.6,-0.150583457000018));
#190278=CARTESIAN_POINT('Ctrl Pts',(10.4259317729999,15.2,-0.150389553000014));
#190279=CARTESIAN_POINT('Ctrl Pts',(10.4259317729999,11.6,-0.150389553000015));
#190280=CARTESIAN_POINT('Ctrl Pts',(10.4246275449999,15.2,-0.150198153000014));
#190281=CARTESIAN_POINT('Ctrl Pts',(10.4246275449999,11.6,-0.150198153000014));
#190282=CARTESIAN_POINT('Ctrl Pts',(10.4233315819999,15.2,-0.150009245000016));
#190283=CARTESIAN_POINT('Ctrl Pts',(10.4233315819999,11.6,-0.150009245000016));
#190284=CARTESIAN_POINT('Ctrl Pts',(10.4220439069999,15.2,-0.149822817000014));
#190285=CARTESIAN_POINT('Ctrl Pts',(10.4220439069999,11.6,-0.149822817000014));
#190286=CARTESIAN_POINT('Ctrl Pts',(10.4207645439999,15.2,-0.149638856000016));
#190287=CARTESIAN_POINT('Ctrl Pts',(10.4207645439999,11.6,-0.149638856000017));
#190288=CARTESIAN_POINT('Ctrl Pts',(10.4194935179999,15.2,-0.149457349000013));
#190289=CARTESIAN_POINT('Ctrl Pts',(10.4194935179999,11.6,-0.149457349000013));
#190290=CARTESIAN_POINT('Ctrl Pts',(10.4182308519999,15.2,-0.149278285000012));
#190291=CARTESIAN_POINT('Ctrl Pts',(10.4182308519999,11.6,-0.149278285000012));
#190292=CARTESIAN_POINT('Ctrl Pts',(10.4169765709999,15.2,-0.149101653000017));
#190293=CARTESIAN_POINT('Ctrl Pts',(10.4169765709999,11.6,-0.149101653000017));
#190294=CARTESIAN_POINT('Ctrl Pts',(10.4157306989999,15.2,-0.148927436000013));
#190295=CARTESIAN_POINT('Ctrl Pts',(10.4157306989999,11.6,-0.148927436000013));
#190296=CARTESIAN_POINT('Ctrl Pts',(10.4144932619999,15.2,-0.148755626000017));
#190297=CARTESIAN_POINT('Ctrl Pts',(10.4144932619999,11.6,-0.148755626000017));
#190298=CARTESIAN_POINT('Ctrl Pts',(10.4132642839999,15.2,-0.148586210000015));
#190299=CARTESIAN_POINT('Ctrl Pts',(10.4132642839999,11.6,-0.148586210000015));
#190300=CARTESIAN_POINT('Ctrl Pts',(10.4120437889999,15.2,-0.148419172000014));
#190301=CARTESIAN_POINT('Ctrl Pts',(10.4120437889999,11.6,-0.148419172000014));
#190302=CARTESIAN_POINT('Ctrl Pts',(10.4108318009999,15.2,-0.148254502000014));
#190303=CARTESIAN_POINT('Ctrl Pts',(10.4108318009999,11.6,-0.148254502000014));
#190304=CARTESIAN_POINT('Ctrl Pts',(10.4096283479999,15.2,-0.148092188000017));
#190305=CARTESIAN_POINT('Ctrl Pts',(10.4096283479999,11.6,-0.148092188000018));
#190306=CARTESIAN_POINT('Ctrl Pts',(10.4084334529999,15.2,-0.147932214000015));
#190307=CARTESIAN_POINT('Ctrl Pts',(10.4084334529999,11.6,-0.147932214000015));
#190308=CARTESIAN_POINT('Ctrl Pts',(10.4072471419999,15.2,-0.147774569000014));
#190309=CARTESIAN_POINT('Ctrl Pts',(10.4072471419999,11.6,-0.147774569000015));
#190310=CARTESIAN_POINT('Ctrl Pts',(10.4060694389999,15.2,-0.147619240000014));
#190311=CARTESIAN_POINT('Ctrl Pts',(10.4060694389999,11.6,-0.147619240000015));
#190312=CARTESIAN_POINT('Ctrl Pts',(10.4049003719999,15.2,-0.147466214000014));
#190313=CARTESIAN_POINT('Ctrl Pts',(10.4049003719999,11.6,-0.147466214000014));
#190314=CARTESIAN_POINT('Ctrl Pts',(10.4037399639999,15.2,-0.147315477000016));
#190315=CARTESIAN_POINT('Ctrl Pts',(10.4037399639999,11.6,-0.147315477000017));
#190316=CARTESIAN_POINT('Ctrl Pts',(10.4025882419999,15.2,-0.147167016000012));
#190317=CARTESIAN_POINT('Ctrl Pts',(10.4025882419999,11.6,-0.147167016000012));
#190318=CARTESIAN_POINT('Ctrl Pts',(10.4014452309999,15.2,-0.147020819000012));
#190319=CARTESIAN_POINT('Ctrl Pts',(10.4014452309999,11.6,-0.147020819000013));
#190320=CARTESIAN_POINT('Ctrl Pts',(10.4003109569999,15.2,-0.146876871000017));
#190321=CARTESIAN_POINT('Ctrl Pts',(10.4003109569999,11.6,-0.146876871000017));
#190322=CARTESIAN_POINT('Ctrl Pts',(10.3991854459999,15.2,-0.146735160000016));
#190323=CARTESIAN_POINT('Ctrl Pts',(10.3991854459999,11.6,-0.146735160000016));
#190324=CARTESIAN_POINT('Ctrl Pts',(10.3980687249999,15.2,-0.146595671000016));
#190325=CARTESIAN_POINT('Ctrl Pts',(10.3980687249999,11.6,-0.146595671000016));
#190326=CARTESIAN_POINT('Ctrl Pts',(10.3969608199999,15.2,-0.146458391000017));
#190327=CARTESIAN_POINT('Ctrl Pts',(10.3969608199999,11.6,-0.146458391000018));
#190328=CARTESIAN_POINT('Ctrl Pts',(10.3958617559999,15.2,-0.146323307000014));
#190329=CARTESIAN_POINT('Ctrl Pts',(10.3958617559999,11.6,-0.146323307000014));
#190330=CARTESIAN_POINT('Ctrl Pts',(10.3947715609999,15.2,-0.146190403000013));
#190331=CARTESIAN_POINT('Ctrl Pts',(10.3947715609999,11.6,-0.146190403000013));
#190332=CARTESIAN_POINT('Ctrl Pts',(10.3936902589999,15.2,-0.146059668000014));
#190333=CARTESIAN_POINT('Ctrl Pts',(10.3936902589999,11.6,-0.146059668000014));
#190334=CARTESIAN_POINT('Ctrl Pts',(10.3926178809999,15.2,-0.145931087000015));
#190335=CARTESIAN_POINT('Ctrl Pts',(10.3926178809999,11.6,-0.145931087000016));
#190336=CARTESIAN_POINT('Ctrl Pts',(10.3915544509999,15.2,-0.145804646000016));
#190337=CARTESIAN_POINT('Ctrl Pts',(10.3915544509999,11.6,-0.145804646000017));
#190338=CARTESIAN_POINT('Ctrl Pts',(10.3904999949999,15.2,-0.145680330000015));
#190339=CARTESIAN_POINT('Ctrl Pts',(10.3904999949999,11.6,-0.145680330000016));
#190340=CARTESIAN_POINT('Ctrl Pts',(10.3894545419999,15.2,-0.145558126000012));
#190341=CARTESIAN_POINT('Ctrl Pts',(10.3894545419999,11.6,-0.145558126000012));
#190342=CARTESIAN_POINT('Ctrl Pts',(10.3884181189999,15.2,-0.145438019000017));
#190343=CARTESIAN_POINT('Ctrl Pts',(10.3884181189999,11.6,-0.145438019000018));
#190344=CARTESIAN_POINT('Ctrl Pts',(10.3873907519999,15.2,-0.145319997000013));
#190345=CARTESIAN_POINT('Ctrl Pts',(10.3873907519999,11.6,-0.145319997000013));
#190346=CARTESIAN_POINT('Ctrl Pts',(10.3863724699999,15.2,-0.145204042000016));
#190347=CARTESIAN_POINT('Ctrl Pts',(10.3863724699999,11.6,-0.145204042000016));
#190348=CARTESIAN_POINT('Ctrl Pts',(10.3853632999999,15.2,-0.145090141000015));
#190349=CARTESIAN_POINT('Ctrl Pts',(10.3853632999999,11.6,-0.145090141000015));
#190350=CARTESIAN_POINT('Ctrl Pts',(10.3843632689999,15.2,-0.144978281000014));
#190351=CARTESIAN_POINT('Ctrl Pts',(10.3843632689999,11.6,-0.144978281000015));
#190352=CARTESIAN_POINT('Ctrl Pts',(10.3833724059999,15.2,-0.144868445000017));
#190353=CARTESIAN_POINT('Ctrl Pts',(10.3833724059999,11.6,-0.144868445000017));
#190354=CARTESIAN_POINT('Ctrl Pts',(10.3823907369999,15.2,-0.144760620000017));
#190355=CARTESIAN_POINT('Ctrl Pts',(10.3823907369999,11.6,-0.144760620000018));
#190356=CARTESIAN_POINT('Ctrl Pts',(10.3814182929999,15.2,-0.144654790000014));
#190357=CARTESIAN_POINT('Ctrl Pts',(10.3814182929999,11.6,-0.144654790000014));
#190358=CARTESIAN_POINT('Ctrl Pts',(10.3804550999999,15.2,-0.144550941000015));
#190359=CARTESIAN_POINT('Ctrl Pts',(10.3804550999999,11.6,-0.144550941000015));
#190360=CARTESIAN_POINT('Ctrl Pts',(10.3795011859999,15.2,-0.144449057000013));
#190361=CARTESIAN_POINT('Ctrl Pts',(10.3795011859999,11.6,-0.144449057000014));
#190362=CARTESIAN_POINT('Ctrl Pts',(10.3785565819999,15.2,-0.144349124000014));
#190363=CARTESIAN_POINT('Ctrl Pts',(10.3785565819999,11.6,-0.144349124000014));
#190364=CARTESIAN_POINT('Ctrl Pts',(10.3776213129999,15.2,-0.144251127000015));
#190365=CARTESIAN_POINT('Ctrl Pts',(10.3776213129999,11.6,-0.144251127000015));
#190366=CARTESIAN_POINT('Ctrl Pts',(10.3766954109999,15.2,-0.144155050000014));
#190367=CARTESIAN_POINT('Ctrl Pts',(10.3766954109999,11.6,-0.144155050000015));
#190368=CARTESIAN_POINT('Ctrl Pts',(10.3757841819999,15.2,-0.144061420000017));
#190369=CARTESIAN_POINT('Ctrl Pts',(10.3757841819999,11.6,-0.144061420000017));
#190370=CARTESIAN_POINT('Ctrl Pts',(10.3750636849999,15.2,-0.143988114000013));
#190371=CARTESIAN_POINT('Ctrl Pts',(10.3750636849999,11.6,-0.143988114000014));
#190372=CARTESIAN_POINT('Ctrl Pts',(10.3745287909999,15.2,-0.143934095000016));
#190373=CARTESIAN_POINT('Ctrl Pts',(10.3745287909999,11.6,-0.143934095000016));
#190374=CARTESIAN_POINT('Ctrl Pts',(10.3741757629999,15.2,-0.143898619000016));
#190375=CARTESIAN_POINT('Ctrl Pts',(10.3741757629999,11.6,-0.143898619000016));
#190376=CARTESIAN_POINT('Ctrl Pts',(10.3740022749999,15.2,-0.143881227000016));
#190377=CARTESIAN_POINT('Ctrl Pts',(10.3740022749999,11.6,-0.143881227000016));
#190378=CARTESIAN_POINT('',(10.3740022745143,12.2,-0.143881227669191));
#190379=CARTESIAN_POINT('',(10.3740022745143,15.2,-0.143881227669191));
#190380=CARTESIAN_POINT('',(10.3740022739999,12.2,-0.143881228000016));
#190381=CARTESIAN_POINT('Ctrl Pts',(11.4869855309999,12.2,-0.546958306000014));
#190382=CARTESIAN_POINT('Ctrl Pts',(11.4836329088539,12.2,-0.545121269824113));
#190383=CARTESIAN_POINT('Ctrl Pts',(11.4802840213634,12.2,-0.543291206986518));
#190384=CARTESIAN_POINT('Ctrl Pts',(11.4769388591068,12.2,-0.541468106410471));
#190385=CARTESIAN_POINT('Ctrl Pts',(11.4735936968502,12.2,-0.539645005834425));
#190386=CARTESIAN_POINT('Ctrl Pts',(11.4702522623749,12.2,-0.537828869725522));
#190387=CARTESIAN_POINT('Ctrl Pts',(11.4669145744124,12.2,-0.536019697075066));
#190388=CARTESIAN_POINT('Ctrl Pts',(11.4635768864498,12.2,-0.53421052442461));
#190389=CARTESIAN_POINT('Ctrl Pts',(11.4602429461721,12.2,-0.532408315160394));
#190390=CARTESIAN_POINT('Ctrl Pts',(11.4569127942509,12.2,-0.530613060641336));
#190391=CARTESIAN_POINT('Ctrl Pts',(11.4535826417247,12.2,-0.528817805796139));
#190392=CARTESIAN_POINT('Ctrl Pts',(11.4502562798913,12.2,-0.52702950746958));
#190393=CARTESIAN_POINT('Ctrl Pts',(11.4469337572423,12.2,-0.525248154128303));
#190394=CARTESIAN_POINT('Ctrl Pts',(11.4436112351968,12.2,-0.523466801110638));
#190395=CARTESIAN_POINT('Ctrl Pts',(11.4402925523679,12.2,-0.521692394659278));
#190396=CARTESIAN_POINT('Ctrl Pts',(11.4369777481137,12.2,-0.519924928099098));
#190397=CARTESIAN_POINT('Ctrl Pts',(11.4336629438594,12.2,-0.518157461538918));
#190398=CARTESIAN_POINT('Ctrl Pts',(11.4303520166751,12.2,-0.516396934242597));
#190399=CARTESIAN_POINT('Ctrl Pts',(11.4270450034886,12.2,-0.514643339715042));
#190400=CARTESIAN_POINT('Ctrl Pts',(11.4237379903021,12.2,-0.512889745187486));
#190401=CARTESIAN_POINT('Ctrl Pts',(11.4204348911314,12.2,-0.511143084062936));
#190402=CARTESIAN_POINT('Ctrl Pts',(11.4171357470279,12.2,-0.509403348034881));
#190403=CARTESIAN_POINT('Ctrl Pts',(11.4138366029244,12.2,-0.507663612006827));
#190404=CARTESIAN_POINT('Ctrl Pts',(11.4105414141562,12.2,-0.505930801676099));
#190405=CARTESIAN_POINT('Ctrl Pts',(11.4072502226087,12.2,-0.504204908613204));
#190406=CARTESIAN_POINT('Ctrl Pts',(11.4039590310613,12.2,-0.502479015550309));
#190407=CARTESIAN_POINT('Ctrl Pts',(11.4006718374802,12.2,-0.500760040078605));
#190408=CARTESIAN_POINT('Ctrl Pts',(11.3973886809323,12.2,-0.499047974889869));
#190409=CARTESIAN_POINT('Ctrl Pts',(11.394105523788,12.2,-0.497335909390109));
#190410=CARTESIAN_POINT('Ctrl Pts',(11.390826404928,12.2,-0.495630752808958));
#190411=CARTESIAN_POINT('Ctrl Pts',(11.3875513632443,12.2,-0.493932498896419));
#190412=CARTESIAN_POINT('Ctrl Pts',(11.3842763221555,12.2,-0.492234245292397));
#190413=CARTESIAN_POINT('Ctrl Pts',(11.3810053589286,12.2,-0.490542893312953));
#190414=CARTESIAN_POINT('Ctrl Pts',(11.3777385150929,12.2,-0.488858436124135));
#190415=CARTESIAN_POINT('Ctrl Pts',(11.3744716712572,12.2,-0.487173978935316));
#190416=CARTESIAN_POINT('Ctrl Pts',(11.3712089465594,12.2,-0.485496416156678));
#190417=CARTESIAN_POINT('Ctrl Pts',(11.3679503829281,12.2,-0.483825738551309));
#190418=CARTESIAN_POINT('Ctrl Pts',(11.3646918192969,12.2,-0.482155060945941));
#190419=CARTESIAN_POINT('Ctrl Pts',(11.3614374165318,12.2,-0.480491269423095));
#190420=CARTESIAN_POINT('Ctrl Pts',(11.3581872154832,12.2,-0.478834355816627));
#190421=CARTESIAN_POINT('Ctrl Pts',(11.3549370144347,12.2,-0.477177442210161));
#190422=CARTESIAN_POINT('Ctrl Pts',(11.3516910159193,12.2,-0.475527406186752));
#190423=CARTESIAN_POINT('Ctrl Pts',(11.3484492608283,12.2,-0.47388423916252));
#190424=CARTESIAN_POINT('Ctrl Pts',(11.3452075057374,12.2,-0.472241072138288));
#190425=CARTESIAN_POINT('Ctrl Pts',(11.3419699946701,12.2,-0.470604774954951));
#190426=CARTESIAN_POINT('Ctrl Pts',(11.3387367688755,12.2,-0.468975337806958));
#190427=CARTESIAN_POINT('Ctrl Pts',(11.335503543081,12.2,-0.467345900658965));
#190428=CARTESIAN_POINT('Ctrl Pts',(11.3322746022863,12.2,-0.465723324144431));
#190429=CARTESIAN_POINT('Ctrl Pts',(11.3290499901946,12.2,-0.464107599577203));
#190430=CARTESIAN_POINT('Ctrl Pts',(11.325825377517,12.2,-0.46249187471645));
#190431=CARTESIAN_POINT('Ctrl Pts',(11.3226050936823,12.2,-0.460883002232627));
#190432=CARTESIAN_POINT('Ctrl Pts',(11.3193891785489,12.2,-0.459280972375732));
#190433=CARTESIAN_POINT('Ctrl Pts',(11.3161732639996,12.2,-0.457678942809872));
#190434=CARTESIAN_POINT('Ctrl Pts',(11.3129617193168,12.2,-0.45608375716865));
#190435=CARTESIAN_POINT('Ctrl Pts',(11.3097545881421,12.2,-0.454495404601949));
#190436=CARTESIAN_POINT('Ctrl Pts',(11.3065474569673,12.2,-0.452907052035249));
#190437=CARTESIAN_POINT('Ctrl Pts',(11.3033447376004,12.2,-0.451325533326077));
#190438=CARTESIAN_POINT('Ctrl Pts',(11.3001464735082,12.2,-0.44975083971663));
#190439=CARTESIAN_POINT('Ctrl Pts',(11.2969482094161,12.2,-0.448176146107184));
#190440=CARTESIAN_POINT('Ctrl Pts',(11.2937544009988,12.2,-0.44660827731411));
#190441=CARTESIAN_POINT('Ctrl Pts',(11.2905650908643,12.2,-0.445047224161904));
#190442=CARTESIAN_POINT('Ctrl Pts',(11.2873757807298,12.2,-0.443486171009697));
#190443=CARTESIAN_POINT('Ctrl Pts',(11.2841909683758,12.2,-0.441931933054628));
#190444=CARTESIAN_POINT('Ctrl Pts',(11.2810106971653,12.2,-0.440384501782759));
#190445=CARTESIAN_POINT('Ctrl Pts',(11.2778304259548,12.2,-0.43883707051089));
#190446=CARTESIAN_POINT('Ctrl Pts',(11.2746546961933,12.2,-0.437296444696212));
#190447=CARTESIAN_POINT('Ctrl Pts',(11.2714835511412,12.2,-0.435762615084349));
#190448=CARTESIAN_POINT('Ctrl Pts',(11.2683124055131,12.2,-0.434228785193839));
#190449=CARTESIAN_POINT('Ctrl Pts',(11.2651458446695,12.2,-0.432701751788574));
#190450=CARTESIAN_POINT('Ctrl Pts',(11.2619839115856,12.2,-0.431181504901892));
#190451=CARTESIAN_POINT('Ctrl Pts',(11.2588219790761,12.2,-0.429661258291389));
#190452=CARTESIAN_POINT('Ctrl Pts',(11.2556646758581,12.2,-0.42814779848052));
#190453=CARTESIAN_POINT('Ctrl Pts',(11.2525120433897,12.2,-0.42664111532752));
#190454=CARTESIAN_POINT('Ctrl Pts',(11.2493594109213,12.2,-0.425134432174519));
#190455=CARTESIAN_POINT('Ctrl Pts',(11.2462114513304,12.2,-0.42363452516778));
#190456=CARTESIAN_POINT('Ctrl Pts',(11.2430682067637,12.2,-0.42214138496528));
#190457=CARTESIAN_POINT('Ctrl Pts',(11.2388772141984,12.2,-0.420150531452365));
#190458=CARTESIAN_POINT('Ctrl Pts',(11.2346946050503,12.2,-0.418171707756432));
#190459=CARTESIAN_POINT('Ctrl Pts',(11.2305204852241,12.2,-0.416204887804882));
#190460=CARTESIAN_POINT('Ctrl Pts',(11.2273898946434,12.2,-0.414729772506245));
#190461=CARTESIAN_POINT('Ctrl Pts',(11.2242640798725,12.2,-0.413261410576182));
#190462=CARTESIAN_POINT('Ctrl Pts',(11.2211430833362,12.2,-0.411799790198013));
#190463=CARTESIAN_POINT('Ctrl Pts',(11.2169817555662,12.2,-0.409850963469666));
#190464=CARTESIAN_POINT('Ctrl Pts',(11.2128289954728,12.2,-0.407914122531416));
#190465=CARTESIAN_POINT('Ctrl Pts',(11.2086849095888,12.2,-0.405989243632441));
#190466=CARTESIAN_POINT('Ctrl Pts',(11.2055768450346,12.2,-0.404545584392643));
#190467=CARTESIAN_POINT('Ctrl Pts',(11.2024736597755,12.2,-0.403108652330341));
#190468=CARTESIAN_POINT('Ctrl Pts',(11.1993753985661,12.2,-0.401678437560079));
#190469=CARTESIAN_POINT('Ctrl Pts',(11.1962771373566,12.2,-0.400248222789816));
#190470=CARTESIAN_POINT('Ctrl Pts',(11.1931838001617,12.2,-0.398824724941605));
#190471=CARTESIAN_POINT('Ctrl Pts',(11.1900954321482,12.2,-0.397407932825503));
#190472=CARTESIAN_POINT('Ctrl Pts',(11.1870070635737,12.2,-0.395991140452016));
#190473=CARTESIAN_POINT('Ctrl Pts',(11.1839236651589,12.2,-0.394581054313751));
#190474=CARTESIAN_POINT('Ctrl Pts',(11.1808452810872,12.2,-0.393177662444036));
#190475=CARTESIAN_POINT('Ctrl Pts',(11.1777668975747,12.2,-0.39177427082927));
#190476=CARTESIAN_POINT('Ctrl Pts',(11.1746935291703,12.2,-0.390377574464148));
#190477=CARTESIAN_POINT('Ctrl Pts',(11.1716252211572,12.2,-0.388987560390236));
#190478=CARTESIAN_POINT('Ctrl Pts',(11.1685569131441,12.2,-0.387597546316323));
#190479=CARTESIAN_POINT('Ctrl Pts',(11.1654936657999,12.2,-0.386214216388258));
#190480=CARTESIAN_POINT('Ctrl Pts',(11.1624355252305,12.2,-0.384837557765384));
#190481=CARTESIAN_POINT('Ctrl Pts',(11.159377384661,12.2,-0.383460899142509));
#190482=CARTESIAN_POINT('Ctrl Pts',(11.1563243500558,12.2,-0.38209091239123));
#190483=CARTESIAN_POINT('Ctrl Pts',(11.153276468986,12.2,-0.380727584767877));
#190484=CARTESIAN_POINT('Ctrl Pts',(11.1492126271905,12.2,-0.378909814438292));
#190485=CARTESIAN_POINT('Ctrl Pts',(11.1451579450302,12.2,-0.377103884222651));
#190486=CARTESIAN_POINT('Ctrl Pts',(11.1411125345885,12.2,-0.375309765181635));
#190487=CARTESIAN_POINT('Ctrl Pts',(11.1370671246979,12.2,-0.373515646385067));
#190488=CARTESIAN_POINT('Ctrl Pts',(11.1330309860561,12.2,-0.371733339120291));
#190489=CARTESIAN_POINT('Ctrl Pts',(11.1290042288292,12.2,-0.369962813653153));
#190490=CARTESIAN_POINT('Ctrl Pts',(11.1249774710536,12.2,-0.368192287944782));
#190491=CARTESIAN_POINT('Ctrl Pts',(11.1209600942279,12.2,-0.366433545350228));
#190492=CARTESIAN_POINT('Ctrl Pts',(11.1169522116434,12.2,-0.36468655427987));
#190493=CARTESIAN_POINT('Ctrl Pts',(11.112944329605,12.2,-0.36293956344754));
#190494=CARTESIAN_POINT('Ctrl Pts',(11.1089459418451,12.2,-0.361204326048066));
#190495=CARTESIAN_POINT('Ctrl Pts',(11.1049571600594,12.2,-0.359480811132644));
#190496=CARTESIAN_POINT('Ctrl Pts',(11.1009683777303,12.2,-0.357757295982392));
#190497=CARTESIAN_POINT('Ctrl Pts',(11.0969892016968,12.2,-0.356045502069655));
#190498=CARTESIAN_POINT('Ctrl Pts',(11.0930197459255,12.2,-0.354345400311095));
#190499=CARTESIAN_POINT('Ctrl Pts',(11.0890502906951,12.2,-0.352645298784174));
#190500=CARTESIAN_POINT('Ctrl Pts',(11.0850905543428,12.2,-0.350956889810494));
#190501=CARTESIAN_POINT('Ctrl Pts',(11.0811406523565,12.2,-0.349280140251676));
#190502=CARTESIAN_POINT('Ctrl Pts',(11.0771907498319,12.2,-0.3476033904644));
#190503=CARTESIAN_POINT('Ctrl Pts',(11.0732506818173,12.2,-0.345938300848709));
#190504=CARTESIAN_POINT('Ctrl Pts',(11.069320563437,12.2,-0.344284839648241));
#190505=CARTESIAN_POINT('Ctrl Pts',(11.0653904455923,12.2,-0.342631378673058));
#190506=CARTESIAN_POINT('Ctrl Pts',(11.0614702769483,12.2,-0.340989545139982));
#190507=CARTESIAN_POINT('Ctrl Pts',(11.0575601731559,12.2,-0.339359307049856));
#190508=CARTESIAN_POINT('Ctrl Pts',(11.0536500688307,12.2,-0.33772906873761));
#190509=CARTESIAN_POINT('Ctrl Pts',(11.0497500299019,12.2,-0.336110426427056));
#190510=CARTESIAN_POINT('Ctrl Pts',(11.0458601735056,12.2,-0.334503345998876));
#190511=CARTESIAN_POINT('Ctrl Pts',(11.0419703176393,12.2,-0.332896265789661));
#190512=CARTESIAN_POINT('Ctrl Pts',(11.0380906431145,12.2,-0.331300747827863));
#190513=CARTESIAN_POINT('Ctrl Pts',(11.0342212693742,12.2,-0.32971675823396));
#190514=CARTESIAN_POINT('Ctrl Pts',(11.0303518951068,12.2,-0.328132768424238));
#190515=CARTESIAN_POINT('Ctrl Pts',(11.0264928214041,12.2,-0.326560306321151));
#190516=CARTESIAN_POINT('Ctrl Pts',(11.0226441657499,12.2,-0.324999337291632));
#190517=CARTESIAN_POINT('Ctrl Pts',(11.0187955100957,12.2,-0.323438368262112));
#190518=CARTESIAN_POINT('Ctrl Pts',(11.0149572732483,12.2,-0.321888894081161));
#190519=CARTESIAN_POINT('Ctrl Pts',(11.0111295743741,12.2,-0.320350876998509));
#190520=CARTESIAN_POINT('Ctrl Pts',(11.0073018760214,12.2,-0.318812860125413));
#190521=CARTESIAN_POINT('Ctrl Pts',(11.0034847161864,12.2,-0.317286302247945));
#190522=CARTESIAN_POINT('Ctrl Pts',(10.9996782157025,12.2,-0.315771165976002));
#190523=CARTESIAN_POINT('Ctrl Pts',(10.9958717146999,12.2,-0.314256029497622));
#190524=CARTESIAN_POINT('Ctrl Pts',(10.9920758723835,12.2,-0.312752315102815));
#190525=CARTESIAN_POINT('Ctrl Pts',(10.9882908101227,12.2,-0.311259986022648));
#190526=CARTESIAN_POINT('Ctrl Pts',(10.9835594825547,12.2,-0.309394574774104));
#190527=CARTESIAN_POINT('Ctrl Pts',(10.9788450003228,12.2,-0.30754695418688));
#190528=CARTESIAN_POINT('Ctrl Pts',(10.9741476003936,12.2,-0.305717049535556));
#190529=CARTESIAN_POINT('Ctrl Pts',(10.9703896807575,12.2,-0.304253125934172));
#190530=CARTESIAN_POINT('Ctrl Pts',(10.9666426956285,12.2,-0.302800541653595));
#190531=CARTESIAN_POINT('Ctrl Pts',(10.9629067678221,12.2,-0.301359256826237));
#190532=CARTESIAN_POINT('Ctrl Pts',(10.9591708395066,12.2,-0.299917971802503));
#190533=CARTESIAN_POINT('Ctrl Pts',(10.9554459682147,12.2,-0.298487987971941));
#190534=CARTESIAN_POINT('Ctrl Pts',(10.9517322784944,12.2,-0.297069264769167));
#190535=CARTESIAN_POINT('Ctrl Pts',(10.9480185892801,12.2,-0.295650541759694));
#190536=CARTESIAN_POINT('Ctrl Pts',(10.9443160825674,12.2,-0.294243080398028));
#190537=CARTESIAN_POINT('Ctrl Pts',(10.9406248835351,12.2,-0.292846840122553));
#190538=CARTESIAN_POINT('Ctrl Pts',(10.9369336839999,12.2,-0.29145059965684));
#190539=CARTESIAN_POINT('Ctrl Pts',(10.9332537922326,12.2,-0.29006558137024));
#190540=CARTESIAN_POINT('Ctrl Pts',(10.9295853347001,12.2,-0.288691744129432));
#190541=CARTESIAN_POINT('Ctrl Pts',(10.9259168776674,12.2,-0.28731790707581));
#190542=CARTESIAN_POINT('Ctrl Pts',(10.9222598558474,12.2,-0.285955250081925));
#190543=CARTESIAN_POINT('Ctrl Pts',(10.9186143959623,12.2,-0.284603733679482));
#190544=CARTESIAN_POINT('Ctrl Pts',(10.9149689355805,12.2,-0.283252217092895));
#190545=CARTESIAN_POINT('Ctrl Pts',(10.9113350371811,12.2,-0.281911840393686));
#190546=CARTESIAN_POINT('Ctrl Pts',(10.9077128302622,12.2,-0.280582560599743));
#190547=CARTESIAN_POINT('Ctrl Pts',(10.9031850718604,12.2,-0.278920960947872));
#190548=CARTESIAN_POINT('Ctrl Pts',(10.8986755801998,12.2,-0.277276702226101));
#190549=CARTESIAN_POINT('Ctrl Pts',(10.8941846109646,12.2,-0.275649699935338));
#190550=CARTESIAN_POINT('Ctrl Pts',(10.8905918358702,12.2,-0.274348098209133));
#190551=CARTESIAN_POINT('Ctrl Pts',(10.8870109143554,12.2,-0.273057540179318));
#190552=CARTESIAN_POINT('Ctrl Pts',(10.8834419784678,12.2,-0.271777981885708));
#190553=CARTESIAN_POINT('Ctrl Pts',(10.8789808082437,12.2,-0.270178533887939));
#190554=CARTESIAN_POINT('Ctrl Pts',(10.8745383625625,12.2,-0.268596275058888));
#190555=CARTESIAN_POINT('Ctrl Pts',(10.870114905756,12.2,-0.26703111533577));
#190556=CARTESIAN_POINT('Ctrl Pts',(10.8665761401179,12.2,-0.265778987489035));
#190557=CARTESIAN_POINT('Ctrl Pts',(10.8630495249284,12.2,-0.264537804054729));
#190558=CARTESIAN_POINT('Ctrl Pts',(10.8595351942377,12.2,-0.263307519432833));
#190559=CARTESIAN_POINT('Ctrl Pts',(10.8560208640258,12.2,-0.262077234978564));
#190560=CARTESIAN_POINT('Ctrl Pts',(10.8525188196687,12.2,-0.260857848346251));
#190561=CARTESIAN_POINT('Ctrl Pts',(10.8490291945563,12.2,-0.259649313883731));
#190562=CARTESIAN_POINT('Ctrl Pts',(10.8455395689685,12.2,-0.258440779256548));
#190563=CARTESIAN_POINT('Ctrl Pts',(10.8420623639215,12.2,-0.257243095903136));
#190564=CARTESIAN_POINT('Ctrl Pts',(10.8385977157334,12.2,-0.256056217894713));
#190565=CARTESIAN_POINT('Ctrl Pts',(10.8351330680175,12.2,-0.254869340048002));
#190566=CARTESIAN_POINT('Ctrl Pts',(10.8316809754046,12.2,-0.253693266357451));
#190567=CARTESIAN_POINT('Ctrl Pts',(10.8282415777956,12.2,-0.252527948673841));
#190568=CARTESIAN_POINT('Ctrl Pts',(10.8248021797179,12.2,-0.251362630831455));
#190569=CARTESIAN_POINT('Ctrl Pts',(10.8213754767546,12.2,-0.250208068436137));
#190570=CARTESIAN_POINT('Ctrl Pts',(10.8179616059976,12.2,-0.249064213757529));
#190571=CARTESIAN_POINT('Ctrl Pts',(10.8145477357056,12.2,-0.247920359234771));
#190572=CARTESIAN_POINT('Ctrl Pts',(10.8111466970838,12.2,-0.246787210765058));
#190573=CARTESIAN_POINT('Ctrl Pts',(10.8077586328038,12.2,-0.245664719633507));
#190574=CARTESIAN_POINT('Ctrl Pts',(10.8043705680623,12.2,-0.244542228349017));
#190575=CARTESIAN_POINT('Ctrl Pts',(10.8009954759054,12.2,-0.243430394209988));
#190576=CARTESIAN_POINT('Ctrl Pts',(10.7976334984999,12.2,-0.242329164483303));
#190577=CARTESIAN_POINT('Ctrl Pts',(10.7942715210944,12.2,-0.241227934756618));
#190578=CARTESIAN_POINT('Ctrl Pts',(10.7909226576766,12.2,-0.240137311931174));
#190579=CARTESIAN_POINT('Ctrl Pts',(10.7875870516629,12.2,-0.239057242540053));
#190580=CARTESIAN_POINT('Ctrl Pts',(10.7842514461036,12.2,-0.237977173296091));
#190581=CARTESIAN_POINT('Ctrl Pts',(10.7809290979606,12.2,-0.236907656688414));
#190582=CARTESIAN_POINT('Ctrl Pts',(10.7776201504938,12.2,-0.235848641492363));
#190583=CARTESIAN_POINT('Ctrl Pts',(10.7743112025762,12.2,-0.23478962615202));
#190584=CARTESIAN_POINT('Ctrl Pts',(10.7710156565991,12.2,-0.233741111310766));
#190585=CARTESIAN_POINT('Ctrl Pts',(10.767733657255,12.2,-0.232703042755253));
#190586=CARTESIAN_POINT('Ctrl Pts',(10.764451658358,12.2,-0.231664974341178));
#190587=CARTESIAN_POINT('Ctrl Pts',(10.7611832059259,12.2,-0.230637352584084));
#190588=CARTESIAN_POINT('Ctrl Pts',(10.7579284470244,12.2,-0.229620123333231));
#190589=CARTESIAN_POINT('Ctrl Pts',(10.7546736876795,12.2,-0.228602893943781));
#190590=CARTESIAN_POINT('Ctrl Pts',(10.751432622162,12.2,-0.227596055778067));
#190591=CARTESIAN_POINT('Ctrl Pts',(10.7482053980483,12.2,-0.226599553063762));
#190592=CARTESIAN_POINT('Ctrl Pts',(10.7449781743744,12.2,-0.22560305048523));
#190593=CARTESIAN_POINT('Ctrl Pts',(10.7417647931259,12.2,-0.224616883622968));
#190594=CARTESIAN_POINT('Ctrl Pts',(10.7385654035532,12.2,-0.223640995813185));
#190595=CARTESIAN_POINT('Ctrl Pts',(10.7345661662604,12.2,-0.222421135951232));
#190596=CARTESIAN_POINT('Ctrl Pts',(10.7305887888932,12.2,-0.221217337023033));
#190597=CARTESIAN_POINT('Ctrl Pts',(10.726633570767,12.2,-0.220029483827759));
#190598=CARTESIAN_POINT('Ctrl Pts',(10.7226783526409,12.2,-0.218841630632484));
#190599=CARTESIAN_POINT('Ctrl Pts',(10.7187452921143,12.2,-0.217669724205901));
#190600=CARTESIAN_POINT('Ctrl Pts',(10.714834688277,12.2,-0.216513649200605));
#190601=CARTESIAN_POINT('Ctrl Pts',(10.7109240844398,12.2,-0.215357574195309));
#190602=CARTESIAN_POINT('Ctrl Pts',(10.7070359377665,12.2,-0.214217329544415));
#190603=CARTESIAN_POINT('Ctrl Pts',(10.7031705515165,12.2,-0.213092795516639));
#190604=CARTESIAN_POINT('Ctrl Pts',(10.6993051652665,12.2,-0.211968261488863));
#190605=CARTESIAN_POINT('Ctrl Pts',(10.6954625399832,12.2,-0.21085943898331));
#190606=CARTESIAN_POINT('Ctrl Pts',(10.6916429812332,12.2,-0.209766206483308));
#190607=CARTESIAN_POINT('Ctrl Pts',(10.6878234224832,12.2,-0.208672973983305));
#190608=CARTESIAN_POINT('Ctrl Pts',(10.6840269327982,12.2,-0.207595331087518));
#190609=CARTESIAN_POINT('Ctrl Pts',(10.6802538215312,12.2,-0.206533152749401));
#190610=CARTESIAN_POINT('Ctrl Pts',(10.6757260881752,12.2,-0.205258538789973));
#190611=CARTESIAN_POINT('Ctrl Pts',(10.6712320193909,12.2,-0.204006195373377));
#190612=CARTESIAN_POINT('Ctrl Pts',(10.6667721629681,12.2,-0.202775898583787));
#190613=CARTESIAN_POINT('Ctrl Pts',(10.6630556158141,12.2,-0.201750651221878));
#190614=CARTESIAN_POINT('Ctrl Pts',(10.6593628272579,12.2,-0.200740715354806));
#190615=CARTESIAN_POINT('Ctrl Pts',(10.655694116215,12.2,-0.199745961048458));
#190616=CARTESIAN_POINT('Ctrl Pts',(10.6505579206749,12.2,-0.198353304997884));
#190617=CARTESIAN_POINT('Ctrl Pts',(10.6454689197468,12.2,-0.196990401379664));
#190618=CARTESIAN_POINT('Ctrl Pts',(10.6404280057812,12.2,-0.19565688142944));
#190619=CARTESIAN_POINT('Ctrl Pts',(10.6368273530047,12.2,-0.194704367194113));
#190620=CARTESIAN_POINT('Ctrl Pts',(10.6332512359276,12.2,-0.193766844250058));
#190621=CARTESIAN_POINT('Ctrl Pts',(10.6296999839844,12.2,-0.192844174181391));
#190622=CARTESIAN_POINT('Ctrl Pts',(10.6261487320413,12.2,-0.191921504112725));
#190623=CARTESIAN_POINT('Ctrl Pts',(10.6226223465778,12.2,-0.191013687017728));
#190624=CARTESIAN_POINT('Ctrl Pts',(10.6191211636269,12.2,-0.190120579404687));
#190625=CARTESIAN_POINT('Ctrl Pts',(10.6156199806759,12.2,-0.189227471791647));
#190626=CARTESIAN_POINT('Ctrl Pts',(10.6121440011632,12.2,-0.18834907546914));
#190627=CARTESIAN_POINT('Ctrl Pts',(10.6086935628319,12.2,-0.187485244428661));
#190628=CARTESIAN_POINT('Ctrl Pts',(10.6052431245007,12.2,-0.186621413388182));
#190629=CARTESIAN_POINT('Ctrl Pts',(10.6018182308698,12.2,-0.185772147645162));
#190630=CARTESIAN_POINT('Ctrl Pts',(10.5984192250386,12.2,-0.18493729688245));
#190631=CARTESIAN_POINT('Ctrl Pts',(10.5950202195779,12.2,-0.184102446210736));
#190632=CARTESIAN_POINT('Ctrl Pts',(10.5916471040972,12.2,-0.183282013924282));
#190633=CARTESIAN_POINT('Ctrl Pts',(10.5883002284877,12.2,-0.182475843872099));
#190634=CARTESIAN_POINT('Ctrl Pts',(10.5849533525133,12.2,-0.181669673732044));
#190635=CARTESIAN_POINT('Ctrl Pts',(10.5816327171829,12.2,-0.180877769213984));
#190636=CARTESIAN_POINT('Ctrl Pts',(10.5783386771807,12.2,-0.180099970810053));
#190637=CARTESIAN_POINT('Ctrl Pts',(10.5737270211059,12.2,-0.179011053027593));
#190638=CARTESIAN_POINT('Ctrl Pts',(10.5691674934979,12.2,-0.177949788899013));
#190639=CARTESIAN_POINT('Ctrl Pts',(10.5646610904766,12.2,-0.176915735558718));
#190640=CARTESIAN_POINT('Ctrl Pts',(10.560798459516,12.2,-0.176029404170184));
#190641=CARTESIAN_POINT('Ctrl Pts',(10.5569748564442,12.2,-0.175163063562843));
#190642=CARTESIAN_POINT('Ctrl Pts',(10.5531909254123,12.2,-0.174316430092268));
#190643=CARTESIAN_POINT('Ctrl Pts',(10.5494069940368,12.2,-0.173469796544791));
#190644=CARTESIAN_POINT('Ctrl Pts',(10.5456627317846,12.2,-0.172642866396811));
#190645=CARTESIAN_POINT('Ctrl Pts',(10.54195879065,12.2,-0.171835348896911));
#190646=CARTESIAN_POINT('Ctrl Pts',(10.5382548498519,12.2,-0.17102783147036));
#190647=CARTESIAN_POINT('Ctrl Pts',(10.5345912315432,12.2,-0.170239724680368));
#190648=CARTESIAN_POINT('Ctrl Pts',(10.5309685997582,12.2,-0.169470725458311));
#190649=CARTESIAN_POINT('Ctrl Pts',(10.5273459679732,12.2,-0.168701726236254));
#190650=CARTESIAN_POINT('Ctrl Pts',(10.5237643214848,12.2,-0.167951834673472));
#190651=CARTESIAN_POINT('Ctrl Pts',(10.5202243403508,12.2,-0.167220739079087));
#190652=CARTESIAN_POINT('Ctrl Pts',(10.5166843588952,12.2,-0.166489643418294));
#190653=CARTESIAN_POINT('Ctrl Pts',(10.513186040767,12.2,-0.165777341977581));
#190654=CARTESIAN_POINT('Ctrl Pts',(10.5097300788315,12.2,-0.165083514441026));
#190655=CARTESIAN_POINT('Ctrl Pts',(10.50627411721,12.2,-0.164389686967494));
#190656=CARTESIAN_POINT('Ctrl Pts',(10.5028605111161,12.2,-0.163714333462085));
#190657=CARTESIAN_POINT('Ctrl Pts',(10.4994899664733,12.2,-0.163057121983021));
#190658=CARTESIAN_POINT('Ctrl Pts',(10.4961194218306,12.2,-0.162399910503956));
#190659=CARTESIAN_POINT('Ctrl Pts',(10.4927919382116,12.2,-0.16176084233712));
#190660=CARTESIAN_POINT('Ctrl Pts',(10.4895082376623,12.2,-0.161139573775585));
#190661=CARTESIAN_POINT('Ctrl Pts',(10.4862245368148,12.2,-0.160518305157617));
#190662=CARTESIAN_POINT('Ctrl Pts',(10.4829846190144,12.2,-0.15991483808353));
#190663=CARTESIAN_POINT('Ctrl Pts',(10.4797892174266,12.2,-0.159328820386113));
#190664=CARTESIAN_POINT('Ctrl Pts',(10.4765938161291,12.2,-0.158742802741927));
#190665=CARTESIAN_POINT('Ctrl Pts',(10.473442932833,12.2,-0.15817423424883));
#190666=CARTESIAN_POINT('Ctrl Pts',(10.4703373212651,12.2,-0.157622752433069));
#190667=CARTESIAN_POINT('Ctrl Pts',(10.4672317096973,12.2,-0.157071270617307));
#190668=CARTESIAN_POINT('Ctrl Pts',(10.4641713672068,12.2,-0.15653687501852));
#190669=CARTESIAN_POINT('Ctrl Pts',(10.461157063981,12.2,-0.156019192286602));
#190670=CARTESIAN_POINT('Ctrl Pts',(10.4581427604814,12.2,-0.155501509507661));
#190671=CARTESIAN_POINT('Ctrl Pts',(10.4551744963291,12.2,-0.155000539055797));
#190672=CARTESIAN_POINT('Ctrl Pts',(10.4522530569231,12.2,-0.154515896197163));
#190673=CARTESIAN_POINT('Ctrl Pts',(10.4493316177824,12.2,-0.154031253382552));
#190674=CARTESIAN_POINT('Ctrl Pts',(10.4464570057329,12.2,-0.153562937449933));
#190675=CARTESIAN_POINT('Ctrl Pts',(10.4436300225877,12.2,-0.153110550717065));
#190676=CARTESIAN_POINT('Ctrl Pts',(10.4403318754137,12.2,-0.152582766167991));
#190677=CARTESIAN_POINT('Ctrl Pts',(10.4370985574772,12.2,-0.15207666472211));
#190678=CARTESIAN_POINT('Ctrl Pts',(10.4339313792373,12.2,-0.15159159047967));
#190679=CARTESIAN_POINT('Ctrl Pts',(10.4312166551726,12.2,-0.15117581257916));
#190680=CARTESIAN_POINT('Ctrl Pts',(10.4285505235436,12.2,-0.150775484964402));
#190681=CARTESIAN_POINT('Ctrl Pts',(10.4259338326408,12.2,-0.150390178979053));
#190682=CARTESIAN_POINT('Ctrl Pts',(10.423317141738,12.2,-0.150004872993703));
#190683=CARTESIAN_POINT('Ctrl Pts',(10.4207498912063,12.2,-0.149634591290477));
#190684=CARTESIAN_POINT('Ctrl Pts',(10.4182329483789,12.2,-0.149278892969435));
#190685=CARTESIAN_POINT('Ctrl Pts',(10.4157160055515,12.2,-0.148923194648394));
#190686=CARTESIAN_POINT('Ctrl Pts',(10.4132493716372,12.2,-0.148582077324715));
#190687=CARTESIAN_POINT('Ctrl Pts',(10.4108339349715,12.2,-0.148255091002302));
#190688=CARTESIAN_POINT('Ctrl Pts',(10.4084184980864,12.2,-0.147928104650187));
#190689=CARTESIAN_POINT('Ctrl Pts',(10.4060542611478,12.2,-0.147615246091123));
#190690=CARTESIAN_POINT('Ctrl Pts',(10.4037421353574,12.2,-0.147316045992075));
#190691=CARTESIAN_POINT('Ctrl Pts',(10.401430009777,12.2,-0.147016845920205));
#190692=CARTESIAN_POINT('Ctrl Pts',(10.3991699947892,12.2,-0.146731306383157));
#190693=CARTESIAN_POINT('Ctrl Pts',(10.3969630302759,12.2,-0.146458939975118));
#190694=CARTESIAN_POINT('Ctrl Pts',(10.39438823821,12.2,-0.146141179149247));
#190695=CARTESIAN_POINT('Ctrl Pts',(10.3918856495939,12.2,-0.145841349057267));
#190696=CARTESIAN_POINT('Ctrl Pts',(10.3894567993783,12.2,-0.145558650261839));
#190697=CARTESIAN_POINT('Ctrl Pts',(10.3873749278729,12.2,-0.145316337021192));
#190698=CARTESIAN_POINT('Ctrl Pts',(10.3853472317298,12.2,-0.145086611134867));
#190699=CARTESIAN_POINT('Ctrl Pts',(10.3833747045424,12.2,-0.144868947725095));
#190700=CARTESIAN_POINT('Ctrl Pts',(10.3800966258014,12.2,-0.144507219987798));
#190701=CARTESIAN_POINT('Ctrl Pts',(10.3769709056722,12.2,-0.144178829281747));
#190702=CARTESIAN_POINT('Ctrl Pts',(10.3740022749999,12.2,-0.143881227000016));
#190703=CARTESIAN_POINT('Ctrl Pts',(10.3740022749999,15.2,-0.143881227000016));
#190704=CARTESIAN_POINT('Ctrl Pts',(10.3757800241214,15.2,-0.144059444586938));
#190705=CARTESIAN_POINT('Ctrl Pts',(10.3776141114604,15.2,-0.144248693896987));
#190706=CARTESIAN_POINT('Ctrl Pts',(10.3795035132429,15.2,-0.144449544719664));
#190707=CARTESIAN_POINT('Ctrl Pts',(10.3814020266759,15.2,-0.144651364146533));
#190708=CARTESIAN_POINT('Ctrl Pts',(10.3833563884146,15.2,-0.144864887714238));
#190709=CARTESIAN_POINT('Ctrl Pts',(10.385365584961,15.2,-0.14509065123853));
#190710=CARTESIAN_POINT('Ctrl Pts',(10.388044513507,15.2,-0.145391669250414));
#190711=CARTESIAN_POINT('Ctrl Pts',(10.3908209228729,15.2,-0.145714448637587));
#190712=CARTESIAN_POINT('Ctrl Pts',(10.3936924900591,15.2,-0.146060206522512));
#190713=CARTESIAN_POINT('Ctrl Pts',(10.3958461653999,15.2,-0.146319524930317));
#190714=CARTESIAN_POINT('Ctrl Pts',(10.3980533672458,15.2,-0.14659176898398));
#190715=CARTESIAN_POINT('Ctrl Pts',(10.4003131477572,15.2,-0.146877430224863));
#190716=CARTESIAN_POINT('Ctrl Pts',(10.4025729282685,15.2,-0.147163091465747));
#190717=CARTESIAN_POINT('Ctrl Pts',(10.4048852841982,15.2,-0.147462171811529));
#190718=CARTESIAN_POINT('Ctrl Pts',(10.4072492937755,15.2,-0.147775147965879));
#190719=CARTESIAN_POINT('Ctrl Pts',(10.4096133035675,15.2,-0.148088124148657));
#190720=CARTESIAN_POINT('Ctrl Pts',(10.412028965728,15.2,-0.148414996054894));
#190721=CARTESIAN_POINT('Ctrl Pts',(10.4144953769886,15.2,-0.148756224508035));
#190722=CARTESIAN_POINT('Ctrl Pts',(10.4169617880251,15.2,-0.149097452930182));
#190723=CARTESIAN_POINT('Ctrl Pts',(10.4194789511848,15.2,-0.149453042596778));
#190724=CARTESIAN_POINT('Ctrl Pts',(10.4220459850082,15.2,-0.149823433749987));
#190725=CARTESIAN_POINT('Ctrl Pts',(10.4246130188316,15.2,-0.150193824903195));
#190726=CARTESIAN_POINT('Ctrl Pts',(10.4272299231919,15.2,-0.150579023848384));
#190727=CARTESIAN_POINT('Ctrl Pts',(10.4298958432254,15.2,-0.150979457936288));
#190728=CARTESIAN_POINT('Ctrl Pts',(10.4325617635011,15.2,-0.151379892060566));
#190729=CARTESIAN_POINT('Ctrl Pts',(10.4352766973889,15.2,-0.151795566197436));
#190730=CARTESIAN_POINT('Ctrl Pts',(10.4380398077927,15.2,-0.152226895305339));
#190731=CARTESIAN_POINT('Ctrl Pts',(10.4408029179456,15.2,-0.152658224374064));
#190732=CARTESIAN_POINT('Ctrl Pts',(10.4436142067169,15.2,-0.153105210956548));
#190733=CARTESIAN_POINT('Ctrl Pts',(10.4464728530428,15.2,-0.153568261691863));
#190734=CARTESIAN_POINT('Ctrl Pts',(10.4493314993687,15.2,-0.154031312427179));
#190735=CARTESIAN_POINT('Ctrl Pts',(10.4522375075401,15.2,-0.154510424983432));
#190736=CARTESIAN_POINT('Ctrl Pts',(10.4551900758475,15.2,-0.155005995714713));
#190737=CARTESIAN_POINT('Ctrl Pts',(10.458142644423,15.2,-0.15550156649101));
#190738=CARTESIAN_POINT('Ctrl Pts',(10.4611417736544,15.2,-0.156013593785998));
#190739=CARTESIAN_POINT('Ctrl Pts',(10.4641866850734,15.2,-0.156542459565971));
#190740=CARTESIAN_POINT('Ctrl Pts',(10.4672315962159,15.2,-0.157071325297905));
#190741=CARTESIAN_POINT('Ctrl Pts',(10.4703222864829,15.2,-0.157617030983772));
#190742=CARTESIAN_POINT('Ctrl Pts',(10.4734579967043,15.2,-0.158179943797402));
#190743=CARTESIAN_POINT('Ctrl Pts',(10.4765937069257,15.2,-0.158742856611032));
#190744=CARTESIAN_POINT('Ctrl Pts',(10.4797744331017,15.2,-0.159322978306633));
#190745=CARTESIAN_POINT('Ctrl Pts',(10.482999430566,15.2,-0.159920667950818));
#190746=CARTESIAN_POINT('Ctrl Pts',(10.4867619278028,15.2,-0.160617972571893));
#190747=CARTESIAN_POINT('Ctrl Pts',(10.4905846827399,15.2,-0.161339189690789));
#190748=CARTESIAN_POINT('Ctrl Pts',(10.4944665360264,15.2,-0.162084868983609));
#190749=CARTESIAN_POINT('Ctrl Pts',(10.4977938386707,15.2,-0.162724022629994));
#190750=CARTESIAN_POINT('Ctrl Pts',(10.5011645619149,15.2,-0.163381150255252));
#190751=CARTESIAN_POINT('Ctrl Pts',(10.504577991539,15.2,-0.164056586729913));
#190752=CARTESIAN_POINT('Ctrl Pts',(10.5079914214732,15.2,-0.164732023265927));
#190753=CARTESIAN_POINT('Ctrl Pts',(10.511447558546,15.2,-0.165425769037539));
#190754=CARTESIAN_POINT('Ctrl Pts',(10.5149457026562,15.2,-0.166138150577636));
#190755=CARTESIAN_POINT('Ctrl Pts',(10.5184438464486,15.2,-0.166850532053025));
#190756=CARTESIAN_POINT('Ctrl Pts',(10.5219840010736,15.2,-0.16758154846736));
#190757=CARTESIAN_POINT('Ctrl Pts',(10.5255654769452,15.2,-0.168331518774267));
#190758=CARTESIAN_POINT('Ctrl Pts',(10.5309376907527,15.2,-0.169456474234627));
#190759=CARTESIAN_POINT('Ctrl Pts',(10.5364028794528,15.2,-0.170624072757087));
#190760=CARTESIAN_POINT('Ctrl Pts',(10.54195879065,15.2,-0.17183534889691));
#190761=CARTESIAN_POINT('Ctrl Pts',(10.5456627317846,15.2,-0.172642866396808));
#190762=CARTESIAN_POINT('Ctrl Pts',(10.5494069940367,15.2,-0.173469796544786));
#190763=CARTESIAN_POINT('Ctrl Pts',(10.5531909254123,15.2,-0.174316430092267));
#190764=CARTESIAN_POINT('Ctrl Pts',(10.5569748564442,15.2,-0.175163063562845));
#190765=CARTESIAN_POINT('Ctrl Pts',(10.560798459516,15.2,-0.176029404170188));
#190766=CARTESIAN_POINT('Ctrl Pts',(10.5646610904766,15.2,-0.176915735558719));
#190767=CARTESIAN_POINT('Ctrl Pts',(10.5685237214373,15.2,-0.177802066947249));
#190768=CARTESIAN_POINT('Ctrl Pts',(10.5724253830885,15.2,-0.178708390075781));
#190769=CARTESIAN_POINT('Ctrl Pts',(10.576365447027,15.2,-0.179634983457898));
#190770=CARTESIAN_POINT('Ctrl Pts',(10.5796488337617,15.2,-0.180407144637717));
#190771=CARTESIAN_POINT('Ctrl Pts',(10.5829588878388,15.2,-0.181193381887345));
#190772=CARTESIAN_POINT('Ctrl Pts',(10.5862952537402,15.2,-0.181993852164381));
#190773=CARTESIAN_POINT('Ctrl Pts',(10.5902988926764,15.2,-0.182954416461924));
#190774=CARTESIAN_POINT('Ctrl Pts',(10.5943404181894,15.2,-0.183935476003593));
#190775=CARTESIAN_POINT('Ctrl Pts',(10.5984192250386,15.2,-0.184937296882449));
#190776=CARTESIAN_POINT('Ctrl Pts',(10.6018182308698,15.2,-0.185772147645162));
#190777=CARTESIAN_POINT('Ctrl Pts',(10.6052431245007,15.2,-0.186621413388184));
#190778=CARTESIAN_POINT('Ctrl Pts',(10.6086935628319,15.2,-0.187485244428661));
#190779=CARTESIAN_POINT('Ctrl Pts',(10.6121440011631,15.2,-0.188349075469137));
#190780=CARTESIAN_POINT('Ctrl Pts',(10.6156199806759,15.2,-0.189227471791648));
#190781=CARTESIAN_POINT('Ctrl Pts',(10.6191211636269,15.2,-0.190120579404687));
#190782=CARTESIAN_POINT('Ctrl Pts',(10.6226223465778,15.2,-0.191013687017726));
#190783=CARTESIAN_POINT('Ctrl Pts',(10.6261487320413,15.2,-0.191921504112721));
#190784=CARTESIAN_POINT('Ctrl Pts',(10.6296999839844,15.2,-0.192844174181391));
#190785=CARTESIAN_POINT('Ctrl Pts',(10.6332512359276,15.2,-0.193766844250061));
#190786=CARTESIAN_POINT('Ctrl Pts',(10.6368273530047,15.2,-0.194704367194112));
#190787=CARTESIAN_POINT('Ctrl Pts',(10.6404280057812,15.2,-0.19565688142944));
#190788=CARTESIAN_POINT('Ctrl Pts',(10.644748788956,15.2,-0.196799898470305));
#190789=CARTESIAN_POINT('Ctrl Pts',(10.6491049027498,15.2,-0.197964503765251));
#190790=CARTESIAN_POINT('Ctrl Pts',(10.6534957812546,15.2,-0.199150928887326));
#190791=CARTESIAN_POINT('Ctrl Pts',(10.6571548468082,15.2,-0.200139616524977));
#190792=CARTESIAN_POINT('Ctrl Pts',(10.6608380563781,15.2,-0.201143458756819));
#190793=CARTESIAN_POINT('Ctrl Pts',(10.6645450875567,15.2,-0.202162586325013));
#190794=CARTESIAN_POINT('Ctrl Pts',(10.6682521187353,15.2,-0.203181713893206));
#190795=CARTESIAN_POINT('Ctrl Pts',(10.6719829715727,15.2,-0.204216126299005));
#190796=CARTESIAN_POINT('Ctrl Pts',(10.6757373296058,15.2,-0.205265953086495));
#190797=CARTESIAN_POINT('Ctrl Pts',(10.679491687639,15.2,-0.206315779873984));
#190798=CARTESIAN_POINT('Ctrl Pts',(10.6832695496582,15.2,-0.207381020669087));
#190799=CARTESIAN_POINT('Ctrl Pts',(10.6870706034764,15.2,-0.208461802196053));
#190800=CARTESIAN_POINT('Ctrl Pts',(10.6908716572947,15.2,-0.20954258372302));
#190801=CARTESIAN_POINT('Ctrl Pts',(10.6946959046941,15.2,-0.210638904294831));
#190802=CARTESIAN_POINT('Ctrl Pts',(10.6985430327484,15.2,-0.211750888460679));
#190803=CARTESIAN_POINT('Ctrl Pts',(10.7023901608028,15.2,-0.212862872626528));
#190804=CARTESIAN_POINT('Ctrl Pts',(10.7062601726189,15.2,-0.213990519292782));
#190805=CARTESIAN_POINT('Ctrl Pts',(10.7101527622704,15.2,-0.215133949916956));
#190806=CARTESIAN_POINT('Ctrl Pts',(10.7148238696827,15.2,-0.216506066616112));
#190807=CARTESIAN_POINT('Ctrl Pts',(10.719527489083,15.2,-0.217900909473521));
#190808=CARTESIAN_POINT('Ctrl Pts',(10.7242631004921,15.2,-0.219318684337112));
#190809=CARTESIAN_POINT('Ctrl Pts',(10.7282094434763,15.2,-0.220500163433032));
#190810=CARTESIAN_POINT('Ctrl Pts',(10.7321780037853,15.2,-0.221697566092568));
#190811=CARTESIAN_POINT('Ctrl Pts',(10.7361684857279,15.2,-0.222911006091261));
#190812=CARTESIAN_POINT('Ctrl Pts',(10.7401589676706,15.2,-0.224124446089953));
#190813=CARTESIAN_POINT('Ctrl Pts',(10.7441713681261,15.2,-0.22535392473877));
#190814=CARTESIAN_POINT('Ctrl Pts',(10.7482053980483,15.2,-0.226599553063764));
#190815=CARTESIAN_POINT('Ctrl Pts',(10.7530462342189,15.2,-0.228094307135222));
#190816=CARTESIAN_POINT('Ctrl Pts',(10.7579182140567,15.2,-0.229612315165725));
#190817=CARTESIAN_POINT('Ctrl Pts',(10.7628208380759,15.2,-0.231153768917997));
#190818=CARTESIAN_POINT('Ctrl Pts',(10.7660892536435,15.2,-0.232181404612829));
#190819=CARTESIAN_POINT('Ctrl Pts',(10.7693712890231,15.2,-0.233219459200759));
#190820=CARTESIAN_POINT('Ctrl Pts',(10.7726667985306,15.2,-0.234267987114358));
#190821=CARTESIAN_POINT('Ctrl Pts',(10.7776100630164,15.2,-0.235840779056186));
#190822=CARTESIAN_POINT('Ctrl Pts',(10.7825836430967,15.2,-0.237437138600533));
#190823=CARTESIAN_POINT('Ctrl Pts',(10.7875870516629,15.2,-0.239057242540053));
#190824=CARTESIAN_POINT('Ctrl Pts',(10.7909226576766,15.2,-0.240137311931172));
#190825=CARTESIAN_POINT('Ctrl Pts',(10.7942715210944,15.2,-0.241227934756618));
#190826=CARTESIAN_POINT('Ctrl Pts',(10.7976334984999,15.2,-0.242329164483303));
#190827=CARTESIAN_POINT('Ctrl Pts',(10.8009954759054,15.2,-0.243430394209989));
#190828=CARTESIAN_POINT('Ctrl Pts',(10.8043705680623,15.2,-0.244542228349019));
#190829=CARTESIAN_POINT('Ctrl Pts',(10.8077586328038,15.2,-0.245664719633506));
#190830=CARTESIAN_POINT('Ctrl Pts',(10.8119937130383,15.2,-0.247067833509706));
#190831=CARTESIAN_POINT('Ctrl Pts',(10.8162490652361,15.2,-0.248487598464472));
#190832=CARTESIAN_POINT('Ctrl Pts',(10.820524412199,15.2,-0.249924113028749));
#190833=CARTESIAN_POINT('Ctrl Pts',(10.8239446903286,15.2,-0.251073324868067));
#190834=CARTESIAN_POINT('Ctrl Pts',(10.8273777670232,15.2,-0.252233255663941));
#190835=CARTESIAN_POINT('Ctrl Pts',(10.8308235037666,15.2,-0.2534039542833));
#190836=CARTESIAN_POINT('Ctrl Pts',(10.8342692405099,15.2,-0.25457465290266));
#190837=CARTESIAN_POINT('Ctrl Pts',(10.8377276367047,15.2,-0.255756119584384));
#190838=CARTESIAN_POINT('Ctrl Pts',(10.8411985547841,15.2,-0.256948403428247));
#190839=CARTESIAN_POINT('Ctrl Pts',(10.8446694723905,15.2,-0.258140687109662));
#190840=CARTESIAN_POINT('Ctrl Pts',(10.8481529131147,15.2,-0.25934378664569));
#190841=CARTESIAN_POINT('Ctrl Pts',(10.8516487394559,15.2,-0.260557750274145));
#190842=CARTESIAN_POINT('Ctrl Pts',(10.8551445662733,15.2,-0.261771714068003));
#190843=CARTESIAN_POINT('Ctrl Pts',(10.8586527798352,15.2,-0.262996540222445));
#190844=CARTESIAN_POINT('Ctrl Pts',(10.8621732440838,15.2,-0.26423227740202));
#190845=CARTESIAN_POINT('Ctrl Pts',(10.8665738241548,15.2,-0.265776948792305));
#190846=CARTESIAN_POINT('Ctrl Pts',(10.87099354659,15.2,-0.267338667316199));
#190847=CARTESIAN_POINT('Ctrl Pts',(10.8754321523555,15.2,-0.26891752120649));
#190848=CARTESIAN_POINT('Ctrl Pts',(10.8798707576371,15.2,-0.270496374924684));
#190849=CARTESIAN_POINT('Ctrl Pts',(10.8843282437872,15.2,-0.272092363677334));
#190850=CARTESIAN_POINT('Ctrl Pts',(10.8888043541311,15.2,-0.273705574263971));
#190851=CARTESIAN_POINT('Ctrl Pts',(10.8932804649629,15.2,-0.275318785026448));
#190852=CARTESIAN_POINT('Ctrl Pts',(10.8977752004055,15.2,-0.276949218713644));
#190853=CARTESIAN_POINT('Ctrl Pts',(10.9022883038763,15.2,-0.278596959267787));
#190854=CARTESIAN_POINT('Ctrl Pts',(10.9058987868496,15.2,-0.279915151782942));
#190855=CARTESIAN_POINT('Ctrl Pts',(10.9095210263433,15.2,-0.281244421230046));
#190856=CARTESIAN_POINT('Ctrl Pts',(10.9131548930024,15.2,-0.282584808475887));
#190857=CARTESIAN_POINT('Ctrl Pts',(10.9167887591663,15.2,-0.2839251955391));
#190858=CARTESIAN_POINT('Ctrl Pts',(10.9204342508077,15.2,-0.285276701309163));
#190859=CARTESIAN_POINT('Ctrl Pts',(10.9240912406187,15.2,-0.28663936825218));
#190860=CARTESIAN_POINT('Ctrl Pts',(10.9286624782561,15.2,-0.288342702070198));
#190861=CARTESIAN_POINT('Ctrl Pts',(10.933251683671,15.2,-0.290063473285158));
#190862=CARTESIAN_POINT('Ctrl Pts',(10.9378586054057,15.2,-0.291801763005941));
#190863=CARTESIAN_POINT('Ctrl Pts',(10.9415441429942,15.2,-0.293192394858356));
#190864=CARTESIAN_POINT('Ctrl Pts',(10.9452410196473,15.2,-0.294594239175797));
#190865=CARTESIAN_POINT('Ctrl Pts',(10.9489491104774,15.2,-0.296007333759269));
#190866=CARTESIAN_POINT('Ctrl Pts',(10.9526572008023,15.2,-0.297420428150207));
#190867=CARTESIAN_POINT('Ctrl Pts',(10.9563765041961,15.2,-0.298844774892099));
#190868=CARTESIAN_POINT('Ctrl Pts',(10.96010689589,15.2,-0.300280411273583));
#190869=CARTESIAN_POINT('Ctrl Pts',(10.9638372880922,15.2,-0.301716047850672));
#190870=CARTESIAN_POINT('Ctrl Pts',(10.9675787682343,15.2,-0.303162975217712));
#190871=CARTESIAN_POINT('Ctrl Pts',(10.9713312132166,15.2,-0.304621232241633));
#190872=CARTESIAN_POINT('Ctrl Pts',(10.9750836581989,15.2,-0.306079489265555));
#190873=CARTESIAN_POINT('Ctrl Pts',(10.9788470681798,15.2,-0.307549075232504));
#190874=CARTESIAN_POINT('Ctrl Pts',(10.9826213191086,15.2,-0.309030027758749));
#190875=CARTESIAN_POINT('Ctrl Pts',(10.9863955695232,15.2,-0.310510980083215));
#190876=CARTESIAN_POINT('Ctrl Pts',(10.990180661984,15.2,-0.312003299567486));
#190877=CARTESIAN_POINT('Ctrl Pts',(10.993976473673,15.2,-0.313507023110482));
#190878=CARTESIAN_POINT('Ctrl Pts',(10.9977722858792,15.2,-0.315010746858359));
#190879=CARTESIAN_POINT('Ctrl Pts',(11.0015788171625,15.2,-0.316525874449976));
#190880=CARTESIAN_POINT('Ctrl Pts',(11.0053959470622,15.2,-0.318052441721547));
#190881=CARTESIAN_POINT('Ctrl Pts',(11.0120759236065,15.2,-0.320723934134804));
#190882=CARTESIAN_POINT('Ctrl Pts',(11.0187883583528,15.2,-0.323430463377752));
#190883=CARTESIAN_POINT('Ctrl Pts',(11.0255326083615,15.2,-0.326172219218818));
#190884=CARTESIAN_POINT('Ctrl Pts',(11.0322768588952,15.2,-0.328913975273349));
#190885=CARTESIAN_POINT('Ctrl Pts',(11.039052925077,15.2,-0.331690955359036));
#190886=CARTESIAN_POINT('Ctrl Pts',(11.0458601735056,15.2,-0.334503345998875));
#190887=CARTESIAN_POINT('Ctrl Pts',(11.0497500299019,15.2,-0.33611042642706));
#190888=CARTESIAN_POINT('Ctrl Pts',(11.0536500688306,15.2,-0.337729068737601));
#190889=CARTESIAN_POINT('Ctrl Pts',(11.0575601731559,15.2,-0.339359307049852));
#190890=CARTESIAN_POINT('Ctrl Pts',(11.0644028549259,15.2,-0.342212223763112));
#190891=CARTESIAN_POINT('Ctrl Pts',(11.0712763598475,15.2,-0.345100650362057));
#190892=CARTESIAN_POINT('Ctrl Pts',(11.0781800703859,15.2,-0.348024763240908));
#190893=CARTESIAN_POINT('Ctrl Pts',(11.0821250482971,15.2,-0.349695685081105));
#190894=CARTESIAN_POINT('Ctrl Pts',(11.0860798900324,15.2,-0.351378258428816));
#190895=CARTESIAN_POINT('Ctrl Pts',(11.0900444790824,15.2,-0.353072516188583));
#190896=CARTESIAN_POINT('Ctrl Pts',(11.0940090675923,15.2,-0.354766773717508));
#190897=CARTESIAN_POINT('Ctrl Pts',(11.0979834043697,15.2,-0.356472715607979));
#190898=CARTESIAN_POINT('Ctrl Pts',(11.1019673755985,15.2,-0.358190371744137));
#190899=CARTESIAN_POINT('Ctrl Pts',(11.1059513473702,15.2,-0.359908028114326));
#190900=CARTESIAN_POINT('Ctrl Pts',(11.1099449541246,15.2,-0.361637398078874));
#190901=CARTESIAN_POINT('Ctrl Pts',(11.1139480825276,15.2,-0.363378514459489));
#190902=CARTESIAN_POINT('Ctrl Pts',(11.1179512103853,15.2,-0.365119630602876));
#190903=CARTESIAN_POINT('Ctrl Pts',(11.1219638605776,15.2,-0.366872491570809));
#190904=CARTESIAN_POINT('Ctrl Pts',(11.125985920359,15.2,-0.368637127703124));
#190905=CARTESIAN_POINT('Ctrl Pts',(11.1300079806883,15.2,-0.37040176407587));
#190906=CARTESIAN_POINT('Ctrl Pts',(11.1340394499741,15.2,-0.372178175419171));
#190907=CARTESIAN_POINT('Ctrl Pts',(11.1380802177499,15.2,-0.373966390516629));
#190908=CARTESIAN_POINT('Ctrl Pts',(11.144141368863,15.2,-0.376648712919171));
#190909=CARTESIAN_POINT('Ctrl Pts',(11.150223442411,15.2,-0.379357595624685));
#190910=CARTESIAN_POINT('Ctrl Pts',(11.1563260656596,15.2,-0.382093132243738));
#190911=CARTESIAN_POINT('Ctrl Pts',(11.1593773772839,15.2,-0.383460900553265));
#190912=CARTESIAN_POINT('Ctrl Pts',(11.1624338258278,15.2,-0.384835332933315));
#190913=CARTESIAN_POINT('Ctrl Pts',(11.1654953658408,15.2,-0.386216440215559));
#190914=CARTESIAN_POINT('Ctrl Pts',(11.1685569064101,15.2,-0.387597547748704));
#190915=CARTESIAN_POINT('Ctrl Pts',(11.1716235383224,15.2,-0.388985332300396));
#190916=CARTESIAN_POINT('Ctrl Pts',(11.1746952154362,15.2,-0.390379802795634));
#190917=CARTESIAN_POINT('Ctrl Pts',(11.1777668919919,15.2,-0.391774273037542));
#190918=CARTESIAN_POINT('Ctrl Pts',(11.1808436140308,15.2,-0.393175430720772));
#190919=CARTESIAN_POINT('Ctrl Pts',(11.1839253355859,15.2,-0.394583286420206));
#190920=CARTESIAN_POINT('Ctrl Pts',(11.187007057141,15.2,-0.395991142119639));
#190921=CARTESIAN_POINT('Ctrl Pts',(11.1900937785343,15.2,-0.397405696546413));
#190922=CARTESIAN_POINT('Ctrl Pts',(11.1931854545194,15.2,-0.398826960251261));
#190923=CARTESIAN_POINT('Ctrl Pts',(11.1962771305045,15.2,-0.400248223956108));
#190924=CARTESIAN_POINT('Ctrl Pts',(11.1993737599957,15.2,-0.401676197327638));
#190925=CARTESIAN_POINT('Ctrl Pts',(11.2024752990221,15.2,-0.403110891448664));
#190926=CARTESIAN_POINT('Ctrl Pts',(11.2076445309205,15.2,-0.405502048403918));
#190927=CARTESIAN_POINT('Ctrl Pts',(11.2128273990221,15.2,-0.407911872788857));
#190928=CARTESIAN_POINT('Ctrl Pts',(11.2180236959666,15.2,-0.410340417233299));
#190929=CARTESIAN_POINT('Ctrl Pts',(11.2221807337487,15.2,-0.412283252894736));
#190930=CARTESIAN_POINT('Ctrl Pts',(11.226346364829,15.2,-0.414238067585351));
#190931=CARTESIAN_POINT('Ctrl Pts',(11.2305204852241,15.2,-0.416204887804882));
#190932=CARTESIAN_POINT('Ctrl Pts',(11.2346946050503,15.2,-0.418171707756433));
#190933=CARTESIAN_POINT('Ctrl Pts',(11.2388772141984,15.2,-0.420150531452363));
#190934=CARTESIAN_POINT('Ctrl Pts',(11.2430682067637,15.2,-0.422141384965282));
#190935=CARTESIAN_POINT('Ctrl Pts',(11.2472591999,15.2,-0.424132238749455));
#190936=CARTESIAN_POINT('Ctrl Pts',(11.2514585765911,15.2,-0.426135121996156));
#190937=CARTESIAN_POINT('Ctrl Pts',(11.2556662324879,15.2,-0.428150058329414));
#190938=CARTESIAN_POINT('Ctrl Pts',(11.2588219741238,15.2,-0.42966126044209));
#190939=CARTESIAN_POINT('Ctrl Pts',(11.2619823732762,15.2,-0.431179242571089));
#190940=CARTESIAN_POINT('Ctrl Pts',(11.2651473863283,15.2,-0.432704014682948));
#190941=CARTESIAN_POINT('Ctrl Pts',(11.2683123993804,15.2,-0.434228786794806));
#190942=CARTESIAN_POINT('Ctrl Pts',(11.2714820257037,15.2,-0.43576034866691));
#190943=CARTESIAN_POINT('Ctrl Pts',(11.2746562223111,15.2,-0.437298710243033));
#190944=CARTESIAN_POINT('Ctrl Pts',(11.2778304189186,15.2,-0.438837071819156));
#190945=CARTESIAN_POINT('Ctrl Pts',(11.2810091860649,15.2,-0.440382231914597));
#190946=CARTESIAN_POINT('Ctrl Pts',(11.2841924797137,15.2,-0.441934201990225));
#190947=CARTESIAN_POINT('Ctrl Pts',(11.2884368716309,15.2,-0.444003495612356));
#190948=CARTESIAN_POINT('Ctrl Pts',(11.2926893109079,15.2,-0.44608489472415));
#190949=CARTESIAN_POINT('Ctrl Pts',(11.2969496966965,15.2,-0.448178421117267));
#190950=CARTESIAN_POINT('Ctrl Pts',(11.3001449857477,15.2,-0.449748565769483));
#190951=CARTESIAN_POINT('Ctrl Pts',(11.303344744782,15.2,-0.451325532279665));
#190952=CARTESIAN_POINT('Ctrl Pts',(11.3065489298742,15.2,-0.452909329889383));
#190953=CARTESIAN_POINT('Ctrl Pts',(11.3097531149665,15.2,-0.454493127499101));
#190954=CARTESIAN_POINT('Ctrl Pts',(11.3129617262,15.2,-0.456083755857998));
#190955=CARTESIAN_POINT('Ctrl Pts',(11.3161747227499,15.2,-0.457681224008297));
#190956=CARTESIAN_POINT('Ctrl Pts',(11.3193877192999,15.2,-0.459278692158597));
#190957=CARTESIAN_POINT('Ctrl Pts',(11.3226050997162,15.2,-0.4608830011336));
#190958=CARTESIAN_POINT('Ctrl Pts',(11.3258268213905,15.2,-0.462494158324467));
#190959=CARTESIAN_POINT('Ctrl Pts',(11.3301224506797,15.2,-0.464642368107419));
#190960=CARTESIAN_POINT('Ctrl Pts',(11.3344258007579,15.2,-0.466802754745619));
#190961=CARTESIAN_POINT('Ctrl Pts',(11.3387367688755,15.2,-0.468975337806954));
#190962=CARTESIAN_POINT('Ctrl Pts',(11.3419699946701,15.2,-0.470604774954949));
#190963=CARTESIAN_POINT('Ctrl Pts',(11.3452075057374,15.2,-0.472241072138293));
#190964=CARTESIAN_POINT('Ctrl Pts',(11.3484492608283,15.2,-0.47388423916252));
#190965=CARTESIAN_POINT('Ctrl Pts',(11.3516910159192,15.2,-0.475527406186747));
#190966=CARTESIAN_POINT('Ctrl Pts',(11.3549370144347,15.2,-0.477177442210163));
#190967=CARTESIAN_POINT('Ctrl Pts',(11.3581872154832,15.2,-0.478834355816626));
#190968=CARTESIAN_POINT('Ctrl Pts',(11.3614374165318,15.2,-0.480491269423089));
#190969=CARTESIAN_POINT('Ctrl Pts',(11.3646918192969,15.2,-0.482155060945944));
#190970=CARTESIAN_POINT('Ctrl Pts',(11.3679503829281,15.2,-0.483825738551313));
#190971=CARTESIAN_POINT('Ctrl Pts',(11.3712089465594,15.2,-0.485496416156681));
#190972=CARTESIAN_POINT('Ctrl Pts',(11.3744716712572,15.2,-0.487173978935321));
#190973=CARTESIAN_POINT('Ctrl Pts',(11.3777385150929,15.2,-0.488858436124135));
#190974=CARTESIAN_POINT('Ctrl Pts',(11.3810053589286,15.2,-0.490542893312949));
#190975=CARTESIAN_POINT('Ctrl Pts',(11.3842763221555,15.2,-0.492234245292398));
#190976=CARTESIAN_POINT('Ctrl Pts',(11.3875513632443,15.2,-0.49393249889642));
#190977=CARTESIAN_POINT('Ctrl Pts',(11.390826404928,15.2,-0.495630752808959));
#190978=CARTESIAN_POINT('Ctrl Pts',(11.394105523788,15.2,-0.497335909390109));
#190979=CARTESIAN_POINT('Ctrl Pts',(11.3973886809323,15.2,-0.499047974889869));
#190980=CARTESIAN_POINT('Ctrl Pts',(11.4017662227974,15.2,-0.501330728371175));
#190981=CARTESIAN_POINT('Ctrl Pts',(11.4061509424338,15.2,-0.503625766992553));
#190982=CARTESIAN_POINT('Ctrl Pts',(11.4105427444076,15.2,-0.505933107636456));
#190983=CARTESIAN_POINT('Ctrl Pts',(11.4160324973237,15.2,-0.508817283677116));
#190984=CARTESIAN_POINT('Ctrl Pts',(11.4215333146442,15.2,-0.51172068206293));
#190985=CARTESIAN_POINT('Ctrl Pts',(11.4270450034886,15.2,-0.514643339715044));
#190986=CARTESIAN_POINT('Ctrl Pts',(11.4303520166751,15.2,-0.516396934242598));
#190987=CARTESIAN_POINT('Ctrl Pts',(11.4336629438595,15.2,-0.518157461538919));
#190988=CARTESIAN_POINT('Ctrl Pts',(11.4369777481137,15.2,-0.519924928099095));
#190989=CARTESIAN_POINT('Ctrl Pts',(11.4402925523679,15.2,-0.521692394659271));
#190990=CARTESIAN_POINT('Ctrl Pts',(11.4436112351968,15.2,-0.523466801110638));
#190991=CARTESIAN_POINT('Ctrl Pts',(11.4469337572423,15.2,-0.525248154128306));
#190992=CARTESIAN_POINT('Ctrl Pts',(11.4502562798913,15.2,-0.527029507469586));
#190993=CARTESIAN_POINT('Ctrl Pts',(11.4535826417247,15.2,-0.528817805796141));
#190994=CARTESIAN_POINT('Ctrl Pts',(11.4569127942509,15.2,-0.530613060641335));
#190995=CARTESIAN_POINT('Ctrl Pts',(11.4624630470496,15.2,-0.533605151289005));
#190996=CARTESIAN_POINT('Ctrl Pts',(11.4680238153293,15.2,-0.536616564596594));
#190997=CARTESIAN_POINT('Ctrl Pts',(11.4735949393046,15.2,-0.539647326903549));
#190998=CARTESIAN_POINT('Ctrl Pts',(11.4780518392134,15.2,-0.542071937145537));
#190999=CARTESIAN_POINT('Ctrl Pts',(11.4825153677325,15.2,-0.54450892420966));
#191000=CARTESIAN_POINT('Ctrl Pts',(11.4869855309999,15.2,-0.546958306000014));
#191001=CARTESIAN_POINT('Origin',(-5.66257110645729E-14,15.2,-1.77635683940025E-14));
#191002=CARTESIAN_POINT('',(10.3708900234023,15.2,0.29200192900193));
#191003=CARTESIAN_POINT('',(10.3708900234023,12.2,0.292001929001926));
#191004=CARTESIAN_POINT('',(10.3708900229999,15.2,0.292001928999985));
#191005=CARTESIAN_POINT('Origin',(-5.66257110645729E-14,12.2,-1.77635683940025E-14));
#191006=CARTESIAN_POINT('Origin',(-5.66257110645729E-14,15.2,-1.77635683940025E-14));
#191007=CARTESIAN_POINT('Origin',(-5.66257110645729E-14,15.2,-1.77635683940025E-14));
#191008=CARTESIAN_POINT('',(11.4780040719999,15.2,0.710930734999984));
#191009=CARTESIAN_POINT('',(11.4479048649999,15.2,1.09337742899998));
#191010=CARTESIAN_POINT('Origin',(-5.66257110645729E-14,15.2,-1.77635683940025E-14));
#191011=CARTESIAN_POINT('',(11.4479048649999,12.2,1.09337742899998));
#191012=CARTESIAN_POINT('',(11.4479048649999,15.2,1.09337742899998));
#191013=CARTESIAN_POINT('',(11.4780040719999,12.2,0.710930734999984));
#191014=CARTESIAN_POINT('Origin',(-5.66257110645729E-14,12.2,-1.77635683940025E-14));
#191015=CARTESIAN_POINT('',(11.4780040719999,15.2,0.710930734999984));
#191016=CARTESIAN_POINT('Ctrl Pts',(11.4479048649999,15.2,1.09337742899998));
#191017=CARTESIAN_POINT('Ctrl Pts',(11.4479048649999,11.6,1.09337742899998));
#191018=CARTESIAN_POINT('Ctrl Pts',(11.4471888789999,15.2,1.09364567099998));
#191019=CARTESIAN_POINT('Ctrl Pts',(11.4471888789999,11.6,1.09364567099998));
#191020=CARTESIAN_POINT('Ctrl Pts',(11.4457572179999,15.2,1.09418172899999));
#191021=CARTESIAN_POINT('Ctrl Pts',(11.4457572179999,11.6,1.09418172899999));
#191022=CARTESIAN_POINT('Ctrl Pts',(11.4436106639999,15.2,1.09498454299999));
#191023=CARTESIAN_POINT('Ctrl Pts',(11.4436106639999,11.6,1.09498454299999));
#191024=CARTESIAN_POINT('Ctrl Pts',(11.4407504639999,15.2,1.09605241699999));
#191025=CARTESIAN_POINT('Ctrl Pts',(11.4407504639999,11.6,1.09605241699999));
#191026=CARTESIAN_POINT('Ctrl Pts',(11.4371783349999,15.2,1.09738301699998));
#191027=CARTESIAN_POINT('Ctrl Pts',(11.4371783349999,11.6,1.09738301699998));
#191028=CARTESIAN_POINT('Ctrl Pts',(11.4336093279999,15.2,1.09870937299998));
#191029=CARTESIAN_POINT('Ctrl Pts',(11.4336093279999,11.6,1.09870937299998));
#191030=CARTESIAN_POINT('Ctrl Pts',(11.4300434449999,15.2,1.10003148899999));
#191031=CARTESIAN_POINT('Ctrl Pts',(11.4300434449999,11.6,1.10003148899999));
#191032=CARTESIAN_POINT('Ctrl Pts',(11.4264806909999,15.2,1.10134936399998));
#191033=CARTESIAN_POINT('Ctrl Pts',(11.4264806909999,11.6,1.10134936399998));
#191034=CARTESIAN_POINT('Ctrl Pts',(11.4229210689999,15.2,1.10266299899999));
#191035=CARTESIAN_POINT('Ctrl Pts',(11.4229210689999,11.6,1.10266299899999));
#191036=CARTESIAN_POINT('Ctrl Pts',(11.4193645909999,15.2,1.10397239899998));
#191037=CARTESIAN_POINT('Ctrl Pts',(11.4193645909999,11.6,1.10397239899998));
#191038=CARTESIAN_POINT('Ctrl Pts',(11.4158112619999,15.2,1.10527756499998));
#191039=CARTESIAN_POINT('Ctrl Pts',(11.4158112619999,11.6,1.10527756499998));
#191040=CARTESIAN_POINT('Ctrl Pts',(11.4122610939999,15.2,1.10657849999999));
#191041=CARTESIAN_POINT('Ctrl Pts',(11.4122610939999,11.6,1.10657849999999));
#191042=CARTESIAN_POINT('Ctrl Pts',(11.4087140989999,15.2,1.10787520999999));
#191043=CARTESIAN_POINT('Ctrl Pts',(11.4087140989999,11.6,1.10787520999999));
#191044=CARTESIAN_POINT('Ctrl Pts',(11.4051702859999,15.2,1.10916769599998));
#191045=CARTESIAN_POINT('Ctrl Pts',(11.4051702859999,11.6,1.10916769599998));
#191046=CARTESIAN_POINT('Ctrl Pts',(11.4016296639999,15.2,1.11045596299999));
#191047=CARTESIAN_POINT('Ctrl Pts',(11.4016296639999,11.6,1.11045596299999));
#191048=CARTESIAN_POINT('Ctrl Pts',(11.3980922449999,15.2,1.11174001299998));
#191049=CARTESIAN_POINT('Ctrl Pts',(11.3980922449999,11.6,1.11174001299998));
#191050=CARTESIAN_POINT('Ctrl Pts',(11.3945580339999,15.2,1.11301984899999));
#191051=CARTESIAN_POINT('Ctrl Pts',(11.3945580339999,11.6,1.11301984899998));
#191052=CARTESIAN_POINT('Ctrl Pts',(11.3910270409999,15.2,1.11429547399998));
#191053=CARTESIAN_POINT('Ctrl Pts',(11.3910270409999,11.6,1.11429547399998));
#191054=CARTESIAN_POINT('Ctrl Pts',(11.3874992709999,15.2,1.11556689099999));
#191055=CARTESIAN_POINT('Ctrl Pts',(11.3874992709999,11.6,1.11556689099999));
#191056=CARTESIAN_POINT('Ctrl Pts',(11.3839747349999,15.2,1.11683410099999));
#191057=CARTESIAN_POINT('Ctrl Pts',(11.3839747349999,11.6,1.11683410099999));
#191058=CARTESIAN_POINT('Ctrl Pts',(11.3804534399999,15.2,1.11809710599998));
#191059=CARTESIAN_POINT('Ctrl Pts',(11.3804534399999,11.6,1.11809710599998));
#191060=CARTESIAN_POINT('Ctrl Pts',(11.3769353939999,15.2,1.11935591199999));
#191061=CARTESIAN_POINT('Ctrl Pts',(11.3769353939999,11.6,1.11935591199999));
#191062=CARTESIAN_POINT('Ctrl Pts',(11.3734206059999,15.2,1.12061051999999));
#191063=CARTESIAN_POINT('Ctrl Pts',(11.3734206059999,11.6,1.12061051999999));
#191064=CARTESIAN_POINT('Ctrl Pts',(11.3699090849999,15.2,1.12186093299998));
#191065=CARTESIAN_POINT('Ctrl Pts',(11.3699090849999,11.6,1.12186093299998));
#191066=CARTESIAN_POINT('Ctrl Pts',(11.3664008399999,15.2,1.12310715499999));
#191067=CARTESIAN_POINT('Ctrl Pts',(11.3664008399999,11.6,1.12310715499999));
#191068=CARTESIAN_POINT('Ctrl Pts',(11.3628958789999,15.2,1.12434918799998));
#191069=CARTESIAN_POINT('Ctrl Pts',(11.3628958789999,11.6,1.12434918799998));
#191070=CARTESIAN_POINT('Ctrl Pts',(11.3593942139999,15.2,1.12558703499999));
#191071=CARTESIAN_POINT('Ctrl Pts',(11.3593942139999,11.6,1.12558703499999));
#191072=CARTESIAN_POINT('Ctrl Pts',(11.3558958509999,15.2,1.12682069999999));
#191073=CARTESIAN_POINT('Ctrl Pts',(11.3558958509999,11.6,1.12682069999999));
#191074=CARTESIAN_POINT('Ctrl Pts',(11.3524007989999,15.2,1.12805018499999));
#191075=CARTESIAN_POINT('Ctrl Pts',(11.3524007989999,11.6,1.12805018499999));
#191076=CARTESIAN_POINT('Ctrl Pts',(11.3489090669999,15.2,1.12927549499998));
#191077=CARTESIAN_POINT('Ctrl Pts',(11.3489090669999,11.6,1.12927549499998));
#191078=CARTESIAN_POINT('Ctrl Pts',(11.3454206639999,15.2,1.13049662999999));
#191079=CARTESIAN_POINT('Ctrl Pts',(11.3454206639999,11.6,1.13049662999999));
#191080=CARTESIAN_POINT('Ctrl Pts',(11.3419355979999,15.2,1.13171359399999));
#191081=CARTESIAN_POINT('Ctrl Pts',(11.3419355979999,11.6,1.13171359399999));
#191082=CARTESIAN_POINT('Ctrl Pts',(11.3384538779999,15.2,1.13292639099999));
#191083=CARTESIAN_POINT('Ctrl Pts',(11.3384538779999,11.6,1.13292639099999));
#191084=CARTESIAN_POINT('Ctrl Pts',(11.3349755119999,15.2,1.13413502399998));
#191085=CARTESIAN_POINT('Ctrl Pts',(11.3349755119999,11.6,1.13413502399998));
#191086=CARTESIAN_POINT('Ctrl Pts',(11.3315005099999,15.2,1.13533949399999));
#191087=CARTESIAN_POINT('Ctrl Pts',(11.3315005099999,11.6,1.13533949399998));
#191088=CARTESIAN_POINT('Ctrl Pts',(11.3280288789999,15.2,1.13653980499999));
#191089=CARTESIAN_POINT('Ctrl Pts',(11.3280288789999,11.6,1.13653980499999));
#191090=CARTESIAN_POINT('Ctrl Pts',(11.3245606299999,15.2,1.13773596199998));
#191091=CARTESIAN_POINT('Ctrl Pts',(11.3245606299999,11.6,1.13773596199998));
#191092=CARTESIAN_POINT('Ctrl Pts',(11.3210957719999,15.2,1.13892796799998));
#191093=CARTESIAN_POINT('Ctrl Pts',(11.3210957719999,11.6,1.13892796799998));
#191094=CARTESIAN_POINT('Ctrl Pts',(11.3176343119999,15.2,1.14011582299999));
#191095=CARTESIAN_POINT('Ctrl Pts',(11.3176343119999,11.6,1.14011582299998));
#191096=CARTESIAN_POINT('Ctrl Pts',(11.3141762599999,15.2,1.14129953199999));
#191097=CARTESIAN_POINT('Ctrl Pts',(11.3141762599999,11.6,1.14129953199999));
#191098=CARTESIAN_POINT('Ctrl Pts',(11.3107216239999,15.2,1.14247909899999));
#191099=CARTESIAN_POINT('Ctrl Pts',(11.3107216239999,11.6,1.14247909899999));
#191100=CARTESIAN_POINT('Ctrl Pts',(11.3072704139999,15.2,1.14365452599999));
#191101=CARTESIAN_POINT('Ctrl Pts',(11.3072704139999,11.6,1.14365452599999));
#191102=CARTESIAN_POINT('Ctrl Pts',(11.3038226389999,15.2,1.14482581599999));
#191103=CARTESIAN_POINT('Ctrl Pts',(11.3038226389999,11.6,1.14482581599999));
#191104=CARTESIAN_POINT('Ctrl Pts',(11.3003783059999,15.2,1.14599297299999));
#191105=CARTESIAN_POINT('Ctrl Pts',(11.3003783059999,11.6,1.14599297299998));
#191106=CARTESIAN_POINT('Ctrl Pts',(11.2969374249999,15.2,1.14715599999998));
#191107=CARTESIAN_POINT('Ctrl Pts',(11.2969374249999,11.6,1.14715599999998));
#191108=CARTESIAN_POINT('Ctrl Pts',(11.2935000059999,15.2,1.14831489899998));
#191109=CARTESIAN_POINT('Ctrl Pts',(11.2935000059999,11.6,1.14831489899998));
#191110=CARTESIAN_POINT('Ctrl Pts',(11.2900660559999,15.2,1.14946967499999));
#191111=CARTESIAN_POINT('Ctrl Pts',(11.2900660559999,11.6,1.14946967499999));
#191112=CARTESIAN_POINT('Ctrl Pts',(11.2866355859999,15.2,1.15062032999999));
#191113=CARTESIAN_POINT('Ctrl Pts',(11.2866355859999,11.6,1.15062032999999));
#191114=CARTESIAN_POINT('Ctrl Pts',(11.2832086039999,15.2,1.15176686799999));
#191115=CARTESIAN_POINT('Ctrl Pts',(11.2832086039999,11.6,1.15176686799999));
#191116=CARTESIAN_POINT('Ctrl Pts',(11.2797851169999,15.2,1.15290929199999));
#191117=CARTESIAN_POINT('Ctrl Pts',(11.2797851169999,11.6,1.15290929199999));
#191118=CARTESIAN_POINT('Ctrl Pts',(11.2763651379999,15.2,1.15404760499999));
#191119=CARTESIAN_POINT('Ctrl Pts',(11.2763651379999,11.6,1.15404760499999));
#191120=CARTESIAN_POINT('Ctrl Pts',(11.2729486729999,15.2,1.15518180999999));
#191121=CARTESIAN_POINT('Ctrl Pts',(11.2729486729999,11.6,1.15518180999999));
#191122=CARTESIAN_POINT('Ctrl Pts',(11.2695357319999,15.2,1.15631191099999));
#191123=CARTESIAN_POINT('Ctrl Pts',(11.2695357319999,11.6,1.15631191099998));
#191124=CARTESIAN_POINT('Ctrl Pts',(11.2661263239999,15.2,1.15743791099999));
#191125=CARTESIAN_POINT('Ctrl Pts',(11.2661263239999,11.6,1.15743791099999));
#191126=CARTESIAN_POINT('Ctrl Pts',(11.2627204589999,15.2,1.15855981299998));
#191127=CARTESIAN_POINT('Ctrl Pts',(11.2627204589999,11.6,1.15855981299998));
#191128=CARTESIAN_POINT('Ctrl Pts',(11.2593181439999,15.2,1.15967762199999));
#191129=CARTESIAN_POINT('Ctrl Pts',(11.2593181439999,11.6,1.15967762199999));
#191130=CARTESIAN_POINT('Ctrl Pts',(11.2559193889999,15.2,1.16079133899999));
#191131=CARTESIAN_POINT('Ctrl Pts',(11.2559193889999,11.6,1.16079133899999));
#191132=CARTESIAN_POINT('Ctrl Pts',(11.2525242039999,15.2,1.16190096799999));
#191133=CARTESIAN_POINT('Ctrl Pts',(11.2525242039999,11.6,1.16190096799999));
#191134=CARTESIAN_POINT('Ctrl Pts',(11.2491325969999,15.2,1.16300651299999));
#191135=CARTESIAN_POINT('Ctrl Pts',(11.2491325969999,11.6,1.16300651299999));
#191136=CARTESIAN_POINT('Ctrl Pts',(11.2457445769999,15.2,1.16410797799999));
#191137=CARTESIAN_POINT('Ctrl Pts',(11.2457445769999,11.6,1.16410797799999));
#191138=CARTESIAN_POINT('Ctrl Pts',(11.2423601539999,15.2,1.16520536499999));
#191139=CARTESIAN_POINT('Ctrl Pts',(11.2423601539999,11.6,1.16520536499999));
#191140=CARTESIAN_POINT('Ctrl Pts',(11.2389793369999,15.2,1.16629867799999));
#191141=CARTESIAN_POINT('Ctrl Pts',(11.2389793369999,11.6,1.16629867799999));
#191142=CARTESIAN_POINT('Ctrl Pts',(11.2356021349999,15.2,1.16738791999999));
#191143=CARTESIAN_POINT('Ctrl Pts',(11.2356021349999,11.6,1.16738791999999));
#191144=CARTESIAN_POINT('Ctrl Pts',(11.2322285569999,15.2,1.16847309399999));
#191145=CARTESIAN_POINT('Ctrl Pts',(11.2322285569999,11.6,1.16847309399999));
#191146=CARTESIAN_POINT('Ctrl Pts',(11.2288586119999,15.2,1.16955420599998));
#191147=CARTESIAN_POINT('Ctrl Pts',(11.2288586119999,11.6,1.16955420599998));
#191148=CARTESIAN_POINT('Ctrl Pts',(11.2254923089999,15.2,1.17063125699998));
#191149=CARTESIAN_POINT('Ctrl Pts',(11.2254923089999,11.6,1.17063125699998));
#191150=CARTESIAN_POINT('Ctrl Pts',(11.2221296589999,15.2,1.17170425099999));
#191151=CARTESIAN_POINT('Ctrl Pts',(11.2221296589999,11.6,1.17170425099998));
#191152=CARTESIAN_POINT('Ctrl Pts',(11.2187706689999,15.2,1.17277319199999));
#191153=CARTESIAN_POINT('Ctrl Pts',(11.2187706689999,11.6,1.17277319199998));
#191154=CARTESIAN_POINT('Ctrl Pts',(11.2154153489999,15.2,1.17383808299998));
#191155=CARTESIAN_POINT('Ctrl Pts',(11.2154153489999,11.6,1.17383808299998));
#191156=CARTESIAN_POINT('Ctrl Pts',(11.2120637079999,15.2,1.17489892799998));
#191157=CARTESIAN_POINT('Ctrl Pts',(11.2120637079999,11.6,1.17489892799998));
#191158=CARTESIAN_POINT('Ctrl Pts',(11.2087157559999,15.2,1.17595572999999));
#191159=CARTESIAN_POINT('Ctrl Pts',(11.2087157559999,11.6,1.17595572999999));
#191160=CARTESIAN_POINT('Ctrl Pts',(11.2053715019999,15.2,1.17700849199998));
#191161=CARTESIAN_POINT('Ctrl Pts',(11.2053715019999,11.6,1.17700849199998));
#191162=CARTESIAN_POINT('Ctrl Pts',(11.2020309559999,15.2,1.17805721999999));
#191163=CARTESIAN_POINT('Ctrl Pts',(11.2020309559999,11.6,1.17805721999999));
#191164=CARTESIAN_POINT('Ctrl Pts',(11.1986941249999,15.2,1.17910191499998));
#191165=CARTESIAN_POINT('Ctrl Pts',(11.1986941249999,11.6,1.17910191499998));
#191166=CARTESIAN_POINT('Ctrl Pts',(11.1953610209999,15.2,1.18014258099999));
#191167=CARTESIAN_POINT('Ctrl Pts',(11.1953610209999,11.6,1.18014258099999));
#191168=CARTESIAN_POINT('Ctrl Pts',(11.1920316519999,15.2,1.18117922199998));
#191169=CARTESIAN_POINT('Ctrl Pts',(11.1920316519999,11.6,1.18117922199998));
#191170=CARTESIAN_POINT('Ctrl Pts',(11.1887060269999,15.2,1.18221184299999));
#191171=CARTESIAN_POINT('Ctrl Pts',(11.1887060269999,11.6,1.18221184299998));
#191172=CARTESIAN_POINT('Ctrl Pts',(11.1853841569999,15.2,1.18324044599999));
#191173=CARTESIAN_POINT('Ctrl Pts',(11.1853841569999,11.6,1.18324044599999));
#191174=CARTESIAN_POINT('Ctrl Pts',(11.1820660499999,15.2,1.18426503499999));
#191175=CARTESIAN_POINT('Ctrl Pts',(11.1820660499999,11.6,1.18426503499998));
#191176=CARTESIAN_POINT('Ctrl Pts',(11.1787517149999,15.2,1.18528561399998));
#191177=CARTESIAN_POINT('Ctrl Pts',(11.1787517149999,11.6,1.18528561399998));
#191178=CARTESIAN_POINT('Ctrl Pts',(11.1754411629999,15.2,1.18630218499999));
#191179=CARTESIAN_POINT('Ctrl Pts',(11.1754411629999,11.6,1.18630218499999));
#191180=CARTESIAN_POINT('Ctrl Pts',(11.1721344009999,15.2,1.18731475499999));
#191181=CARTESIAN_POINT('Ctrl Pts',(11.1721344009999,11.6,1.18731475499999));
#191182=CARTESIAN_POINT('Ctrl Pts',(11.1688314409999,15.2,1.18832332399998));
#191183=CARTESIAN_POINT('Ctrl Pts',(11.1688314409999,11.6,1.18832332399998));
#191184=CARTESIAN_POINT('Ctrl Pts',(11.1655322919999,15.2,1.18932789899999));
#191185=CARTESIAN_POINT('Ctrl Pts',(11.1655322919999,11.6,1.18932789899999));
#191186=CARTESIAN_POINT('Ctrl Pts',(11.1622369629999,15.2,1.19032848099998));
#191187=CARTESIAN_POINT('Ctrl Pts',(11.1622369629999,11.6,1.19032848099998));
#191188=CARTESIAN_POINT('Ctrl Pts',(11.1589454619999,15.2,1.19132507599998));
#191189=CARTESIAN_POINT('Ctrl Pts',(11.1589454619999,11.6,1.19132507599998));
#191190=CARTESIAN_POINT('Ctrl Pts',(11.1556577999999,15.2,1.19231768599999));
#191191=CARTESIAN_POINT('Ctrl Pts',(11.1556577999999,11.6,1.19231768599999));
#191192=CARTESIAN_POINT('Ctrl Pts',(11.1523739879999,15.2,1.19330631599999));
#191193=CARTESIAN_POINT('Ctrl Pts',(11.1523739879999,11.6,1.19330631599999));
#191194=CARTESIAN_POINT('Ctrl Pts',(11.1490940329999,15.2,1.19429096899998));
#191195=CARTESIAN_POINT('Ctrl Pts',(11.1490940329999,11.6,1.19429096899998));
#191196=CARTESIAN_POINT('Ctrl Pts',(11.1458179459999,15.2,1.19527164899999));
#191197=CARTESIAN_POINT('Ctrl Pts',(11.1458179459999,11.6,1.19527164899999));
#191198=CARTESIAN_POINT('Ctrl Pts',(11.1425457349999,15.2,1.19624835999999));
#191199=CARTESIAN_POINT('Ctrl Pts',(11.1425457349999,11.6,1.19624835999998));
#191200=CARTESIAN_POINT('Ctrl Pts',(11.1392774109999,15.2,1.19722110599998));
#191201=CARTESIAN_POINT('Ctrl Pts',(11.1392774109999,11.6,1.19722110599998));
#191202=CARTESIAN_POINT('Ctrl Pts',(11.1360129839999,15.2,1.19818988999999));
#191203=CARTESIAN_POINT('Ctrl Pts',(11.1360129839999,11.6,1.19818988999999));
#191204=CARTESIAN_POINT('Ctrl Pts',(11.1327524619999,15.2,1.19915471699999));
#191205=CARTESIAN_POINT('Ctrl Pts',(11.1327524619999,11.6,1.19915471699999));
#191206=CARTESIAN_POINT('Ctrl Pts',(11.1294958549999,15.2,1.20011559099999));
#191207=CARTESIAN_POINT('Ctrl Pts',(11.1294958549999,11.6,1.20011559099999));
#191208=CARTESIAN_POINT('Ctrl Pts',(11.1262431739999,15.2,1.20107251499999));
#191209=CARTESIAN_POINT('Ctrl Pts',(11.1262431739999,11.6,1.20107251499999));
#191210=CARTESIAN_POINT('Ctrl Pts',(11.1229944269999,15.2,1.20202549299998));
#191211=CARTESIAN_POINT('Ctrl Pts',(11.1229944269999,11.6,1.20202549299998));
#191212=CARTESIAN_POINT('Ctrl Pts',(11.1197496249999,15.2,1.20297452899999));
#191213=CARTESIAN_POINT('Ctrl Pts',(11.1197496249999,11.6,1.20297452899999));
#191214=CARTESIAN_POINT('Ctrl Pts',(11.1165087779999,15.2,1.20391962699999));
#191215=CARTESIAN_POINT('Ctrl Pts',(11.1165087779999,11.6,1.20391962699998));
#191216=CARTESIAN_POINT('Ctrl Pts',(11.1132718939999,15.2,1.20486079099999));
#191217=CARTESIAN_POINT('Ctrl Pts',(11.1132718939999,11.6,1.20486079099999));
#191218=CARTESIAN_POINT('Ctrl Pts',(11.1100389819999,15.2,1.20579802499998));
#191219=CARTESIAN_POINT('Ctrl Pts',(11.1100389819999,11.6,1.20579802499998));
#191220=CARTESIAN_POINT('Ctrl Pts',(11.1068100549999,15.2,1.20673133399999));
#191221=CARTESIAN_POINT('Ctrl Pts',(11.1068100549999,11.6,1.20673133399999));
#191222=CARTESIAN_POINT('Ctrl Pts',(11.1035851209999,15.2,1.20766071999999));
#191223=CARTESIAN_POINT('Ctrl Pts',(11.1035851209999,11.6,1.20766071999999));
#191224=CARTESIAN_POINT('Ctrl Pts',(11.1003641889999,15.2,1.20858618799998));
#191225=CARTESIAN_POINT('Ctrl Pts',(11.1003641889999,11.6,1.20858618799998));
#191226=CARTESIAN_POINT('Ctrl Pts',(11.0971472699999,15.2,1.20950774199999));
#191227=CARTESIAN_POINT('Ctrl Pts',(11.0971472699999,11.6,1.20950774199999));
#191228=CARTESIAN_POINT('Ctrl Pts',(11.0939343729999,15.2,1.21042538699998));
#191229=CARTESIAN_POINT('Ctrl Pts',(11.0939343729999,11.6,1.21042538699998));
#191230=CARTESIAN_POINT('Ctrl Pts',(11.0907255089999,15.2,1.21133912599999));
#191231=CARTESIAN_POINT('Ctrl Pts',(11.0907255089999,11.6,1.21133912599999));
#191232=CARTESIAN_POINT('Ctrl Pts',(11.0875206859999,15.2,1.21224896199998));
#191233=CARTESIAN_POINT('Ctrl Pts',(11.0875206859999,11.6,1.21224896199998));
#191234=CARTESIAN_POINT('Ctrl Pts',(11.0843199139999,15.2,1.21315490199999));
#191235=CARTESIAN_POINT('Ctrl Pts',(11.0843199139999,11.6,1.21315490199999));
#191236=CARTESIAN_POINT('Ctrl Pts',(11.0811232049999,15.2,1.21405694799999));
#191237=CARTESIAN_POINT('Ctrl Pts',(11.0811232049999,11.6,1.21405694799999));
#191238=CARTESIAN_POINT('Ctrl Pts',(11.0779305669999,15.2,1.21495510399999));
#191239=CARTESIAN_POINT('Ctrl Pts',(11.0779305669999,11.6,1.21495510399999));
#191240=CARTESIAN_POINT('Ctrl Pts',(11.0747420099999,15.2,1.21584937499998));
#191241=CARTESIAN_POINT('Ctrl Pts',(11.0747420099999,11.6,1.21584937499998));
#191242=CARTESIAN_POINT('Ctrl Pts',(11.0715575449999,15.2,1.21673976599999));
#191243=CARTESIAN_POINT('Ctrl Pts',(11.0715575449999,11.6,1.21673976599999));
#191244=CARTESIAN_POINT('Ctrl Pts',(11.0683771819999,15.2,1.21762627999999));
#191245=CARTESIAN_POINT('Ctrl Pts',(11.0683771819999,11.6,1.21762627999999));
#191246=CARTESIAN_POINT('Ctrl Pts',(11.0652009289999,15.2,1.21850892099999));
#191247=CARTESIAN_POINT('Ctrl Pts',(11.0652009289999,11.6,1.21850892099999));
#191248=CARTESIAN_POINT('Ctrl Pts',(11.0620287979999,15.2,1.21938769199998));
#191249=CARTESIAN_POINT('Ctrl Pts',(11.0620287979999,11.6,1.21938769199998));
#191250=CARTESIAN_POINT('Ctrl Pts',(11.0588607969999,15.2,1.22026260099998));
#191251=CARTESIAN_POINT('Ctrl Pts',(11.0588607969999,11.6,1.22026260099998));
#191252=CARTESIAN_POINT('Ctrl Pts',(11.0556969379999,15.2,1.22113364899999));
#191253=CARTESIAN_POINT('Ctrl Pts',(11.0556969379999,11.6,1.22113364899999));
#191254=CARTESIAN_POINT('Ctrl Pts',(11.0525372299999,15.2,1.22200084099998));
#191255=CARTESIAN_POINT('Ctrl Pts',(11.0525372299999,11.6,1.22200084099998));
#191256=CARTESIAN_POINT('Ctrl Pts',(11.0493816829999,15.2,1.22286418199999));
#191257=CARTESIAN_POINT('Ctrl Pts',(11.0493816829999,11.6,1.22286418199998));
#191258=CARTESIAN_POINT('Ctrl Pts',(11.0462303079999,15.2,1.22372367599999));
#191259=CARTESIAN_POINT('Ctrl Pts',(11.0462303079999,11.6,1.22372367599999));
#191260=CARTESIAN_POINT('Ctrl Pts',(11.0430831139999,15.2,1.22457932799998));
#191261=CARTESIAN_POINT('Ctrl Pts',(11.0430831139999,11.6,1.22457932799998));
#191262=CARTESIAN_POINT('Ctrl Pts',(11.0399401109999,15.2,1.22543113999999));
#191263=CARTESIAN_POINT('Ctrl Pts',(11.0399401109999,11.6,1.22543113999999));
#191264=CARTESIAN_POINT('Ctrl Pts',(11.0368013089999,15.2,1.22627911899999));
#191265=CARTESIAN_POINT('Ctrl Pts',(11.0368013089999,11.6,1.22627911899999));
#191266=CARTESIAN_POINT('Ctrl Pts',(11.0336667189999,15.2,1.22712326699999));
#191267=CARTESIAN_POINT('Ctrl Pts',(11.0336667189999,11.6,1.22712326699998));
#191268=CARTESIAN_POINT('Ctrl Pts',(11.0305363499999,15.2,1.22796359099999));
#191269=CARTESIAN_POINT('Ctrl Pts',(11.0305363499999,11.6,1.22796359099999));
#191270=CARTESIAN_POINT('Ctrl Pts',(11.0274102129999,15.2,1.22880009299998));
#191271=CARTESIAN_POINT('Ctrl Pts',(11.0274102129999,11.6,1.22880009299998));
#191272=CARTESIAN_POINT('Ctrl Pts',(11.0242883189999,15.2,1.22963277999999));
#191273=CARTESIAN_POINT('Ctrl Pts',(11.0242883189999,11.6,1.22963277999998));
#191274=CARTESIAN_POINT('Ctrl Pts',(11.0211706759999,15.2,1.23046165299999));
#191275=CARTESIAN_POINT('Ctrl Pts',(11.0211706759999,11.6,1.23046165299999));
#191276=CARTESIAN_POINT('Ctrl Pts',(11.0180572959999,15.2,1.23128671899998));
#191277=CARTESIAN_POINT('Ctrl Pts',(11.0180572959999,11.6,1.23128671899998));
#191278=CARTESIAN_POINT('Ctrl Pts',(11.0149481889999,15.2,1.23210798199999));
#191279=CARTESIAN_POINT('Ctrl Pts',(11.0149481889999,11.6,1.23210798199999));
#191280=CARTESIAN_POINT('Ctrl Pts',(11.0118433639999,15.2,1.23292544599999));
#191281=CARTESIAN_POINT('Ctrl Pts',(11.0118433639999,11.6,1.23292544599999));
#191282=CARTESIAN_POINT('Ctrl Pts',(11.0087428319999,15.2,1.23373911599999));
#191283=CARTESIAN_POINT('Ctrl Pts',(11.0087428319999,11.6,1.23373911599999));
#191284=CARTESIAN_POINT('Ctrl Pts',(11.0056466049999,15.2,1.23454899599999));
#191285=CARTESIAN_POINT('Ctrl Pts',(11.0056466049999,11.6,1.23454899599999));
#191286=CARTESIAN_POINT('Ctrl Pts',(11.0025546899999,15.2,1.23535509099999));
#191287=CARTESIAN_POINT('Ctrl Pts',(11.0025546899999,11.6,1.23535509099999));
#191288=CARTESIAN_POINT('Ctrl Pts',(10.9994670979999,15.2,1.23615740499998));
#191289=CARTESIAN_POINT('Ctrl Pts',(10.9994670979999,11.6,1.23615740499998));
#191290=CARTESIAN_POINT('Ctrl Pts',(10.9963838419999,15.2,1.23695594399999));
#191291=CARTESIAN_POINT('Ctrl Pts',(10.9963838419999,11.6,1.23695594399999));
#191292=CARTESIAN_POINT('Ctrl Pts',(10.9933049299999,15.2,1.23775071099999));
#191293=CARTESIAN_POINT('Ctrl Pts',(10.9933049299999,11.6,1.23775071099998));
#191294=CARTESIAN_POINT('Ctrl Pts',(10.9902303719999,15.2,1.23854171099998));
#191295=CARTESIAN_POINT('Ctrl Pts',(10.9902303719999,11.6,1.23854171099998));
#191296=CARTESIAN_POINT('Ctrl Pts',(10.9871601809999,15.2,1.23932894899998));
#191297=CARTESIAN_POINT('Ctrl Pts',(10.9871601809999,11.6,1.23932894899998));
#191298=CARTESIAN_POINT('Ctrl Pts',(10.9840943639999,15.2,1.24011242999998));
#191299=CARTESIAN_POINT('Ctrl Pts',(10.9840943639999,11.6,1.24011242999998));
#191300=CARTESIAN_POINT('Ctrl Pts',(10.9810329339999,15.2,1.24089215599998));
#191301=CARTESIAN_POINT('Ctrl Pts',(10.9810329339999,11.6,1.24089215599998));
#191302=CARTESIAN_POINT('Ctrl Pts',(10.9779759009999,15.2,1.24166813599999));
#191303=CARTESIAN_POINT('Ctrl Pts',(10.9779759009999,11.6,1.24166813599999));
#191304=CARTESIAN_POINT('Ctrl Pts',(10.9749232749999,15.2,1.24244037199999));
#191305=CARTESIAN_POINT('Ctrl Pts',(10.9749232749999,11.6,1.24244037199999));
#191306=CARTESIAN_POINT('Ctrl Pts',(10.9718750649999,15.2,1.24320886799998));
#191307=CARTESIAN_POINT('Ctrl Pts',(10.9718750649999,11.6,1.24320886799998));
#191308=CARTESIAN_POINT('Ctrl Pts',(10.9688312839999,15.2,1.24397363099999));
#191309=CARTESIAN_POINT('Ctrl Pts',(10.9688312839999,11.6,1.24397363099999));
#191310=CARTESIAN_POINT('Ctrl Pts',(10.9657919419999,15.2,1.24473466399999));
#191311=CARTESIAN_POINT('Ctrl Pts',(10.9657919419999,11.6,1.24473466399999));
#191312=CARTESIAN_POINT('Ctrl Pts',(10.9627570469999,15.2,1.24549197299999));
#191313=CARTESIAN_POINT('Ctrl Pts',(10.9627570469999,11.6,1.24549197299999));
#191314=CARTESIAN_POINT('Ctrl Pts',(10.9597266129999,15.2,1.24624556199999));
#191315=CARTESIAN_POINT('Ctrl Pts',(10.9597266129999,11.6,1.24624556199999));
#191316=CARTESIAN_POINT('Ctrl Pts',(10.9567006489999,15.2,1.24699543599998));
#191317=CARTESIAN_POINT('Ctrl Pts',(10.9567006489999,11.6,1.24699543599998));
#191318=CARTESIAN_POINT('Ctrl Pts',(10.9536791659999,15.2,1.24774160099999));
#191319=CARTESIAN_POINT('Ctrl Pts',(10.9536791659999,11.6,1.24774160099998));
#191320=CARTESIAN_POINT('Ctrl Pts',(10.9506621729999,15.2,1.24848405899999));
#191321=CARTESIAN_POINT('Ctrl Pts',(10.9506621729999,11.6,1.24848405899999));
#191322=CARTESIAN_POINT('Ctrl Pts',(10.9476496829999,15.2,1.24922281699998));
#191323=CARTESIAN_POINT('Ctrl Pts',(10.9476496829999,11.6,1.24922281699998));
#191324=CARTESIAN_POINT('Ctrl Pts',(10.9446417049999,15.2,1.24995787999998));
#191325=CARTESIAN_POINT('Ctrl Pts',(10.9446417049999,11.6,1.24995787999998));
#191326=CARTESIAN_POINT('Ctrl Pts',(10.9416382509999,15.2,1.25068925199999));
#191327=CARTESIAN_POINT('Ctrl Pts',(10.9416382509999,11.6,1.25068925199999));
#191328=CARTESIAN_POINT('Ctrl Pts',(10.9386393289999,15.2,1.25141693899999));
#191329=CARTESIAN_POINT('Ctrl Pts',(10.9386393289999,11.6,1.25141693899998));
#191330=CARTESIAN_POINT('Ctrl Pts',(10.9356449539999,15.2,1.25214094399999));
#191331=CARTESIAN_POINT('Ctrl Pts',(10.9356449539999,11.6,1.25214094399999));
#191332=CARTESIAN_POINT('Ctrl Pts',(10.9326551319999,15.2,1.25286127399999));
#191333=CARTESIAN_POINT('Ctrl Pts',(10.9326551319999,11.6,1.25286127399999));
#191334=CARTESIAN_POINT('Ctrl Pts',(10.9296698779999,15.2,1.25357793199999));
#191335=CARTESIAN_POINT('Ctrl Pts',(10.9296698779999,11.6,1.25357793199999));
#191336=CARTESIAN_POINT('Ctrl Pts',(10.9266891999999,15.2,1.25429092499999));
#191337=CARTESIAN_POINT('Ctrl Pts',(10.9266891999999,11.6,1.25429092499999));
#191338=CARTESIAN_POINT('Ctrl Pts',(10.9237131089999,15.2,1.25500025699999));
#191339=CARTESIAN_POINT('Ctrl Pts',(10.9237131089999,11.6,1.25500025699999));
#191340=CARTESIAN_POINT('Ctrl Pts',(10.9207416159999,15.2,1.25570593399999));
#191341=CARTESIAN_POINT('Ctrl Pts',(10.9207416159999,11.6,1.25570593399999));
#191342=CARTESIAN_POINT('Ctrl Pts',(10.9177747329999,15.2,1.25640795999999));
#191343=CARTESIAN_POINT('Ctrl Pts',(10.9177747329999,11.6,1.25640795999999));
#191344=CARTESIAN_POINT('Ctrl Pts',(10.9148124699999,15.2,1.25710633999998));
#191345=CARTESIAN_POINT('Ctrl Pts',(10.9148124699999,11.6,1.25710633999998));
#191346=CARTESIAN_POINT('Ctrl Pts',(10.9118548369999,15.2,1.25780107899998));
#191347=CARTESIAN_POINT('Ctrl Pts',(10.9118548369999,11.6,1.25780107899998));
#191348=CARTESIAN_POINT('Ctrl Pts',(10.9089018469999,15.2,1.25849218299999));
#191349=CARTESIAN_POINT('Ctrl Pts',(10.9089018469999,11.6,1.25849218299999));
#191350=CARTESIAN_POINT('Ctrl Pts',(10.9059535079999,15.2,1.25917965599998));
#191351=CARTESIAN_POINT('Ctrl Pts',(10.9059535079999,11.6,1.25917965599998));
#191352=CARTESIAN_POINT('Ctrl Pts',(10.9030098339999,15.2,1.25986350499999));
#191353=CARTESIAN_POINT('Ctrl Pts',(10.9030098339999,11.6,1.25986350499998));
#191354=CARTESIAN_POINT('Ctrl Pts',(10.9000708339999,15.2,1.26054373299999));
#191355=CARTESIAN_POINT('Ctrl Pts',(10.9000708339999,11.6,1.26054373299999));
#191356=CARTESIAN_POINT('Ctrl Pts',(10.8971365199999,15.2,1.26122034599998));
#191357=CARTESIAN_POINT('Ctrl Pts',(10.8971365199999,11.6,1.26122034599998));
#191358=CARTESIAN_POINT('Ctrl Pts',(10.8942069009999,15.2,1.26189335099999));
#191359=CARTESIAN_POINT('Ctrl Pts',(10.8942069009999,11.6,1.26189335099998));
#191360=CARTESIAN_POINT('Ctrl Pts',(10.8912819899999,15.2,1.26256274999998));
#191361=CARTESIAN_POINT('Ctrl Pts',(10.8912819899999,11.6,1.26256274999998));
#191362=CARTESIAN_POINT('Ctrl Pts',(10.8883617979999,15.2,1.26322854999998));
#191363=CARTESIAN_POINT('Ctrl Pts',(10.8883617979999,11.6,1.26322854999998));
#191364=CARTESIAN_POINT('Ctrl Pts',(10.8854463339999,15.2,1.26389075699999));
#191365=CARTESIAN_POINT('Ctrl Pts',(10.8854463339999,11.6,1.26389075699999));
#191366=CARTESIAN_POINT('Ctrl Pts',(10.8825356119999,15.2,1.26454937599998));
#191367=CARTESIAN_POINT('Ctrl Pts',(10.8825356119999,11.6,1.26454937599998));
#191368=CARTESIAN_POINT('Ctrl Pts',(10.8796296409999,15.2,1.26520441099998));
#191369=CARTESIAN_POINT('Ctrl Pts',(10.8796296409999,11.6,1.26520441099998));
#191370=CARTESIAN_POINT('Ctrl Pts',(10.8767284329999,15.2,1.26585586799999));
#191371=CARTESIAN_POINT('Ctrl Pts',(10.8767284329999,11.6,1.26585586799999));
#191372=CARTESIAN_POINT('Ctrl Pts',(10.8738319979999,15.2,1.26650375199999));
#191373=CARTESIAN_POINT('Ctrl Pts',(10.8738319979999,11.6,1.26650375199999));
#191374=CARTESIAN_POINT('Ctrl Pts',(10.8709403489999,15.2,1.26714806999999));
#191375=CARTESIAN_POINT('Ctrl Pts',(10.8709403489999,11.6,1.26714806999999));
#191376=CARTESIAN_POINT('Ctrl Pts',(10.8680534959999,15.2,1.26778882499998));
#191377=CARTESIAN_POINT('Ctrl Pts',(10.8680534959999,11.6,1.26778882499998));
#191378=CARTESIAN_POINT('Ctrl Pts',(10.8651714489999,15.2,1.26842602399998));
#191379=CARTESIAN_POINT('Ctrl Pts',(10.8651714489999,11.6,1.26842602399998));
#191380=CARTESIAN_POINT('Ctrl Pts',(10.8622942209999,15.2,1.26905967299999));
#191381=CARTESIAN_POINT('Ctrl Pts',(10.8622942209999,11.6,1.26905967299999));
#191382=CARTESIAN_POINT('Ctrl Pts',(10.8594218239999,15.2,1.26968977599998));
#191383=CARTESIAN_POINT('Ctrl Pts',(10.8594218239999,11.6,1.26968977599998));
#191384=CARTESIAN_POINT('Ctrl Pts',(10.8565542679999,15.2,1.27031633899998));
#191385=CARTESIAN_POINT('Ctrl Pts',(10.8565542679999,11.6,1.27031633899998));
#191386=CARTESIAN_POINT('Ctrl Pts',(10.8536915629999,15.2,1.27093936699998));
#191387=CARTESIAN_POINT('Ctrl Pts',(10.8536915629999,11.6,1.27093936699998));
#191388=CARTESIAN_POINT('Ctrl Pts',(10.8508337229999,15.2,1.27155886699999));
#191389=CARTESIAN_POINT('Ctrl Pts',(10.8508337229999,11.6,1.27155886699999));
#191390=CARTESIAN_POINT('Ctrl Pts',(10.8479807569999,15.2,1.27217484299999));
#191391=CARTESIAN_POINT('Ctrl Pts',(10.8479807569999,11.6,1.27217484299999));
#191392=CARTESIAN_POINT('Ctrl Pts',(10.8451326779999,15.2,1.27278730199999));
#191393=CARTESIAN_POINT('Ctrl Pts',(10.8451326779999,11.6,1.27278730199999));
#191394=CARTESIAN_POINT('Ctrl Pts',(10.8422894959999,15.2,1.27339624799998));
#191395=CARTESIAN_POINT('Ctrl Pts',(10.8422894959999,11.6,1.27339624799998));
#191396=CARTESIAN_POINT('Ctrl Pts',(10.8394512219999,15.2,1.27400168799999));
#191397=CARTESIAN_POINT('Ctrl Pts',(10.8394512219999,11.6,1.27400168799999));
#191398=CARTESIAN_POINT('Ctrl Pts',(10.8366178699999,15.2,1.27460362699999));
#191399=CARTESIAN_POINT('Ctrl Pts',(10.8366178699999,11.6,1.27460362699999));
#191400=CARTESIAN_POINT('Ctrl Pts',(10.8337894499999,15.2,1.27520206999999));
#191401=CARTESIAN_POINT('Ctrl Pts',(10.8337894499999,11.6,1.27520206999999));
#191402=CARTESIAN_POINT('Ctrl Pts',(10.8309659719999,15.2,1.27579702399998));
#191403=CARTESIAN_POINT('Ctrl Pts',(10.8309659719999,11.6,1.27579702399998));
#191404=CARTESIAN_POINT('Ctrl Pts',(10.8281474499999,15.2,1.27638849299998));
#191405=CARTESIAN_POINT('Ctrl Pts',(10.8281474499999,11.6,1.27638849299998));
#191406=CARTESIAN_POINT('Ctrl Pts',(10.8253338939999,15.2,1.27697648499999));
#191407=CARTESIAN_POINT('Ctrl Pts',(10.8253338939999,11.6,1.27697648499998));
#191408=CARTESIAN_POINT('Ctrl Pts',(10.8225253159999,15.2,1.27756100399999));
#191409=CARTESIAN_POINT('Ctrl Pts',(10.8225253159999,11.6,1.27756100399999));
#191410=CARTESIAN_POINT('Ctrl Pts',(10.8197217269999,15.2,1.27814205699998));
#191411=CARTESIAN_POINT('Ctrl Pts',(10.8197217269999,11.6,1.27814205699998));
#191412=CARTESIAN_POINT('Ctrl Pts',(10.8169231379999,15.2,1.27871964799999));
#191413=CARTESIAN_POINT('Ctrl Pts',(10.8169231379999,11.6,1.27871964799999));
#191414=CARTESIAN_POINT('Ctrl Pts',(10.8141295629999,15.2,1.27929378499998));
#191415=CARTESIAN_POINT('Ctrl Pts',(10.8141295629999,11.6,1.27929378499998));
#191416=CARTESIAN_POINT('Ctrl Pts',(10.8113410119999,15.2,1.27986447199998));
#191417=CARTESIAN_POINT('Ctrl Pts',(10.8113410119999,11.6,1.27986447199998));
#191418=CARTESIAN_POINT('Ctrl Pts',(10.8085574969999,15.2,1.28043171599999));
#191419=CARTESIAN_POINT('Ctrl Pts',(10.8085574969999,11.6,1.28043171599999));
#191420=CARTESIAN_POINT('Ctrl Pts',(10.8057790279999,15.2,1.28099552199998));
#191421=CARTESIAN_POINT('Ctrl Pts',(10.8057790279999,11.6,1.28099552199998));
#191422=CARTESIAN_POINT('Ctrl Pts',(10.8030056189999,15.2,1.28155589599999));
#191423=CARTESIAN_POINT('Ctrl Pts',(10.8030056189999,11.6,1.28155589599999));
#191424=CARTESIAN_POINT('Ctrl Pts',(10.8002372809999,15.2,1.28211284599999));
#191425=CARTESIAN_POINT('Ctrl Pts',(10.8002372809999,11.6,1.28211284599998));
#191426=CARTESIAN_POINT('Ctrl Pts',(10.7974740259999,15.2,1.28266637499999));
#191427=CARTESIAN_POINT('Ctrl Pts',(10.7974740259999,11.6,1.28266637499999));
#191428=CARTESIAN_POINT('Ctrl Pts',(10.7947158649999,15.2,1.28321648999998));
#191429=CARTESIAN_POINT('Ctrl Pts',(10.7947158649999,11.6,1.28321648999998));
#191430=CARTESIAN_POINT('Ctrl Pts',(10.7919628099999,15.2,1.28376319699999));
#191431=CARTESIAN_POINT('Ctrl Pts',(10.7919628099999,11.6,1.28376319699999));
#191432=CARTESIAN_POINT('Ctrl Pts',(10.7892148729999,15.2,1.28430650299999));
#191433=CARTESIAN_POINT('Ctrl Pts',(10.7892148729999,11.6,1.28430650299999));
#191434=CARTESIAN_POINT('Ctrl Pts',(10.7864720659999,15.2,1.28484641299998));
#191435=CARTESIAN_POINT('Ctrl Pts',(10.7864720659999,11.6,1.28484641299998));
#191436=CARTESIAN_POINT('Ctrl Pts',(10.7837344009999,15.2,1.28538293399998));
#191437=CARTESIAN_POINT('Ctrl Pts',(10.7837344009999,11.6,1.28538293399998));
#191438=CARTESIAN_POINT('Ctrl Pts',(10.7810018879999,15.2,1.28591607099999));
#191439=CARTESIAN_POINT('Ctrl Pts',(10.7810018879999,11.6,1.28591607099999));
#191440=CARTESIAN_POINT('Ctrl Pts',(10.7782745419999,15.2,1.28644583099998));
#191441=CARTESIAN_POINT('Ctrl Pts',(10.7782745419999,11.6,1.28644583099998));
#191442=CARTESIAN_POINT('Ctrl Pts',(10.7755523729999,15.2,1.28697221799999));
#191443=CARTESIAN_POINT('Ctrl Pts',(10.7755523729999,11.6,1.28697221799999));
#191444=CARTESIAN_POINT('Ctrl Pts',(10.7728353919999,15.2,1.28749524099999));
#191445=CARTESIAN_POINT('Ctrl Pts',(10.7728353919999,11.6,1.28749524099998));
#191446=CARTESIAN_POINT('Ctrl Pts',(10.7701236149999,15.2,1.28801490499999));
#191447=CARTESIAN_POINT('Ctrl Pts',(10.7701236149999,11.6,1.28801490499999));
#191448=CARTESIAN_POINT('Ctrl Pts',(10.7674170489999,15.2,1.28853121599999));
#191449=CARTESIAN_POINT('Ctrl Pts',(10.7674170489999,11.6,1.28853121599999));
#191450=CARTESIAN_POINT('Ctrl Pts',(10.7647157089999,15.2,1.28904418099999));
#191451=CARTESIAN_POINT('Ctrl Pts',(10.7647157089999,11.6,1.28904418099998));
#191452=CARTESIAN_POINT('Ctrl Pts',(10.7620196059999,15.2,1.28955380499999));
#191453=CARTESIAN_POINT('Ctrl Pts',(10.7620196059999,11.6,1.28955380499999));
#191454=CARTESIAN_POINT('Ctrl Pts',(10.7593287539999,15.2,1.29006009499999));
#191455=CARTESIAN_POINT('Ctrl Pts',(10.7593287539999,11.6,1.29006009499998));
#191456=CARTESIAN_POINT('Ctrl Pts',(10.7566431619999,15.2,1.29056305799998));
#191457=CARTESIAN_POINT('Ctrl Pts',(10.7566431619999,11.6,1.29056305799998));
#191458=CARTESIAN_POINT('Ctrl Pts',(10.7539628449999,15.2,1.29106269999999));
#191459=CARTESIAN_POINT('Ctrl Pts',(10.7539628449999,11.6,1.29106269999998));
#191460=CARTESIAN_POINT('Ctrl Pts',(10.7512878129999,15.2,1.29155902599999));
#191461=CARTESIAN_POINT('Ctrl Pts',(10.7512878129999,11.6,1.29155902599999));
#191462=CARTESIAN_POINT('Ctrl Pts',(10.7486180789999,15.2,1.29205204399998));
#191463=CARTESIAN_POINT('Ctrl Pts',(10.7486180789999,11.6,1.29205204399998));
#191464=CARTESIAN_POINT('Ctrl Pts',(10.7459536549999,15.2,1.29254175999999));
#191465=CARTESIAN_POINT('Ctrl Pts',(10.7459536549999,11.6,1.29254175999999));
#191466=CARTESIAN_POINT('Ctrl Pts',(10.7432945539999,15.2,1.29302817899998));
#191467=CARTESIAN_POINT('Ctrl Pts',(10.7432945539999,11.6,1.29302817899998));
#191468=CARTESIAN_POINT('Ctrl Pts',(10.7406407879999,15.2,1.29351130999999));
#191469=CARTESIAN_POINT('Ctrl Pts',(10.7406407879999,11.6,1.29351130999999));
#191470=CARTESIAN_POINT('Ctrl Pts',(10.7379923689999,15.2,1.29399115799998));
#191471=CARTESIAN_POINT('Ctrl Pts',(10.7379923689999,11.6,1.29399115799998));
#191472=CARTESIAN_POINT('Ctrl Pts',(10.7353493089999,15.2,1.29446772899998));
#191473=CARTESIAN_POINT('Ctrl Pts',(10.7353493089999,11.6,1.29446772899998));
#191474=CARTESIAN_POINT('Ctrl Pts',(10.7327116219999,15.2,1.29494102999999));
#191475=CARTESIAN_POINT('Ctrl Pts',(10.7327116219999,11.6,1.29494102999998));
#191476=CARTESIAN_POINT('Ctrl Pts',(10.7300793179999,15.2,1.29541106899998));
#191477=CARTESIAN_POINT('Ctrl Pts',(10.7300793179999,11.6,1.29541106899998));
#191478=CARTESIAN_POINT('Ctrl Pts',(10.7274524109999,15.2,1.29587785099998));
#191479=CARTESIAN_POINT('Ctrl Pts',(10.7274524109999,11.6,1.29587785099998));
#191480=CARTESIAN_POINT('Ctrl Pts',(10.7248309119999,15.2,1.29634138299998));
#191481=CARTESIAN_POINT('Ctrl Pts',(10.7248309119999,11.6,1.29634138299998));
#191482=CARTESIAN_POINT('Ctrl Pts',(10.7222148359999,15.2,1.29680166999998));
#191483=CARTESIAN_POINT('Ctrl Pts',(10.7222148359999,11.6,1.29680166999998));
#191484=CARTESIAN_POINT('Ctrl Pts',(10.7196041929999,15.2,1.29725872299999));
#191485=CARTESIAN_POINT('Ctrl Pts',(10.7196041929999,11.6,1.29725872299999));
#191486=CARTESIAN_POINT('Ctrl Pts',(10.7169989959999,15.2,1.29771254499999));
#191487=CARTESIAN_POINT('Ctrl Pts',(10.7169989959999,11.6,1.29771254499999));
#191488=CARTESIAN_POINT('Ctrl Pts',(10.7143992589999,15.2,1.29816314299998));
#191489=CARTESIAN_POINT('Ctrl Pts',(10.7143992589999,11.6,1.29816314299998));
#191490=CARTESIAN_POINT('Ctrl Pts',(10.7118049929999,15.2,1.29861052499999));
#191491=CARTESIAN_POINT('Ctrl Pts',(10.7118049929999,11.6,1.29861052499999));
#191492=CARTESIAN_POINT('Ctrl Pts',(10.7092162099999,15.2,1.29905469699999));
#191493=CARTESIAN_POINT('Ctrl Pts',(10.7092162099999,11.6,1.29905469699999));
#191494=CARTESIAN_POINT('Ctrl Pts',(10.7066329249999,15.2,1.29949566599999));
#191495=CARTESIAN_POINT('Ctrl Pts',(10.7066329249999,11.6,1.29949566599999));
#191496=CARTESIAN_POINT('Ctrl Pts',(10.7040551489999,15.2,1.29993343899999));
#191497=CARTESIAN_POINT('Ctrl Pts',(10.7040551489999,11.6,1.29993343899998));
#191498=CARTESIAN_POINT('Ctrl Pts',(10.7014828959999,15.2,1.30036802199998));
#191499=CARTESIAN_POINT('Ctrl Pts',(10.7014828959999,11.6,1.30036802199998));
#191500=CARTESIAN_POINT('Ctrl Pts',(10.6989161759999,15.2,1.30079942299998));
#191501=CARTESIAN_POINT('Ctrl Pts',(10.6989161759999,11.6,1.30079942299998));
#191502=CARTESIAN_POINT('Ctrl Pts',(10.6963550049999,15.2,1.30122764799999));
#191503=CARTESIAN_POINT('Ctrl Pts',(10.6963550049999,11.6,1.30122764799998));
#191504=CARTESIAN_POINT('Ctrl Pts',(10.6937993929999,15.2,1.30165270599999));
#191505=CARTESIAN_POINT('Ctrl Pts',(10.6937993929999,11.6,1.30165270599999));
#191506=CARTESIAN_POINT('Ctrl Pts',(10.6912493539999,15.2,1.30207460099999));
#191507=CARTESIAN_POINT('Ctrl Pts',(10.6912493539999,11.6,1.30207460099998));
#191508=CARTESIAN_POINT('Ctrl Pts',(10.6887049019999,15.2,1.30249334199998));
#191509=CARTESIAN_POINT('Ctrl Pts',(10.6887049019999,11.6,1.30249334199998));
#191510=CARTESIAN_POINT('Ctrl Pts',(10.6861660479999,15.2,1.30290893499998));
#191511=CARTESIAN_POINT('Ctrl Pts',(10.6861660479999,11.6,1.30290893499998));
#191512=CARTESIAN_POINT('Ctrl Pts',(10.6836328059999,15.2,1.30332138799998));
#191513=CARTESIAN_POINT('Ctrl Pts',(10.6836328059999,11.6,1.30332138799998));
#191514=CARTESIAN_POINT('Ctrl Pts',(10.6811051889999,15.2,1.30373070699998));
#191515=CARTESIAN_POINT('Ctrl Pts',(10.6811051889999,11.6,1.30373070699998));
#191516=CARTESIAN_POINT('Ctrl Pts',(10.6785832079999,15.2,1.30413689899999));
#191517=CARTESIAN_POINT('Ctrl Pts',(10.6785832079999,11.6,1.30413689899999));
#191518=CARTESIAN_POINT('Ctrl Pts',(10.6760668779999,15.2,1.30453997299998));
#191519=CARTESIAN_POINT('Ctrl Pts',(10.6760668779999,11.6,1.30453997299998));
#191520=CARTESIAN_POINT('Ctrl Pts',(10.6735562119999,15.2,1.30493993399998));
#191521=CARTESIAN_POINT('Ctrl Pts',(10.6735562119999,11.6,1.30493993399998));
#191522=CARTESIAN_POINT('Ctrl Pts',(10.6710512209999,15.2,1.30533679099999));
#191523=CARTESIAN_POINT('Ctrl Pts',(10.6710512209999,11.6,1.30533679099999));
#191524=CARTESIAN_POINT('Ctrl Pts',(10.6685519209999,15.2,1.30573054999998));
#191525=CARTESIAN_POINT('Ctrl Pts',(10.6685519209999,11.6,1.30573054999998));
#191526=CARTESIAN_POINT('Ctrl Pts',(10.6660583229999,15.2,1.30612121799999));
#191527=CARTESIAN_POINT('Ctrl Pts',(10.6660583229999,11.6,1.30612121799999));
#191528=CARTESIAN_POINT('Ctrl Pts',(10.6635704409999,15.2,1.30650880399998));
#191529=CARTESIAN_POINT('Ctrl Pts',(10.6635704409999,11.6,1.30650880399998));
#191530=CARTESIAN_POINT('Ctrl Pts',(10.6610882879999,15.2,1.30689331299998));
#191531=CARTESIAN_POINT('Ctrl Pts',(10.6610882879999,11.6,1.30689331299998));
#191532=CARTESIAN_POINT('Ctrl Pts',(10.6586118759999,15.2,1.30727475299999));
#191533=CARTESIAN_POINT('Ctrl Pts',(10.6586118759999,11.6,1.30727475299999));
#191534=CARTESIAN_POINT('Ctrl Pts',(10.6561412199999,15.2,1.30765313299999));
#191535=CARTESIAN_POINT('Ctrl Pts',(10.6561412199999,11.6,1.30765313299999));
#191536=CARTESIAN_POINT('Ctrl Pts',(10.6536763329999,15.2,1.30802845899999));
#191537=CARTESIAN_POINT('Ctrl Pts',(10.6536763329999,11.6,1.30802845899999));
#191538=CARTESIAN_POINT('Ctrl Pts',(10.6512172259999,15.2,1.30840073799999));
#191539=CARTESIAN_POINT('Ctrl Pts',(10.6512172259999,11.6,1.30840073799999));
#191540=CARTESIAN_POINT('Ctrl Pts',(10.6487639159999,15.2,1.30876997899998));
#191541=CARTESIAN_POINT('Ctrl Pts',(10.6487639159999,11.6,1.30876997899998));
#191542=CARTESIAN_POINT('Ctrl Pts',(10.6463164129999,15.2,1.30913618899998));
#191543=CARTESIAN_POINT('Ctrl Pts',(10.6463164129999,11.6,1.30913618899998));
#191544=CARTESIAN_POINT('Ctrl Pts',(10.6438747329999,15.2,1.30949937399999));
#191545=CARTESIAN_POINT('Ctrl Pts',(10.6438747329999,11.6,1.30949937399999));
#191546=CARTESIAN_POINT('Ctrl Pts',(10.6414388879999,15.2,1.30985954199998));
#191547=CARTESIAN_POINT('Ctrl Pts',(10.6414388879999,11.6,1.30985954199998));
#191548=CARTESIAN_POINT('Ctrl Pts',(10.6390088909999,15.2,1.31021670299999));
#191549=CARTESIAN_POINT('Ctrl Pts',(10.6390088909999,11.6,1.31021670299999));
#191550=CARTESIAN_POINT('Ctrl Pts',(10.6365847569999,15.2,1.31057086099998));
#191551=CARTESIAN_POINT('Ctrl Pts',(10.6365847569999,11.6,1.31057086099998));
#191552=CARTESIAN_POINT('Ctrl Pts',(10.6341664979999,15.2,1.31092202699998));
#191553=CARTESIAN_POINT('Ctrl Pts',(10.6341664979999,11.6,1.31092202699998));
#191554=CARTESIAN_POINT('Ctrl Pts',(10.6317541279999,15.2,1.31127020699998));
#191555=CARTESIAN_POINT('Ctrl Pts',(10.6317541279999,11.6,1.31127020699998));
#191556=CARTESIAN_POINT('Ctrl Pts',(10.6293476599999,15.2,1.31161540699999));
#191557=CARTESIAN_POINT('Ctrl Pts',(10.6293476599999,11.6,1.31161540699999));
#191558=CARTESIAN_POINT('Ctrl Pts',(10.6269471099999,15.2,1.31195763899999));
#191559=CARTESIAN_POINT('Ctrl Pts',(10.6269471099999,11.6,1.31195763899999));
#191560=CARTESIAN_POINT('Ctrl Pts',(10.6245524889999,15.2,1.31229690699998));
#191561=CARTESIAN_POINT('Ctrl Pts',(10.6245524889999,11.6,1.31229690699998));
#191562=CARTESIAN_POINT('Ctrl Pts',(10.6221638119999,15.2,1.31263321999999));
#191563=CARTESIAN_POINT('Ctrl Pts',(10.6221638119999,11.6,1.31263321999999));
#191564=CARTESIAN_POINT('Ctrl Pts',(10.6197810909999,15.2,1.31296658599998));
#191565=CARTESIAN_POINT('Ctrl Pts',(10.6197810909999,11.6,1.31296658599998));
#191566=CARTESIAN_POINT('Ctrl Pts',(10.6174043419999,15.2,1.31329701299999));
#191567=CARTESIAN_POINT('Ctrl Pts',(10.6174043419999,11.6,1.31329701299999));
#191568=CARTESIAN_POINT('Ctrl Pts',(10.6150335779999,15.2,1.31362450999998));
#191569=CARTESIAN_POINT('Ctrl Pts',(10.6150335779999,11.6,1.31362450999998));
#191570=CARTESIAN_POINT('Ctrl Pts',(10.6126688119999,15.2,1.31394908099999));
#191571=CARTESIAN_POINT('Ctrl Pts',(10.6126688119999,11.6,1.31394908099998));
#191572=CARTESIAN_POINT('Ctrl Pts',(10.6103100589999,15.2,1.31427073799999));
#191573=CARTESIAN_POINT('Ctrl Pts',(10.6103100589999,11.6,1.31427073799998));
#191574=CARTESIAN_POINT('Ctrl Pts',(10.6079573329999,15.2,1.31458948699999));
#191575=CARTESIAN_POINT('Ctrl Pts',(10.6079573329999,11.6,1.31458948699999));
#191576=CARTESIAN_POINT('Ctrl Pts',(10.6056106459999,15.2,1.31490533699999));
#191577=CARTESIAN_POINT('Ctrl Pts',(10.6056106459999,11.6,1.31490533699999));
#191578=CARTESIAN_POINT('Ctrl Pts',(10.6032700129999,15.2,1.31521829699999));
#191579=CARTESIAN_POINT('Ctrl Pts',(10.6032700129999,11.6,1.31521829699999));
#191580=CARTESIAN_POINT('Ctrl Pts',(10.6009354489999,15.2,1.31552837099999));
#191581=CARTESIAN_POINT('Ctrl Pts',(10.6009354489999,11.6,1.31552837099999));
#191582=CARTESIAN_POINT('Ctrl Pts',(10.5986069669999,15.2,1.31583557099999));
#191583=CARTESIAN_POINT('Ctrl Pts',(10.5986069669999,11.6,1.31583557099999));
#191584=CARTESIAN_POINT('Ctrl Pts',(10.5962845809999,15.2,1.31613990499998));
#191585=CARTESIAN_POINT('Ctrl Pts',(10.5962845809999,11.6,1.31613990499998));
#191586=CARTESIAN_POINT('Ctrl Pts',(10.5939683049999,15.2,1.31644137899999));
#191587=CARTESIAN_POINT('Ctrl Pts',(10.5939683049999,11.6,1.31644137899999));
#191588=CARTESIAN_POINT('Ctrl Pts',(10.5916581539999,15.2,1.31674000199999));
#191589=CARTESIAN_POINT('Ctrl Pts',(10.5916581539999,11.6,1.31674000199998));
#191590=CARTESIAN_POINT('Ctrl Pts',(10.5893541409999,15.2,1.31703578299998));
#191591=CARTESIAN_POINT('Ctrl Pts',(10.5893541409999,11.6,1.31703578299998));
#191592=CARTESIAN_POINT('Ctrl Pts',(10.5870562799999,15.2,1.31732872999998));
#191593=CARTESIAN_POINT('Ctrl Pts',(10.5870562799999,11.6,1.31732872999998));
#191594=CARTESIAN_POINT('Ctrl Pts',(10.5847645859999,15.2,1.31761885099999));
#191595=CARTESIAN_POINT('Ctrl Pts',(10.5847645859999,11.6,1.31761885099999));
#191596=CARTESIAN_POINT('Ctrl Pts',(10.5824790749999,15.2,1.31790615499999));
#191597=CARTESIAN_POINT('Ctrl Pts',(10.5824790749999,11.6,1.31790615499999));
#191598=CARTESIAN_POINT('Ctrl Pts',(10.5801997579999,15.2,1.31819064899998));
#191599=CARTESIAN_POINT('Ctrl Pts',(10.5801997579999,11.6,1.31819064899998));
#191600=CARTESIAN_POINT('Ctrl Pts',(10.5779266509999,15.2,1.31847234299999));
#191601=CARTESIAN_POINT('Ctrl Pts',(10.5779266509999,11.6,1.31847234299999));
#191602=CARTESIAN_POINT('Ctrl Pts',(10.5756597679999,15.2,1.31875124499999));
#191603=CARTESIAN_POINT('Ctrl Pts',(10.5756597679999,11.6,1.31875124499999));
#191604=CARTESIAN_POINT('Ctrl Pts',(10.5733991249999,15.2,1.31902736299998));
#191605=CARTESIAN_POINT('Ctrl Pts',(10.5733991249999,11.6,1.31902736299998));
#191606=CARTESIAN_POINT('Ctrl Pts',(10.5711447329999,15.2,1.31930070599998));
#191607=CARTESIAN_POINT('Ctrl Pts',(10.5711447329999,11.6,1.31930070599998));
#191608=CARTESIAN_POINT('Ctrl Pts',(10.5688966099999,15.2,1.31957128299999));
#191609=CARTESIAN_POINT('Ctrl Pts',(10.5688966099999,11.6,1.31957128299998));
#191610=CARTESIAN_POINT('Ctrl Pts',(10.5666547689999,15.2,1.31983910099999));
#191611=CARTESIAN_POINT('Ctrl Pts',(10.5666547689999,11.6,1.31983910099999));
#191612=CARTESIAN_POINT('Ctrl Pts',(10.5644192249999,15.2,1.32010417099998));
#191613=CARTESIAN_POINT('Ctrl Pts',(10.5644192249999,11.6,1.32010417099998));
#191614=CARTESIAN_POINT('Ctrl Pts',(10.5621899909999,15.2,1.32036649799999));
#191615=CARTESIAN_POINT('Ctrl Pts',(10.5621899909999,11.6,1.32036649799998));
#191616=CARTESIAN_POINT('Ctrl Pts',(10.5599670829999,15.2,1.32062609399998));
#191617=CARTESIAN_POINT('Ctrl Pts',(10.5599670829999,11.6,1.32062609399998));
#191618=CARTESIAN_POINT('Ctrl Pts',(10.5577505169999,15.2,1.32088296799999));
#191619=CARTESIAN_POINT('Ctrl Pts',(10.5577505169999,11.6,1.32088296799999));
#191620=CARTESIAN_POINT('Ctrl Pts',(10.5555403039999,15.2,1.32113712699998));
#191621=CARTESIAN_POINT('Ctrl Pts',(10.5555403039999,11.6,1.32113712699998));
#191622=CARTESIAN_POINT('Ctrl Pts',(10.5533364629999,15.2,1.32138857999998));
#191623=CARTESIAN_POINT('Ctrl Pts',(10.5533364629999,11.6,1.32138857999998));
#191624=CARTESIAN_POINT('Ctrl Pts',(10.5511390059999,15.2,1.32163733699999));
#191625=CARTESIAN_POINT('Ctrl Pts',(10.5511390059999,11.6,1.32163733699999));
#191626=CARTESIAN_POINT('Ctrl Pts',(10.5489479479999,15.2,1.32188340599999));
#191627=CARTESIAN_POINT('Ctrl Pts',(10.5489479479999,11.6,1.32188340599999));
#191628=CARTESIAN_POINT('Ctrl Pts',(10.5467633059999,15.2,1.32212679499998));
#191629=CARTESIAN_POINT('Ctrl Pts',(10.5467633059999,11.6,1.32212679499998));
#191630=CARTESIAN_POINT('Ctrl Pts',(10.5445850929999,15.2,1.32236751399998));
#191631=CARTESIAN_POINT('Ctrl Pts',(10.5445850929999,11.6,1.32236751399998));
#191632=CARTESIAN_POINT('Ctrl Pts',(10.5424133229999,15.2,1.32260557299999));
#191633=CARTESIAN_POINT('Ctrl Pts',(10.5424133229999,11.6,1.32260557299999));
#191634=CARTESIAN_POINT('Ctrl Pts',(10.5402480139999,15.2,1.32284097999999));
#191635=CARTESIAN_POINT('Ctrl Pts',(10.5402480139999,11.6,1.32284097999999));
#191636=CARTESIAN_POINT('Ctrl Pts',(10.5380891789999,15.2,1.32307374399999));
#191637=CARTESIAN_POINT('Ctrl Pts',(10.5380891789999,11.6,1.32307374399998));
#191638=CARTESIAN_POINT('Ctrl Pts',(10.5359368329999,15.2,1.32330387399998));
#191639=CARTESIAN_POINT('Ctrl Pts',(10.5359368329999,11.6,1.32330387399998));
#191640=CARTESIAN_POINT('Ctrl Pts',(10.5337909929999,15.2,1.32353137899999));
#191641=CARTESIAN_POINT('Ctrl Pts',(10.5337909929999,11.6,1.32353137899999));
#191642=CARTESIAN_POINT('Ctrl Pts',(10.5316516719999,15.2,1.32375626999998));
#191643=CARTESIAN_POINT('Ctrl Pts',(10.5316516719999,11.6,1.32375626999998));
#191644=CARTESIAN_POINT('Ctrl Pts',(10.5295188859999,15.2,1.32397855399998));
#191645=CARTESIAN_POINT('Ctrl Pts',(10.5295188859999,11.6,1.32397855399998));
#191646=CARTESIAN_POINT('Ctrl Pts',(10.5273926489999,15.2,1.32419824099999));
#191647=CARTESIAN_POINT('Ctrl Pts',(10.5273926489999,11.6,1.32419824099998));
#191648=CARTESIAN_POINT('Ctrl Pts',(10.5252729789999,15.2,1.32441534099998));
#191649=CARTESIAN_POINT('Ctrl Pts',(10.5252729789999,11.6,1.32441534099998));
#191650=CARTESIAN_POINT('Ctrl Pts',(10.5231598899999,15.2,1.32462986199998));
#191651=CARTESIAN_POINT('Ctrl Pts',(10.5231598899999,11.6,1.32462986199998));
#191652=CARTESIAN_POINT('Ctrl Pts',(10.5210533959999,15.2,1.32484181499999));
#191653=CARTESIAN_POINT('Ctrl Pts',(10.5210533959999,11.6,1.32484181499999));
#191654=CARTESIAN_POINT('Ctrl Pts',(10.5189535149999,15.2,1.32505120799999));
#191655=CARTESIAN_POINT('Ctrl Pts',(10.5189535149999,11.6,1.32505120799998));
#191656=CARTESIAN_POINT('Ctrl Pts',(10.5168602599999,15.2,1.32525805099998));
#191657=CARTESIAN_POINT('Ctrl Pts',(10.5168602599999,11.6,1.32525805099998));
#191658=CARTESIAN_POINT('Ctrl Pts',(10.5147736479999,15.2,1.32546235499999));
#191659=CARTESIAN_POINT('Ctrl Pts',(10.5147736479999,11.6,1.32546235499999));
#191660=CARTESIAN_POINT('Ctrl Pts',(10.5126936939999,15.2,1.32566412699999));
#191661=CARTESIAN_POINT('Ctrl Pts',(10.5126936939999,11.6,1.32566412699999));
#191662=CARTESIAN_POINT('Ctrl Pts',(10.5106204149999,15.2,1.32586337799999));
#191663=CARTESIAN_POINT('Ctrl Pts',(10.5106204149999,11.6,1.32586337799998));
#191664=CARTESIAN_POINT('Ctrl Pts',(10.5085538239999,15.2,1.32606011699998));
#191665=CARTESIAN_POINT('Ctrl Pts',(10.5085538239999,11.6,1.32606011699998));
#191666=CARTESIAN_POINT('Ctrl Pts',(10.5064939389999,15.2,1.32625435499999));
#191667=CARTESIAN_POINT('Ctrl Pts',(10.5064939389999,11.6,1.32625435499999));
#191668=CARTESIAN_POINT('Ctrl Pts',(10.5044407749999,15.2,1.32644610099999));
#191669=CARTESIAN_POINT('Ctrl Pts',(10.5044407749999,11.6,1.32644610099998));
#191670=CARTESIAN_POINT('Ctrl Pts',(10.5023943459999,15.2,1.32663536299999));
#191671=CARTESIAN_POINT('Ctrl Pts',(10.5023943459999,11.6,1.32663536299999));
#191672=CARTESIAN_POINT('Ctrl Pts',(10.5003546709999,15.2,1.32682215399999));
#191673=CARTESIAN_POINT('Ctrl Pts',(10.5003546709999,11.6,1.32682215399999));
#191674=CARTESIAN_POINT('Ctrl Pts',(10.4983217629999,15.2,1.32700648099998));
#191675=CARTESIAN_POINT('Ctrl Pts',(10.4983217629999,11.6,1.32700648099998));
#191676=CARTESIAN_POINT('Ctrl Pts',(10.4962956399999,15.2,1.32718835599999));
#191677=CARTESIAN_POINT('Ctrl Pts',(10.4962956399999,11.6,1.32718835599999));
#191678=CARTESIAN_POINT('Ctrl Pts',(10.4942763159999,15.2,1.32736778799998));
#191679=CARTESIAN_POINT('Ctrl Pts',(10.4942763159999,11.6,1.32736778799998));
#191680=CARTESIAN_POINT('Ctrl Pts',(10.4922638099999,15.2,1.32754478599999));
#191681=CARTESIAN_POINT('Ctrl Pts',(10.4922638099999,11.6,1.32754478599999));
#191682=CARTESIAN_POINT('Ctrl Pts',(10.4902581349999,15.2,1.32771936199998));
#191683=CARTESIAN_POINT('Ctrl Pts',(10.4902581349999,11.6,1.32771936199998));
#191684=CARTESIAN_POINT('Ctrl Pts',(10.4882593079999,15.2,1.32789152599999));
#191685=CARTESIAN_POINT('Ctrl Pts',(10.4882593079999,11.6,1.32789152599999));
#191686=CARTESIAN_POINT('Ctrl Pts',(10.4862673459999,15.2,1.32806128699999));
#191687=CARTESIAN_POINT('Ctrl Pts',(10.4862673459999,11.6,1.32806128699999));
#191688=CARTESIAN_POINT('Ctrl Pts',(10.4842822649999,15.2,1.32822865399998));
#191689=CARTESIAN_POINT('Ctrl Pts',(10.4842822649999,11.6,1.32822865399998));
#191690=CARTESIAN_POINT('Ctrl Pts',(10.4823040789999,15.2,1.32839363899999));
#191691=CARTESIAN_POINT('Ctrl Pts',(10.4823040789999,11.6,1.32839363899999));
#191692=CARTESIAN_POINT('Ctrl Pts',(10.4803328079999,15.2,1.32855625199999));
#191693=CARTESIAN_POINT('Ctrl Pts',(10.4803328079999,11.6,1.32855625199999));
#191694=CARTESIAN_POINT('Ctrl Pts',(10.4783684649999,15.2,1.32871650399998));
#191695=CARTESIAN_POINT('Ctrl Pts',(10.4783684649999,11.6,1.32871650399998));
#191696=CARTESIAN_POINT('Ctrl Pts',(10.4764110689999,15.2,1.32887440299998));
#191697=CARTESIAN_POINT('Ctrl Pts',(10.4764110689999,11.6,1.32887440299998));
#191698=CARTESIAN_POINT('Ctrl Pts',(10.4744606349999,15.2,1.32902996199999));
#191699=CARTESIAN_POINT('Ctrl Pts',(10.4744606349999,11.6,1.32902996199999));
#191700=CARTESIAN_POINT('Ctrl Pts',(10.4725171799999,15.2,1.32918318999999));
#191701=CARTESIAN_POINT('Ctrl Pts',(10.4725171799999,11.6,1.32918318999998));
#191702=CARTESIAN_POINT('Ctrl Pts',(10.4705807189999,15.2,1.32933409699998));
#191703=CARTESIAN_POINT('Ctrl Pts',(10.4705807189999,11.6,1.32933409699998));
#191704=CARTESIAN_POINT('Ctrl Pts',(10.4686512709999,15.2,1.32948269499999));
#191705=CARTESIAN_POINT('Ctrl Pts',(10.4686512709999,11.6,1.32948269499999));
#191706=CARTESIAN_POINT('Ctrl Pts',(10.4667288519999,15.2,1.32962899399999));
#191707=CARTESIAN_POINT('Ctrl Pts',(10.4667288519999,11.6,1.32962899399998));
#191708=CARTESIAN_POINT('Ctrl Pts',(10.4648134769999,15.2,1.32977300399999));
#191709=CARTESIAN_POINT('Ctrl Pts',(10.4648134769999,11.6,1.32977300399999));
#191710=CARTESIAN_POINT('Ctrl Pts',(10.4629051649999,15.2,1.32991473599999));
#191711=CARTESIAN_POINT('Ctrl Pts',(10.4629051649999,11.6,1.32991473599999));
#191712=CARTESIAN_POINT('Ctrl Pts',(10.4610039309999,15.2,1.33005419999999));
#191713=CARTESIAN_POINT('Ctrl Pts',(10.4610039309999,11.6,1.33005419999999));
#191714=CARTESIAN_POINT('Ctrl Pts',(10.4591097919999,15.2,1.33019140799998));
#191715=CARTESIAN_POINT('Ctrl Pts',(10.4591097919999,11.6,1.33019140799998));
#191716=CARTESIAN_POINT('Ctrl Pts',(10.4572227669999,15.2,1.33032637099999));
#191717=CARTESIAN_POINT('Ctrl Pts',(10.4572227669999,11.6,1.33032637099999));
#191718=CARTESIAN_POINT('Ctrl Pts',(10.4553428709999,15.2,1.33045909899999));
#191719=CARTESIAN_POINT('Ctrl Pts',(10.4553428709999,11.6,1.33045909899998));
#191720=CARTESIAN_POINT('Ctrl Pts',(10.4534701199999,15.2,1.33058960299998));
#191721=CARTESIAN_POINT('Ctrl Pts',(10.4534701199999,11.6,1.33058960299998));
#191722=CARTESIAN_POINT('Ctrl Pts',(10.4516045329999,15.2,1.33071789399999));
#191723=CARTESIAN_POINT('Ctrl Pts',(10.4516045329999,11.6,1.33071789399999));
#191724=CARTESIAN_POINT('Ctrl Pts',(10.4497461279999,15.2,1.33084398299999));
#191725=CARTESIAN_POINT('Ctrl Pts',(10.4497461279999,11.6,1.33084398299998));
#191726=CARTESIAN_POINT('Ctrl Pts',(10.4478949189999,15.2,1.33096787999999));
#191727=CARTESIAN_POINT('Ctrl Pts',(10.4478949189999,11.6,1.33096787999999));
#191728=CARTESIAN_POINT('Ctrl Pts',(10.4460509249999,15.2,1.33108959799999));
#191729=CARTESIAN_POINT('Ctrl Pts',(10.4460509249999,11.6,1.33108959799999));
#191730=CARTESIAN_POINT('Ctrl Pts',(10.4442141639999,15.2,1.33120914799999));
#191731=CARTESIAN_POINT('Ctrl Pts',(10.4442141639999,11.6,1.33120914799999));
#191732=CARTESIAN_POINT('Ctrl Pts',(10.4423846519999,15.2,1.33132653899999));
#191733=CARTESIAN_POINT('Ctrl Pts',(10.4423846519999,11.6,1.33132653899999));
#191734=CARTESIAN_POINT('Ctrl Pts',(10.4405624069999,15.2,1.33144178399998));
#191735=CARTESIAN_POINT('Ctrl Pts',(10.4405624069999,11.6,1.33144178399998));
#191736=CARTESIAN_POINT('Ctrl Pts',(10.4387474469999,15.2,1.33155489399998));
#191737=CARTESIAN_POINT('Ctrl Pts',(10.4387474469999,11.6,1.33155489399998));
#191738=CARTESIAN_POINT('Ctrl Pts',(10.4369397879999,15.2,1.33166588099999));
#191739=CARTESIAN_POINT('Ctrl Pts',(10.4369397879999,11.6,1.33166588099999));
#191740=CARTESIAN_POINT('Ctrl Pts',(10.4351394479999,15.2,1.33177475499998));
#191741=CARTESIAN_POINT('Ctrl Pts',(10.4351394479999,11.6,1.33177475499998));
#191742=CARTESIAN_POINT('Ctrl Pts',(10.4333464449999,15.2,1.33188152799999));
#191743=CARTESIAN_POINT('Ctrl Pts',(10.4333464449999,11.6,1.33188152799998));
#191744=CARTESIAN_POINT('Ctrl Pts',(10.4315607969999,15.2,1.33198621299998));
#191745=CARTESIAN_POINT('Ctrl Pts',(10.4315607969999,11.6,1.33198621299998));
#191746=CARTESIAN_POINT('Ctrl Pts',(10.4297825219999,15.2,1.33208881899999));
#191747=CARTESIAN_POINT('Ctrl Pts',(10.4297825219999,11.6,1.33208881899999));
#191748=CARTESIAN_POINT('Ctrl Pts',(10.4280116349999,15.2,1.33218935899999));
#191749=CARTESIAN_POINT('Ctrl Pts',(10.4280116349999,11.6,1.33218935899999));
#191750=CARTESIAN_POINT('Ctrl Pts',(10.4262481579999,15.2,1.33228784499998));
#191751=CARTESIAN_POINT('Ctrl Pts',(10.4262481579999,11.6,1.33228784499998));
#191752=CARTESIAN_POINT('Ctrl Pts',(10.4244921049999,15.2,1.33238428799999));
#191753=CARTESIAN_POINT('Ctrl Pts',(10.4244921049999,11.6,1.33238428799999));
#191754=CARTESIAN_POINT('Ctrl Pts',(10.4227434979999,15.2,1.33247869999999));
#191755=CARTESIAN_POINT('Ctrl Pts',(10.4227434979999,11.6,1.33247869999999));
#191756=CARTESIAN_POINT('Ctrl Pts',(10.4210023509999,15.2,1.33257109199999));
#191757=CARTESIAN_POINT('Ctrl Pts',(10.4210023509999,11.6,1.33257109199999));
#191758=CARTESIAN_POINT('Ctrl Pts',(10.4192686839999,15.2,1.33266147799999));
#191759=CARTESIAN_POINT('Ctrl Pts',(10.4192686839999,11.6,1.33266147799999));
#191760=CARTESIAN_POINT('Ctrl Pts',(10.4175425149999,15.2,1.33274986699998));
#191761=CARTESIAN_POINT('Ctrl Pts',(10.4175425149999,11.6,1.33274986699998));
#191762=CARTESIAN_POINT('Ctrl Pts',(10.4158238619999,15.2,1.33283627399999));
#191763=CARTESIAN_POINT('Ctrl Pts',(10.4158238619999,11.6,1.33283627399999));
#191764=CARTESIAN_POINT('Ctrl Pts',(10.4141127429999,15.2,1.33292070899998));
#191765=CARTESIAN_POINT('Ctrl Pts',(10.4141127429999,11.6,1.33292070899998));
#191766=CARTESIAN_POINT('Ctrl Pts',(10.4124091789999,15.2,1.33300318499999));
#191767=CARTESIAN_POINT('Ctrl Pts',(10.4124091789999,11.6,1.33300318499999));
#191768=CARTESIAN_POINT('Ctrl Pts',(10.4107131829999,15.2,1.33308371299998));
#191769=CARTESIAN_POINT('Ctrl Pts',(10.4107131829999,11.6,1.33308371299998));
#191770=CARTESIAN_POINT('Ctrl Pts',(10.4090247779999,15.2,1.33316230699998));
#191771=CARTESIAN_POINT('Ctrl Pts',(10.4090247779999,11.6,1.33316230699998));
#191772=CARTESIAN_POINT('Ctrl Pts',(10.4073439809999,15.2,1.33323897699999));
#191773=CARTESIAN_POINT('Ctrl Pts',(10.4073439809999,11.6,1.33323897699999));
#191774=CARTESIAN_POINT('Ctrl Pts',(10.4056708099999,15.2,1.33331373699999));
#191775=CARTESIAN_POINT('Ctrl Pts',(10.4056708099999,11.6,1.33331373699999));
#191776=CARTESIAN_POINT('Ctrl Pts',(10.4040052849999,15.2,1.33338659999998));
#191777=CARTESIAN_POINT('Ctrl Pts',(10.4040052849999,11.6,1.33338659999998));
#191778=CARTESIAN_POINT('Ctrl Pts',(10.4023474229999,15.2,1.33345757799999));
#191779=CARTESIAN_POINT('Ctrl Pts',(10.4023474229999,11.6,1.33345757799999));
#191780=CARTESIAN_POINT('Ctrl Pts',(10.4006972429999,15.2,1.33352668099999));
#191781=CARTESIAN_POINT('Ctrl Pts',(10.4006972429999,11.6,1.33352668099999));
#191782=CARTESIAN_POINT('Ctrl Pts',(10.3990547659999,15.2,1.33359392399999));
#191783=CARTESIAN_POINT('Ctrl Pts',(10.3990547659999,11.6,1.33359392399999));
#191784=CARTESIAN_POINT('Ctrl Pts',(10.3974200079999,15.2,1.33365931999998));
#191785=CARTESIAN_POINT('Ctrl Pts',(10.3974200079999,11.6,1.33365931999998));
#191786=CARTESIAN_POINT('Ctrl Pts',(10.3957929889999,15.2,1.33372287999999));
#191787=CARTESIAN_POINT('Ctrl Pts',(10.3957929889999,11.6,1.33372287999999));
#191788=CARTESIAN_POINT('Ctrl Pts',(10.3941737289999,15.2,1.33378461799999));
#191789=CARTESIAN_POINT('Ctrl Pts',(10.3941737289999,11.6,1.33378461799999));
#191790=CARTESIAN_POINT('Ctrl Pts',(10.3925622469999,15.2,1.33384454499998));
#191791=CARTESIAN_POINT('Ctrl Pts',(10.3925622469999,11.6,1.33384454499998));
#191792=CARTESIAN_POINT('Ctrl Pts',(10.3909585599999,15.2,1.33390267699999));
#191793=CARTESIAN_POINT('Ctrl Pts',(10.3909585599999,11.6,1.33390267699998));
#191794=CARTESIAN_POINT('Ctrl Pts',(10.3893626899999,15.2,1.33395902399998));
#191795=CARTESIAN_POINT('Ctrl Pts',(10.3893626899999,11.6,1.33395902399998));
#191796=CARTESIAN_POINT('Ctrl Pts',(10.3877746539999,15.2,1.33401360099999));
#191797=CARTESIAN_POINT('Ctrl Pts',(10.3877746539999,11.6,1.33401360099999));
#191798=CARTESIAN_POINT('Ctrl Pts',(10.3861944729999,15.2,1.33406641899999));
#191799=CARTESIAN_POINT('Ctrl Pts',(10.3861944729999,11.6,1.33406641899999));
#191800=CARTESIAN_POINT('Ctrl Pts',(10.3846221649999,15.2,1.33411749199999));
#191801=CARTESIAN_POINT('Ctrl Pts',(10.3846221649999,11.6,1.33411749199999));
#191802=CARTESIAN_POINT('Ctrl Pts',(10.3830577499999,15.2,1.33416683399998));
#191803=CARTESIAN_POINT('Ctrl Pts',(10.3830577499999,11.6,1.33416683399998));
#191804=CARTESIAN_POINT('Ctrl Pts',(10.3815012489999,15.2,1.33421445799998));
#191805=CARTESIAN_POINT('Ctrl Pts',(10.3815012489999,11.6,1.33421445799998));
#191806=CARTESIAN_POINT('Ctrl Pts',(10.3799526789999,15.2,1.33426037599999));
#191807=CARTESIAN_POINT('Ctrl Pts',(10.3799526789999,11.6,1.33426037599999));
#191808=CARTESIAN_POINT('Ctrl Pts',(10.3784120619999,15.2,1.33430460199999));
#191809=CARTESIAN_POINT('Ctrl Pts',(10.3784120619999,11.6,1.33430460199999));
#191810=CARTESIAN_POINT('Ctrl Pts',(10.3768794159999,15.2,1.33434714999999));
#191811=CARTESIAN_POINT('Ctrl Pts',(10.3768794159999,11.6,1.33434714999999));
#191812=CARTESIAN_POINT('Ctrl Pts',(10.3753547629999,15.2,1.33438803399998));
#191813=CARTESIAN_POINT('Ctrl Pts',(10.3753547629999,11.6,1.33438803399998));
#191814=CARTESIAN_POINT('Ctrl Pts',(10.3738381209999,15.2,1.33442726599998));
#191815=CARTESIAN_POINT('Ctrl Pts',(10.3738381209999,11.6,1.33442726599998));
#191816=CARTESIAN_POINT('Ctrl Pts',(10.3723295099999,15.2,1.33446485899999));
#191817=CARTESIAN_POINT('Ctrl Pts',(10.3723295099999,11.6,1.33446485899999));
#191818=CARTESIAN_POINT('Ctrl Pts',(10.3708289509999,15.2,1.33450082899999));
#191819=CARTESIAN_POINT('Ctrl Pts',(10.3708289509999,11.6,1.33450082899999));
#191820=CARTESIAN_POINT('Ctrl Pts',(10.3693364639999,15.2,1.33453518899998));
#191821=CARTESIAN_POINT('Ctrl Pts',(10.3693364639999,11.6,1.33453518899998));
#191822=CARTESIAN_POINT('Ctrl Pts',(10.3678520689999,15.2,1.33456795199999));
#191823=CARTESIAN_POINT('Ctrl Pts',(10.3678520689999,11.6,1.33456795199998));
#191824=CARTESIAN_POINT('Ctrl Pts',(10.3663757859999,15.2,1.33459913299999));
#191825=CARTESIAN_POINT('Ctrl Pts',(10.3663757859999,11.6,1.33459913299998));
#191826=CARTESIAN_POINT('Ctrl Pts',(10.3649076359999,15.2,1.33462874399998));
#191827=CARTESIAN_POINT('Ctrl Pts',(10.3649076359999,11.6,1.33462874399998));
#191828=CARTESIAN_POINT('Ctrl Pts',(10.3634476389999,15.2,1.33465680099999));
#191829=CARTESIAN_POINT('Ctrl Pts',(10.3634476389999,11.6,1.33465680099999));
#191830=CARTESIAN_POINT('Ctrl Pts',(10.3619958159999,15.2,1.33468331699999));
#191831=CARTESIAN_POINT('Ctrl Pts',(10.3619958159999,11.6,1.33468331699999));
#191832=CARTESIAN_POINT('Ctrl Pts',(10.3605521859999,15.2,1.33470830799999));
#191833=CARTESIAN_POINT('Ctrl Pts',(10.3605521859999,11.6,1.33470830799999));
#191834=CARTESIAN_POINT('Ctrl Pts',(10.3591167719999,15.2,1.33473178499999));
#191835=CARTESIAN_POINT('Ctrl Pts',(10.3591167719999,11.6,1.33473178499999));
#191836=CARTESIAN_POINT('Ctrl Pts',(10.3576895929999,15.2,1.33475376599999));
#191837=CARTESIAN_POINT('Ctrl Pts',(10.3576895929999,11.6,1.33475376599998));
#191838=CARTESIAN_POINT('Ctrl Pts',(10.3562706699999,15.2,1.33477426199998));
#191839=CARTESIAN_POINT('Ctrl Pts',(10.3562706699999,11.6,1.33477426199998));
#191840=CARTESIAN_POINT('Ctrl Pts',(10.3548600249999,15.2,1.33479328899998));
#191841=CARTESIAN_POINT('Ctrl Pts',(10.3548600249999,11.6,1.33479328899998));
#191842=CARTESIAN_POINT('Ctrl Pts',(10.3534576789999,15.2,1.33481086299998));
#191843=CARTESIAN_POINT('Ctrl Pts',(10.3534576789999,11.6,1.33481086299998));
#191844=CARTESIAN_POINT('Ctrl Pts',(10.3520636509999,15.2,1.33482699499998));
#191845=CARTESIAN_POINT('Ctrl Pts',(10.3520636509999,11.6,1.33482699499998));
#191846=CARTESIAN_POINT('Ctrl Pts',(10.3506779649999,15.2,1.33484170199999));
#191847=CARTESIAN_POINT('Ctrl Pts',(10.3506779649999,11.6,1.33484170199999));
#191848=CARTESIAN_POINT('Ctrl Pts',(10.3493006389999,15.2,1.33485499899999));
#191849=CARTESIAN_POINT('Ctrl Pts',(10.3493006389999,11.6,1.33485499899999));
#191850=CARTESIAN_POINT('Ctrl Pts',(10.3479316969999,15.2,1.33486689999998));
#191851=CARTESIAN_POINT('Ctrl Pts',(10.3479316969999,11.6,1.33486689999998));
#191852=CARTESIAN_POINT('Ctrl Pts',(10.3465711599999,15.2,1.33487741899998));
#191853=CARTESIAN_POINT('Ctrl Pts',(10.3465711599999,11.6,1.33487741899998));
#191854=CARTESIAN_POINT('Ctrl Pts',(10.3452190479999,15.2,1.33488657399999));
#191855=CARTESIAN_POINT('Ctrl Pts',(10.3452190479999,11.6,1.33488657399999));
#191856=CARTESIAN_POINT('Ctrl Pts',(10.3438753839999,15.2,1.33489437599998));
#191857=CARTESIAN_POINT('Ctrl Pts',(10.3438753839999,11.6,1.33489437599998));
#191858=CARTESIAN_POINT('Ctrl Pts',(10.3425401889999,15.2,1.33490084399998));
#191859=CARTESIAN_POINT('Ctrl Pts',(10.3425401889999,11.6,1.33490084399998));
#191860=CARTESIAN_POINT('Ctrl Pts',(10.3412134849999,15.2,1.33490598999999));
#191861=CARTESIAN_POINT('Ctrl Pts',(10.3412134849999,11.6,1.33490598999999));
#191862=CARTESIAN_POINT('Ctrl Pts',(10.3398952939999,15.2,1.33490982999998));
#191863=CARTESIAN_POINT('Ctrl Pts',(10.3398952939999,11.6,1.33490982999998));
#191864=CARTESIAN_POINT('Ctrl Pts',(10.3385856379999,15.2,1.33491238099999));
#191865=CARTESIAN_POINT('Ctrl Pts',(10.3385856379999,11.6,1.33491238099999));
#191866=CARTESIAN_POINT('Ctrl Pts',(10.3372845369999,15.2,1.33491365699999));
#191867=CARTESIAN_POINT('Ctrl Pts',(10.3372845369999,11.6,1.33491365699998));
#191868=CARTESIAN_POINT('Ctrl Pts',(10.3359920159999,15.2,1.33491367299999));
#191869=CARTESIAN_POINT('Ctrl Pts',(10.3359920159999,11.6,1.33491367299999));
#191870=CARTESIAN_POINT('Ctrl Pts',(10.3347080959999,15.2,1.33491244599998));
#191871=CARTESIAN_POINT('Ctrl Pts',(10.3347080959999,11.6,1.33491244599998));
#191872=CARTESIAN_POINT('Ctrl Pts',(10.3334327989999,15.2,1.33490999099998));
#191873=CARTESIAN_POINT('Ctrl Pts',(10.3334327989999,11.6,1.33490999099998));
#191874=CARTESIAN_POINT('Ctrl Pts',(10.3321661469999,15.2,1.33490632399999));
#191875=CARTESIAN_POINT('Ctrl Pts',(10.3321661469999,11.6,1.33490632399999));
#191876=CARTESIAN_POINT('Ctrl Pts',(10.3309081639999,15.2,1.33490145999998));
#191877=CARTESIAN_POINT('Ctrl Pts',(10.3309081639999,11.6,1.33490145999998));
#191878=CARTESIAN_POINT('Ctrl Pts',(10.3296588699999,15.2,1.33489541599999));
#191879=CARTESIAN_POINT('Ctrl Pts',(10.3296588699999,11.6,1.33489541599999));
#191880=CARTESIAN_POINT('Ctrl Pts',(10.3284182899999,15.2,1.33488820699998));
#191881=CARTESIAN_POINT('Ctrl Pts',(10.3284182899999,11.6,1.33488820699998));
#191882=CARTESIAN_POINT('Ctrl Pts',(10.3271864459999,15.2,1.33487984899999));
#191883=CARTESIAN_POINT('Ctrl Pts',(10.3271864459999,11.6,1.33487984899999));
#191884=CARTESIAN_POINT('Ctrl Pts',(10.3259633609999,15.2,1.33487035899998));
#191885=CARTESIAN_POINT('Ctrl Pts',(10.3259633609999,11.6,1.33487035899998));
#191886=CARTESIAN_POINT('Ctrl Pts',(10.3247490569999,15.2,1.33485975299998));
#191887=CARTESIAN_POINT('Ctrl Pts',(10.3247490569999,11.6,1.33485975299998));
#191888=CARTESIAN_POINT('Ctrl Pts',(10.3235435579999,15.2,1.33484804699998));
#191889=CARTESIAN_POINT('Ctrl Pts',(10.3235435579999,11.6,1.33484804699998));
#191890=CARTESIAN_POINT('Ctrl Pts',(10.3223468859999,15.2,1.33483525699999));
#191891=CARTESIAN_POINT('Ctrl Pts',(10.3223468859999,11.6,1.33483525699999));
#191892=CARTESIAN_POINT('Ctrl Pts',(10.3211590649999,15.2,1.33482139999999));
